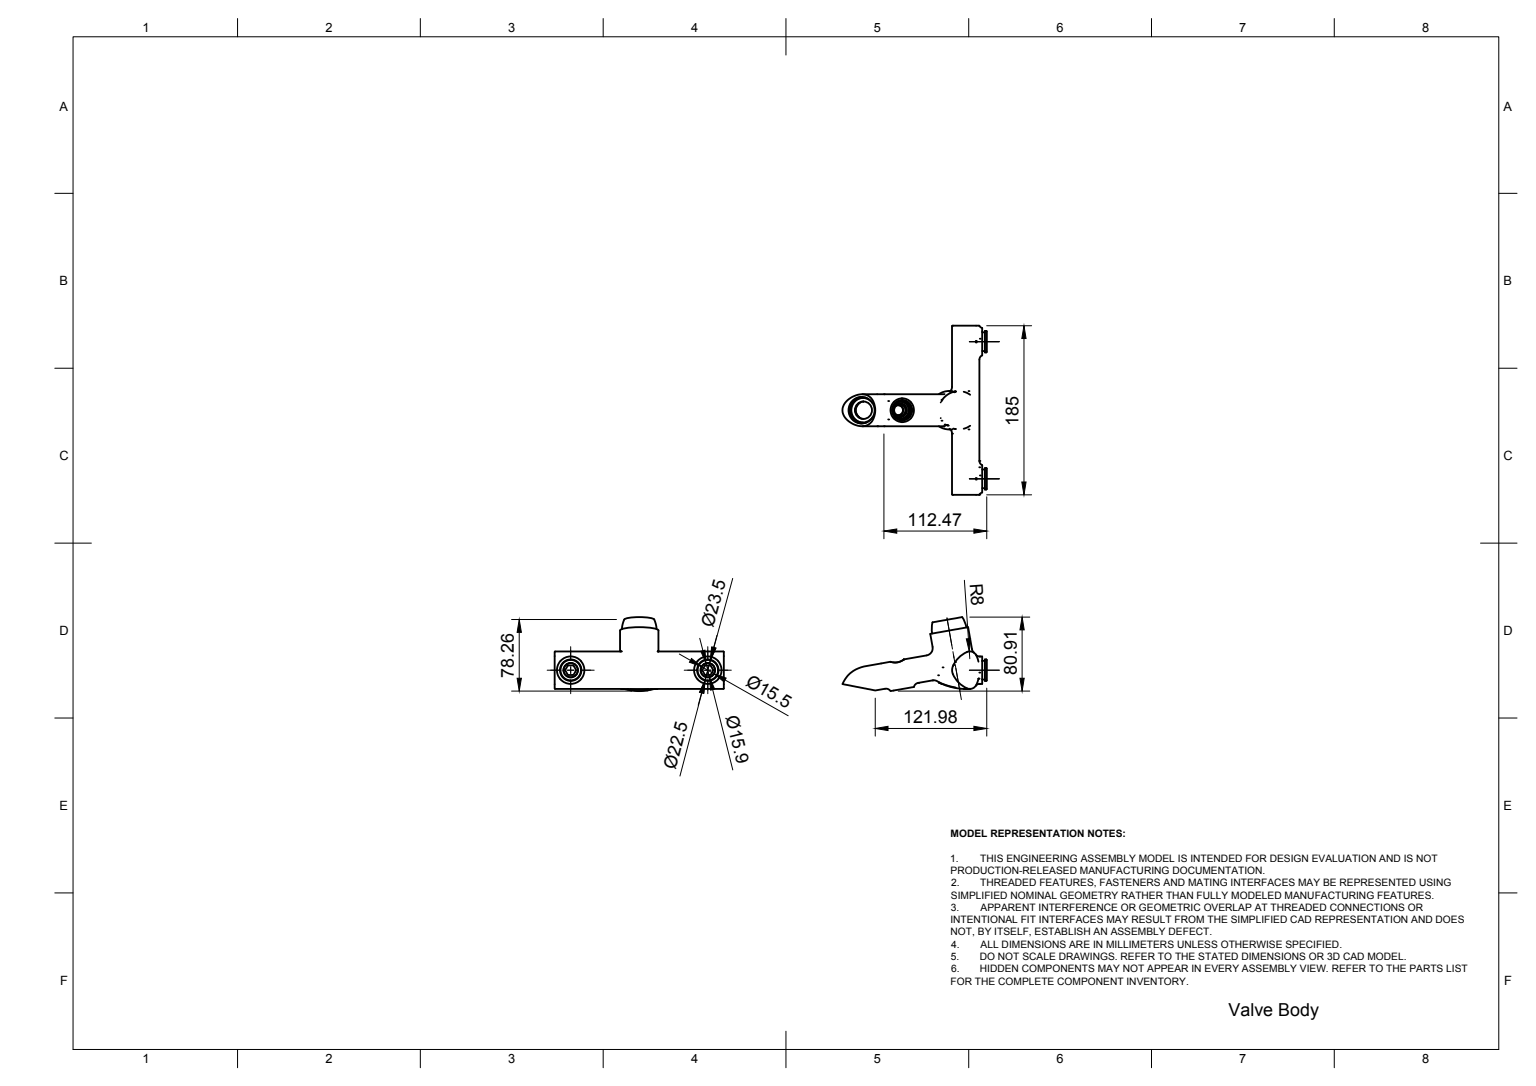
ISO-10303-21;
HEADER;
/* Generated by software containing ST-Developer
 * from STEP Tools, Inc. (www.steptools.com) 
 */

FILE_DESCRIPTION(
/* description */ ('STEP AP214'),
/* implementation_level */ '2;1');

FILE_NAME(
/* name */ 'Valve Body.step',
/* time_stamp */ '2026-10-05T23:18:41-07:00',
/* author */ (''),
/* organization */ (''),
/* preprocessor_version */ 'ST-DEVELOPER v20.2',
/* originating_system */ 'Autodesk Translation Framework v15.15.0.0',
/* authorisation */ '');

FILE_SCHEMA (('AUTOMOTIVE_DESIGN { 1 0 10303 214 3 1 1 }'));
ENDSEC;

DATA;
#10=MECHANICAL_DESIGN_GEOMETRIC_PRESENTATION_REPRESENTATION('',(#100),#221662);
#74=SHAPE_REPRESENTATION_RELATIONSHIP('SRR','None',#221709,#87);
#87=ADVANCED_BREP_SHAPE_REPRESENTATION('',(#79336),#221649);
#100=STYLED_ITEM('',(#221783),#79336);
#113=B_SPLINE_SURFACE_WITH_KNOTS('',3,3,((#122040,#122041,#122042,#122043,
#122044,#122045,#122046,#122047,#122048,#122049,#122050),(#122051,#122052,
#122053,#122054,#122055,#122056,#122057,#122058,#122059,#122060,#122061),
(#122062,#122063,#122064,#122065,#122066,#122067,#122068,#122069,#122070,
#122071,#122072),(#122073,#122074,#122075,#122076,#122077,#122078,#122079,
#122080,#122081,#122082,#122083)),.UNSPECIFIED.,.F.,.F.,.F.,(4,4),(4,1,
1,1,1,1,1,1,4),(0.,1.),(0.,0.125,0.249999999999986,0.374999999999913,0.499999999999809,
0.625000000000008,0.749999999999904,0.8749999999998,1.),.UNSPECIFIED.);
#114=B_SPLINE_SURFACE_WITH_KNOTS('',3,3,((#122246,#122247,#122248,#122249,
#122250,#122251,#122252,#122253,#122254,#122255,#122256),(#122257,#122258,
#122259,#122260,#122261,#122262,#122263,#122264,#122265,#122266,#122267),
(#122268,#122269,#122270,#122271,#122272,#122273,#122274,#122275,#122276,
#122277,#122278),(#122279,#122280,#122281,#122282,#122283,#122284,#122285,
#122286,#122287,#122288,#122289),(#122290,#122291,#122292,#122293,#122294,
#122295,#122296,#122297,#122298,#122299,#122300),(#122301,#122302,#122303,
#122304,#122305,#122306,#122307,#122308,#122309,#122310,#122311),(#122312,
#122313,#122314,#122315,#122316,#122317,#122318,#122319,#122320,#122321,
#122322),(#122323,#122324,#122325,#122326,#122327,#122328,#122329,#122330,
#122331,#122332,#122333),(#122334,#122335,#122336,#122337,#122338,#122339,
#122340,#122341,#122342,#122343,#122344),(#122345,#122346,#122347,#122348,
#122349,#122350,#122351,#122352,#122353,#122354,#122355)),.UNSPECIFIED.,
 .F.,.F.,.F.,(4,3,3,4),(4,1,1,1,1,1,1,1,4),(-0.01,0.,0.978175299313866,
1.),(0.,0.125000000000015,0.25000000000002,0.374999999999975,0.500000000000081,
0.625000000000188,0.750000000000041,0.875000000000148,1.),.UNSPECIFIED.);
#115=B_SPLINE_SURFACE_WITH_KNOTS('',3,3,((#122432,#122433,#122434,#122435,
#122436,#122437,#122438,#122439,#122440,#122441,#122442,#122443,#122444,
#122445,#122446,#122447,#122448,#122449,#122450),(#122451,#122452,#122453,
#122454,#122455,#122456,#122457,#122458,#122459,#122460,#122461,#122462,
#122463,#122464,#122465,#122466,#122467,#122468,#122469),(#122470,#122471,
#122472,#122473,#122474,#122475,#122476,#122477,#122478,#122479,#122480,
#122481,#122482,#122483,#122484,#122485,#122486,#122487,#122488),(#122489,
#122490,#122491,#122492,#122493,#122494,#122495,#122496,#122497,#122498,
#122499,#122500,#122501,#122502,#122503,#122504,#122505,#122506,#122507)),
 .UNSPECIFIED.,.F.,.F.,.F.,(4,4),(4,1,1,1,1,1,1,1,1,1,1,1,1,1,1,1,4),(0.,
1.),(0.,0.0625000000000019,0.12499999999999,0.187499999999977,0.249999999999904,
0.312500000000014,0.37499999999992,0.43750000000003,0.499999999999936,0.562500000000046,
0.624999999999952,0.687499999999859,0.749999999999968,0.812499999999875,
0.874999999999984,0.937499999999891,1.),.UNSPECIFIED.);
#116=B_SPLINE_SURFACE_WITH_KNOTS('',3,3,((#122509,#122510,#122511,#122512,
#122513,#122514,#122515,#122516,#122517,#122518,#122519,#122520,#122521,
#122522,#122523,#122524,#122525,#122526,#122527,#122528,#122529,#122530,
#122531,#122532,#122533,#122534,#122535,#122536,#122537,#122538,#122539,
#122540,#122541,#122542,#122543),(#122544,#122545,#122546,#122547,#122548,
#122549,#122550,#122551,#122552,#122553,#122554,#122555,#122556,#122557,
#122558,#122559,#122560,#122561,#122562,#122563,#122564,#122565,#122566,
#122567,#122568,#122569,#122570,#122571,#122572,#122573,#122574,#122575,
#122576,#122577,#122578),(#122579,#122580,#122581,#122582,#122583,#122584,
#122585,#122586,#122587,#122588,#122589,#122590,#122591,#122592,#122593,
#122594,#122595,#122596,#122597,#122598,#122599,#122600,#122601,#122602,
#122603,#122604,#122605,#122606,#122607,#122608,#122609,#122610,#122611,
#122612,#122613),(#122614,#122615,#122616,#122617,#122618,#122619,#122620,
#122621,#122622,#122623,#122624,#122625,#122626,#122627,#122628,#122629,
#122630,#122631,#122632,#122633,#122634,#122635,#122636,#122637,#122638,
#122639,#122640,#122641,#122642,#122643,#122644,#122645,#122646,#122647,
#122648)),.UNSPECIFIED.,.F.,.F.,.F.,(4,4),(4,1,1,1,1,1,1,1,1,1,1,1,1,1,
1,1,1,1,1,1,1,1,1,1,1,1,1,1,1,1,1,1,4),(0.,1.),(0.,0.031249999999986,0.0625000000000033,
0.0937499999999268,0.124999999999954,0.156249999999982,0.187499999999906,
0.218749999999933,0.249999999999961,0.281249999999885,0.312499999999912,
0.343749999999836,0.374999999999863,0.406249999999891,0.437499999999815,
0.468749999999842,0.49999999999987,0.531249999999794,0.562499999999821,
0.593749999999849,0.624999999999772,0.6562499999998,0.687499999999724,0.718749999999751,
0.749999999999779,0.781249999999703,0.81249999999973,0.843749999999758,
0.874999999999681,0.906249999999709,0.937499999999633,0.96874999999966,
1.),.UNSPECIFIED.);
#117=B_SPLINE_SURFACE_WITH_KNOTS('',3,3,((#122930,#122931,#122932,#122933,
#122934,#122935,#122936,#122937,#122938,#122939,#122940,#122941,#122942,
#122943,#122944,#122945,#122946,#122947,#122948,#122949,#122950,#122951,
#122952,#122953,#122954,#122955,#122956,#122957,#122958,#122959,#122960,
#122961,#122962,#122963,#122964),(#122965,#122966,#122967,#122968,#122969,
#122970,#122971,#122972,#122973,#122974,#122975,#122976,#122977,#122978,
#122979,#122980,#122981,#122982,#122983,#122984,#122985,#122986,#122987,
#122988,#122989,#122990,#122991,#122992,#122993,#122994,#122995,#122996,
#122997,#122998,#122999),(#123000,#123001,#123002,#123003,#123004,#123005,
#123006,#123007,#123008,#123009,#123010,#123011,#123012,#123013,#123014,
#123015,#123016,#123017,#123018,#123019,#123020,#123021,#123022,#123023,
#123024,#123025,#123026,#123027,#123028,#123029,#123030,#123031,#123032,
#123033,#123034),(#123035,#123036,#123037,#123038,#123039,#123040,#123041,
#123042,#123043,#123044,#123045,#123046,#123047,#123048,#123049,#123050,
#123051,#123052,#123053,#123054,#123055,#123056,#123057,#123058,#123059,
#123060,#123061,#123062,#123063,#123064,#123065,#123066,#123067,#123068,
#123069)),.UNSPECIFIED.,.F.,.F.,.F.,(4,4),(4,1,1,1,1,1,1,1,1,1,1,1,1,1,
1,1,1,1,1,1,1,1,1,1,1,1,1,1,1,1,1,1,4),(0.,1.),(0.,0.0312499999999875,0.0624999999999539,
0.0937500000000046,0.12499999999995,0.15625,0.187499999999946,0.218749999999891,
0.249999999999942,0.281249999999887,0.312499999999938,0.343749999999883,
0.374999999999934,0.40624999999988,0.43749999999993,0.468749999999876,0.499999999999821,
0.531249999999872,0.562499999999817,0.593749999999868,0.624999999999813,
0.656249999999864,0.687499999999809,0.71874999999986,0.749999999999805,
0.781249999999751,0.812499999999801,0.843749999999747,0.874999999999797,
0.906249999999743,0.937499999999793,0.968749999999739,1.),.UNSPECIFIED.);
#118=B_SPLINE_SURFACE_WITH_KNOTS('',3,3,((#123453,#123454,#123455,#123456,
#123457,#123458,#123459,#123460,#123461,#123462,#123463,#123464,#123465,
#123466,#123467,#123468,#123469,#123470,#123471,#123472,#123473,#123474,
#123475,#123476,#123477,#123478,#123479,#123480,#123481,#123482,#123483,
#123484,#123485),(#123486,#123487,#123488,#123489,#123490,#123491,#123492,
#123493,#123494,#123495,#123496,#123497,#123498,#123499,#123500,#123501,
#123502,#123503,#123504,#123505,#123506,#123507,#123508,#123509,#123510,
#123511,#123512,#123513,#123514,#123515,#123516,#123517,#123518),(#123519,
#123520,#123521,#123522,#123523,#123524,#123525,#123526,#123527,#123528,
#123529,#123530,#123531,#123532,#123533,#123534,#123535,#123536,#123537,
#123538,#123539,#123540,#123541,#123542,#123543,#123544,#123545,#123546,
#123547,#123548,#123549,#123550,#123551),(#123552,#123553,#123554,#123555,
#123556,#123557,#123558,#123559,#123560,#123561,#123562,#123563,#123564,
#123565,#123566,#123567,#123568,#123569,#123570,#123571,#123572,#123573,
#123574,#123575,#123576,#123577,#123578,#123579,#123580,#123581,#123582,
#123583,#123584)),.UNSPECIFIED.,.F.,.F.,.F.,(4,4),(4,1,1,1,1,1,1,1,1,1,
1,1,1,1,1,1,1,1,1,1,1,1,1,1,1,1,1,1,1,1,4),(0.,1.),(0.,0.0624999999999647,
0.0937499999999471,0.125000000000042,0.156250000000025,0.187500000000007,
0.218749999999989,0.249999999999972,0.281249999999954,0.312499999999937,
0.343750000000032,0.375000000000014,0.40625,0.437499999999979,0.468749999999961,
0.499999999999944,0.531250000000039,0.562500000000021,0.59375,0.624999999999986,
0.656249999999968,0.687499999999951,0.718749999999933,0.750000000000028,
0.781250000000011,0.8125,0.843749999999975,0.874999999999958,0.90624999999994,
0.937499999999923,1.),.UNSPECIFIED.);
#119=B_SPLINE_SURFACE_WITH_KNOTS('',3,3,((#128648,#128649,#128650,#128651,
#128652,#128653,#128654,#128655,#128656,#128657,#128658),(#128659,#128660,
#128661,#128662,#128663,#128664,#128665,#128666,#128667,#128668,#128669),
(#128670,#128671,#128672,#128673,#128674,#128675,#128676,#128677,#128678,
#128679,#128680),(#128681,#128682,#128683,#128684,#128685,#128686,#128687,
#128688,#128689,#128690,#128691)),.UNSPECIFIED.,.F.,.F.,.F.,(4,4),(4,1,
1,1,1,1,1,1,4),(0.,1.),(0.,0.125,0.249999999999986,0.374999999999913,0.499999999999809,
0.625000000000008,0.749999999999904,0.8749999999998,1.),.UNSPECIFIED.);
#120=B_SPLINE_SURFACE_WITH_KNOTS('',3,3,((#128722,#128723,#128724,#128725,
#128726,#128727,#128728,#128729,#128730,#128731,#128732,#128733,#128734,
#128735,#128736,#128737,#128738,#128739,#128740),(#128741,#128742,#128743,
#128744,#128745,#128746,#128747,#128748,#128749,#128750,#128751,#128752,
#128753,#128754,#128755,#128756,#128757,#128758,#128759),(#128760,#128761,
#128762,#128763,#128764,#128765,#128766,#128767,#128768,#128769,#128770,
#128771,#128772,#128773,#128774,#128775,#128776,#128777,#128778),(#128779,
#128780,#128781,#128782,#128783,#128784,#128785,#128786,#128787,#128788,
#128789,#128790,#128791,#128792,#128793,#128794,#128795,#128796,#128797)),
 .UNSPECIFIED.,.F.,.F.,.F.,(4,4),(4,1,1,1,1,1,1,1,1,1,1,1,1,1,1,1,4),(0.,
1.),(0.,0.0625000000000019,0.12499999999999,0.187499999999977,0.249999999999904,
0.312500000000014,0.37499999999992,0.43750000000003,0.499999999999936,0.562500000000046,
0.624999999999952,0.687499999999859,0.749999999999968,0.812499999999875,
0.874999999999984,0.937499999999891,1.),.UNSPECIFIED.);
#121=B_SPLINE_SURFACE_WITH_KNOTS('',3,3,((#128874,#128875,#128876,#128877,
#128878,#128879,#128880,#128881,#128882,#128883,#128884),(#128885,#128886,
#128887,#128888,#128889,#128890,#128891,#128892,#128893,#128894,#128895),
(#128896,#128897,#128898,#128899,#128900,#128901,#128902,#128903,#128904,
#128905,#128906),(#128907,#128908,#128909,#128910,#128911,#128912,#128913,
#128914,#128915,#128916,#128917),(#128918,#128919,#128920,#128921,#128922,
#128923,#128924,#128925,#128926,#128927,#128928),(#128929,#128930,#128931,
#128932,#128933,#128934,#128935,#128936,#128937,#128938,#128939),(#128940,
#128941,#128942,#128943,#128944,#128945,#128946,#128947,#128948,#128949,
#128950)),.UNSPECIFIED.,.F.,.F.,.F.,(4,3,4),(4,1,1,1,1,1,1,1,4),(0.,0.978284469703565,
1.),(0.,0.125000000000015,0.25000000000002,0.374999999999975,0.500000000000081,
0.625000000000188,0.750000000000041,0.875000000000148,1.),.UNSPECIFIED.);
#122=B_SPLINE_SURFACE_WITH_KNOTS('',3,3,((#128952,#128953,#128954,#128955,
#128956,#128957,#128958,#128959,#128960,#128961,#128962,#128963,#128964,
#128965,#128966,#128967,#128968,#128969,#128970,#128971,#128972,#128973,
#128974,#128975,#128976,#128977,#128978,#128979,#128980,#128981,#128982,
#128983,#128984,#128985,#128986),(#128987,#128988,#128989,#128990,#128991,
#128992,#128993,#128994,#128995,#128996,#128997,#128998,#128999,#129000,
#129001,#129002,#129003,#129004,#129005,#129006,#129007,#129008,#129009,
#129010,#129011,#129012,#129013,#129014,#129015,#129016,#129017,#129018,
#129019,#129020,#129021),(#129022,#129023,#129024,#129025,#129026,#129027,
#129028,#129029,#129030,#129031,#129032,#129033,#129034,#129035,#129036,
#129037,#129038,#129039,#129040,#129041,#129042,#129043,#129044,#129045,
#129046,#129047,#129048,#129049,#129050,#129051,#129052,#129053,#129054,
#129055,#129056),(#129057,#129058,#129059,#129060,#129061,#129062,#129063,
#129064,#129065,#129066,#129067,#129068,#129069,#129070,#129071,#129072,
#129073,#129074,#129075,#129076,#129077,#129078,#129079,#129080,#129081,
#129082,#129083,#129084,#129085,#129086,#129087,#129088,#129089,#129090,
#129091)),.UNSPECIFIED.,.F.,.F.,.F.,(4,4),(4,1,1,1,1,1,1,1,1,1,1,1,1,1,
1,1,1,1,1,1,1,1,1,1,1,1,1,1,1,1,1,1,4),(0.,1.),(0.,0.031249999999986,0.0625000000000033,
0.0937499999999268,0.124999999999954,0.156249999999982,0.187499999999906,
0.218749999999933,0.249999999999961,0.281249999999885,0.312499999999912,
0.343749999999836,0.374999999999863,0.406249999999891,0.437499999999815,
0.468749999999842,0.49999999999987,0.531249999999794,0.562499999999821,
0.593749999999849,0.624999999999772,0.6562499999998,0.687499999999724,0.718749999999751,
0.749999999999779,0.781249999999703,0.81249999999973,0.843749999999758,
0.874999999999681,0.906249999999709,0.937499999999633,0.96874999999966,
1.),.UNSPECIFIED.);
#123=B_SPLINE_SURFACE_WITH_KNOTS('',3,3,((#129371,#129372,#129373,#129374,
#129375,#129376,#129377,#129378,#129379,#129380,#129381,#129382,#129383,
#129384,#129385,#129386,#129387,#129388,#129389,#129390,#129391,#129392,
#129393,#129394,#129395,#129396,#129397,#129398,#129399,#129400,#129401,
#129402,#129403),(#129404,#129405,#129406,#129407,#129408,#129409,#129410,
#129411,#129412,#129413,#129414,#129415,#129416,#129417,#129418,#129419,
#129420,#129421,#129422,#129423,#129424,#129425,#129426,#129427,#129428,
#129429,#129430,#129431,#129432,#129433,#129434,#129435,#129436),(#129437,
#129438,#129439,#129440,#129441,#129442,#129443,#129444,#129445,#129446,
#129447,#129448,#129449,#129450,#129451,#129452,#129453,#129454,#129455,
#129456,#129457,#129458,#129459,#129460,#129461,#129462,#129463,#129464,
#129465,#129466,#129467,#129468,#129469),(#129470,#129471,#129472,#129473,
#129474,#129475,#129476,#129477,#129478,#129479,#129480,#129481,#129482,
#129483,#129484,#129485,#129486,#129487,#129488,#129489,#129490,#129491,
#129492,#129493,#129494,#129495,#129496,#129497,#129498,#129499,#129500,
#129501,#129502)),.UNSPECIFIED.,.F.,.F.,.F.,(4,4),(4,1,1,1,1,1,1,1,1,1,
1,1,1,1,1,1,1,1,1,1,1,1,1,1,1,1,1,1,1,1,4),(0.,1.),(0.,0.0624999999999647,
0.0937499999999471,0.125000000000042,0.156250000000025,0.187500000000007,
0.218749999999989,0.249999999999972,0.281249999999954,0.312499999999937,
0.343750000000032,0.375000000000014,0.40625,0.437499999999979,0.468749999999961,
0.499999999999944,0.531250000000039,0.562500000000021,0.59375,0.624999999999986,
0.656249999999968,0.687499999999951,0.718749999999933,0.750000000000028,
0.781250000000011,0.8125,0.843749999999975,0.874999999999958,0.90624999999994,
0.937499999999923,1.),.UNSPECIFIED.);
#124=B_SPLINE_SURFACE_WITH_KNOTS('',3,3,((#129824,#129825,#129826,#129827,
#129828,#129829,#129830,#129831,#129832,#129833,#129834,#129835,#129836,
#129837,#129838,#129839,#129840,#129841,#129842,#129843,#129844,#129845,
#129846,#129847,#129848,#129849,#129850,#129851,#129852,#129853,#129854,
#129855,#129856,#129857,#129858),(#129859,#129860,#129861,#129862,#129863,
#129864,#129865,#129866,#129867,#129868,#129869,#129870,#129871,#129872,
#129873,#129874,#129875,#129876,#129877,#129878,#129879,#129880,#129881,
#129882,#129883,#129884,#129885,#129886,#129887,#129888,#129889,#129890,
#129891,#129892,#129893),(#129894,#129895,#129896,#129897,#129898,#129899,
#129900,#129901,#129902,#129903,#129904,#129905,#129906,#129907,#129908,
#129909,#129910,#129911,#129912,#129913,#129914,#129915,#129916,#129917,
#129918,#129919,#129920,#129921,#129922,#129923,#129924,#129925,#129926,
#129927,#129928),(#129929,#129930,#129931,#129932,#129933,#129934,#129935,
#129936,#129937,#129938,#129939,#129940,#129941,#129942,#129943,#129944,
#129945,#129946,#129947,#129948,#129949,#129950,#129951,#129952,#129953,
#129954,#129955,#129956,#129957,#129958,#129959,#129960,#129961,#129962,
#129963)),.UNSPECIFIED.,.F.,.F.,.F.,(4,4),(4,1,1,1,1,1,1,1,1,1,1,1,1,1,
1,1,1,1,1,1,1,1,1,1,1,1,1,1,1,1,1,1,4),(0.,1.),(0.,0.0312499999999977,0.0624999999999638,
0.0937500000000142,0.124999999999959,0.15625000000001,0.187499999999955,
0.2187499999999,0.24999999999995,0.281249999999895,0.312499999999945,0.34374999999989,
0.374999999999941,0.406249999999886,0.437499999999936,0.468749999999881,
0.499999999999826,0.531249999999877,0.562499999999822,0.593749999999872,
0.624999999999817,0.656249999999867,0.687499999999812,0.718749999999863,
0.749999999999808,0.781249999999753,0.812499999999803,0.843749999999749,
0.874999999999799,0.906249999999744,0.937499999999794,0.968749999999739,
1.),.UNSPECIFIED.);
#125=B_SPLINE_SURFACE_WITH_KNOTS('',1,3,((#129975,#129976,#129977,#129978,
#129979,#129980,#129981,#129982,#129983,#129984,#129985,#129986,#129987,
#129988,#129989,#129990,#129991,#129992,#129993,#129994,#129995,#129996,
#129997,#129998,#129999,#130000,#130001,#130002,#130003,#130004,#130005,
#130006,#130007,#130008,#130009,#130010,#130011,#130012,#130013,#130014,
#130015,#130016,#130017,#130018,#130019,#130020,#130021,#130022,#130023,
#130024,#130025,#130026,#130027,#130028,#130029,#130030,#130031,#130032,
#130033,#130034,#130035,#130036,#130037,#130038,#130039,#130040,#130041,
#130042,#130043,#130044,#130045,#130046,#130047,#130048,#130049,#130050,
#130051,#130052,#130053,#130054,#130055,#130056,#130057,#130058,#130059),
(#130060,#130061,#130062,#130063,#130064,#130065,#130066,#130067,#130068,
#130069,#130070,#130071,#130072,#130073,#130074,#130075,#130076,#130077,
#130078,#130079,#130080,#130081,#130082,#130083,#130084,#130085,#130086,
#130087,#130088,#130089,#130090,#130091,#130092,#130093,#130094,#130095,
#130096,#130097,#130098,#130099,#130100,#130101,#130102,#130103,#130104,
#130105,#130106,#130107,#130108,#130109,#130110,#130111,#130112,#130113,
#130114,#130115,#130116,#130117,#130118,#130119,#130120,#130121,#130122,
#130123,#130124,#130125,#130126,#130127,#130128,#130129,#130130,#130131,
#130132,#130133,#130134,#130135,#130136,#130137,#130138,#130139,#130140,
#130141,#130142,#130143,#130144)),.UNSPECIFIED.,.F.,.F.,.F.,(2,2),(4,1,
1,1,1,1,1,1,1,1,1,1,1,1,1,1,1,1,1,1,1,1,1,1,1,1,1,1,1,1,1,1,1,1,1,1,1,1,
1,1,1,1,1,1,1,1,1,1,1,1,1,1,1,1,1,1,1,1,1,1,1,1,1,1,1,1,1,1,1,1,1,1,1,1,
1,1,1,1,1,1,1,1,4),(0.,1.),(0.,0.0122851866641497,0.0245703733282994,0.0368555599924492,
0.0491407466565989,0.0614259333207486,0.0737111199848983,0.085996306649048,
0.0982814933131977,0.110566679977347,0.122851866641497,0.135137053305647,
0.147422239969797,0.159707426633946,0.171992613298096,0.184277799962246,
0.196562986626395,0.208848173290545,0.221133359954695,0.233418546618845,
0.245703733282994,0.257988919947144,0.270274106611294,0.282559293275443,
0.294844479939593,0.307129666603743,0.319414853267893,0.331700039932042,
0.343985226596192,0.356270413260342,0.368555599924492,0.380840786588641,
0.393125973252791,0.405411159916941,0.41769634658109,0.42998153324524,0.44226671990939,
0.45455190657354,0.466837093237689,0.479122279901839,0.491407466565989,
0.503692653230138,0.515977839894288,0.528263026558438,0.540548213222588,
0.552833399886737,0.565118586550887,0.577403773215037,0.589688959879186,
0.601974146543336,0.614259333207486,0.626544519871636,0.638829706535785,
0.651114893199935,0.663400079864085,0.675685266528234,0.687970453192384,
0.700255639856534,0.712540826520684,0.724826013184833,0.737111199848983,
0.749396386513133,0.761681573177282,0.773966759841432,0.786251946505582,
0.798537133169732,0.810822319833881,0.823107506498031,0.835392693162181,
0.847677879826331,0.85996306649048,0.87224825315463,0.88453343981878,0.896818626482929,
0.909103813147079,0.921388999811229,0.933674186475379,0.945959373139528,
0.958244559803678,0.970529746467828,0.982814933131977,0.995100119796127,
1.),.UNSPECIFIED.);
#126=B_SPLINE_SURFACE_WITH_KNOTS('',1,3,((#130146,#130147,#130148,#130149,
#130150,#130151,#130152,#130153,#130154,#130155,#130156,#130157,#130158,
#130159,#130160,#130161,#130162,#130163,#130164,#130165,#130166,#130167,
#130168,#130169,#130170,#130171,#130172,#130173,#130174,#130175,#130176,
#130177,#130178,#130179,#130180,#130181,#130182,#130183,#130184,#130185,
#130186,#130187,#130188,#130189,#130190,#130191,#130192,#130193,#130194,
#130195,#130196,#130197,#130198,#130199,#130200,#130201,#130202,#130203,
#130204,#130205,#130206,#130207,#130208,#130209,#130210,#130211,#130212,
#130213,#130214,#130215,#130216,#130217,#130218,#130219,#130220,#130221,
#130222,#130223,#130224,#130225,#130226,#130227,#130228,#130229,#130230),
(#130231,#130232,#130233,#130234,#130235,#130236,#130237,#130238,#130239,
#130240,#130241,#130242,#130243,#130244,#130245,#130246,#130247,#130248,
#130249,#130250,#130251,#130252,#130253,#130254,#130255,#130256,#130257,
#130258,#130259,#130260,#130261,#130262,#130263,#130264,#130265,#130266,
#130267,#130268,#130269,#130270,#130271,#130272,#130273,#130274,#130275,
#130276,#130277,#130278,#130279,#130280,#130281,#130282,#130283,#130284,
#130285,#130286,#130287,#130288,#130289,#130290,#130291,#130292,#130293,
#130294,#130295,#130296,#130297,#130298,#130299,#130300,#130301,#130302,
#130303,#130304,#130305,#130306,#130307,#130308,#130309,#130310,#130311,
#130312,#130313,#130314,#130315)),.UNSPECIFIED.,.F.,.F.,.F.,(2,2),(4,1,
1,1,1,1,1,1,1,1,1,1,1,1,1,1,1,1,1,1,1,1,1,1,1,1,1,1,1,1,1,1,1,1,1,1,1,1,
1,1,1,1,1,1,1,1,1,1,1,1,1,1,1,1,1,1,1,1,1,1,1,1,1,1,1,1,1,1,1,1,1,1,1,1,
1,1,1,1,1,1,1,1,4),(0.,1.),(0.,0.0122851866641497,0.0245703733282994,0.0368555599924492,
0.0491407466565989,0.0614259333207486,0.0737111199848983,0.085996306649048,
0.0982814933131977,0.110566679977347,0.122851866641497,0.135137053305647,
0.147422239969797,0.159707426633946,0.171992613298096,0.184277799962246,
0.196562986626395,0.208848173290545,0.221133359954695,0.233418546618845,
0.245703733282994,0.257988919947144,0.270274106611294,0.282559293275443,
0.294844479939593,0.307129666603743,0.319414853267893,0.331700039932042,
0.343985226596192,0.356270413260342,0.368555599924492,0.380840786588641,
0.393125973252791,0.405411159916941,0.41769634658109,0.42998153324524,0.44226671990939,
0.45455190657354,0.466837093237689,0.479122279901839,0.491407466565989,
0.503692653230138,0.515977839894288,0.528263026558438,0.540548213222588,
0.552833399886737,0.565118586550887,0.577403773215037,0.589688959879186,
0.601974146543336,0.614259333207486,0.626544519871636,0.638829706535785,
0.651114893199935,0.663400079864085,0.675685266528234,0.687970453192384,
0.700255639856534,0.712540826520684,0.724826013184833,0.737111199848983,
0.749396386513133,0.761681573177282,0.773966759841432,0.786251946505582,
0.798537133169732,0.810822319833881,0.823107506498031,0.835392693162181,
0.847677879826331,0.85996306649048,0.87224825315463,0.88453343981878,0.896818626482929,
0.909103813147079,0.921388999811229,0.933674186475379,0.945959373139528,
0.958244559803678,0.970529746467828,0.982814933131977,0.995100119796127,
1.),.UNSPECIFIED.);
#127=B_SPLINE_SURFACE_WITH_KNOTS('',3,3,((#132433,#132434,#132435,#132436,
#132437,#132438,#132439,#132440,#132441),(#132442,#132443,#132444,#132445,
#132446,#132447,#132448,#132449,#132450),(#132451,#132452,#132453,#132454,
#132455,#132456,#132457,#132458,#132459),(#132460,#132461,#132462,#132463,
#132464,#132465,#132466,#132467,#132468),(#132469,#132470,#132471,#132472,
#132473,#132474,#132475,#132476,#132477),(#132478,#132479,#132480,#132481,
#132482,#132483,#132484,#132485,#132486)),.UNSPECIFIED.,.F.,.F.,.F.,(4,
2,4),(4,2,3,4),(0.,0.5,1.),(-0.00320679271163163,1.21084430265805,2.42168860531611,
6.01951071788134),.UNSPECIFIED.);
#128=B_SPLINE_SURFACE_WITH_KNOTS('',3,3,((#136533,#136534,#136535,#136536,
#136537,#136538,#136539,#136540,#136541,#136542,#136543,#136544,#136545,
#136546,#136547,#136548,#136549,#136550,#136551,#136552,#136553,#136554),
(#136555,#136556,#136557,#136558,#136559,#136560,#136561,#136562,#136563,
#136564,#136565,#136566,#136567,#136568,#136569,#136570,#136571,#136572,
#136573,#136574,#136575,#136576),(#136577,#136578,#136579,#136580,#136581,
#136582,#136583,#136584,#136585,#136586,#136587,#136588,#136589,#136590,
#136591,#136592,#136593,#136594,#136595,#136596,#136597,#136598),(#136599,
#136600,#136601,#136602,#136603,#136604,#136605,#136606,#136607,#136608,
#136609,#136610,#136611,#136612,#136613,#136614,#136615,#136616,#136617,
#136618,#136619,#136620),(#136621,#136622,#136623,#136624,#136625,#136626,
#136627,#136628,#136629,#136630,#136631,#136632,#136633,#136634,#136635,
#136636,#136637,#136638,#136639,#136640,#136641,#136642),(#136643,#136644,
#136645,#136646,#136647,#136648,#136649,#136650,#136651,#136652,#136653,
#136654,#136655,#136656,#136657,#136658,#136659,#136660,#136661,#136662,
#136663,#136664),(#136665,#136666,#136667,#136668,#136669,#136670,#136671,
#136672,#136673,#136674,#136675,#136676,#136677,#136678,#136679,#136680,
#136681,#136682,#136683,#136684,#136685,#136686),(#136687,#136688,#136689,
#136690,#136691,#136692,#136693,#136694,#136695,#136696,#136697,#136698,
#136699,#136700,#136701,#136702,#136703,#136704,#136705,#136706,#136707,
#136708),(#136709,#136710,#136711,#136712,#136713,#136714,#136715,#136716,
#136717,#136718,#136719,#136720,#136721,#136722,#136723,#136724,#136725,
#136726,#136727,#136728,#136729,#136730),(#136731,#136732,#136733,#136734,
#136735,#136736,#136737,#136738,#136739,#136740,#136741,#136742,#136743,
#136744,#136745,#136746,#136747,#136748,#136749,#136750,#136751,#136752),
(#136753,#136754,#136755,#136756,#136757,#136758,#136759,#136760,#136761,
#136762,#136763,#136764,#136765,#136766,#136767,#136768,#136769,#136770,
#136771,#136772,#136773,#136774),(#136775,#136776,#136777,#136778,#136779,
#136780,#136781,#136782,#136783,#136784,#136785,#136786,#136787,#136788,
#136789,#136790,#136791,#136792,#136793,#136794,#136795,#136796),(#136797,
#136798,#136799,#136800,#136801,#136802,#136803,#136804,#136805,#136806,
#136807,#136808,#136809,#136810,#136811,#136812,#136813,#136814,#136815,
#136816,#136817,#136818)),.UNSPECIFIED.,.F.,.F.,.F.,(4,1,1,1,1,1,1,1,1,
1,4),(4,1,1,1,1,1,1,1,1,1,1,1,1,1,1,1,1,1,1,4),(0.,0.0709766854731603,0.132271619181511,
0.254861486598212,0.377451354014914,0.500041221431615,0.622631088848316,
0.745220956265018,0.867810823681719,0.92910575739007,1.),(0.,0.13235257180777,
0.254901630119635,0.316176159275667,0.346813423853634,0.354472739998076,
0.358302398070297,0.362132056142617,0.369791372287059,0.3774506884316,0.438725217587533,
0.499999746743466,0.622548805055332,0.683823334211265,0.745097863367198,
0.80637239252323,0.867646921679163,0.928921450835096,0.990195979991028,
1.),.UNSPECIFIED.);
#129=B_SPLINE_SURFACE_WITH_KNOTS('',3,3,((#136902,#136903,#136904,#136905,
#136906,#136907,#136908,#136909,#136910,#136911,#136912,#136913,#136914,
#136915,#136916,#136917,#136918,#136919,#136920,#136921,#136922,#136923),
(#136924,#136925,#136926,#136927,#136928,#136929,#136930,#136931,#136932,
#136933,#136934,#136935,#136936,#136937,#136938,#136939,#136940,#136941,
#136942,#136943,#136944,#136945),(#136946,#136947,#136948,#136949,#136950,
#136951,#136952,#136953,#136954,#136955,#136956,#136957,#136958,#136959,
#136960,#136961,#136962,#136963,#136964,#136965,#136966,#136967),(#136968,
#136969,#136970,#136971,#136972,#136973,#136974,#136975,#136976,#136977,
#136978,#136979,#136980,#136981,#136982,#136983,#136984,#136985,#136986,
#136987,#136988,#136989),(#136990,#136991,#136992,#136993,#136994,#136995,
#136996,#136997,#136998,#136999,#137000,#137001,#137002,#137003,#137004,
#137005,#137006,#137007,#137008,#137009,#137010,#137011),(#137012,#137013,
#137014,#137015,#137016,#137017,#137018,#137019,#137020,#137021,#137022,
#137023,#137024,#137025,#137026,#137027,#137028,#137029,#137030,#137031,
#137032,#137033),(#137034,#137035,#137036,#137037,#137038,#137039,#137040,
#137041,#137042,#137043,#137044,#137045,#137046,#137047,#137048,#137049,
#137050,#137051,#137052,#137053,#137054,#137055),(#137056,#137057,#137058,
#137059,#137060,#137061,#137062,#137063,#137064,#137065,#137066,#137067,
#137068,#137069,#137070,#137071,#137072,#137073,#137074,#137075,#137076,
#137077),(#137078,#137079,#137080,#137081,#137082,#137083,#137084,#137085,
#137086,#137087,#137088,#137089,#137090,#137091,#137092,#137093,#137094,
#137095,#137096,#137097,#137098,#137099),(#137100,#137101,#137102,#137103,
#137104,#137105,#137106,#137107,#137108,#137109,#137110,#137111,#137112,
#137113,#137114,#137115,#137116,#137117,#137118,#137119,#137120,#137121),
(#137122,#137123,#137124,#137125,#137126,#137127,#137128,#137129,#137130,
#137131,#137132,#137133,#137134,#137135,#137136,#137137,#137138,#137139,
#137140,#137141,#137142,#137143),(#137144,#137145,#137146,#137147,#137148,
#137149,#137150,#137151,#137152,#137153,#137154,#137155,#137156,#137157,
#137158,#137159,#137160,#137161,#137162,#137163,#137164,#137165),(#137166,
#137167,#137168,#137169,#137170,#137171,#137172,#137173,#137174,#137175,
#137176,#137177,#137178,#137179,#137180,#137181,#137182,#137183,#137184,
#137185,#137186,#137187)),.UNSPECIFIED.,.F.,.F.,.F.,(4,1,1,1,1,1,1,1,1,
1,4),(4,1,1,1,1,1,1,1,1,1,1,1,1,1,1,1,1,1,1,4),(0.,0.0709778601999125,0.132273968651597,
0.254866185554966,0.377458402458335,0.500050619361704,0.622642836265073,
0.745235053168442,0.86782727007181,0.929123378523495,1.),(0.,0.132351844415717,
0.254900175335541,0.316174340795552,0.346811423525508,0.354470694207947,
0.358300329549167,0.362129964890486,0.369789235572925,0.377448506255464,
0.438722671715376,0.499996837175288,0.622545168095112,0.683819333555024,
0.745093499014936,0.806367664474947,0.867641829934859,0.928915995394771,
0.990190160854683,1.),.UNSPECIFIED.);
#130=B_SPLINE_SURFACE_WITH_KNOTS('',3,3,((#137610,#137611,#137612,#137613,
#137614,#137615,#137616,#137617,#137618,#137619,#137620,#137621,#137622,
#137623,#137624,#137625),(#137626,#137627,#137628,#137629,#137630,#137631,
#137632,#137633,#137634,#137635,#137636,#137637,#137638,#137639,#137640,
#137641),(#137642,#137643,#137644,#137645,#137646,#137647,#137648,#137649,
#137650,#137651,#137652,#137653,#137654,#137655,#137656,#137657),(#137658,
#137659,#137660,#137661,#137662,#137663,#137664,#137665,#137666,#137667,
#137668,#137669,#137670,#137671,#137672,#137673),(#137674,#137675,#137676,
#137677,#137678,#137679,#137680,#137681,#137682,#137683,#137684,#137685,
#137686,#137687,#137688,#137689),(#137690,#137691,#137692,#137693,#137694,
#137695,#137696,#137697,#137698,#137699,#137700,#137701,#137702,#137703,
#137704,#137705),(#137706,#137707,#137708,#137709,#137710,#137711,#137712,
#137713,#137714,#137715,#137716,#137717,#137718,#137719,#137720,#137721),
(#137722,#137723,#137724,#137725,#137726,#137727,#137728,#137729,#137730,
#137731,#137732,#137733,#137734,#137735,#137736,#137737),(#137738,#137739,
#137740,#137741,#137742,#137743,#137744,#137745,#137746,#137747,#137748,
#137749,#137750,#137751,#137752,#137753),(#137754,#137755,#137756,#137757,
#137758,#137759,#137760,#137761,#137762,#137763,#137764,#137765,#137766,
#137767,#137768,#137769),(#137770,#137771,#137772,#137773,#137774,#137775,
#137776,#137777,#137778,#137779,#137780,#137781,#137782,#137783,#137784,
#137785),(#137786,#137787,#137788,#137789,#137790,#137791,#137792,#137793,
#137794,#137795,#137796,#137797,#137798,#137799,#137800,#137801),(#137802,
#137803,#137804,#137805,#137806,#137807,#137808,#137809,#137810,#137811,
#137812,#137813,#137814,#137815,#137816,#137817),(#137818,#137819,#137820,
#137821,#137822,#137823,#137824,#137825,#137826,#137827,#137828,#137829,
#137830,#137831,#137832,#137833)),.UNSPECIFIED.,.F.,.F.,.F.,(4,1,1,1,1,
1,1,1,1,1,1,4),(4,1,1,1,1,1,1,1,1,1,1,1,1,4),(0.,0.134085205134682,0.255951223187441,
0.3778172412402,0.499683259292959,0.621549277345718,0.682482286372097,0.743415295398476,
0.804348304424856,0.865281313451235,0.926214322477615,1.),(0.,0.132446393239555,
0.193720576817934,0.254994760396314,0.316268943974693,0.377543127553072,
0.408180219342262,0.438817311131451,0.469454402920641,0.500091494709831,
0.56136567828821,0.622639861866589,0.745188229023347,1.),.UNSPECIFIED.);
#131=B_SPLINE_SURFACE_WITH_KNOTS('',3,3,((#138125,#138126,#138127,#138128,
#138129,#138130,#138131,#138132,#138133),(#138134,#138135,#138136,#138137,
#138138,#138139,#138140,#138141,#138142),(#138143,#138144,#138145,#138146,
#138147,#138148,#138149,#138150,#138151),(#138152,#138153,#138154,#138155,
#138156,#138157,#138158,#138159,#138160),(#138161,#138162,#138163,#138164,
#138165,#138166,#138167,#138168,#138169),(#138170,#138171,#138172,#138173,
#138174,#138175,#138176,#138177,#138178),(#138179,#138180,#138181,#138182,
#138183,#138184,#138185,#138186,#138187),(#138188,#138189,#138190,#138191,
#138192,#138193,#138194,#138195,#138196),(#138197,#138198,#138199,#138200,
#138201,#138202,#138203,#138204,#138205),(#138206,#138207,#138208,#138209,
#138210,#138211,#138212,#138213,#138214),(#138215,#138216,#138217,#138218,
#138219,#138220,#138221,#138222,#138223),(#138224,#138225,#138226,#138227,
#138228,#138229,#138230,#138231,#138232)),.UNSPECIFIED.,.F.,.F.,.F.,(4,
1,1,1,1,1,1,1,1,4),(4,1,1,1,1,1,4),(0.,0.133433046999215,0.194394733712586,
0.255356420425957,0.316318107139328,0.377279793852699,0.499203167279441,
0.621126540706183,0.743049914132925,1.),(0.,0.267979296737124,0.384002950769135,
0.500026604801238,0.616050258833249,0.73207391286526,1.),.UNSPECIFIED.);
#132=B_SPLINE_SURFACE_WITH_KNOTS('',3,3,((#138251,#138252,#138253,#138254,
#138255,#138256,#138257,#138258,#138259),(#138260,#138261,#138262,#138263,
#138264,#138265,#138266,#138267,#138268),(#138269,#138270,#138271,#138272,
#138273,#138274,#138275,#138276,#138277),(#138278,#138279,#138280,#138281,
#138282,#138283,#138284,#138285,#138286),(#138287,#138288,#138289,#138290,
#138291,#138292,#138293,#138294,#138295),(#138296,#138297,#138298,#138299,
#138300,#138301,#138302,#138303,#138304),(#138305,#138306,#138307,#138308,
#138309,#138310,#138311,#138312,#138313),(#138314,#138315,#138316,#138317,
#138318,#138319,#138320,#138321,#138322),(#138323,#138324,#138325,#138326,
#138327,#138328,#138329,#138330,#138331),(#138332,#138333,#138334,#138335,
#138336,#138337,#138338,#138339,#138340),(#138341,#138342,#138343,#138344,
#138345,#138346,#138347,#138348,#138349),(#138350,#138351,#138352,#138353,
#138354,#138355,#138356,#138357,#138358),(#138359,#138360,#138361,#138362,
#138363,#138364,#138365,#138366,#138367)),.UNSPECIFIED.,.F.,.F.,.F.,(4,
1,1,1,1,1,1,1,1,1,4),(4,1,1,1,1,1,4),(0.,0.133046842649236,0.255715309974117,
0.378383777298997,0.501052244623878,0.623720711948759,0.746389179273639,
0.807723412936079,0.86905764659852,0.93039188026096,1.),(0.,0.268199906405258,
0.384249094355361,0.500298282305557,0.61634747025566,0.732396658205762,
1.),.UNSPECIFIED.);
#133=B_SPLINE_SURFACE_WITH_KNOTS('',3,3,((#138412,#138413,#138414,#138415,
#138416,#138417,#138418,#138419,#138420),(#138421,#138422,#138423,#138424,
#138425,#138426,#138427,#138428,#138429),(#138430,#138431,#138432,#138433,
#138434,#138435,#138436,#138437,#138438),(#138439,#138440,#138441,#138442,
#138443,#138444,#138445,#138446,#138447),(#138448,#138449,#138450,#138451,
#138452,#138453,#138454,#138455,#138456),(#138457,#138458,#138459,#138460,
#138461,#138462,#138463,#138464,#138465),(#138466,#138467,#138468,#138469,
#138470,#138471,#138472,#138473,#138474),(#138475,#138476,#138477,#138478,
#138479,#138480,#138481,#138482,#138483),(#138484,#138485,#138486,#138487,
#138488,#138489,#138490,#138491,#138492),(#138493,#138494,#138495,#138496,
#138497,#138498,#138499,#138500,#138501),(#138502,#138503,#138504,#138505,
#138506,#138507,#138508,#138509,#138510),(#138511,#138512,#138513,#138514,
#138515,#138516,#138517,#138518,#138519),(#138520,#138521,#138522,#138523,
#138524,#138525,#138526,#138527,#138528),(#138529,#138530,#138531,#138532,
#138533,#138534,#138535,#138536,#138537),(#138538,#138539,#138540,#138541,
#138542,#138543,#138544,#138545,#138546),(#138547,#138548,#138549,#138550,
#138551,#138552,#138553,#138554,#138555)),.UNSPECIFIED.,.F.,.F.,.F.,(4,
1,1,1,1,1,1,1,1,1,1,1,1,4),(4,1,1,1,1,1,4),(0.,0.130820538487595,0.192157288159239,
0.253494037830883,0.314830787502527,0.376167537174171,0.437504286845815,
0.498841036517459,0.560177786189103,0.621514535860747,0.682851285532391,
0.744188035204036,0.866861534547324,1.),(0.,0.268122375620859,0.384109336577756,
0.500096297534654,0.616083258491645,0.732070219448542,1.),.UNSPECIFIED.);
#134=B_SPLINE_SURFACE_WITH_KNOTS('',3,3,((#138565,#138566,#138567,#138568,
#138569,#138570,#138571),(#138572,#138573,#138574,#138575,#138576,#138577,
#138578),(#138579,#138580,#138581,#138582,#138583,#138584,#138585),(#138586,
#138587,#138588,#138589,#138590,#138591,#138592),(#138593,#138594,#138595,
#138596,#138597,#138598,#138599),(#138600,#138601,#138602,#138603,#138604,
#138605,#138606),(#138607,#138608,#138609,#138610,#138611,#138612,#138613),
(#138614,#138615,#138616,#138617,#138618,#138619,#138620),(#138621,#138622,
#138623,#138624,#138625,#138626,#138627),(#138628,#138629,#138630,#138631,
#138632,#138633,#138634),(#138635,#138636,#138637,#138638,#138639,#138640,
#138641),(#138642,#138643,#138644,#138645,#138646,#138647,#138648)),
 .UNSPECIFIED.,.F.,.F.,.F.,(4,1,1,1,1,1,1,1,1,4),(4,1,1,1,4),(0.,0.25699883636701,
0.378859719476966,0.500720602586923,0.561651044141901,0.622581485696879,
0.683511927251857,0.744442368806835,0.866303251916792,1.),(0.,0.268023493710597,
0.500050957704942,0.732078421699288,1.),.UNSPECIFIED.);
#135=B_SPLINE_SURFACE_WITH_KNOTS('',3,3,((#138716,#138717,#138718,#138719,
#138720,#138721,#138722,#138723,#138724,#138725,#138726,#138727,#138728,
#138729,#138730,#138731),(#138732,#138733,#138734,#138735,#138736,#138737,
#138738,#138739,#138740,#138741,#138742,#138743,#138744,#138745,#138746,
#138747),(#138748,#138749,#138750,#138751,#138752,#138753,#138754,#138755,
#138756,#138757,#138758,#138759,#138760,#138761,#138762,#138763),(#138764,
#138765,#138766,#138767,#138768,#138769,#138770,#138771,#138772,#138773,
#138774,#138775,#138776,#138777,#138778,#138779),(#138780,#138781,#138782,
#138783,#138784,#138785,#138786,#138787,#138788,#138789,#138790,#138791,
#138792,#138793,#138794,#138795),(#138796,#138797,#138798,#138799,#138800,
#138801,#138802,#138803,#138804,#138805,#138806,#138807,#138808,#138809,
#138810,#138811),(#138812,#138813,#138814,#138815,#138816,#138817,#138818,
#138819,#138820,#138821,#138822,#138823,#138824,#138825,#138826,#138827),
(#138828,#138829,#138830,#138831,#138832,#138833,#138834,#138835,#138836,
#138837,#138838,#138839,#138840,#138841,#138842,#138843),(#138844,#138845,
#138846,#138847,#138848,#138849,#138850,#138851,#138852,#138853,#138854,
#138855,#138856,#138857,#138858,#138859),(#138860,#138861,#138862,#138863,
#138864,#138865,#138866,#138867,#138868,#138869,#138870,#138871,#138872,
#138873,#138874,#138875),(#138876,#138877,#138878,#138879,#138880,#138881,
#138882,#138883,#138884,#138885,#138886,#138887,#138888,#138889,#138890,
#138891),(#138892,#138893,#138894,#138895,#138896,#138897,#138898,#138899,
#138900,#138901,#138902,#138903,#138904,#138905,#138906,#138907),(#138908,
#138909,#138910,#138911,#138912,#138913,#138914,#138915,#138916,#138917,
#138918,#138919,#138920,#138921,#138922,#138923),(#138924,#138925,#138926,
#138927,#138928,#138929,#138930,#138931,#138932,#138933,#138934,#138935,
#138936,#138937,#138938,#138939)),.UNSPECIFIED.,.F.,.F.,.F.,(4,1,1,1,1,
1,1,1,1,1,1,4),(4,1,1,1,1,1,1,1,1,1,1,1,1,4),(0.,0.134085205130259,0.25595122318364,
0.377817241237021,0.499683259290403,0.621549277343784,0.682482286370475,
0.743415295397166,0.804348304423856,0.865281313450547,0.926214322477238,
1.),(0.,0.132425037814215,0.193700746780136,0.254976455746057,0.316252164711979,
0.3775278736779,0.40816572816086,0.438803582643821,0.469441437126781,0.500079291609742,
0.561355000575663,0.622630709541584,0.745182127473427,1.),.UNSPECIFIED.);
#136=B_SPLINE_SURFACE_WITH_KNOTS('',3,3,((#140502,#140503,#140504,#140505,
#140506,#140507),(#140508,#140509,#140510,#140511,#140512,#140513),(#140514,
#140515,#140516,#140517,#140518,#140519),(#140520,#140521,#140522,#140523,
#140524,#140525),(#140526,#140527,#140528,#140529,#140530,#140531)),
 .UNSPECIFIED.,.F.,.F.,.F.,(4,1,4),(4,1,1,4),(0.,0.369957079162583,1.),
(0.,0.342988625591935,0.659504826702446,1.),.UNSPECIFIED.);
#137=B_SPLINE_SURFACE_WITH_KNOTS('',3,3,((#141306,#141307,#141308,#141309,
#141310,#141311,#141312,#141313),(#141314,#141315,#141316,#141317,#141318,
#141319,#141320,#141321),(#141322,#141323,#141324,#141325,#141326,#141327,
#141328,#141329),(#141330,#141331,#141332,#141333,#141334,#141335,#141336,
#141337),(#141338,#141339,#141340,#141341,#141342,#141343,#141344,#141345),
(#141346,#141347,#141348,#141349,#141350,#141351,#141352,#141353),(#141354,
#141355,#141356,#141357,#141358,#141359,#141360,#141361),(#141362,#141363,
#141364,#141365,#141366,#141367,#141368,#141369),(#141370,#141371,#141372,
#141373,#141374,#141375,#141376,#141377),(#141378,#141379,#141380,#141381,
#141382,#141383,#141384,#141385),(#141386,#141387,#141388,#141389,#141390,
#141391,#141392,#141393),(#141394,#141395,#141396,#141397,#141398,#141399,
#141400,#141401)),.UNSPECIFIED.,.F.,.F.,.F.,(4,1,1,1,1,1,1,1,1,4),(4,1,
1,1,1,4),(0.,0.132237188173058,0.254692642818978,0.499603552110817,0.622059006756737,
0.744514461402656,0.805742188725616,0.866969916048576,0.928197643371536,
1.),(0.,0.368244530951745,0.72001943774428,0.807963164442414,0.895906891140547,
1.),.UNSPECIFIED.);
#138=B_SPLINE_SURFACE_WITH_KNOTS('',3,3,((#142290,#142291,#142292,#142293,
#142294,#142295,#142296,#142297,#142298,#142299,#142300,#142301,#142302,
#142303,#142304,#142305,#142306),(#142307,#142308,#142309,#142310,#142311,
#142312,#142313,#142314,#142315,#142316,#142317,#142318,#142319,#142320,
#142321,#142322,#142323),(#142324,#142325,#142326,#142327,#142328,#142329,
#142330,#142331,#142332,#142333,#142334,#142335,#142336,#142337,#142338,
#142339,#142340),(#142341,#142342,#142343,#142344,#142345,#142346,#142347,
#142348,#142349,#142350,#142351,#142352,#142353,#142354,#142355,#142356,
#142357),(#142358,#142359,#142360,#142361,#142362,#142363,#142364,#142365,
#142366,#142367,#142368,#142369,#142370,#142371,#142372,#142373,#142374),
(#142375,#142376,#142377,#142378,#142379,#142380,#142381,#142382,#142383,
#142384,#142385,#142386,#142387,#142388,#142389,#142390,#142391),(#142392,
#142393,#142394,#142395,#142396,#142397,#142398,#142399,#142400,#142401,
#142402,#142403,#142404,#142405,#142406,#142407,#142408),(#142409,#142410,
#142411,#142412,#142413,#142414,#142415,#142416,#142417,#142418,#142419,
#142420,#142421,#142422,#142423,#142424,#142425),(#142426,#142427,#142428,
#142429,#142430,#142431,#142432,#142433,#142434,#142435,#142436,#142437,
#142438,#142439,#142440,#142441,#142442),(#142443,#142444,#142445,#142446,
#142447,#142448,#142449,#142450,#142451,#142452,#142453,#142454,#142455,
#142456,#142457,#142458,#142459),(#142460,#142461,#142462,#142463,#142464,
#142465,#142466,#142467,#142468,#142469,#142470,#142471,#142472,#142473,
#142474,#142475,#142476)),.UNSPECIFIED.,.F.,.F.,.F.,(4,1,1,1,1,1,1,1,4),
(4,1,1,1,1,1,1,1,1,1,1,1,1,1,4),(0.,0.0889679837912601,0.269044155127216,
0.449120326463171,0.629196497799126,0.719234583467104,0.809272669135082,
0.899313189025203,1.),(0.,0.0299186510352439,0.0465421302688725,0.0548538698856868,
0.0631656095025011,0.0714773491193154,0.0797890887361297,0.0964125679697582,
0.113036047203387,0.146283005670644,0.212776922605158,0.279270839539673,
0.412258673408701,0.678234341146759,1.),.UNSPECIFIED.);
#139=B_SPLINE_SURFACE_WITH_KNOTS('',3,3,((#142494,#142495,#142496,#142497,
#142498,#142499,#142500,#142501,#142502,#142503,#142504,#142505,#142506,
#142507,#142508,#142509,#142510),(#142511,#142512,#142513,#142514,#142515,
#142516,#142517,#142518,#142519,#142520,#142521,#142522,#142523,#142524,
#142525,#142526,#142527),(#142528,#142529,#142530,#142531,#142532,#142533,
#142534,#142535,#142536,#142537,#142538,#142539,#142540,#142541,#142542,
#142543,#142544),(#142545,#142546,#142547,#142548,#142549,#142550,#142551,
#142552,#142553,#142554,#142555,#142556,#142557,#142558,#142559,#142560,
#142561),(#142562,#142563,#142564,#142565,#142566,#142567,#142568,#142569,
#142570,#142571,#142572,#142573,#142574,#142575,#142576,#142577,#142578),
(#142579,#142580,#142581,#142582,#142583,#142584,#142585,#142586,#142587,
#142588,#142589,#142590,#142591,#142592,#142593,#142594,#142595),(#142596,
#142597,#142598,#142599,#142600,#142601,#142602,#142603,#142604,#142605,
#142606,#142607,#142608,#142609,#142610,#142611,#142612),(#142613,#142614,
#142615,#142616,#142617,#142618,#142619,#142620,#142621,#142622,#142623,
#142624,#142625,#142626,#142627,#142628,#142629),(#142630,#142631,#142632,
#142633,#142634,#142635,#142636,#142637,#142638,#142639,#142640,#142641,
#142642,#142643,#142644,#142645,#142646),(#142647,#142648,#142649,#142650,
#142651,#142652,#142653,#142654,#142655,#142656,#142657,#142658,#142659,
#142660,#142661,#142662,#142663),(#142664,#142665,#142666,#142667,#142668,
#142669,#142670,#142671,#142672,#142673,#142674,#142675,#142676,#142677,
#142678,#142679,#142680)),.UNSPECIFIED.,.F.,.F.,.F.,(4,1,1,1,1,1,1,1,4),
(4,1,1,1,1,1,1,1,1,1,1,1,1,1,4),(0.,0.100847834071465,0.1908968616028,0.280915298912381,
0.370933736221962,0.550970610841123,0.731007485460285,0.911044360079447,
1.),(0.,0.0299179598037716,0.0465410175397665,0.054852546407764,0.0631640752757615,
0.0714756041437589,0.0797871330117564,0.0964101907477513,0.113033248483746,
0.146279363955736,0.212771594899716,0.279263825843695,0.412248287731655,
0.678217211507574,1.),.UNSPECIFIED.);
#140=B_SPLINE_SURFACE_WITH_KNOTS('',3,3,((#142692,#142693,#142694,#142695,
#142696,#142697,#142698,#142699),(#142700,#142701,#142702,#142703,#142704,
#142705,#142706,#142707),(#142708,#142709,#142710,#142711,#142712,#142713,
#142714,#142715),(#142716,#142717,#142718,#142719,#142720,#142721,#142722,
#142723),(#142724,#142725,#142726,#142727,#142728,#142729,#142730,#142731),
(#142732,#142733,#142734,#142735,#142736,#142737,#142738,#142739),(#142740,
#142741,#142742,#142743,#142744,#142745,#142746,#142747),(#142748,#142749,
#142750,#142751,#142752,#142753,#142754,#142755),(#142756,#142757,#142758,
#142759,#142760,#142761,#142762,#142763),(#142764,#142765,#142766,#142767,
#142768,#142769,#142770,#142771),(#142772,#142773,#142774,#142775,#142776,
#142777,#142778,#142779),(#142780,#142781,#142782,#142783,#142784,#142785,
#142786,#142787)),.UNSPECIFIED.,.F.,.F.,.F.,(4,1,1,1,1,1,1,1,1,4),(4,1,
1,1,1,4),(0.,0.0720826203636762,0.133291887827124,0.194500937409253,0.255709986991381,
0.378128086155638,0.500546185319895,0.745382383648409,0.867800482812665,
1.),(0.,0.368244531554185,0.720019439162548,0.807963166064639,0.895906892966729,
1.),.UNSPECIFIED.);
#141=B_SPLINE_SURFACE_WITH_KNOTS('',3,3,((#144028,#144029,#144030,#144031),
(#144032,#144033,#144034,#144035),(#144036,#144037,#144038,#144039),(#144040,
#144041,#144042,#144043),(#144044,#144045,#144046,#144047),(#144048,#144049,
#144050,#144051),(#144052,#144053,#144054,#144055)),.UNSPECIFIED.,.F.,.F.,
 .F.,(4,1,1,1,4),(4,4),(0.,0.244135329830522,0.48749215556374,0.730848981296959,
1.),(0.,1.),.UNSPECIFIED.);
#142=B_SPLINE_SURFACE_WITH_KNOTS('',3,3,((#144080,#144081,#144082,#144083),
(#144084,#144085,#144086,#144087),(#144088,#144089,#144090,#144091),(#144092,
#144093,#144094,#144095)),.UNSPECIFIED.,.F.,.F.,.F.,(4,4),(4,4),(0.,1.),
(0.,1.),.UNSPECIFIED.);
#143=B_SPLINE_SURFACE_WITH_KNOTS('',3,3,((#144143,#144144,#144145,#144146),
(#144147,#144148,#144149,#144150),(#144151,#144152,#144153,#144154),(#144155,
#144156,#144157,#144158)),.UNSPECIFIED.,.F.,.F.,.F.,(4,4),(4,4),(0.,1.),
(0.,1.),.UNSPECIFIED.);
#144=B_SPLINE_SURFACE_WITH_KNOTS('',3,3,((#144194,#144195,#144196,#144197),
(#144198,#144199,#144200,#144201),(#144202,#144203,#144204,#144205),(#144206,
#144207,#144208,#144209)),.UNSPECIFIED.,.F.,.F.,.F.,(4,4),(4,4),(0.,1.),
(0.,1.),.UNSPECIFIED.);
#145=B_SPLINE_SURFACE_WITH_KNOTS('',3,3,((#144342,#144343,#144344,#144345,
#144346,#144347),(#144348,#144349,#144350,#144351,#144352,#144353),(#144354,
#144355,#144356,#144357,#144358,#144359),(#144360,#144361,#144362,#144363,
#144364,#144365),(#144366,#144367,#144368,#144369,#144370,#144371)),
 .UNSPECIFIED.,.F.,.F.,.F.,(4,1,4),(4,1,1,4),(0.,0.697012231186303,1.),
(0.,0.257158083013883,0.500013148495854,1.),.UNSPECIFIED.);
#146=B_SPLINE_SURFACE_WITH_KNOTS('',3,3,((#144608,#144609,#144610,#144611,
#144612,#144613,#144614,#144615,#144616),(#144617,#144618,#144619,#144620,
#144621,#144622,#144623,#144624,#144625),(#144626,#144627,#144628,#144629,
#144630,#144631,#144632,#144633,#144634),(#144635,#144636,#144637,#144638,
#144639,#144640,#144641,#144642,#144643),(#144644,#144645,#144646,#144647,
#144648,#144649,#144650,#144651,#144652),(#144653,#144654,#144655,#144656,
#144657,#144658,#144659,#144660,#144661)),.UNSPECIFIED.,.F.,.F.,.F.,(4,
1,1,4),(4,1,1,1,1,1,4),(0.,0.131537245772329,0.300810603491857,1.),(0.,
0.135760677797667,0.257212789613593,0.378664901429518,0.500117013245444,
0.743021236877295,1.),.UNSPECIFIED.);
#147=B_SPLINE_SURFACE_WITH_KNOTS('',3,3,((#144666,#144667,#144668,#144669),
(#144670,#144671,#144672,#144673),(#144674,#144675,#144676,#144677),(#144678,
#144679,#144680,#144681)),.UNSPECIFIED.,.F.,.F.,.F.,(4,4),(4,4),(0.,1.),
(0.,1.),.UNSPECIFIED.);
#148=B_SPLINE_SURFACE_WITH_KNOTS('',3,3,((#144814,#144815,#144816,#144817,
#144818,#144819,#144820),(#144821,#144822,#144823,#144824,#144825,#144826,
#144827),(#144828,#144829,#144830,#144831,#144832,#144833,#144834),(#144835,
#144836,#144837,#144838,#144839,#144840,#144841),(#144842,#144843,#144844,
#144845,#144846,#144847,#144848)),.UNSPECIFIED.,.F.,.F.,.F.,(4,1,4),(4,
1,1,1,4),(0.,0.434785331173339,1.),(0.,0.317132125632511,0.510431545616903,
0.703730965601296,1.),.UNSPECIFIED.);
#149=B_SPLINE_SURFACE_WITH_KNOTS('',3,3,((#145067,#145068,#145069,#145070,
#145071,#145072,#145073),(#145074,#145075,#145076,#145077,#145078,#145079,
#145080),(#145081,#145082,#145083,#145084,#145085,#145086,#145087),(#145088,
#145089,#145090,#145091,#145092,#145093,#145094)),.UNSPECIFIED.,.F.,.F.,
 .F.,(4,4),(4,1,1,1,4),(0.,1.),(0.,0.317106921791329,0.510285028193446,
0.703322658299063,1.),.UNSPECIFIED.);
#150=B_SPLINE_SURFACE_WITH_KNOTS('',3,3,((#145106,#145107,#145108,#145109,
#145110,#145111),(#145112,#145113,#145114,#145115,#145116,#145117),(#145118,
#145119,#145120,#145121,#145122,#145123),(#145124,#145125,#145126,#145127,
#145128,#145129)),.UNSPECIFIED.,.F.,.F.,.F.,(4,4),(4,1,1,4),(0.,1.),(0.,
0.342987585047177,0.659504136375237,1.),.UNSPECIFIED.);
#151=B_SPLINE_SURFACE_WITH_KNOTS('',3,3,((#145239,#145240,#145241,#145242),
(#145243,#145244,#145245,#145246),(#145247,#145248,#145249,#145250),(#145251,
#145252,#145253,#145254)),.UNSPECIFIED.,.F.,.F.,.F.,(4,4),(4,4),(0.,1.),
(0.,1.),.UNSPECIFIED.);
#152=B_SPLINE_SURFACE_WITH_KNOTS('',3,3,((#147022,#147023,#147024,#147025,
#147026),(#147027,#147028,#147029,#147030,#147031),(#147032,#147033,#147034,
#147035,#147036),(#147037,#147038,#147039,#147040,#147041),(#147042,#147043,
#147044,#147045,#147046),(#147047,#147048,#147049,#147050,#147051),(#147052,
#147053,#147054,#147055,#147056),(#147057,#147058,#147059,#147060,#147061),
(#147062,#147063,#147064,#147065,#147066),(#147067,#147068,#147069,#147070,
#147071),(#147072,#147073,#147074,#147075,#147076),(#147077,#147078,#147079,
#147080,#147081),(#147082,#147083,#147084,#147085,#147086),(#147087,#147088,
#147089,#147090,#147091),(#147092,#147093,#147094,#147095,#147096)),
 .UNSPECIFIED.,.F.,.F.,.F.,(4,1,1,1,1,1,1,1,1,1,1,1,4),(4,1,4),(0.,0.132758396201778,
0.255171695067938,0.316378344501018,0.377584993934098,0.438791643367178,
0.499998292800258,0.561204942233338,0.622411591666418,0.683618241099498,
0.744824890532579,0.867238189398739,1.),(0.,0.579456290792951,1.),
 .UNSPECIFIED.);
#153=B_SPLINE_SURFACE_WITH_KNOTS('',3,3,((#148668,#148669,#148670,#148671,
#148672,#148673,#148674),(#148675,#148676,#148677,#148678,#148679,#148680,
#148681),(#148682,#148683,#148684,#148685,#148686,#148687,#148688),(#148689,
#148690,#148691,#148692,#148693,#148694,#148695),(#148696,#148697,#148698,
#148699,#148700,#148701,#148702),(#148703,#148704,#148705,#148706,#148707,
#148708,#148709),(#148710,#148711,#148712,#148713,#148714,#148715,#148716),
(#148717,#148718,#148719,#148720,#148721,#148722,#148723),(#148724,#148725,
#148726,#148727,#148728,#148729,#148730)),.UNSPECIFIED.,.F.,.F.,.F.,(4,
1,1,1,1,1,4),(4,1,1,1,4),(0.,0.132239664806569,0.254822586974579,0.4999884313106,
0.62257135347861,0.74515427564662,1.),(0.,0.263399375189117,0.5001298925661,
0.736860409943177,1.),.UNSPECIFIED.);
#154=B_SPLINE_SURFACE_WITH_KNOTS('',3,3,((#149012,#149013,#149014,#149015,
#149016,#149017,#149018),(#149019,#149020,#149021,#149022,#149023,#149024,
#149025),(#149026,#149027,#149028,#149029,#149030,#149031,#149032),(#149033,
#149034,#149035,#149036,#149037,#149038,#149039),(#149040,#149041,#149042,
#149043,#149044,#149045,#149046),(#149047,#149048,#149049,#149050,#149051,
#149052,#149053),(#149054,#149055,#149056,#149057,#149058,#149059,#149060),
(#149061,#149062,#149063,#149064,#149065,#149066,#149067),(#149068,#149069,
#149070,#149071,#149072,#149073,#149074),(#149075,#149076,#149077,#149078,
#149079,#149080,#149081),(#149082,#149083,#149084,#149085,#149086,#149087,
#149088),(#149089,#149090,#149091,#149092,#149093,#149094,#149095),(#149096,
#149097,#149098,#149099,#149100,#149101,#149102),(#149103,#149104,#149105,
#149106,#149107,#149108,#149109),(#149110,#149111,#149112,#149113,#149114,
#149115,#149116)),.UNSPECIFIED.,.F.,.F.,.F.,(4,1,1,1,1,1,1,1,1,1,1,1,4),
(4,1,1,1,4),(0.,0.132202892489769,0.193512430520198,0.254821968550627,0.316131506581056,
0.377441044611485,0.438750582641914,0.500060120672344,0.561369658702773,
0.622679196733201,0.74529827279406,0.867917348854918,1.),(0.,0.262289949012551,
0.500131074192934,0.737972199373412,1.),.UNSPECIFIED.);
#155=B_SPLINE_SURFACE_WITH_KNOTS('',3,3,((#149465,#149466,#149467,#149468,
#149469,#149470,#149471),(#149472,#149473,#149474,#149475,#149476,#149477,
#149478),(#149479,#149480,#149481,#149482,#149483,#149484,#149485),(#149486,
#149487,#149488,#149489,#149490,#149491,#149492),(#149493,#149494,#149495,
#149496,#149497,#149498,#149499),(#149500,#149501,#149502,#149503,#149504,
#149505,#149506),(#149507,#149508,#149509,#149510,#149511,#149512,#149513),
(#149514,#149515,#149516,#149517,#149518,#149519,#149520),(#149521,#149522,
#149523,#149524,#149525,#149526,#149527)),.UNSPECIFIED.,.F.,.F.,.F.,(4,
1,1,1,1,1,4),(4,1,1,1,4),(0.,0.132239677404676,0.254822595509748,0.499988431719892,
0.622571349824964,0.745154267930036,1.),(0.,0.263425190538822,0.500155220443197,
0.736885250347666,1.),.UNSPECIFIED.);
#156=B_SPLINE_SURFACE_WITH_KNOTS('',3,3,((#149635,#149636,#149637,#149638,
#149639,#149640,#149641),(#149642,#149643,#149644,#149645,#149646,#149647,
#149648),(#149649,#149650,#149651,#149652,#149653,#149654,#149655),(#149656,
#149657,#149658,#149659,#149660,#149661,#149662),(#149663,#149664,#149665,
#149666,#149667,#149668,#149669),(#149670,#149671,#149672,#149673,#149674,
#149675,#149676),(#149677,#149678,#149679,#149680,#149681,#149682,#149683),
(#149684,#149685,#149686,#149687,#149688,#149689,#149690),(#149691,#149692,
#149693,#149694,#149695,#149696,#149697),(#149698,#149699,#149700,#149701,
#149702,#149703,#149704),(#149705,#149706,#149707,#149708,#149709,#149710,
#149711),(#149712,#149713,#149714,#149715,#149716,#149717,#149718),(#149719,
#149720,#149721,#149722,#149723,#149724,#149725)),.UNSPECIFIED.,.F.,.F.,
 .F.,(4,1,1,1,1,1,1,1,1,1,4),(4,1,1,1,4),(0.,0.132545826215179,0.255032336533119,
0.377518846851059,0.438762102010029,0.500005357168999,0.561248612327969,
0.622491867486939,0.744978377804879,0.867464888122819,1.),(0.,0.262900516152029,
0.500175417475005,0.737450318797982,1.),.UNSPECIFIED.);
#157=B_SPLINE_SURFACE_WITH_KNOTS('',3,3,((#150344,#150345,#150346,#150347,
#150348,#150349,#150350),(#150351,#150352,#150353,#150354,#150355,#150356,
#150357),(#150358,#150359,#150360,#150361,#150362,#150363,#150364),(#150365,
#150366,#150367,#150368,#150369,#150370,#150371),(#150372,#150373,#150374,
#150375,#150376,#150377,#150378),(#150379,#150380,#150381,#150382,#150383,
#150384,#150385),(#150386,#150387,#150388,#150389,#150390,#150391,#150392),
(#150393,#150394,#150395,#150396,#150397,#150398,#150399),(#150400,#150401,
#150402,#150403,#150404,#150405,#150406)),.UNSPECIFIED.,.F.,.F.,.F.,(4,
1,1,1,1,1,4),(4,1,1,1,4),(0.,0.132239677404625,0.254822595509704,0.499988431719863,
0.622571349824942,0.745154267930021,1.),(0.,0.26342519053886,0.500155220443287,
0.736885250347713,1.),.UNSPECIFIED.);
#158=B_SPLINE_SURFACE_WITH_KNOTS('',3,3,((#150712,#150713,#150714,#150715,
#150716,#150717,#150718),(#150719,#150720,#150721,#150722,#150723,#150724,
#150725),(#150726,#150727,#150728,#150729,#150730,#150731,#150732),(#150733,
#150734,#150735,#150736,#150737,#150738,#150739),(#150740,#150741,#150742,
#150743,#150744,#150745,#150746),(#150747,#150748,#150749,#150750,#150751,
#150752,#150753),(#150754,#150755,#150756,#150757,#150758,#150759,#150760),
(#150761,#150762,#150763,#150764,#150765,#150766,#150767),(#150768,#150769,
#150770,#150771,#150772,#150773,#150774),(#150775,#150776,#150777,#150778,
#150779,#150780,#150781),(#150782,#150783,#150784,#150785,#150786,#150787,
#150788),(#150789,#150790,#150791,#150792,#150793,#150794,#150795),(#150796,
#150797,#150798,#150799,#150800,#150801,#150802)),.UNSPECIFIED.,.F.,.F.,
 .F.,(4,1,1,1,1,1,1,1,1,1,4),(4,1,1,1,4),(0.,0.132545826214933,0.255032336532908,
0.377518846850882,0.43876210200987,0.500005357168857,0.561248612327844,
0.622491867486832,0.744978377804806,0.867464888122781,1.),(0.,0.262905612958216,
0.500178847936523,0.737452082914831,1.),.UNSPECIFIED.);
#159=B_SPLINE_SURFACE_WITH_KNOTS('',3,3,((#150892,#150893,#150894,#150895,
#150896,#150897,#150898),(#150899,#150900,#150901,#150902,#150903,#150904,
#150905),(#150906,#150907,#150908,#150909,#150910,#150911,#150912),(#150913,
#150914,#150915,#150916,#150917,#150918,#150919),(#150920,#150921,#150922,
#150923,#150924,#150925,#150926),(#150927,#150928,#150929,#150930,#150931,
#150932,#150933),(#150934,#150935,#150936,#150937,#150938,#150939,#150940),
(#150941,#150942,#150943,#150944,#150945,#150946,#150947),(#150948,#150949,
#150950,#150951,#150952,#150953,#150954)),.UNSPECIFIED.,.F.,.F.,.F.,(4,
1,1,1,1,1,4),(4,1,1,1,4),(0.,0.132239664806391,0.254822586974288,0.499988431310081,
0.622571353477978,0.745154275645875,1.),(0.,0.263399375189117,0.5001298925661,
0.736860409943082,1.),.UNSPECIFIED.);
#160=B_SPLINE_SURFACE_WITH_KNOTS('',3,3,((#151226,#151227,#151228,#151229,
#151230,#151231,#151232),(#151233,#151234,#151235,#151236,#151237,#151238,
#151239),(#151240,#151241,#151242,#151243,#151244,#151245,#151246),(#151247,
#151248,#151249,#151250,#151251,#151252,#151253),(#151254,#151255,#151256,
#151257,#151258,#151259,#151260),(#151261,#151262,#151263,#151264,#151265,
#151266,#151267),(#151268,#151269,#151270,#151271,#151272,#151273,#151274),
(#151275,#151276,#151277,#151278,#151279,#151280,#151281),(#151282,#151283,
#151284,#151285,#151286,#151287,#151288),(#151289,#151290,#151291,#151292,
#151293,#151294,#151295),(#151296,#151297,#151298,#151299,#151300,#151301,
#151302),(#151303,#151304,#151305,#151306,#151307,#151308,#151309),(#151310,
#151311,#151312,#151313,#151314,#151315,#151316),(#151317,#151318,#151319,
#151320,#151321,#151322,#151323),(#151324,#151325,#151326,#151327,#151328,
#151329,#151330)),.UNSPECIFIED.,.F.,.F.,.F.,(4,1,1,1,1,1,1,1,1,1,1,1,4),
(4,1,1,1,4),(0.,0.132202892489662,0.193512430520099,0.254821968550535,0.316131506580972,
0.377441044611408,0.438750582641845,0.500060120672282,0.561369658702718,
0.622679196733155,0.745298272794028,0.867917348854901,1.),(0.,0.262289949012583,
0.500131074192996,0.737972199373408,1.),.UNSPECIFIED.);
#161=B_SPLINE_SURFACE_WITH_KNOTS('',3,3,((#151468,#151469,#151470,#151471,
#151472,#151473,#151474,#151475,#151476,#151477,#151478),(#151479,#151480,
#151481,#151482,#151483,#151484,#151485,#151486,#151487,#151488,#151489),
(#151490,#151491,#151492,#151493,#151494,#151495,#151496,#151497,#151498,
#151499,#151500),(#151501,#151502,#151503,#151504,#151505,#151506,#151507,
#151508,#151509,#151510,#151511),(#151512,#151513,#151514,#151515,#151516,
#151517,#151518,#151519,#151520,#151521,#151522),(#151523,#151524,#151525,
#151526,#151527,#151528,#151529,#151530,#151531,#151532,#151533),(#151534,
#151535,#151536,#151537,#151538,#151539,#151540,#151541,#151542,#151543,
#151544),(#151545,#151546,#151547,#151548,#151549,#151550,#151551,#151552,
#151553,#151554,#151555),(#151556,#151557,#151558,#151559,#151560,#151561,
#151562,#151563,#151564,#151565,#151566)),.UNSPECIFIED.,.F.,.F.,.F.,(4,
1,1,1,1,1,4),(4,1,1,1,1,1,1,1,4),(0.,0.254208751460181,0.499694013842769,
0.622436645034063,0.745179276225357,0.86792190741665,1.),(0.,0.138828491142032,
0.259244177039013,0.379659862935897,0.500075548832782,0.620491234729763,
0.740906920626647,0.861322606523628,1.),.UNSPECIFIED.);
#162=B_SPLINE_SURFACE_WITH_KNOTS('',3,3,((#151636,#151637,#151638,#151639,
#151640,#151641,#151642),(#151643,#151644,#151645,#151646,#151647,#151648,
#151649),(#151650,#151651,#151652,#151653,#151654,#151655,#151656),(#151657,
#151658,#151659,#151660,#151661,#151662,#151663),(#151664,#151665,#151666,
#151667,#151668,#151669,#151670),(#151671,#151672,#151673,#151674,#151675,
#151676,#151677),(#151678,#151679,#151680,#151681,#151682,#151683,#151684)),
 .UNSPECIFIED.,.F.,.F.,.F.,(4,1,1,1,4),(4,1,1,1,4),(0.,0.257623699974245,
0.499835655335243,0.742047610696241,1.),(0.,0.259937323174334,0.500055099785869,
0.740172876397403,1.),.UNSPECIFIED.);
#163=B_SPLINE_SURFACE_WITH_KNOTS('',3,3,((#151804,#151805,#151806,#151807,
#151808,#151809,#151810,#151811,#151812,#151813,#151814),(#151815,#151816,
#151817,#151818,#151819,#151820,#151821,#151822,#151823,#151824,#151825),
(#151826,#151827,#151828,#151829,#151830,#151831,#151832,#151833,#151834,
#151835,#151836),(#151837,#151838,#151839,#151840,#151841,#151842,#151843,
#151844,#151845,#151846,#151847),(#151848,#151849,#151850,#151851,#151852,
#151853,#151854,#151855,#151856,#151857,#151858),(#151859,#151860,#151861,
#151862,#151863,#151864,#151865,#151866,#151867,#151868,#151869),(#151870,
#151871,#151872,#151873,#151874,#151875,#151876,#151877,#151878,#151879,
#151880)),.UNSPECIFIED.,.F.,.F.,.F.,(4,1,1,1,4),(4,1,1,1,1,1,1,1,4),(0.,
0.258806803182955,0.500771503994781,0.742736204806219,1.),(0.,0.146126082968561,
0.264104099863688,0.382082116758815,0.500060133653942,0.618038150549069,
0.736016167444196,0.853994184339323,1.),.UNSPECIFIED.);
#164=B_SPLINE_SURFACE_WITH_KNOTS('',3,3,((#151953,#151954,#151955,#151956,
#151957,#151958,#151959),(#151960,#151961,#151962,#151963,#151964,#151965,
#151966),(#151967,#151968,#151969,#151970,#151971,#151972,#151973),(#151974,
#151975,#151976,#151977,#151978,#151979,#151980),(#151981,#151982,#151983,
#151984,#151985,#151986,#151987),(#151988,#151989,#151990,#151991,#151992,
#151993,#151994),(#151995,#151996,#151997,#151998,#151999,#152000,#152001),
(#152002,#152003,#152004,#152005,#152006,#152007,#152008),(#152009,#152010,
#152011,#152012,#152013,#152014,#152015),(#152016,#152017,#152018,#152019,
#152020,#152021,#152022),(#152023,#152024,#152025,#152026,#152027,#152028,
#152029),(#152030,#152031,#152032,#152033,#152034,#152035,#152036),(#152037,
#152038,#152039,#152040,#152041,#152042,#152043),(#152044,#152045,#152046,
#152047,#152048,#152049,#152050),(#152051,#152052,#152053,#152054,#152055,
#152056,#152057),(#152058,#152059,#152060,#152061,#152062,#152063,#152064),
(#152065,#152066,#152067,#152068,#152069,#152070,#152071),(#152072,#152073,
#152074,#152075,#152076,#152077,#152078),(#152079,#152080,#152081,#152082,
#152083,#152084,#152085),(#152086,#152087,#152088,#152089,#152090,#152091,
#152092),(#152093,#152094,#152095,#152096,#152097,#152098,#152099),(#152100,
#152101,#152102,#152103,#152104,#152105,#152106),(#152107,#152108,#152109,
#152110,#152111,#152112,#152113),(#152114,#152115,#152116,#152117,#152118,
#152119,#152120),(#152121,#152122,#152123,#152124,#152125,#152126,#152127),
(#152128,#152129,#152130,#152131,#152132,#152133,#152134),(#152135,#152136,
#152137,#152138,#152139,#152140,#152141),(#152142,#152143,#152144,#152145,
#152146,#152147,#152148),(#152149,#152150,#152151,#152152,#152153,#152154,
#152155),(#152156,#152157,#152158,#152159,#152160,#152161,#152162),(#152163,
#152164,#152165,#152166,#152167,#152168,#152169),(#152170,#152171,#152172,
#152173,#152174,#152175,#152176),(#152177,#152178,#152179,#152180,#152181,
#152182,#152183)),.UNSPECIFIED.,.F.,.F.,.F.,(4,1,1,1,1,1,1,1,1,1,1,1,1,
1,1,1,1,1,1,1,1,1,1,1,1,1,1,1,1,1,4),(4,1,1,1,4),(0.,0.0658304936520168,
0.0968410489872127,0.127851604322409,0.158862159657605,0.1898727149928,
0.220883270327996,0.251893825663192,0.313914936333584,0.34492549166878,
0.375936047003976,0.391441324671574,0.406946602339172,0.437957157674368,
0.468967713009564,0.49997826834476,0.530988823679956,0.561999379015152,
0.593009934350347,0.608515212017945,0.624020489685543,0.655031045020739,
0.686041600355935,0.748062711026327,0.779073266361523,0.810083821696719,
0.841094377031915,0.872104932367111,0.903115487702307,0.934126043037503,
1.),(0.,0.336621216511749,0.510184141880342,0.683747067249001,1.),
 .UNSPECIFIED.);
#165=B_SPLINE_SURFACE_WITH_KNOTS('',3,3,((#152443,#152444,#152445,#152446,
#152447,#152448,#152449,#152450,#152451,#152452,#152453),(#152454,#152455,
#152456,#152457,#152458,#152459,#152460,#152461,#152462,#152463,#152464),
(#152465,#152466,#152467,#152468,#152469,#152470,#152471,#152472,#152473,
#152474,#152475),(#152476,#152477,#152478,#152479,#152480,#152481,#152482,
#152483,#152484,#152485,#152486),(#152487,#152488,#152489,#152490,#152491,
#152492,#152493,#152494,#152495,#152496,#152497),(#152498,#152499,#152500,
#152501,#152502,#152503,#152504,#152505,#152506,#152507,#152508),(#152509,
#152510,#152511,#152512,#152513,#152514,#152515,#152516,#152517,#152518,
#152519),(#152520,#152521,#152522,#152523,#152524,#152525,#152526,#152527,
#152528,#152529,#152530),(#152531,#152532,#152533,#152534,#152535,#152536,
#152537,#152538,#152539,#152540,#152541),(#152542,#152543,#152544,#152545,
#152546,#152547,#152548,#152549,#152550,#152551,#152552),(#152553,#152554,
#152555,#152556,#152557,#152558,#152559,#152560,#152561,#152562,#152563),
(#152564,#152565,#152566,#152567,#152568,#152569,#152570,#152571,#152572,
#152573,#152574),(#152575,#152576,#152577,#152578,#152579,#152580,#152581,
#152582,#152583,#152584,#152585),(#152586,#152587,#152588,#152589,#152590,
#152591,#152592,#152593,#152594,#152595,#152596),(#152597,#152598,#152599,
#152600,#152601,#152602,#152603,#152604,#152605,#152606,#152607),(#152608,
#152609,#152610,#152611,#152612,#152613,#152614,#152615,#152616,#152617,
#152618),(#152619,#152620,#152621,#152622,#152623,#152624,#152625,#152626,
#152627,#152628,#152629),(#152630,#152631,#152632,#152633,#152634,#152635,
#152636,#152637,#152638,#152639,#152640),(#152641,#152642,#152643,#152644,
#152645,#152646,#152647,#152648,#152649,#152650,#152651),(#152652,#152653,
#152654,#152655,#152656,#152657,#152658,#152659,#152660,#152661,#152662)),
 .UNSPECIFIED.,.F.,.F.,.F.,(4,1,1,1,1,1,1,1,1,1,1,1,1,1,1,1,1,4),(4,1,1,
1,1,1,1,1,4),(0.,0.0708680261420804,0.132162830392948,0.254752438894683,
0.316047243145551,0.377342047396419,0.438636851647286,0.46928425377272,
0.499931655898154,0.530579058023588,0.561226460149022,0.622521264399889,
0.683816068650757,0.745110872901625,0.806405677152492,0.86770048140336,
0.928995285654228,1.),(0.,0.136846366314673,0.257938577852228,0.379030789389783,
0.500123000927338,0.621215212464893,0.742307424002448,0.863399635540003,
1.),.UNSPECIFIED.);
#166=B_SPLINE_SURFACE_WITH_KNOTS('',3,3,((#152674,#152675,#152676,#152677,
#152678,#152679,#152680,#152681,#152682,#152683,#152684),(#152685,#152686,
#152687,#152688,#152689,#152690,#152691,#152692,#152693,#152694,#152695),
(#152696,#152697,#152698,#152699,#152700,#152701,#152702,#152703,#152704,
#152705,#152706),(#152707,#152708,#152709,#152710,#152711,#152712,#152713,
#152714,#152715,#152716,#152717),(#152718,#152719,#152720,#152721,#152722,
#152723,#152724,#152725,#152726,#152727,#152728),(#152729,#152730,#152731,
#152732,#152733,#152734,#152735,#152736,#152737,#152738,#152739),(#152740,
#152741,#152742,#152743,#152744,#152745,#152746,#152747,#152748,#152749,
#152750),(#152751,#152752,#152753,#152754,#152755,#152756,#152757,#152758,
#152759,#152760,#152761),(#152762,#152763,#152764,#152765,#152766,#152767,
#152768,#152769,#152770,#152771,#152772),(#152773,#152774,#152775,#152776,
#152777,#152778,#152779,#152780,#152781,#152782,#152783)),.UNSPECIFIED.,
 .F.,.F.,.F.,(4,1,1,1,1,1,1,4),(4,1,1,1,1,1,1,1,4),(0.,0.132043267539266,
0.254787356474467,0.377531445409669,0.500275534344871,0.623019623280073,
0.745763712215274,1.),(0.,0.138828554116791,0.259244178532127,0.379659802947559,
0.500075427362895,0.620491051778231,0.740906676193567,0.861322300609,1.),
 .UNSPECIFIED.);
#167=B_SPLINE_SURFACE_WITH_KNOTS('',3,3,((#153064,#153065,#153066,#153067,
#153068,#153069,#153070,#153071,#153072),(#153073,#153074,#153075,#153076,
#153077,#153078,#153079,#153080,#153081),(#153082,#153083,#153084,#153085,
#153086,#153087,#153088,#153089,#153090),(#153091,#153092,#153093,#153094,
#153095,#153096,#153097,#153098,#153099),(#153100,#153101,#153102,#153103,
#153104,#153105,#153106,#153107,#153108),(#153109,#153110,#153111,#153112,
#153113,#153114,#153115,#153116,#153117),(#153118,#153119,#153120,#153121,
#153122,#153123,#153124,#153125,#153126)),.UNSPECIFIED.,.F.,.F.,.F.,(4,
1,1,1,4),(4,1,1,1,1,1,4),(0.,0.257122326414864,0.49891834990865,0.740714373402823,
1.),(0.,0.264098460225707,0.382080501845444,0.500062543465087,0.618044585084824,
0.736026626704467,1.),.UNSPECIFIED.);
#168=B_SPLINE_SURFACE_WITH_KNOTS('',3,3,((#153186,#153187,#153188,#153189,
#153190,#153191,#153192),(#153193,#153194,#153195,#153196,#153197,#153198,
#153199),(#153200,#153201,#153202,#153203,#153204,#153205,#153206),(#153207,
#153208,#153209,#153210,#153211,#153212,#153213),(#153214,#153215,#153216,
#153217,#153218,#153219,#153220),(#153221,#153222,#153223,#153224,#153225,
#153226,#153227),(#153228,#153229,#153230,#153231,#153232,#153233,#153234)),
 .UNSPECIFIED.,.F.,.F.,.F.,(4,1,1,1,4),(4,1,1,1,4),(0.,0.257735074161703,
0.499844908300334,0.741954742438964,1.),(0.,0.259940639367695,0.500057872218097,
0.740175105068594,1.),.UNSPECIFIED.);
#169=B_SPLINE_SURFACE_WITH_KNOTS('',3,3,((#153359,#153360,#153361,#153362,
#153363,#153364,#153365),(#153366,#153367,#153368,#153369,#153370,#153371,
#153372),(#153373,#153374,#153375,#153376,#153377,#153378,#153379),(#153380,
#153381,#153382,#153383,#153384,#153385,#153386),(#153387,#153388,#153389,
#153390,#153391,#153392,#153393),(#153394,#153395,#153396,#153397,#153398,
#153399,#153400),(#153401,#153402,#153403,#153404,#153405,#153406,#153407),
(#153408,#153409,#153410,#153411,#153412,#153413,#153414),(#153415,#153416,
#153417,#153418,#153419,#153420,#153421),(#153422,#153423,#153424,#153425,
#153426,#153427,#153428),(#153429,#153430,#153431,#153432,#153433,#153434,
#153435),(#153436,#153437,#153438,#153439,#153440,#153441,#153442)),
 .UNSPECIFIED.,.F.,.F.,.F.,(4,1,1,1,1,1,1,1,1,4),(4,1,1,1,4),(0.,0.131942207186592,
0.254618794764067,0.377295382341543,0.499971969919018,0.561310263707756,
0.622648557496493,0.745325145073969,0.868001732651444,1.),(0.,0.257681345106317,
0.499753140798927,0.741824936491634,1.),.UNSPECIFIED.);
#170=B_SPLINE_SURFACE_WITH_KNOTS('',3,3,((#153886,#153887,#153888,#153889,
#153890,#153891,#153892),(#153893,#153894,#153895,#153896,#153897,#153898,
#153899),(#153900,#153901,#153902,#153903,#153904,#153905,#153906),(#153907,
#153908,#153909,#153910,#153911,#153912,#153913),(#153914,#153915,#153916,
#153917,#153918,#153919,#153920),(#153921,#153922,#153923,#153924,#153925,
#153926,#153927),(#153928,#153929,#153930,#153931,#153932,#153933,#153934),
(#153935,#153936,#153937,#153938,#153939,#153940,#153941),(#153942,#153943,
#153944,#153945,#153946,#153947,#153948),(#153949,#153950,#153951,#153952,
#153953,#153954,#153955),(#153956,#153957,#153958,#153959,#153960,#153961,
#153962),(#153963,#153964,#153965,#153966,#153967,#153968,#153969),(#153970,
#153971,#153972,#153973,#153974,#153975,#153976),(#153977,#153978,#153979,
#153980,#153981,#153982,#153983)),.UNSPECIFIED.,.F.,.F.,.F.,(4,1,1,1,1,
1,1,1,1,1,1,4),(4,1,1,1,4),(0.,0.132195054850011,0.254794129835051,0.316093667327571,
0.377393204820091,0.438692742312611,0.499992279805131,0.561291817297652,
0.622591354790172,0.745190429775212,0.867789504760252,1.),(0.,0.261340468241408,
0.500099147644516,0.738857827047623,1.),.UNSPECIFIED.);
#171=B_SPLINE_SURFACE_WITH_KNOTS('',3,3,((#154202,#154203,#154204,#154205,
#154206),(#154207,#154208,#154209,#154210,#154211),(#154212,#154213,#154214,
#154215,#154216),(#154217,#154218,#154219,#154220,#154221)),
 .UNSPECIFIED.,.F.,.F.,.F.,(4,4),(4,1,4),(0.,1.),(0.,0.50287827766393,1.),
 .UNSPECIFIED.);
#172=B_SPLINE_SURFACE_WITH_KNOTS('',3,3,((#154416,#154417,#154418,#154419,
#154420,#154421,#154422),(#154423,#154424,#154425,#154426,#154427,#154428,
#154429),(#154430,#154431,#154432,#154433,#154434,#154435,#154436),(#154437,
#154438,#154439,#154440,#154441,#154442,#154443),(#154444,#154445,#154446,
#154447,#154448,#154449,#154450),(#154451,#154452,#154453,#154454,#154455,
#154456,#154457),(#154458,#154459,#154460,#154461,#154462,#154463,#154464),
(#154465,#154466,#154467,#154468,#154469,#154470,#154471),(#154472,#154473,
#154474,#154475,#154476,#154477,#154478),(#154479,#154480,#154481,#154482,
#154483,#154484,#154485),(#154486,#154487,#154488,#154489,#154490,#154491,
#154492),(#154493,#154494,#154495,#154496,#154497,#154498,#154499),(#154500,
#154501,#154502,#154503,#154504,#154505,#154506),(#154507,#154508,#154509,
#154510,#154511,#154512,#154513)),.UNSPECIFIED.,.F.,.F.,.F.,(4,1,1,1,1,
1,1,1,1,1,1,4),(4,1,1,1,4),(0.,0.132195054849916,0.25479412983497,0.316093667327497,
0.377393204820023,0.43869274231255,0.499992279805077,0.561291817297604,
0.622591354790131,0.745190429775184,0.867789504760238,1.),(0.,0.261340468241415,
0.50009914764452,0.738857827047626,1.),.UNSPECIFIED.);
#173=B_SPLINE_SURFACE_WITH_KNOTS('',3,3,((#154716,#154717,#154718,#154719,
#154720,#154721,#154722),(#154723,#154724,#154725,#154726,#154727,#154728,
#154729),(#154730,#154731,#154732,#154733,#154734,#154735,#154736),(#154737,
#154738,#154739,#154740,#154741,#154742,#154743),(#154744,#154745,#154746,
#154747,#154748,#154749,#154750),(#154751,#154752,#154753,#154754,#154755,
#154756,#154757),(#154758,#154759,#154760,#154761,#154762,#154763,#154764),
(#154765,#154766,#154767,#154768,#154769,#154770,#154771),(#154772,#154773,
#154774,#154775,#154776,#154777,#154778),(#154779,#154780,#154781,#154782,
#154783,#154784,#154785),(#154786,#154787,#154788,#154789,#154790,#154791,
#154792),(#154793,#154794,#154795,#154796,#154797,#154798,#154799),(#154800,
#154801,#154802,#154803,#154804,#154805,#154806)),.UNSPECIFIED.,.F.,.F.,
 .F.,(4,1,1,1,1,1,1,1,1,1,4),(4,1,1,1,4),(0.,0.132030874480919,0.19336634824744,
0.254701822013961,0.316037295780482,0.377372769547002,0.500043717080044,
0.622714664613086,0.745385612146127,0.868056559679169,1.),(0.,0.260567545092337,
0.500088901308193,0.73961025752405,1.),.UNSPECIFIED.);
#174=B_SPLINE_SURFACE_WITH_KNOTS('',3,3,((#155084,#155085,#155086,#155087),
(#155088,#155089,#155090,#155091),(#155092,#155093,#155094,#155095),(#155096,
#155097,#155098,#155099),(#155100,#155101,#155102,#155103),(#155104,#155105,
#155106,#155107),(#155108,#155109,#155110,#155111),(#155112,#155113,#155114,
#155115),(#155116,#155117,#155118,#155119),(#155120,#155121,#155122,#155123),
(#155124,#155125,#155126,#155127),(#155128,#155129,#155130,#155131),(#155132,
#155133,#155134,#155135),(#155136,#155137,#155138,#155139),(#155140,#155141,
#155142,#155143),(#155144,#155145,#155146,#155147)),.UNSPECIFIED.,.F.,.F.,
 .F.,(4,1,1,1,1,1,1,1,1,1,1,1,1,4),(4,4),(0.,0.131636988977778,0.193017807710131,
0.254398626442485,0.315779445174839,0.377160263907192,0.499921901371899,
0.561302720104253,0.622683538836606,0.68406435756896,0.745445176301313,
0.806825995033667,0.86820681376602,1.),(0.,1.),.UNSPECIFIED.);
#175=B_SPLINE_SURFACE_WITH_KNOTS('',3,3,((#155542,#155543,#155544,#155545,
#155546),(#155547,#155548,#155549,#155550,#155551),(#155552,#155553,#155554,
#155555,#155556),(#155557,#155558,#155559,#155560,#155561),(#155562,#155563,
#155564,#155565,#155566),(#155567,#155568,#155569,#155570,#155571),(#155572,
#155573,#155574,#155575,#155576),(#155577,#155578,#155579,#155580,#155581),
(#155582,#155583,#155584,#155585,#155586),(#155587,#155588,#155589,#155590,
#155591),(#155592,#155593,#155594,#155595,#155596),(#155597,#155598,#155599,
#155600,#155601),(#155602,#155603,#155604,#155605,#155606),(#155607,#155608,
#155609,#155610,#155611),(#155612,#155613,#155614,#155615,#155616)),
 .UNSPECIFIED.,.F.,.F.,.F.,(4,1,1,1,1,1,1,1,1,1,1,1,4),(4,1,4),(0.,0.132758396228893,
0.255171695213975,0.316378344706517,0.377584994199058,0.438791643691599,
0.49999829318414,0.561204942676681,0.622411592169222,0.683618241661764,
0.744824891154305,0.867238190139387,1.),(0.,0.579500129312416,1.),
 .UNSPECIFIED.);
#245=FACE_BOUND('',#23999,.T.);
#246=FACE_BOUND('',#24007,.T.);
#247=FACE_BOUND('',#24009,.T.);
#248=FACE_BOUND('',#24078,.T.);
#249=FACE_BOUND('',#24086,.T.);
#250=FACE_BOUND('',#24088,.T.);
#251=FACE_BOUND('',#24096,.T.);
#252=FACE_BOUND('',#24098,.T.);
#253=FACE_BOUND('',#24167,.T.);
#254=FACE_BOUND('',#24175,.T.);
#255=FACE_BOUND('',#24180,.T.);
#256=FACE_BOUND('',#24242,.T.);
#257=FACE_BOUND('',#24244,.T.);
#258=FACE_BOUND('',#24267,.T.);
#259=FACE_BOUND('',#24269,.T.);
#260=FACE_BOUND('',#24271,.T.);
#261=FACE_BOUND('',#24339,.T.);
#262=FACE_BOUND('',#24341,.T.);
#263=FACE_BOUND('',#24394,.T.);
#264=FACE_BOUND('',#24425,.T.);
#265=FACE_BOUND('',#24455,.T.);
#266=FACE_BOUND('',#24474,.T.);
#267=FACE_BOUND('',#24478,.T.);
#268=FACE_BOUND('',#24480,.T.);
#1729=(
BOUNDED_CURVE()
B_SPLINE_CURVE(3,(#113475,#113476,#113477,#113478,#113479,#113480,#113481,
#113482,#113483,#113484,#113485,#113486,#113487,#113488,#113489,#113490),
 .UNSPECIFIED.,.F.,.F.)
B_SPLINE_CURVE_WITH_KNOTS((4,1,1,1,1,1,1,1,1,1,1,1,1,4),(0.,0.060042788247584,
0.141371222377395,0.225595544932924,0.308864429207092,0.38816486004432,
0.463257434984739,0.536512885135913,0.611617817006763,0.691030118817633,
0.774478150226589,0.858703197204449,0.940023204544441,1.),.UNSPECIFIED.)
CURVE()
GEOMETRIC_REPRESENTATION_ITEM()
RATIONAL_B_SPLINE_CURVE((1.00001389582334,1.00001389582334,1.00001389582334,
1.00001389582334,1.00001389582334,1.00001389582334,1.00001389582334,1.00001389582334,
1.00001389582334,1.00001389582334,1.00001389582334,1.00001389582334,1.00001389582334,
1.00001389582334,1.00001389582334,1.00001389582334))
REPRESENTATION_ITEM('')
);
#1730=(
BOUNDED_CURVE()
B_SPLINE_CURVE(3,(#113496,#113497,#113498,#113499,#113500,#113501,#113502,
#113503,#113504,#113505,#113506,#113507,#113508,#113509,#113510,#113511),
 .UNSPECIFIED.,.F.,.F.)
B_SPLINE_CURVE_WITH_KNOTS((4,1,1,1,1,1,1,1,1,1,1,1,1,4),(0.,0.0613883734612031,
0.142549216299429,0.226569566267063,0.309514053988871,0.388483661117508,
0.463334217441732,0.536400941313595,0.611266764348142,0.690361351445686,
0.773496593681541,0.857520919530913,0.93867542130663,1.),.UNSPECIFIED.)
CURVE()
GEOMETRIC_REPRESENTATION_ITEM()
RATIONAL_B_SPLINE_CURVE((1.00001399653248,1.00001399653248,1.00001399653248,
1.00001399653248,1.00001399653248,1.00001399653248,1.00001399653248,1.00001399653248,
1.00001399653248,1.00001399653248,1.00001399653248,1.00001399653248,1.00001399653248,
1.00001399653248,1.00001399653248,1.00001399653248))
REPRESENTATION_ITEM('')
);
#1731=(
BOUNDED_CURVE()
B_SPLINE_CURVE(2,(#115636,#115637,#115638),.UNSPECIFIED.,.F.,.F.)
B_SPLINE_CURVE_WITH_KNOTS((3,3),(-1.23975190889131,-0.413328514141033),
 .UNSPECIFIED.)
CURVE()
GEOMETRIC_REPRESENTATION_ITEM()
RATIONAL_B_SPLINE_CURVE((1.30231782319316,1.50378709162254,1.30231782319316))
REPRESENTATION_ITEM('')
);
#1732=(
BOUNDED_CURVE()
B_SPLINE_CURVE(2,(#115640,#115641,#115642),.UNSPECIFIED.,.F.,.F.)
B_SPLINE_CURVE_WITH_KNOTS((3,3),(-1.23975190893748,-0.413328514094878),
 .UNSPECIFIED.)
CURVE()
GEOMETRIC_REPRESENTATION_ITEM()
RATIONAL_B_SPLINE_CURVE((1.30231782317067,1.50378709164506,1.30231782317066))
REPRESENTATION_ITEM('')
);
#1733=(
BOUNDED_CURVE()
B_SPLINE_CURVE(2,(#115644,#115645,#115646),.UNSPECIFIED.,.F.,.F.)
B_SPLINE_CURVE_WITH_KNOTS((3,3),(-1.23975190893749,-0.413328514094885),
 .UNSPECIFIED.)
CURVE()
GEOMETRIC_REPRESENTATION_ITEM()
RATIONAL_B_SPLINE_CURVE((1.30231782317067,1.50378709164507,1.30231782317067))
REPRESENTATION_ITEM('')
);
#1734=(
BOUNDED_CURVE()
B_SPLINE_CURVE(2,(#115648,#115649,#115650),.UNSPECIFIED.,.F.,.F.)
B_SPLINE_CURVE_WITH_KNOTS((3,3),(0.413328514141046,0.826540211516179),
 .UNSPECIFIED.)
CURVE()
GEOMETRIC_REPRESENTATION_ITEM()
RATIONAL_B_SPLINE_CURVE((1.30231782319316,1.40305245740785,1.40305245740785))
REPRESENTATION_ITEM('')
);
#1735=(
BOUNDED_CURVE()
B_SPLINE_CURVE(2,(#115653,#115654,#115655),.UNSPECIFIED.,.F.,.F.)
B_SPLINE_CURVE_WITH_KNOTS((3,3),(0.826540211516179,1.23975190889131),
 .UNSPECIFIED.)
CURVE()
GEOMETRIC_REPRESENTATION_ITEM()
RATIONAL_B_SPLINE_CURVE((1.40305245740785,1.40305245740785,1.30231782319316))
REPRESENTATION_ITEM('')
);
#1736=(
BOUNDED_CURVE()
B_SPLINE_CURVE(2,(#115657,#115658,#115659),.UNSPECIFIED.,.F.,.F.)
B_SPLINE_CURVE_WITH_KNOTS((3,3),(0.413328514094879,1.23975190893749),
 .UNSPECIFIED.)
CURVE()
GEOMETRIC_REPRESENTATION_ITEM()
RATIONAL_B_SPLINE_CURVE((1.30231782317066,1.50378709164507,1.30231782317066))
REPRESENTATION_ITEM('')
);
#1737=(
BOUNDED_CURVE()
B_SPLINE_CURVE(2,(#115660,#115661,#115662),.UNSPECIFIED.,.F.,.F.)
B_SPLINE_CURVE_WITH_KNOTS((3,3),(0.413328514094884,1.23975190893748),
 .UNSPECIFIED.)
CURVE()
GEOMETRIC_REPRESENTATION_ITEM()
RATIONAL_B_SPLINE_CURVE((1.30231782317066,1.50378709164505,1.30231782317065))
REPRESENTATION_ITEM('')
);
#1738=(
BOUNDED_CURVE()
B_SPLINE_CURVE(3,(#116718,#116719,#116720,#116721,#116722,#116723,#116724,
#116725,#116726),.UNSPECIFIED.,.F.,.F.)
B_SPLINE_CURVE_WITH_KNOTS((4,1,1,1,1,1,4),(0.498245638802688,0.561105453430608,
0.658744313843059,0.756748145426417,0.857662812773838,0.964062246408474,
1.),.UNSPECIFIED.)
CURVE()
GEOMETRIC_REPRESENTATION_ITEM()
RATIONAL_B_SPLINE_CURVE((1.1080784066728,1.1080784066728,1.1080784066728,
1.1080784066728,1.1080784066728,1.1080784066728,1.1080784066728,1.1080784066728,
1.1080784066728))
REPRESENTATION_ITEM('')
);
#1739=(
BOUNDED_CURVE()
B_SPLINE_CURVE(2,(#116783,#116784,#116785),.UNSPECIFIED.,.F.,.F.)
B_SPLINE_CURVE_WITH_KNOTS((3,3),(-1.23975190889132,-0.413328514141037),
 .UNSPECIFIED.)
CURVE()
GEOMETRIC_REPRESENTATION_ITEM()
RATIONAL_B_SPLINE_CURVE((1.30231782319316,1.50378709162254,1.30231782319316))
REPRESENTATION_ITEM('')
);
#1740=(
BOUNDED_CURVE()
B_SPLINE_CURVE(2,(#116787,#116788,#116789),.UNSPECIFIED.,.F.,.F.)
B_SPLINE_CURVE_WITH_KNOTS((3,3),(-1.23975190893749,-0.413328514094873),
 .UNSPECIFIED.)
CURVE()
GEOMETRIC_REPRESENTATION_ITEM()
RATIONAL_B_SPLINE_CURVE((1.30231782317066,1.50378709164507,1.30231782317066))
REPRESENTATION_ITEM('')
);
#1741=(
BOUNDED_CURVE()
B_SPLINE_CURVE(2,(#116791,#116792,#116793),.UNSPECIFIED.,.F.,.F.)
B_SPLINE_CURVE_WITH_KNOTS((3,3),(-1.23975190893748,-0.413328514094879),
 .UNSPECIFIED.)
CURVE()
GEOMETRIC_REPRESENTATION_ITEM()
RATIONAL_B_SPLINE_CURVE((1.30231782317065,1.50378709164505,1.30231782317066))
REPRESENTATION_ITEM('')
);
#1742=(
BOUNDED_CURVE()
B_SPLINE_CURVE(2,(#116795,#116796,#116797),.UNSPECIFIED.,.F.,.F.)
B_SPLINE_CURVE_WITH_KNOTS((3,3),(0.413328514141045,0.826540211516179),
 .UNSPECIFIED.)
CURVE()
GEOMETRIC_REPRESENTATION_ITEM()
RATIONAL_B_SPLINE_CURVE((1.30231782319316,1.40305245740785,1.40305245740785))
REPRESENTATION_ITEM('')
);
#1743=(
BOUNDED_CURVE()
B_SPLINE_CURVE(2,(#116800,#116801,#116802),.UNSPECIFIED.,.F.,.F.)
B_SPLINE_CURVE_WITH_KNOTS((3,3),(0.826540211516179,1.23975190889132),
 .UNSPECIFIED.)
CURVE()
GEOMETRIC_REPRESENTATION_ITEM()
RATIONAL_B_SPLINE_CURVE((1.40305245740785,1.40305245740785,1.30231782319316))
REPRESENTATION_ITEM('')
);
#1744=(
BOUNDED_CURVE()
B_SPLINE_CURVE(2,(#116804,#116805,#116806),.UNSPECIFIED.,.F.,.F.)
B_SPLINE_CURVE_WITH_KNOTS((3,3),(0.41332851409488,1.23975190893749),
 .UNSPECIFIED.)
CURVE()
GEOMETRIC_REPRESENTATION_ITEM()
RATIONAL_B_SPLINE_CURVE((1.30231782317066,1.50378709164506,1.30231782317066))
REPRESENTATION_ITEM('')
);
#1745=(
BOUNDED_CURVE()
B_SPLINE_CURVE(2,(#116807,#116808,#116809),.UNSPECIFIED.,.F.,.F.)
B_SPLINE_CURVE_WITH_KNOTS((3,3),(0.413328514094886,1.23975190893748),
 .UNSPECIFIED.)
CURVE()
GEOMETRIC_REPRESENTATION_ITEM()
RATIONAL_B_SPLINE_CURVE((1.30231782317066,1.50378709164505,1.30231782317066))
REPRESENTATION_ITEM('')
);
#1746=(
BOUNDED_CURVE()
B_SPLINE_CURVE(3,(#117409,#117410,#117411,#117412,#117413,#117414,#117415,
#117416,#117417),.UNSPECIFIED.,.F.,.F.)
B_SPLINE_CURVE_WITH_KNOTS((4,1,1,1,1,1,4),(0.,0.135223490006101,0.368372760690441,
0.577807692760591,0.764911637581468,0.932796326685917,1.),.UNSPECIFIED.)
CURVE()
GEOMETRIC_REPRESENTATION_ITEM()
RATIONAL_B_SPLINE_CURVE((1.17156684956244,1.17156684956244,1.17156684956244,
1.17156684956244,1.17156684956244,1.17156684956244,1.17156684956244,1.17156684956244,
1.17156684956244))
REPRESENTATION_ITEM('')
);
#1747=(
BOUNDED_CURVE()
B_SPLINE_CURVE(3,(#117607,#117608,#117609,#117610,#117611,#117612,#117613),
 .UNSPECIFIED.,.F.,.F.)
B_SPLINE_CURVE_WITH_KNOTS((4,1,1,1,4),(0.,0.291641690547774,0.569344832932309,
0.824487948659488,0.999999966448407),.UNSPECIFIED.)
CURVE()
GEOMETRIC_REPRESENTATION_ITEM()
RATIONAL_B_SPLINE_CURVE((1.14438518125604,1.14438518125604,1.14438518125604,
1.14438518125604,1.14438518125604,1.14438518125604,1.14438518125604))
REPRESENTATION_ITEM('')
);
#1748=(
BOUNDED_CURVE()
B_SPLINE_CURVE(3,(#118540,#118541,#118542,#118543),.UNSPECIFIED.,.F.,.F.)
B_SPLINE_CURVE_WITH_KNOTS((4,4),(0.,1.),.UNSPECIFIED.)
CURVE()
GEOMETRIC_REPRESENTATION_ITEM()
RATIONAL_B_SPLINE_CURVE((1.02979156448796,0.990068747199373,0.990069478517477,
1.02979375844227))
REPRESENTATION_ITEM('')
);
#1749=(
BOUNDED_CURVE()
B_SPLINE_CURVE(3,(#120387,#120388,#120389,#120390),.UNSPECIFIED.,.F.,.F.)
B_SPLINE_CURVE_WITH_KNOTS((4,4),(0.,1.),.UNSPECIFIED.)
CURVE()
GEOMETRIC_REPRESENTATION_ITEM()
RATIONAL_B_SPLINE_CURVE((1.0350339969107,0.988321903155915,0.988322001030004,
1.03503429053297))
REPRESENTATION_ITEM('')
);
#1750=(
BOUNDED_CURVE()
B_SPLINE_CURVE(3,(#125894,#125895,#125896,#125897),.UNSPECIFIED.,.F.,.F.)
B_SPLINE_CURVE_WITH_KNOTS((4,4),(0.,1.),.UNSPECIFIED.)
CURVE()
GEOMETRIC_REPRESENTATION_ITEM()
RATIONAL_B_SPLINE_CURVE((1.1194923501161,1.03775180012471,0.997948145087754,
1.00008138500524))
REPRESENTATION_ITEM('')
);
#1751=(
BOUNDED_CURVE()
B_SPLINE_CURVE(3,(#125956,#125957,#125958,#125959,#125960,#125961),
 .UNSPECIFIED.,.F.,.F.)
B_SPLINE_CURVE_WITH_KNOTS((4,1,1,4),(0.,0.0439726678853666,0.554904538801605,
1.),.UNSPECIFIED.)
CURVE()
GEOMETRIC_REPRESENTATION_ITEM()
RATIONAL_B_SPLINE_CURVE((1.11949037511337,1.11949037511337,1.11949037511337,
1.11949037511337,1.11949037511337,1.11949037511337))
REPRESENTATION_ITEM('')
);
#1752=(
BOUNDED_CURVE()
B_SPLINE_CURVE(3,(#126614,#126615,#126616,#126617),.UNSPECIFIED.,.F.,.F.)
B_SPLINE_CURVE_WITH_KNOTS((4,4),(0.,0.999999993839391),.UNSPECIFIED.)
CURVE()
GEOMETRIC_REPRESENTATION_ITEM()
RATIONAL_B_SPLINE_CURVE((1.03503360228858,0.988322081496627,0.988322132570662,
1.03503375551068))
REPRESENTATION_ITEM('')
);
#1753=(
BOUNDED_CURVE()
B_SPLINE_CURVE(3,(#126731,#126732,#126733,#126734),.UNSPECIFIED.,.F.,.F.)
B_SPLINE_CURVE_WITH_KNOTS((4,4),(0.,1.),.UNSPECIFIED.)
CURVE()
GEOMETRIC_REPRESENTATION_ITEM()
RATIONAL_B_SPLINE_CURVE((1.03503398156237,0.988321878442041,0.988322006146192,
1.03503436467482))
REPRESENTATION_ITEM('')
);
#1754=(
BOUNDED_CURVE()
B_SPLINE_CURVE(3,(#131531,#131532,#131533,#131534),.UNSPECIFIED.,.F.,.F.)
B_SPLINE_CURVE_WITH_KNOTS((4,4),(2.53618980579517E-5,1.),.UNSPECIFIED.)
CURVE()
GEOMETRIC_REPRESENTATION_ITEM()
RATIONAL_B_SPLINE_CURVE((1.00144258776943,0.992211728886904,1.02728082050576,
1.10664986262599))
REPRESENTATION_ITEM('')
);
#1755=(
BOUNDED_CURVE()
B_SPLINE_CURVE(3,(#131667,#131668,#131669,#131670),.UNSPECIFIED.,.F.,.F.)
B_SPLINE_CURVE_WITH_KNOTS((4,4),(0.,0.99998151481627),.UNSPECIFIED.)
CURVE()
GEOMETRIC_REPRESENTATION_ITEM()
RATIONAL_B_SPLINE_CURVE((1.10666105100836,1.05697038096492,1.02464192514604,
1.00967568355171))
REPRESENTATION_ITEM('')
);
#1756=(
BOUNDED_CURVE()
B_SPLINE_CURVE(3,(#135216,#135217,#135218,#135219),.UNSPECIFIED.,.F.,.F.)
B_SPLINE_CURVE_WITH_KNOTS((4,4),(0.,1.),.UNSPECIFIED.)
CURVE()
GEOMETRIC_REPRESENTATION_ITEM()
RATIONAL_B_SPLINE_CURVE((1.1715918217896,0.942817810547867,0.942802727064813,
1.17154657134044))
REPRESENTATION_ITEM('')
);
#1757=(
BOUNDED_CURVE()
B_SPLINE_CURVE(3,(#139977,#139978,#139979,#139980),.UNSPECIFIED.,.F.,.F.)
B_SPLINE_CURVE_WITH_KNOTS((4,4),(0.,1.),.UNSPECIFIED.)
CURVE()
GEOMETRIC_REPRESENTATION_ITEM()
RATIONAL_B_SPLINE_CURVE((1.1728399592297,0.86224977517439,0.970253168357341,
1.49685013877855))
REPRESENTATION_ITEM('')
);
#1758=(
BOUNDED_CURVE()
B_SPLINE_CURVE(3,(#145857,#145858,#145859,#145860,#145861,#145862,#145863,
#145864,#145865,#145866,#145867,#145868,#145869),.UNSPECIFIED.,.F.,.F.)
B_SPLINE_CURVE_WITH_KNOTS((4,1,1,1,1,1,1,1,1,1,4),(0.,0.0361770017020252,
0.110322638446908,0.191341394631034,0.279299595253617,0.374729923390192,
0.478819817310066,0.592531700959653,0.717431194571663,0.855542845896087,
1.),.UNSPECIFIED.)
CURVE()
GEOMETRIC_REPRESENTATION_ITEM()
RATIONAL_B_SPLINE_CURVE((1.17157173846247,1.17157173846247,1.17157173846247,
1.17157173846247,1.17157173846247,1.17157173846247,1.17157173846247,1.17157173846247,
1.17157173846247,1.17157173846247,1.17157173846247,1.17157173846247,1.17157173846247))
REPRESENTATION_ITEM('')
);
#1759=(
BOUNDED_CURVE()
B_SPLINE_CURVE(3,(#146006,#146007,#146008,#146009),.UNSPECIFIED.,.F.,.F.)
B_SPLINE_CURVE_WITH_KNOTS((4,4),(0.,0.999997706678458),.UNSPECIFIED.)
CURVE()
GEOMETRIC_REPRESENTATION_ITEM()
RATIONAL_B_SPLINE_CURVE((1.17153882871445,0.942808335086217,0.942820391063934,
1.1715749966476))
REPRESENTATION_ITEM('')
);
#1760=(
BOUNDED_CURVE()
B_SPLINE_CURVE(3,(#146190,#146191,#146192,#146193),.UNSPECIFIED.,.F.,.F.)
B_SPLINE_CURVE_WITH_KNOTS((4,4),(0.,1.),.UNSPECIFIED.)
CURVE()
GEOMETRIC_REPRESENTATION_ITEM()
RATIONAL_B_SPLINE_CURVE((1.07476116149506,0.975082344906196,0.975079612909692,
1.07475296550555))
REPRESENTATION_ITEM('')
);
#1761=(
BOUNDED_CURVE()
B_SPLINE_CURVE(3,(#148249,#148250,#148251,#148252),.UNSPECIFIED.,.F.,.F.)
B_SPLINE_CURVE_WITH_KNOTS((4,4),(0.,1.),.UNSPECIFIED.)
CURVE()
GEOMETRIC_REPRESENTATION_ITEM()
RATIONAL_B_SPLINE_CURVE((1.06562254279167,0.920748224239219,1.01575223807641,
1.35063458430324))
REPRESENTATION_ITEM('')
);
#1762=(
BOUNDED_CURVE()
B_SPLINE_CURVE(3,(#155076,#155077,#155078,#155079),.UNSPECIFIED.,.F.,.F.)
B_SPLINE_CURVE_WITH_KNOTS((4,4),(0.,1.),.UNSPECIFIED.)
CURVE()
GEOMETRIC_REPRESENTATION_ITEM()
RATIONAL_B_SPLINE_CURVE((1.00307588690503,1.01543948096341,1.06507487566662,
1.15198207101464))
REPRESENTATION_ITEM('')
);
#1763=(
BOUNDED_CURVE()
B_SPLINE_CURVE(3,(#155449,#155450,#155451,#155452),.UNSPECIFIED.,.F.,.F.)
B_SPLINE_CURVE_WITH_KNOTS((4,4),(0.,1.),.UNSPECIFIED.)
CURVE()
GEOMETRIC_REPRESENTATION_ITEM()
RATIONAL_B_SPLINE_CURVE((1.02461141564327,0.991255872256879,0.991805091524064,
1.02625907344483))
REPRESENTATION_ITEM('')
);
#1764=(
BOUNDED_CURVE()
B_SPLINE_CURVE(3,(#156152,#156153,#156154,#156155),.UNSPECIFIED.,.F.,.F.)
B_SPLINE_CURVE_WITH_KNOTS((4,4),(1.38694351006516E-5,1.),.UNSPECIFIED.)
CURVE()
GEOMETRIC_REPRESENTATION_ITEM()
RATIONAL_B_SPLINE_CURVE((1.12701103586907,0.957656401969315,0.957662988299714,
1.12703079486027))
REPRESENTATION_ITEM('')
);
#1765=(
BOUNDED_CURVE()
B_SPLINE_CURVE(3,(#156811,#156812,#156813,#156814,#156815,#156816,#156817,
#156818,#156819,#156820),.UNSPECIFIED.,.F.,.F.)
B_SPLINE_CURVE_WITH_KNOTS((4,1,1,1,1,1,1,4),(0.,0.137093559948487,0.289586259168106,
0.458249167268145,0.635927168939495,0.81211997438687,0.983002488738192,
0.999999802202788),.UNSPECIFIED.)
CURVE()
GEOMETRIC_REPRESENTATION_ITEM()
RATIONAL_B_SPLINE_CURVE((1.17111220952591,1.17111220952591,1.17111220952591,
1.17111220952591,1.17111220952591,1.17111220952591,1.17111220952591,1.17111220952591,
1.17111220952591,1.17111220952591))
REPRESENTATION_ITEM('')
);
#1806=TOROIDAL_SURFACE('',#79562,11.,0.5);
#1807=TOROIDAL_SURFACE('',#79569,11.75,0.5);
#1808=TOROIDAL_SURFACE('',#79572,10.5,0.5);
#1809=TOROIDAL_SURFACE('',#79582,10.5,0.5);
#1810=TOROIDAL_SURFACE('',#79596,8.25,0.5);
#1811=TOROIDAL_SURFACE('',#79627,7.,0.5);
#1812=TOROIDAL_SURFACE('',#79657,10.,0.5);
#1813=TOROIDAL_SURFACE('',#79691,10.,0.5);
#1814=TOROIDAL_SURFACE('',#79762,26.,1.5);
#1815=TOROIDAL_SURFACE('',#79767,7.,1.5);
#1816=TOROIDAL_SURFACE('',#79770,26.,1.5);
#1817=TOROIDAL_SURFACE('',#79776,66.,1.5);
#1818=TOROIDAL_SURFACE('',#79792,4.,1.5);
#1819=TOROIDAL_SURFACE('',#79796,4.,1.5);
#1820=TOROIDAL_SURFACE('',#79803,4.,1.5);
#1821=TOROIDAL_SURFACE('',#79808,4.,1.5);
#1822=TOROIDAL_SURFACE('',#79811,36.,1.5);
#1823=TOROIDAL_SURFACE('',#79813,36.,1.5);
#1824=TOROIDAL_SURFACE('',#79817,36.,1.5);
#1825=TOROIDAL_SURFACE('',#79885,66.,1.5);
#1826=TOROIDAL_SURFACE('',#79890,26.,1.5);
#1827=TOROIDAL_SURFACE('',#79895,7.,1.5);
#1828=TOROIDAL_SURFACE('',#79898,26.,1.5);
#1829=TOROIDAL_SURFACE('',#79903,4.,1.5);
#1830=TOROIDAL_SURFACE('',#79906,36.,1.5);
#1831=TOROIDAL_SURFACE('',#79908,36.,1.5);
#1832=TOROIDAL_SURFACE('',#79910,4.,1.5);
#1833=TOROIDAL_SURFACE('',#79914,4.,1.5);
#1834=TOROIDAL_SURFACE('',#79921,4.,1.5);
#1835=TOROIDAL_SURFACE('',#79928,36.,1.5);
#1836=TOROIDAL_SURFACE('',#80002,36.5,1.);
#1837=TOROIDAL_SURFACE('',#80005,66.5,1.);
#1838=TOROIDAL_SURFACE('',#80008,4.5,1.);
#1839=TOROIDAL_SURFACE('',#80012,4.5,1.);
#1840=TOROIDAL_SURFACE('',#80022,14.,1.5);
#1841=TOROIDAL_SURFACE('',#80027,14.,1.5);
#1842=TOROIDAL_SURFACE('',#80031,8.016437378118,1.5);
#1843=TOROIDAL_SURFACE('',#80089,4.498378496899,1.);
#1844=TOROIDAL_SURFACE('',#80091,14.5,1.);
#1845=TOROIDAL_SURFACE('',#80097,14.5,1.);
#1846=TOROIDAL_SURFACE('',#80104,14.5,1.);
#1847=TOROIDAL_SURFACE('',#80111,14.5,1.);
#1848=TOROIDAL_SURFACE('',#80114,4.498378496898,1.);
#1849=TOROIDAL_SURFACE('',#80131,26.64683059909,1.);
#1850=TOROIDAL_SURFACE('',#80154,10.5,1.);
#1851=TOROIDAL_SURFACE('',#80169,10.5,1.);
#1852=TOROIDAL_SURFACE('',#80170,10.55051025722,1.);
#1853=TOROIDAL_SURFACE('',#80173,2.449489742783,1.);
#1854=TOROIDAL_SURFACE('',#80182,2.449489742783,1.);
#1855=TOROIDAL_SURFACE('',#80184,10.55051025722,1.);
#1856=TOROIDAL_SURFACE('',#80186,13.,1.5);
#1857=TOROIDAL_SURFACE('',#80197,3.998378496899,1.5);
#1858=TOROIDAL_SURFACE('',#80227,39.5,0.5);
#1859=TOROIDAL_SURFACE('',#80239,39.5,0.5);
#1860=TOROIDAL_SURFACE('',#80264,7.5,0.5);
#1861=TOROIDAL_SURFACE('',#80267,29.5,0.5);
#1862=TOROIDAL_SURFACE('',#80270,29.5,0.5);
#1863=TOROIDAL_SURFACE('',#80276,7.5,0.5);
#1864=TOROIDAL_SURFACE('',#80284,29.5,0.5);
#1865=TOROIDAL_SURFACE('',#80287,29.5,0.5);
#1866=TOROIDAL_SURFACE('',#80290,7.5,0.5);
#1867=TOROIDAL_SURFACE('',#80294,7.5,0.5);
#1868=TOROIDAL_SURFACE('',#80326,3.998378496898,1.5);
#1869=TOROIDAL_SURFACE('',#80333,13.,1.5);
#1870=TOROIDAL_SURFACE('',#80345,3.,1.5);
#1871=TOROIDAL_SURFACE('',#80355,3.,1.5);
#1872=TOROIDAL_SURFACE('',#80359,36.5,1.);
#1873=TOROIDAL_SURFACE('',#80360,66.5,1.);
#1874=TOROIDAL_SURFACE('',#80367,14.,1.5);
#1875=TOROIDAL_SURFACE('',#80370,14.,1.5);
#1876=TOROIDAL_SURFACE('',#80371,26.6468278765,1.);
#1877=TOROIDAL_SURFACE('',#80375,8.,1.5);
#1910=CONICAL_SURFACE('',#79555,9.799780026165,0.785375619840672);
#1911=CONICAL_SURFACE('',#79616,13.79977495601,0.785381825805275);
#1912=CONICAL_SURFACE('',#79634,5.799851372624,0.785372339464152);
#1913=CONICAL_SURFACE('',#79652,16.375,0.21711131448682);
#1914=CONICAL_SURFACE('',#79653,17.175,0.7853981625);
#1915=CONICAL_SURFACE('',#79664,8.699805279292,0.785376526397671);
#1916=CONICAL_SURFACE('',#79681,11.25,0.7853981625);
#1917=CONICAL_SURFACE('',#79688,7.75000000000001,1.04719755);
#1918=CONICAL_SURFACE('',#79689,7.95,0.7853981625);
#1919=CONICAL_SURFACE('',#79698,8.699805279292,0.785376526397671);
#1920=CONICAL_SURFACE('',#79716,11.25,0.7853981625);
#1921=CONICAL_SURFACE('',#79723,7.75000000000001,1.04719755);
#1922=CONICAL_SURFACE('',#79724,7.95,0.7853981625);
#1923=CONICAL_SURFACE('',#80315,9.79989529474,0.785387399312301);
#1975=ORIENTED_CLOSED_SHELL('',*,#79318,.F.);
#1976=ORIENTED_CLOSED_SHELL('',*,#79319,.F.);
#1977=ORIENTED_CLOSED_SHELL('',*,#79320,.F.);
#1978=ORIENTED_CLOSED_SHELL('',*,#79321,.F.);
#1980=CYLINDRICAL_SURFACE('',#79490,1.5);
#1981=CYLINDRICAL_SURFACE('',#79491,20.5);
#1982=CYLINDRICAL_SURFACE('',#79498,1.5);
#1983=CYLINDRICAL_SURFACE('',#79499,20.5);
#1984=CYLINDRICAL_SURFACE('',#79500,20.5);
#1985=CYLINDRICAL_SURFACE('',#79503,1.5);
#1986=CYLINDRICAL_SURFACE('',#79507,20.5);
#1987=CYLINDRICAL_SURFACE('',#79512,1.5);
#1988=CYLINDRICAL_SURFACE('',#79515,8.4);
#1989=CYLINDRICAL_SURFACE('',#79517,8.4);
#1990=CYLINDRICAL_SURFACE('',#79518,8.4);
#1991=CYLINDRICAL_SURFACE('',#79519,8.4);
#1992=CYLINDRICAL_SURFACE('',#79521,8.4);
#1993=CYLINDRICAL_SURFACE('',#79522,8.4);
#1994=CYLINDRICAL_SURFACE('',#79524,17.);
#1995=CYLINDRICAL_SURFACE('',#79525,17.);
#1996=CYLINDRICAL_SURFACE('',#79526,17.);
#1997=CYLINDRICAL_SURFACE('',#79527,17.);
#1998=CYLINDRICAL_SURFACE('',#79528,17.);
#1999=CYLINDRICAL_SURFACE('',#79530,16.375);
#2000=CYLINDRICAL_SURFACE('',#79533,16.375);
#2001=CYLINDRICAL_SURFACE('',#79534,16.375);
#2002=CYLINDRICAL_SURFACE('',#79539,20.5);
#2003=CYLINDRICAL_SURFACE('',#79549,11.);
#2004=CYLINDRICAL_SURFACE('',#79558,10.5);
#2005=CYLINDRICAL_SURFACE('',#79565,11.25);
#2006=CYLINDRICAL_SURFACE('',#79577,11.);
#2007=CYLINDRICAL_SURFACE('',#79578,21.);
#2008=CYLINDRICAL_SURFACE('',#79586,40.);
#2009=CYLINDRICAL_SURFACE('',#79593,9.500000000001);
#2010=CYLINDRICAL_SURFACE('',#79601,7.75);
#2011=CYLINDRICAL_SURFACE('',#79603,6.5);
#2012=CYLINDRICAL_SURFACE('',#79607,9.5);
#2013=CYLINDRICAL_SURFACE('',#79612,13.5);
#2014=CYLINDRICAL_SURFACE('',#79618,14.5);
#2015=CYLINDRICAL_SURFACE('',#79621,7.25);
#2016=CYLINDRICAL_SURFACE('',#79632,6.5);
#2017=CYLINDRICAL_SURFACE('',#79638,5.5);
#2018=CYLINDRICAL_SURFACE('',#79641,9.50000000000001);
#2019=CYLINDRICAL_SURFACE('',#79644,37.5);
#2020=CYLINDRICAL_SURFACE('',#79647,16.375);
#2021=CYLINDRICAL_SURFACE('',#79648,16.);
#2022=CYLINDRICAL_SURFACE('',#79656,17.);
#2023=CYLINDRICAL_SURFACE('',#79662,9.49999999999999);
#2024=CYLINDRICAL_SURFACE('',#79666,8.4);
#2025=CYLINDRICAL_SURFACE('',#79667,12.);
#2026=CYLINDRICAL_SURFACE('',#79669,37.5);
#2027=CYLINDRICAL_SURFACE('',#79672,8.5);
#2028=CYLINDRICAL_SURFACE('',#79674,10.25);
#2029=CYLINDRICAL_SURFACE('',#79677,11.75);
#2030=CYLINDRICAL_SURFACE('',#79683,7.75000000000001);
#2031=CYLINDRICAL_SURFACE('',#79696,9.49999999999999);
#2032=CYLINDRICAL_SURFACE('',#79700,8.4);
#2033=CYLINDRICAL_SURFACE('',#79702,12.);
#2034=CYLINDRICAL_SURFACE('',#79704,37.5);
#2035=CYLINDRICAL_SURFACE('',#79707,8.5);
#2036=CYLINDRICAL_SURFACE('',#79709,10.25);
#2037=CYLINDRICAL_SURFACE('',#79712,11.75);
#2038=CYLINDRICAL_SURFACE('',#79718,7.75000000000001);
#2039=CYLINDRICAL_SURFACE('',#79735,1.5);
#2040=CYLINDRICAL_SURFACE('',#79740,18.5);
#2041=CYLINDRICAL_SURFACE('',#79748,0.999999999999999);
#2042=CYLINDRICAL_SURFACE('',#79753,1.5);
#2043=CYLINDRICAL_SURFACE('',#79755,20.5);
#2044=CYLINDRICAL_SURFACE('',#79757,0.999999999999999);
#2045=CYLINDRICAL_SURFACE('',#79775,1.5);
#2046=CYLINDRICAL_SURFACE('',#79795,27.5);
#2047=CYLINDRICAL_SURFACE('',#79806,27.5);
#2048=CYLINDRICAL_SURFACE('',#79807,67.5);
#2049=CYLINDRICAL_SURFACE('',#79812,1.5);
#2050=CYLINDRICAL_SURFACE('',#79814,5.5);
#2051=CYLINDRICAL_SURFACE('',#79815,37.5);
#2052=CYLINDRICAL_SURFACE('',#79819,37.5);
#2053=CYLINDRICAL_SURFACE('',#79820,5.5);
#2054=CYLINDRICAL_SURFACE('',#79844,1.5);
#2055=CYLINDRICAL_SURFACE('',#79848,1.);
#2056=CYLINDRICAL_SURFACE('',#79851,0.999999999999999);
#2057=CYLINDRICAL_SURFACE('',#79853,1.5);
#2058=CYLINDRICAL_SURFACE('',#79861,18.5);
#2059=CYLINDRICAL_SURFACE('',#79865,20.5);
#2060=CYLINDRICAL_SURFACE('',#79888,1.5);
#2061=CYLINDRICAL_SURFACE('',#79902,27.5);
#2062=CYLINDRICAL_SURFACE('',#79907,1.5);
#2063=CYLINDRICAL_SURFACE('',#79912,67.5);
#2064=CYLINDRICAL_SURFACE('',#79913,27.5);
#2065=CYLINDRICAL_SURFACE('',#79924,5.5);
#2066=CYLINDRICAL_SURFACE('',#79925,5.5);
#2067=CYLINDRICAL_SURFACE('',#79926,37.5);
#2068=CYLINDRICAL_SURFACE('',#79930,37.5);
#2069=CYLINDRICAL_SURFACE('',#79963,1.5);
#2070=CYLINDRICAL_SURFACE('',#79968,15.5);
#2071=CYLINDRICAL_SURFACE('',#79971,15.5);
#2072=CYLINDRICAL_SURFACE('',#79974,5.498378496899);
#2073=CYLINDRICAL_SURFACE('',#79976,5.498378496898);
#2074=CYLINDRICAL_SURFACE('',#79979,1.);
#2075=CYLINDRICAL_SURFACE('',#79981,1.);
#2076=CYLINDRICAL_SURFACE('',#79985,1.5);
#2077=CYLINDRICAL_SURFACE('',#79986,1.5);
#2078=CYLINDRICAL_SURFACE('',#80010,5.5);
#2079=CYLINDRICAL_SURFACE('',#80018,1.5);
#2080=CYLINDRICAL_SURFACE('',#80024,15.5);
#2081=CYLINDRICAL_SURFACE('',#80035,9.51643737811801);
#2082=CYLINDRICAL_SURFACE('',#80039,9.51643737811801);
#2083=CYLINDRICAL_SURFACE('',#80049,12.);
#2084=CYLINDRICAL_SURFACE('',#80053,12.);
#2085=CYLINDRICAL_SURFACE('',#80057,18.);
#2086=CYLINDRICAL_SURFACE('',#80062,18.);
#2087=CYLINDRICAL_SURFACE('',#80064,8.);
#2088=CYLINDRICAL_SURFACE('',#80066,8.);
#2089=CYLINDRICAL_SURFACE('',#80079,1.5);
#2090=CYLINDRICAL_SURFACE('',#80082,15.5);
#2091=CYLINDRICAL_SURFACE('',#80087,5.498378496899);
#2092=CYLINDRICAL_SURFACE('',#80094,0.999999999999999);
#2093=CYLINDRICAL_SURFACE('',#80100,0.999999999999999);
#2094=CYLINDRICAL_SURFACE('',#80101,1.5);
#2095=CYLINDRICAL_SURFACE('',#80108,0.999999999999999);
#2096=CYLINDRICAL_SURFACE('',#80116,5.498378496898);
#2097=CYLINDRICAL_SURFACE('',#80117,27.6468278765);
#2098=CYLINDRICAL_SURFACE('',#80122,27.64683059909);
#2099=CYLINDRICAL_SURFACE('',#80135,1.5);
#2100=CYLINDRICAL_SURFACE('',#80137,1.5);
#2101=CYLINDRICAL_SURFACE('',#80142,1.5);
#2102=CYLINDRICAL_SURFACE('',#80143,9.500000000001);
#2103=CYLINDRICAL_SURFACE('',#80159,11.5);
#2104=CYLINDRICAL_SURFACE('',#80160,11.5);
#2105=CYLINDRICAL_SURFACE('',#80162,1.);
#2106=CYLINDRICAL_SURFACE('',#80165,1.);
#2107=CYLINDRICAL_SURFACE('',#80174,1.5);
#2108=CYLINDRICAL_SURFACE('',#80176,1.);
#2109=CYLINDRICAL_SURFACE('',#80188,1.5);
#2110=CYLINDRICAL_SURFACE('',#80192,1.5);
#2111=CYLINDRICAL_SURFACE('',#80202,27.49622463646);
#2112=CYLINDRICAL_SURFACE('',#80205,1.5);
#2113=CYLINDRICAL_SURFACE('',#80206,18.5);
#2114=CYLINDRICAL_SURFACE('',#80207,18.5);
#2115=CYLINDRICAL_SURFACE('',#80219,15.);
#2116=CYLINDRICAL_SURFACE('',#80223,15.);
#2117=CYLINDRICAL_SURFACE('',#80233,40.);
#2118=CYLINDRICAL_SURFACE('',#80234,8.);
#2119=CYLINDRICAL_SURFACE('',#80237,40.);
#2120=CYLINDRICAL_SURFACE('',#80244,40.);
#2121=CYLINDRICAL_SURFACE('',#80245,8.);
#2122=CYLINDRICAL_SURFACE('',#80261,15.);
#2123=CYLINDRICAL_SURFACE('',#80262,15.);
#2124=CYLINDRICAL_SURFACE('',#80263,40.);
#2125=CYLINDRICAL_SURFACE('',#80277,30.);
#2126=CYLINDRICAL_SURFACE('',#80279,30.);
#2127=CYLINDRICAL_SURFACE('',#80281,30.);
#2128=CYLINDRICAL_SURFACE('',#80297,30.);
#2129=CYLINDRICAL_SURFACE('',#80301,30.);
#2130=CYLINDRICAL_SURFACE('',#80304,30.);
#2131=CYLINDRICAL_SURFACE('',#80310,13.);
#2132=CYLINDRICAL_SURFACE('',#80311,13.);
#2133=CYLINDRICAL_SURFACE('',#80316,1.5);
#2134=CYLINDRICAL_SURFACE('',#80331,1.5);
#2135=CYLINDRICAL_SURFACE('',#80332,1.5);
#2136=CYLINDRICAL_SURFACE('',#80334,1.5);
#2137=CYLINDRICAL_SURFACE('',#80340,1.5);
#2138=CYLINDRICAL_SURFACE('',#80341,70.);
#2139=CYLINDRICAL_SURFACE('',#80342,30.);
#2140=CYLINDRICAL_SURFACE('',#80343,1.5);
#2141=CYLINDRICAL_SURFACE('',#80347,67.5);
#2142=CYLINDRICAL_SURFACE('',#80349,1.5);
#2143=CYLINDRICAL_SURFACE('',#80352,1.5);
#2144=CYLINDRICAL_SURFACE('',#80357,1.5);
#2145=CYLINDRICAL_SURFACE('',#80361,1.5);
#2146=CYLINDRICAL_SURFACE('',#80368,1.5);
#2147=CYLINDRICAL_SURFACE('',#80369,1.5);
#2148=CYLINDRICAL_SURFACE('',#80373,0.999999999999999);
#2149=CYLINDRICAL_SURFACE('',#80378,20.5);
#2389=(
BOUNDED_SURFACE()
B_SPLINE_SURFACE(3,3,((#106617,#106618,#106619,#106620,#106621,#106622,
#106623,#106624,#106625),(#106626,#106627,#106628,#106629,#106630,#106631,
#106632,#106633,#106634),(#106635,#106636,#106637,#106638,#106639,#106640,
#106641,#106642,#106643),(#106644,#106645,#106646,#106647,#106648,#106649,
#106650,#106651,#106652)),.UNSPECIFIED.,.F.,.F.,.F.)
B_SPLINE_SURFACE_WITH_KNOTS((4,4),(4,1,1,1,1,1,4),(0.,1.),(0.,0.170731713964461,
0.369331369271742,0.571283666971615,0.772321449964879,0.980780822111612,
1.),.UNSPECIFIED.)
GEOMETRIC_REPRESENTATION_ITEM()
RATIONAL_B_SPLINE_SURFACE(((1.469253866242,1.469253866242,1.469253866242,
1.469253866242,1.469253866242,1.469253866242,1.469253866242,1.469253866242,
1.469253866242),(0.843582044586,0.843582044586,0.843582044586,0.843582044586,
0.843582044586,0.843582044586,0.843582044586,0.843582044586,0.843582044586),
(0.843582044586,0.843582044586,0.843582044586,0.843582044586,0.843582044586,
0.843582044586,0.843582044586,0.843582044586,0.843582044586),(1.469253866242,
1.469253866242,1.469253866242,1.469253866242,1.469253866242,1.469253866242,
1.469253866242,1.469253866242,1.469253866242)))
REPRESENTATION_ITEM('')
SURFACE()
);
#2390=(
BOUNDED_SURFACE()
B_SPLINE_SURFACE(3,3,((#106672,#106673,#106674,#106675,#106676,#106677,
#106678,#106679,#106680,#106681,#106682,#106683,#106684,#106685,#106686,
#106687,#106688,#106689,#106690,#106691),(#106692,#106693,#106694,#106695,
#106696,#106697,#106698,#106699,#106700,#106701,#106702,#106703,#106704,
#106705,#106706,#106707,#106708,#106709,#106710,#106711),(#106712,#106713,
#106714,#106715,#106716,#106717,#106718,#106719,#106720,#106721,#106722,
#106723,#106724,#106725,#106726,#106727,#106728,#106729,#106730,#106731),
(#106732,#106733,#106734,#106735,#106736,#106737,#106738,#106739,#106740,
#106741,#106742,#106743,#106744,#106745,#106746,#106747,#106748,#106749,
#106750,#106751)),.UNSPECIFIED.,.F.,.F.,.F.)
B_SPLINE_SURFACE_WITH_KNOTS((4,4),(4,1,1,1,1,1,1,1,1,1,1,1,1,1,1,1,1,4),
(0.,1.),(0.,0.0396611801962909,0.0991280080993822,0.158967060305227,0.213500355613908,
0.265743805592041,0.31877970559442,0.372320929804579,0.42550049560743,0.477326879186013,
0.531755535132276,0.594383860510548,0.661759309442457,0.728996536779342,
0.791903310438717,0.857857310969531,0.931521029517504,1.),.UNSPECIFIED.)
GEOMETRIC_REPRESENTATION_ITEM()
RATIONAL_B_SPLINE_SURFACE(((1.186027134151,1.186027134151,1.186027134151,
1.186027134151,1.186027134151,1.186027134151,1.186027134151,1.186027134151,
1.186027134151,1.186027134151,1.186027134151,1.186027134151,1.186027134151,
1.186027134151,1.186027134151,1.186027134151,1.186027134151,1.186027134151,
1.186027134151,1.186027134151),(0.9379909552829,0.9379909552829,0.9379909552829,
0.9379909552829,0.9379909552829,0.9379909552829,0.9379909552829,0.9379909552829,
0.9379909552829,0.9379909552829,0.9379909552829,0.9379909552829,0.9379909552829,
0.9379909552829,0.9379909552829,0.9379909552829,0.9379909552829,0.9379909552829,
0.9379909552829,0.9379909552829),(0.9379909552829,0.9379909552829,0.9379909552829,
0.9379909552829,0.9379909552829,0.9379909552829,0.9379909552829,0.9379909552829,
0.9379909552829,0.9379909552829,0.9379909552829,0.9379909552829,0.9379909552829,
0.9379909552829,0.9379909552829,0.9379909552829,0.9379909552829,0.9379909552829,
0.9379909552829,0.9379909552829),(1.186027134151,1.186027134151,1.186027134151,
1.186027134151,1.186027134151,1.186027134151,1.186027134151,1.186027134151,
1.186027134151,1.186027134151,1.186027134151,1.186027134151,1.186027134151,
1.186027134151,1.186027134151,1.186027134151,1.186027134151,1.186027134151,
1.186027134151,1.186027134151)))
REPRESENTATION_ITEM('')
SURFACE()
);
#2391=(
BOUNDED_SURFACE()
B_SPLINE_SURFACE(3,3,((#106769,#106770,#106771,#106772,#106773,#106774,
#106775,#106776,#106777,#106778,#106779,#106780,#106781,#106782,#106783,
#106784,#106785,#106786,#106787,#106788),(#106789,#106790,#106791,#106792,
#106793,#106794,#106795,#106796,#106797,#106798,#106799,#106800,#106801,
#106802,#106803,#106804,#106805,#106806,#106807,#106808),(#106809,#106810,
#106811,#106812,#106813,#106814,#106815,#106816,#106817,#106818,#106819,
#106820,#106821,#106822,#106823,#106824,#106825,#106826,#106827,#106828),
(#106829,#106830,#106831,#106832,#106833,#106834,#106835,#106836,#106837,
#106838,#106839,#106840,#106841,#106842,#106843,#106844,#106845,#106846,
#106847,#106848)),.UNSPECIFIED.,.F.,.F.,.F.)
B_SPLINE_SURFACE_WITH_KNOTS((4,4),(4,1,1,1,1,1,1,1,1,1,1,1,1,1,1,1,1,4),
(0.,1.),(0.,0.0294841287779505,0.0658109628884052,0.105749498424659,0.149530724255755,
0.197388379273207,0.249559161241624,0.306281102763413,0.367810676903299,
0.434427999245631,0.506607662324375,0.585506710794748,0.670705086525465,
0.75370766324414,0.832219267034226,0.905244950763814,0.970572923362877,
1.),.UNSPECIFIED.)
GEOMETRIC_REPRESENTATION_ITEM()
RATIONAL_B_SPLINE_SURFACE(((1.204673293213,1.204673293213,1.204673293213,
1.204673293213,1.204673293213,1.204673293213,1.204673293213,1.204673293213,
1.204673293213,1.204673293213,1.204673293213,1.204673293213,1.204673293213,
1.204673293213,1.204673293213,1.204673293213,1.204673293213,1.204673293213,
1.204673293213,1.204673293213),(0.931775568929,0.931775568929,0.931775568929,
0.931775568929,0.931775568929,0.931775568929,0.931775568929,0.931775568929,
0.931775568929,0.931775568929,0.931775568929,0.931775568929,0.931775568929,
0.931775568929,0.931775568929,0.931775568929,0.931775568929,0.931775568929,
0.931775568929,0.931775568929),(0.931775568929,0.931775568929,0.931775568929,
0.931775568929,0.931775568929,0.931775568929,0.931775568929,0.931775568929,
0.931775568929,0.931775568929,0.931775568929,0.931775568929,0.931775568929,
0.931775568929,0.931775568929,0.931775568929,0.931775568929,0.931775568929,
0.931775568929,0.931775568929),(1.204673293213,1.204673293213,1.204673293213,
1.204673293213,1.204673293213,1.204673293213,1.204673293213,1.204673293213,
1.204673293213,1.204673293213,1.204673293213,1.204673293213,1.204673293213,
1.204673293213,1.204673293213,1.204673293213,1.204673293213,1.204673293213,
1.204673293213,1.204673293213)))
REPRESENTATION_ITEM('')
SURFACE()
);
#2392=(
BOUNDED_SURFACE()
B_SPLINE_SURFACE(3,3,((#106891,#106892,#106893,#106894,#106895,#106896,
#106897,#106898,#106899),(#106900,#106901,#106902,#106903,#106904,#106905,
#106906,#106907,#106908),(#106909,#106910,#106911,#106912,#106913,#106914,
#106915,#106916,#106917),(#106918,#106919,#106920,#106921,#106922,#106923,
#106924,#106925,#106926)),.UNSPECIFIED.,.F.,.F.,.F.)
B_SPLINE_SURFACE_WITH_KNOTS((4,4),(4,1,1,1,1,1,4),(0.,1.),(0.,0.0142463491922952,
0.215979712627769,0.410391612199461,0.611571691500493,0.81768157648455,
1.),.UNSPECIFIED.)
GEOMETRIC_REPRESENTATION_ITEM()
RATIONAL_B_SPLINE_SURFACE(((1.469254032395,1.469254032395,1.469254032395,
1.469254032395,1.469254032395,1.469254032395,1.469254032395,1.469254032395,
1.469254032395),(0.8435819892018,0.8435819892018,0.8435819892018,0.8435819892018,
0.8435819892018,0.8435819892018,0.8435819892018,0.8435819892018,0.8435819892018),
(0.8435819892018,0.8435819892018,0.8435819892018,0.8435819892018,0.8435819892018,
0.8435819892018,0.8435819892018,0.8435819892018,0.8435819892018),(1.469254032395,
1.469254032395,1.469254032395,1.469254032395,1.469254032395,1.469254032395,
1.469254032395,1.469254032395,1.469254032395)))
REPRESENTATION_ITEM('')
SURFACE()
);
#2393=(
BOUNDED_SURFACE()
B_SPLINE_SURFACE(3,3,((#106952,#106953,#106954,#106955,#106956,#106957,
#106958,#106959,#106960,#106961,#106962,#106963,#106964,#106965,#106966,
#106967,#106968,#106969,#106970),(#106971,#106972,#106973,#106974,#106975,
#106976,#106977,#106978,#106979,#106980,#106981,#106982,#106983,#106984,
#106985,#106986,#106987,#106988,#106989),(#106990,#106991,#106992,#106993,
#106994,#106995,#106996,#106997,#106998,#106999,#107000,#107001,#107002,
#107003,#107004,#107005,#107006,#107007,#107008),(#107009,#107010,#107011,
#107012,#107013,#107014,#107015,#107016,#107017,#107018,#107019,#107020,
#107021,#107022,#107023,#107024,#107025,#107026,#107027)),.UNSPECIFIED.,
 .F.,.F.,.F.)
B_SPLINE_SURFACE_WITH_KNOTS((4,4),(4,1,1,1,1,1,1,1,1,1,1,1,1,1,1,1,4),(0.,
1.),(0.,0.036181255324217,0.099722007940329,0.168833416481539,0.243160050304141,
0.324333552794184,0.412835986179286,0.500211138210296,0.582010035481769,
0.656172226852367,0.722805119287517,0.782471486007149,0.835893769847624,
0.883837058018828,0.927058268252567,0.966313597455318,1.),.UNSPECIFIED.)
GEOMETRIC_REPRESENTATION_ITEM()
RATIONAL_B_SPLINE_SURFACE(((1.204709660399,1.204709660399,1.204709660399,
1.204709660399,1.204709660399,1.204709660399,1.204709660399,1.204709660399,
1.204709660399,1.204709660399,1.204709660399,1.204709660399,1.204709660399,
1.204709660399,1.204709660399,1.204709660399,1.204709660399,1.204709660399,
1.204709660399),(0.9317634465338,0.9317634465338,0.9317634465338,0.9317634465338,
0.9317634465338,0.9317634465338,0.9317634465338,0.9317634465338,0.9317634465338,
0.9317634465338,0.9317634465338,0.9317634465338,0.9317634465338,0.9317634465338,
0.9317634465338,0.9317634465338,0.9317634465338,0.9317634465338,0.9317634465338),
(0.9317634465338,0.9317634465338,0.9317634465338,0.9317634465338,0.9317634465338,
0.9317634465338,0.9317634465338,0.9317634465338,0.9317634465338,0.9317634465338,
0.9317634465338,0.9317634465338,0.9317634465338,0.9317634465338,0.9317634465338,
0.9317634465338,0.9317634465338,0.9317634465338,0.9317634465338),(1.204709660399,
1.204709660399,1.204709660399,1.204709660399,1.204709660399,1.204709660399,
1.204709660399,1.204709660399,1.204709660399,1.204709660399,1.204709660399,
1.204709660399,1.204709660399,1.204709660399,1.204709660399,1.204709660399,
1.204709660399,1.204709660399,1.204709660399)))
REPRESENTATION_ITEM('')
SURFACE()
);
#2394=(
BOUNDED_SURFACE()
B_SPLINE_SURFACE(3,3,((#107055,#107056,#107057,#107058,#107059,#107060,
#107061,#107062,#107063,#107064,#107065,#107066,#107067,#107068,#107069,
#107070,#107071,#107072,#107073,#107074),(#107075,#107076,#107077,#107078,
#107079,#107080,#107081,#107082,#107083,#107084,#107085,#107086,#107087,
#107088,#107089,#107090,#107091,#107092,#107093,#107094),(#107095,#107096,
#107097,#107098,#107099,#107100,#107101,#107102,#107103,#107104,#107105,
#107106,#107107,#107108,#107109,#107110,#107111,#107112,#107113,#107114),
(#107115,#107116,#107117,#107118,#107119,#107120,#107121,#107122,#107123,
#107124,#107125,#107126,#107127,#107128,#107129,#107130,#107131,#107132,
#107133,#107134)),.UNSPECIFIED.,.F.,.F.,.F.)
B_SPLINE_SURFACE_WITH_KNOTS((4,4),(4,1,1,1,1,1,1,1,1,1,1,1,1,1,1,1,1,4),
(0.,1.),(0.,0.0634473073458767,0.137474475480583,0.203439315591922,0.266070813426101,
0.333494447777073,0.401437472430427,0.464401084256882,0.51858368764375,
0.569769560865856,0.622221496328389,0.67514181525029,0.727526446084146,
0.778774499915783,0.832231436034466,0.891640084181608,0.951727885385323,
1.),.UNSPECIFIED.)
GEOMETRIC_REPRESENTATION_ITEM()
RATIONAL_B_SPLINE_SURFACE(((1.186029185783,1.186029185783,1.186029185783,
1.186029185783,1.186029185783,1.186029185783,1.186029185783,1.186029185783,
1.186029185783,1.186029185783,1.186029185783,1.186029185783,1.186029185783,
1.186029185783,1.186029185783,1.186029185783,1.186029185783,1.186029185783,
1.186029185783,1.186029185783),(0.9379902714058,0.9379902714058,0.9379902714058,
0.9379902714058,0.9379902714058,0.9379902714058,0.9379902714058,0.9379902714058,
0.9379902714058,0.9379902714058,0.9379902714058,0.9379902714058,0.9379902714058,
0.9379902714058,0.9379902714058,0.9379902714058,0.9379902714058,0.9379902714058,
0.9379902714058,0.9379902714058),(0.9379902714058,0.9379902714058,0.9379902714058,
0.9379902714058,0.9379902714058,0.9379902714058,0.9379902714058,0.9379902714058,
0.9379902714058,0.9379902714058,0.9379902714058,0.9379902714058,0.9379902714058,
0.9379902714058,0.9379902714058,0.9379902714058,0.9379902714058,0.9379902714058,
0.9379902714058,0.9379902714058),(1.186029185783,1.186029185783,1.186029185783,
1.186029185783,1.186029185783,1.186029185783,1.186029185783,1.186029185783,
1.186029185783,1.186029185783,1.186029185783,1.186029185783,1.186029185783,
1.186029185783,1.186029185783,1.186029185783,1.186029185783,1.186029185783,
1.186029185783,1.186029185783)))
REPRESENTATION_ITEM('')
SURFACE()
);
#2395=(
BOUNDED_SURFACE()
B_SPLINE_SURFACE(3,3,((#107227,#107228,#107229,#107230,#107231,#107232,
#107233,#107234,#107235,#107236,#107237,#107238,#107239,#107240,#107241,
#107242,#107243,#107244),(#107245,#107246,#107247,#107248,#107249,#107250,
#107251,#107252,#107253,#107254,#107255,#107256,#107257,#107258,#107259,
#107260,#107261,#107262),(#107263,#107264,#107265,#107266,#107267,#107268,
#107269,#107270,#107271,#107272,#107273,#107274,#107275,#107276,#107277,
#107278,#107279,#107280),(#107281,#107282,#107283,#107284,#107285,#107286,
#107287,#107288,#107289,#107290,#107291,#107292,#107293,#107294,#107295,
#107296,#107297,#107298)),.UNSPECIFIED.,.F.,.F.,.F.)
B_SPLINE_SURFACE_WITH_KNOTS((4,4),(4,1,1,1,1,1,1,1,1,1,1,1,1,1,1,4),(0.,
1.),(0.,0.10132397085951,0.219927044777174,0.32793320705097,0.424979133082566,
0.511366209904966,0.588468326001569,0.657700207042955,0.720289724582783,
0.776922704267249,0.828179553385519,0.874662083720489,0.91698653274977,
0.955782383375446,0.991693741530312,1.),.UNSPECIFIED.)
GEOMETRIC_REPRESENTATION_ITEM()
RATIONAL_B_SPLINE_SURFACE(((1.284279766139,1.284279766139,1.284279766139,
1.284279766139,1.284279766139,1.284279766139,1.284279766139,1.284279766139,
1.284279766139,1.284279766139,1.284279766139,1.284279766139,1.284279766139,
1.284279766139,1.284279766139,1.284279766139,1.284279766139,1.284279766139),
(0.9052400779535,0.9052400779535,0.9052400779535,0.9052400779535,0.9052400779535,
0.9052400779535,0.9052400779535,0.9052400779535,0.9052400779535,0.9052400779535,
0.9052400779535,0.9052400779535,0.9052400779535,0.9052400779535,0.9052400779535,
0.9052400779535,0.9052400779535,0.9052400779535),(0.9052400779535,0.9052400779535,
0.9052400779535,0.9052400779535,0.9052400779535,0.9052400779535,0.9052400779535,
0.9052400779535,0.9052400779535,0.9052400779535,0.9052400779535,0.9052400779535,
0.9052400779535,0.9052400779535,0.9052400779535,0.9052400779535,0.9052400779535,
0.9052400779535),(1.284279766139,1.284279766139,1.284279766139,1.284279766139,
1.284279766139,1.284279766139,1.284279766139,1.284279766139,1.284279766139,
1.284279766139,1.284279766139,1.284279766139,1.284279766139,1.284279766139,
1.284279766139,1.284279766139,1.284279766139,1.284279766139)))
REPRESENTATION_ITEM('')
SURFACE()
);
#2396=(
BOUNDED_SURFACE()
B_SPLINE_SURFACE(3,3,((#107767,#107768,#107769,#107770,#107771,#107772,
#107773,#107774,#107775,#107776,#107777,#107778,#107779,#107780,#107781,
#107782,#107783,#107784,#107785,#107786,#107787,#107788,#107789,#107790,
#107791,#107792,#107793,#107794,#107795,#107796,#107797,#107798,#107799),
(#107800,#107801,#107802,#107803,#107804,#107805,#107806,#107807,#107808,
#107809,#107810,#107811,#107812,#107813,#107814,#107815,#107816,#107817,
#107818,#107819,#107820,#107821,#107822,#107823,#107824,#107825,#107826,
#107827,#107828,#107829,#107830,#107831,#107832),(#107833,#107834,#107835,
#107836,#107837,#107838,#107839,#107840,#107841,#107842,#107843,#107844,
#107845,#107846,#107847,#107848,#107849,#107850,#107851,#107852,#107853,
#107854,#107855,#107856,#107857,#107858,#107859,#107860,#107861,#107862,
#107863,#107864,#107865),(#107866,#107867,#107868,#107869,#107870,#107871,
#107872,#107873,#107874,#107875,#107876,#107877,#107878,#107879,#107880,
#107881,#107882,#107883,#107884,#107885,#107886,#107887,#107888,#107889,
#107890,#107891,#107892,#107893,#107894,#107895,#107896,#107897,#107898)),
 .UNSPECIFIED.,.F.,.F.,.F.)
B_SPLINE_SURFACE_WITH_KNOTS((4,4),(4,1,1,1,1,1,1,1,1,1,1,1,1,1,1,1,1,1,
1,1,1,1,1,1,1,1,1,1,1,1,4),(0.,1.),(0.,0.0644716348476169,0.137167075810373,
0.211054732176919,0.283781237138607,0.353003626042113,0.416381685205945,
0.471964431181103,0.521223312478128,0.565576440751156,0.605617803352698,
0.641934173237287,0.675008141068028,0.705215849646144,0.732928243655327,
0.758516244890887,0.78233549305937,0.804479039034365,0.824836899490745,
0.843461996593347,0.860503635413291,0.876112967850447,0.890506098780472,
0.904021603335236,0.917013597842901,0.930049136530003,0.944066490933434,
0.959054067042945,0.973766036233171,0.986879426257445,1.),.UNSPECIFIED.)
GEOMETRIC_REPRESENTATION_ITEM()
RATIONAL_B_SPLINE_SURFACE(((1.095545407101,1.095545407101,1.095545407101,
1.095545407101,1.095545407101,1.095545407101,1.095545407101,1.095545407101,
1.095545407101,1.095545407101,1.095545407101,1.095545407101,1.095545407101,
1.095545407101,1.095545407101,1.095545407101,1.095545407101,1.095545407101,
1.095545407101,1.095545407101,1.095545407101,1.095545407101,1.095545407101,
1.095545407101,1.095545407101,1.095545407101,1.095545407101,1.095545407101,
1.095545407101,1.095545407101,1.095545407101,1.095545407101,1.095545407101),
(0.9681515309662,0.9681515309662,0.9681515309662,0.9681515309662,0.9681515309662,
0.9681515309662,0.9681515309662,0.9681515309662,0.9681515309662,0.9681515309662,
0.9681515309662,0.9681515309662,0.9681515309662,0.9681515309662,0.9681515309662,
0.9681515309662,0.9681515309662,0.9681515309662,0.9681515309662,0.9681515309662,
0.9681515309662,0.9681515309662,0.9681515309662,0.9681515309662,0.9681515309662,
0.9681515309662,0.9681515309662,0.9681515309662,0.9681515309662,0.9681515309662,
0.9681515309662,0.9681515309662,0.9681515309662),(0.9681515309662,0.9681515309662,
0.9681515309662,0.9681515309662,0.9681515309662,0.9681515309662,0.9681515309662,
0.9681515309662,0.9681515309662,0.9681515309662,0.9681515309662,0.9681515309662,
0.9681515309662,0.9681515309662,0.9681515309662,0.9681515309662,0.9681515309662,
0.9681515309662,0.9681515309662,0.9681515309662,0.9681515309662,0.9681515309662,
0.9681515309662,0.9681515309662,0.9681515309662,0.9681515309662,0.9681515309662,
0.9681515309662,0.9681515309662,0.9681515309662,0.9681515309662,0.9681515309662,
0.9681515309662),(1.095545407101,1.095545407101,1.095545407101,1.095545407101,
1.095545407101,1.095545407101,1.095545407101,1.095545407101,1.095545407101,
1.095545407101,1.095545407101,1.095545407101,1.095545407101,1.095545407101,
1.095545407101,1.095545407101,1.095545407101,1.095545407101,1.095545407101,
1.095545407101,1.095545407101,1.095545407101,1.095545407101,1.095545407101,
1.095545407101,1.095545407101,1.095545407101,1.095545407101,1.095545407101,
1.095545407101,1.095545407101,1.095545407101,1.095545407101)))
REPRESENTATION_ITEM('')
SURFACE()
);
#2397=(
BOUNDED_SURFACE()
B_SPLINE_SURFACE(3,3,((#107915,#107916,#107917,#107918,#107919,#107920,
#107921,#107922,#107923,#107924,#107925,#107926,#107927,#107928,#107929,
#107930,#107931),(#107932,#107933,#107934,#107935,#107936,#107937,#107938,
#107939,#107940,#107941,#107942,#107943,#107944,#107945,#107946,#107947,
#107948),(#107949,#107950,#107951,#107952,#107953,#107954,#107955,#107956,
#107957,#107958,#107959,#107960,#107961,#107962,#107963,#107964,#107965),
(#107966,#107967,#107968,#107969,#107970,#107971,#107972,#107973,#107974,
#107975,#107976,#107977,#107978,#107979,#107980,#107981,#107982)),
 .UNSPECIFIED.,.F.,.F.,.F.)
B_SPLINE_SURFACE_WITH_KNOTS((4,4),(4,1,1,1,1,1,1,1,1,1,1,1,1,1,4),(0.,1.),
(0.,0.0956146431540125,0.200570336486981,0.29617085639003,0.382446369780954,
0.459533334763256,0.527981368507571,0.590340486919798,0.649866246025106,
0.709565784246277,0.769912468560832,0.830222740675431,0.890369247895391,
0.9504555950694,1.),.UNSPECIFIED.)
GEOMETRIC_REPRESENTATION_ITEM()
RATIONAL_B_SPLINE_SURFACE(((1.220899632035,1.220899632035,1.220899632035,
1.220899632035,1.220899632035,1.220899632035,1.220899632035,1.220899632035,
1.220899632035,1.220899632035,1.220899632035,1.220899632035,1.220899632035,
1.220899632035,1.220899632035,1.220899632035,1.220899632035),(0.9263667893217,
0.9263667893217,0.9263667893217,0.9263667893217,0.9263667893217,0.9263667893217,
0.9263667893217,0.9263667893217,0.9263667893217,0.9263667893217,0.9263667893217,
0.9263667893217,0.9263667893217,0.9263667893217,0.9263667893217,0.9263667893217,
0.9263667893217),(0.9263667893217,0.9263667893217,0.9263667893217,0.9263667893217,
0.9263667893217,0.9263667893217,0.9263667893217,0.9263667893217,0.9263667893217,
0.9263667893217,0.9263667893217,0.9263667893217,0.9263667893217,0.9263667893217,
0.9263667893217,0.9263667893217,0.9263667893217),(1.220899632035,1.220899632035,
1.220899632035,1.220899632035,1.220899632035,1.220899632035,1.220899632035,
1.220899632035,1.220899632035,1.220899632035,1.220899632035,1.220899632035,
1.220899632035,1.220899632035,1.220899632035,1.220899632035,1.220899632035)))
REPRESENTATION_ITEM('')
SURFACE()
);
#2398=(
BOUNDED_SURFACE()
B_SPLINE_SURFACE(3,3,((#107984,#107985,#107986,#107987,#107988,#107989,
#107990,#107991,#107992,#107993,#107994,#107995,#107996,#107997),(#107998,
#107999,#108000,#108001,#108002,#108003,#108004,#108005,#108006,#108007,
#108008,#108009,#108010,#108011),(#108012,#108013,#108014,#108015,#108016,
#108017,#108018,#108019,#108020,#108021,#108022,#108023,#108024,#108025),
(#108026,#108027,#108028,#108029,#108030,#108031,#108032,#108033,#108034,
#108035,#108036,#108037,#108038,#108039),(#108040,#108041,#108042,#108043,
#108044,#108045,#108046,#108047,#108048,#108049,#108050,#108051,#108052,
#108053),(#108054,#108055,#108056,#108057,#108058,#108059,#108060,#108061,
#108062,#108063,#108064,#108065,#108066,#108067),(#108068,#108069,#108070,
#108071,#108072,#108073,#108074,#108075,#108076,#108077,#108078,#108079,
#108080,#108081)),.UNSPECIFIED.,.F.,.F.,.F.)
B_SPLINE_SURFACE_WITH_KNOTS((4,3,4),(4,1,1,1,1,1,1,1,1,1,1,4),(0.,0.5,1.),
(0.,0.0583353807888762,0.12799724109847,0.204577536604604,0.288006073180643,
0.378737316341168,0.478075810040363,0.587386075028147,0.707620337333203,
0.838547292329974,0.975947862327006,1.),.UNSPECIFIED.)
GEOMETRIC_REPRESENTATION_ITEM()
RATIONAL_B_SPLINE_SURFACE(((1.174660538235,1.174660538235,1.174660538235,
1.174660538235,1.174660538235,1.174660538235,1.174660538235,1.174660538235,
1.174660538235,1.174660538235,1.174660538235,1.174660538235,1.174660538235,
1.174660538235),(0.9417798205884,0.9417798205884,0.9417798205884,0.9417798205884,
0.9417798205884,0.9417798205884,0.9417798205884,0.9417798205884,0.9417798205884,
0.9417798205884,0.9417798205884,0.9417798205884,0.9417798205884,0.9417798205884),
(0.9417798205884,0.9417798205884,0.9417798205884,0.9417798205884,0.9417798205884,
0.9417798205884,0.9417798205884,0.9417798205884,0.9417798205884,0.9417798205884,
0.9417798205884,0.9417798205884,0.9417798205884,0.9417798205884),(1.174660538235,
1.174660538235,1.174660538235,1.174660538235,1.174660538235,1.174660538235,
1.174660538235,1.174660538235,1.174660538235,1.174660538235,1.174660538235,
1.174660538235,1.174660538235,1.174660538235),(0.9417798205884,0.9417798205884,
0.9417798205884,0.9417798205884,0.9417798205884,0.9417798205884,0.9417798205884,
0.9417798205884,0.9417798205884,0.9417798205884,0.9417798205884,0.9417798205884,
0.9417798205884,0.9417798205884),(0.9417798205884,0.9417798205884,0.9417798205884,
0.9417798205884,0.9417798205884,0.9417798205884,0.9417798205884,0.9417798205884,
0.9417798205884,0.9417798205884,0.9417798205884,0.9417798205884,0.9417798205884,
0.9417798205884),(1.174660538235,1.174660538235,1.174660538235,1.174660538235,
1.174660538235,1.174660538235,1.174660538235,1.174660538235,1.174660538235,
1.174660538235,1.174660538235,1.174660538235,1.174660538235,1.174660538235)))
REPRESENTATION_ITEM('')
SURFACE()
);
#2399=(
BOUNDED_SURFACE()
B_SPLINE_SURFACE(3,3,((#108137,#108138,#108139,#108140,#108141,#108142,
#108143,#108144,#108145,#108146,#108147,#108148,#108149,#108150,#108151,
#108152,#108153),(#108154,#108155,#108156,#108157,#108158,#108159,#108160,
#108161,#108162,#108163,#108164,#108165,#108166,#108167,#108168,#108169,
#108170),(#108171,#108172,#108173,#108174,#108175,#108176,#108177,#108178,
#108179,#108180,#108181,#108182,#108183,#108184,#108185,#108186,#108187),
(#108188,#108189,#108190,#108191,#108192,#108193,#108194,#108195,#108196,
#108197,#108198,#108199,#108200,#108201,#108202,#108203,#108204)),
 .UNSPECIFIED.,.F.,.F.,.F.)
B_SPLINE_SURFACE_WITH_KNOTS((4,4),(4,1,1,1,1,1,1,1,1,1,1,1,1,1,4),(0.,1.),
(0.,0.0421741349720486,0.122382017207444,0.194203536901675,0.257534399271218,
0.321534135544779,0.38726227689901,0.452657895941669,0.516567929355648,
0.579748305445392,0.647421910672303,0.723873761459194,0.810175603109662,
0.905570261612151,1.),.UNSPECIFIED.)
GEOMETRIC_REPRESENTATION_ITEM()
RATIONAL_B_SPLINE_SURFACE(((1.219577374139,1.219577374139,1.219577374139,
1.219577374139,1.219577374139,1.219577374139,1.219577374139,1.219577374139,
1.219577374139,1.219577374139,1.219577374139,1.219577374139,1.219577374139,
1.219577374139,1.219577374139,1.219577374139,1.219577374139),(0.9268075419537,
0.9268075419537,0.9268075419537,0.9268075419537,0.9268075419537,0.9268075419537,
0.9268075419537,0.9268075419537,0.9268075419537,0.9268075419537,0.9268075419537,
0.9268075419537,0.9268075419537,0.9268075419537,0.9268075419537,0.9268075419537,
0.9268075419537),(0.9268075419537,0.9268075419537,0.9268075419537,0.9268075419537,
0.9268075419537,0.9268075419537,0.9268075419537,0.9268075419537,0.9268075419537,
0.9268075419537,0.9268075419537,0.9268075419537,0.9268075419537,0.9268075419537,
0.9268075419537,0.9268075419537,0.9268075419537),(1.219577374139,1.219577374139,
1.219577374139,1.219577374139,1.219577374139,1.219577374139,1.219577374139,
1.219577374139,1.219577374139,1.219577374139,1.219577374139,1.219577374139,
1.219577374139,1.219577374139,1.219577374139,1.219577374139,1.219577374139)))
REPRESENTATION_ITEM('')
SURFACE()
);
#2400=(
BOUNDED_SURFACE()
B_SPLINE_SURFACE(3,3,((#108545,#108546,#108547,#108548,#108549,#108550,
#108551,#108552,#108553,#108554,#108555,#108556,#108557,#108558,#108559,
#108560,#108561,#108562),(#108563,#108564,#108565,#108566,#108567,#108568,
#108569,#108570,#108571,#108572,#108573,#108574,#108575,#108576,#108577,
#108578,#108579,#108580),(#108581,#108582,#108583,#108584,#108585,#108586,
#108587,#108588,#108589,#108590,#108591,#108592,#108593,#108594,#108595,
#108596,#108597,#108598),(#108599,#108600,#108601,#108602,#108603,#108604,
#108605,#108606,#108607,#108608,#108609,#108610,#108611,#108612,#108613,
#108614,#108615,#108616)),.UNSPECIFIED.,.F.,.F.,.F.)
B_SPLINE_SURFACE_WITH_KNOTS((4,4),(4,1,1,1,1,1,1,1,1,1,1,1,1,1,1,4),(0.,
1.),(0.,0.00785484539651376,0.0438075231225187,0.0829336925491939,0.125798873740089,
0.172955219979332,0.224941148148525,0.282279526175794,0.345470718132813,
0.415012619574855,0.491463209282815,0.575434444650706,0.667777195884821,
0.770833971303908,0.887651863786679,1.),.UNSPECIFIED.)
GEOMETRIC_REPRESENTATION_ITEM()
RATIONAL_B_SPLINE_SURFACE(((1.284338682996,1.284338682996,1.284338682996,
1.284338682996,1.284338682996,1.284338682996,1.284338682996,1.284338682996,
1.284338682996,1.284338682996,1.284338682996,1.284338682996,1.284338682996,
1.284338682996,1.284338682996,1.284338682996,1.284338682996,1.284338682996),
(0.9052204390014,0.9052204390014,0.9052204390014,0.9052204390014,0.9052204390014,
0.9052204390014,0.9052204390014,0.9052204390014,0.9052204390014,0.9052204390014,
0.9052204390014,0.9052204390014,0.9052204390014,0.9052204390014,0.9052204390014,
0.9052204390014,0.9052204390014,0.9052204390014),(0.9052204390014,0.9052204390014,
0.9052204390014,0.9052204390014,0.9052204390014,0.9052204390014,0.9052204390014,
0.9052204390014,0.9052204390014,0.9052204390014,0.9052204390014,0.9052204390014,
0.9052204390014,0.9052204390014,0.9052204390014,0.9052204390014,0.9052204390014,
0.9052204390014),(1.284338682996,1.284338682996,1.284338682996,1.284338682996,
1.284338682996,1.284338682996,1.284338682996,1.284338682996,1.284338682996,
1.284338682996,1.284338682996,1.284338682996,1.284338682996,1.284338682996,
1.284338682996,1.284338682996,1.284338682996,1.284338682996)))
REPRESENTATION_ITEM('')
SURFACE()
);
#2401=(
BOUNDED_SURFACE()
B_SPLINE_SURFACE(3,3,((#108761,#108762,#108763,#108764,#108765,#108766,
#108767),(#108768,#108769,#108770,#108771,#108772,#108773,#108774),(#108775,
#108776,#108777,#108778,#108779,#108780,#108781),(#108782,#108783,#108784,
#108785,#108786,#108787,#108788)),.UNSPECIFIED.,.F.,.F.,.F.)
B_SPLINE_SURFACE_WITH_KNOTS((4,4),(4,1,1,1,4),(0.173609205866266,0.826397151609457),
(0.734662338499708,0.745916192959342,0.809036419626865,0.87313299624406,
0.92104874395541),.UNSPECIFIED.)
GEOMETRIC_REPRESENTATION_ITEM()
RATIONAL_B_SPLINE_SURFACE(((1.0407131654991,1.0407131654991,1.0407131654991,
1.0407131654991,1.0407131654991,1.0407131654991,1.0407131654991),(0.98642841615643,
0.98642841615643,0.98642841615643,0.98642841615643,0.98642841615643,0.98642841615643,
0.98642841615643),(0.986428944838583,0.986428944838583,0.986428944838583,
0.986428944838583,0.986428944838583,0.986428944838583,0.986428944838583),
(1.04071475154556,1.04071475154556,1.04071475154556,1.04071475154556,1.04071475154556,
1.04071475154556,1.04071475154556)))
REPRESENTATION_ITEM('')
SURFACE()
);
#2402=(
BOUNDED_SURFACE()
B_SPLINE_SURFACE(3,3,((#108828,#108829,#108830,#108831,#108832,#108833,
#108834,#108835,#108836,#108837,#108838,#108839,#108840,#108841,#108842,
#108843,#108844),(#108845,#108846,#108847,#108848,#108849,#108850,#108851,
#108852,#108853,#108854,#108855,#108856,#108857,#108858,#108859,#108860,
#108861),(#108862,#108863,#108864,#108865,#108866,#108867,#108868,#108869,
#108870,#108871,#108872,#108873,#108874,#108875,#108876,#108877,#108878),
(#108879,#108880,#108881,#108882,#108883,#108884,#108885,#108886,#108887,
#108888,#108889,#108890,#108891,#108892,#108893,#108894,#108895)),
 .UNSPECIFIED.,.F.,.F.,.F.)
B_SPLINE_SURFACE_WITH_KNOTS((4,4),(4,1,1,1,1,1,1,1,1,1,1,1,1,1,4),(0.,1.),
(0.,0.0494607190127907,0.109552090730043,0.169758737534662,0.230148354533949,
0.290560261854406,0.350306525877549,0.40987255925942,0.472274987329372,
0.540774950770296,0.617873523590501,0.704101656323432,0.799618934750072,
0.904474902078167,1.),.UNSPECIFIED.)
GEOMETRIC_REPRESENTATION_ITEM()
RATIONAL_B_SPLINE_SURFACE(((1.220899718882,1.220899718882,1.220899718882,
1.220899718882,1.220899718882,1.220899718882,1.220899718882,1.220899718882,
1.220899718882,1.220899718882,1.220899718882,1.220899718882,1.220899718882,
1.220899718882,1.220899718882,1.220899718882,1.220899718882),(0.9263667603727,
0.9263667603727,0.9263667603727,0.9263667603727,0.9263667603727,0.9263667603727,
0.9263667603727,0.9263667603727,0.9263667603727,0.9263667603727,0.9263667603727,
0.9263667603727,0.9263667603727,0.9263667603727,0.9263667603727,0.9263667603727,
0.9263667603727),(0.9263667603727,0.9263667603727,0.9263667603727,0.9263667603727,
0.9263667603727,0.9263667603727,0.9263667603727,0.9263667603727,0.9263667603727,
0.9263667603727,0.9263667603727,0.9263667603727,0.9263667603727,0.9263667603727,
0.9263667603727,0.9263667603727,0.9263667603727),(1.220899718882,1.220899718882,
1.220899718882,1.220899718882,1.220899718882,1.220899718882,1.220899718882,
1.220899718882,1.220899718882,1.220899718882,1.220899718882,1.220899718882,
1.220899718882,1.220899718882,1.220899718882,1.220899718882,1.220899718882)))
REPRESENTATION_ITEM('')
SURFACE()
);
#2403=(
BOUNDED_SURFACE()
B_SPLINE_SURFACE(3,3,((#108897,#108898,#108899,#108900,#108901,#108902,
#108903,#108904,#108905,#108906,#108907,#108908,#108909,#108910,#108911,
#108912,#108913),(#108914,#108915,#108916,#108917,#108918,#108919,#108920,
#108921,#108922,#108923,#108924,#108925,#108926,#108927,#108928,#108929,
#108930),(#108931,#108932,#108933,#108934,#108935,#108936,#108937,#108938,
#108939,#108940,#108941,#108942,#108943,#108944,#108945,#108946,#108947),
(#108948,#108949,#108950,#108951,#108952,#108953,#108954,#108955,#108956,
#108957,#108958,#108959,#108960,#108961,#108962,#108963,#108964)),
 .UNSPECIFIED.,.F.,.F.,.F.)
B_SPLINE_SURFACE_WITH_KNOTS((4,4),(4,1,1,1,1,1,1,1,1,1,1,1,1,1,4),(0.,1.),
(0.,0.0934555018707438,0.190098316562109,0.277412276927369,0.35430591142789,
0.422006518582467,0.485074288423762,0.548771616802643,0.613848873864871,
0.679223443651306,0.742843206526981,0.805944165791561,0.877524725574254,
0.957638281560363,1.),.UNSPECIFIED.)
GEOMETRIC_REPRESENTATION_ITEM()
RATIONAL_B_SPLINE_SURFACE(((1.219577491546,1.219577491546,1.219577491546,
1.219577491546,1.219577491546,1.219577491546,1.219577491546,1.219577491546,
1.219577491546,1.219577491546,1.219577491546,1.219577491546,1.219577491546,
1.219577491546,1.219577491546,1.219577491546,1.219577491546),(0.9268075028179,
0.9268075028179,0.9268075028179,0.9268075028179,0.9268075028179,0.9268075028179,
0.9268075028179,0.9268075028179,0.9268075028179,0.9268075028179,0.9268075028179,
0.9268075028179,0.9268075028179,0.9268075028179,0.9268075028179,0.9268075028179,
0.9268075028179),(0.9268075028179,0.9268075028179,0.9268075028179,0.9268075028179,
0.9268075028179,0.9268075028179,0.9268075028179,0.9268075028179,0.9268075028179,
0.9268075028179,0.9268075028179,0.9268075028179,0.9268075028179,0.9268075028179,
0.9268075028179,0.9268075028179,0.9268075028179),(1.219577491546,1.219577491546,
1.219577491546,1.219577491546,1.219577491546,1.219577491546,1.219577491546,
1.219577491546,1.219577491546,1.219577491546,1.219577491546,1.219577491546,
1.219577491546,1.219577491546,1.219577491546,1.219577491546,1.219577491546)))
REPRESENTATION_ITEM('')
SURFACE()
);
#2404=(
BOUNDED_SURFACE()
B_SPLINE_SURFACE(3,3,((#108983,#108984,#108985,#108986,#108987,#108988,
#108989,#108990,#108991,#108992,#108993,#108994,#108995,#108996),(#108997,
#108998,#108999,#109000,#109001,#109002,#109003,#109004,#109005,#109006,
#109007,#109008,#109009,#109010),(#109011,#109012,#109013,#109014,#109015,
#109016,#109017,#109018,#109019,#109020,#109021,#109022,#109023,#109024),
(#109025,#109026,#109027,#109028,#109029,#109030,#109031,#109032,#109033,
#109034,#109035,#109036,#109037,#109038),(#109039,#109040,#109041,#109042,
#109043,#109044,#109045,#109046,#109047,#109048,#109049,#109050,#109051,
#109052),(#109053,#109054,#109055,#109056,#109057,#109058,#109059,#109060,
#109061,#109062,#109063,#109064,#109065,#109066),(#109067,#109068,#109069,
#109070,#109071,#109072,#109073,#109074,#109075,#109076,#109077,#109078,
#109079,#109080)),.UNSPECIFIED.,.F.,.F.,.F.)
B_SPLINE_SURFACE_WITH_KNOTS((4,3,4),(4,1,1,1,1,1,1,1,1,1,1,4),(0.,0.5,1.),
(0.,0.0457158190500442,0.186722884538372,0.317871899774413,0.436483936855332,
0.542898565175996,0.638400280945175,0.724959173697019,0.804412779028879,
0.877341467334142,0.943792148331645,1.),.UNSPECIFIED.)
GEOMETRIC_REPRESENTATION_ITEM()
RATIONAL_B_SPLINE_SURFACE(((1.174644569129,1.174644569129,1.174644569129,
1.174644569129,1.174644569129,1.174644569129,1.174644569129,1.174644569129,
1.174644569129,1.174644569129,1.174644569129,1.174644569129,1.174644569129,
1.174644569129),(0.9417851436237,0.9417851436237,0.9417851436237,0.9417851436237,
0.9417851436237,0.9417851436237,0.9417851436237,0.9417851436237,0.9417851436237,
0.9417851436237,0.9417851436237,0.9417851436237,0.9417851436237,0.9417851436237),
(0.9417851436237,0.9417851436237,0.9417851436237,0.9417851436237,0.9417851436237,
0.9417851436237,0.9417851436237,0.9417851436237,0.9417851436237,0.9417851436237,
0.9417851436237,0.9417851436237,0.9417851436237,0.9417851436237),(1.174644569129,
1.174644569129,1.174644569129,1.174644569129,1.174644569129,1.174644569129,
1.174644569129,1.174644569129,1.174644569129,1.174644569129,1.174644569129,
1.174644569129,1.174644569129,1.174644569129),(0.9417851436237,0.9417851436237,
0.9417851436237,0.9417851436237,0.9417851436237,0.9417851436237,0.9417851436237,
0.9417851436237,0.9417851436237,0.9417851436237,0.9417851436237,0.9417851436237,
0.9417851436237,0.9417851436237),(0.9417851436237,0.9417851436237,0.9417851436237,
0.9417851436237,0.9417851436237,0.9417851436237,0.9417851436237,0.9417851436237,
0.9417851436237,0.9417851436237,0.9417851436237,0.9417851436237,0.9417851436237,
0.9417851436237),(1.174644569129,1.174644569129,1.174644569129,1.174644569129,
1.174644569129,1.174644569129,1.174644569129,1.174644569129,1.174644569129,
1.174644569129,1.174644569129,1.174644569129,1.174644569129,1.174644569129)))
REPRESENTATION_ITEM('')
SURFACE()
);
#2405=(
BOUNDED_SURFACE()
B_SPLINE_SURFACE(2,2,((#111271,#111272,#111273,#111274,#111275,#111276,
#111277,#111278,#111279),(#111280,#111281,#111282,#111283,#111284,#111285,
#111286,#111287,#111288),(#111289,#111290,#111291,#111292,#111293,#111294,
#111295,#111296,#111297)),.UNSPECIFIED.,.F.,.T.,.F.)
B_SPLINE_SURFACE_WITH_KNOTS((3,3),(3,2,2,2,3),(-0.000347234788822782,0.411138013168365),
(-3.14159265358979,-1.5707963267949,0.,1.5707963267949,3.14159265358979),
 .UNSPECIFIED.)
GEOMETRIC_REPRESENTATION_ITEM()
RATIONAL_B_SPLINE_SURFACE(((1.,0.707106781186548,1.,0.707106781186548,1.,
0.707106781186548,1.,0.707106781186548,1.),(0.978909540707877,0.692193574402748,
0.978909540707877,0.692193574402748,0.978909540707877,0.692193574402748,
0.978909540707877,0.692193574402748,0.978909540707877),(1.,0.707106781186548,
1.,0.707106781186548,1.,0.707106781186548,1.,0.707106781186548,1.)))
REPRESENTATION_ITEM('')
SURFACE()
);
#2406=(
BOUNDED_SURFACE()
B_SPLINE_SURFACE(3,3,((#116850,#116851,#116852,#116853,#116854,#116855,
#116856,#116857),(#116858,#116859,#116860,#116861,#116862,#116863,#116864,
#116865),(#116866,#116867,#116868,#116869,#116870,#116871,#116872,#116873),
(#116874,#116875,#116876,#116877,#116878,#116879,#116880,#116881)),
 .UNSPECIFIED.,.F.,.F.,.F.)
B_SPLINE_SURFACE_WITH_KNOTS((4,4),(4,1,1,1,1,4),(0.,1.),(0.,0.029644668996018,
0.295068368107701,0.594721077667762,0.933272474288206,1.),.UNSPECIFIED.)
GEOMETRIC_REPRESENTATION_ITEM()
RATIONAL_B_SPLINE_SURFACE(((1.155703625555,1.155703625555,1.155703625555,
1.155703625555,1.155703625555,1.155703625555,1.155703625555,1.155703625555),
(0.9480987914817,0.9480987914817,0.9480987914817,0.9480987914817,0.9480987914817,
0.9480987914817,0.9480987914817,0.9480987914817),(0.9480987914817,0.9480987914817,
0.9480987914817,0.9480987914817,0.9480987914817,0.9480987914817,0.9480987914817,
0.9480987914817),(1.155703625555,1.155703625555,1.155703625555,1.155703625555,
1.155703625555,1.155703625555,1.155703625555,1.155703625555)))
REPRESENTATION_ITEM('')
SURFACE()
);
#2407=(
BOUNDED_SURFACE()
B_SPLINE_SURFACE(3,3,((#116993,#116994,#116995,#116996,#116997,#116998,
#116999,#117000,#117001,#117002,#117003,#117004,#117005,#117006),(#117007,
#117008,#117009,#117010,#117011,#117012,#117013,#117014,#117015,#117016,
#117017,#117018,#117019,#117020),(#117021,#117022,#117023,#117024,#117025,
#117026,#117027,#117028,#117029,#117030,#117031,#117032,#117033,#117034),
(#117035,#117036,#117037,#117038,#117039,#117040,#117041,#117042,#117043,
#117044,#117045,#117046,#117047,#117048)),.UNSPECIFIED.,.F.,.F.,.F.)
B_SPLINE_SURFACE_WITH_KNOTS((4,4),(4,1,1,1,1,1,1,1,1,1,1,4),(0.,1.),(0.,
0.0973878961741514,0.197407551664285,0.282741541036489,0.368602466936746,
0.462528035468287,0.558082759241583,0.651875585473768,0.746019006514905,
0.842958604322709,0.945166921256564,1.),.UNSPECIFIED.)
GEOMETRIC_REPRESENTATION_ITEM()
RATIONAL_B_SPLINE_SURFACE(((1.120036296291,1.120036296291,1.120036296291,
1.120036296291,1.120036296291,1.120036296291,1.120036296291,1.120036296291,
1.120036296291,1.120036296291,1.120036296291,1.120036296291,1.120036296291,
1.120036296291),(0.9599879012363,0.9599879012363,0.9599879012363,0.9599879012363,
0.9599879012363,0.9599879012363,0.9599879012363,0.9599879012363,0.9599879012363,
0.9599879012363,0.9599879012363,0.9599879012363,0.9599879012363,0.9599879012363),
(0.9599879012363,0.9599879012363,0.9599879012363,0.9599879012363,0.9599879012363,
0.9599879012363,0.9599879012363,0.9599879012363,0.9599879012363,0.9599879012363,
0.9599879012363,0.9599879012363,0.9599879012363,0.9599879012363),(1.120036296291,
1.120036296291,1.120036296291,1.120036296291,1.120036296291,1.120036296291,
1.120036296291,1.120036296291,1.120036296291,1.120036296291,1.120036296291,
1.120036296291,1.120036296291,1.120036296291)))
REPRESENTATION_ITEM('')
SURFACE()
);
#2408=(
BOUNDED_SURFACE()
B_SPLINE_SURFACE(3,3,((#117119,#117120,#117121,#117122,#117123,#117124,
#117125,#117126,#117127,#117128,#117129,#117130,#117131),(#117132,#117133,
#117134,#117135,#117136,#117137,#117138,#117139,#117140,#117141,#117142,
#117143,#117144),(#117145,#117146,#117147,#117148,#117149,#117150,#117151,
#117152,#117153,#117154,#117155,#117156,#117157),(#117158,#117159,#117160,
#117161,#117162,#117163,#117164,#117165,#117166,#117167,#117168,#117169,
#117170)),.UNSPECIFIED.,.F.,.F.,.F.)
B_SPLINE_SURFACE_WITH_KNOTS((4,4),(4,1,1,1,1,1,1,1,1,1,4),(0.,1.),(0.,0.0998120955522525,
0.242016858642978,0.370462774661701,0.48666884032665,0.592130131858907,
0.688274163622353,0.775605045484402,0.855250354769886,0.929728823459487,
1.),.UNSPECIFIED.)
GEOMETRIC_REPRESENTATION_ITEM()
RATIONAL_B_SPLINE_SURFACE(((1.293938747545,1.293938747545,1.293938747545,
1.293938747545,1.293938747545,1.293938747545,1.293938747545,1.293938747545,
1.293938747545,1.293938747545,1.293938747545,1.293938747545,1.293938747545),
(0.9020204174849,0.9020204174849,0.9020204174849,0.9020204174849,0.9020204174849,
0.9020204174849,0.9020204174849,0.9020204174849,0.9020204174849,0.9020204174849,
0.9020204174849,0.9020204174849,0.9020204174849),(0.9020204174849,0.9020204174849,
0.9020204174849,0.9020204174849,0.9020204174849,0.9020204174849,0.9020204174849,
0.9020204174849,0.9020204174849,0.9020204174849,0.9020204174849,0.9020204174849,
0.9020204174849),(1.293938747545,1.293938747545,1.293938747545,1.293938747545,
1.293938747545,1.293938747545,1.293938747545,1.293938747545,1.293938747545,
1.293938747545,1.293938747545,1.293938747545,1.293938747545)))
REPRESENTATION_ITEM('')
SURFACE()
);
#2409=(
BOUNDED_SURFACE()
B_SPLINE_SURFACE(3,3,((#117275,#117276,#117277,#117278,#117279,#117280),
(#117281,#117282,#117283,#117284,#117285,#117286),(#117287,#117288,#117289,
#117290,#117291,#117292),(#117293,#117294,#117295,#117296,#117297,#117298)),
 .UNSPECIFIED.,.F.,.F.,.F.)
B_SPLINE_SURFACE_WITH_KNOTS((4,4),(4,1,1,4),(0.,1.),(0.,0.285815104154731,
0.750510867666097,1.),.UNSPECIFIED.)
GEOMETRIC_REPRESENTATION_ITEM()
RATIONAL_B_SPLINE_SURFACE(((1.365416124288,1.365416124288,1.365416124288,
1.365416124288,1.365416124288,1.365416124288),(0.8781946252374,0.8781946252374,
0.8781946252374,0.8781946252374,0.8781946252374,0.8781946252374),(0.8781946252374,
0.8781946252374,0.8781946252374,0.8781946252374,0.8781946252374,0.8781946252374),
(1.365416124288,1.365416124288,1.365416124288,1.365416124288,1.365416124288,
1.365416124288)))
REPRESENTATION_ITEM('')
SURFACE()
);
#2410=(
BOUNDED_SURFACE()
B_SPLINE_SURFACE(3,3,((#117370,#117371,#117372,#117373,#117374,#117375,
#117376,#117377,#117378),(#117379,#117380,#117381,#117382,#117383,#117384,
#117385,#117386,#117387),(#117388,#117389,#117390,#117391,#117392,#117393,
#117394,#117395,#117396),(#117397,#117398,#117399,#117400,#117401,#117402,
#117403,#117404,#117405)),.UNSPECIFIED.,.F.,.F.,.F.)
B_SPLINE_SURFACE_WITH_KNOTS((4,4),(4,1,1,1,1,1,4),(0.,1.),(0.,0.16964553092277,
0.380015263105082,0.568987634495723,0.737810837959708,0.889292577451102,
1.),.UNSPECIFIED.)
GEOMETRIC_REPRESENTATION_ITEM()
RATIONAL_B_SPLINE_SURFACE(((1.365402191724,1.365402191724,1.365402191724,
1.365402191724,1.365402191724,1.365402191724,1.365402191724,1.365402191724,
1.365402191724),(0.8781992694255,0.8781992694255,0.8781992694255,0.8781992694255,
0.8781992694255,0.8781992694255,0.8781992694255,0.8781992694255,0.8781992694255),
(0.8781992694255,0.8781992694255,0.8781992694255,0.8781992694255,0.8781992694255,
0.8781992694255,0.8781992694255,0.8781992694255,0.8781992694255),(1.365402191724,
1.365402191724,1.365402191724,1.365402191724,1.365402191724,1.365402191724,
1.365402191724,1.365402191724,1.365402191724)))
REPRESENTATION_ITEM('')
SURFACE()
);
#2411=(
BOUNDED_SURFACE()
B_SPLINE_SURFACE(3,3,((#117540,#117541,#117542,#117543,#117544,#117545,
#117546,#117547,#117548,#117549,#117550,#117551,#117552,#117553,#117554),
(#117555,#117556,#117557,#117558,#117559,#117560,#117561,#117562,#117563,
#117564,#117565,#117566,#117567,#117568,#117569),(#117570,#117571,#117572,
#117573,#117574,#117575,#117576,#117577,#117578,#117579,#117580,#117581,
#117582,#117583,#117584),(#117585,#117586,#117587,#117588,#117589,#117590,
#117591,#117592,#117593,#117594,#117595,#117596,#117597,#117598,#117599)),
 .UNSPECIFIED.,.F.,.F.,.F.)
B_SPLINE_SURFACE_WITH_KNOTS((4,4),(4,1,1,1,1,1,1,1,1,1,1,1,4),(0.,1.),(0.,
0.0133121513771896,0.155629666020943,0.286186478435823,0.406137126501649,
0.515333723729991,0.614145412195474,0.703320557553204,0.783598098684785,
0.855708888389128,0.920381450070005,0.978344668750669,1.),.UNSPECIFIED.)
GEOMETRIC_REPRESENTATION_ITEM()
RATIONAL_B_SPLINE_SURFACE(((1.250202018407,1.250202018407,1.250202018407,
1.250202018407,1.250202018407,1.250202018407,1.250202018407,1.250202018407,
1.250202018407,1.250202018407,1.250202018407,1.250202018407,1.250202018407,
1.250202018407,1.250202018407),(0.9165993271976,0.9165993271976,0.9165993271976,
0.9165993271976,0.9165993271976,0.9165993271976,0.9165993271976,0.9165993271976,
0.9165993271976,0.9165993271976,0.9165993271976,0.9165993271976,0.9165993271976,
0.9165993271976,0.9165993271976),(0.9165993271976,0.9165993271976,0.9165993271976,
0.9165993271976,0.9165993271976,0.9165993271976,0.9165993271976,0.9165993271976,
0.9165993271976,0.9165993271976,0.9165993271976,0.9165993271976,0.9165993271976,
0.9165993271976,0.9165993271976),(1.250202018407,1.250202018407,1.250202018407,
1.250202018407,1.250202018407,1.250202018407,1.250202018407,1.250202018407,
1.250202018407,1.250202018407,1.250202018407,1.250202018407,1.250202018407,
1.250202018407,1.250202018407)))
REPRESENTATION_ITEM('')
SURFACE()
);
#2412=(
BOUNDED_SURFACE()
B_SPLINE_SURFACE(3,3,((#117620,#117621,#117622,#117623,#117624,#117625,
#117626,#117627,#117628,#117629,#117630,#117631,#117632,#117633,#117634),
(#117635,#117636,#117637,#117638,#117639,#117640,#117641,#117642,#117643,
#117644,#117645,#117646,#117647,#117648,#117649),(#117650,#117651,#117652,
#117653,#117654,#117655,#117656,#117657,#117658,#117659,#117660,#117661,
#117662,#117663,#117664),(#117665,#117666,#117667,#117668,#117669,#117670,
#117671,#117672,#117673,#117674,#117675,#117676,#117677,#117678,#117679)),
 .UNSPECIFIED.,.F.,.F.,.F.)
B_SPLINE_SURFACE_WITH_KNOTS((4,4),(4,1,1,1,1,1,1,1,1,1,1,1,4),(0.,1.),(0.,
0.0993304258737296,0.195288926245669,0.279764193611795,0.357478306071918,
0.437884275258005,0.519144483225908,0.599505042528899,0.680729928008849,
0.764271760028651,0.850469396333162,0.939451116239952,1.),.UNSPECIFIED.)
GEOMETRIC_REPRESENTATION_ITEM()
RATIONAL_B_SPLINE_SURFACE(((1.519035604992,1.519035604992,1.519035604992,
1.519035604992,1.519035604992,1.519035604992,1.519035604992,1.519035604992,
1.519035604992,1.519035604992,1.519035604992,1.519035604992,1.519035604992,
1.519035604992,1.519035604992),(0.8269881316694,0.8269881316694,0.8269881316694,
0.8269881316694,0.8269881316694,0.8269881316694,0.8269881316694,0.8269881316694,
0.8269881316694,0.8269881316694,0.8269881316694,0.8269881316694,0.8269881316694,
0.8269881316694,0.8269881316694),(0.8269881316694,0.8269881316694,0.8269881316694,
0.8269881316694,0.8269881316694,0.8269881316694,0.8269881316694,0.8269881316694,
0.8269881316694,0.8269881316694,0.8269881316694,0.8269881316694,0.8269881316694,
0.8269881316694,0.8269881316694),(1.519035604992,1.519035604992,1.519035604992,
1.519035604992,1.519035604992,1.519035604992,1.519035604992,1.519035604992,
1.519035604992,1.519035604992,1.519035604992,1.519035604992,1.519035604992,
1.519035604992,1.519035604992)))
REPRESENTATION_ITEM('')
SURFACE()
);
#2413=(
BOUNDED_SURFACE()
B_SPLINE_SURFACE(3,3,((#117877,#117878,#117879,#117880,#117881,#117882,
#117883,#117884,#117885),(#117886,#117887,#117888,#117889,#117890,#117891,
#117892,#117893,#117894),(#117895,#117896,#117897,#117898,#117899,#117900,
#117901,#117902,#117903),(#117904,#117905,#117906,#117907,#117908,#117909,
#117910,#117911,#117912)),.UNSPECIFIED.,.F.,.F.,.F.)
B_SPLINE_SURFACE_WITH_KNOTS((4,4),(4,1,1,1,1,1,4),(0.,1.),(0.,0.192791195394506,
0.411717423884289,0.621651126749646,0.812473561049781,0.973652979997317,
1.),.UNSPECIFIED.)
GEOMETRIC_REPRESENTATION_ITEM()
RATIONAL_B_SPLINE_SURFACE(((1.365114458785,1.365114458785,1.365114458785,
1.365114458785,1.365114458785,1.365114458785,1.365114458785,1.365114458785,
1.365114458785),(0.878295180405,0.878295180405,0.878295180405,0.878295180405,
0.878295180405,0.878295180405,0.878295180405,0.878295180405,0.878295180405),
(0.878295180405,0.878295180405,0.878295180405,0.878295180405,0.878295180405,
0.878295180405,0.878295180405,0.878295180405,0.878295180405),(1.365114458785,
1.365114458785,1.365114458785,1.365114458785,1.365114458785,1.365114458785,
1.365114458785,1.365114458785,1.365114458785)))
REPRESENTATION_ITEM('')
SURFACE()
);
#2414=(
BOUNDED_SURFACE()
B_SPLINE_SURFACE(3,3,((#117949,#117950,#117951,#117952,#117953,#117954,
#117955,#117956,#117957,#117958,#117959,#117960,#117961,#117962,#117963,
#117964,#117965),(#117966,#117967,#117968,#117969,#117970,#117971,#117972,
#117973,#117974,#117975,#117976,#117977,#117978,#117979,#117980,#117981,
#117982),(#117983,#117984,#117985,#117986,#117987,#117988,#117989,#117990,
#117991,#117992,#117993,#117994,#117995,#117996,#117997,#117998,#117999),
(#118000,#118001,#118002,#118003,#118004,#118005,#118006,#118007,#118008,
#118009,#118010,#118011,#118012,#118013,#118014,#118015,#118016)),
 .UNSPECIFIED.,.F.,.F.,.F.)
B_SPLINE_SURFACE_WITH_KNOTS((4,4),(4,1,1,1,1,1,1,1,1,1,1,1,1,1,4),(0.,1.),
(0.,0.0494607190127907,0.109552090730043,0.169758737534662,0.230148354533949,
0.290560261854406,0.350306525877549,0.40987255925942,0.472274987329372,
0.540774950770296,0.617873523590501,0.704101656323432,0.799618934750072,
0.904474902078167,1.),.UNSPECIFIED.)
GEOMETRIC_REPRESENTATION_ITEM()
RATIONAL_B_SPLINE_SURFACE(((1.220899718882,1.220899718882,1.220899718882,
1.220899718882,1.220899718882,1.220899718882,1.220899718882,1.220899718882,
1.220899718882,1.220899718882,1.220899718882,1.220899718882,1.220899718882,
1.220899718882,1.220899718882,1.220899718882,1.220899718882),(0.9263667603727,
0.9263667603727,0.9263667603727,0.9263667603727,0.9263667603727,0.9263667603727,
0.9263667603727,0.9263667603727,0.9263667603727,0.9263667603727,0.9263667603727,
0.9263667603727,0.9263667603727,0.9263667603727,0.9263667603727,0.9263667603727,
0.9263667603727),(0.9263667603727,0.9263667603727,0.9263667603727,0.9263667603727,
0.9263667603727,0.9263667603727,0.9263667603727,0.9263667603727,0.9263667603727,
0.9263667603727,0.9263667603727,0.9263667603727,0.9263667603727,0.9263667603727,
0.9263667603727,0.9263667603727,0.9263667603727),(1.220899718882,1.220899718882,
1.220899718882,1.220899718882,1.220899718882,1.220899718882,1.220899718882,
1.220899718882,1.220899718882,1.220899718882,1.220899718882,1.220899718882,
1.220899718882,1.220899718882,1.220899718882,1.220899718882,1.220899718882)))
REPRESENTATION_ITEM('')
SURFACE()
);
#2415=(
BOUNDED_SURFACE()
B_SPLINE_SURFACE(3,3,((#118215,#118216,#118217,#118218,#118219,#118220),
(#118221,#118222,#118223,#118224,#118225,#118226),(#118227,#118228,#118229,
#118230,#118231,#118232),(#118233,#118234,#118235,#118236,#118237,#118238)),
 .UNSPECIFIED.,.F.,.F.,.F.)
B_SPLINE_SURFACE_WITH_KNOTS((4,4),(4,1,1,4),(0.,1.),(0.,0.447612208701937,
0.9386901437205,1.),.UNSPECIFIED.)
GEOMETRIC_REPRESENTATION_ITEM()
RATIONAL_B_SPLINE_SURFACE(((1.132184188967,1.132184188967,1.132184188967,
1.132184188967,1.132184188967,1.132184188967),(0.9559386036777,0.9559386036777,
0.9559386036777,0.9559386036777,0.9559386036777,0.9559386036777),(0.9559386036777,
0.9559386036777,0.9559386036777,0.9559386036777,0.9559386036777,0.9559386036777),
(1.132184188967,1.132184188967,1.132184188967,1.132184188967,1.132184188967,
1.132184188967)))
REPRESENTATION_ITEM('')
SURFACE()
);
#2416=(
BOUNDED_SURFACE()
B_SPLINE_SURFACE(3,3,((#118311,#118312,#118313,#118314,#118315,#118316,
#118317,#118318,#118319,#118320,#118321,#118322,#118323),(#118324,#118325,
#118326,#118327,#118328,#118329,#118330,#118331,#118332,#118333,#118334,
#118335,#118336),(#118337,#118338,#118339,#118340,#118341,#118342,#118343,
#118344,#118345,#118346,#118347,#118348,#118349),(#118350,#118351,#118352,
#118353,#118354,#118355,#118356,#118357,#118358,#118359,#118360,#118361,
#118362)),.UNSPECIFIED.,.F.,.F.,.F.)
B_SPLINE_SURFACE_WITH_KNOTS((4,4),(4,1,1,1,1,1,1,1,1,1,4),(0.,1.),(0.,0.0726579731238688,
0.165540666880435,0.265778081450179,0.365083883521996,0.460784315560169,
0.55478726880033,0.657326573221902,0.774847166279867,0.904679558230862,
1.),.UNSPECIFIED.)
GEOMETRIC_REPRESENTATION_ITEM()
RATIONAL_B_SPLINE_SURFACE(((1.132183962178,1.132183962178,1.132183962178,
1.132183962178,1.132183962178,1.132183962178,1.132183962178,1.132183962178,
1.132183962178,1.132183962178,1.132183962178,1.132183962178,1.132183962178),
(0.955938679274,0.955938679274,0.955938679274,0.955938679274,0.955938679274,
0.955938679274,0.955938679274,0.955938679274,0.955938679274,0.955938679274,
0.955938679274,0.955938679274,0.955938679274),(0.955938679274,0.955938679274,
0.955938679274,0.955938679274,0.955938679274,0.955938679274,0.955938679274,
0.955938679274,0.955938679274,0.955938679274,0.955938679274,0.955938679274,
0.955938679274),(1.132183962178,1.132183962178,1.132183962178,1.132183962178,
1.132183962178,1.132183962178,1.132183962178,1.132183962178,1.132183962178,
1.132183962178,1.132183962178,1.132183962178,1.132183962178)))
REPRESENTATION_ITEM('')
SURFACE()
);
#2417=(
BOUNDED_SURFACE()
B_SPLINE_SURFACE(3,3,((#118632,#118633,#118634,#118635,#118636,#118637,
#118638,#118639,#118640,#118641,#118642,#118643,#118644,#118645,#118646,
#118647,#118648,#118649,#118650,#118651,#118652,#118653),(#118654,#118655,
#118656,#118657,#118658,#118659,#118660,#118661,#118662,#118663,#118664,
#118665,#118666,#118667,#118668,#118669,#118670,#118671,#118672,#118673,
#118674,#118675),(#118676,#118677,#118678,#118679,#118680,#118681,#118682,
#118683,#118684,#118685,#118686,#118687,#118688,#118689,#118690,#118691,
#118692,#118693,#118694,#118695,#118696,#118697),(#118698,#118699,#118700,
#118701,#118702,#118703,#118704,#118705,#118706,#118707,#118708,#118709,
#118710,#118711,#118712,#118713,#118714,#118715,#118716,#118717,#118718,
#118719)),.UNSPECIFIED.,.F.,.F.,.F.)
B_SPLINE_SURFACE_WITH_KNOTS((4,4),(4,1,1,1,1,1,1,1,1,1,1,1,1,1,1,1,1,1,
1,4),(0.,1.),(0.,0.00179852648676455,0.0684134361341035,0.138569448512766,
0.212049560253872,0.281023409010827,0.341871044231178,0.39611355557608,
0.444140369343199,0.487339341535663,0.530585789342856,0.575339323721559,
0.620494040055896,0.664485227938823,0.706756351680787,0.752682439877936,
0.80459823145977,0.863065026247903,0.928980423200659,1.),.UNSPECIFIED.)
GEOMETRIC_REPRESENTATION_ITEM()
RATIONAL_B_SPLINE_SURFACE(((1.255321138723,1.255321138723,1.255321138723,
1.255321138723,1.255321138723,1.255321138723,1.255321138723,1.255321138723,
1.255321138723,1.255321138723,1.255321138723,1.255321138723,1.255321138723,
1.255321138723,1.255321138723,1.255321138723,1.255321138723,1.255321138723,
1.255321138723,1.255321138723,1.255321138723,1.255321138723),(0.914892953759,
0.914892953759,0.914892953759,0.914892953759,0.914892953759,0.914892953759,
0.914892953759,0.914892953759,0.914892953759,0.914892953759,0.914892953759,
0.914892953759,0.914892953759,0.914892953759,0.914892953759,0.914892953759,
0.914892953759,0.914892953759,0.914892953759,0.914892953759,0.914892953759,
0.914892953759),(0.914892953759,0.914892953759,0.914892953759,0.914892953759,
0.914892953759,0.914892953759,0.914892953759,0.914892953759,0.914892953759,
0.914892953759,0.914892953759,0.914892953759,0.914892953759,0.914892953759,
0.914892953759,0.914892953759,0.914892953759,0.914892953759,0.914892953759,
0.914892953759,0.914892953759,0.914892953759),(1.255321138723,1.255321138723,
1.255321138723,1.255321138723,1.255321138723,1.255321138723,1.255321138723,
1.255321138723,1.255321138723,1.255321138723,1.255321138723,1.255321138723,
1.255321138723,1.255321138723,1.255321138723,1.255321138723,1.255321138723,
1.255321138723,1.255321138723,1.255321138723,1.255321138723,1.255321138723)))
REPRESENTATION_ITEM('')
SURFACE()
);
#2418=(
BOUNDED_SURFACE()
B_SPLINE_SURFACE(3,3,((#118976,#118977,#118978,#118979,#118980),(#118981,
#118982,#118983,#118984,#118985),(#118986,#118987,#118988,#118989,#118990),
(#118991,#118992,#118993,#118994,#118995)),.UNSPECIFIED.,.F.,.F.,.F.)
B_SPLINE_SURFACE_WITH_KNOTS((4,4),(4,1,4),(0.,1.),(0.,0.469552763526497,
1.),.UNSPECIFIED.)
GEOMETRIC_REPRESENTATION_ITEM()
RATIONAL_B_SPLINE_SURFACE(((1.365422134914,1.365422134914,1.365422134914,
1.365422134914,1.365422134914),(0.8781926216954,0.8781926216954,0.8781926216954,
0.8781926216954,0.8781926216954),(0.8781926216954,0.8781926216954,0.8781926216954,
0.8781926216954,0.8781926216954),(1.365422134914,1.365422134914,1.365422134914,
1.365422134914,1.365422134914)))
REPRESENTATION_ITEM('')
SURFACE()
);
#2419=(
BOUNDED_SURFACE()
B_SPLINE_SURFACE(3,3,((#119003,#119004,#119005,#119006,#119007,#119008,
#119009,#119010,#119011,#119012,#119013,#119014,#119015,#119016,#119017),
(#119018,#119019,#119020,#119021,#119022,#119023,#119024,#119025,#119026,
#119027,#119028,#119029,#119030,#119031,#119032),(#119033,#119034,#119035,
#119036,#119037,#119038,#119039,#119040,#119041,#119042,#119043,#119044,
#119045,#119046,#119047),(#119048,#119049,#119050,#119051,#119052,#119053,
#119054,#119055,#119056,#119057,#119058,#119059,#119060,#119061,#119062)),
 .UNSPECIFIED.,.F.,.F.,.F.)
B_SPLINE_SURFACE_WITH_KNOTS((4,4),(4,1,1,1,1,1,1,1,1,1,1,1,4),(0.,1.),(0.,
0.0436634499300064,0.166198886318839,0.276683120299012,0.375301849455497,
0.46256216640866,0.540611125333518,0.612179050794216,0.680223368266989,
0.748962133643248,0.825081182648611,0.91081093482415,1.),.UNSPECIFIED.)
GEOMETRIC_REPRESENTATION_ITEM()
RATIONAL_B_SPLINE_SURFACE(((1.351003587175,1.351003587175,1.351003587175,
1.351003587175,1.351003587175,1.351003587175,1.351003587175,1.351003587175,
1.351003587175,1.351003587175,1.351003587175,1.351003587175,1.351003587175,
1.351003587175,1.351003587175),(0.882998804275,0.882998804275,0.882998804275,
0.882998804275,0.882998804275,0.882998804275,0.882998804275,0.882998804275,
0.882998804275,0.882998804275,0.882998804275,0.882998804275,0.882998804275,
0.882998804275,0.882998804275),(0.882998804275,0.882998804275,0.882998804275,
0.882998804275,0.882998804275,0.882998804275,0.882998804275,0.882998804275,
0.882998804275,0.882998804275,0.882998804275,0.882998804275,0.882998804275,
0.882998804275,0.882998804275),(1.351003587175,1.351003587175,1.351003587175,
1.351003587175,1.351003587175,1.351003587175,1.351003587175,1.351003587175,
1.351003587175,1.351003587175,1.351003587175,1.351003587175,1.351003587175,
1.351003587175,1.351003587175)))
REPRESENTATION_ITEM('')
SURFACE()
);
#2420=(
BOUNDED_SURFACE()
B_SPLINE_SURFACE(3,3,((#119272,#119273,#119274,#119275,#119276,#119277,
#119278,#119279,#119280,#119281,#119282,#119283,#119284,#119285,#119286,
#119287,#119288),(#119289,#119290,#119291,#119292,#119293,#119294,#119295,
#119296,#119297,#119298,#119299,#119300,#119301,#119302,#119303,#119304,
#119305),(#119306,#119307,#119308,#119309,#119310,#119311,#119312,#119313,
#119314,#119315,#119316,#119317,#119318,#119319,#119320,#119321,#119322),
(#119323,#119324,#119325,#119326,#119327,#119328,#119329,#119330,#119331,
#119332,#119333,#119334,#119335,#119336,#119337,#119338,#119339)),
 .UNSPECIFIED.,.F.,.F.,.F.)
B_SPLINE_SURFACE_WITH_KNOTS((4,4),(4,1,1,1,1,1,1,1,1,1,1,1,1,1,4),(0.,1.),
(0.,0.0934555018707438,0.190098316562109,0.277412276927369,0.35430591142789,
0.422006518582467,0.485074288423762,0.548771616802643,0.613848873864871,
0.679223443651306,0.742843206526981,0.805944165791561,0.877524725574254,
0.957638281560363,1.),.UNSPECIFIED.)
GEOMETRIC_REPRESENTATION_ITEM()
RATIONAL_B_SPLINE_SURFACE(((1.219577491546,1.219577491546,1.219577491546,
1.219577491546,1.219577491546,1.219577491546,1.219577491546,1.219577491546,
1.219577491546,1.219577491546,1.219577491546,1.219577491546,1.219577491546,
1.219577491546,1.219577491546,1.219577491546,1.219577491546),(0.9268075028179,
0.9268075028179,0.9268075028179,0.9268075028179,0.9268075028179,0.9268075028179,
0.9268075028179,0.9268075028179,0.9268075028179,0.9268075028179,0.9268075028179,
0.9268075028179,0.9268075028179,0.9268075028179,0.9268075028179,0.9268075028179,
0.9268075028179),(0.9268075028179,0.9268075028179,0.9268075028179,0.9268075028179,
0.9268075028179,0.9268075028179,0.9268075028179,0.9268075028179,0.9268075028179,
0.9268075028179,0.9268075028179,0.9268075028179,0.9268075028179,0.9268075028179,
0.9268075028179,0.9268075028179,0.9268075028179),(1.219577491546,1.219577491546,
1.219577491546,1.219577491546,1.219577491546,1.219577491546,1.219577491546,
1.219577491546,1.219577491546,1.219577491546,1.219577491546,1.219577491546,
1.219577491546,1.219577491546,1.219577491546,1.219577491546,1.219577491546)))
REPRESENTATION_ITEM('')
SURFACE()
);
#2421=(
BOUNDED_SURFACE()
B_SPLINE_SURFACE(3,3,((#119374,#119375,#119376,#119377,#119378,#119379,
#119380,#119381,#119382,#119383,#119384,#119385),(#119386,#119387,#119388,
#119389,#119390,#119391,#119392,#119393,#119394,#119395,#119396,#119397),
(#119398,#119399,#119400,#119401,#119402,#119403,#119404,#119405,#119406,
#119407,#119408,#119409),(#119410,#119411,#119412,#119413,#119414,#119415,
#119416,#119417,#119418,#119419,#119420,#119421)),.UNSPECIFIED.,.F.,.F.,
 .F.)
B_SPLINE_SURFACE_WITH_KNOTS((4,4),(4,1,1,1,1,1,1,1,1,4),(0.,1.),(0.,0.0491574788676924,
0.219592918841423,0.374383193798209,0.513141463206398,0.639408605121616,
0.757222110220193,0.870630976300795,0.983497613603143,1.),.UNSPECIFIED.)
GEOMETRIC_REPRESENTATION_ITEM()
RATIONAL_B_SPLINE_SURFACE(((1.035729017359,1.035729017359,1.035729017359,
1.035729017359,1.035729017359,1.035729017359,1.035729017359,1.035729017359,
1.035729017359,1.035729017359,1.035729017359,1.035729017359),(0.988090327547,
0.988090327547,0.988090327547,0.988090327547,0.988090327547,0.988090327547,
0.988090327547,0.988090327547,0.988090327547,0.988090327547,0.988090327547,
0.988090327547),(0.988090327547,0.988090327547,0.988090327547,0.988090327547,
0.988090327547,0.988090327547,0.988090327547,0.988090327547,0.988090327547,
0.988090327547,0.988090327547,0.988090327547),(1.035729017359,1.035729017359,
1.035729017359,1.035729017359,1.035729017359,1.035729017359,1.035729017359,
1.035729017359,1.035729017359,1.035729017359,1.035729017359,1.035729017359)))
REPRESENTATION_ITEM('')
SURFACE()
);
#2422=(
BOUNDED_SURFACE()
B_SPLINE_SURFACE(3,3,((#119834,#119835,#119836,#119837,#119838,#119839,
#119840,#119841,#119842),(#119843,#119844,#119845,#119846,#119847,#119848,
#119849,#119850,#119851),(#119852,#119853,#119854,#119855,#119856,#119857,
#119858,#119859,#119860),(#119861,#119862,#119863,#119864,#119865,#119866,
#119867,#119868,#119869)),.UNSPECIFIED.,.F.,.F.,.F.)
B_SPLINE_SURFACE_WITH_KNOTS((4,4),(4,1,1,1,1,1,4),(0.,1.),(0.,0.124217072598013,
0.310755649966071,0.499972699325182,0.689255533447521,0.875770604197989,
1.),.UNSPECIFIED.)
GEOMETRIC_REPRESENTATION_ITEM()
RATIONAL_B_SPLINE_SURFACE(((1.043303594112,1.043303594112,1.043303594112,
1.043303594112,1.043303594112,1.043303594112,1.043303594112,1.043303594112,
1.043303594112),(0.9855654686295,0.9855654686295,0.9855654686295,0.9855654686295,
0.9855654686295,0.9855654686295,0.9855654686295,0.9855654686295,0.9855654686295),
(0.9855654686295,0.9855654686295,0.9855654686295,0.9855654686295,0.9855654686295,
0.9855654686295,0.9855654686295,0.9855654686295,0.9855654686295),(1.043303594112,
1.043303594112,1.043303594112,1.043303594112,1.043303594112,1.043303594112,
1.043303594112,1.043303594112,1.043303594112)))
REPRESENTATION_ITEM('')
SURFACE()
);
#2423=(
BOUNDED_SURFACE()
B_SPLINE_SURFACE(3,3,((#119949,#119950,#119951,#119952,#119953,#119954),
(#119955,#119956,#119957,#119958,#119959,#119960),(#119961,#119962,#119963,
#119964,#119965,#119966),(#119967,#119968,#119969,#119970,#119971,#119972)),
 .UNSPECIFIED.,.F.,.F.,.F.)
B_SPLINE_SURFACE_WITH_KNOTS((4,4),(4,1,1,4),(0.,1.),(0.,0.290351630545127,
0.6856968431484,1.),.UNSPECIFIED.)
GEOMETRIC_REPRESENTATION_ITEM()
RATIONAL_B_SPLINE_SURFACE(((1.04998815347,1.04998815347,1.04998815347,1.04998815347,
1.04998815347,1.04998815347),(0.9833372821767,0.9833372821767,0.9833372821767,
0.9833372821767,0.9833372821767,0.9833372821767),(0.9833372821767,0.9833372821767,
0.9833372821767,0.9833372821767,0.9833372821767,0.9833372821767),(1.04998815347,
1.04998815347,1.04998815347,1.04998815347,1.04998815347,1.04998815347)))
REPRESENTATION_ITEM('')
SURFACE()
);
#2424=(
BOUNDED_SURFACE()
B_SPLINE_SURFACE(3,3,((#119986,#119987,#119988,#119989,#119990,#119991,
#119992,#119993,#119994,#119995,#119996,#119997,#119998,#119999,#120000,
#120001,#120002,#120003,#120004,#120005,#120006,#120007,#120008,#120009,
#120010,#120011),(#120012,#120013,#120014,#120015,#120016,#120017,#120018,
#120019,#120020,#120021,#120022,#120023,#120024,#120025,#120026,#120027,
#120028,#120029,#120030,#120031,#120032,#120033,#120034,#120035,#120036,
#120037),(#120038,#120039,#120040,#120041,#120042,#120043,#120044,#120045,
#120046,#120047,#120048,#120049,#120050,#120051,#120052,#120053,#120054,
#120055,#120056,#120057,#120058,#120059,#120060,#120061,#120062,#120063),
(#120064,#120065,#120066,#120067,#120068,#120069,#120070,#120071,#120072,
#120073,#120074,#120075,#120076,#120077,#120078,#120079,#120080,#120081,
#120082,#120083,#120084,#120085,#120086,#120087,#120088,#120089)),
 .UNSPECIFIED.,.F.,.F.,.F.)
B_SPLINE_SURFACE_WITH_KNOTS((4,4),(4,1,1,1,1,1,1,1,1,1,1,1,1,1,1,1,1,1,
1,1,1,1,1,4),(0.,1.),(0.,0.0604690860171424,0.125750773183185,0.184471262697933,
0.23763259918399,0.285727129729686,0.328587237304838,0.367339669645258,
0.404193671801395,0.441150852354512,0.478525964786371,0.515930821440246,
0.552912972270284,0.589583703038061,0.62782560752874,0.669834379167559,
0.716144402441833,0.760844285447638,0.806281350038666,0.853281683657045,
0.900484124800725,0.947112731733202,0.993172991216528,1.),.UNSPECIFIED.)
GEOMETRIC_REPRESENTATION_ITEM()
RATIONAL_B_SPLINE_SURFACE(((1.050211534691,1.050211534691,1.050211534691,
1.050211534691,1.050211534691,1.050211534691,1.050211534691,1.050211534691,
1.050211534691,1.050211534691,1.050211534691,1.050211534691,1.050211534691,
1.050211534691,1.050211534691,1.050211534691,1.050211534691,1.050211534691,
1.050211534691,1.050211534691,1.050211534691,1.050211534691,1.050211534691,
1.050211534691,1.050211534691,1.050211534691),(0.9832628217698,0.9832628217698,
0.9832628217698,0.9832628217698,0.9832628217698,0.9832628217698,0.9832628217698,
0.9832628217698,0.9832628217698,0.9832628217698,0.9832628217698,0.9832628217698,
0.9832628217698,0.9832628217698,0.9832628217698,0.9832628217698,0.9832628217698,
0.9832628217698,0.9832628217698,0.9832628217698,0.9832628217698,0.9832628217698,
0.9832628217698,0.9832628217698,0.9832628217698,0.9832628217698),(0.9832628217698,
0.9832628217698,0.9832628217698,0.9832628217698,0.9832628217698,0.9832628217698,
0.9832628217698,0.9832628217698,0.9832628217698,0.9832628217698,0.9832628217698,
0.9832628217698,0.9832628217698,0.9832628217698,0.9832628217698,0.9832628217698,
0.9832628217698,0.9832628217698,0.9832628217698,0.9832628217698,0.9832628217698,
0.9832628217698,0.9832628217698,0.9832628217698,0.9832628217698,0.9832628217698),
(1.050211534691,1.050211534691,1.050211534691,1.050211534691,1.050211534691,
1.050211534691,1.050211534691,1.050211534691,1.050211534691,1.050211534691,
1.050211534691,1.050211534691,1.050211534691,1.050211534691,1.050211534691,
1.050211534691,1.050211534691,1.050211534691,1.050211534691,1.050211534691,
1.050211534691,1.050211534691,1.050211534691,1.050211534691,1.050211534691,
1.050211534691)))
REPRESENTATION_ITEM('')
SURFACE()
);
#2425=(
BOUNDED_SURFACE()
B_SPLINE_SURFACE(3,3,((#120354,#120355,#120356,#120357,#120358,#120359,
#120360,#120361),(#120362,#120363,#120364,#120365,#120366,#120367,#120368,
#120369),(#120370,#120371,#120372,#120373,#120374,#120375,#120376,#120377),
(#120378,#120379,#120380,#120381,#120382,#120383,#120384,#120385)),
 .UNSPECIFIED.,.F.,.F.,.F.)
B_SPLINE_SURFACE_WITH_KNOTS((4,4),(4,1,1,1,1,4),(0.,1.),(0.,0.115906347737713,
0.324457197714345,0.557614394200552,0.816082473111432,1.),.UNSPECIFIED.)
GEOMETRIC_REPRESENTATION_ITEM()
RATIONAL_B_SPLINE_SURFACE(((1.04998793531,1.04998793531,1.04998793531,1.04998793531,
1.04998793531,1.04998793531,1.04998793531,1.04998793531),(0.9833373548966,
0.9833373548966,0.9833373548966,0.9833373548966,0.9833373548966,0.9833373548966,
0.9833373548966,0.9833373548966),(0.9833373548966,0.9833373548966,0.9833373548966,
0.9833373548966,0.9833373548966,0.9833373548966,0.9833373548966,0.9833373548966),
(1.04998793531,1.04998793531,1.04998793531,1.04998793531,1.04998793531,
1.04998793531,1.04998793531,1.04998793531)))
REPRESENTATION_ITEM('')
SURFACE()
);
#2426=(
BOUNDED_SURFACE()
B_SPLINE_SURFACE(3,3,((#120428,#120429,#120430,#120431,#120432,#120433),
(#120434,#120435,#120436,#120437,#120438,#120439),(#120440,#120441,#120442,
#120443,#120444,#120445),(#120446,#120447,#120448,#120449,#120450,#120451)),
 .UNSPECIFIED.,.F.,.F.,.F.)
B_SPLINE_SURFACE_WITH_KNOTS((4,4),(4,1,1,4),(0.,1.),(0.,0.261439365657105,
0.646008272416107,1.),.UNSPECIFIED.)
GEOMETRIC_REPRESENTATION_ITEM()
RATIONAL_B_SPLINE_SURFACE(((1.043303932823,1.043303932823,1.043303932823,
1.043303932823,1.043303932823,1.043303932823),(0.9855653557257,0.9855653557257,
0.9855653557257,0.9855653557257,0.9855653557257,0.9855653557257),(0.9855653557257,
0.9855653557257,0.9855653557257,0.9855653557257,0.9855653557257,0.9855653557257),
(1.043303932823,1.043303932823,1.043303932823,1.043303932823,1.043303932823,
1.043303932823)))
REPRESENTATION_ITEM('')
SURFACE()
);
#2427=(
BOUNDED_SURFACE()
B_SPLINE_SURFACE(3,3,((#120512,#120513,#120514,#120515,#120516,#120517),
(#120518,#120519,#120520,#120521,#120522,#120523),(#120524,#120525,#120526,
#120527,#120528,#120529),(#120530,#120531,#120532,#120533,#120534,#120535)),
 .UNSPECIFIED.,.F.,.F.,.F.)
B_SPLINE_SURFACE_WITH_KNOTS((4,4),(4,1,1,4),(0.,1.),(0.,0.338411219840004,
0.730847710170391,1.),.UNSPECIFIED.)
GEOMETRIC_REPRESENTATION_ITEM()
RATIONAL_B_SPLINE_SURFACE(((1.043304304122,1.043304304122,1.043304304122,
1.043304304122,1.043304304122,1.043304304122),(0.9855652319594,0.9855652319594,
0.9855652319594,0.9855652319594,0.9855652319594,0.9855652319594),(0.9855652319594,
0.9855652319594,0.9855652319594,0.9855652319594,0.9855652319594,0.9855652319594),
(1.043304304122,1.043304304122,1.043304304122,1.043304304122,1.043304304122,
1.043304304122)))
REPRESENTATION_ITEM('')
SURFACE()
);
#2428=(
BOUNDED_SURFACE()
B_SPLINE_SURFACE(3,3,((#120599,#120600,#120601,#120602,#120603,#120604,
#120605,#120606,#120607),(#120608,#120609,#120610,#120611,#120612,#120613,
#120614,#120615,#120616),(#120617,#120618,#120619,#120620,#120621,#120622,
#120623,#120624,#120625),(#120626,#120627,#120628,#120629,#120630,#120631,
#120632,#120633,#120634)),.UNSPECIFIED.,.F.,.F.,.F.)
B_SPLINE_SURFACE_WITH_KNOTS((4,4),(4,1,1,1,1,1,4),(0.,1.),(0.,0.145600865509264,
0.314399883400269,0.481396351840591,0.652048510615264,0.82890573043304,
1.),.UNSPECIFIED.)
GEOMETRIC_REPRESENTATION_ITEM()
RATIONAL_B_SPLINE_SURFACE(((1.057416537047,1.057416537047,1.057416537047,
1.057416537047,1.057416537047,1.057416537047,1.057416537047,1.057416537047,
1.057416537047),(0.9808611543175,0.9808611543175,0.9808611543175,0.9808611543175,
0.9808611543175,0.9808611543175,0.9808611543175,0.9808611543175,0.9808611543175),
(0.9808611543175,0.9808611543175,0.9808611543175,0.9808611543175,0.9808611543175,
0.9808611543175,0.9808611543175,0.9808611543175,0.9808611543175),(1.057416537047,
1.057416537047,1.057416537047,1.057416537047,1.057416537047,1.057416537047,
1.057416537047,1.057416537047,1.057416537047)))
REPRESENTATION_ITEM('')
SURFACE()
);
#2429=(
BOUNDED_SURFACE()
B_SPLINE_SURFACE(3,3,((#120749,#120750,#120751,#120752,#120753,#120754,
#120755,#120756,#120757),(#120758,#120759,#120760,#120761,#120762,#120763,
#120764,#120765,#120766),(#120767,#120768,#120769,#120770,#120771,#120772,
#120773,#120774,#120775),(#120776,#120777,#120778,#120779,#120780,#120781,
#120782,#120783,#120784)),.UNSPECIFIED.,.F.,.F.,.F.)
B_SPLINE_SURFACE_WITH_KNOTS((4,4),(4,1,1,1,1,1,4),(0.,1.),(0.,0.145967497811959,
0.326469868263455,0.503631939312401,0.67673102833901,0.85125569646002,1.),
 .UNSPECIFIED.)
GEOMETRIC_REPRESENTATION_ITEM()
RATIONAL_B_SPLINE_SURFACE(((1.057410488177,1.057410488177,1.057410488177,
1.057410488177,1.057410488177,1.057410488177,1.057410488177,1.057410488177,
1.057410488177),(0.9808631706077,0.9808631706077,0.9808631706077,0.9808631706077,
0.9808631706077,0.9808631706077,0.9808631706077,0.9808631706077,0.9808631706077),
(0.9808631706077,0.9808631706077,0.9808631706077,0.9808631706077,0.9808631706077,
0.9808631706077,0.9808631706077,0.9808631706077,0.9808631706077),(1.057410488177,
1.057410488177,1.057410488177,1.057410488177,1.057410488177,1.057410488177,
1.057410488177,1.057410488177,1.057410488177)))
REPRESENTATION_ITEM('')
SURFACE()
);
#2430=(
BOUNDED_SURFACE()
B_SPLINE_SURFACE(3,3,((#120879,#120880,#120881,#120882,#120883,#120884,
#120885,#120886,#120887,#120888),(#120889,#120890,#120891,#120892,#120893,
#120894,#120895,#120896,#120897,#120898),(#120899,#120900,#120901,#120902,
#120903,#120904,#120905,#120906,#120907,#120908),(#120909,#120910,#120911,
#120912,#120913,#120914,#120915,#120916,#120917,#120918),(#120919,#120920,
#120921,#120922,#120923,#120924,#120925,#120926,#120927,#120928),(#120929,
#120930,#120931,#120932,#120933,#120934,#120935,#120936,#120937,#120938),
(#120939,#120940,#120941,#120942,#120943,#120944,#120945,#120946,#120947,
#120948)),.UNSPECIFIED.,.F.,.F.,.F.)
B_SPLINE_SURFACE_WITH_KNOTS((4,3,4),(4,1,1,1,1,1,1,4),(0.,0.5,1.),(0.,0.161025004538591,
0.369602103221435,0.554126466977726,0.718053106645468,0.864942898489644,
0.996691241096418,1.),.UNSPECIFIED.)
GEOMETRIC_REPRESENTATION_ITEM()
RATIONAL_B_SPLINE_SURFACE(((1.201213809876,1.201213809876,1.201213809876,
1.201213809876,1.201213809876,1.201213809876,1.201213809876,1.201213809876,
1.201213809876,1.201213809876),(0.9329287300413,0.9329287300413,0.9329287300413,
0.9329287300413,0.9329287300413,0.9329287300413,0.9329287300413,0.9329287300413,
0.9329287300413,0.9329287300413),(0.9329287300413,0.9329287300413,0.9329287300413,
0.9329287300413,0.9329287300413,0.9329287300413,0.9329287300413,0.9329287300413,
0.9329287300413,0.9329287300413),(1.201213809876,1.201213809876,1.201213809876,
1.201213809876,1.201213809876,1.201213809876,1.201213809876,1.201213809876,
1.201213809876,1.201213809876),(0.9329287300413,0.9329287300413,0.9329287300413,
0.9329287300413,0.9329287300413,0.9329287300413,0.9329287300413,0.9329287300413,
0.9329287300413,0.9329287300413),(0.9329287300413,0.9329287300413,0.9329287300413,
0.9329287300413,0.9329287300413,0.9329287300413,0.9329287300413,0.9329287300413,
0.9329287300413,0.9329287300413),(1.201213809876,1.201213809876,1.201213809876,
1.201213809876,1.201213809876,1.201213809876,1.201213809876,1.201213809876,
1.201213809876,1.201213809876)))
REPRESENTATION_ITEM('')
SURFACE()
);
#2431=(
BOUNDED_SURFACE()
B_SPLINE_SURFACE(3,3,((#121035,#121036,#121037,#121038,#121039,#121040,
#121041,#121042,#121043,#121044),(#121045,#121046,#121047,#121048,#121049,
#121050,#121051,#121052,#121053,#121054),(#121055,#121056,#121057,#121058,
#121059,#121060,#121061,#121062,#121063,#121064),(#121065,#121066,#121067,
#121068,#121069,#121070,#121071,#121072,#121073,#121074),(#121075,#121076,
#121077,#121078,#121079,#121080,#121081,#121082,#121083,#121084),(#121085,
#121086,#121087,#121088,#121089,#121090,#121091,#121092,#121093,#121094),
(#121095,#121096,#121097,#121098,#121099,#121100,#121101,#121102,#121103,
#121104)),.UNSPECIFIED.,.F.,.F.,.F.)
B_SPLINE_SURFACE_WITH_KNOTS((4,3,4),(4,1,1,1,1,1,1,4),(0.,0.5,1.),(0.,0.00259132042105358,
0.133683284416713,0.278707201971115,0.438527579442401,0.616079075546092,
0.815708952652196,1.),.UNSPECIFIED.)
GEOMETRIC_REPRESENTATION_ITEM()
RATIONAL_B_SPLINE_SURFACE(((1.201171733823,1.201171733823,1.201171733823,
1.201171733823,1.201171733823,1.201171733823,1.201171733823,1.201171733823,
1.201171733823,1.201171733823),(0.9329427553922,0.9329427553922,0.9329427553922,
0.9329427553922,0.9329427553922,0.9329427553922,0.9329427553922,0.9329427553922,
0.9329427553922,0.9329427553922),(0.9329427553922,0.9329427553922,0.9329427553922,
0.9329427553922,0.9329427553922,0.9329427553922,0.9329427553922,0.9329427553922,
0.9329427553922,0.9329427553922),(1.201171733823,1.201171733823,1.201171733823,
1.201171733823,1.201171733823,1.201171733823,1.201171733823,1.201171733823,
1.201171733823,1.201171733823),(0.9329427553922,0.9329427553922,0.9329427553922,
0.9329427553922,0.9329427553922,0.9329427553922,0.9329427553922,0.9329427553922,
0.9329427553922,0.9329427553922),(0.9329427553922,0.9329427553922,0.9329427553922,
0.9329427553922,0.9329427553922,0.9329427553922,0.9329427553922,0.9329427553922,
0.9329427553922,0.9329427553922),(1.201171733823,1.201171733823,1.201171733823,
1.201171733823,1.201171733823,1.201171733823,1.201171733823,1.201171733823,
1.201171733823,1.201171733823)))
REPRESENTATION_ITEM('')
SURFACE()
);
#2432=(
BOUNDED_SURFACE()
B_SPLINE_SURFACE(3,3,((#121106,#121107,#121108,#121109,#121110,#121111,
#121112,#121113,#121114,#121115,#121116,#121117),(#121118,#121119,#121120,
#121121,#121122,#121123,#121124,#121125,#121126,#121127,#121128,#121129),
(#121130,#121131,#121132,#121133,#121134,#121135,#121136,#121137,#121138,
#121139,#121140,#121141),(#121142,#121143,#121144,#121145,#121146,#121147,
#121148,#121149,#121150,#121151,#121152,#121153),(#121154,#121155,#121156,
#121157,#121158,#121159,#121160,#121161,#121162,#121163,#121164,#121165),
(#121166,#121167,#121168,#121169,#121170,#121171,#121172,#121173,#121174,
#121175,#121176,#121177),(#121178,#121179,#121180,#121181,#121182,#121183,
#121184,#121185,#121186,#121187,#121188,#121189)),.UNSPECIFIED.,.F.,.F.,
 .F.)
B_SPLINE_SURFACE_WITH_KNOTS((4,3,4),(4,1,1,1,1,1,1,1,1,4),(0.,0.5,1.),(0.,
0.000255491591619197,0.127239783683594,0.253487500080297,0.379079641346161,
0.504106145120676,0.628664885620248,0.752853160032759,0.87675838090237,
1.),.UNSPECIFIED.)
GEOMETRIC_REPRESENTATION_ITEM()
RATIONAL_B_SPLINE_SURFACE(((1.193844362293,1.193844362293,1.193844362293,
1.193844362293,1.193844362293,1.193844362293,1.193844362293,1.193844362293,
1.193844362293,1.193844362293,1.193844362293,1.193844362293),(0.9353852125691,
0.9353852125691,0.9353852125691,0.9353852125691,0.9353852125691,0.9353852125691,
0.9353852125691,0.9353852125691,0.9353852125691,0.9353852125691,0.9353852125691,
0.9353852125691),(0.9353852125691,0.9353852125691,0.9353852125691,0.9353852125691,
0.9353852125691,0.9353852125691,0.9353852125691,0.9353852125691,0.9353852125691,
0.9353852125691,0.9353852125691,0.9353852125691),(1.193844362293,1.193844362293,
1.193844362293,1.193844362293,1.193844362293,1.193844362293,1.193844362293,
1.193844362293,1.193844362293,1.193844362293,1.193844362293,1.193844362293),
(0.9353852125691,0.9353852125691,0.9353852125691,0.9353852125691,0.9353852125691,
0.9353852125691,0.9353852125691,0.9353852125691,0.9353852125691,0.9353852125691,
0.9353852125691,0.9353852125691),(0.9353852125691,0.9353852125691,0.9353852125691,
0.9353852125691,0.9353852125691,0.9353852125691,0.9353852125691,0.9353852125691,
0.9353852125691,0.9353852125691,0.9353852125691,0.9353852125691),(1.193844362293,
1.193844362293,1.193844362293,1.193844362293,1.193844362293,1.193844362293,
1.193844362293,1.193844362293,1.193844362293,1.193844362293,1.193844362293,
1.193844362293)))
REPRESENTATION_ITEM('')
SURFACE()
);
#2433=(
BOUNDED_SURFACE()
B_SPLINE_SURFACE(3,3,((#121191,#121192,#121193,#121194,#121195,#121196,
#121197,#121198,#121199,#121200,#121201,#121202,#121203,#121204,#121205,
#121206,#121207,#121208,#121209,#121210,#121211,#121212,#121213,#121214,
#121215,#121216,#121217,#121218,#121219,#121220,#121221,#121222,#121223,
#121224),(#121225,#121226,#121227,#121228,#121229,#121230,#121231,#121232,
#121233,#121234,#121235,#121236,#121237,#121238,#121239,#121240,#121241,
#121242,#121243,#121244,#121245,#121246,#121247,#121248,#121249,#121250,
#121251,#121252,#121253,#121254,#121255,#121256,#121257,#121258),(#121259,
#121260,#121261,#121262,#121263,#121264,#121265,#121266,#121267,#121268,
#121269,#121270,#121271,#121272,#121273,#121274,#121275,#121276,#121277,
#121278,#121279,#121280,#121281,#121282,#121283,#121284,#121285,#121286,
#121287,#121288,#121289,#121290,#121291,#121292),(#121293,#121294,#121295,
#121296,#121297,#121298,#121299,#121300,#121301,#121302,#121303,#121304,
#121305,#121306,#121307,#121308,#121309,#121310,#121311,#121312,#121313,
#121314,#121315,#121316,#121317,#121318,#121319,#121320,#121321,#121322,
#121323,#121324,#121325,#121326),(#121327,#121328,#121329,#121330,#121331,
#121332,#121333,#121334,#121335,#121336,#121337,#121338,#121339,#121340,
#121341,#121342,#121343,#121344,#121345,#121346,#121347,#121348,#121349,
#121350,#121351,#121352,#121353,#121354,#121355,#121356,#121357,#121358,
#121359,#121360),(#121361,#121362,#121363,#121364,#121365,#121366,#121367,
#121368,#121369,#121370,#121371,#121372,#121373,#121374,#121375,#121376,
#121377,#121378,#121379,#121380,#121381,#121382,#121383,#121384,#121385,
#121386,#121387,#121388,#121389,#121390,#121391,#121392,#121393,#121394),
(#121395,#121396,#121397,#121398,#121399,#121400,#121401,#121402,#121403,
#121404,#121405,#121406,#121407,#121408,#121409,#121410,#121411,#121412,
#121413,#121414,#121415,#121416,#121417,#121418,#121419,#121420,#121421,
#121422,#121423,#121424,#121425,#121426,#121427,#121428)),.UNSPECIFIED.,
 .F.,.F.,.F.)
B_SPLINE_SURFACE_WITH_KNOTS((4,3,4),(4,1,1,1,1,1,1,1,1,1,1,1,1,1,1,1,1,
1,1,1,1,1,1,1,1,1,1,1,1,1,1,4),(0.,0.5,1.),(0.,0.00390411019570353,0.0280798877427953,
0.0549594760925253,0.084482057830751,0.116603170427511,0.15129817037668,
0.188488834966683,0.227507129809145,0.267411106706363,0.307272885523456,
0.346360547263377,0.385850664440005,0.42467066457681,0.461154766662463,
0.495850904898193,0.529827873260416,0.564306064772395,0.600347337077154,
0.637306063447508,0.674154674464573,0.71211198969174,0.750908172946504,
0.789490910831634,0.826793915174607,0.861784930834985,0.894042278866944,
0.923582402081779,0.950408852900018,0.974512143542049,0.995871943984923,
1.),.UNSPECIFIED.)
GEOMETRIC_REPRESENTATION_ITEM()
RATIONAL_B_SPLINE_SURFACE(((1.182964165402,1.182964165402,1.182964165402,
1.182964165402,1.182964165402,1.182964165402,1.182964165402,1.182964165402,
1.182964165402,1.182964165402,1.182964165402,1.182964165402,1.182964165402,
1.182964165402,1.182964165402,1.182964165402,1.182964165402,1.182964165402,
1.182964165402,1.182964165402,1.182964165402,1.182964165402,1.182964165402,
1.182964165402,1.182964165402,1.182964165402,1.182964165402,1.182964165402,
1.182964165402,1.182964165402,1.182964165402,1.182964165402,1.182964165402,
1.182964165402),(0.9390119448661,0.9390119448661,0.9390119448661,0.9390119448661,
0.9390119448661,0.9390119448661,0.9390119448661,0.9390119448661,0.9390119448661,
0.9390119448661,0.9390119448661,0.9390119448661,0.9390119448661,0.9390119448661,
0.9390119448661,0.9390119448661,0.9390119448661,0.9390119448661,0.9390119448661,
0.9390119448661,0.9390119448661,0.9390119448661,0.9390119448661,0.9390119448661,
0.9390119448661,0.9390119448661,0.9390119448661,0.9390119448661,0.9390119448661,
0.9390119448661,0.9390119448661,0.9390119448661,0.9390119448661,0.9390119448661),
(0.9390119448661,0.9390119448661,0.9390119448661,0.9390119448661,0.9390119448661,
0.9390119448661,0.9390119448661,0.9390119448661,0.9390119448661,0.9390119448661,
0.9390119448661,0.9390119448661,0.9390119448661,0.9390119448661,0.9390119448661,
0.9390119448661,0.9390119448661,0.9390119448661,0.9390119448661,0.9390119448661,
0.9390119448661,0.9390119448661,0.9390119448661,0.9390119448661,0.9390119448661,
0.9390119448661,0.9390119448661,0.9390119448661,0.9390119448661,0.9390119448661,
0.9390119448661,0.9390119448661,0.9390119448661,0.9390119448661),(1.182964165402,
1.182964165402,1.182964165402,1.182964165402,1.182964165402,1.182964165402,
1.182964165402,1.182964165402,1.182964165402,1.182964165402,1.182964165402,
1.182964165402,1.182964165402,1.182964165402,1.182964165402,1.182964165402,
1.182964165402,1.182964165402,1.182964165402,1.182964165402,1.182964165402,
1.182964165402,1.182964165402,1.182964165402,1.182964165402,1.182964165402,
1.182964165402,1.182964165402,1.182964165402,1.182964165402,1.182964165402,
1.182964165402,1.182964165402,1.182964165402),(0.9390119448661,0.9390119448661,
0.9390119448661,0.9390119448661,0.9390119448661,0.9390119448661,0.9390119448661,
0.9390119448661,0.9390119448661,0.9390119448661,0.9390119448661,0.9390119448661,
0.9390119448661,0.9390119448661,0.9390119448661,0.9390119448661,0.9390119448661,
0.9390119448661,0.9390119448661,0.9390119448661,0.9390119448661,0.9390119448661,
0.9390119448661,0.9390119448661,0.9390119448661,0.9390119448661,0.9390119448661,
0.9390119448661,0.9390119448661,0.9390119448661,0.9390119448661,0.9390119448661,
0.9390119448661,0.9390119448661),(0.9390119448661,0.9390119448661,0.9390119448661,
0.9390119448661,0.9390119448661,0.9390119448661,0.9390119448661,0.9390119448661,
0.9390119448661,0.9390119448661,0.9390119448661,0.9390119448661,0.9390119448661,
0.9390119448661,0.9390119448661,0.9390119448661,0.9390119448661,0.9390119448661,
0.9390119448661,0.9390119448661,0.9390119448661,0.9390119448661,0.9390119448661,
0.9390119448661,0.9390119448661,0.9390119448661,0.9390119448661,0.9390119448661,
0.9390119448661,0.9390119448661,0.9390119448661,0.9390119448661,0.9390119448661,
0.9390119448661),(1.182964165402,1.182964165402,1.182964165402,1.182964165402,
1.182964165402,1.182964165402,1.182964165402,1.182964165402,1.182964165402,
1.182964165402,1.182964165402,1.182964165402,1.182964165402,1.182964165402,
1.182964165402,1.182964165402,1.182964165402,1.182964165402,1.182964165402,
1.182964165402,1.182964165402,1.182964165402,1.182964165402,1.182964165402,
1.182964165402,1.182964165402,1.182964165402,1.182964165402,1.182964165402,
1.182964165402,1.182964165402,1.182964165402,1.182964165402,1.182964165402)))
REPRESENTATION_ITEM('')
SURFACE()
);
#2434=(
BOUNDED_SURFACE()
B_SPLINE_SURFACE(3,3,((#121430,#121431,#121432,#121433,#121434,#121435,
#121436,#121437,#121438,#121439,#121440,#121441),(#121442,#121443,#121444,
#121445,#121446,#121447,#121448,#121449,#121450,#121451,#121452,#121453),
(#121454,#121455,#121456,#121457,#121458,#121459,#121460,#121461,#121462,
#121463,#121464,#121465),(#121466,#121467,#121468,#121469,#121470,#121471,
#121472,#121473,#121474,#121475,#121476,#121477),(#121478,#121479,#121480,
#121481,#121482,#121483,#121484,#121485,#121486,#121487,#121488,#121489),
(#121490,#121491,#121492,#121493,#121494,#121495,#121496,#121497,#121498,
#121499,#121500,#121501),(#121502,#121503,#121504,#121505,#121506,#121507,
#121508,#121509,#121510,#121511,#121512,#121513)),.UNSPECIFIED.,.F.,.F.,
 .F.)
B_SPLINE_SURFACE_WITH_KNOTS((4,3,4),(4,1,1,1,1,1,1,1,1,4),(0.,0.5,1.),(0.,
0.121577744739987,0.2454785297075,0.369661120308666,0.494217098932518,0.61923924716235,
0.744819531284461,0.871051615748787,0.998028327089304,1.),.UNSPECIFIED.)
GEOMETRIC_REPRESENTATION_ITEM()
RATIONAL_B_SPLINE_SURFACE(((1.193843399739,1.193843399739,1.193843399739,
1.193843399739,1.193843399739,1.193843399739,1.193843399739,1.193843399739,
1.193843399739,1.193843399739,1.193843399739,1.193843399739),(0.9353855334202,
0.9353855334202,0.9353855334202,0.9353855334202,0.9353855334202,0.9353855334202,
0.9353855334202,0.9353855334202,0.9353855334202,0.9353855334202,0.9353855334202,
0.9353855334202),(0.9353855334202,0.9353855334202,0.9353855334202,0.9353855334202,
0.9353855334202,0.9353855334202,0.9353855334202,0.9353855334202,0.9353855334202,
0.9353855334202,0.9353855334202,0.9353855334202),(1.193843399739,1.193843399739,
1.193843399739,1.193843399739,1.193843399739,1.193843399739,1.193843399739,
1.193843399739,1.193843399739,1.193843399739,1.193843399739,1.193843399739),
(0.9353855334202,0.9353855334202,0.9353855334202,0.9353855334202,0.9353855334202,
0.9353855334202,0.9353855334202,0.9353855334202,0.9353855334202,0.9353855334202,
0.9353855334202,0.9353855334202),(0.9353855334202,0.9353855334202,0.9353855334202,
0.9353855334202,0.9353855334202,0.9353855334202,0.9353855334202,0.9353855334202,
0.9353855334202,0.9353855334202,0.9353855334202,0.9353855334202),(1.193843399739,
1.193843399739,1.193843399739,1.193843399739,1.193843399739,1.193843399739,
1.193843399739,1.193843399739,1.193843399739,1.193843399739,1.193843399739,
1.193843399739)))
REPRESENTATION_ITEM('')
SURFACE()
);
#2435=(
BOUNDED_SURFACE()
B_SPLINE_SURFACE(3,3,((#121515,#121516,#121517,#121518,#121519,#121520,
#121521,#121522,#121523,#121524),(#121525,#121526,#121527,#121528,#121529,
#121530,#121531,#121532,#121533,#121534),(#121535,#121536,#121537,#121538,
#121539,#121540,#121541,#121542,#121543,#121544),(#121545,#121546,#121547,
#121548,#121549,#121550,#121551,#121552,#121553,#121554),(#121555,#121556,
#121557,#121558,#121559,#121560,#121561,#121562,#121563,#121564),(#121565,
#121566,#121567,#121568,#121569,#121570,#121571,#121572,#121573,#121574),
(#121575,#121576,#121577,#121578,#121579,#121580,#121581,#121582,#121583,
#121584)),.UNSPECIFIED.,.F.,.F.,.F.)
B_SPLINE_SURFACE_WITH_KNOTS((4,3,4),(4,1,1,1,1,1,1,4),(0.,0.5,1.),(0.,0.213585163989469,
0.405450323624376,0.577282704132798,0.731642183256355,0.871392511498999,
0.997433055266827,1.),.UNSPECIFIED.)
GEOMETRIC_REPRESENTATION_ITEM()
RATIONAL_B_SPLINE_SURFACE(((1.201113977633,1.201113977633,1.201113977633,
1.201113977633,1.201113977633,1.201113977633,1.201113977633,1.201113977633,
1.201113977633,1.201113977633),(0.9329620074556,0.9329620074556,0.9329620074556,
0.9329620074556,0.9329620074556,0.9329620074556,0.9329620074556,0.9329620074556,
0.9329620074556,0.9329620074556),(0.9329620074556,0.9329620074556,0.9329620074556,
0.9329620074556,0.9329620074556,0.9329620074556,0.9329620074556,0.9329620074556,
0.9329620074556,0.9329620074556),(1.201113977633,1.201113977633,1.201113977633,
1.201113977633,1.201113977633,1.201113977633,1.201113977633,1.201113977633,
1.201113977633,1.201113977633),(0.9329620074556,0.9329620074556,0.9329620074556,
0.9329620074556,0.9329620074556,0.9329620074556,0.9329620074556,0.9329620074556,
0.9329620074556,0.9329620074556),(0.9329620074556,0.9329620074556,0.9329620074556,
0.9329620074556,0.9329620074556,0.9329620074556,0.9329620074556,0.9329620074556,
0.9329620074556,0.9329620074556),(1.201113977633,1.201113977633,1.201113977633,
1.201113977633,1.201113977633,1.201113977633,1.201113977633,1.201113977633,
1.201113977633,1.201113977633)))
REPRESENTATION_ITEM('')
SURFACE()
);
#2436=(
BOUNDED_SURFACE()
B_SPLINE_SURFACE(3,3,((#121603,#121604,#121605,#121606,#121607,#121608,
#121609,#121610,#121611,#121612,#121613),(#121614,#121615,#121616,#121617,
#121618,#121619,#121620,#121621,#121622,#121623,#121624),(#121625,#121626,
#121627,#121628,#121629,#121630,#121631,#121632,#121633,#121634,#121635),
(#121636,#121637,#121638,#121639,#121640,#121641,#121642,#121643,#121644,
#121645,#121646),(#121647,#121648,#121649,#121650,#121651,#121652,#121653,
#121654,#121655,#121656,#121657),(#121658,#121659,#121660,#121661,#121662,
#121663,#121664,#121665,#121666,#121667,#121668),(#121669,#121670,#121671,
#121672,#121673,#121674,#121675,#121676,#121677,#121678,#121679)),
 .UNSPECIFIED.,.F.,.F.,.F.)
B_SPLINE_SURFACE_WITH_KNOTS((4,3,4),(4,1,1,1,1,1,1,1,4),(0.,0.5,1.),(0.,
0.00181797331928698,0.105490767602339,0.219958045817536,0.345909152683817,
0.484805134723122,0.638614040911334,0.809850477822227,1.),.UNSPECIFIED.)
GEOMETRIC_REPRESENTATION_ITEM()
RATIONAL_B_SPLINE_SURFACE(((1.201132896331,1.201132896331,1.201132896331,
1.201132896331,1.201132896331,1.201132896331,1.201132896331,1.201132896331,
1.201132896331,1.201132896331,1.201132896331),(0.932955701223,0.932955701223,
0.932955701223,0.932955701223,0.932955701223,0.932955701223,0.932955701223,
0.932955701223,0.932955701223,0.932955701223,0.932955701223),(0.932955701223,
0.932955701223,0.932955701223,0.932955701223,0.932955701223,0.932955701223,
0.932955701223,0.932955701223,0.932955701223,0.932955701223,0.932955701223),
(1.201132896331,1.201132896331,1.201132896331,1.201132896331,1.201132896331,
1.201132896331,1.201132896331,1.201132896331,1.201132896331,1.201132896331,
1.201132896331),(0.932955701223,0.932955701223,0.932955701223,0.932955701223,
0.932955701223,0.932955701223,0.932955701223,0.932955701223,0.932955701223,
0.932955701223,0.932955701223),(0.932955701223,0.932955701223,0.932955701223,
0.932955701223,0.932955701223,0.932955701223,0.932955701223,0.932955701223,
0.932955701223,0.932955701223,0.932955701223),(1.201132896331,1.201132896331,
1.201132896331,1.201132896331,1.201132896331,1.201132896331,1.201132896331,
1.201132896331,1.201132896331,1.201132896331,1.201132896331)))
REPRESENTATION_ITEM('')
SURFACE()
);
#2437=(
BOUNDED_SURFACE()
B_SPLINE_SURFACE(3,3,((#121681,#121682,#121683,#121684,#121685,#121686,
#121687,#121688,#121689),(#121690,#121691,#121692,#121693,#121694,#121695,
#121696,#121697,#121698),(#121699,#121700,#121701,#121702,#121703,#121704,
#121705,#121706,#121707),(#121708,#121709,#121710,#121711,#121712,#121713,
#121714,#121715,#121716),(#121717,#121718,#121719,#121720,#121721,#121722,
#121723,#121724,#121725),(#121726,#121727,#121728,#121729,#121730,#121731,
#121732,#121733,#121734),(#121735,#121736,#121737,#121738,#121739,#121740,
#121741,#121742,#121743)),.UNSPECIFIED.,.F.,.F.,.F.)
B_SPLINE_SURFACE_WITH_KNOTS((4,3,4),(4,1,1,1,1,1,4),(0.,0.5,1.),(0.,0.146812258466779,
0.312562551467087,0.499888765632735,0.688675725217384,0.852980904228354,
1.),.UNSPECIFIED.)
GEOMETRIC_REPRESENTATION_ITEM()
RATIONAL_B_SPLINE_SURFACE(((1.193840868885,1.193840868885,1.193840868885,
1.193840868885,1.193840868885,1.193840868885,1.193840868885,1.193840868885,
1.193840868885),(0.9353863770384,0.9353863770384,0.9353863770384,0.9353863770384,
0.9353863770384,0.9353863770384,0.9353863770384,0.9353863770384,0.9353863770384),
(0.9353863770384,0.9353863770384,0.9353863770384,0.9353863770384,0.9353863770384,
0.9353863770384,0.9353863770384,0.9353863770384,0.9353863770384),(1.193840868885,
1.193840868885,1.193840868885,1.193840868885,1.193840868885,1.193840868885,
1.193840868885,1.193840868885,1.193840868885),(0.9353863770384,0.9353863770384,
0.9353863770384,0.9353863770384,0.9353863770384,0.9353863770384,0.9353863770384,
0.9353863770384,0.9353863770384),(0.9353863770384,0.9353863770384,0.9353863770384,
0.9353863770384,0.9353863770384,0.9353863770384,0.9353863770384,0.9353863770384,
0.9353863770384),(1.193840868885,1.193840868885,1.193840868885,1.193840868885,
1.193840868885,1.193840868885,1.193840868885,1.193840868885,1.193840868885)))
REPRESENTATION_ITEM('')
SURFACE()
);
#2438=(
BOUNDED_SURFACE()
B_SPLINE_SURFACE(3,3,((#121820,#121821,#121822,#121823,#121824,#121825,
#121826,#121827,#121828,#121829,#121830,#121831),(#121832,#121833,#121834,
#121835,#121836,#121837,#121838,#121839,#121840,#121841,#121842,#121843),
(#121844,#121845,#121846,#121847,#121848,#121849,#121850,#121851,#121852,
#121853,#121854,#121855),(#121856,#121857,#121858,#121859,#121860,#121861,
#121862,#121863,#121864,#121865,#121866,#121867),(#121868,#121869,#121870,
#121871,#121872,#121873,#121874,#121875,#121876,#121877,#121878,#121879),
(#121880,#121881,#121882,#121883,#121884,#121885,#121886,#121887,#121888,
#121889,#121890,#121891),(#121892,#121893,#121894,#121895,#121896,#121897,
#121898,#121899,#121900,#121901,#121902,#121903)),.UNSPECIFIED.,.F.,.F.,
 .F.)
B_SPLINE_SURFACE_WITH_KNOTS((4,3,4),(4,1,1,1,1,1,1,1,1,4),(0.,0.5,1.),(0.,
0.1150816828504,0.247731000070067,0.394496984674143,0.542441014806786,0.677432974789258,
0.797298327727755,0.903511214341264,0.999875262137635,1.),.UNSPECIFIED.)
GEOMETRIC_REPRESENTATION_ITEM()
RATIONAL_B_SPLINE_SURFACE(((1.193841606841,1.193841606841,1.193841606841,
1.193841606841,1.193841606841,1.193841606841,1.193841606841,1.193841606841,
1.193841606841,1.193841606841,1.193841606841,1.193841606841),(0.9353861310531,
0.9353861310531,0.9353861310531,0.9353861310531,0.9353861310531,0.9353861310531,
0.9353861310531,0.9353861310531,0.9353861310531,0.9353861310531,0.9353861310531,
0.9353861310531),(0.9353861310531,0.9353861310531,0.9353861310531,0.9353861310531,
0.9353861310531,0.9353861310531,0.9353861310531,0.9353861310531,0.9353861310531,
0.9353861310531,0.9353861310531,0.9353861310531),(1.193841606841,1.193841606841,
1.193841606841,1.193841606841,1.193841606841,1.193841606841,1.193841606841,
1.193841606841,1.193841606841,1.193841606841,1.193841606841,1.193841606841),
(0.9353861310531,0.9353861310531,0.9353861310531,0.9353861310531,0.9353861310531,
0.9353861310531,0.9353861310531,0.9353861310531,0.9353861310531,0.9353861310531,
0.9353861310531,0.9353861310531),(0.9353861310531,0.9353861310531,0.9353861310531,
0.9353861310531,0.9353861310531,0.9353861310531,0.9353861310531,0.9353861310531,
0.9353861310531,0.9353861310531,0.9353861310531,0.9353861310531),(1.193841606841,
1.193841606841,1.193841606841,1.193841606841,1.193841606841,1.193841606841,
1.193841606841,1.193841606841,1.193841606841,1.193841606841,1.193841606841,
1.193841606841)))
REPRESENTATION_ITEM('')
SURFACE()
);
#2439=(
BOUNDED_SURFACE()
B_SPLINE_SURFACE(3,3,((#123619,#123620,#123621,#123622,#123623,#123624,
#123625,#123626),(#123627,#123628,#123629,#123630,#123631,#123632,#123633,
#123634),(#123635,#123636,#123637,#123638,#123639,#123640,#123641,#123642),
(#123643,#123644,#123645,#123646,#123647,#123648,#123649,#123650)),
 .UNSPECIFIED.,.F.,.F.,.F.)
B_SPLINE_SURFACE_WITH_KNOTS((4,4),(4,1,1,1,1,4),(0.,1.),(0.,0.0246171264152833,
0.291238908164661,0.592562353394222,0.933298045148062,1.),.UNSPECIFIED.)
GEOMETRIC_REPRESENTATION_ITEM()
RATIONAL_B_SPLINE_SURFACE(((1.155702096291,1.155702096291,1.155702096291,
1.155702096291,1.155702096291,1.155702096291,1.155702096291,1.155702096291),
(0.9480993012362,0.9480993012362,0.9480993012362,0.9480993012362,0.9480993012362,
0.9480993012362,0.9480993012362,0.9480993012362),(0.9480993012362,0.9480993012362,
0.9480993012362,0.9480993012362,0.9480993012362,0.9480993012362,0.9480993012362,
0.9480993012362),(1.155702096291,1.155702096291,1.155702096291,1.155702096291,
1.155702096291,1.155702096291,1.155702096291,1.155702096291)))
REPRESENTATION_ITEM('')
SURFACE()
);
#2440=(
BOUNDED_SURFACE()
B_SPLINE_SURFACE(3,3,((#123749,#123750,#123751,#123752,#123753,#123754,
#123755,#123756,#123757,#123758,#123759,#123760,#123761,#123762,#123763),
(#123764,#123765,#123766,#123767,#123768,#123769,#123770,#123771,#123772,
#123773,#123774,#123775,#123776,#123777,#123778),(#123779,#123780,#123781,
#123782,#123783,#123784,#123785,#123786,#123787,#123788,#123789,#123790,
#123791,#123792,#123793),(#123794,#123795,#123796,#123797,#123798,#123799,
#123800,#123801,#123802,#123803,#123804,#123805,#123806,#123807,#123808)),
 .UNSPECIFIED.,.F.,.F.,.F.)
B_SPLINE_SURFACE_WITH_KNOTS((4,4),(4,1,1,1,1,1,1,1,1,1,1,1,4),(0.,1.),(0.,
0.0727177819492164,0.16359452595188,0.250961907386609,0.334788546033315,
0.415442620198573,0.49511203377138,0.575859115958059,0.655273963838798,
0.731996243944222,0.814480068027282,0.906324996644106,1.),.UNSPECIFIED.)
GEOMETRIC_REPRESENTATION_ITEM()
RATIONAL_B_SPLINE_SURFACE(((1.519033843966,1.519033843966,1.519033843966,
1.519033843966,1.519033843966,1.519033843966,1.519033843966,1.519033843966,
1.519033843966,1.519033843966,1.519033843966,1.519033843966,1.519033843966,
1.519033843966,1.519033843966),(0.8269887186781,0.8269887186781,0.8269887186781,
0.8269887186781,0.8269887186781,0.8269887186781,0.8269887186781,0.8269887186781,
0.8269887186781,0.8269887186781,0.8269887186781,0.8269887186781,0.8269887186781,
0.8269887186781,0.8269887186781),(0.8269887186781,0.8269887186781,0.8269887186781,
0.8269887186781,0.8269887186781,0.8269887186781,0.8269887186781,0.8269887186781,
0.8269887186781,0.8269887186781,0.8269887186781,0.8269887186781,0.8269887186781,
0.8269887186781,0.8269887186781),(1.519033843966,1.519033843966,1.519033843966,
1.519033843966,1.519033843966,1.519033843966,1.519033843966,1.519033843966,
1.519033843966,1.519033843966,1.519033843966,1.519033843966,1.519033843966,
1.519033843966,1.519033843966)))
REPRESENTATION_ITEM('')
SURFACE()
);
#2441=(
BOUNDED_SURFACE()
B_SPLINE_SURFACE(3,3,((#124103,#124104,#124105,#124106,#124107,#124108,
#124109,#124110,#124111,#124112),(#124113,#124114,#124115,#124116,#124117,
#124118,#124119,#124120,#124121,#124122),(#124123,#124124,#124125,#124126,
#124127,#124128,#124129,#124130,#124131,#124132),(#124133,#124134,#124135,
#124136,#124137,#124138,#124139,#124140,#124141,#124142)),.UNSPECIFIED.,
 .F.,.F.,.F.)
B_SPLINE_SURFACE_WITH_KNOTS((4,4),(4,1,1,1,1,1,1,4),(0.,1.),(0.,0.0442218692304281,
0.265842058411036,0.466113430548006,0.645383516910958,0.805695668205441,
0.948933238513881,1.),.UNSPECIFIED.)
GEOMETRIC_REPRESENTATION_ITEM()
RATIONAL_B_SPLINE_SURFACE(((1.365422972509,1.365422972509,1.365422972509,
1.365422972509,1.365422972509,1.365422972509,1.365422972509,1.365422972509,
1.365422972509,1.365422972509),(0.878192342497,0.878192342497,0.878192342497,
0.878192342497,0.878192342497,0.878192342497,0.878192342497,0.878192342497,
0.878192342497,0.878192342497),(0.878192342497,0.878192342497,0.878192342497,
0.878192342497,0.878192342497,0.878192342497,0.878192342497,0.878192342497,
0.878192342497,0.878192342497),(1.365422972509,1.365422972509,1.365422972509,
1.365422972509,1.365422972509,1.365422972509,1.365422972509,1.365422972509,
1.365422972509,1.365422972509)))
REPRESENTATION_ITEM('')
SURFACE()
);
#2442=(
BOUNDED_SURFACE()
B_SPLINE_SURFACE(3,3,((#124201,#124202,#124203,#124204,#124205,#124206,
#124207,#124208,#124209,#124210,#124211,#124212,#124213,#124214,#124215),
(#124216,#124217,#124218,#124219,#124220,#124221,#124222,#124223,#124224,
#124225,#124226,#124227,#124228,#124229,#124230),(#124231,#124232,#124233,
#124234,#124235,#124236,#124237,#124238,#124239,#124240,#124241,#124242,
#124243,#124244,#124245),(#124246,#124247,#124248,#124249,#124250,#124251,
#124252,#124253,#124254,#124255,#124256,#124257,#124258,#124259,#124260)),
 .UNSPECIFIED.,.F.,.F.,.F.)
B_SPLINE_SURFACE_WITH_KNOTS((4,4),(4,1,1,1,1,1,1,1,1,1,1,1,4),(0.,1.),(0.,
0.0084168370653201,0.153296921706747,0.285251477789455,0.405485980176222,
0.5143437021125,0.612495974405379,0.700795271015088,0.780077840916837,0.851172072538887,
0.914904276103888,0.972101275929351,1.),.UNSPECIFIED.)
GEOMETRIC_REPRESENTATION_ITEM()
RATIONAL_B_SPLINE_SURFACE(((1.250208738268,1.250208738268,1.250208738268,
1.250208738268,1.250208738268,1.250208738268,1.250208738268,1.250208738268,
1.250208738268,1.250208738268,1.250208738268,1.250208738268,1.250208738268,
1.250208738268,1.250208738268),(0.916597087244,0.916597087244,0.916597087244,
0.916597087244,0.916597087244,0.916597087244,0.916597087244,0.916597087244,
0.916597087244,0.916597087244,0.916597087244,0.916597087244,0.916597087244,
0.916597087244,0.916597087244),(0.916597087244,0.916597087244,0.916597087244,
0.916597087244,0.916597087244,0.916597087244,0.916597087244,0.916597087244,
0.916597087244,0.916597087244,0.916597087244,0.916597087244,0.916597087244,
0.916597087244,0.916597087244),(1.250208738268,1.250208738268,1.250208738268,
1.250208738268,1.250208738268,1.250208738268,1.250208738268,1.250208738268,
1.250208738268,1.250208738268,1.250208738268,1.250208738268,1.250208738268,
1.250208738268,1.250208738268)))
REPRESENTATION_ITEM('')
SURFACE()
);
#2443=(
BOUNDED_SURFACE()
B_SPLINE_SURFACE(3,3,((#124437,#124438,#124439,#124440,#124441,#124442),
(#124443,#124444,#124445,#124446,#124447,#124448),(#124449,#124450,#124451,
#124452,#124453,#124454),(#124455,#124456,#124457,#124458,#124459,#124460)),
 .UNSPECIFIED.,.F.,.F.,.F.)
B_SPLINE_SURFACE_WITH_KNOTS((4,4),(4,1,1,4),(0.,1.),(0.,0.0668296872169646,
0.628269522946755,1.),.UNSPECIFIED.)
GEOMETRIC_REPRESENTATION_ITEM()
RATIONAL_B_SPLINE_SURFACE(((1.365416977784,1.365416977784,1.365416977784,
1.365416977784,1.365416977784,1.365416977784),(0.8781943407385,0.8781943407385,
0.8781943407385,0.8781943407385,0.8781943407385,0.8781943407385),(0.8781943407385,
0.8781943407385,0.8781943407385,0.8781943407385,0.8781943407385,0.8781943407385),
(1.365416977784,1.365416977784,1.365416977784,1.365416977784,1.365416977784,
1.365416977784)))
REPRESENTATION_ITEM('')
SURFACE()
);
#2444=(
BOUNDED_SURFACE()
B_SPLINE_SURFACE(3,3,((#124474,#124475,#124476,#124477,#124478,#124479,
#124480,#124481,#124482,#124483,#124484,#124485,#124486,#124487,#124488),
(#124489,#124490,#124491,#124492,#124493,#124494,#124495,#124496,#124497,
#124498,#124499,#124500,#124501,#124502,#124503),(#124504,#124505,#124506,
#124507,#124508,#124509,#124510,#124511,#124512,#124513,#124514,#124515,
#124516,#124517,#124518),(#124519,#124520,#124521,#124522,#124523,#124524,
#124525,#124526,#124527,#124528,#124529,#124530,#124531,#124532,#124533)),
 .UNSPECIFIED.,.F.,.F.,.F.)
B_SPLINE_SURFACE_WITH_KNOTS((4,4),(4,1,1,1,1,1,1,1,1,1,1,1,4),(0.,1.),(0.,
0.100036646536872,0.223693703070815,0.335641994831635,0.437371524654234,
0.529770444704687,0.614003043110945,0.692082215426747,0.767474713817308,
0.84177692890213,0.916098301259391,0.991595887369207,1.),.UNSPECIFIED.)
GEOMETRIC_REPRESENTATION_ITEM()
RATIONAL_B_SPLINE_SURFACE(((1.293938210524,1.293938210524,1.293938210524,
1.293938210524,1.293938210524,1.293938210524,1.293938210524,1.293938210524,
1.293938210524,1.293938210524,1.293938210524,1.293938210524,1.293938210524,
1.293938210524,1.293938210524),(0.9020205964919,0.9020205964919,0.9020205964919,
0.9020205964919,0.9020205964919,0.9020205964919,0.9020205964919,0.9020205964919,
0.9020205964919,0.9020205964919,0.9020205964919,0.9020205964919,0.9020205964919,
0.9020205964919,0.9020205964919),(0.9020205964919,0.9020205964919,0.9020205964919,
0.9020205964919,0.9020205964919,0.9020205964919,0.9020205964919,0.9020205964919,
0.9020205964919,0.9020205964919,0.9020205964919,0.9020205964919,0.9020205964919,
0.9020205964919,0.9020205964919),(1.293938210524,1.293938210524,1.293938210524,
1.293938210524,1.293938210524,1.293938210524,1.293938210524,1.293938210524,
1.293938210524,1.293938210524,1.293938210524,1.293938210524,1.293938210524,
1.293938210524,1.293938210524)))
REPRESENTATION_ITEM('')
SURFACE()
);
#2445=(
BOUNDED_SURFACE()
B_SPLINE_SURFACE(3,3,((#124740,#124741,#124742,#124743,#124744,#124745,
#124746,#124747),(#124748,#124749,#124750,#124751,#124752,#124753,#124754,
#124755),(#124756,#124757,#124758,#124759,#124760,#124761,#124762,#124763),
(#124764,#124765,#124766,#124767,#124768,#124769,#124770,#124771)),
 .UNSPECIFIED.,.F.,.F.,.F.)
B_SPLINE_SURFACE_WITH_KNOTS((4,4),(4,1,1,1,1,4),(0.,1.),(0.,0.156651639089242,
0.358591440264207,0.564674709448518,0.789411493920748,1.),.UNSPECIFIED.)
GEOMETRIC_REPRESENTATION_ITEM()
RATIONAL_B_SPLINE_SURFACE(((1.12003765321,1.12003765321,1.12003765321,1.12003765321,
1.12003765321,1.12003765321,1.12003765321,1.12003765321),(0.9599874489302,
0.9599874489302,0.9599874489302,0.9599874489302,0.9599874489302,0.9599874489302,
0.9599874489302,0.9599874489302),(0.9599874489302,0.9599874489302,0.9599874489302,
0.9599874489302,0.9599874489302,0.9599874489302,0.9599874489302,0.9599874489302),
(1.12003765321,1.12003765321,1.12003765321,1.12003765321,1.12003765321,
1.12003765321,1.12003765321,1.12003765321)))
REPRESENTATION_ITEM('')
SURFACE()
);
#2446=(
BOUNDED_SURFACE()
B_SPLINE_SURFACE(3,3,((#124774,#124775,#124776,#124777,#124778,#124779,
#124780,#124781,#124782,#124783,#124784,#124785,#124786,#124787,#124788,
#124789,#124790),(#124791,#124792,#124793,#124794,#124795,#124796,#124797,
#124798,#124799,#124800,#124801,#124802,#124803,#124804,#124805,#124806,
#124807),(#124808,#124809,#124810,#124811,#124812,#124813,#124814,#124815,
#124816,#124817,#124818,#124819,#124820,#124821,#124822,#124823,#124824),
(#124825,#124826,#124827,#124828,#124829,#124830,#124831,#124832,#124833,
#124834,#124835,#124836,#124837,#124838,#124839,#124840,#124841)),
 .UNSPECIFIED.,.F.,.F.,.F.)
B_SPLINE_SURFACE_WITH_KNOTS((4,4),(4,1,1,1,1,1,1,1,1,1,1,1,1,1,4),(0.,1.),
(0.,0.0956146431540125,0.200570336486981,0.29617085639003,0.382446369780954,
0.459533334763256,0.527981368507571,0.590340486919798,0.649866246025106,
0.709565784246277,0.769912468560832,0.830222740675431,0.890369247895391,
0.9504555950694,1.),.UNSPECIFIED.)
GEOMETRIC_REPRESENTATION_ITEM()
RATIONAL_B_SPLINE_SURFACE(((1.220899632035,1.220899632035,1.220899632035,
1.220899632035,1.220899632035,1.220899632035,1.220899632035,1.220899632035,
1.220899632035,1.220899632035,1.220899632035,1.220899632035,1.220899632035,
1.220899632035,1.220899632035,1.220899632035,1.220899632035),(0.9263667893217,
0.9263667893217,0.9263667893217,0.9263667893217,0.9263667893217,0.9263667893217,
0.9263667893217,0.9263667893217,0.9263667893217,0.9263667893217,0.9263667893217,
0.9263667893217,0.9263667893217,0.9263667893217,0.9263667893217,0.9263667893217,
0.9263667893217),(0.9263667893217,0.9263667893217,0.9263667893217,0.9263667893217,
0.9263667893217,0.9263667893217,0.9263667893217,0.9263667893217,0.9263667893217,
0.9263667893217,0.9263667893217,0.9263667893217,0.9263667893217,0.9263667893217,
0.9263667893217,0.9263667893217,0.9263667893217),(1.220899632035,1.220899632035,
1.220899632035,1.220899632035,1.220899632035,1.220899632035,1.220899632035,
1.220899632035,1.220899632035,1.220899632035,1.220899632035,1.220899632035,
1.220899632035,1.220899632035,1.220899632035,1.220899632035,1.220899632035)))
REPRESENTATION_ITEM('')
SURFACE()
);
#2447=(
BOUNDED_SURFACE()
B_SPLINE_SURFACE(3,3,((#125007,#125008,#125009,#125010,#125011,#125012,
#125013,#125014,#125015,#125016),(#125017,#125018,#125019,#125020,#125021,
#125022,#125023,#125024,#125025,#125026),(#125027,#125028,#125029,#125030,
#125031,#125032,#125033,#125034,#125035,#125036),(#125037,#125038,#125039,
#125040,#125041,#125042,#125043,#125044,#125045,#125046)),.UNSPECIFIED.,
 .F.,.F.,.F.)
B_SPLINE_SURFACE_WITH_KNOTS((4,4),(4,1,1,1,1,1,1,4),(0.,1.),(0.,0.0291077785832009,
0.175697498314966,0.342920964150671,0.52427955765036,0.713524484672767,
0.905557751001572,1.),.UNSPECIFIED.)
GEOMETRIC_REPRESENTATION_ITEM()
RATIONAL_B_SPLINE_SURFACE(((1.365112687886,1.365112687886,1.365112687886,
1.365112687886,1.365112687886,1.365112687886,1.365112687886,1.365112687886,
1.365112687886,1.365112687886),(0.8782957707048,0.8782957707048,0.8782957707048,
0.8782957707048,0.8782957707048,0.8782957707048,0.8782957707048,0.8782957707048,
0.8782957707048,0.8782957707048),(0.8782957707048,0.8782957707048,0.8782957707048,
0.8782957707048,0.8782957707048,0.8782957707048,0.8782957707048,0.8782957707048,
0.8782957707048,0.8782957707048),(1.365112687886,1.365112687886,1.365112687886,
1.365112687886,1.365112687886,1.365112687886,1.365112687886,1.365112687886,
1.365112687886,1.365112687886)))
REPRESENTATION_ITEM('')
SURFACE()
);
#2448=(
BOUNDED_SURFACE()
B_SPLINE_SURFACE(3,3,((#125089,#125090,#125091,#125092,#125093),(#125094,
#125095,#125096,#125097,#125098),(#125099,#125100,#125101,#125102,#125103),
(#125104,#125105,#125106,#125107,#125108)),.UNSPECIFIED.,.F.,.F.,.F.)
B_SPLINE_SURFACE_WITH_KNOTS((4,4),(4,1,4),(0.,1.),(0.,0.328690768122142,
1.),.UNSPECIFIED.)
GEOMETRIC_REPRESENTATION_ITEM()
RATIONAL_B_SPLINE_SURFACE(((1.365414096237,1.365414096237,1.365414096237,
1.365414096237,1.365414096237),(0.8781953012543,0.8781953012543,0.8781953012543,
0.8781953012543,0.8781953012543),(0.8781953012543,0.8781953012543,0.8781953012543,
0.8781953012543,0.8781953012543),(1.365414096237,1.365414096237,1.365414096237,
1.365414096237,1.365414096237)))
REPRESENTATION_ITEM('')
SURFACE()
);
#2449=(
BOUNDED_SURFACE()
B_SPLINE_SURFACE(3,3,((#125118,#125119,#125120,#125121,#125122,#125123,
#125124,#125125,#125126,#125127,#125128,#125129,#125130,#125131,#125132,
#125133,#125134,#125135,#125136,#125137),(#125138,#125139,#125140,#125141,
#125142,#125143,#125144,#125145,#125146,#125147,#125148,#125149,#125150,
#125151,#125152,#125153,#125154,#125155,#125156,#125157),(#125158,#125159,
#125160,#125161,#125162,#125163,#125164,#125165,#125166,#125167,#125168,
#125169,#125170,#125171,#125172,#125173,#125174,#125175,#125176,#125177),
(#125178,#125179,#125180,#125181,#125182,#125183,#125184,#125185,#125186,
#125187,#125188,#125189,#125190,#125191,#125192,#125193,#125194,#125195,
#125196,#125197)),.UNSPECIFIED.,.F.,.F.,.F.)
B_SPLINE_SURFACE_WITH_KNOTS((4,4),(4,1,1,1,1,1,1,1,1,1,1,1,1,1,1,1,1,4),
(0.,1.),(0.,0.0437810757388625,0.14954997921505,0.246647238721872,0.335632768061324,
0.417102216875795,0.491694466527586,0.560145818346898,0.623130978563885,
0.681070799832575,0.734496942850944,0.783914635620664,0.829348379595357,
0.870873757986737,0.909008250330309,0.944496730233535,0.978199195579797,
1.),.UNSPECIFIED.)
GEOMETRIC_REPRESENTATION_ITEM()
RATIONAL_B_SPLINE_SURFACE(((1.350953897201,1.350953897201,1.350953897201,
1.350953897201,1.350953897201,1.350953897201,1.350953897201,1.350953897201,
1.350953897201,1.350953897201,1.350953897201,1.350953897201,1.350953897201,
1.350953897201,1.350953897201,1.350953897201,1.350953897201,1.350953897201,
1.350953897201,1.350953897201),(0.8830153675996,0.8830153675996,0.8830153675996,
0.8830153675996,0.8830153675996,0.8830153675996,0.8830153675996,0.8830153675996,
0.8830153675996,0.8830153675996,0.8830153675996,0.8830153675996,0.8830153675996,
0.8830153675996,0.8830153675996,0.8830153675996,0.8830153675996,0.8830153675996,
0.8830153675996,0.8830153675996),(0.8830153675996,0.8830153675996,0.8830153675996,
0.8830153675996,0.8830153675996,0.8830153675996,0.8830153675996,0.8830153675996,
0.8830153675996,0.8830153675996,0.8830153675996,0.8830153675996,0.8830153675996,
0.8830153675996,0.8830153675996,0.8830153675996,0.8830153675996,0.8830153675996,
0.8830153675996,0.8830153675996),(1.350953897201,1.350953897201,1.350953897201,
1.350953897201,1.350953897201,1.350953897201,1.350953897201,1.350953897201,
1.350953897201,1.350953897201,1.350953897201,1.350953897201,1.350953897201,
1.350953897201,1.350953897201,1.350953897201,1.350953897201,1.350953897201,
1.350953897201,1.350953897201)))
REPRESENTATION_ITEM('')
SURFACE()
);
#2450=(
BOUNDED_SURFACE()
B_SPLINE_SURFACE(3,3,((#125421,#125422,#125423,#125424,#125425,#125426,
#125427,#125428,#125429,#125430,#125431,#125432,#125433,#125434,#125435,
#125436,#125437,#125438,#125439,#125440,#125441,#125442),(#125443,#125444,
#125445,#125446,#125447,#125448,#125449,#125450,#125451,#125452,#125453,
#125454,#125455,#125456,#125457,#125458,#125459,#125460,#125461,#125462,
#125463,#125464),(#125465,#125466,#125467,#125468,#125469,#125470,#125471,
#125472,#125473,#125474,#125475,#125476,#125477,#125478,#125479,#125480,
#125481,#125482,#125483,#125484,#125485,#125486),(#125487,#125488,#125489,
#125490,#125491,#125492,#125493,#125494,#125495,#125496,#125497,#125498,
#125499,#125500,#125501,#125502,#125503,#125504,#125505,#125506,#125507,
#125508)),.UNSPECIFIED.,.F.,.F.,.F.)
B_SPLINE_SURFACE_WITH_KNOTS((4,4),(4,1,1,1,1,1,1,1,1,1,1,1,1,1,1,1,1,1,
1,4),(0.,1.),(0.,0.0711383255328258,0.137163359302248,0.195720435393546,
0.247715273019436,0.293698370802659,0.336008737306656,0.380005256943101,
0.425168878602564,0.469947554154179,0.513213820955286,0.55641075188751,
0.604436817371917,0.658671873052936,0.719515049298376,0.788488856663347,
0.862062739446009,0.932266724631227,0.998927768427254,1.),.UNSPECIFIED.)
GEOMETRIC_REPRESENTATION_ITEM()
RATIONAL_B_SPLINE_SURFACE(((1.255321345493,1.255321345493,1.255321345493,
1.255321345493,1.255321345493,1.255321345493,1.255321345493,1.255321345493,
1.255321345493,1.255321345493,1.255321345493,1.255321345493,1.255321345493,
1.255321345493,1.255321345493,1.255321345493,1.255321345493,1.255321345493,
1.255321345493,1.255321345493,1.255321345493,1.255321345493),(0.9148928848357,
0.9148928848357,0.9148928848357,0.9148928848357,0.9148928848357,0.9148928848357,
0.9148928848357,0.9148928848357,0.9148928848357,0.9148928848357,0.9148928848357,
0.9148928848357,0.9148928848357,0.9148928848357,0.9148928848357,0.9148928848357,
0.9148928848357,0.9148928848357,0.9148928848357,0.9148928848357,0.9148928848357,
0.9148928848357),(0.9148928848357,0.9148928848357,0.9148928848357,0.9148928848357,
0.9148928848357,0.9148928848357,0.9148928848357,0.9148928848357,0.9148928848357,
0.9148928848357,0.9148928848357,0.9148928848357,0.9148928848357,0.9148928848357,
0.9148928848357,0.9148928848357,0.9148928848357,0.9148928848357,0.9148928848357,
0.9148928848357,0.9148928848357,0.9148928848357),(1.255321345493,1.255321345493,
1.255321345493,1.255321345493,1.255321345493,1.255321345493,1.255321345493,
1.255321345493,1.255321345493,1.255321345493,1.255321345493,1.255321345493,
1.255321345493,1.255321345493,1.255321345493,1.255321345493,1.255321345493,
1.255321345493,1.255321345493,1.255321345493,1.255321345493,1.255321345493)))
REPRESENTATION_ITEM('')
SURFACE()
);
#2451=(
BOUNDED_SURFACE()
B_SPLINE_SURFACE(3,3,((#125841,#125842,#125843,#125844,#125845,#125846,
#125847,#125848,#125849,#125850,#125851,#125852,#125853),(#125854,#125855,
#125856,#125857,#125858,#125859,#125860,#125861,#125862,#125863,#125864,
#125865,#125866),(#125867,#125868,#125869,#125870,#125871,#125872,#125873,
#125874,#125875,#125876,#125877,#125878,#125879),(#125880,#125881,#125882,
#125883,#125884,#125885,#125886,#125887,#125888,#125889,#125890,#125891,
#125892)),.UNSPECIFIED.,.F.,.F.,.F.)
B_SPLINE_SURFACE_WITH_KNOTS((4,4),(4,1,1,1,1,1,1,1,1,1,4),(0.,1.),(0.,0.0952638051529656,
0.22509444570554,0.342634254506935,0.445180680757504,0.539182519786869,
0.634901504810863,0.734230912844932,0.834482617338388,0.927390396537817,
1.),.UNSPECIFIED.)
GEOMETRIC_REPRESENTATION_ITEM()
RATIONAL_B_SPLINE_SURFACE(((1.132183978984,1.132183978984,1.132183978984,
1.132183978984,1.132183978984,1.132183978984,1.132183978984,1.132183978984,
1.132183978984,1.132183978984,1.132183978984,1.132183978984,1.132183978984),
(0.9559386736722,0.9559386736722,0.9559386736722,0.9559386736722,0.9559386736722,
0.9559386736722,0.9559386736722,0.9559386736722,0.9559386736722,0.9559386736722,
0.9559386736722,0.9559386736722,0.9559386736722),(0.9559386736722,0.9559386736722,
0.9559386736722,0.9559386736722,0.9559386736722,0.9559386736722,0.9559386736722,
0.9559386736722,0.9559386736722,0.9559386736722,0.9559386736722,0.9559386736722,
0.9559386736722),(1.132183978984,1.132183978984,1.132183978984,1.132183978984,
1.132183978984,1.132183978984,1.132183978984,1.132183978984,1.132183978984,
1.132183978984,1.132183978984,1.132183978984,1.132183978984)))
REPRESENTATION_ITEM('')
SURFACE()
);
#2452=(
BOUNDED_SURFACE()
B_SPLINE_SURFACE(3,3,((#125932,#125933,#125934,#125935,#125936,#125937),
(#125938,#125939,#125940,#125941,#125942,#125943),(#125944,#125945,#125946,
#125947,#125948,#125949),(#125950,#125951,#125952,#125953,#125954,#125955)),
 .UNSPECIFIED.,.F.,.F.,.F.)
B_SPLINE_SURFACE_WITH_KNOTS((4,4),(4,1,1,4),(0.,1.),(0.,0.0615355941999108,
0.552403092261162,1.),.UNSPECIFIED.)
GEOMETRIC_REPRESENTATION_ITEM()
RATIONAL_B_SPLINE_SURFACE(((1.132184177625,1.132184177625,1.132184177625,
1.132184177625,1.132184177625,1.132184177625),(0.9559386074585,0.9559386074585,
0.9559386074585,0.9559386074585,0.9559386074585,0.9559386074585),(0.9559386074585,
0.9559386074585,0.9559386074585,0.9559386074585,0.9559386074585,0.9559386074585),
(1.132184177625,1.132184177625,1.132184177625,1.132184177625,1.132184177625,
1.132184177625)))
REPRESENTATION_ITEM('')
SURFACE()
);
#2453=(
BOUNDED_SURFACE()
B_SPLINE_SURFACE(3,3,((#125982,#125983,#125984,#125985,#125986,#125987,
#125988,#125989,#125990,#125991,#125992,#125993,#125994,#125995,#125996,
#125997,#125998),(#125999,#126000,#126001,#126002,#126003,#126004,#126005,
#126006,#126007,#126008,#126009,#126010,#126011,#126012,#126013,#126014,
#126015),(#126016,#126017,#126018,#126019,#126020,#126021,#126022,#126023,
#126024,#126025,#126026,#126027,#126028,#126029,#126030,#126031,#126032),
(#126033,#126034,#126035,#126036,#126037,#126038,#126039,#126040,#126041,
#126042,#126043,#126044,#126045,#126046,#126047,#126048,#126049)),
 .UNSPECIFIED.,.F.,.F.,.F.)
B_SPLINE_SURFACE_WITH_KNOTS((4,4),(4,1,1,1,1,1,1,1,1,1,1,1,1,1,4),(0.,1.),
(0.,0.0421741349720486,0.122382017207444,0.194203536901675,0.257534399271218,
0.321534135544779,0.38726227689901,0.452657895941669,0.516567929355648,
0.579748305445392,0.647421910672303,0.723873761459194,0.810175603109662,
0.905570261612151,1.),.UNSPECIFIED.)
GEOMETRIC_REPRESENTATION_ITEM()
RATIONAL_B_SPLINE_SURFACE(((1.219577374139,1.219577374139,1.219577374139,
1.219577374139,1.219577374139,1.219577374139,1.219577374139,1.219577374139,
1.219577374139,1.219577374139,1.219577374139,1.219577374139,1.219577374139,
1.219577374139,1.219577374139,1.219577374139,1.219577374139),(0.9268075419537,
0.9268075419537,0.9268075419537,0.9268075419537,0.9268075419537,0.9268075419537,
0.9268075419537,0.9268075419537,0.9268075419537,0.9268075419537,0.9268075419537,
0.9268075419537,0.9268075419537,0.9268075419537,0.9268075419537,0.9268075419537,
0.9268075419537),(0.9268075419537,0.9268075419537,0.9268075419537,0.9268075419537,
0.9268075419537,0.9268075419537,0.9268075419537,0.9268075419537,0.9268075419537,
0.9268075419537,0.9268075419537,0.9268075419537,0.9268075419537,0.9268075419537,
0.9268075419537,0.9268075419537,0.9268075419537),(1.219577374139,1.219577374139,
1.219577374139,1.219577374139,1.219577374139,1.219577374139,1.219577374139,
1.219577374139,1.219577374139,1.219577374139,1.219577374139,1.219577374139,
1.219577374139,1.219577374139,1.219577374139,1.219577374139,1.219577374139)))
REPRESENTATION_ITEM('')
SURFACE()
);
#2454=(
BOUNDED_SURFACE()
B_SPLINE_SURFACE(3,3,((#126077,#126078,#126079,#126080,#126081,#126082,
#126083,#126084,#126085,#126086,#126087,#126088),(#126089,#126090,#126091,
#126092,#126093,#126094,#126095,#126096,#126097,#126098,#126099,#126100),
(#126101,#126102,#126103,#126104,#126105,#126106,#126107,#126108,#126109,
#126110,#126111,#126112),(#126113,#126114,#126115,#126116,#126117,#126118,
#126119,#126120,#126121,#126122,#126123,#126124)),.UNSPECIFIED.,.F.,.F.,
 .F.)
B_SPLINE_SURFACE_WITH_KNOTS((4,4),(4,1,1,1,1,1,1,1,1,4),(0.,1.),(0.,0.0164345215705728,
0.129301162013314,0.242710853927909,0.360524593523248,0.486789420086521,
0.625540658542323,0.780319654457662,0.950754978076216,1.),.UNSPECIFIED.)
GEOMETRIC_REPRESENTATION_ITEM()
RATIONAL_B_SPLINE_SURFACE(((1.03572903915,1.03572903915,1.03572903915,1.03572903915,
1.03572903915,1.03572903915,1.03572903915,1.03572903915,1.03572903915,1.03572903915,
1.03572903915,1.03572903915),(0.9880903202835,0.9880903202835,0.9880903202835,
0.9880903202835,0.9880903202835,0.9880903202835,0.9880903202835,0.9880903202835,
0.9880903202835,0.9880903202835,0.9880903202835,0.9880903202835),(0.9880903202835,
0.9880903202835,0.9880903202835,0.9880903202835,0.9880903202835,0.9880903202835,
0.9880903202835,0.9880903202835,0.9880903202835,0.9880903202835,0.9880903202835,
0.9880903202835),(1.03572903915,1.03572903915,1.03572903915,1.03572903915,
1.03572903915,1.03572903915,1.03572903915,1.03572903915,1.03572903915,1.03572903915,
1.03572903915,1.03572903915)))
REPRESENTATION_ITEM('')
SURFACE()
);
#2455=(
BOUNDED_SURFACE()
B_SPLINE_SURFACE(3,3,((#126575,#126576,#126577,#126578,#126579,#126580,
#126581,#126582,#126583),(#126584,#126585,#126586,#126587,#126588,#126589,
#126590,#126591,#126592),(#126593,#126594,#126595,#126596,#126597,#126598,
#126599,#126600,#126601),(#126602,#126603,#126604,#126605,#126606,#126607,
#126608,#126609,#126610)),.UNSPECIFIED.,.F.,.F.,.F.)
B_SPLINE_SURFACE_WITH_KNOTS((4,4),(4,1,1,1,1,1,4),(0.,1.),(0.,0.124217072386526,
0.310755650559109,0.499972700734522,0.689255535673335,0.875770607228338,
1.),.UNSPECIFIED.)
GEOMETRIC_REPRESENTATION_ITEM()
RATIONAL_B_SPLINE_SURFACE(((1.04330354939,1.04330354939,1.04330354939,1.04330354939,
1.04330354939,1.04330354939,1.04330354939,1.04330354939,1.04330354939),
(0.9855654835368,0.9855654835368,0.9855654835368,0.9855654835368,0.9855654835368,
0.9855654835368,0.9855654835368,0.9855654835368,0.9855654835368),(0.9855654835368,
0.9855654835368,0.9855654835368,0.9855654835368,0.9855654835368,0.9855654835368,
0.9855654835368,0.9855654835368,0.9855654835368),(1.04330354939,1.04330354939,
1.04330354939,1.04330354939,1.04330354939,1.04330354939,1.04330354939,1.04330354939,
1.04330354939)))
REPRESENTATION_ITEM('')
SURFACE()
);
#2456=(
BOUNDED_SURFACE()
B_SPLINE_SURFACE(3,3,((#126654,#126655,#126656,#126657,#126658,#126659,
#126660,#126661,#126662,#126663,#126664,#126665,#126666,#126667,#126668,
#126669,#126670,#126671,#126672),(#126673,#126674,#126675,#126676,#126677,
#126678,#126679,#126680,#126681,#126682,#126683,#126684,#126685,#126686,
#126687,#126688,#126689,#126690,#126691),(#126692,#126693,#126694,#126695,
#126696,#126697,#126698,#126699,#126700,#126701,#126702,#126703,#126704,
#126705,#126706,#126707,#126708,#126709,#126710),(#126711,#126712,#126713,
#126714,#126715,#126716,#126717,#126718,#126719,#126720,#126721,#126722,
#126723,#126724,#126725,#126726,#126727,#126728,#126729)),.UNSPECIFIED.,
 .F.,.F.,.F.)
B_SPLINE_SURFACE_WITH_KNOTS((4,4),(4,1,1,1,1,1,1,1,1,1,1,1,1,1,1,1,4),(0.,
1.),(0.,0.0799280122799653,0.16360439135842,0.238188789720562,0.304013208895698,
0.361552441990052,0.412607959769593,0.462371825350478,0.513679071869309,
0.566147489952465,0.617336562641754,0.665597869256093,0.718768591516355,
0.778520204495205,0.846090350205214,0.922943284356756,1.),.UNSPECIFIED.)
GEOMETRIC_REPRESENTATION_ITEM()
RATIONAL_B_SPLINE_SURFACE(((1.057421706335,1.057421706335,1.057421706335,
1.057421706335,1.057421706335,1.057421706335,1.057421706335,1.057421706335,
1.057421706335,1.057421706335,1.057421706335,1.057421706335,1.057421706335,
1.057421706335,1.057421706335,1.057421706335,1.057421706335,1.057421706335,
1.057421706335),(0.9808594312216,0.9808594312216,0.9808594312216,0.9808594312216,
0.9808594312216,0.9808594312216,0.9808594312216,0.9808594312216,0.9808594312216,
0.9808594312216,0.9808594312216,0.9808594312216,0.9808594312216,0.9808594312216,
0.9808594312216,0.9808594312216,0.9808594312216,0.9808594312216,0.9808594312216),
(0.9808594312216,0.9808594312216,0.9808594312216,0.9808594312216,0.9808594312216,
0.9808594312216,0.9808594312216,0.9808594312216,0.9808594312216,0.9808594312216,
0.9808594312216,0.9808594312216,0.9808594312216,0.9808594312216,0.9808594312216,
0.9808594312216,0.9808594312216,0.9808594312216,0.9808594312216),(1.057421706335,
1.057421706335,1.057421706335,1.057421706335,1.057421706335,1.057421706335,
1.057421706335,1.057421706335,1.057421706335,1.057421706335,1.057421706335,
1.057421706335,1.057421706335,1.057421706335,1.057421706335,1.057421706335,
1.057421706335,1.057421706335,1.057421706335)))
REPRESENTATION_ITEM('')
SURFACE()
);
#2457=(
BOUNDED_SURFACE()
B_SPLINE_SURFACE(3,3,((#126949,#126950,#126951,#126952,#126953,#126954),
(#126955,#126956,#126957,#126958,#126959,#126960),(#126961,#126962,#126963,
#126964,#126965,#126966),(#126967,#126968,#126969,#126970,#126971,#126972)),
 .UNSPECIFIED.,.F.,.F.,.F.)
B_SPLINE_SURFACE_WITH_KNOTS((4,4),(4,1,1,4),(0.,1.),(0.,0.261439365399046,
0.646008272605236,1.),.UNSPECIFIED.)
GEOMETRIC_REPRESENTATION_ITEM()
RATIONAL_B_SPLINE_SURFACE(((1.043303915571,1.043303915571,1.043303915571,
1.043303915571,1.043303915571,1.043303915571),(0.9855653614763,0.9855653614763,
0.9855653614763,0.9855653614763,0.9855653614763,0.9855653614763),(0.9855653614763,
0.9855653614763,0.9855653614763,0.9855653614763,0.9855653614763,0.9855653614763),
(1.043303915571,1.043303915571,1.043303915571,1.043303915571,1.043303915571,
1.043303915571)))
REPRESENTATION_ITEM('')
SURFACE()
);
#2458=(
BOUNDED_SURFACE()
B_SPLINE_SURFACE(3,3,((#127033,#127034,#127035,#127036,#127037,#127038),
(#127039,#127040,#127041,#127042,#127043,#127044),(#127045,#127046,#127047,
#127048,#127049,#127050),(#127051,#127052,#127053,#127054,#127055,#127056)),
 .UNSPECIFIED.,.F.,.F.,.F.)
B_SPLINE_SURFACE_WITH_KNOTS((4,4),(4,1,1,4),(0.,1.),(0.,0.338411218706876,
0.730847706276313,1.),.UNSPECIFIED.)
GEOMETRIC_REPRESENTATION_ITEM()
RATIONAL_B_SPLINE_SURFACE(((1.043304339832,1.043304339832,1.043304339832,
1.043304339832,1.043304339832,1.043304339832),(0.9855652200561,0.9855652200561,
0.9855652200561,0.9855652200561,0.9855652200561,0.9855652200561),(0.9855652200561,
0.9855652200561,0.9855652200561,0.9855652200561,0.9855652200561,0.9855652200561),
(1.043304339832,1.043304339832,1.043304339832,1.043304339832,1.043304339832,
1.043304339832)))
REPRESENTATION_ITEM('')
SURFACE()
);
#2459=(
BOUNDED_SURFACE()
B_SPLINE_SURFACE(3,3,((#127120,#127121,#127122,#127123,#127124,#127125),
(#127126,#127127,#127128,#127129,#127130,#127131),(#127132,#127133,#127134,
#127135,#127136,#127137),(#127138,#127139,#127140,#127141,#127142,#127143)),
 .UNSPECIFIED.,.F.,.F.,.F.)
B_SPLINE_SURFACE_WITH_KNOTS((4,4),(4,1,1,4),(0.,1.),(0.,0.29605416480998,
0.688995950644091,1.),.UNSPECIFIED.)
GEOMETRIC_REPRESENTATION_ITEM()
RATIONAL_B_SPLINE_SURFACE(((1.049988055972,1.049988055972,1.049988055972,
1.049988055972,1.049988055972,1.049988055972),(0.983337314676,0.983337314676,
0.983337314676,0.983337314676,0.983337314676,0.983337314676),(0.983337314676,
0.983337314676,0.983337314676,0.983337314676,0.983337314676,0.983337314676),
(1.049988055972,1.049988055972,1.049988055972,1.049988055972,1.049988055972,
1.049988055972)))
REPRESENTATION_ITEM('')
SURFACE()
);
#2460=(
BOUNDED_SURFACE()
B_SPLINE_SURFACE(3,3,((#127157,#127158,#127159,#127160,#127161,#127162,
#127163,#127164,#127165,#127166,#127167,#127168),(#127169,#127170,#127171,
#127172,#127173,#127174,#127175,#127176,#127177,#127178,#127179,#127180),
(#127181,#127182,#127183,#127184,#127185,#127186,#127187,#127188,#127189,
#127190,#127191,#127192),(#127193,#127194,#127195,#127196,#127197,#127198,
#127199,#127200,#127201,#127202,#127203,#127204)),.UNSPECIFIED.,.F.,.F.,
 .F.)
B_SPLINE_SURFACE_WITH_KNOTS((4,4),(4,1,1,1,1,1,1,1,1,4),(0.,1.),(0.,0.0415070947502971,
0.154210972284995,0.269286157242448,0.38315843713789,0.490653949298758,
0.603397292452659,0.728418373951416,0.867462240539534,1.),.UNSPECIFIED.)
GEOMETRIC_REPRESENTATION_ITEM()
RATIONAL_B_SPLINE_SURFACE(((1.050209251113,1.050209251113,1.050209251113,
1.050209251113,1.050209251113,1.050209251113,1.050209251113,1.050209251113,
1.050209251113,1.050209251113,1.050209251113,1.050209251113),(0.9832635829624,
0.9832635829624,0.9832635829624,0.9832635829624,0.9832635829624,0.9832635829624,
0.9832635829624,0.9832635829624,0.9832635829624,0.9832635829624,0.9832635829624,
0.9832635829624),(0.9832635829624,0.9832635829624,0.9832635829624,0.9832635829624,
0.9832635829624,0.9832635829624,0.9832635829624,0.9832635829624,0.9832635829624,
0.9832635829624,0.9832635829624,0.9832635829624),(1.050209251113,1.050209251113,
1.050209251113,1.050209251113,1.050209251113,1.050209251113,1.050209251113,
1.050209251113,1.050209251113,1.050209251113,1.050209251113,1.050209251113)))
REPRESENTATION_ITEM('')
SURFACE()
);
#2461=(
BOUNDED_SURFACE()
B_SPLINE_SURFACE(3,3,((#127358,#127359,#127360,#127361,#127362,#127363,
#127364,#127365),(#127366,#127367,#127368,#127369,#127370,#127371,#127372,
#127373),(#127374,#127375,#127376,#127377,#127378,#127379,#127380,#127381),
(#127382,#127383,#127384,#127385,#127386,#127387,#127388,#127389)),
 .UNSPECIFIED.,.F.,.F.,.F.)
B_SPLINE_SURFACE_WITH_KNOTS((4,4),(4,1,1,1,1,4),(0.,1.),(0.,0.20131167769844,
0.447511967106375,0.696970531427775,0.944927146503993,1.),.UNSPECIFIED.)
GEOMETRIC_REPRESENTATION_ITEM()
RATIONAL_B_SPLINE_SURFACE(((1.050193937179,1.050193937179,1.050193937179,
1.050193937179,1.050193937179,1.050193937179,1.050193937179,1.050193937179),
(0.9832686876072,0.9832686876072,0.9832686876072,0.9832686876072,0.9832686876071,
0.9832686876072,0.9832686876072,0.9832686876072),(0.9832686876072,0.9832686876072,
0.9832686876072,0.9832686876072,0.9832686876071,0.9832686876072,0.9832686876072,
0.9832686876072),(1.050193937179,1.050193937179,1.050193937179,1.050193937179,
1.050193937179,1.050193937179,1.050193937179,1.050193937179)))
REPRESENTATION_ITEM('')
SURFACE()
);
#2462=(
BOUNDED_SURFACE()
B_SPLINE_SURFACE(3,3,((#127425,#127426,#127427,#127428,#127429,#127430),
(#127431,#127432,#127433,#127434,#127435,#127436),(#127437,#127438,#127439,
#127440,#127441,#127442),(#127443,#127444,#127445,#127446,#127447,#127448)),
 .UNSPECIFIED.,.F.,.F.,.F.)
B_SPLINE_SURFACE_WITH_KNOTS((4,4),(4,1,1,4),(0.,1.),(0.,0.314367621060507,
0.711949844500348,1.),.UNSPECIFIED.)
GEOMETRIC_REPRESENTATION_ITEM()
RATIONAL_B_SPLINE_SURFACE(((1.049987137241,1.049987137241,1.049987137241,
1.049987137241,1.049987137241,1.049987137241),(0.9833376209197,0.9833376209197,
0.9833376209197,0.9833376209197,0.9833376209197,0.9833376209197),(0.9833376209197,
0.9833376209197,0.9833376209197,0.9833376209197,0.9833376209197,0.9833376209197),
(1.049987137241,1.049987137241,1.049987137241,1.049987137241,1.049987137241,
1.049987137241)))
REPRESENTATION_ITEM('')
SURFACE()
);
#2463=(
BOUNDED_SURFACE()
B_SPLINE_SURFACE(3,3,((#127489,#127490,#127491,#127492,#127493,#127494,
#127495,#127496,#127497,#127498),(#127499,#127500,#127501,#127502,#127503,
#127504,#127505,#127506,#127507,#127508),(#127509,#127510,#127511,#127512,
#127513,#127514,#127515,#127516,#127517,#127518),(#127519,#127520,#127521,
#127522,#127523,#127524,#127525,#127526,#127527,#127528),(#127529,#127530,
#127531,#127532,#127533,#127534,#127535,#127536,#127537,#127538),(#127539,
#127540,#127541,#127542,#127543,#127544,#127545,#127546,#127547,#127548),
(#127549,#127550,#127551,#127552,#127553,#127554,#127555,#127556,#127557,
#127558)),.UNSPECIFIED.,.F.,.F.,.F.)
B_SPLINE_SURFACE_WITH_KNOTS((4,3,4),(4,1,1,1,1,1,1,4),(0.,0.5,1.),(0.,0.161024836461119,
0.369601718395748,0.554125890569757,0.718052359943506,0.864941999117123,
0.996690204747089,1.),.UNSPECIFIED.)
GEOMETRIC_REPRESENTATION_ITEM()
RATIONAL_B_SPLINE_SURFACE(((1.201213809875,1.201213809875,1.201213809875,
1.201213809875,1.201213809875,1.201213809875,1.201213809875,1.201213809875,
1.201213809875,1.201213809875),(0.9329287300417,0.9329287300417,0.9329287300417,
0.9329287300417,0.9329287300417,0.9329287300417,0.9329287300417,0.9329287300417,
0.9329287300417,0.9329287300417),(0.9329287300417,0.9329287300417,0.9329287300417,
0.9329287300417,0.9329287300417,0.9329287300417,0.9329287300417,0.9329287300417,
0.9329287300417,0.9329287300417),(1.201213809875,1.201213809875,1.201213809875,
1.201213809875,1.201213809875,1.201213809875,1.201213809875,1.201213809875,
1.201213809875,1.201213809875),(0.9329287300417,0.9329287300417,0.9329287300417,
0.9329287300417,0.9329287300417,0.9329287300417,0.9329287300417,0.9329287300417,
0.9329287300417,0.9329287300417),(0.9329287300417,0.9329287300417,0.9329287300417,
0.9329287300417,0.9329287300417,0.9329287300417,0.9329287300417,0.9329287300417,
0.9329287300417,0.9329287300417),(1.201213809875,1.201213809875,1.201213809875,
1.201213809875,1.201213809875,1.201213809875,1.201213809875,1.201213809875,
1.201213809875,1.201213809875)))
REPRESENTATION_ITEM('')
SURFACE()
);
#2464=(
BOUNDED_SURFACE()
B_SPLINE_SURFACE(3,3,((#127645,#127646,#127647,#127648,#127649,#127650,
#127651,#127652,#127653,#127654),(#127655,#127656,#127657,#127658,#127659,
#127660,#127661,#127662,#127663,#127664),(#127665,#127666,#127667,#127668,
#127669,#127670,#127671,#127672,#127673,#127674),(#127675,#127676,#127677,
#127678,#127679,#127680,#127681,#127682,#127683,#127684),(#127685,#127686,
#127687,#127688,#127689,#127690,#127691,#127692,#127693,#127694),(#127695,
#127696,#127697,#127698,#127699,#127700,#127701,#127702,#127703,#127704),
(#127705,#127706,#127707,#127708,#127709,#127710,#127711,#127712,#127713,
#127714)),.UNSPECIFIED.,.F.,.F.,.F.)
B_SPLINE_SURFACE_WITH_KNOTS((4,3,4),(4,1,1,1,1,1,1,4),(0.,0.5,1.),(0.,0.0025907538636228,
0.133682793303005,0.278706793926935,0.438527262608492,0.616078859653579,
0.815708849792895,1.),.UNSPECIFIED.)
GEOMETRIC_REPRESENTATION_ITEM()
RATIONAL_B_SPLINE_SURFACE(((1.201171733822,1.201171733822,1.201171733822,
1.201171733822,1.201171733822,1.201171733822,1.201171733822,1.201171733822,
1.201171733822,1.201171733822),(0.9329427553926,0.9329427553926,0.9329427553926,
0.9329427553926,0.9329427553926,0.9329427553926,0.9329427553926,0.9329427553926,
0.9329427553926,0.9329427553926),(0.9329427553926,0.9329427553926,0.9329427553926,
0.9329427553926,0.9329427553926,0.9329427553926,0.9329427553926,0.9329427553926,
0.9329427553926,0.9329427553926),(1.201171733822,1.201171733822,1.201171733822,
1.201171733822,1.201171733822,1.201171733822,1.201171733822,1.201171733822,
1.201171733822,1.201171733822),(0.9329427553926,0.9329427553926,0.9329427553926,
0.9329427553926,0.9329427553926,0.9329427553926,0.9329427553926,0.9329427553926,
0.9329427553926,0.9329427553926),(0.9329427553926,0.9329427553926,0.9329427553926,
0.9329427553926,0.9329427553926,0.9329427553926,0.9329427553926,0.9329427553926,
0.9329427553926,0.9329427553926),(1.201171733822,1.201171733822,1.201171733822,
1.201171733822,1.201171733822,1.201171733822,1.201171733822,1.201171733822,
1.201171733822,1.201171733822)))
REPRESENTATION_ITEM('')
SURFACE()
);
#2465=(
BOUNDED_SURFACE()
B_SPLINE_SURFACE(3,3,((#127716,#127717,#127718,#127719,#127720,#127721,
#127722,#127723,#127724,#127725,#127726,#127727,#127728,#127729,#127730,
#127731,#127732,#127733,#127734,#127735,#127736,#127737,#127738,#127739,
#127740,#127741),(#127742,#127743,#127744,#127745,#127746,#127747,#127748,
#127749,#127750,#127751,#127752,#127753,#127754,#127755,#127756,#127757,
#127758,#127759,#127760,#127761,#127762,#127763,#127764,#127765,#127766,
#127767),(#127768,#127769,#127770,#127771,#127772,#127773,#127774,#127775,
#127776,#127777,#127778,#127779,#127780,#127781,#127782,#127783,#127784,
#127785,#127786,#127787,#127788,#127789,#127790,#127791,#127792,#127793),
(#127794,#127795,#127796,#127797,#127798,#127799,#127800,#127801,#127802,
#127803,#127804,#127805,#127806,#127807,#127808,#127809,#127810,#127811,
#127812,#127813,#127814,#127815,#127816,#127817,#127818,#127819),(#127820,
#127821,#127822,#127823,#127824,#127825,#127826,#127827,#127828,#127829,
#127830,#127831,#127832,#127833,#127834,#127835,#127836,#127837,#127838,
#127839,#127840,#127841,#127842,#127843,#127844,#127845),(#127846,#127847,
#127848,#127849,#127850,#127851,#127852,#127853,#127854,#127855,#127856,
#127857,#127858,#127859,#127860,#127861,#127862,#127863,#127864,#127865,
#127866,#127867,#127868,#127869,#127870,#127871),(#127872,#127873,#127874,
#127875,#127876,#127877,#127878,#127879,#127880,#127881,#127882,#127883,
#127884,#127885,#127886,#127887,#127888,#127889,#127890,#127891,#127892,
#127893,#127894,#127895,#127896,#127897)),.UNSPECIFIED.,.F.,.F.,.F.)
B_SPLINE_SURFACE_WITH_KNOTS((4,3,4),(4,1,1,1,1,1,1,1,1,1,1,1,1,1,1,1,1,
1,1,1,1,1,1,4),(0.,0.5,1.),(0.,0.00338709104151123,0.0292031644766076,0.0596169482905785,
0.0941190289168756,0.132291998012268,0.173832504660512,0.218910698019246,
0.268547982014753,0.323764747156882,0.385760267159764,0.456177213623959,
0.530980523979295,0.603593295594907,0.667945269850854,0.724945053578612,
0.775984643286146,0.822177899369198,0.864653703764676,0.903649038429262,
0.93888404941214,0.969960836451304,0.99638734008221,1.),.UNSPECIFIED.)
GEOMETRIC_REPRESENTATION_ITEM()
RATIONAL_B_SPLINE_SURFACE(((1.193841844068,1.193841844068,1.193841844068,
1.193841844068,1.193841844068,1.193841844068,1.193841844068,1.193841844068,
1.193841844068,1.193841844068,1.193841844068,1.193841844068,1.193841844068,
1.193841844068,1.193841844068,1.193841844068,1.193841844068,1.193841844068,
1.193841844068,1.193841844068,1.193841844068,1.193841844068,1.193841844068,
1.193841844068,1.193841844068,1.193841844068),(0.9353860519774,0.9353860519774,
0.9353860519774,0.9353860519774,0.9353860519774,0.9353860519774,0.9353860519774,
0.9353860519774,0.9353860519774,0.9353860519774,0.9353860519774,0.9353860519774,
0.9353860519774,0.9353860519774,0.9353860519774,0.9353860519774,0.9353860519774,
0.9353860519774,0.9353860519774,0.9353860519774,0.9353860519774,0.9353860519774,
0.9353860519774,0.9353860519774,0.9353860519774,0.9353860519774),(0.9353860519774,
0.9353860519774,0.9353860519774,0.9353860519774,0.9353860519774,0.9353860519774,
0.9353860519774,0.9353860519774,0.9353860519774,0.9353860519774,0.9353860519774,
0.9353860519774,0.9353860519774,0.9353860519774,0.9353860519774,0.9353860519774,
0.9353860519774,0.9353860519774,0.9353860519774,0.9353860519774,0.9353860519774,
0.9353860519774,0.9353860519774,0.9353860519774,0.9353860519774,0.9353860519774),
(1.193841844068,1.193841844068,1.193841844068,1.193841844068,1.193841844068,
1.193841844068,1.193841844068,1.193841844068,1.193841844068,1.193841844068,
1.193841844068,1.193841844068,1.193841844068,1.193841844068,1.193841844068,
1.193841844068,1.193841844068,1.193841844068,1.193841844068,1.193841844068,
1.193841844068,1.193841844068,1.193841844068,1.193841844068,1.193841844068,
1.193841844068),(0.9353860519774,0.9353860519774,0.9353860519774,0.9353860519774,
0.9353860519774,0.9353860519774,0.9353860519774,0.9353860519774,0.9353860519774,
0.9353860519774,0.9353860519774,0.9353860519774,0.9353860519774,0.9353860519774,
0.9353860519774,0.9353860519774,0.9353860519774,0.9353860519774,0.9353860519774,
0.9353860519774,0.9353860519774,0.9353860519774,0.9353860519774,0.9353860519774,
0.9353860519774,0.9353860519774),(0.9353860519774,0.9353860519774,0.9353860519774,
0.9353860519774,0.9353860519774,0.9353860519774,0.9353860519774,0.9353860519774,
0.9353860519774,0.9353860519774,0.9353860519774,0.9353860519774,0.9353860519774,
0.9353860519774,0.9353860519774,0.9353860519774,0.9353860519774,0.9353860519774,
0.9353860519774,0.9353860519774,0.9353860519774,0.9353860519774,0.9353860519774,
0.9353860519774,0.9353860519774,0.9353860519774),(1.193841844068,1.193841844068,
1.193841844068,1.193841844068,1.193841844068,1.193841844068,1.193841844068,
1.193841844068,1.193841844068,1.193841844068,1.193841844068,1.193841844068,
1.193841844068,1.193841844068,1.193841844068,1.193841844068,1.193841844068,
1.193841844068,1.193841844068,1.193841844068,1.193841844068,1.193841844068,
1.193841844068,1.193841844068,1.193841844068,1.193841844068)))
REPRESENTATION_ITEM('')
SURFACE()
);
#2466=(
BOUNDED_SURFACE()
B_SPLINE_SURFACE(3,3,((#127899,#127900,#127901,#127902,#127903,#127904,
#127905,#127906,#127907,#127908),(#127909,#127910,#127911,#127912,#127913,
#127914,#127915,#127916,#127917,#127918),(#127919,#127920,#127921,#127922,
#127923,#127924,#127925,#127926,#127927,#127928),(#127929,#127930,#127931,
#127932,#127933,#127934,#127935,#127936,#127937,#127938),(#127939,#127940,
#127941,#127942,#127943,#127944,#127945,#127946,#127947,#127948),(#127949,
#127950,#127951,#127952,#127953,#127954,#127955,#127956,#127957,#127958),
(#127959,#127960,#127961,#127962,#127963,#127964,#127965,#127966,#127967,
#127968)),.UNSPECIFIED.,.F.,.F.,.F.)
B_SPLINE_SURFACE_WITH_KNOTS((4,3,4),(4,1,1,1,1,1,1,4),(0.,0.5,1.),(0.,0.213585283551531,
0.4054505508447,0.577283027769576,0.731642593504136,0.871393000159704,0.997433614646813,
1.),.UNSPECIFIED.)
GEOMETRIC_REPRESENTATION_ITEM()
RATIONAL_B_SPLINE_SURFACE(((1.201113977633,1.201113977633,1.201113977633,
1.201113977633,1.201113977633,1.201113977633,1.201113977633,1.201113977633,
1.201113977633,1.201113977633),(0.9329620074556,0.9329620074556,0.9329620074556,
0.9329620074556,0.9329620074556,0.9329620074556,0.9329620074556,0.9329620074556,
0.9329620074556,0.9329620074556),(0.9329620074556,0.9329620074556,0.9329620074556,
0.9329620074556,0.9329620074556,0.9329620074556,0.9329620074556,0.9329620074556,
0.9329620074556,0.9329620074556),(1.201113977633,1.201113977633,1.201113977633,
1.201113977633,1.201113977633,1.201113977633,1.201113977633,1.201113977633,
1.201113977633,1.201113977633),(0.9329620074556,0.9329620074556,0.9329620074556,
0.9329620074556,0.9329620074556,0.9329620074556,0.9329620074556,0.9329620074556,
0.9329620074556,0.9329620074556),(0.9329620074556,0.9329620074556,0.9329620074556,
0.9329620074556,0.9329620074556,0.9329620074556,0.9329620074556,0.9329620074556,
0.9329620074556,0.9329620074556),(1.201113977633,1.201113977633,1.201113977633,
1.201113977633,1.201113977633,1.201113977633,1.201113977633,1.201113977633,
1.201113977633,1.201113977633)))
REPRESENTATION_ITEM('')
SURFACE()
);
#2467=(
BOUNDED_SURFACE()
B_SPLINE_SURFACE(3,3,((#127987,#127988,#127989,#127990,#127991,#127992,
#127993,#127994,#127995,#127996,#127997),(#127998,#127999,#128000,#128001,
#128002,#128003,#128004,#128005,#128006,#128007,#128008),(#128009,#128010,
#128011,#128012,#128013,#128014,#128015,#128016,#128017,#128018,#128019),
(#128020,#128021,#128022,#128023,#128024,#128025,#128026,#128027,#128028,
#128029,#128030),(#128031,#128032,#128033,#128034,#128035,#128036,#128037,
#128038,#128039,#128040,#128041),(#128042,#128043,#128044,#128045,#128046,
#128047,#128048,#128049,#128050,#128051,#128052),(#128053,#128054,#128055,
#128056,#128057,#128058,#128059,#128060,#128061,#128062,#128063)),
 .UNSPECIFIED.,.F.,.F.,.F.)
B_SPLINE_SURFACE_WITH_KNOTS((4,3,4),(4,1,1,1,1,1,1,1,4),(0.,0.5,1.),(0.,
0.00181835876594797,0.105491111993237,0.219958345253759,0.345909403004321,
0.484805331232095,0.638614178236773,0.80985054968314,1.),.UNSPECIFIED.)
GEOMETRIC_REPRESENTATION_ITEM()
RATIONAL_B_SPLINE_SURFACE(((1.201132896331,1.201132896331,1.201132896331,
1.201132896331,1.201132896331,1.201132896331,1.201132896331,1.201132896331,
1.201132896331,1.201132896331,1.201132896331),(0.9329557012229,0.9329557012229,
0.9329557012229,0.9329557012229,0.9329557012229,0.9329557012229,0.9329557012229,
0.9329557012229,0.9329557012229,0.9329557012229,0.9329557012229),(0.9329557012229,
0.9329557012229,0.9329557012229,0.9329557012229,0.9329557012229,0.9329557012229,
0.9329557012229,0.9329557012229,0.9329557012229,0.9329557012229,0.9329557012229),
(1.201132896331,1.201132896331,1.201132896331,1.201132896331,1.201132896331,
1.201132896331,1.201132896331,1.201132896331,1.201132896331,1.201132896331,
1.201132896331),(0.9329557012229,0.9329557012229,0.9329557012229,0.9329557012229,
0.9329557012229,0.9329557012229,0.9329557012229,0.9329557012229,0.9329557012229,
0.9329557012229,0.9329557012229),(0.9329557012229,0.9329557012229,0.9329557012229,
0.9329557012229,0.9329557012229,0.9329557012229,0.9329557012229,0.9329557012229,
0.9329557012229,0.9329557012229,0.9329557012229),(1.201132896331,1.201132896331,
1.201132896331,1.201132896331,1.201132896331,1.201132896331,1.201132896331,
1.201132896331,1.201132896331,1.201132896331,1.201132896331)))
REPRESENTATION_ITEM('')
SURFACE()
);
#2468=(
BOUNDED_SURFACE()
B_SPLINE_SURFACE(3,3,((#128065,#128066,#128067,#128068,#128069,#128070,
#128071,#128072,#128073,#128074,#128075,#128076),(#128077,#128078,#128079,
#128080,#128081,#128082,#128083,#128084,#128085,#128086,#128087,#128088),
(#128089,#128090,#128091,#128092,#128093,#128094,#128095,#128096,#128097,
#128098,#128099,#128100),(#128101,#128102,#128103,#128104,#128105,#128106,
#128107,#128108,#128109,#128110,#128111,#128112),(#128113,#128114,#128115,
#128116,#128117,#128118,#128119,#128120,#128121,#128122,#128123,#128124),
(#128125,#128126,#128127,#128128,#128129,#128130,#128131,#128132,#128133,
#128134,#128135,#128136),(#128137,#128138,#128139,#128140,#128141,#128142,
#128143,#128144,#128145,#128146,#128147,#128148)),.UNSPECIFIED.,.F.,.F.,
 .F.)
B_SPLINE_SURFACE_WITH_KNOTS((4,3,4),(4,1,1,1,1,1,1,1,1,4),(0.,0.5,1.),(0.,
0.000255346721705583,0.127238168179912,0.25348490093621,0.379076505598381,
0.504103162940652,0.628662748636027,0.752852442580265,0.876759085909055,
1.),.UNSPECIFIED.)
GEOMETRIC_REPRESENTATION_ITEM()
RATIONAL_B_SPLINE_SURFACE(((1.193842470635,1.193842470635,1.193842470635,
1.193842470635,1.193842470635,1.193842470635,1.193842470635,1.193842470635,
1.193842470635,1.193842470635,1.193842470635,1.193842470635),(0.9353858431218,
0.9353858431218,0.9353858431218,0.9353858431218,0.9353858431218,0.9353858431218,
0.9353858431218,0.9353858431218,0.9353858431218,0.9353858431218,0.9353858431218,
0.9353858431218),(0.9353858431218,0.9353858431218,0.9353858431218,0.9353858431218,
0.9353858431218,0.9353858431218,0.9353858431218,0.9353858431218,0.9353858431218,
0.9353858431218,0.9353858431218,0.9353858431218),(1.193842470635,1.193842470635,
1.193842470635,1.193842470635,1.193842470635,1.193842470635,1.193842470635,
1.193842470635,1.193842470635,1.193842470635,1.193842470635,1.193842470635),
(0.9353858431218,0.9353858431218,0.9353858431218,0.9353858431218,0.9353858431218,
0.9353858431218,0.9353858431218,0.9353858431218,0.9353858431218,0.9353858431218,
0.9353858431218,0.9353858431218),(0.9353858431218,0.9353858431218,0.9353858431218,
0.9353858431218,0.9353858431218,0.9353858431218,0.9353858431218,0.9353858431218,
0.9353858431218,0.9353858431218,0.9353858431218,0.9353858431218),(1.193842470635,
1.193842470635,1.193842470635,1.193842470635,1.193842470635,1.193842470635,
1.193842470635,1.193842470635,1.193842470635,1.193842470635,1.193842470635,
1.193842470635)))
REPRESENTATION_ITEM('')
SURFACE()
);
#2469=(
BOUNDED_SURFACE()
B_SPLINE_SURFACE(3,3,((#128150,#128151,#128152,#128153,#128154,#128155,
#128156,#128157,#128158,#128159,#128160,#128161,#128162,#128163,#128164,
#128165,#128166,#128167,#128168,#128169),(#128170,#128171,#128172,#128173,
#128174,#128175,#128176,#128177,#128178,#128179,#128180,#128181,#128182,
#128183,#128184,#128185,#128186,#128187,#128188,#128189),(#128190,#128191,
#128192,#128193,#128194,#128195,#128196,#128197,#128198,#128199,#128200,
#128201,#128202,#128203,#128204,#128205,#128206,#128207,#128208,#128209),
(#128210,#128211,#128212,#128213,#128214,#128215,#128216,#128217,#128218,
#128219,#128220,#128221,#128222,#128223,#128224,#128225,#128226,#128227,
#128228,#128229),(#128230,#128231,#128232,#128233,#128234,#128235,#128236,
#128237,#128238,#128239,#128240,#128241,#128242,#128243,#128244,#128245,
#128246,#128247,#128248,#128249),(#128250,#128251,#128252,#128253,#128254,
#128255,#128256,#128257,#128258,#128259,#128260,#128261,#128262,#128263,
#128264,#128265,#128266,#128267,#128268,#128269),(#128270,#128271,#128272,
#128273,#128274,#128275,#128276,#128277,#128278,#128279,#128280,#128281,
#128282,#128283,#128284,#128285,#128286,#128287,#128288,#128289)),
 .UNSPECIFIED.,.F.,.F.,.F.)
B_SPLINE_SURFACE_WITH_KNOTS((4,3,4),(4,1,1,1,1,1,1,1,1,1,1,1,1,1,1,1,1,
4),(0.,0.5,1.),(0.,0.0489590947384862,0.106545697307053,0.169926417435894,
0.240019733012254,0.317744348497442,0.399711066482656,0.479868307731546,
0.557020357792415,0.630152704112907,0.698243580475678,0.760671732039233,
0.81767991258728,0.869583135240796,0.916669699502804,0.959206322109519,
0.997448988846953,1.),.UNSPECIFIED.)
GEOMETRIC_REPRESENTATION_ITEM()
RATIONAL_B_SPLINE_SURFACE(((1.182965384822,1.182965384822,1.182965384822,
1.182965384822,1.182965384822,1.182965384822,1.182965384822,1.182965384822,
1.182965384822,1.182965384822,1.182965384822,1.182965384822,1.182965384822,
1.182965384822,1.182965384822,1.182965384822,1.182965384822,1.182965384822,
1.182965384822,1.182965384822),(0.9390115383926,0.9390115383926,0.9390115383926,
0.9390115383926,0.9390115383926,0.9390115383926,0.9390115383926,0.9390115383926,
0.9390115383926,0.9390115383926,0.9390115383926,0.9390115383926,0.9390115383926,
0.9390115383926,0.9390115383926,0.9390115383926,0.9390115383926,0.9390115383926,
0.9390115383926,0.9390115383926),(0.9390115383926,0.9390115383926,0.9390115383926,
0.9390115383926,0.9390115383926,0.9390115383926,0.9390115383926,0.9390115383926,
0.9390115383926,0.9390115383926,0.9390115383926,0.9390115383926,0.9390115383926,
0.9390115383926,0.9390115383926,0.9390115383926,0.9390115383926,0.9390115383926,
0.9390115383926,0.9390115383926),(1.182965384822,1.182965384822,1.182965384822,
1.182965384822,1.182965384822,1.182965384822,1.182965384822,1.182965384822,
1.182965384822,1.182965384822,1.182965384822,1.182965384822,1.182965384822,
1.182965384822,1.182965384822,1.182965384822,1.182965384822,1.182965384822,
1.182965384822,1.182965384822),(0.9390115383926,0.9390115383926,0.9390115383926,
0.9390115383926,0.9390115383926,0.9390115383926,0.9390115383926,0.9390115383926,
0.9390115383926,0.9390115383926,0.9390115383926,0.9390115383926,0.9390115383926,
0.9390115383926,0.9390115383926,0.9390115383926,0.9390115383926,0.9390115383926,
0.9390115383926,0.9390115383926),(0.9390115383926,0.9390115383926,0.9390115383926,
0.9390115383926,0.9390115383926,0.9390115383926,0.9390115383926,0.9390115383926,
0.9390115383926,0.9390115383926,0.9390115383926,0.9390115383926,0.9390115383926,
0.9390115383926,0.9390115383926,0.9390115383926,0.9390115383926,0.9390115383926,
0.9390115383926,0.9390115383926),(1.182965384822,1.182965384822,1.182965384822,
1.182965384822,1.182965384822,1.182965384822,1.182965384822,1.182965384822,
1.182965384822,1.182965384822,1.182965384822,1.182965384822,1.182965384822,
1.182965384822,1.182965384822,1.182965384822,1.182965384822,1.182965384822,
1.182965384822,1.182965384822)))
REPRESENTATION_ITEM('')
SURFACE()
);
#2470=(
BOUNDED_SURFACE()
B_SPLINE_SURFACE(3,3,((#128308,#128309,#128310,#128311,#128312,#128313,
#128314,#128315,#128316,#128317,#128318,#128319,#128320,#128321,#128322,
#128323,#128324,#128325,#128326),(#128327,#128328,#128329,#128330,#128331,
#128332,#128333,#128334,#128335,#128336,#128337,#128338,#128339,#128340,
#128341,#128342,#128343,#128344,#128345),(#128346,#128347,#128348,#128349,
#128350,#128351,#128352,#128353,#128354,#128355,#128356,#128357,#128358,
#128359,#128360,#128361,#128362,#128363,#128364),(#128365,#128366,#128367,
#128368,#128369,#128370,#128371,#128372,#128373,#128374,#128375,#128376,
#128377,#128378,#128379,#128380,#128381,#128382,#128383),(#128384,#128385,
#128386,#128387,#128388,#128389,#128390,#128391,#128392,#128393,#128394,
#128395,#128396,#128397,#128398,#128399,#128400,#128401,#128402),(#128403,
#128404,#128405,#128406,#128407,#128408,#128409,#128410,#128411,#128412,
#128413,#128414,#128415,#128416,#128417,#128418,#128419,#128420,#128421),
(#128422,#128423,#128424,#128425,#128426,#128427,#128428,#128429,#128430,
#128431,#128432,#128433,#128434,#128435,#128436,#128437,#128438,#128439,
#128440)),.UNSPECIFIED.,.F.,.F.,.F.)
B_SPLINE_SURFACE_WITH_KNOTS((4,3,4),(4,1,1,1,1,1,1,1,1,1,1,1,1,1,1,1,4),
(0.,0.5,1.),(0.,0.00198169918793633,0.0506821482100691,0.105488478666356,
0.16376961522165,0.222938538024466,0.281407831568016,0.339150728322178,
0.397207423178538,0.457726780737408,0.522920886388937,0.594978378611854,
0.675924491902483,0.762809530116442,0.849642958155992,0.931396381678324,
1.),.UNSPECIFIED.)
GEOMETRIC_REPRESENTATION_ITEM()
RATIONAL_B_SPLINE_SURFACE(((1.18298561069,1.18298561069,1.18298561069,1.18298561069,
1.18298561069,1.18298561069,1.18298561069,1.18298561069,1.18298561069,1.18298561069,
1.18298561069,1.18298561069,1.18298561069,1.18298561069,1.18298561069,1.18298561069,
1.18298561069,1.18298561069,1.18298561069),(0.9390047964366,0.9390047964366,
0.9390047964366,0.9390047964366,0.9390047964366,0.9390047964366,0.9390047964366,
0.9390047964366,0.9390047964366,0.9390047964366,0.9390047964366,0.9390047964366,
0.9390047964366,0.9390047964366,0.9390047964366,0.9390047964366,0.9390047964366,
0.9390047964366,0.9390047964366),(0.9390047964366,0.9390047964366,0.9390047964366,
0.9390047964366,0.9390047964366,0.9390047964366,0.9390047964366,0.9390047964366,
0.9390047964366,0.9390047964366,0.9390047964366,0.9390047964366,0.9390047964366,
0.9390047964366,0.9390047964366,0.9390047964366,0.9390047964366,0.9390047964366,
0.9390047964366),(1.18298561069,1.18298561069,1.18298561069,1.18298561069,
1.18298561069,1.18298561069,1.18298561069,1.18298561069,1.18298561069,1.18298561069,
1.18298561069,1.18298561069,1.18298561069,1.18298561069,1.18298561069,1.18298561069,
1.18298561069,1.18298561069,1.18298561069),(0.9390047964366,0.9390047964366,
0.9390047964366,0.9390047964366,0.9390047964366,0.9390047964366,0.9390047964366,
0.9390047964366,0.9390047964366,0.9390047964366,0.9390047964366,0.9390047964366,
0.9390047964366,0.9390047964366,0.9390047964366,0.9390047964366,0.9390047964366,
0.9390047964366,0.9390047964366),(0.9390047964366,0.9390047964366,0.9390047964366,
0.9390047964366,0.9390047964366,0.9390047964366,0.9390047964366,0.9390047964366,
0.9390047964366,0.9390047964366,0.9390047964366,0.9390047964366,0.9390047964366,
0.9390047964366,0.9390047964366,0.9390047964366,0.9390047964366,0.9390047964366,
0.9390047964366),(1.18298561069,1.18298561069,1.18298561069,1.18298561069,
1.18298561069,1.18298561069,1.18298561069,1.18298561069,1.18298561069,1.18298561069,
1.18298561069,1.18298561069,1.18298561069,1.18298561069,1.18298561069,1.18298561069,
1.18298561069,1.18298561069,1.18298561069)))
REPRESENTATION_ITEM('')
SURFACE()
);
#2471=(
BOUNDED_SURFACE()
B_SPLINE_SURFACE(3,3,((#128523,#128524,#128525,#128526,#128527,#128528,
#128529,#128530,#128531,#128532,#128533,#128534),(#128535,#128536,#128537,
#128538,#128539,#128540,#128541,#128542,#128543,#128544,#128545,#128546),
(#128547,#128548,#128549,#128550,#128551,#128552,#128553,#128554,#128555,
#128556,#128557,#128558),(#128559,#128560,#128561,#128562,#128563,#128564,
#128565,#128566,#128567,#128568,#128569,#128570),(#128571,#128572,#128573,
#128574,#128575,#128576,#128577,#128578,#128579,#128580,#128581,#128582),
(#128583,#128584,#128585,#128586,#128587,#128588,#128589,#128590,#128591,
#128592,#128593,#128594),(#128595,#128596,#128597,#128598,#128599,#128600,
#128601,#128602,#128603,#128604,#128605,#128606)),.UNSPECIFIED.,.F.,.F.,
 .F.)
B_SPLINE_SURFACE_WITH_KNOTS((4,3,4),(4,1,1,1,1,1,1,1,1,4),(0.,0.5,1.),(0.,
0.121564102375813,0.245468926981195,0.369653809053026,0.494206194236183,
0.619223276452004,0.744802842314215,0.871034840780298,0.998000117655881,
1.),.UNSPECIFIED.)
GEOMETRIC_REPRESENTATION_ITEM()
RATIONAL_B_SPLINE_SURFACE(((1.193853494575,1.193853494575,1.193853494575,
1.193853494575,1.193853494575,1.193853494575,1.193853494575,1.193853494575,
1.193853494575,1.193853494575,1.193853494575,1.193853494575),(0.9353821684751,
0.9353821684751,0.9353821684751,0.9353821684751,0.9353821684751,0.9353821684751,
0.9353821684751,0.9353821684751,0.9353821684751,0.9353821684751,0.9353821684751,
0.9353821684751),(0.9353821684751,0.9353821684751,0.9353821684751,0.9353821684751,
0.9353821684751,0.9353821684751,0.9353821684751,0.9353821684751,0.9353821684751,
0.9353821684751,0.9353821684751,0.9353821684751),(1.193853494575,1.193853494575,
1.193853494575,1.193853494575,1.193853494575,1.193853494575,1.193853494575,
1.193853494575,1.193853494575,1.193853494575,1.193853494575,1.193853494575),
(0.9353821684751,0.9353821684751,0.9353821684751,0.9353821684751,0.9353821684751,
0.9353821684751,0.9353821684751,0.9353821684751,0.9353821684751,0.9353821684751,
0.9353821684751,0.9353821684751),(0.9353821684751,0.9353821684751,0.9353821684751,
0.9353821684751,0.9353821684751,0.9353821684751,0.9353821684751,0.9353821684751,
0.9353821684751,0.9353821684751,0.9353821684751,0.9353821684751),(1.193853494575,
1.193853494575,1.193853494575,1.193853494575,1.193853494575,1.193853494575,
1.193853494575,1.193853494575,1.193853494575,1.193853494575,1.193853494575,
1.193853494575)))
REPRESENTATION_ITEM('')
SURFACE()
);
#2472=(
BOUNDED_SURFACE()
B_SPLINE_SURFACE(3,3,((#130378,#130379,#130380,#130381,#130382),(#130383,
#130384,#130385,#130386,#130387),(#130388,#130389,#130390,#130391,#130392),
(#130393,#130394,#130395,#130396,#130397)),.UNSPECIFIED.,.F.,.F.,.F.)
B_SPLINE_SURFACE_WITH_KNOTS((4,4),(4,1,4),(0.,1.),(0.,0.0723197122150453,
1.),.UNSPECIFIED.)
GEOMETRIC_REPRESENTATION_ITEM()
RATIONAL_B_SPLINE_SURFACE(((1.229651833258,1.229651833258,1.229651833258,
1.229651833258,1.229651833258),(0.9234493889141,0.9234493889141,0.9234493889141,
0.9234493889141,0.9234493889141),(0.9234493889141,0.9234493889141,0.9234493889141,
0.9234493889141,0.9234493889141),(1.229651833258,1.229651833258,1.229651833258,
1.229651833258,1.229651833258)))
REPRESENTATION_ITEM('')
SURFACE()
);
#2473=(
BOUNDED_SURFACE()
B_SPLINE_SURFACE(3,3,((#130463,#130464,#130465,#130466,#130467,#130468,
#130469,#130470,#130471,#130472,#130473,#130474,#130475,#130476,#130477,
#130478,#130479,#130480,#130481,#130482),(#130483,#130484,#130485,#130486,
#130487,#130488,#130489,#130490,#130491,#130492,#130493,#130494,#130495,
#130496,#130497,#130498,#130499,#130500,#130501,#130502),(#130503,#130504,
#130505,#130506,#130507,#130508,#130509,#130510,#130511,#130512,#130513,
#130514,#130515,#130516,#130517,#130518,#130519,#130520,#130521,#130522),
(#130523,#130524,#130525,#130526,#130527,#130528,#130529,#130530,#130531,
#130532,#130533,#130534,#130535,#130536,#130537,#130538,#130539,#130540,
#130541,#130542)),.UNSPECIFIED.,.F.,.F.,.F.)
B_SPLINE_SURFACE_WITH_KNOTS((4,4),(4,1,1,1,1,1,1,1,1,1,1,1,1,1,1,1,1,4),
(0.,1.),(0.,0.0396611801962909,0.0991280080993822,0.158967060305227,0.213500355613908,
0.265743805592041,0.31877970559442,0.372320929804579,0.42550049560743,0.477326879186013,
0.531755535132276,0.594383860510548,0.661759309442457,0.728996536779342,
0.791903310438717,0.857857310969531,0.931521029517504,1.),.UNSPECIFIED.)
GEOMETRIC_REPRESENTATION_ITEM()
RATIONAL_B_SPLINE_SURFACE(((1.186027134151,1.186027134151,1.186027134151,
1.186027134151,1.186027134151,1.186027134151,1.186027134151,1.186027134151,
1.186027134151,1.186027134151,1.186027134151,1.186027134151,1.186027134151,
1.186027134151,1.186027134151,1.186027134151,1.186027134151,1.186027134151,
1.186027134151,1.186027134151),(0.9379909552829,0.9379909552829,0.9379909552829,
0.9379909552829,0.9379909552829,0.9379909552829,0.9379909552829,0.9379909552829,
0.9379909552829,0.9379909552829,0.9379909552829,0.9379909552829,0.9379909552829,
0.9379909552829,0.9379909552829,0.9379909552829,0.9379909552829,0.9379909552829,
0.9379909552829,0.9379909552829),(0.9379909552829,0.9379909552829,0.9379909552829,
0.9379909552829,0.9379909552829,0.9379909552829,0.9379909552829,0.9379909552829,
0.9379909552829,0.9379909552829,0.9379909552829,0.9379909552829,0.9379909552829,
0.9379909552829,0.9379909552829,0.9379909552829,0.9379909552829,0.9379909552829,
0.9379909552829,0.9379909552829),(1.186027134151,1.186027134151,1.186027134151,
1.186027134151,1.186027134151,1.186027134151,1.186027134151,1.186027134151,
1.186027134151,1.186027134151,1.186027134151,1.186027134151,1.186027134151,
1.186027134151,1.186027134151,1.186027134151,1.186027134151,1.186027134151,
1.186027134151,1.186027134151)))
REPRESENTATION_ITEM('')
SURFACE()
);
#2474=(
BOUNDED_SURFACE()
B_SPLINE_SURFACE(3,3,((#131452,#131453,#131454,#131455,#131456,#131457,
#131458,#131459,#131460,#131461,#131462,#131463,#131464,#131465,#131466,
#131467,#131468,#131469),(#131470,#131471,#131472,#131473,#131474,#131475,
#131476,#131477,#131478,#131479,#131480,#131481,#131482,#131483,#131484,
#131485,#131486,#131487),(#131488,#131489,#131490,#131491,#131492,#131493,
#131494,#131495,#131496,#131497,#131498,#131499,#131500,#131501,#131502,
#131503,#131504,#131505),(#131506,#131507,#131508,#131509,#131510,#131511,
#131512,#131513,#131514,#131515,#131516,#131517,#131518,#131519,#131520,
#131521,#131522,#131523)),.UNSPECIFIED.,.F.,.F.,.F.)
B_SPLINE_SURFACE_WITH_KNOTS((4,4),(4,1,1,1,1,1,1,1,1,1,1,1,1,1,1,4),(0.,
1.),(0.,0.0565664707614419,0.138737193301063,0.216966583065079,0.292764930742884,
0.367550058790166,0.442396912571936,0.51714275336354,0.591290850026512,
0.664372024038177,0.735878178033487,0.805267355840292,0.8719728304485,0.935407611159442,
0.994981558271123,1.),.UNSPECIFIED.)
GEOMETRIC_REPRESENTATION_ITEM()
RATIONAL_B_SPLINE_SURFACE(((1.117361802752,1.117361802752,1.117361802752,
1.117361802752,1.117361802752,1.117361802752,1.117361802752,1.117361802752,
1.117361802752,1.117361802752,1.117361802752,1.117361802752,1.117361802752,
1.117361802752,1.117361802752,1.117361802752,1.117361802752,1.117361802752),
(0.9608793990826,0.9608793990826,0.9608793990826,0.9608793990826,0.9608793990826,
0.9608793990826,0.9608793990826,0.9608793990826,0.9608793990826,0.9608793990826,
0.9608793990826,0.9608793990826,0.9608793990826,0.9608793990826,0.9608793990826,
0.9608793990826,0.9608793990826,0.9608793990826),(0.9608793990826,0.9608793990826,
0.9608793990826,0.9608793990826,0.9608793990826,0.9608793990826,0.9608793990826,
0.9608793990826,0.9608793990826,0.9608793990826,0.9608793990826,0.9608793990826,
0.9608793990826,0.9608793990826,0.9608793990826,0.9608793990826,0.9608793990826,
0.9608793990826),(1.117361802752,1.117361802752,1.117361802752,1.117361802752,
1.117361802752,1.117361802752,1.117361802752,1.117361802752,1.117361802752,
1.117361802752,1.117361802752,1.117361802752,1.117361802752,1.117361802752,
1.117361802752,1.117361802752,1.117361802752,1.117361802752)))
REPRESENTATION_ITEM('')
SURFACE()
);
#2475=(
BOUNDED_SURFACE()
B_SPLINE_SURFACE(3,3,((#131671,#131672,#131673,#131674,#131675,#131676,
#131677,#131678,#131679,#131680,#131681,#131682,#131683,#131684,#131685),
(#131686,#131687,#131688,#131689,#131690,#131691,#131692,#131693,#131694,
#131695,#131696,#131697,#131698,#131699,#131700),(#131701,#131702,#131703,
#131704,#131705,#131706,#131707,#131708,#131709,#131710,#131711,#131712,
#131713,#131714,#131715),(#131716,#131717,#131718,#131719,#131720,#131721,
#131722,#131723,#131724,#131725,#131726,#131727,#131728,#131729,#131730)),
 .UNSPECIFIED.,.F.,.F.,.F.)
B_SPLINE_SURFACE_WITH_KNOTS((4,4),(4,1,1,1,1,1,1,1,1,1,1,1,4),(0.,1.),(0.,
0.00433344281298221,0.0666934882632817,0.132801776489929,0.205016366496403,
0.284357715917161,0.370665202265106,0.46484948769096,0.568277692564041,
0.682614773264253,0.810064514841178,0.952973196107536,1.),.UNSPECIFIED.)
GEOMETRIC_REPRESENTATION_ITEM()
RATIONAL_B_SPLINE_SURFACE(((1.116717554521,1.116717554521,1.116717554521,
1.116717554521,1.116717554521,1.116717554521,1.116717554521,1.116717554521,
1.116717554521,1.116717554521,1.116717554521,1.116717554521,1.116717554521,
1.116717554521,1.116717554521),(0.9610941484931,0.9610941484931,0.9610941484931,
0.9610941484931,0.9610941484931,0.9610941484931,0.9610941484931,0.9610941484931,
0.9610941484931,0.9610941484931,0.9610941484931,0.9610941484931,0.9610941484931,
0.9610941484931,0.9610941484931),(0.9610941484931,0.9610941484931,0.9610941484931,
0.9610941484931,0.9610941484931,0.9610941484931,0.9610941484931,0.9610941484931,
0.9610941484931,0.9610941484931,0.9610941484931,0.9610941484931,0.9610941484931,
0.9610941484931,0.9610941484931),(1.116717554521,1.116717554521,1.116717554521,
1.116717554521,1.116717554521,1.116717554521,1.116717554521,1.116717554521,
1.116717554521,1.116717554521,1.116717554521,1.116717554521,1.116717554521,
1.116717554521,1.116717554521)))
REPRESENTATION_ITEM('')
SURFACE()
);
#2476=(
BOUNDED_SURFACE()
B_SPLINE_SURFACE(3,3,((#131768,#131769,#131770,#131771),(#131772,#131773,
#131774,#131775),(#131776,#131777,#131778,#131779),(#131780,#131781,#131782,
#131783)),.UNSPECIFIED.,.F.,.F.,.F.)
B_SPLINE_SURFACE_WITH_KNOTS((4,4),(4,4),(0.,1.),(0.,1.),.UNSPECIFIED.)
GEOMETRIC_REPRESENTATION_ITEM()
RATIONAL_B_SPLINE_SURFACE(((1.1173473569,1.1173473569,1.1173473569,1.1173473569),
(0.9608842143667,0.9608842143667,0.9608842143667,0.9608842143667),(0.9608842143667,
0.9608842143667,0.9608842143667,0.9608842143667),(1.1173473569,1.1173473569,
1.1173473569,1.1173473569)))
REPRESENTATION_ITEM('')
SURFACE()
);
#2477=(
BOUNDED_SURFACE()
B_SPLINE_SURFACE(3,3,((#131784,#131785,#131786,#131787,#131788,#131789,
#131790,#131791,#131792,#131793,#131794,#131795,#131796,#131797,#131798,
#131799,#131800,#131801,#131802,#131803),(#131804,#131805,#131806,#131807,
#131808,#131809,#131810,#131811,#131812,#131813,#131814,#131815,#131816,
#131817,#131818,#131819,#131820,#131821,#131822,#131823),(#131824,#131825,
#131826,#131827,#131828,#131829,#131830,#131831,#131832,#131833,#131834,
#131835,#131836,#131837,#131838,#131839,#131840,#131841,#131842,#131843),
(#131844,#131845,#131846,#131847,#131848,#131849,#131850,#131851,#131852,
#131853,#131854,#131855,#131856,#131857,#131858,#131859,#131860,#131861,
#131862,#131863)),.UNSPECIFIED.,.F.,.F.,.F.)
B_SPLINE_SURFACE_WITH_KNOTS((4,4),(4,1,1,1,1,1,1,1,1,1,1,1,1,1,1,1,1,4),
(0.,1.),(0.,0.0634473073458767,0.137474475480583,0.203439315591922,0.266070813426101,
0.333494447777073,0.401437472430427,0.464401084256882,0.51858368764375,
0.569769560865856,0.622221496328389,0.67514181525029,0.727526446084146,
0.778774499915783,0.832231436034466,0.891640084181608,0.951727885385323,
1.),.UNSPECIFIED.)
GEOMETRIC_REPRESENTATION_ITEM()
RATIONAL_B_SPLINE_SURFACE(((1.186029185783,1.186029185783,1.186029185783,
1.186029185783,1.186029185783,1.186029185783,1.186029185783,1.186029185783,
1.186029185783,1.186029185783,1.186029185783,1.186029185783,1.186029185783,
1.186029185783,1.186029185783,1.186029185783,1.186029185783,1.186029185783,
1.186029185783,1.186029185783),(0.9379902714058,0.9379902714058,0.9379902714058,
0.9379902714058,0.9379902714058,0.9379902714058,0.9379902714058,0.9379902714058,
0.9379902714058,0.9379902714058,0.9379902714058,0.9379902714058,0.9379902714058,
0.9379902714058,0.9379902714058,0.9379902714058,0.9379902714058,0.9379902714058,
0.9379902714058,0.9379902714058),(0.9379902714058,0.9379902714058,0.9379902714058,
0.9379902714058,0.9379902714058,0.9379902714058,0.9379902714058,0.9379902714058,
0.9379902714058,0.9379902714058,0.9379902714058,0.9379902714058,0.9379902714058,
0.9379902714058,0.9379902714058,0.9379902714058,0.9379902714058,0.9379902714058,
0.9379902714058,0.9379902714058),(1.186029185783,1.186029185783,1.186029185783,
1.186029185783,1.186029185783,1.186029185783,1.186029185783,1.186029185783,
1.186029185783,1.186029185783,1.186029185783,1.186029185783,1.186029185783,
1.186029185783,1.186029185783,1.186029185783,1.186029185783,1.186029185783,
1.186029185783,1.186029185783)))
REPRESENTATION_ITEM('')
SURFACE()
);
#2478=(
BOUNDED_SURFACE()
B_SPLINE_SURFACE(3,3,((#131894,#131895,#131896,#131897,#131898,#131899,
#131900,#131901,#131902,#131903,#131904,#131905,#131906,#131907),(#131908,
#131909,#131910,#131911,#131912,#131913,#131914,#131915,#131916,#131917,
#131918,#131919,#131920,#131921),(#131922,#131923,#131924,#131925,#131926,
#131927,#131928,#131929,#131930,#131931,#131932,#131933,#131934,#131935),
(#131936,#131937,#131938,#131939,#131940,#131941,#131942,#131943,#131944,
#131945,#131946,#131947,#131948,#131949)),.UNSPECIFIED.,.F.,.F.,.F.)
B_SPLINE_SURFACE_WITH_KNOTS((4,4),(4,1,1,1,1,1,1,1,1,1,1,4),(0.,1.),(0.,
0.025958376473271,0.179859171762141,0.318182203672271,0.441108132212019,
0.551634708740777,0.651710515506557,0.743010369069283,0.826230829945666,
0.901572688650554,0.970015580606343,1.),.UNSPECIFIED.)
GEOMETRIC_REPRESENTATION_ITEM()
RATIONAL_B_SPLINE_SURFACE(((1.116719050321,1.116719050321,1.116719050321,
1.116719050321,1.116719050321,1.116719050321,1.116719050321,1.116719050321,
1.116719050321,1.116719050321,1.116719050321,1.116719050321,1.116719050321,
1.116719050321),(0.961093649893,0.961093649893,0.961093649893,0.961093649893,
0.961093649893,0.961093649893,0.961093649893,0.961093649893,0.961093649893,
0.961093649893,0.961093649893,0.961093649893,0.961093649893,0.961093649893),
(0.961093649893,0.961093649893,0.961093649893,0.961093649893,0.961093649893,
0.961093649893,0.961093649893,0.961093649893,0.961093649893,0.961093649893,
0.961093649893,0.961093649893,0.961093649893,0.961093649893),(1.116719050321,
1.116719050321,1.116719050321,1.116719050321,1.116719050321,1.116719050321,
1.116719050321,1.116719050321,1.116719050321,1.116719050321,1.116719050321,
1.116719050321,1.116719050321,1.116719050321)))
REPRESENTATION_ITEM('')
SURFACE()
);
#2479=(
BOUNDED_SURFACE()
B_SPLINE_SURFACE(3,3,((#131951,#131952,#131953,#131954),(#131955,#131956,
#131957,#131958),(#131959,#131960,#131961,#131962),(#131963,#131964,#131965,
#131966)),.UNSPECIFIED.,.F.,.F.,.F.)
B_SPLINE_SURFACE_WITH_KNOTS((4,4),(4,4),(0.,1.),(0.,1.),.UNSPECIFIED.)
GEOMETRIC_REPRESENTATION_ITEM()
RATIONAL_B_SPLINE_SURFACE(((1.117354081969,1.117354081969,1.117354081969,
1.117354081969),(0.9608819726769,0.9608819726769,0.9608819726769,0.9608819726769),
(0.9608819726769,0.9608819726769,0.9608819726769,0.9608819726769),(1.117354081969,
1.117354081969,1.117354081969,1.117354081969)))
REPRESENTATION_ITEM('')
SURFACE()
);
#2480=(
BOUNDED_SURFACE()
B_SPLINE_SURFACE(3,3,((#131977,#131978,#131979,#131980,#131981,#131982,
#131983,#131984,#131985,#131986,#131987,#131988,#131989,#131990,#131991,
#131992,#131993,#131994),(#131995,#131996,#131997,#131998,#131999,#132000,
#132001,#132002,#132003,#132004,#132005,#132006,#132007,#132008,#132009,
#132010,#132011,#132012),(#132013,#132014,#132015,#132016,#132017,#132018,
#132019,#132020,#132021,#132022,#132023,#132024,#132025,#132026,#132027,
#132028,#132029,#132030),(#132031,#132032,#132033,#132034,#132035,#132036,
#132037,#132038,#132039,#132040,#132041,#132042,#132043,#132044,#132045,
#132046,#132047,#132048)),.UNSPECIFIED.,.F.,.F.,.F.)
B_SPLINE_SURFACE_WITH_KNOTS((4,4),(4,1,1,1,1,1,1,1,1,1,1,1,1,1,1,4),(0.,
1.),(0.,0.000242963129974397,0.0605980029967337,0.126012042753347,0.195352701343378,
0.267486808827858,0.341302963992409,0.415716209072041,0.489674476326956,
0.56246465276733,0.634611827570827,0.706994977225878,0.780514441156784,
0.856110535001656,0.934799701636564,1.),.UNSPECIFIED.)
GEOMETRIC_REPRESENTATION_ITEM()
RATIONAL_B_SPLINE_SURFACE(((1.117353920691,1.117353920691,1.117353920691,
1.117353920691,1.117353920691,1.117353920691,1.117353920691,1.117353920691,
1.117353920691,1.117353920691,1.117353920691,1.117353920691,1.117353920691,
1.117353920691,1.117353920691,1.117353920691,1.117353920691,1.117353920691),
(0.9608820264364,0.9608820264364,0.9608820264364,0.9608820264364,0.9608820264364,
0.9608820264364,0.9608820264364,0.9608820264364,0.9608820264364,0.9608820264364,
0.9608820264364,0.9608820264364,0.9608820264364,0.9608820264364,0.9608820264364,
0.9608820264364,0.9608820264364,0.9608820264364),(0.9608820264364,0.9608820264364,
0.9608820264364,0.9608820264364,0.9608820264364,0.9608820264364,0.9608820264364,
0.9608820264364,0.9608820264364,0.9608820264364,0.9608820264364,0.9608820264364,
0.9608820264364,0.9608820264364,0.9608820264364,0.9608820264364,0.9608820264364,
0.9608820264364),(1.117353920691,1.117353920691,1.117353920691,1.117353920691,
1.117353920691,1.117353920691,1.117353920691,1.117353920691,1.117353920691,
1.117353920691,1.117353920691,1.117353920691,1.117353920691,1.117353920691,
1.117353920691,1.117353920691,1.117353920691,1.117353920691)))
REPRESENTATION_ITEM('')
SURFACE()
);
#2481=(
BOUNDED_SURFACE()
B_SPLINE_SURFACE(3,3,((#132299,#132300,#132301,#132302,#132303,#132304,
#132305,#132306),(#132307,#132308,#132309,#132310,#132311,#132312,#132313,
#132314),(#132315,#132316,#132317,#132318,#132319,#132320,#132321,#132322),
(#132323,#132324,#132325,#132326,#132327,#132328,#132329,#132330)),
 .UNSPECIFIED.,.F.,.F.,.F.)
B_SPLINE_SURFACE_WITH_KNOTS((4,4),(4,1,1,1,1,4),(0.,1.),(0.,0.120712626123964,
0.331920437096621,0.562126515133101,0.816265604424358,1.),.UNSPECIFIED.)
GEOMETRIC_REPRESENTATION_ITEM()
RATIONAL_B_SPLINE_SURFACE(((1.229639485543,1.229639485543,1.229639485543,
1.229639485543,1.229639485543,1.229639485543,1.229639485543,1.229639485543),
(0.9234535048188,0.9234535048188,0.9234535048188,0.9234535048188,0.9234535048188,
0.9234535048188,0.9234535048188,0.9234535048188),(0.9234535048188,0.9234535048188,
0.9234535048188,0.9234535048188,0.9234535048188,0.9234535048188,0.9234535048188,
0.9234535048188),(1.229639485543,1.229639485543,1.229639485543,1.229639485543,
1.229639485543,1.229639485543,1.229639485543,1.229639485543)))
REPRESENTATION_ITEM('')
SURFACE()
);
#2482=(
BOUNDED_SURFACE()
B_SPLINE_SURFACE(3,3,((#132549,#132550,#132551,#132552,#132553,#132554,
#132555,#132556,#132557),(#132558,#132559,#132560,#132561,#132562,#132563,
#132564,#132565,#132566),(#132567,#132568,#132569,#132570,#132571,#132572,
#132573,#132574,#132575),(#132576,#132577,#132578,#132579,#132580,#132581,
#132582,#132583,#132584)),.UNSPECIFIED.,.F.,.F.,.F.)
B_SPLINE_SURFACE_WITH_KNOTS((4,4),(4,1,1,1,1,1,4),(0.,1.),(0.,0.0837316477041681,
0.294311209377657,0.486443539434301,0.667285087674737,0.84576890430481,
1.),.UNSPECIFIED.)
GEOMETRIC_REPRESENTATION_ITEM()
RATIONAL_B_SPLINE_SURFACE(((1.00893514375611,1.00893514375611,1.00893514375611,
1.00893514375611,1.00893514375611,1.00893514375611,1.00893514375611,1.00893514375611,
1.00893514375611),(1.01179069517864,1.01179069517864,1.01179069517864,1.01179069517864,
1.01179069517864,1.01179069517864,1.01179069517864,1.01179069517864,1.01179069517864),
(1.01533069338925,1.01533069338925,1.01533069338925,1.01533069338925,1.01533069338925,
1.01533069338925,1.01533069338925,1.01533069338925,1.01533069338925),(1.01955513838796,
1.01955513838796,1.01955513838796,1.01955513838796,1.01955513838796,1.01955513838796,
1.01955513838796,1.01955513838796,1.01955513838796)))
REPRESENTATION_ITEM('')
SURFACE()
);
#2483=(
BOUNDED_SURFACE()
B_SPLINE_SURFACE(3,3,((#132594,#132595,#132596,#132597,#132598,#132599,
#132600,#132601,#132602),(#132603,#132604,#132605,#132606,#132607,#132608,
#132609,#132610,#132611),(#132612,#132613,#132614,#132615,#132616,#132617,
#132618,#132619,#132620),(#132621,#132622,#132623,#132624,#132625,#132626,
#132627,#132628,#132629)),.UNSPECIFIED.,.F.,.F.,.F.)
B_SPLINE_SURFACE_WITH_KNOTS((4,4),(4,1,1,1,1,1,4),(0.,1.),(0.,0.0837316477041681,
0.294311209377657,0.486443539434301,0.667285087674737,0.84576890430481,
1.),.UNSPECIFIED.)
GEOMETRIC_REPRESENTATION_ITEM()
RATIONAL_B_SPLINE_SURFACE(((1.01955513838796,1.01955513838796,1.01955513838796,
1.01955513838796,1.01955513838796,1.01955513838796,1.01955513838796,1.01955513838796,
1.01955513838796),(1.03766231011378,1.03766231011378,1.03766231011378,1.03766231011378,
1.03766231011378,1.03766231011378,1.03766231011378,1.03766231011378,1.03766231011378),
(1.06834429701362,1.06834429701362,1.06834429701362,1.06834429701362,1.06834429701362,
1.06834429701362,1.06834429701362,1.06834429701362,1.06834429701362),(1.11160109908747,
1.11160109908747,1.11160109908747,1.11160109908747,1.11160109908747,1.11160109908747,
1.11160109908747,1.11160109908747,1.11160109908747)))
REPRESENTATION_ITEM('')
SURFACE()
);
#2484=(
BOUNDED_SURFACE()
B_SPLINE_SURFACE(3,3,((#132643,#132644,#132645,#132646,#132647,#132648,
#132649,#132650,#132651,#132652,#132653,#132654,#132655,#132656,#132657,
#132658,#132659,#132660,#132661,#132662,#132663),(#132664,#132665,#132666,
#132667,#132668,#132669,#132670,#132671,#132672,#132673,#132674,#132675,
#132676,#132677,#132678,#132679,#132680,#132681,#132682,#132683,#132684),
(#132685,#132686,#132687,#132688,#132689,#132690,#132691,#132692,#132693,
#132694,#132695,#132696,#132697,#132698,#132699,#132700,#132701,#132702,
#132703,#132704,#132705),(#132706,#132707,#132708,#132709,#132710,#132711,
#132712,#132713,#132714,#132715,#132716,#132717,#132718,#132719,#132720,
#132721,#132722,#132723,#132724,#132725,#132726)),.UNSPECIFIED.,.F.,.F.,
 .F.)
B_SPLINE_SURFACE_WITH_KNOTS((4,4),(4,1,1,1,1,1,1,1,1,1,1,1,1,1,1,1,1,1,
4),(0.,1.),(0.,0.0546624749950295,0.160757685575355,0.256729617165409,0.343735196321369,
0.422731592898268,0.494638559250071,0.560248549174547,0.620252323655667,
0.6753431121518,0.726138185608107,0.772911121896331,0.815853204906754,0.855219379345603,
0.891312858927466,0.92449329904142,0.955123399607878,0.983429063756098,
1.),.UNSPECIFIED.)
GEOMETRIC_REPRESENTATION_ITEM()
RATIONAL_B_SPLINE_SURFACE(((1.11300250285163,1.11300250285163,1.11300250285163,
1.11300250285163,1.11300250285163,1.11300250285163,1.11300250285163,1.11300250285163,
1.11300250285163,1.11300250285163,1.11300250285163,1.11300250285163,1.11300250285163,
1.11300250285163,1.11300250285163,1.11300250285163,1.11300250285163,1.11300250285163,
1.11300250285163,1.11300250285163,1.11300250285163),(1.04579493402343,1.04579493402343,
1.04579493402343,1.04579493402343,1.04579493402343,1.04579493402343,1.04579493402343,
1.04579493402343,1.04579493402343,1.04579493402343,1.04579493402343,1.04579493402343,
1.04579493402343,1.04579493402343,1.04579493402343,1.04579493402343,1.04579493402343,
1.04579493402343,1.04579493402343,1.04579493402343,1.04579493402343),(1.00856584262147,
1.00856584262147,1.00856584262147,1.00856584262147,1.00856584262147,1.00856584262147,
1.00856584262147,1.00856584262147,1.00856584262147,1.00856584262147,1.00856584262147,
1.00856584262147,1.00856584262147,1.00856584262147,1.00856584262147,1.00856584262147,
1.00856584262147,1.00856584262147,1.00856584262147,1.00856584262147,1.00856584262147),
(1.00131522864575,1.00131522864575,1.00131522864575,1.00131522864575,1.00131522864575,
1.00131522864575,1.00131522864575,1.00131522864575,1.00131522864575,1.00131522864575,
1.00131522864575,1.00131522864575,1.00131522864575,1.00131522864575,1.00131522864575,
1.00131522864575,1.00131522864575,1.00131522864575,1.00131522864575,1.00131522864575,
1.00131522864575)))
REPRESENTATION_ITEM('')
SURFACE()
);
#2485=(
BOUNDED_SURFACE()
B_SPLINE_SURFACE(3,3,((#132823,#132824,#132825,#132826,#132827,#132828),
(#132829,#132830,#132831,#132832,#132833,#132834),(#132835,#132836,#132837,
#132838,#132839,#132840),(#132841,#132842,#132843,#132844,#132845,#132846)),
 .UNSPECIFIED.,.F.,.F.,.F.)
B_SPLINE_SURFACE_WITH_KNOTS((4,4),(4,1,1,4),(0.,1.),(0.,0.0270381251289528,
0.669758370381433,1.),.UNSPECIFIED.)
GEOMETRIC_REPRESENTATION_ITEM()
RATIONAL_B_SPLINE_SURFACE(((1.02521912049085,1.02521912049085,1.02521912049085,
1.02521912049085,1.02521912049085,1.02521912049085),(1.01907532458687,1.01907532458687,
1.01907532458687,1.01907532458687,1.01907532458687,1.01907532458687),(1.0140540765962,
1.0140540765962,1.0140540765962,1.0140540765962,1.0140540765962,1.0140540765962),
(1.01015537651883,1.01015537651883,1.01015537651883,1.01015537651883,1.01015537651883,
1.01015537651883)))
REPRESENTATION_ITEM('')
SURFACE()
);
#2486=(
BOUNDED_SURFACE()
B_SPLINE_SURFACE(3,3,((#132883,#132884,#132885,#132886,#132887,#132888,
#132889,#132890),(#132891,#132892,#132893,#132894,#132895,#132896,#132897,
#132898),(#132899,#132900,#132901,#132902,#132903,#132904,#132905,#132906),
(#132907,#132908,#132909,#132910,#132911,#132912,#132913,#132914)),
 .UNSPECIFIED.,.F.,.F.,.F.)
B_SPLINE_SURFACE_WITH_KNOTS((4,4),(4,1,1,1,1,4),(0.,1.),(0.,0.105738953419075,
0.324437351992926,0.56483220773929,0.829287264033599,1.),.UNSPECIFIED.)
GEOMETRIC_REPRESENTATION_ITEM()
RATIONAL_B_SPLINE_SURFACE(((1.01015537651883,1.01015537651883,1.01015537651883,
1.01015537651883,1.01015537651883,1.01015537651883,1.01015537651883,1.01015537651883),
(1.00780920781131,1.00780920781131,1.00780920781131,1.00780920781131,1.00780920781131,
1.00780920781131,1.00780920781131,1.00780920781131),(1.00586956078178,1.00586956078178,
1.00586956078178,1.00586956078178,1.00586956078178,1.00586956078178,1.00586956078178,
1.00586956078178),(1.00433643543025,1.00433643543025,1.00433643543025,1.00433643543025,
1.00433643543025,1.00433643543025,1.00433643543025,1.00433643543025)))
REPRESENTATION_ITEM('')
SURFACE()
);
#2487=(
BOUNDED_SURFACE()
B_SPLINE_SURFACE(3,3,((#132933,#132934,#132935,#132936,#132937,#132938,
#132939,#132940),(#132941,#132942,#132943,#132944,#132945,#132946,#132947,
#132948),(#132949,#132950,#132951,#132952,#132953,#132954,#132955,#132956),
(#132957,#132958,#132959,#132960,#132961,#132962,#132963,#132964)),
 .UNSPECIFIED.,.F.,.F.,.F.)
B_SPLINE_SURFACE_WITH_KNOTS((4,4),(4,1,1,1,1,4),(0.,1.),(0.,0.105738953419075,
0.324437351992926,0.56483220773929,0.829287264033599,1.),.UNSPECIFIED.)
GEOMETRIC_REPRESENTATION_ITEM()
RATIONAL_B_SPLINE_SURFACE(((1.02521912049085,1.02521912049085,1.02521912049085,
1.02521912049085,1.02521912049085,1.02521912049085,1.02521912049085,1.02521912049085),
(1.01907532458687,1.01907532458687,1.01907532458687,1.01907532458687,1.01907532458687,
1.01907532458687,1.01907532458687,1.01907532458687),(1.0140540765962,1.0140540765962,
1.0140540765962,1.0140540765962,1.0140540765962,1.0140540765962,1.0140540765962,
1.0140540765962),(1.01015537651883,1.01015537651883,1.01015537651883,1.01015537651883,
1.01015537651883,1.01015537651883,1.01015537651883,1.01015537651883)))
REPRESENTATION_ITEM('')
SURFACE()
);
#2488=(
BOUNDED_SURFACE()
B_SPLINE_SURFACE(3,3,((#132996,#132997,#132998,#132999,#133000,#133001,
#133002,#133003,#133004,#133005,#133006,#133007,#133008,#133009,#133010,
#133011),(#133012,#133013,#133014,#133015,#133016,#133017,#133018,#133019,
#133020,#133021,#133022,#133023,#133024,#133025,#133026,#133027),(#133028,
#133029,#133030,#133031,#133032,#133033,#133034,#133035,#133036,#133037,
#133038,#133039,#133040,#133041,#133042,#133043),(#133044,#133045,#133046,
#133047,#133048,#133049,#133050,#133051,#133052,#133053,#133054,#133055,
#133056,#133057,#133058,#133059)),.UNSPECIFIED.,.F.,.F.,.F.)
B_SPLINE_SURFACE_WITH_KNOTS((4,4),(4,1,1,1,1,1,1,1,1,1,1,1,1,4),(0.,1.),
(0.,0.0186503236401621,0.0681861826858635,0.122274864726643,0.181134794327188,
0.244976288689619,0.314185121458223,0.389489559305443,0.47162927932211,
0.561313355930194,0.659220518921088,0.766025144246682,0.882569333512905,
1.),.UNSPECIFIED.)
GEOMETRIC_REPRESENTATION_ITEM()
RATIONAL_B_SPLINE_SURFACE(((1.00001053115096,1.00001053115096,1.00001053115096,
1.00001053115096,1.00001053115096,1.00001053115096,1.00001053115096,1.00001053115096,
1.00001053115096,1.00001053115096,1.00001053115096,1.00001053115096,1.00001053115096,
1.00001053115096,1.00001053115096,1.00001053115096),(0.999657107718199,
0.999657107718199,0.999657107718199,0.999657107718199,0.999657107718199,
0.999657107718199,0.999657107718199,0.999657107718199,0.999657107718199,
0.999657107718199,0.999657107718199,0.999657107718199,0.999657107718199,
0.999657107718199,0.999657107718199,0.999657107718199),(1.0081993019117,
1.0081993019117,1.0081993019117,1.0081993019117,1.0081993019117,1.0081993019117,
1.0081993019117,1.0081993019117,1.0081993019117,1.0081993019117,1.0081993019117,
1.0081993019117,1.0081993019117,1.0081993019117,1.0081993019117,1.0081993019117),
(1.02563711373146,1.02563711373146,1.02563711373146,1.02563711373146,1.02563711373146,
1.02563711373146,1.02563711373146,1.02563711373146,1.02563711373146,1.02563711373146,
1.02563711373146,1.02563711373146,1.02563711373146,1.02563711373146,1.02563711373146,
1.02563711373146)))
REPRESENTATION_ITEM('')
SURFACE()
);
#2489=(
BOUNDED_SURFACE()
B_SPLINE_SURFACE(3,3,((#133129,#133130,#133131,#133132,#133133,#133134),
(#133135,#133136,#133137,#133138,#133139,#133140),(#133141,#133142,#133143,
#133144,#133145,#133146),(#133147,#133148,#133149,#133150,#133151,#133152)),
 .UNSPECIFIED.,.F.,.F.,.F.)
B_SPLINE_SURFACE_WITH_KNOTS((4,4),(4,1,1,4),(0.,1.),(0.,0.0271721067421099,
0.646141430958428,1.),.UNSPECIFIED.)
GEOMETRIC_REPRESENTATION_ITEM()
RATIONAL_B_SPLINE_SURFACE(((1.00945321541545,1.00945321541545,1.00945321541545,
1.00945321541545,1.00945321541545,1.00945321541545),(1.01344341494481,1.01344341494481,
1.01344341494481,1.01344341494481,1.01344341494481,1.01344341494481),(1.01869681103622,
1.01869681103622,1.01869681103622,1.01869681103622,1.01869681103622,1.01869681103622),
(1.02521340368968,1.02521340368968,1.02521340368968,1.02521340368968,1.02521340368968,
1.02521340368968)))
REPRESENTATION_ITEM('')
SURFACE()
);
#2490=(
BOUNDED_SURFACE()
B_SPLINE_SURFACE(3,3,((#133174,#133175,#133176,#133177,#133178,#133179,
#133180,#133181),(#133182,#133183,#133184,#133185,#133186,#133187,#133188,
#133189),(#133190,#133191,#133192,#133193,#133194,#133195,#133196,#133197),
(#133198,#133199,#133200,#133201,#133202,#133203,#133204,#133205)),
 .UNSPECIFIED.,.F.,.F.,.F.)
B_SPLINE_SURFACE_WITH_KNOTS((4,4),(4,1,1,1,1,4),(0.,1.),(-0.00146608837293589,
0.0970814361513046,0.317736262577814,0.559494757859586,0.822645521844187,
1.00146608855681),.UNSPECIFIED.)
GEOMETRIC_REPRESENTATION_ITEM()
RATIONAL_B_SPLINE_SURFACE(((1.00945321541545,1.00945321541545,1.00945321541545,
1.00945321541545,1.00945321541545,1.00945321541545,1.00945321541545,1.00945321541545),
(1.01344341494481,1.01344341494481,1.01344341494481,1.01344341494481,1.01344341494481,
1.01344341494481,1.01344341494481,1.01344341494481),(1.01869681103622,1.01869681103622,
1.01869681103622,1.01869681103622,1.01869681103622,1.01869681103622,1.01869681103622,
1.01869681103622),(1.02521340368968,1.02521340368968,1.02521340368968,1.02521340368968,
1.02521340368968,1.02521340368968,1.02521340368968,1.02521340368968)))
REPRESENTATION_ITEM('')
SURFACE()
);
#2491=(
BOUNDED_SURFACE()
B_SPLINE_SURFACE(3,3,((#133216,#133217,#133218,#133219,#133220,#133221,
#133222,#133223),(#133224,#133225,#133226,#133227,#133228,#133229,#133230,
#133231),(#133232,#133233,#133234,#133235,#133236,#133237,#133238,#133239),
(#133240,#133241,#133242,#133243,#133244,#133245,#133246,#133247)),
 .UNSPECIFIED.,.F.,.F.,.F.)
B_SPLINE_SURFACE_WITH_KNOTS((4,4),(4,1,1,1,1,4),(0.,1.),(0.,0.0970814361513046,
0.317736262577814,0.559494757859586,0.822645521844187,1.),.UNSPECIFIED.)
GEOMETRIC_REPRESENTATION_ITEM()
RATIONAL_B_SPLINE_SURFACE(((1.00417423477067,1.00417423477067,1.00417423477067,
1.00417423477067,1.00417423477067,1.00417423477067,1.00417423477067,1.00417423477067),
(1.00557922143849,1.00557922143849,1.00557922143849,1.00557922143849,1.00557922143849,
1.00557922143849,1.00557922143849,1.00557922143849),(1.00733888165342,1.00733888165342,
1.00733888165342,1.00733888165342,1.00733888165342,1.00733888165342,1.00733888165342,
1.00733888165342),(1.00945321541545,1.00945321541545,1.00945321541545,1.00945321541545,
1.00945321541545,1.00945321541545,1.00945321541545,1.00945321541545)))
REPRESENTATION_ITEM('')
SURFACE()
);
#2492=(
BOUNDED_SURFACE()
B_SPLINE_SURFACE(3,3,((#133254,#133255,#133256,#133257,#133258,#133259,
#133260,#133261,#133262,#133263,#133264,#133265,#133266,#133267,#133268,
#133269,#133270),(#133271,#133272,#133273,#133274,#133275,#133276,#133277,
#133278,#133279,#133280,#133281,#133282,#133283,#133284,#133285,#133286,
#133287),(#133288,#133289,#133290,#133291,#133292,#133293,#133294,#133295,
#133296,#133297,#133298,#133299,#133300,#133301,#133302,#133303,#133304),
(#133305,#133306,#133307,#133308,#133309,#133310,#133311,#133312,#133313,
#133314,#133315,#133316,#133317,#133318,#133319,#133320,#133321)),
 .UNSPECIFIED.,.F.,.F.,.F.)
B_SPLINE_SURFACE_WITH_KNOTS((4,4),(4,1,1,1,1,1,1,1,1,1,1,1,1,1,4),(0.,1.),
(0.,0.0169119460810613,0.0654242130848353,0.118166345404895,0.175802236516308,
0.238929210760529,0.307690566088615,0.381894800562219,0.461375561007429,
0.546721723948187,0.639112945312709,0.739719346812922,0.849650913359874,
0.96995594614347,1.),.UNSPECIFIED.)
GEOMETRIC_REPRESENTATION_ITEM()
RATIONAL_B_SPLINE_SURFACE(((1.00000962163611,1.00000962163611,1.00000962163611,
1.00000962163611,1.00000962163611,1.00000962163611,1.00000962163611,1.00000962163611,
1.00000962163611,1.00000962163611,1.00000962163611,1.00000962163611,1.00000962163611,
1.00000962163611,1.00000962163611,1.00000962163611,1.00000962163611),(1.00033430815833,
1.00033430815833,1.00033430815833,1.00033430815833,1.00033430815833,1.00033430815833,
1.00033430815833,1.00033430815833,1.00033430815833,1.00033430815833,1.00033430815833,
1.00033430815833,1.00033430815833,1.00033430815833,1.00033430815833,1.00033430815833,
1.00033430815833),(1.00887651633456,1.00887651633456,1.00887651633456,1.00887651633456,
1.00887651633456,1.00887651633456,1.00887651633456,1.00887651633456,1.00887651633456,
1.00887651633456,1.00887651633456,1.00887651633456,1.00887651633456,1.00887651633456,
1.00887651633456,1.00887651633456,1.00887651633456),(1.02563624616481,1.02563624616481,
1.02563624616481,1.02563624616481,1.02563624616481,1.02563624616481,1.02563624616481,
1.02563624616481,1.02563624616481,1.02563624616481,1.02563624616481,1.02563624616481,
1.02563624616481,1.02563624616481,1.02563624616481,1.02563624616481,1.02563624616481)))
REPRESENTATION_ITEM('')
SURFACE()
);
#2493=(
BOUNDED_SURFACE()
B_SPLINE_SURFACE(3,3,((#133528,#133529,#133530,#133531,#133532,#133533,
#133534,#133535,#133536,#133537,#133538,#133539,#133540,#133541,#133542,
#133543,#133544,#133545,#133546,#133547),(#133548,#133549,#133550,#133551,
#133552,#133553,#133554,#133555,#133556,#133557,#133558,#133559,#133560,
#133561,#133562,#133563,#133564,#133565,#133566,#133567),(#133568,#133569,
#133570,#133571,#133572,#133573,#133574,#133575,#133576,#133577,#133578,
#133579,#133580,#133581,#133582,#133583,#133584,#133585,#133586,#133587),
(#133588,#133589,#133590,#133591,#133592,#133593,#133594,#133595,#133596,
#133597,#133598,#133599,#133600,#133601,#133602,#133603,#133604,#133605,
#133606,#133607)),.UNSPECIFIED.,.F.,.F.,.F.)
B_SPLINE_SURFACE_WITH_KNOTS((4,4),(4,1,1,1,1,1,1,1,1,1,1,1,1,1,1,1,1,4),
(0.,1.),(0.,0.0396611801962909,0.0991280080993822,0.158967060305227,0.213500355613908,
0.265743805592041,0.31877970559442,0.372320929804579,0.42550049560743,0.477326879186013,
0.531755535132276,0.594383860510548,0.661759309442457,0.728996536779342,
0.791903310438717,0.857857310969531,0.931521029517504,1.),.UNSPECIFIED.)
GEOMETRIC_REPRESENTATION_ITEM()
RATIONAL_B_SPLINE_SURFACE(((1.186027134151,1.186027134151,1.186027134151,
1.186027134151,1.186027134151,1.186027134151,1.186027134151,1.186027134151,
1.186027134151,1.186027134151,1.186027134151,1.186027134151,1.186027134151,
1.186027134151,1.186027134151,1.186027134151,1.186027134151,1.186027134151,
1.186027134151,1.186027134151),(0.9379909552829,0.9379909552829,0.9379909552829,
0.9379909552829,0.9379909552829,0.9379909552829,0.9379909552829,0.9379909552829,
0.9379909552829,0.9379909552829,0.9379909552829,0.9379909552829,0.9379909552829,
0.9379909552829,0.9379909552829,0.9379909552829,0.9379909552829,0.9379909552829,
0.9379909552829,0.9379909552829),(0.9379909552829,0.9379909552829,0.9379909552829,
0.9379909552829,0.9379909552829,0.9379909552829,0.9379909552829,0.9379909552829,
0.9379909552829,0.9379909552829,0.9379909552829,0.9379909552829,0.9379909552829,
0.9379909552829,0.9379909552829,0.9379909552829,0.9379909552829,0.9379909552829,
0.9379909552829,0.9379909552829),(1.186027134151,1.186027134151,1.186027134151,
1.186027134151,1.186027134151,1.186027134151,1.186027134151,1.186027134151,
1.186027134151,1.186027134151,1.186027134151,1.186027134151,1.186027134151,
1.186027134151,1.186027134151,1.186027134151,1.186027134151,1.186027134151,
1.186027134151,1.186027134151)))
REPRESENTATION_ITEM('')
SURFACE()
);
#2494=(
BOUNDED_SURFACE()
B_SPLINE_SURFACE(3,3,((#133731,#133732,#133733,#133734,#133735,#133736,
#133737,#133738,#133739,#133740),(#133741,#133742,#133743,#133744,#133745,
#133746,#133747,#133748,#133749,#133750),(#133751,#133752,#133753,#133754,
#133755,#133756,#133757,#133758,#133759,#133760),(#133761,#133762,#133763,
#133764,#133765,#133766,#133767,#133768,#133769,#133770)),.UNSPECIFIED.,
 .F.,.F.,.F.)
B_SPLINE_SURFACE_WITH_KNOTS((4,4),(4,1,1,1,1,1,1,4),(0.,1.),(0.,0.180483144409011,
0.376627636825192,0.555380925262604,0.717719202974124,0.864187978201653,
0.995189047099047,1.),.UNSPECIFIED.)
GEOMETRIC_REPRESENTATION_ITEM()
RATIONAL_B_SPLINE_SURFACE(((1.543563279584,1.543563279584,1.543563279584,
1.543563279584,1.543563279584,1.543563279584,1.543563279584,1.543563279584,
1.543563279584,1.543563279584),(0.8188122401388,0.8188122401388,0.8188122401388,
0.8188122401388,0.8188122401388,0.8188122401388,0.8188122401388,0.8188122401388,
0.8188122401388,0.8188122401388),(0.8188122401388,0.8188122401388,0.8188122401388,
0.8188122401388,0.8188122401388,0.8188122401388,0.8188122401388,0.8188122401388,
0.8188122401388,0.8188122401388),(1.543563279584,1.543563279584,1.543563279584,
1.543563279584,1.543563279584,1.543563279584,1.543563279584,1.543563279584,
1.543563279584,1.543563279584)))
REPRESENTATION_ITEM('')
SURFACE()
);
#2495=(
BOUNDED_SURFACE()
B_SPLINE_SURFACE(3,3,((#134090,#134091,#134092,#134093,#134094,#134095,
#134096,#134097,#134098,#134099),(#134100,#134101,#134102,#134103,#134104,
#134105,#134106,#134107,#134108,#134109),(#134110,#134111,#134112,#134113,
#134114,#134115,#134116,#134117,#134118,#134119),(#134120,#134121,#134122,
#134123,#134124,#134125,#134126,#134127,#134128,#134129)),.UNSPECIFIED.,
 .F.,.F.,.F.)
B_SPLINE_SURFACE_WITH_KNOTS((4,4),(4,1,1,1,1,1,1,4),(0.,1.),(0.,0.0801033777080447,
0.269947183593058,0.444907444701882,0.606049850917101,0.757247797830559,
0.903019663307709,1.),.UNSPECIFIED.)
GEOMETRIC_REPRESENTATION_ITEM()
RATIONAL_B_SPLINE_SURFACE(((1.289190167752,1.289190167752,1.289190167752,
1.289190167752,1.289190167752,1.289190167752,1.289190167752,1.289190167752,
1.289190167752,1.289190167752),(0.9036032774159,0.9036032774159,0.9036032774159,
0.9036032774159,0.9036032774159,0.9036032774159,0.9036032774159,0.9036032774159,
0.9036032774159,0.9036032774159),(0.9036032774159,0.9036032774159,0.9036032774159,
0.9036032774159,0.9036032774159,0.9036032774159,0.9036032774159,0.9036032774159,
0.9036032774159,0.9036032774159),(1.289190167752,1.289190167752,1.289190167752,
1.289190167752,1.289190167752,1.289190167752,1.289190167752,1.289190167752,
1.289190167752,1.289190167752)))
REPRESENTATION_ITEM('')
SURFACE()
);
#2496=(
BOUNDED_SURFACE()
B_SPLINE_SURFACE(3,3,((#134254,#134255,#134256,#134257,#134258,#134259,
#134260,#134261,#134262,#134263,#134264,#134265,#134266,#134267,#134268,
#134269,#134270,#134271,#134272,#134273,#134274,#134275,#134276),(#134277,
#134278,#134279,#134280,#134281,#134282,#134283,#134284,#134285,#134286,
#134287,#134288,#134289,#134290,#134291,#134292,#134293,#134294,#134295,
#134296,#134297,#134298,#134299),(#134300,#134301,#134302,#134303,#134304,
#134305,#134306,#134307,#134308,#134309,#134310,#134311,#134312,#134313,
#134314,#134315,#134316,#134317,#134318,#134319,#134320,#134321,#134322),
(#134323,#134324,#134325,#134326,#134327,#134328,#134329,#134330,#134331,
#134332,#134333,#134334,#134335,#134336,#134337,#134338,#134339,#134340,
#134341,#134342,#134343,#134344,#134345)),.UNSPECIFIED.,.F.,.F.,.F.)
B_SPLINE_SURFACE_WITH_KNOTS((4,4),(4,3,1,1,1,1,1,1,1,1,1,1,1,1,1,1,1,1,
4),(0.,1.),(-0.0877127999650316,0.,0.0438526529104932,0.0936371717010089,
0.147143943539872,0.203180298908346,0.261023062007613,0.320175420604179,
0.380280116633112,0.441075199270649,0.502372544364654,0.564033875272927,
0.62595494019857,0.68805881886387,0.75029079479597,0.812614800050668,0.875010812287183,
0.937472218801071,1.),.UNSPECIFIED.)
GEOMETRIC_REPRESENTATION_ITEM()
RATIONAL_B_SPLINE_SURFACE(((1.,1.,1.,1.,1.,1.,1.,1.,1.,1.,1.,1.,1.,1.,1.,
1.,1.,1.,1.,1.,1.,1.,1.),(0.776946963780595,0.776946963780595,0.776946963780595,
0.776946963780595,0.776946963780595,0.776946963780595,0.776946963780595,
0.776946963780595,0.776946963780595,0.776946963780595,0.776946963780596,
0.776946963780595,0.776946963780595,0.776946963780595,0.776946963780595,
0.776946963780595,0.776946963780595,0.776946963780595,0.776946963780595,
0.776946963780595,0.776946963780595,0.776946963780595,0.776946963780595),
(0.776946963780595,0.776946963780595,0.776946963780595,0.776946963780595,
0.776946963780595,0.776946963780595,0.776946963780595,0.776946963780595,
0.776946963780595,0.776946963780595,0.776946963780596,0.776946963780595,
0.776946963780595,0.776946963780595,0.776946963780595,0.776946963780595,
0.776946963780595,0.776946963780595,0.776946963780595,0.776946963780595,
0.776946963780595,0.776946963780595,0.776946963780595),(1.,1.,1.,1.,1.,
1.,1.,1.,1.,1.,1.,1.,1.,1.,1.,1.,1.,1.,1.,1.,1.,1.,1.)))
REPRESENTATION_ITEM('')
SURFACE()
);
#2497=(
BOUNDED_SURFACE()
B_SPLINE_SURFACE(3,3,((#134718,#134719,#134720,#134721,#134722,#134723),
(#134724,#134725,#134726,#134727,#134728,#134729),(#134730,#134731,#134732,
#134733,#134734,#134735),(#134736,#134737,#134738,#134739,#134740,#134741)),
 .UNSPECIFIED.,.F.,.F.,.F.)
B_SPLINE_SURFACE_WITH_KNOTS((4,4),(4,1,1,4),(0.,1.),(0.,0.291618855427959,
0.679839163052527,1.),.UNSPECIFIED.)
GEOMETRIC_REPRESENTATION_ITEM()
RATIONAL_B_SPLINE_SURFACE(((1.268105254047,1.268105254047,1.268105254047,
1.268105254047,1.268105254047,1.268105254047),(0.9106315819844,0.9106315819844,
0.9106315819844,0.9106315819844,0.9106315819844,0.9106315819844),(0.9106315819844,
0.9106315819844,0.9106315819844,0.9106315819844,0.9106315819844,0.9106315819844),
(1.268105254047,1.268105254047,1.268105254047,1.268105254047,1.268105254047,
1.268105254047)))
REPRESENTATION_ITEM('')
SURFACE()
);
#2498=(
BOUNDED_SURFACE()
B_SPLINE_SURFACE(3,3,((#134864,#134865,#134866,#134867,#134868,#134869,
#134870,#134871,#134872,#134873),(#134874,#134875,#134876,#134877,#134878,
#134879,#134880,#134881,#134882,#134883),(#134884,#134885,#134886,#134887,
#134888,#134889,#134890,#134891,#134892,#134893),(#134894,#134895,#134896,
#134897,#134898,#134899,#134900,#134901,#134902,#134903)),.UNSPECIFIED.,
 .F.,.F.,.F.)
B_SPLINE_SURFACE_WITH_KNOTS((4,4),(4,1,1,1,1,1,1,4),(0.,1.),(0.,0.0598844757860275,
0.21530560800185,0.388152655537293,0.569077055547832,0.736795344088362,
0.884453290136092,1.),.UNSPECIFIED.)
GEOMETRIC_REPRESENTATION_ITEM()
RATIONAL_B_SPLINE_SURFACE(((1.625548306272,1.625548306272,1.625548306272,
1.625548306272,1.625548306272,1.625548306272,1.625548306272,1.625548306272,
1.625548306272,1.625548306272),(0.7914838979093,0.7914838979093,0.7914838979093,
0.7914838979093,0.7914838979093,0.7914838979093,0.7914838979093,0.7914838979093,
0.7914838979093,0.7914838979093),(0.7914838979093,0.7914838979093,0.7914838979093,
0.7914838979093,0.7914838979093,0.7914838979093,0.7914838979093,0.7914838979093,
0.7914838979093,0.7914838979093),(1.625548306272,1.625548306272,1.625548306272,
1.625548306272,1.625548306272,1.625548306272,1.625548306272,1.625548306272,
1.625548306272,1.625548306272)))
REPRESENTATION_ITEM('')
SURFACE()
);
#2499=(
BOUNDED_SURFACE()
B_SPLINE_SURFACE(3,3,((#134994,#134995,#134996,#134997,#134998,#134999,
#135000,#135001,#135002,#135003),(#135004,#135005,#135006,#135007,#135008,
#135009,#135010,#135011,#135012,#135013),(#135014,#135015,#135016,#135017,
#135018,#135019,#135020,#135021,#135022,#135023),(#135024,#135025,#135026,
#135027,#135028,#135029,#135030,#135031,#135032,#135033)),.UNSPECIFIED.,
 .F.,.F.,.F.)
B_SPLINE_SURFACE_WITH_KNOTS((4,4),(4,1,1,1,1,1,1,4),(0.,1.),(0.,0.118544207568657,
0.266810022823391,0.435219131927487,0.616475909576636,0.78883439689268,
0.943447617027774,1.),.UNSPECIFIED.)
GEOMETRIC_REPRESENTATION_ITEM()
RATIONAL_B_SPLINE_SURFACE(((1.62577582512,1.62577582512,1.62577582512,1.62577582512,
1.62577582512,1.62577582512,1.62577582512,1.62577582512,1.62577582512,1.62577582512),
(0.7914080582935,0.7914080582935,0.7914080582935,0.7914080582935,0.7914080582935,
0.7914080582935,0.7914080582935,0.7914080582935,0.7914080582935,0.7914080582935),
(0.7914080582935,0.7914080582935,0.7914080582935,0.7914080582935,0.7914080582935,
0.7914080582935,0.7914080582935,0.7914080582935,0.7914080582935,0.7914080582935),
(1.62577582512,1.62577582512,1.62577582512,1.62577582512,1.62577582512,
1.62577582512,1.62577582512,1.62577582512,1.62577582512,1.62577582512)))
REPRESENTATION_ITEM('')
SURFACE()
);
#2500=(
BOUNDED_SURFACE()
B_SPLINE_SURFACE(3,3,((#135155,#135156,#135157,#135158,#135159,#135160,
#135161,#135162,#135163,#135164,#135165,#135166,#135167,#135168,#135169),
(#135170,#135171,#135172,#135173,#135174,#135175,#135176,#135177,#135178,
#135179,#135180,#135181,#135182,#135183,#135184),(#135185,#135186,#135187,
#135188,#135189,#135190,#135191,#135192,#135193,#135194,#135195,#135196,
#135197,#135198,#135199),(#135200,#135201,#135202,#135203,#135204,#135205,
#135206,#135207,#135208,#135209,#135210,#135211,#135212,#135213,#135214)),
 .UNSPECIFIED.,.F.,.F.,.F.)
B_SPLINE_SURFACE_WITH_KNOTS((4,4),(4,1,1,1,1,1,1,1,1,1,1,1,4),(0.,1.),(0.,
0.0167135648045114,0.156510702717728,0.290602098832967,0.41291935039186,
0.522243745128064,0.620141294857168,0.708532612403636,0.788779269412781,
0.861957662054057,0.928247897390154,0.98772116750503,1.),.UNSPECIFIED.)
GEOMETRIC_REPRESENTATION_ITEM()
RATIONAL_B_SPLINE_SURFACE(((1.289190114461,1.289190114461,1.289190114461,
1.289190114461,1.289190114461,1.289190114461,1.289190114461,1.289190114461,
1.289190114461,1.289190114461,1.289190114461,1.289190114461,1.289190114461,
1.289190114461,1.289190114461),(0.9036032951798,0.9036032951798,0.9036032951798,
0.9036032951798,0.9036032951798,0.9036032951798,0.9036032951798,0.9036032951798,
0.9036032951798,0.9036032951798,0.9036032951798,0.9036032951798,0.9036032951798,
0.9036032951798,0.9036032951798),(0.9036032951798,0.9036032951798,0.9036032951798,
0.9036032951798,0.9036032951798,0.9036032951798,0.9036032951798,0.9036032951798,
0.9036032951798,0.9036032951798,0.9036032951798,0.9036032951798,0.9036032951798,
0.9036032951798,0.9036032951798),(1.289190114461,1.289190114461,1.289190114461,
1.289190114461,1.289190114461,1.289190114461,1.289190114461,1.289190114461,
1.289190114461,1.289190114461,1.289190114461,1.289190114461,1.289190114461,
1.289190114461,1.289190114461)))
REPRESENTATION_ITEM('')
SURFACE()
);
#2501=(
BOUNDED_SURFACE()
B_SPLINE_SURFACE(3,3,((#135581,#135582,#135583,#135584,#135585,#135586),
(#135587,#135588,#135589,#135590,#135591,#135592),(#135593,#135594,#135595,
#135596,#135597,#135598),(#135599,#135600,#135601,#135602,#135603,#135604)),
 .UNSPECIFIED.,.F.,.F.,.F.)
B_SPLINE_SURFACE_WITH_KNOTS((4,4),(4,1,1,4),(0.,1.),(0.,0.235053155447178,
0.807846173326003,1.),.UNSPECIFIED.)
GEOMETRIC_REPRESENTATION_ITEM()
RATIONAL_B_SPLINE_SURFACE(((1.190144115645,1.190144115645,1.190144115645,
1.190144115645,1.190144115645,1.190144115645),(0.9366186281184,0.9366186281184,
0.9366186281184,0.9366186281184,0.9366186281184,0.9366186281184),(0.9366186281184,
0.9366186281184,0.9366186281184,0.9366186281184,0.9366186281184,0.9366186281184),
(1.190144115645,1.190144115645,1.190144115645,1.190144115645,1.190144115645,
1.190144115645)))
REPRESENTATION_ITEM('')
SURFACE()
);
#2502=(
BOUNDED_SURFACE()
B_SPLINE_SURFACE(3,3,((#135839,#135840,#135841,#135842,#135843,#135844,
#135845,#135846,#135847,#135848,#135849,#135850,#135851,#135852,#135853,
#135854),(#135855,#135856,#135857,#135858,#135859,#135860,#135861,#135862,
#135863,#135864,#135865,#135866,#135867,#135868,#135869,#135870),(#135871,
#135872,#135873,#135874,#135875,#135876,#135877,#135878,#135879,#135880,
#135881,#135882,#135883,#135884,#135885,#135886),(#135887,#135888,#135889,
#135890,#135891,#135892,#135893,#135894,#135895,#135896,#135897,#135898,
#135899,#135900,#135901,#135902),(#135903,#135904,#135905,#135906,#135907,
#135908,#135909,#135910,#135911,#135912,#135913,#135914,#135915,#135916,
#135917,#135918),(#135919,#135920,#135921,#135922,#135923,#135924,#135925,
#135926,#135927,#135928,#135929,#135930,#135931,#135932,#135933,#135934),
(#135935,#135936,#135937,#135938,#135939,#135940,#135941,#135942,#135943,
#135944,#135945,#135946,#135947,#135948,#135949,#135950)),.UNSPECIFIED.,
 .F.,.F.,.F.)
B_SPLINE_SURFACE_WITH_KNOTS((4,3,4),(4,1,1,1,1,1,1,1,1,1,1,1,1,4),(0.,0.5,
1.),(0.,0.0687092176565791,0.148436322486723,0.231002296681117,0.312631644850041,
0.390370677084989,0.463984704679376,0.535797779848878,0.609423921069924,
0.687272621576965,0.769077589534318,0.851644273887414,0.931363117848373,
1.),.UNSPECIFIED.)
GEOMETRIC_REPRESENTATION_ITEM()
RATIONAL_B_SPLINE_SURFACE(((1.308864936088,1.308864936088,1.308864936088,
1.308864936088,1.308864936088,1.308864936088,1.308864936088,1.308864936088,
1.308864936088,1.308864936088,1.308864936088,1.308864936088,1.308864936088,
1.308864936088,1.308864936088,1.308864936088),(0.8970450213041,0.8970450213041,
0.8970450213041,0.8970450213041,0.8970450213041,0.8970450213041,0.8970450213041,
0.8970450213041,0.8970450213041,0.8970450213041,0.8970450213041,0.8970450213041,
0.8970450213041,0.8970450213041,0.8970450213041,0.8970450213041),(0.8970450213041,
0.8970450213041,0.8970450213041,0.8970450213041,0.8970450213041,0.8970450213041,
0.8970450213041,0.8970450213041,0.8970450213041,0.8970450213041,0.8970450213041,
0.8970450213041,0.8970450213041,0.8970450213041,0.8970450213041,0.8970450213041),
(1.308864936088,1.308864936088,1.308864936088,1.308864936088,1.308864936088,
1.308864936088,1.308864936088,1.308864936088,1.308864936088,1.308864936088,
1.308864936088,1.308864936088,1.308864936088,1.308864936088,1.308864936088,
1.308864936088),(0.8970450213041,0.8970450213041,0.8970450213041,0.8970450213041,
0.8970450213041,0.8970450213041,0.8970450213041,0.8970450213041,0.8970450213041,
0.8970450213041,0.8970450213041,0.8970450213041,0.8970450213041,0.8970450213041,
0.8970450213041,0.8970450213041),(0.8970450213041,0.8970450213041,0.8970450213041,
0.8970450213041,0.8970450213041,0.8970450213041,0.8970450213041,0.8970450213041,
0.8970450213041,0.8970450213041,0.8970450213041,0.8970450213041,0.8970450213041,
0.8970450213041,0.8970450213041,0.8970450213041),(1.308864936088,1.308864936088,
1.308864936088,1.308864936088,1.308864936088,1.308864936088,1.308864936088,
1.308864936088,1.308864936088,1.308864936088,1.308864936088,1.308864936088,
1.308864936088,1.308864936088,1.308864936088,1.308864936088)))
REPRESENTATION_ITEM('')
SURFACE()
);
#2503=(
BOUNDED_SURFACE()
B_SPLINE_SURFACE(3,3,((#135952,#135953,#135954,#135955,#135956,#135957),
(#135958,#135959,#135960,#135961,#135962,#135963),(#135964,#135965,#135966,
#135967,#135968,#135969),(#135970,#135971,#135972,#135973,#135974,#135975)),
 .UNSPECIFIED.,.F.,.F.,.F.)
B_SPLINE_SURFACE_WITH_KNOTS((4,4),(4,1,1,4),(0.,1.),(0.,0.0809027375127101,
0.709349370148383,1.),.UNSPECIFIED.)
GEOMETRIC_REPRESENTATION_ITEM()
RATIONAL_B_SPLINE_SURFACE(((1.190145701779,1.190145701779,1.190145701779,
1.190145701779,1.190145701779,1.190145701779),(0.936618099407,0.936618099407,
0.936618099407,0.936618099407,0.936618099407,0.936618099407),(0.936618099407,
0.936618099407,0.936618099407,0.936618099407,0.936618099407,0.936618099407),
(1.190145701779,1.190145701779,1.190145701779,1.190145701779,1.190145701779,
1.190145701779)))
REPRESENTATION_ITEM('')
SURFACE()
);
#2504=(
BOUNDED_SURFACE()
B_SPLINE_SURFACE(3,3,((#135977,#135978,#135979,#135980,#135981,#135982),
(#135983,#135984,#135985,#135986,#135987,#135988),(#135989,#135990,#135991,
#135992,#135993,#135994),(#135995,#135996,#135997,#135998,#135999,#136000),
(#136001,#136002,#136003,#136004,#136005,#136006),(#136007,#136008,#136009,
#136010,#136011,#136012),(#136013,#136014,#136015,#136016,#136017,#136018)),
 .UNSPECIFIED.,.F.,.F.,.F.)
B_SPLINE_SURFACE_WITH_KNOTS((4,3,4),(4,1,1,4),(0.,0.5,1.),(0.,0.274607544356056,
0.733821408099398,1.),.UNSPECIFIED.)
GEOMETRIC_REPRESENTATION_ITEM()
RATIONAL_B_SPLINE_SURFACE(((1.232615246856,1.232615246856,1.232615246856,
1.232615246856,1.232615246856,1.232615246856),(0.9224615843814,0.9224615843814,
0.9224615843814,0.9224615843814,0.9224615843814,0.9224615843814),(0.9224615843814,
0.9224615843814,0.9224615843814,0.9224615843814,0.9224615843814,0.9224615843814),
(1.232615246856,1.232615246856,1.232615246856,1.232615246856,1.232615246856,
1.232615246856),(0.9224615843814,0.9224615843814,0.9224615843814,0.9224615843814,
0.9224615843814,0.9224615843814),(0.9224615843814,0.9224615843814,0.9224615843814,
0.9224615843814,0.9224615843814,0.9224615843814),(1.232615246856,1.232615246856,
1.232615246856,1.232615246856,1.232615246856,1.232615246856)))
REPRESENTATION_ITEM('')
SURFACE()
);
#2505=(
BOUNDED_SURFACE()
B_SPLINE_SURFACE(3,3,((#136020,#136021,#136022,#136023,#136024,#136025),
(#136026,#136027,#136028,#136029,#136030,#136031),(#136032,#136033,#136034,
#136035,#136036,#136037),(#136038,#136039,#136040,#136041,#136042,#136043)),
 .UNSPECIFIED.,.F.,.F.,.F.)
B_SPLINE_SURFACE_WITH_KNOTS((4,4),(4,1,1,4),(0.,1.),(0.,0.0915158091820991,
0.730870545365667,1.),.UNSPECIFIED.)
GEOMETRIC_REPRESENTATION_ITEM()
RATIONAL_B_SPLINE_SURFACE(((1.190145739571,1.190145739571,1.190145739571,
1.190145739571,1.190145739571,1.190145739571),(0.9366180868096,0.9366180868096,
0.9366180868096,0.9366180868096,0.9366180868096,0.9366180868096),(0.9366180868096,
0.9366180868096,0.9366180868096,0.9366180868096,0.9366180868096,0.9366180868096),
(1.190145739571,1.190145739571,1.190145739571,1.190145739571,1.190145739571,
1.190145739571)))
REPRESENTATION_ITEM('')
SURFACE()
);
#2506=(
BOUNDED_SURFACE()
B_SPLINE_SURFACE(3,3,((#136045,#136046,#136047,#136048,#136049,#136050,
#136051,#136052,#136053,#136054,#136055,#136056,#136057,#136058,#136059,
#136060),(#136061,#136062,#136063,#136064,#136065,#136066,#136067,#136068,
#136069,#136070,#136071,#136072,#136073,#136074,#136075,#136076),(#136077,
#136078,#136079,#136080,#136081,#136082,#136083,#136084,#136085,#136086,
#136087,#136088,#136089,#136090,#136091,#136092),(#136093,#136094,#136095,
#136096,#136097,#136098,#136099,#136100,#136101,#136102,#136103,#136104,
#136105,#136106,#136107,#136108),(#136109,#136110,#136111,#136112,#136113,
#136114,#136115,#136116,#136117,#136118,#136119,#136120,#136121,#136122,
#136123,#136124),(#136125,#136126,#136127,#136128,#136129,#136130,#136131,
#136132,#136133,#136134,#136135,#136136,#136137,#136138,#136139,#136140),
(#136141,#136142,#136143,#136144,#136145,#136146,#136147,#136148,#136149,
#136150,#136151,#136152,#136153,#136154,#136155,#136156)),.UNSPECIFIED.,
 .F.,.F.,.F.)
B_SPLINE_SURFACE_WITH_KNOTS((4,3,4),(4,1,1,1,1,1,1,1,1,1,1,1,1,4),(0.,0.5,
1.),(0.,0.0700282448367935,0.149591065260121,0.231957090335842,0.31326843643496,
0.39068316564619,0.464059946408323,0.535688017619035,0.609079764496469,
0.686617012874269,0.768115357612328,0.85048528028637,0.930041884500008,
1.),.UNSPECIFIED.)
GEOMETRIC_REPRESENTATION_ITEM()
RATIONAL_B_SPLINE_SURFACE(((1.308862041161,1.308862041161,1.308862041161,
1.308862041161,1.308862041161,1.308862041161,1.308862041161,1.308862041161,
1.308862041161,1.308862041161,1.308862041161,1.308862041161,1.308862041161,
1.308862041161,1.308862041161,1.308862041161),(0.8970459862798,0.8970459862798,
0.8970459862798,0.8970459862798,0.8970459862798,0.8970459862798,0.8970459862798,
0.8970459862798,0.8970459862798,0.8970459862798,0.8970459862798,0.8970459862798,
0.8970459862798,0.8970459862798,0.8970459862798,0.8970459862798),(0.8970459862798,
0.8970459862798,0.8970459862798,0.8970459862798,0.8970459862798,0.8970459862798,
0.8970459862798,0.8970459862798,0.8970459862798,0.8970459862798,0.8970459862798,
0.8970459862798,0.8970459862798,0.8970459862798,0.8970459862798,0.8970459862798),
(1.308862041161,1.308862041161,1.308862041161,1.308862041161,1.308862041161,
1.308862041161,1.308862041161,1.308862041161,1.308862041161,1.308862041161,
1.308862041161,1.308862041161,1.308862041161,1.308862041161,1.308862041161,
1.308862041161),(0.8970459862798,0.8970459862798,0.8970459862798,0.8970459862798,
0.8970459862798,0.8970459862798,0.8970459862798,0.8970459862798,0.8970459862798,
0.8970459862798,0.8970459862798,0.8970459862798,0.8970459862798,0.8970459862798,
0.8970459862798,0.8970459862798),(0.8970459862798,0.8970459862798,0.8970459862798,
0.8970459862798,0.8970459862798,0.8970459862798,0.8970459862798,0.8970459862798,
0.8970459862798,0.8970459862798,0.8970459862798,0.8970459862798,0.8970459862798,
0.8970459862798,0.8970459862798,0.8970459862798),(1.308862041161,1.308862041161,
1.308862041161,1.308862041161,1.308862041161,1.308862041161,1.308862041161,
1.308862041161,1.308862041161,1.308862041161,1.308862041161,1.308862041161,
1.308862041161,1.308862041161,1.308862041161,1.308862041161)))
REPRESENTATION_ITEM('')
SURFACE()
);
#2507=(
BOUNDED_SURFACE()
B_SPLINE_SURFACE(3,3,((#138377,#138378,#138379,#138380),(#138381,#138382,
#138383,#138384),(#138385,#138386,#138387,#138388),(#138389,#138390,#138391,
#138392)),.UNSPECIFIED.,.F.,.F.,.F.)
B_SPLINE_SURFACE_WITH_KNOTS((4,4),(4,4),(0.,1.),(0.,1.),.UNSPECIFIED.)
GEOMETRIC_REPRESENTATION_ITEM()
RATIONAL_B_SPLINE_SURFACE(((1.008822121122,0.8033151890331,0.8032831812337,
1.008726097724),(1.008912249556,0.8013058203417,0.8012734855446,1.008815245165),
(1.008912321853,0.8013042085275,0.8012718734681,1.008815316675),(1.008822107526,
0.8033154921495,0.8032834843994,1.008726084276)))
REPRESENTATION_ITEM('')
SURFACE()
);
#2508=(
BOUNDED_SURFACE()
B_SPLINE_SURFACE(3,3,((#139238,#139239,#139240,#139241,#139242,#139243,
#139244,#139245,#139246,#139247,#139248,#139249,#139250,#139251,#139252,
#139253,#139254,#139255,#139256,#139257,#139258,#139259,#139260,#139261,
#139262,#139263,#139264,#139265,#139266,#139267,#139268,#139269,#139270,
#139271,#139272,#139273,#139274,#139275,#139276,#139277,#139278,#139279,
#139280,#139281,#139282,#139283,#139284,#139285,#139286,#139287,#139288,
#139289,#139290,#139291,#139292,#139293,#139294),(#139295,#139296,#139297,
#139298,#139299,#139300,#139301,#139302,#139303,#139304,#139305,#139306,
#139307,#139308,#139309,#139310,#139311,#139312,#139313,#139314,#139315,
#139316,#139317,#139318,#139319,#139320,#139321,#139322,#139323,#139324,
#139325,#139326,#139327,#139328,#139329,#139330,#139331,#139332,#139333,
#139334,#139335,#139336,#139337,#139338,#139339,#139340,#139341,#139342,
#139343,#139344,#139345,#139346,#139347,#139348,#139349,#139350,#139351),
(#139352,#139353,#139354,#139355,#139356,#139357,#139358,#139359,#139360,
#139361,#139362,#139363,#139364,#139365,#139366,#139367,#139368,#139369,
#139370,#139371,#139372,#139373,#139374,#139375,#139376,#139377,#139378,
#139379,#139380,#139381,#139382,#139383,#139384,#139385,#139386,#139387,
#139388,#139389,#139390,#139391,#139392,#139393,#139394,#139395,#139396,
#139397,#139398,#139399,#139400,#139401,#139402,#139403,#139404,#139405,
#139406,#139407,#139408),(#139409,#139410,#139411,#139412,#139413,#139414,
#139415,#139416,#139417,#139418,#139419,#139420,#139421,#139422,#139423,
#139424,#139425,#139426,#139427,#139428,#139429,#139430,#139431,#139432,
#139433,#139434,#139435,#139436,#139437,#139438,#139439,#139440,#139441,
#139442,#139443,#139444,#139445,#139446,#139447,#139448,#139449,#139450,
#139451,#139452,#139453,#139454,#139455,#139456,#139457,#139458,#139459,
#139460,#139461,#139462,#139463,#139464,#139465)),.UNSPECIFIED.,.F.,.F.,
 .F.)
B_SPLINE_SURFACE_WITH_KNOTS((4,4),(4,1,1,1,1,1,1,1,1,1,1,1,1,1,1,1,1,1,
1,1,1,1,1,1,1,1,1,1,1,1,1,1,1,1,1,1,1,1,1,1,1,1,1,1,1,1,1,1,1,1,1,1,1,1,
4),(0.,1.),(0.,0.00436594588687658,0.0182600210166181,0.0336361494826213,
0.0506183732771892,0.0693310885947867,0.0898968700401271,0.112502721901119,
0.137670869409112,0.166010055644541,0.197488961679859,0.231803117837838,
0.269453903656424,0.310997004277211,0.356845197598653,0.407613486217267,
0.459741003658159,0.507079603017427,0.548859184651959,0.586033851963287,
0.619338629530692,0.649347424630681,0.676440228532917,0.701038763414989,
0.723416730015481,0.743823676714273,0.762471787524201,0.779541489745329,
0.795189394601638,0.809554049025702,0.822746458983589,0.834875103495141,
0.846051713912006,0.856380231241817,0.865896925803063,0.874602749195169,
0.88252206935229,0.889825047977363,0.896737634924824,0.903485575835366,
0.910246440119728,0.917100212565293,0.923938121747363,0.930419691089745,
0.936750575754955,0.94324323866504,0.949721357335021,0.955738934700183,
0.961744884998761,0.96808108564707,0.974379967180707,0.981030794925491,
0.98771333105686,0.994327233714889,1.),.UNSPECIFIED.)
GEOMETRIC_REPRESENTATION_ITEM()
RATIONAL_B_SPLINE_SURFACE(((1.753204797659,1.753204797659,1.753204797659,
1.753204797659,1.753204797659,1.753204797659,1.753204797659,1.753204797659,
1.753204797659,1.753204797659,1.753204797659,1.753204797659,1.753204797659,
1.753204797659,1.753204797659,1.753204797659,1.753204797659,1.753204797659,
1.753204797659,1.753204797659,1.753204797659,1.753204797659,1.753204797659,
1.753204797659,1.753204797659,1.753204797659,1.753204797659,1.753204797659,
1.753204797659,1.753204797659,1.753204797659,1.753204797659,1.753204797659,
1.753204797659,1.753204797659,1.753204797659,1.753204797659,1.753204797659,
1.753204797659,1.753204797659,1.753204797659,1.753204797659,1.753204797659,
1.753204797659,1.753204797659,1.753204797659,1.753204797659,1.753204797659,
1.753204797659,1.753204797659,1.753204797659,1.753204797659,1.753204797659,
1.753204797659,1.753204797659,1.753204797659,1.753204797659),(0.7489317341138,
0.7489317341138,0.7489317341138,0.7489317341138,0.7489317341138,0.7489317341138,
0.7489317341138,0.7489317341138,0.7489317341138,0.7489317341138,0.7489317341138,
0.7489317341138,0.7489317341138,0.7489317341138,0.7489317341138,0.7489317341138,
0.7489317341138,0.7489317341138,0.7489317341138,0.7489317341138,0.7489317341138,
0.7489317341138,0.7489317341138,0.7489317341138,0.7489317341138,0.7489317341138,
0.7489317341138,0.7489317341138,0.7489317341138,0.7489317341138,0.7489317341138,
0.7489317341138,0.7489317341138,0.7489317341138,0.7489317341138,0.7489317341138,
0.7489317341138,0.7489317341138,0.7489317341138,0.7489317341138,0.7489317341138,
0.7489317341138,0.7489317341138,0.7489317341138,0.7489317341138,0.7489317341138,
0.7489317341138,0.7489317341138,0.7489317341138,0.7489317341138,0.7489317341138,
0.7489317341138,0.7489317341138,0.7489317341138,0.7489317341138,0.7489317341138,
0.7489317341138),(0.7489317341138,0.7489317341138,0.7489317341138,0.7489317341138,
0.7489317341138,0.7489317341138,0.7489317341138,0.7489317341138,0.7489317341138,
0.7489317341138,0.7489317341138,0.7489317341138,0.7489317341138,0.7489317341138,
0.7489317341138,0.7489317341138,0.7489317341138,0.7489317341138,0.7489317341138,
0.7489317341138,0.7489317341138,0.7489317341138,0.7489317341138,0.7489317341138,
0.7489317341138,0.7489317341138,0.7489317341138,0.7489317341138,0.7489317341138,
0.7489317341138,0.7489317341138,0.7489317341138,0.7489317341138,0.7489317341138,
0.7489317341138,0.7489317341138,0.7489317341138,0.7489317341138,0.7489317341138,
0.7489317341138,0.7489317341138,0.7489317341138,0.7489317341138,0.7489317341138,
0.7489317341138,0.7489317341138,0.7489317341138,0.7489317341138,0.7489317341138,
0.7489317341138,0.7489317341138,0.7489317341138,0.7489317341138,0.7489317341138,
0.7489317341138,0.7489317341138,0.7489317341138),(1.753204797659,1.753204797659,
1.753204797659,1.753204797659,1.753204797659,1.753204797659,1.753204797659,
1.753204797659,1.753204797659,1.753204797659,1.753204797659,1.753204797659,
1.753204797659,1.753204797659,1.753204797659,1.753204797659,1.753204797659,
1.753204797659,1.753204797659,1.753204797659,1.753204797659,1.753204797659,
1.753204797659,1.753204797659,1.753204797659,1.753204797659,1.753204797659,
1.753204797659,1.753204797659,1.753204797659,1.753204797659,1.753204797659,
1.753204797659,1.753204797659,1.753204797659,1.753204797659,1.753204797659,
1.753204797659,1.753204797659,1.753204797659,1.753204797659,1.753204797659,
1.753204797659,1.753204797659,1.753204797659,1.753204797659,1.753204797659,
1.753204797659,1.753204797659,1.753204797659,1.753204797659,1.753204797659,
1.753204797659,1.753204797659,1.753204797659,1.753204797659,1.753204797659)))
REPRESENTATION_ITEM('')
SURFACE()
);
#2509=(
BOUNDED_SURFACE()
B_SPLINE_SURFACE(3,3,((#139981,#139982,#139983,#139984,#139985,#139986,
#139987,#139988,#139989,#139990,#139991,#139992,#139993,#139994,#139995,
#139996,#139997),(#139998,#139999,#140000,#140001,#140002,#140003,#140004,
#140005,#140006,#140007,#140008,#140009,#140010,#140011,#140012,#140013,
#140014),(#140015,#140016,#140017,#140018,#140019,#140020,#140021,#140022,
#140023,#140024,#140025,#140026,#140027,#140028,#140029,#140030,#140031),
(#140032,#140033,#140034,#140035,#140036,#140037,#140038,#140039,#140040,
#140041,#140042,#140043,#140044,#140045,#140046,#140047,#140048)),
 .UNSPECIFIED.,.F.,.F.,.F.)
B_SPLINE_SURFACE_WITH_KNOTS((4,4),(4,1,1,1,1,1,1,1,1,1,1,1,1,1,4),(0.,1.),
(0.,0.0309106984649458,0.0767351380515422,0.126422877856924,0.180395940015139,
0.239061834418011,0.302825261448321,0.372125224244129,0.447415877060644,
0.529151218103455,0.61776396940816,0.713738372609746,0.817824498173652,
0.93084881910144,1.),.UNSPECIFIED.)
GEOMETRIC_REPRESENTATION_ITEM()
RATIONAL_B_SPLINE_SURFACE(((1.477765587143,1.477765587143,1.477765587143,
1.477765587143,1.477765587143,1.477765587143,1.477765587143,1.477765587143,
1.477765587143,1.477765587143,1.477765587143,1.477765587143,1.477765587143,
1.477765587143,1.477765587143,1.477765587143,1.477765587143),(0.8407448042857,
0.8407448042857,0.8407448042857,0.8407448042857,0.8407448042857,0.8407448042857,
0.8407448042857,0.8407448042857,0.8407448042857,0.8407448042857,0.8407448042857,
0.8407448042857,0.8407448042857,0.8407448042857,0.8407448042857,0.8407448042857,
0.8407448042857),(0.8407448042857,0.8407448042857,0.8407448042857,0.8407448042857,
0.8407448042857,0.8407448042857,0.8407448042857,0.8407448042857,0.8407448042857,
0.8407448042857,0.8407448042857,0.8407448042857,0.8407448042857,0.8407448042857,
0.8407448042857,0.8407448042857,0.8407448042857),(1.477765587143,1.477765587143,
1.477765587143,1.477765587143,1.477765587143,1.477765587143,1.477765587143,
1.477765587143,1.477765587143,1.477765587143,1.477765587143,1.477765587143,
1.477765587143,1.477765587143,1.477765587143,1.477765587143,1.477765587143)))
REPRESENTATION_ITEM('')
SURFACE()
);
#2510=(
BOUNDED_SURFACE()
B_SPLINE_SURFACE(3,3,((#140136,#140137,#140138,#140139,#140140,#140141,
#140142,#140143,#140144,#140145),(#140146,#140147,#140148,#140149,#140150,
#140151,#140152,#140153,#140154,#140155),(#140156,#140157,#140158,#140159,
#140160,#140161,#140162,#140163,#140164,#140165),(#140166,#140167,#140168,
#140169,#140170,#140171,#140172,#140173,#140174,#140175)),.UNSPECIFIED.,
 .F.,.F.,.F.)
B_SPLINE_SURFACE_WITH_KNOTS((4,4),(4,1,1,1,1,1,1,4),(0.,1.),(0.,0.128230369083995,
0.280285083819611,0.448824676206344,0.626406055676366,0.804550055721658,
0.977970892840894,1.),.UNSPECIFIED.)
GEOMETRIC_REPRESENTATION_ITEM()
RATIONAL_B_SPLINE_SURFACE(((1.391693969077,1.391693969077,1.391693969077,
1.391693969077,1.391693969077,1.391693969077,1.391693969077,1.391693969077,
1.391693969077,1.391693969077),(0.8694353436408,0.8694353436408,0.8694353436408,
0.8694353436408,0.8694353436408,0.8694353436408,0.8694353436408,0.8694353436408,
0.8694353436408,0.8694353436408),(0.8694353436408,0.8694353436408,0.8694353436408,
0.8694353436408,0.8694353436408,0.8694353436408,0.8694353436408,0.8694353436408,
0.8694353436408,0.8694353436408),(1.391693969077,1.391693969077,1.391693969077,
1.391693969077,1.391693969077,1.391693969077,1.391693969077,1.391693969077,
1.391693969077,1.391693969077)))
REPRESENTATION_ITEM('')
SURFACE()
);
#2511=(
BOUNDED_SURFACE()
B_SPLINE_SURFACE(3,3,((#140424,#140425,#140426,#140427),(#140428,#140429,
#140430,#140431),(#140432,#140433,#140434,#140435),(#140436,#140437,#140438,
#140439)),.UNSPECIFIED.,.F.,.F.,.F.)
B_SPLINE_SURFACE_WITH_KNOTS((4,4),(4,4),(0.,1.),(0.,1.),.UNSPECIFIED.)
GEOMETRIC_REPRESENTATION_ITEM()
RATIONAL_B_SPLINE_SURFACE(((1.292957414843,1.292957414843,1.292957414843,
1.292957414843),(0.9023475283856,0.9023475283856,0.9023475283856,0.9023475283856),
(0.9023475283856,0.9023475283856,0.9023475283856,0.9023475283856),(1.292957414843,
1.292957414843,1.292957414843,1.292957414843)))
REPRESENTATION_ITEM('')
SURFACE()
);
#2512=(
BOUNDED_SURFACE()
B_SPLINE_SURFACE(3,3,((#140565,#140566,#140567,#140568,#140569,#140570,
#140571),(#140572,#140573,#140574,#140575,#140576,#140577,#140578),(#140579,
#140580,#140581,#140582,#140583,#140584,#140585),(#140586,#140587,#140588,
#140589,#140590,#140591,#140592)),.UNSPECIFIED.,.F.,.F.,.F.)
B_SPLINE_SURFACE_WITH_KNOTS((4,4),(4,1,1,1,4),(0.,1.),(0.,0.222752526718504,
0.482252641961039,0.73941984056398,1.),.UNSPECIFIED.)
GEOMETRIC_REPRESENTATION_ITEM()
RATIONAL_B_SPLINE_SURFACE(((1.400806786583,1.400806786583,1.400806786583,
1.400806786583,1.400806786583,1.400806786583,1.400806786583),(0.8663977378056,
0.8663977378056,0.8663977378056,0.8663977378056,0.8663977378056,0.8663977378056,
0.8663977378056),(0.8663977378056,0.8663977378056,0.8663977378056,0.8663977378056,
0.8663977378056,0.8663977378056,0.8663977378056),(1.400806786583,1.400806786583,
1.400806786583,1.400806786583,1.400806786583,1.400806786583,1.400806786583)))
REPRESENTATION_ITEM('')
SURFACE()
);
#2513=(
BOUNDED_SURFACE()
B_SPLINE_SURFACE(3,3,((#141054,#141055,#141056,#141057,#141058,#141059,
#141060,#141061,#141062,#141063),(#141064,#141065,#141066,#141067,#141068,
#141069,#141070,#141071,#141072,#141073),(#141074,#141075,#141076,#141077,
#141078,#141079,#141080,#141081,#141082,#141083),(#141084,#141085,#141086,
#141087,#141088,#141089,#141090,#141091,#141092,#141093)),.UNSPECIFIED.,
 .F.,.F.,.F.)
B_SPLINE_SURFACE_WITH_KNOTS((4,4),(4,1,1,1,1,1,1,4),(0.,1.),(0.,0.0210781168668079,
0.19449715108835,0.372688328304436,0.550339588756535,0.718994260976883,
0.87136168298915,1.),.UNSPECIFIED.)
GEOMETRIC_REPRESENTATION_ITEM()
RATIONAL_B_SPLINE_SURFACE(((1.391693714632,1.391693714632,1.391693714632,
1.391693714632,1.391693714632,1.391693714632,1.391693714632,1.391693714632,
1.391693714632,1.391693714632),(0.8694354284561,0.8694354284561,0.8694354284561,
0.8694354284561,0.8694354284561,0.8694354284561,0.8694354284561,0.8694354284561,
0.8694354284561,0.8694354284561),(0.8694354284561,0.8694354284561,0.8694354284561,
0.8694354284561,0.8694354284561,0.8694354284561,0.8694354284561,0.8694354284561,
0.8694354284561,0.8694354284561),(1.391693714632,1.391693714632,1.391693714632,
1.391693714632,1.391693714632,1.391693714632,1.391693714632,1.391693714632,
1.391693714632,1.391693714632)))
REPRESENTATION_ITEM('')
SURFACE()
);
#2514=(
BOUNDED_SURFACE()
B_SPLINE_SURFACE(3,3,((#141536,#141537,#141538,#141539,#141540,#141541,
#141542,#141543,#141544,#141545,#141546,#141547,#141548,#141549,#141550,
#141551,#141552),(#141553,#141554,#141555,#141556,#141557,#141558,#141559,
#141560,#141561,#141562,#141563,#141564,#141565,#141566,#141567,#141568,
#141569),(#141570,#141571,#141572,#141573,#141574,#141575,#141576,#141577,
#141578,#141579,#141580,#141581,#141582,#141583,#141584,#141585,#141586),
(#141587,#141588,#141589,#141590,#141591,#141592,#141593,#141594,#141595,
#141596,#141597,#141598,#141599,#141600,#141601,#141602,#141603)),
 .UNSPECIFIED.,.F.,.F.,.F.)
B_SPLINE_SURFACE_WITH_KNOTS((4,4),(4,1,1,1,1,1,1,1,1,1,1,1,1,1,4),(0.,1.),
(0.,0.069890317865961,0.183519863377166,0.288095357886999,0.384463811683335,
0.473385027678461,0.555345635364338,0.630785683183373,0.700166793190766,
0.763949567937318,0.82257831309593,0.876462900672047,0.926018168114661,
0.971673401817449,1.),.UNSPECIFIED.)
GEOMETRIC_REPRESENTATION_ITEM()
RATIONAL_B_SPLINE_SURFACE(((1.47776666642,1.47776666642,1.47776666642,1.47776666642,
1.47776666642,1.47776666642,1.47776666642,1.47776666642,1.47776666642,1.47776666642,
1.47776666642,1.47776666642,1.47776666642,1.47776666642,1.47776666642,1.47776666642,
1.47776666642),(0.8407444445268,0.8407444445268,0.8407444445268,0.8407444445268,
0.8407444445268,0.8407444445268,0.8407444445268,0.8407444445268,0.8407444445268,
0.8407444445268,0.8407444445268,0.8407444445268,0.8407444445268,0.8407444445268,
0.8407444445268,0.8407444445268,0.8407444445268),(0.8407444445268,0.8407444445268,
0.8407444445268,0.8407444445268,0.8407444445268,0.8407444445268,0.8407444445268,
0.8407444445268,0.8407444445268,0.8407444445268,0.8407444445268,0.8407444445268,
0.8407444445268,0.8407444445268,0.8407444445268,0.8407444445268,0.8407444445268),
(1.47776666642,1.47776666642,1.47776666642,1.47776666642,1.47776666642,
1.47776666642,1.47776666642,1.47776666642,1.47776666642,1.47776666642,1.47776666642,
1.47776666642,1.47776666642,1.47776666642,1.47776666642,1.47776666642,1.47776666642)))
REPRESENTATION_ITEM('')
SURFACE()
);
#2515=(
BOUNDED_SURFACE()
B_SPLINE_SURFACE(3,3,((#141677,#141678,#141679,#141680,#141681,#141682,
#141683,#141684,#141685,#141686,#141687,#141688,#141689,#141690,#141691,
#141692,#141693,#141694,#141695,#141696,#141697,#141698,#141699,#141700,
#141701,#141702,#141703,#141704,#141705,#141706,#141707,#141708,#141709,
#141710,#141711,#141712,#141713,#141714,#141715,#141716,#141717,#141718,
#141719,#141720,#141721,#141722,#141723,#141724,#141725,#141726,#141727,
#141728,#141729,#141730,#141731,#141732,#141733),(#141734,#141735,#141736,
#141737,#141738,#141739,#141740,#141741,#141742,#141743,#141744,#141745,
#141746,#141747,#141748,#141749,#141750,#141751,#141752,#141753,#141754,
#141755,#141756,#141757,#141758,#141759,#141760,#141761,#141762,#141763,
#141764,#141765,#141766,#141767,#141768,#141769,#141770,#141771,#141772,
#141773,#141774,#141775,#141776,#141777,#141778,#141779,#141780,#141781,
#141782,#141783,#141784,#141785,#141786,#141787,#141788,#141789,#141790),
(#141791,#141792,#141793,#141794,#141795,#141796,#141797,#141798,#141799,
#141800,#141801,#141802,#141803,#141804,#141805,#141806,#141807,#141808,
#141809,#141810,#141811,#141812,#141813,#141814,#141815,#141816,#141817,
#141818,#141819,#141820,#141821,#141822,#141823,#141824,#141825,#141826,
#141827,#141828,#141829,#141830,#141831,#141832,#141833,#141834,#141835,
#141836,#141837,#141838,#141839,#141840,#141841,#141842,#141843,#141844,
#141845,#141846,#141847),(#141848,#141849,#141850,#141851,#141852,#141853,
#141854,#141855,#141856,#141857,#141858,#141859,#141860,#141861,#141862,
#141863,#141864,#141865,#141866,#141867,#141868,#141869,#141870,#141871,
#141872,#141873,#141874,#141875,#141876,#141877,#141878,#141879,#141880,
#141881,#141882,#141883,#141884,#141885,#141886,#141887,#141888,#141889,
#141890,#141891,#141892,#141893,#141894,#141895,#141896,#141897,#141898,
#141899,#141900,#141901,#141902,#141903,#141904)),.UNSPECIFIED.,.F.,.F.,
 .F.)
B_SPLINE_SURFACE_WITH_KNOTS((4,4),(4,1,1,1,1,1,1,1,1,1,1,1,1,1,1,1,1,1,
1,1,1,1,1,1,1,1,1,1,1,1,1,1,1,1,1,1,1,1,1,1,1,1,1,1,1,1,1,1,1,1,1,1,1,1,
4),(0.,1.),(0.,0.00102850105811001,0.00759318438410793,0.0139342463721671,
0.0202721319015908,0.0267573495732106,0.0334153340449433,0.0399168198355134,
0.045663172318244,0.0517104759733391,0.0580362016986109,0.0643601149605132,
0.0709346866883761,0.078010969765109,0.0857264910323804,0.0941395929016807,
0.103307185168012,0.113276381440939,0.124079872938569,0.135753629220017,
0.148375964850575,0.162042755872641,0.176849244103508,0.192893057298682,
0.210287271282822,0.229156444467865,0.249639202539587,0.271887793018783,
0.296073149179171,0.322391880247146,0.351041060424109,0.382305717422001,
0.416405241220516,0.453678246748928,0.494467807818825,0.539245592433777,
0.5885590237456,0.638055262903253,0.681623741762806,0.720070723334701,0.754284171425329,
0.784974928394346,0.812861516420407,0.838339911838843,0.861378440096615,
0.882356404231104,0.901543934509106,0.919072351149281,0.935063242320242,
0.949632381127728,0.962891435925974,0.974950552369462,0.985929151039583,
0.995930274056731,1.),.UNSPECIFIED.)
GEOMETRIC_REPRESENTATION_ITEM()
RATIONAL_B_SPLINE_SURFACE(((1.753204347239,1.753204347239,1.753204347239,
1.753204347239,1.753204347239,1.753204347239,1.753204347239,1.753204347239,
1.753204347239,1.753204347239,1.753204347239,1.753204347239,1.753204347239,
1.753204347239,1.753204347239,1.753204347239,1.753204347239,1.753204347239,
1.753204347239,1.753204347239,1.753204347239,1.753204347239,1.753204347239,
1.753204347239,1.753204347239,1.753204347239,1.753204347239,1.753204347239,
1.753204347239,1.753204347239,1.753204347239,1.753204347239,1.753204347239,
1.753204347239,1.753204347239,1.753204347239,1.753204347239,1.753204347239,
1.753204347239,1.753204347239,1.753204347239,1.753204347239,1.753204347239,
1.753204347239,1.753204347239,1.753204347239,1.753204347239,1.753204347239,
1.753204347239,1.753204347239,1.753204347239,1.753204347239,1.753204347239,
1.753204347239,1.753204347239,1.753204347239,1.753204347239),(0.7489318842535,
0.7489318842535,0.7489318842535,0.7489318842535,0.7489318842535,0.7489318842535,
0.7489318842535,0.7489318842535,0.7489318842535,0.7489318842535,0.7489318842535,
0.7489318842535,0.7489318842535,0.7489318842535,0.7489318842535,0.7489318842535,
0.7489318842535,0.7489318842535,0.7489318842535,0.7489318842535,0.7489318842535,
0.7489318842535,0.7489318842535,0.7489318842535,0.7489318842535,0.7489318842535,
0.7489318842535,0.7489318842535,0.7489318842535,0.7489318842535,0.7489318842535,
0.7489318842535,0.7489318842535,0.7489318842535,0.7489318842535,0.7489318842535,
0.7489318842535,0.7489318842535,0.7489318842535,0.7489318842535,0.7489318842535,
0.7489318842535,0.7489318842535,0.7489318842535,0.7489318842535,0.7489318842535,
0.7489318842535,0.7489318842535,0.7489318842535,0.7489318842535,0.7489318842535,
0.7489318842535,0.7489318842535,0.7489318842535,0.7489318842535,0.7489318842535,
0.7489318842535),(0.7489318842535,0.7489318842535,0.7489318842535,0.7489318842535,
0.7489318842535,0.7489318842535,0.7489318842535,0.7489318842535,0.7489318842535,
0.7489318842535,0.7489318842535,0.7489318842535,0.7489318842535,0.7489318842535,
0.7489318842535,0.7489318842535,0.7489318842535,0.7489318842535,0.7489318842535,
0.7489318842535,0.7489318842535,0.7489318842535,0.7489318842535,0.7489318842535,
0.7489318842535,0.7489318842535,0.7489318842535,0.7489318842535,0.7489318842535,
0.7489318842535,0.7489318842535,0.7489318842535,0.7489318842535,0.7489318842535,
0.7489318842535,0.7489318842535,0.7489318842535,0.7489318842535,0.7489318842535,
0.7489318842535,0.7489318842535,0.7489318842535,0.7489318842535,0.7489318842535,
0.7489318842535,0.7489318842535,0.7489318842535,0.7489318842535,0.7489318842535,
0.7489318842535,0.7489318842535,0.7489318842535,0.7489318842535,0.7489318842535,
0.7489318842535,0.7489318842535,0.7489318842535),(1.753204347239,1.753204347239,
1.753204347239,1.753204347239,1.753204347239,1.753204347239,1.753204347239,
1.753204347239,1.753204347239,1.753204347239,1.753204347239,1.753204347239,
1.753204347239,1.753204347239,1.753204347239,1.753204347239,1.753204347239,
1.753204347239,1.753204347239,1.753204347239,1.753204347239,1.753204347239,
1.753204347239,1.753204347239,1.753204347239,1.753204347239,1.753204347239,
1.753204347239,1.753204347239,1.753204347239,1.753204347239,1.753204347239,
1.753204347239,1.753204347239,1.753204347239,1.753204347239,1.753204347239,
1.753204347239,1.753204347239,1.753204347239,1.753204347239,1.753204347239,
1.753204347239,1.753204347239,1.753204347239,1.753204347239,1.753204347239,
1.753204347239,1.753204347239,1.753204347239,1.753204347239,1.753204347239,
1.753204347239,1.753204347239,1.753204347239,1.753204347239,1.753204347239)))
REPRESENTATION_ITEM('')
SURFACE()
);
#2516=(
BOUNDED_SURFACE()
B_SPLINE_SURFACE(3,3,((#143029,#143030,#143031,#143032,#143033,#143034),
(#143035,#143036,#143037,#143038,#143039,#143040),(#143041,#143042,#143043,
#143044,#143045,#143046),(#143047,#143048,#143049,#143050,#143051,#143052)),
 .UNSPECIFIED.,.F.,.F.,.F.)
B_SPLINE_SURFACE_WITH_KNOTS((4,4),(4,1,1,4),(0.,1.),(0.,0.431751876033485,
0.936198433808859,1.),.UNSPECIFIED.)
GEOMETRIC_REPRESENTATION_ITEM()
RATIONAL_B_SPLINE_SURFACE(((1.289342975298,1.289342975298,1.289342975298,
1.289342975298,1.289342975298,1.289342975298),(0.9035523415674,0.9035523415674,
0.9035523415674,0.9035523415674,0.9035523415674,0.9035523415674),(0.9035523415674,
0.9035523415674,0.9035523415674,0.9035523415674,0.9035523415674,0.9035523415674),
(1.289342975298,1.289342975298,1.289342975298,1.289342975298,1.289342975298,
1.289342975298)))
REPRESENTATION_ITEM('')
SURFACE()
);
#2517=(
BOUNDED_SURFACE()
B_SPLINE_SURFACE(3,3,((#143070,#143071,#143072,#143073,#143074,#143075,
#143076,#143077,#143078,#143079),(#143080,#143081,#143082,#143083,#143084,
#143085,#143086,#143087,#143088,#143089),(#143090,#143091,#143092,#143093,
#143094,#143095,#143096,#143097,#143098,#143099),(#143100,#143101,#143102,
#143103,#143104,#143105,#143106,#143107,#143108,#143109)),.UNSPECIFIED.,
 .F.,.F.,.F.)
B_SPLINE_SURFACE_WITH_KNOTS((4,4),(4,1,1,1,1,1,1,4),(0.,1.),(0.,0.0532774375645769,
0.208329877010428,0.378436697484889,0.575701395918878,0.790211251619391,
0.990473980866038,1.),.UNSPECIFIED.)
GEOMETRIC_REPRESENTATION_ITEM()
RATIONAL_B_SPLINE_SURFACE(((1.478656999093,1.478656999093,1.478656999093,
1.478656999093,1.478656999093,1.478656999093,1.478656999093,1.478656999093,
1.478656999093,1.478656999093),(0.8404476669691,0.8404476669691,0.8404476669691,
0.8404476669691,0.8404476669691,0.8404476669691,0.8404476669691,0.8404476669691,
0.8404476669691,0.8404476669691),(0.8404476669691,0.8404476669691,0.8404476669691,
0.8404476669691,0.8404476669691,0.8404476669691,0.8404476669691,0.8404476669691,
0.8404476669691,0.8404476669691),(1.478656999093,1.478656999093,1.478656999093,
1.478656999093,1.478656999093,1.478656999093,1.478656999093,1.478656999093,
1.478656999093,1.478656999093)))
REPRESENTATION_ITEM('')
SURFACE()
);
#2518=(
BOUNDED_SURFACE()
B_SPLINE_SURFACE(3,3,((#143313,#143314,#143315,#143316,#143317,#143318,
#143319,#143320,#143321,#143322),(#143323,#143324,#143325,#143326,#143327,
#143328,#143329,#143330,#143331,#143332),(#143333,#143334,#143335,#143336,
#143337,#143338,#143339,#143340,#143341,#143342),(#143343,#143344,#143345,
#143346,#143347,#143348,#143349,#143350,#143351,#143352)),.UNSPECIFIED.,
 .F.,.F.,.F.)
B_SPLINE_SURFACE_WITH_KNOTS((4,4),(4,1,1,1,1,1,1,4),(0.,1.),(0.,0.0779252083993214,
0.243678133170507,0.415917299399803,0.596243537777757,0.781438784892872,
0.967855482654964,1.),.UNSPECIFIED.)
GEOMETRIC_REPRESENTATION_ITEM()
RATIONAL_B_SPLINE_SURFACE(((1.474156190063,1.474156190063,1.474156190063,
1.474156190063,1.474156190063,1.474156190063,1.474156190063,1.474156190063,
1.474156190063,1.474156190063),(0.8419479366457,0.8419479366457,0.8419479366457,
0.8419479366457,0.8419479366457,0.8419479366457,0.8419479366457,0.8419479366457,
0.8419479366457,0.8419479366457),(0.8419479366457,0.8419479366457,0.8419479366457,
0.8419479366457,0.8419479366457,0.8419479366457,0.8419479366457,0.8419479366457,
0.8419479366457,0.8419479366457),(1.474156190063,1.474156190063,1.474156190063,
1.474156190063,1.474156190063,1.474156190063,1.474156190063,1.474156190063,
1.474156190063,1.474156190063)))
REPRESENTATION_ITEM('')
SURFACE()
);
#2519=(
BOUNDED_SURFACE()
B_SPLINE_SURFACE(3,3,((#143483,#143484,#143485,#143486,#143487,#143488,
#143489,#143490,#143491,#143492),(#143493,#143494,#143495,#143496,#143497,
#143498,#143499,#143500,#143501,#143502),(#143503,#143504,#143505,#143506,
#143507,#143508,#143509,#143510,#143511,#143512),(#143513,#143514,#143515,
#143516,#143517,#143518,#143519,#143520,#143521,#143522)),.UNSPECIFIED.,
 .F.,.F.,.F.)
B_SPLINE_SURFACE_WITH_KNOTS((4,4),(4,1,1,1,1,1,1,4),(0.,1.),(0.,0.0147775451285446,
0.185822509142439,0.356344875612291,0.525759183537156,0.694014694357844,
0.861570783923705,1.),.UNSPECIFIED.)
GEOMETRIC_REPRESENTATION_ITEM()
RATIONAL_B_SPLINE_SURFACE(((1.474127146691,1.474127146691,1.474127146691,
1.474127146691,1.474127146691,1.474127146691,1.474127146691,1.474127146691,
1.474127146691,1.474127146691),(0.8419576177696,0.8419576177696,0.8419576177696,
0.8419576177696,0.8419576177696,0.8419576177696,0.8419576177696,0.8419576177696,
0.8419576177696,0.8419576177696),(0.8419576177696,0.8419576177696,0.8419576177696,
0.8419576177696,0.8419576177696,0.8419576177696,0.8419576177696,0.8419576177696,
0.8419576177696,0.8419576177696),(1.474127146691,1.474127146691,1.474127146691,
1.474127146691,1.474127146691,1.474127146691,1.474127146691,1.474127146691,
1.474127146691,1.474127146691)))
REPRESENTATION_ITEM('')
SURFACE()
);
#2520=(
BOUNDED_SURFACE()
B_SPLINE_SURFACE(3,3,((#143587,#143588,#143589,#143590,#143591,#143592,
#143593,#143594,#143595),(#143596,#143597,#143598,#143599,#143600,#143601,
#143602,#143603,#143604),(#143605,#143606,#143607,#143608,#143609,#143610,
#143611,#143612,#143613),(#143614,#143615,#143616,#143617,#143618,#143619,
#143620,#143621,#143622)),.UNSPECIFIED.,.F.,.F.,.F.)
B_SPLINE_SURFACE_WITH_KNOTS((4,4),(4,1,1,1,1,1,4),(0.,1.),(0.,0.125272810862783,
0.299863569490546,0.48106636157826,0.670112397030726,0.863600947542818,
1.),.UNSPECIFIED.)
GEOMETRIC_REPRESENTATION_ITEM()
RATIONAL_B_SPLINE_SURFACE(((1.30708297461,1.30708297461,1.30708297461,1.30708297461,
1.30708297461,1.30708297461,1.30708297461,1.30708297461,1.30708297461),
(0.8976390084633,0.8976390084633,0.8976390084633,0.8976390084633,0.8976390084633,
0.8976390084633,0.8976390084633,0.8976390084633,0.8976390084633),(0.8976390084633,
0.8976390084633,0.8976390084633,0.8976390084633,0.8976390084633,0.8976390084633,
0.8976390084633,0.8976390084633,0.8976390084633),(1.30708297461,1.30708297461,
1.30708297461,1.30708297461,1.30708297461,1.30708297461,1.30708297461,1.30708297461,
1.30708297461)))
REPRESENTATION_ITEM('')
SURFACE()
);
#2521=(
BOUNDED_SURFACE()
B_SPLINE_SURFACE(3,3,((#143655,#143656,#143657,#143658,#143659,#143660,
#143661,#143662),(#143663,#143664,#143665,#143666,#143667,#143668,#143669,
#143670),(#143671,#143672,#143673,#143674,#143675,#143676,#143677,#143678),
(#143679,#143680,#143681,#143682,#143683,#143684,#143685,#143686)),
 .UNSPECIFIED.,.F.,.F.,.F.)
B_SPLINE_SURFACE_WITH_KNOTS((4,4),(4,1,1,1,1,4),(0.,1.),(0.,0.0104550154603523,
0.283607455569876,0.586586557478444,0.907836751474964,1.),.UNSPECIFIED.)
GEOMETRIC_REPRESENTATION_ITEM()
RATIONAL_B_SPLINE_SURFACE(((1.053280938608,1.053280938608,1.053280938608,
1.053280938608,1.053280938608,1.053280938608,1.053280938608,1.053280938608),
(0.9822396871305,0.9822396871305,0.9822396871305,0.9822396871305,0.9822396871305,
0.9822396871305,0.9822396871305,0.9822396871305),(0.9822396871305,0.9822396871305,
0.9822396871305,0.9822396871305,0.9822396871305,0.9822396871305,0.9822396871305,
0.9822396871305),(1.053280938608,1.053280938608,1.053280938608,1.053280938608,
1.053280938608,1.053280938608,1.053280938608,1.053280938608)))
REPRESENTATION_ITEM('')
SURFACE()
);
#2522=(
BOUNDED_SURFACE()
B_SPLINE_SURFACE(3,3,((#143709,#143710,#143711,#143712,#143713,#143714,
#143715,#143716,#143717),(#143718,#143719,#143720,#143721,#143722,#143723,
#143724,#143725,#143726),(#143727,#143728,#143729,#143730,#143731,#143732,
#143733,#143734,#143735),(#143736,#143737,#143738,#143739,#143740,#143741,
#143742,#143743,#143744)),.UNSPECIFIED.,.F.,.F.,.F.)
B_SPLINE_SURFACE_WITH_KNOTS((4,4),(4,1,1,1,1,1,4),(0.,1.),(0.,0.142766734134771,
0.334374398032124,0.521585124423469,0.701026212149163,0.873921879053949,
1.),.UNSPECIFIED.)
GEOMETRIC_REPRESENTATION_ITEM()
RATIONAL_B_SPLINE_SURFACE(((1.307082945987,1.307082945987,1.307082945987,
1.307082945987,1.307082945987,1.307082945987,1.307082945987,1.307082945987,
1.307082945987),(0.8976390180043,0.8976390180043,0.8976390180043,0.8976390180043,
0.8976390180043,0.8976390180043,0.8976390180043,0.8976390180043,0.8976390180043),
(0.8976390180043,0.8976390180043,0.8976390180043,0.8976390180043,0.8976390180043,
0.8976390180043,0.8976390180043,0.8976390180043,0.8976390180043),(1.307082945987,
1.307082945987,1.307082945987,1.307082945987,1.307082945987,1.307082945987,
1.307082945987,1.307082945987,1.307082945987)))
REPRESENTATION_ITEM('')
SURFACE()
);
#2523=(
BOUNDED_SURFACE()
B_SPLINE_SURFACE(3,3,((#143751,#143752,#143753,#143754,#143755,#143756,
#143757,#143758,#143759,#143760),(#143761,#143762,#143763,#143764,#143765,
#143766,#143767,#143768,#143769,#143770),(#143771,#143772,#143773,#143774,
#143775,#143776,#143777,#143778,#143779,#143780),(#143781,#143782,#143783,
#143784,#143785,#143786,#143787,#143788,#143789,#143790)),.UNSPECIFIED.,
 .F.,.F.,.F.)
B_SPLINE_SURFACE_WITH_KNOTS((4,4),(4,1,1,1,1,1,1,4),(0.,1.),(0.,0.140512983352509,
0.308388853051919,0.476969773176465,0.646706159656357,0.81755755850554,
0.988926783135651,1.),.UNSPECIFIED.)
GEOMETRIC_REPRESENTATION_ITEM()
RATIONAL_B_SPLINE_SURFACE(((1.474127154187,1.474127154187,1.474127154187,
1.474127154187,1.474127154187,1.474127154187,1.474127154187,1.474127154187,
1.474127154187,1.474127154187),(0.8419576152711,0.8419576152711,0.8419576152711,
0.8419576152711,0.8419576152711,0.8419576152711,0.8419576152711,0.8419576152711,
0.8419576152711,0.8419576152711),(0.8419576152711,0.8419576152711,0.8419576152711,
0.8419576152711,0.8419576152711,0.8419576152711,0.8419576152711,0.8419576152711,
0.8419576152711,0.8419576152711),(1.474127154187,1.474127154187,1.474127154187,
1.474127154187,1.474127154187,1.474127154187,1.474127154187,1.474127154187,
1.474127154187,1.474127154187)))
REPRESENTATION_ITEM('')
SURFACE()
);
#2524=(
BOUNDED_SURFACE()
B_SPLINE_SURFACE(3,3,((#143855,#143856,#143857,#143858,#143859,#143860,
#143861,#143862,#143863,#143864),(#143865,#143866,#143867,#143868,#143869,
#143870,#143871,#143872,#143873,#143874),(#143875,#143876,#143877,#143878,
#143879,#143880,#143881,#143882,#143883,#143884),(#143885,#143886,#143887,
#143888,#143889,#143890,#143891,#143892,#143893,#143894)),.UNSPECIFIED.,
 .F.,.F.,.F.)
B_SPLINE_SURFACE_WITH_KNOTS((4,4),(4,1,1,1,1,1,1,4),(0.,1.),(0.,0.0339830500431831,
0.220389385504102,0.405800841682597,0.58634133762222,0.758214941734974,
0.924667979715977,1.),.UNSPECIFIED.)
GEOMETRIC_REPRESENTATION_ITEM()
RATIONAL_B_SPLINE_SURFACE(((1.474147508313,1.474147508313,1.474147508313,
1.474147508313,1.474147508313,1.474147508313,1.474147508313,1.474147508313,
1.474147508313,1.474147508313),(0.8419508305625,0.8419508305625,0.8419508305625,
0.8419508305625,0.8419508305625,0.8419508305625,0.8419508305625,0.8419508305625,
0.8419508305625,0.8419508305625),(0.8419508305625,0.8419508305625,0.8419508305625,
0.8419508305625,0.8419508305625,0.8419508305625,0.8419508305625,0.8419508305625,
0.8419508305625,0.8419508305625),(1.474147508313,1.474147508313,1.474147508313,
1.474147508313,1.474147508313,1.474147508313,1.474147508313,1.474147508313,
1.474147508313,1.474147508313)))
REPRESENTATION_ITEM('')
SURFACE()
);
#2525=(
BOUNDED_SURFACE()
B_SPLINE_SURFACE(3,3,((#144431,#144432,#144433,#144434,#144435,#144436,
#144437,#144438,#144439,#144440,#144441,#144442),(#144443,#144444,#144445,
#144446,#144447,#144448,#144449,#144450,#144451,#144452,#144453,#144454),
(#144455,#144456,#144457,#144458,#144459,#144460,#144461,#144462,#144463,
#144464,#144465,#144466),(#144467,#144468,#144469,#144470,#144471,#144472,
#144473,#144474,#144475,#144476,#144477,#144478)),.UNSPECIFIED.,.F.,.F.,
 .F.)
B_SPLINE_SURFACE_WITH_KNOTS((4,4),(4,1,1,1,1,1,1,1,1,4),(0.,1.),(0.,0.138818488903363,
0.265940452688414,0.381533804843745,0.48830798531101,0.587709442370304,
0.691765681012883,0.798051585674866,0.902466958148731,1.),.UNSPECIFIED.)
GEOMETRIC_REPRESENTATION_ITEM()
RATIONAL_B_SPLINE_SURFACE(((1.438707812053,1.438707812053,1.438707812053,
1.438707812053,1.438707812053,1.438707812053,1.438707812053,1.438707812053,
1.438707812053,1.438707812053,1.438707812053,1.438707812053),(0.853764062649,
0.853764062649,0.853764062649,0.853764062649,0.853764062649,0.853764062649,
0.853764062649,0.853764062649,0.853764062649,0.853764062649,0.853764062649,
0.853764062649),(0.853764062649,0.853764062649,0.853764062649,0.853764062649,
0.853764062649,0.853764062649,0.853764062649,0.853764062649,0.853764062649,
0.853764062649,0.853764062649,0.853764062649),(1.438707812053,1.438707812053,
1.438707812053,1.438707812053,1.438707812053,1.438707812053,1.438707812053,
1.438707812053,1.438707812053,1.438707812053,1.438707812053,1.438707812053)))
REPRESENTATION_ITEM('')
SURFACE()
);
#2526=(
BOUNDED_SURFACE()
B_SPLINE_SURFACE(3,3,((#144481,#144482,#144483,#144484,#144485,#144486,
#144487,#144488,#144489,#144490,#144491,#144492,#144493,#144494,#144495,
#144496),(#144497,#144498,#144499,#144500,#144501,#144502,#144503,#144504,
#144505,#144506,#144507,#144508,#144509,#144510,#144511,#144512),(#144513,
#144514,#144515,#144516,#144517,#144518,#144519,#144520,#144521,#144522,
#144523,#144524,#144525,#144526,#144527,#144528),(#144529,#144530,#144531,
#144532,#144533,#144534,#144535,#144536,#144537,#144538,#144539,#144540,
#144541,#144542,#144543,#144544)),.UNSPECIFIED.,.F.,.F.,.F.)
B_SPLINE_SURFACE_WITH_KNOTS((4,4),(4,1,1,1,1,1,1,1,1,1,1,1,1,4),(0.,1.),
(0.,0.0400287123538256,0.085970757690431,0.136438109413432,0.191920076265951,
0.252892665741402,0.319816049166386,0.393195571222119,0.473564327244262,
0.561361330336151,0.656626165655672,0.760754425605914,0.875598191304292,
1.),.UNSPECIFIED.)
GEOMETRIC_REPRESENTATION_ITEM()
RATIONAL_B_SPLINE_SURFACE(((1.438707901845,1.438707901845,1.438707901845,
1.438707901845,1.438707901845,1.438707901845,1.438707901845,1.438707901845,
1.438707901845,1.438707901845,1.438707901845,1.438707901845,1.438707901845,
1.438707901845,1.438707901845,1.438707901845),(0.8537640327185,0.8537640327185,
0.8537640327185,0.8537640327185,0.8537640327185,0.8537640327185,0.8537640327185,
0.8537640327185,0.8537640327185,0.8537640327185,0.8537640327185,0.8537640327185,
0.8537640327185,0.8537640327185,0.8537640327185,0.8537640327185),(0.8537640327185,
0.8537640327185,0.8537640327185,0.8537640327185,0.8537640327185,0.8537640327185,
0.8537640327185,0.8537640327185,0.8537640327185,0.8537640327185,0.8537640327185,
0.8537640327185,0.8537640327185,0.8537640327185,0.8537640327185,0.8537640327185),
(1.438707901845,1.438707901845,1.438707901845,1.438707901845,1.438707901845,
1.438707901845,1.438707901845,1.438707901845,1.438707901845,1.438707901845,
1.438707901845,1.438707901845,1.438707901845,1.438707901845,1.438707901845,
1.438707901845)))
REPRESENTATION_ITEM('')
SURFACE()
);
#2527=(
BOUNDED_SURFACE()
B_SPLINE_SURFACE(3,3,((#144697,#144698,#144699,#144700,#144701,#144702,
#144703),(#144704,#144705,#144706,#144707,#144708,#144709,#144710),(#144711,
#144712,#144713,#144714,#144715,#144716,#144717),(#144718,#144719,#144720,
#144721,#144722,#144723,#144724)),.UNSPECIFIED.,.F.,.F.,.F.)
B_SPLINE_SURFACE_WITH_KNOTS((4,4),(4,1,1,1,4),(0.,1.),(0.,0.0527467299113482,
0.354834542652793,0.677277799939644,1.),.UNSPECIFIED.)
GEOMETRIC_REPRESENTATION_ITEM()
RATIONAL_B_SPLINE_SURFACE(((1.416282589503,1.416282589503,1.416282589503,
1.416282589503,1.416282589503,1.416282589503,1.416282589503),(0.8612391368322,
0.8612391368322,0.8612391368322,0.8612391368322,0.8612391368322,0.8612391368322,
0.8612391368322),(0.8612391368322,0.8612391368322,0.8612391368322,0.8612391368322,
0.8612391368322,0.8612391368322,0.8612391368322),(1.416282589503,1.416282589503,
1.416282589503,1.416282589503,1.416282589503,1.416282589503,1.416282589503)))
REPRESENTATION_ITEM('')
SURFACE()
);
#2528=(
BOUNDED_SURFACE()
B_SPLINE_SURFACE(3,3,((#144726,#144727,#144728,#144729,#144730,#144731,
#144732,#144733,#144734,#144735,#144736,#144737),(#144738,#144739,#144740,
#144741,#144742,#144743,#144744,#144745,#144746,#144747,#144748,#144749),
(#144750,#144751,#144752,#144753,#144754,#144755,#144756,#144757,#144758,
#144759,#144760,#144761),(#144762,#144763,#144764,#144765,#144766,#144767,
#144768,#144769,#144770,#144771,#144772,#144773)),.UNSPECIFIED.,.F.,.F.,
 .F.)
B_SPLINE_SURFACE_WITH_KNOTS((4,4),(4,1,1,1,1,1,1,1,1,4),(0.,1.),(0.,0.113647120730493,
0.219125808734348,0.329468109271596,0.439978777291567,0.551628244914102,
0.666572223899566,0.781504772087705,0.893407203154914,1.),.UNSPECIFIED.)
GEOMETRIC_REPRESENTATION_ITEM()
RATIONAL_B_SPLINE_SURFACE(((1.411871186478,1.411871186478,1.411871186478,
1.411871186478,1.411871186478,1.411871186478,1.411871186478,1.411871186478,
1.411871186478,1.411871186478,1.411871186478,1.411871186478),(0.8627096045073,
0.8627096045073,0.8627096045073,0.8627096045073,0.8627096045073,0.8627096045073,
0.8627096045073,0.8627096045073,0.8627096045073,0.8627096045073,0.8627096045073,
0.8627096045073),(0.8627096045073,0.8627096045073,0.8627096045073,0.8627096045073,
0.8627096045073,0.8627096045073,0.8627096045073,0.8627096045073,0.8627096045073,
0.8627096045073,0.8627096045073,0.8627096045073),(1.411871186478,1.411871186478,
1.411871186478,1.411871186478,1.411871186478,1.411871186478,1.411871186478,
1.411871186478,1.411871186478,1.411871186478,1.411871186478,1.411871186478)))
REPRESENTATION_ITEM('')
SURFACE()
);
#2529=(
BOUNDED_SURFACE()
B_SPLINE_SURFACE(3,3,((#144849,#144850,#144851,#144852,#144853,#144854),
(#144855,#144856,#144857,#144858,#144859,#144860),(#144861,#144862,#144863,
#144864,#144865,#144866),(#144867,#144868,#144869,#144870,#144871,#144872)),
 .UNSPECIFIED.,.F.,.F.,.F.)
B_SPLINE_SURFACE_WITH_KNOTS((4,4),(4,1,1,4),(0.,1.),(0.,0.373237854628505,
0.718584603248465,1.),.UNSPECIFIED.)
GEOMETRIC_REPRESENTATION_ITEM()
RATIONAL_B_SPLINE_SURFACE(((1.416338033926,1.416338033926,1.416338033926,
1.416338033926,1.416338033926,1.416338033926),(0.861220655358,0.861220655358,
0.861220655358,0.861220655358,0.861220655358,0.861220655358),(0.861220655358,
0.861220655358,0.861220655358,0.861220655358,0.861220655358,0.861220655358),
(1.416338033926,1.416338033926,1.416338033926,1.416338033926,1.416338033926,
1.416338033926)))
REPRESENTATION_ITEM('')
SURFACE()
);
#2530=(
BOUNDED_SURFACE()
B_SPLINE_SURFACE(3,3,((#144894,#144895,#144896,#144897,#144898,#144899,
#144900,#144901,#144902,#144903,#144904,#144905,#144906,#144907),(#144908,
#144909,#144910,#144911,#144912,#144913,#144914,#144915,#144916,#144917,
#144918,#144919,#144920,#144921),(#144922,#144923,#144924,#144925,#144926,
#144927,#144928,#144929,#144930,#144931,#144932,#144933,#144934,#144935),
(#144936,#144937,#144938,#144939,#144940,#144941,#144942,#144943,#144944,
#144945,#144946,#144947,#144948,#144949)),.UNSPECIFIED.,.F.,.F.,.F.)
B_SPLINE_SURFACE_WITH_KNOTS((4,4),(4,1,1,1,1,1,1,1,1,1,1,4),(0.,1.),(0.,
0.0189196969648684,0.123026245101233,0.22799245863482,0.333423755560677,
0.4381783971276,0.543725879883426,0.653238579359784,0.762171136752647,0.869991259904252,
0.976017729140831,1.),.UNSPECIFIED.)
GEOMETRIC_REPRESENTATION_ITEM()
RATIONAL_B_SPLINE_SURFACE(((1.411894266579,1.411894266579,1.411894266579,
1.411894266579,1.411894266579,1.411894266579,1.411894266579,1.411894266579,
1.411894266579,1.411894266579,1.411894266579,1.411894266579,1.411894266579,
1.411894266579),(0.8627019111402,0.8627019111402,0.8627019111402,0.8627019111402,
0.8627019111402,0.8627019111402,0.8627019111402,0.8627019111402,0.8627019111402,
0.8627019111402,0.8627019111402,0.8627019111402,0.8627019111402,0.8627019111402),
(0.8627019111402,0.8627019111402,0.8627019111402,0.8627019111402,0.8627019111402,
0.8627019111402,0.8627019111402,0.8627019111402,0.8627019111402,0.8627019111402,
0.8627019111402,0.8627019111402,0.8627019111402,0.8627019111402),(1.411894266579,
1.411894266579,1.411894266579,1.411894266579,1.411894266579,1.411894266579,
1.411894266579,1.411894266579,1.411894266579,1.411894266579,1.411894266579,
1.411894266579,1.411894266579,1.411894266579)))
REPRESENTATION_ITEM('')
SURFACE()
);
#2531=(
BOUNDED_SURFACE()
B_SPLINE_SURFACE(3,3,((#145190,#145191,#145192,#145193,#145194,#145195,
#145196,#145197),(#145198,#145199,#145200,#145201,#145202,#145203,#145204,
#145205),(#145206,#145207,#145208,#145209,#145210,#145211,#145212,#145213),
(#145214,#145215,#145216,#145217,#145218,#145219,#145220,#145221)),
 .UNSPECIFIED.,.F.,.F.,.F.)
B_SPLINE_SURFACE_WITH_KNOTS((4,4),(4,1,1,1,1,4),(0.,1.),(0.,0.0014184679519637,
0.26748144230672,0.529910202206513,0.793736319541623,1.),.UNSPECIFIED.)
GEOMETRIC_REPRESENTATION_ITEM()
RATIONAL_B_SPLINE_SURFACE(((1.400814311523,1.400814311523,1.400814311523,
1.400814311523,1.400814311523,1.400814311523,1.400814311523,1.400814311523),
(0.8663952294922,0.8663952294922,0.8663952294922,0.8663952294922,0.8663952294922,
0.8663952294922,0.8663952294922,0.8663952294922),(0.8663952294922,0.8663952294922,
0.8663952294922,0.8663952294922,0.8663952294922,0.8663952294922,0.8663952294922,
0.8663952294922),(1.400814311523,1.400814311523,1.400814311523,1.400814311523,
1.400814311523,1.400814311523,1.400814311523,1.400814311523)))
REPRESENTATION_ITEM('')
SURFACE()
);
#2532=(
BOUNDED_SURFACE()
B_SPLINE_SURFACE(3,3,((#145223,#145224,#145225,#145226),(#145227,#145228,
#145229,#145230),(#145231,#145232,#145233,#145234),(#145235,#145236,#145237,
#145238)),.UNSPECIFIED.,.F.,.F.,.F.)
B_SPLINE_SURFACE_WITH_KNOTS((4,4),(4,4),(0.,1.),(0.,1.),.UNSPECIFIED.)
GEOMETRIC_REPRESENTATION_ITEM()
RATIONAL_B_SPLINE_SURFACE(((1.292992000439,1.292992000439,1.292992000439,
1.292992000439),(0.9023359998537,0.9023359998537,0.9023359998537,0.9023359998537),
(0.9023359998537,0.9023359998537,0.9023359998537,0.9023359998537),(1.292992000439,
1.292992000439,1.292992000439,1.292992000439)))
REPRESENTATION_ITEM('')
SURFACE()
);
#2533=(
BOUNDED_SURFACE()
B_SPLINE_SURFACE(3,3,((#145638,#145639,#145640,#145641,#145642,#145643,
#145644,#145645,#145646,#145647,#145648,#145649,#145650,#145651,#145652,
#145653),(#145654,#145655,#145656,#145657,#145658,#145659,#145660,#145661,
#145662,#145663,#145664,#145665,#145666,#145667,#145668,#145669),(#145670,
#145671,#145672,#145673,#145674,#145675,#145676,#145677,#145678,#145679,
#145680,#145681,#145682,#145683,#145684,#145685),(#145686,#145687,#145688,
#145689,#145690,#145691,#145692,#145693,#145694,#145695,#145696,#145697,
#145698,#145699,#145700,#145701)),.UNSPECIFIED.,.F.,.F.,.F.)
B_SPLINE_SURFACE_WITH_KNOTS((4,4),(4,1,1,1,1,1,1,1,1,1,1,1,1,4),(0.,1.),
(0.,0.0559219040610143,0.119566494393519,0.185306102594679,0.252047391027673,
0.319960693178036,0.38890975610616,0.458498614355498,0.530499085950225,
0.608940039864404,0.696077429834816,0.792156237533156,0.898636382678449,
1.),.UNSPECIFIED.)
GEOMETRIC_REPRESENTATION_ITEM()
RATIONAL_B_SPLINE_SURFACE(((1.307002971129,1.307002971129,1.307002971129,
1.307002971129,1.307002971129,1.307002971129,1.307002971129,1.307002971129,
1.307002971129,1.307002971129,1.307002971129,1.307002971129,1.307002971129,
1.307002971129,1.307002971129,1.307002971129),(0.8976656762905,0.8976656762905,
0.8976656762905,0.8976656762905,0.8976656762905,0.8976656762905,0.8976656762905,
0.8976656762905,0.8976656762905,0.8976656762905,0.8976656762905,0.8976656762905,
0.8976656762905,0.8976656762905,0.8976656762905,0.8976656762905),(0.8976656762905,
0.8976656762905,0.8976656762905,0.8976656762905,0.8976656762905,0.8976656762905,
0.8976656762905,0.8976656762905,0.8976656762905,0.8976656762905,0.8976656762905,
0.8976656762905,0.8976656762905,0.8976656762905,0.8976656762905,0.8976656762905),
(1.307002971129,1.307002971129,1.307002971129,1.307002971129,1.307002971129,
1.307002971129,1.307002971129,1.307002971129,1.307002971129,1.307002971129,
1.307002971129,1.307002971129,1.307002971129,1.307002971129,1.307002971129,
1.307002971129)))
REPRESENTATION_ITEM('')
SURFACE()
);
#2534=(
BOUNDED_SURFACE()
B_SPLINE_SURFACE(3,3,((#145952,#145953,#145954,#145955,#145956,#145957,
#145958,#145959,#145960,#145961,#145962,#145963,#145964),(#145965,#145966,
#145967,#145968,#145969,#145970,#145971,#145972,#145973,#145974,#145975,
#145976,#145977),(#145978,#145979,#145980,#145981,#145982,#145983,#145984,
#145985,#145986,#145987,#145988,#145989,#145990),(#145991,#145992,#145993,
#145994,#145995,#145996,#145997,#145998,#145999,#146000,#146001,#146002,
#146003)),.UNSPECIFIED.,.F.,.F.,.F.)
B_SPLINE_SURFACE_WITH_KNOTS((4,4),(4,1,1,1,1,1,1,1,1,1,4),(0.,1.),(0.,0.0361770017020252,
0.110322638446908,0.191341394631034,0.279299595253617,0.374729923390192,
0.478819817310066,0.592531700959653,0.717431194571663,0.855542845896087,
1.),.UNSPECIFIED.)
GEOMETRIC_REPRESENTATION_ITEM()
RATIONAL_B_SPLINE_SURFACE(((1.17157330090261,1.17157330090261,1.17157330090261,
1.17157330090261,1.17157330090261,1.17157330090261,1.17157330090261,1.17157330090261,
1.17157330090261,1.17157330090261,1.17157330090261,1.17157330090261,1.17157330090261),
(0.942808938970757,0.942808938970757,0.942808938970757,0.942808938970757,
0.942808938970757,0.942808938970757,0.942808938970757,0.942808938970757,
0.942808938970757,0.942808938970757,0.942808938970757,0.942808938970757,
0.942808938970757),(0.942808899699103,0.942808899699103,0.942808899699103,
0.942808899699103,0.942808899699103,0.942808899699103,0.942808899699103,
0.942808899699103,0.942808899699103,0.942808899699103,0.942808899699103,
0.942808899699103,0.942808899699103),(1.17157318308765,1.17157318308765,
1.17157318308765,1.17157318308765,1.17157318308765,1.17157318308765,1.17157318308765,
1.17157318308765,1.17157318308765,1.17157318308765,1.17157318308765,1.17157318308765,
1.17157318308765)))
REPRESENTATION_ITEM('')
SURFACE()
);
#2535=(
BOUNDED_SURFACE()
B_SPLINE_SURFACE(3,3,((#146010,#146011,#146012,#146013,#146014,#146015),
(#146016,#146017,#146018,#146019,#146020,#146021),(#146022,#146023,#146024,
#146025,#146026,#146027),(#146028,#146029,#146030,#146031,#146032,#146033)),
 .UNSPECIFIED.,.F.,.F.,.F.)
B_SPLINE_SURFACE_WITH_KNOTS((4,4),(4,1,1,4),(0.,1.),(0.,0.143192077928725,
0.593387555486125,1.),.UNSPECIFIED.)
GEOMETRIC_REPRESENTATION_ITEM()
RATIONAL_B_SPLINE_SURFACE(((1.365448016002,1.365448016002,1.365448016002,
1.365448016002,1.365448016002,1.365448016002),(0.878183994666,0.878183994666,
0.878183994666,0.878183994666,0.878183994666,0.878183994666),(0.878183994666,
0.878183994666,0.878183994666,0.878183994666,0.878183994666,0.878183994666),
(1.365448016002,1.365448016002,1.365448016002,1.365448016002,1.365448016002,
1.365448016002)))
REPRESENTATION_ITEM('')
SURFACE()
);
#2536=(
BOUNDED_SURFACE()
B_SPLINE_SURFACE(3,3,((#146131,#146132,#146133,#146134,#146135,#146136,
#146137,#146138,#146139),(#146140,#146141,#146142,#146143,#146144,#146145,
#146146,#146147,#146148),(#146149,#146150,#146151,#146152,#146153,#146154,
#146155,#146156,#146157),(#146158,#146159,#146160,#146161,#146162,#146163,
#146164,#146165,#146166)),.UNSPECIFIED.,.F.,.F.,.F.)
B_SPLINE_SURFACE_WITH_KNOTS((4,4),(4,1,1,1,1,1,4),(0.,1.),(0.,0.210945365171019,
0.440528327664717,0.642835784013808,0.823409899665082,0.985793689031676,
1.),.UNSPECIFIED.)
GEOMETRIC_REPRESENTATION_ITEM()
RATIONAL_B_SPLINE_SURFACE(((1.289189279229,1.289189279229,1.289189279229,
1.289189279229,1.289189279229,1.289189279229,1.289189279229,1.289189279229,
1.289189279229),(0.9036035735905,0.9036035735905,0.9036035735905,0.9036035735905,
0.9036035735905,0.9036035735905,0.9036035735905,0.9036035735905,0.9036035735905),
(0.9036035735905,0.9036035735905,0.9036035735905,0.9036035735905,0.9036035735905,
0.9036035735905,0.9036035735905,0.9036035735905,0.9036035735905),(1.289189279229,
1.289189279229,1.289189279229,1.289189279229,1.289189279229,1.289189279229,
1.289189279229,1.289189279229,1.289189279229)))
REPRESENTATION_ITEM('')
SURFACE()
);
#2537=(
BOUNDED_SURFACE()
B_SPLINE_SURFACE(3,3,((#146194,#146195,#146196,#146197,#146198,#146199,
#146200,#146201),(#146202,#146203,#146204,#146205,#146206,#146207,#146208,
#146209),(#146210,#146211,#146212,#146213,#146214,#146215,#146216,#146217),
(#146218,#146219,#146220,#146221,#146222,#146223,#146224,#146225)),
 .UNSPECIFIED.,.F.,.F.,.F.)
B_SPLINE_SURFACE_WITH_KNOTS((4,4),(4,1,1,1,1,4),(0.,1.),(0.,0.0487760373381725,
0.313271775641559,0.605696041835668,0.929388134239699,1.),.UNSPECIFIED.)
GEOMETRIC_REPRESENTATION_ITEM()
RATIONAL_B_SPLINE_SURFACE(((1.19718919652,1.19718919652,1.19718919652,1.19718919652,
1.19718919652,1.19718919652,1.19718919652,1.19718919652),(0.9342702678265,
0.9342702678265,0.9342702678265,0.9342702678265,0.9342702678265,0.9342702678265,
0.9342702678265,0.9342702678265),(0.9342702678265,0.9342702678265,0.9342702678265,
0.9342702678265,0.9342702678265,0.9342702678265,0.9342702678265,0.9342702678265),
(1.19718919652,1.19718919652,1.19718919652,1.19718919652,1.19718919652,
1.19718919652,1.19718919652,1.19718919652)))
REPRESENTATION_ITEM('')
SURFACE()
);
#2538=(
BOUNDED_SURFACE()
B_SPLINE_SURFACE(3,3,((#146429,#146430,#146431,#146432,#146433,#146434,
#146435,#146436),(#146437,#146438,#146439,#146440,#146441,#146442,#146443,
#146444),(#146445,#146446,#146447,#146448,#146449,#146450,#146451,#146452),
(#146453,#146454,#146455,#146456,#146457,#146458,#146459,#146460)),
 .UNSPECIFIED.,.F.,.F.,.F.)
B_SPLINE_SURFACE_WITH_KNOTS((4,4),(4,1,1,1,1,4),(0.,1.),(0.,0.218953851268331,
0.474954346235349,0.702206697993898,0.905113568673651,1.),.UNSPECIFIED.)
GEOMETRIC_REPRESENTATION_ITEM()
RATIONAL_B_SPLINE_SURFACE(((1.289211918215,1.289211918215,1.289211918215,
1.289211918215,1.289211918215,1.289211918215,1.289211918215,1.289211918215),
(0.9035960272617,0.9035960272617,0.9035960272617,0.9035960272617,0.9035960272617,
0.9035960272617,0.9035960272617,0.9035960272617),(0.9035960272617,0.9035960272617,
0.9035960272617,0.9035960272617,0.9035960272617,0.9035960272617,0.9035960272617,
0.9035960272617),(1.289211918215,1.289211918215,1.289211918215,1.289211918215,
1.289211918215,1.289211918215,1.289211918215,1.289211918215)))
REPRESENTATION_ITEM('')
SURFACE()
);
#2539=(
BOUNDED_SURFACE()
B_SPLINE_SURFACE(3,3,((#146696,#146697,#146698,#146699,#146700,#146701,
#146702,#146703,#146704,#146705,#146706,#146707,#146708),(#146709,#146710,
#146711,#146712,#146713,#146714,#146715,#146716,#146717,#146718,#146719,
#146720,#146721),(#146722,#146723,#146724,#146725,#146726,#146727,#146728,
#146729,#146730,#146731,#146732,#146733,#146734),(#146735,#146736,#146737,
#146738,#146739,#146740,#146741,#146742,#146743,#146744,#146745,#146746,
#146747)),.UNSPECIFIED.,.F.,.F.,.F.)
B_SPLINE_SURFACE_WITH_KNOTS((4,4),(4,1,1,1,1,1,1,1,1,1,4),(0.,1.),(0.,0.0617308889043711,
0.222967927738356,0.364574399931382,0.491340784341846,0.605251267138888,
0.708180598151713,0.801277211250371,0.885526519088398,0.96089518018748,
1.),.UNSPECIFIED.)
GEOMETRIC_REPRESENTATION_ITEM()
RATIONAL_B_SPLINE_SURFACE(((1.225181244217,1.225181244217,1.225181244217,
1.225181244217,1.225181244217,1.225181244217,1.225181244217,1.225181244217,
1.225181244217,1.225181244217,1.225181244217,1.225181244217,1.225181244217),
(0.9249395852609,0.9249395852609,0.9249395852609,0.9249395852609,0.9249395852609,
0.9249395852609,0.9249395852609,0.9249395852609,0.9249395852609,0.9249395852609,
0.9249395852609,0.9249395852609,0.9249395852609),(0.9249395852609,0.9249395852609,
0.9249395852609,0.9249395852609,0.9249395852609,0.9249395852609,0.9249395852609,
0.9249395852609,0.9249395852609,0.9249395852609,0.9249395852609,0.9249395852609,
0.9249395852609),(1.225181244217,1.225181244217,1.225181244217,1.225181244217,
1.225181244217,1.225181244217,1.225181244217,1.225181244217,1.225181244217,
1.225181244217,1.225181244217,1.225181244217,1.225181244217)))
REPRESENTATION_ITEM('')
SURFACE()
);
#2540=(
BOUNDED_SURFACE()
B_SPLINE_SURFACE(3,3,((#146837,#146838,#146839,#146840,#146841,#146842,
#146843,#146844,#146845,#146846,#146847,#146848,#146849,#146850,#146851,
#146852,#146853),(#146854,#146855,#146856,#146857,#146858,#146859,#146860,
#146861,#146862,#146863,#146864,#146865,#146866,#146867,#146868,#146869,
#146870),(#146871,#146872,#146873,#146874,#146875,#146876,#146877,#146878,
#146879,#146880,#146881,#146882,#146883,#146884,#146885,#146886,#146887),
(#146888,#146889,#146890,#146891,#146892,#146893,#146894,#146895,#146896,
#146897,#146898,#146899,#146900,#146901,#146902,#146903,#146904)),
 .UNSPECIFIED.,.F.,.F.,.F.)
B_SPLINE_SURFACE_WITH_KNOTS((4,4),(4,1,1,1,1,1,1,1,1,1,1,1,1,1,4),(0.,1.),
(0.,0.0169119460810613,0.0654242130848353,0.118166345404895,0.175802236516308,
0.238929210760529,0.307690566088615,0.381894800562219,0.461375561007429,
0.546721723948187,0.639112945312709,0.739719346812922,0.849650913359874,
0.96995594614347,1.),.UNSPECIFIED.)
GEOMETRIC_REPRESENTATION_ITEM()
RATIONAL_B_SPLINE_SURFACE(((1.02563715093864,1.02563715093864,1.02563715093864,
1.02563715093864,1.02563715093864,1.02563715093864,1.02563715093864,1.02563715093864,
1.02563715093864,1.02563715093864,1.02563715093864,1.02563715093864,1.02563715093864,
1.02563715093864,1.02563715093864,1.02563715093864,1.02563715093864),(1.00821461019054,
1.00821461019054,1.00821461019054,1.00821461019054,1.00821461019054,1.00821461019054,
1.00821461019054,1.00821461019054,1.00821461019054,1.00821461019054,1.00821461019054,
1.00821461019054,1.00821461019054,1.00821461019054,1.00821461019054,1.00821461019054,
1.00821461019054),(0.999672100423032,0.999672100423032,0.999672100423032,
0.999672100423032,0.999672100423032,0.999672100423032,0.999672100423032,
0.999672100423032,0.999672100423032,0.999672100423032,0.999672100423032,
0.999672100423032,0.999672100423032,0.999672100423032,0.999672100423032,
0.999672100423032,0.999672100423032),(1.00000962163611,1.00000962163611,
1.00000962163611,1.00000962163611,1.00000962163611,1.00000962163611,1.00000962163611,
1.00000962163611,1.00000962163611,1.00000962163611,1.00000962163611,1.00000962163611,
1.00000962163611,1.00000962163611,1.00000962163611,1.00000962163611,1.00000962163611)))
REPRESENTATION_ITEM('')
SURFACE()
);
#2541=(
BOUNDED_SURFACE()
B_SPLINE_SURFACE(3,3,((#146935,#146936,#146937,#146938,#146939,#146940),
(#146941,#146942,#146943,#146944,#146945,#146946),(#146947,#146948,#146949,
#146950,#146951,#146952),(#146953,#146954,#146955,#146956,#146957,#146958)),
 .UNSPECIFIED.,.F.,.F.,.F.)
B_SPLINE_SURFACE_WITH_KNOTS((4,4),(4,1,1,4),(0.,1.),(0.,0.330743299833935,
0.694013975265241,1.),.UNSPECIFIED.)
GEOMETRIC_REPRESENTATION_ITEM()
RATIONAL_B_SPLINE_SURFACE(((1.289433315103,1.289433315103,1.289433315103,
1.289433315103,1.289433315103,1.289433315103),(0.9035222282991,0.9035222282991,
0.9035222282991,0.9035222282991,0.9035222282991,0.9035222282991),(0.9035222282991,
0.9035222282991,0.9035222282991,0.9035222282991,0.9035222282991,0.9035222282991),
(1.289433315103,1.289433315103,1.289433315103,1.289433315103,1.289433315103,
1.289433315103)))
REPRESENTATION_ITEM('')
SURFACE()
);
#2542=(
BOUNDED_SURFACE()
B_SPLINE_SURFACE(3,3,((#147219,#147220,#147221,#147222,#147223,#147224,
#147225,#147226,#147227,#147228,#147229),(#147230,#147231,#147232,#147233,
#147234,#147235,#147236,#147237,#147238,#147239,#147240),(#147241,#147242,
#147243,#147244,#147245,#147246,#147247,#147248,#147249,#147250,#147251),
(#147252,#147253,#147254,#147255,#147256,#147257,#147258,#147259,#147260,
#147261,#147262)),.UNSPECIFIED.,.F.,.F.,.F.)
B_SPLINE_SURFACE_WITH_KNOTS((4,4),(4,1,1,1,1,1,1,1,4),(0.,1.),(0.,0.09718625494397,
0.209222889679937,0.33412363069135,0.473952091224752,0.627037941696765,
0.768578301480889,0.892964492195342,1.),.UNSPECIFIED.)
GEOMETRIC_REPRESENTATION_ITEM()
RATIONAL_B_SPLINE_SURFACE(((1.155039452605,1.155039452605,1.155039452605,
1.155039452605,1.155039452605,1.155039452605,1.155039452605,1.155039452605,
1.155039452605,1.155039452605,1.155039452605),(0.9483201824649,0.9483201824649,
0.9483201824649,0.9483201824649,0.9483201824649,0.9483201824649,0.9483201824649,
0.9483201824649,0.9483201824649,0.9483201824649,0.9483201824649),(0.9483201824649,
0.9483201824649,0.9483201824649,0.9483201824649,0.9483201824649,0.9483201824649,
0.9483201824649,0.9483201824649,0.9483201824649,0.9483201824649,0.9483201824649),
(1.155039452605,1.155039452605,1.155039452605,1.155039452605,1.155039452605,
1.155039452605,1.155039452605,1.155039452605,1.155039452605,1.155039452605,
1.155039452605)))
REPRESENTATION_ITEM('')
SURFACE()
);
#2543=(
BOUNDED_SURFACE()
B_SPLINE_SURFACE(3,3,((#147376,#147377,#147378,#147379,#147380,#147381),
(#147382,#147383,#147384,#147385,#147386,#147387),(#147388,#147389,#147390,
#147391,#147392,#147393),(#147394,#147395,#147396,#147397,#147398,#147399)),
 .UNSPECIFIED.,.F.,.F.,.F.)
B_SPLINE_SURFACE_WITH_KNOTS((4,4),(4,1,1,4),(0.,1.),(0.,0.335198257973395,
0.677912136352372,1.),.UNSPECIFIED.)
GEOMETRIC_REPRESENTATION_ITEM()
RATIONAL_B_SPLINE_SURFACE(((1.097833560248,1.097833560248,1.097833560248,
1.097833560248,1.097833560248,1.097833560248),(0.9673888132507,0.9673888132507,
0.9673888132507,0.9673888132507,0.9673888132507,0.9673888132507),(0.9673888132507,
0.9673888132507,0.9673888132507,0.9673888132507,0.9673888132507,0.9673888132507),
(1.097833560248,1.097833560248,1.097833560248,1.097833560248,1.097833560248,
1.097833560248)))
REPRESENTATION_ITEM('')
SURFACE()
);
#2544=(
BOUNDED_SURFACE()
B_SPLINE_SURFACE(3,3,((#147427,#147428,#147429,#147430),(#147431,#147432,
#147433,#147434),(#147435,#147436,#147437,#147438),(#147439,#147440,#147441,
#147442)),.UNSPECIFIED.,.F.,.F.,.F.)
B_SPLINE_SURFACE_WITH_KNOTS((4,4),(4,4),(0.,1.),(0.,1.),.UNSPECIFIED.)
GEOMETRIC_REPRESENTATION_ITEM()
RATIONAL_B_SPLINE_SURFACE(((1.007258252712,0.8716678894048,0.857683274695,
0.9653044085823),(1.006827278554,0.879287880805,0.8661336322704,0.9673645329503),
(1.00640304118,0.8867887601249,0.8744518978764,0.9693924544342),(1.006012840932,
0.8936878339527,0.882102778005,0.971257673089)))
REPRESENTATION_ITEM('')
SURFACE()
);
#2545=(
BOUNDED_SURFACE()
B_SPLINE_SURFACE(3,3,((#147485,#147486,#147487,#147488,#147489,#147490,
#147491,#147492,#147493,#147494,#147495,#147496,#147497,#147498,#147499,
#147500,#147501,#147502,#147503,#147504,#147505,#147506),(#147507,#147508,
#147509,#147510,#147511,#147512,#147513,#147514,#147515,#147516,#147517,
#147518,#147519,#147520,#147521,#147522,#147523,#147524,#147525,#147526,
#147527,#147528),(#147529,#147530,#147531,#147532,#147533,#147534,#147535,
#147536,#147537,#147538,#147539,#147540,#147541,#147542,#147543,#147544,
#147545,#147546,#147547,#147548,#147549,#147550),(#147551,#147552,#147553,
#147554,#147555,#147556,#147557,#147558,#147559,#147560,#147561,#147562,
#147563,#147564,#147565,#147566,#147567,#147568,#147569,#147570,#147571,
#147572)),.UNSPECIFIED.,.F.,.F.,.F.)
B_SPLINE_SURFACE_WITH_KNOTS((4,4),(4,1,1,1,1,1,1,1,1,1,1,1,1,1,1,1,1,1,
1,4),(0.,1.),(0.,0.0711383255328258,0.137163359302248,0.195720435393546,
0.247715273019436,0.293698370802659,0.336008737306656,0.380005256943101,
0.425168878602564,0.469947554154179,0.513213820955286,0.55641075188751,
0.604436817371917,0.658671873052936,0.719515049298376,0.788488856663347,
0.862062739446009,0.932266724631227,0.998927768427254,1.),.UNSPECIFIED.)
GEOMETRIC_REPRESENTATION_ITEM()
RATIONAL_B_SPLINE_SURFACE(((1.255321345493,1.255321345493,1.255321345493,
1.255321345493,1.255321345493,1.255321345493,1.255321345493,1.255321345493,
1.255321345493,1.255321345493,1.255321345493,1.255321345493,1.255321345493,
1.255321345493,1.255321345493,1.255321345493,1.255321345493,1.255321345493,
1.255321345493,1.255321345493,1.255321345493,1.255321345493),(0.9148928848357,
0.9148928848357,0.9148928848357,0.9148928848357,0.9148928848357,0.9148928848357,
0.9148928848357,0.9148928848357,0.9148928848357,0.9148928848357,0.9148928848357,
0.9148928848357,0.9148928848357,0.9148928848357,0.9148928848357,0.9148928848357,
0.9148928848357,0.9148928848357,0.9148928848357,0.9148928848357,0.9148928848357,
0.9148928848357),(0.9148928848357,0.9148928848357,0.9148928848357,0.9148928848357,
0.9148928848357,0.9148928848357,0.9148928848357,0.9148928848357,0.9148928848357,
0.9148928848357,0.9148928848357,0.9148928848357,0.9148928848357,0.9148928848357,
0.9148928848357,0.9148928848357,0.9148928848357,0.9148928848357,0.9148928848357,
0.9148928848357,0.9148928848357,0.9148928848357),(1.255321345493,1.255321345493,
1.255321345493,1.255321345493,1.255321345493,1.255321345493,1.255321345493,
1.255321345493,1.255321345493,1.255321345493,1.255321345493,1.255321345493,
1.255321345493,1.255321345493,1.255321345493,1.255321345493,1.255321345493,
1.255321345493,1.255321345493,1.255321345493,1.255321345493,1.255321345493)))
REPRESENTATION_ITEM('')
SURFACE()
);
#2546=(
BOUNDED_SURFACE()
B_SPLINE_SURFACE(3,3,((#147722,#147723,#147724,#147725,#147726,#147727,
#147728,#147729,#147730,#147731,#147732,#147733,#147734,#147735,#147736),
(#147737,#147738,#147739,#147740,#147741,#147742,#147743,#147744,#147745,
#147746,#147747,#147748,#147749,#147750,#147751),(#147752,#147753,#147754,
#147755,#147756,#147757,#147758,#147759,#147760,#147761,#147762,#147763,
#147764,#147765,#147766),(#147767,#147768,#147769,#147770,#147771,#147772,
#147773,#147774,#147775,#147776,#147777,#147778,#147779,#147780,#147781)),
 .UNSPECIFIED.,.F.,.F.,.F.)
B_SPLINE_SURFACE_WITH_KNOTS((4,4),(4,1,1,1,1,1,1,1,1,1,1,1,4),(0.,1.),(0.,
0.00433344281298221,0.0666934882632817,0.132801776489929,0.205016366496403,
0.284357715917161,0.370665202265106,0.46484948769096,0.568277692564041,
0.682614773264253,0.810064514841178,0.952973196107536,1.),.UNSPECIFIED.)
GEOMETRIC_REPRESENTATION_ITEM()
RATIONAL_B_SPLINE_SURFACE(((1.116717554521,1.116717554521,1.116717554521,
1.116717554521,1.116717554521,1.116717554521,1.116717554521,1.116717554521,
1.116717554521,1.116717554521,1.116717554521,1.116717554521,1.116717554521,
1.116717554521,1.116717554521),(0.9610941484931,0.9610941484931,0.9610941484931,
0.9610941484931,0.9610941484931,0.9610941484931,0.9610941484931,0.9610941484931,
0.9610941484931,0.9610941484931,0.9610941484931,0.9610941484931,0.9610941484931,
0.9610941484931,0.9610941484931),(0.9610941484931,0.9610941484931,0.9610941484931,
0.9610941484931,0.9610941484931,0.9610941484931,0.9610941484931,0.9610941484931,
0.9610941484931,0.9610941484931,0.9610941484931,0.9610941484931,0.9610941484931,
0.9610941484931,0.9610941484931),(1.116717554521,1.116717554521,1.116717554521,
1.116717554521,1.116717554521,1.116717554521,1.116717554521,1.116717554521,
1.116717554521,1.116717554521,1.116717554521,1.116717554521,1.116717554521,
1.116717554521,1.116717554521)))
REPRESENTATION_ITEM('')
SURFACE()
);
#2547=(
BOUNDED_SURFACE()
B_SPLINE_SURFACE(3,3,((#147835,#147836,#147837,#147838,#147839,#147840,
#147841,#147842,#147843,#147844,#147845,#147846,#147847,#147848,#147849,
#147850,#147851,#147852,#147853,#147854,#147855,#147856,#147857,#147858,
#147859,#147860,#147861,#147862,#147863,#147864,#147865,#147866),(#147867,
#147868,#147869,#147870,#147871,#147872,#147873,#147874,#147875,#147876,
#147877,#147878,#147879,#147880,#147881,#147882,#147883,#147884,#147885,
#147886,#147887,#147888,#147889,#147890,#147891,#147892,#147893,#147894,
#147895,#147896,#147897,#147898),(#147899,#147900,#147901,#147902,#147903,
#147904,#147905,#147906,#147907,#147908,#147909,#147910,#147911,#147912,
#147913,#147914,#147915,#147916,#147917,#147918,#147919,#147920,#147921,
#147922,#147923,#147924,#147925,#147926,#147927,#147928,#147929,#147930),
(#147931,#147932,#147933,#147934,#147935,#147936,#147937,#147938,#147939,
#147940,#147941,#147942,#147943,#147944,#147945,#147946,#147947,#147948,
#147949,#147950,#147951,#147952,#147953,#147954,#147955,#147956,#147957,
#147958,#147959,#147960,#147961,#147962)),.UNSPECIFIED.,.F.,.F.,.F.)
B_SPLINE_SURFACE_WITH_KNOTS((4,4),(4,1,1,1,1,1,1,1,1,1,1,1,1,1,1,1,1,1,
1,1,1,1,1,1,1,1,1,1,1,4),(0.,1.),(0.,0.00739679806268109,0.0171434919654321,
0.0278671486052808,0.0396906394914082,0.0527364856978208,0.0671005283054457,
0.0828041080432213,0.09991535616353,0.118571172417619,0.13891405612076,
0.161058401251212,0.185059763604759,0.211052408434658,0.23922330365136,
0.269821407003499,0.303084978001006,0.338803301575319,0.377356136968251,
0.419277131157154,0.465109562725025,0.515198516585569,0.569694099550452,
0.628581626647206,0.692308097186769,0.762043150357223,0.838144940217723,
0.913367566845421,0.976864842465518,1.),.UNSPECIFIED.)
GEOMETRIC_REPRESENTATION_ITEM()
RATIONAL_B_SPLINE_SURFACE(((1.778014213746,1.778014213746,1.778014213746,
1.778014213746,1.778014213746,1.778014213746,1.778014213746,1.778014213746,
1.778014213746,1.778014213746,1.778014213746,1.778014213746,1.778014213746,
1.778014213746,1.778014213746,1.778014213746,1.778014213746,1.778014213746,
1.778014213746,1.778014213746,1.778014213746,1.778014213746,1.778014213746,
1.778014213746,1.778014213746,1.778014213746,1.778014213746,1.778014213746,
1.778014213746,1.778014213746,1.778014213746,1.778014213746),(0.7406619287514,
0.7406619287514,0.7406619287514,0.7406619287514,0.7406619287514,0.7406619287514,
0.7406619287514,0.7406619287514,0.7406619287514,0.7406619287514,0.7406619287514,
0.7406619287514,0.7406619287514,0.7406619287514,0.7406619287514,0.7406619287514,
0.7406619287514,0.7406619287514,0.7406619287514,0.7406619287514,0.7406619287514,
0.7406619287514,0.7406619287514,0.7406619287514,0.7406619287514,0.7406619287514,
0.7406619287514,0.7406619287514,0.7406619287514,0.7406619287514,0.7406619287514,
0.7406619287514),(0.7406619287514,0.7406619287514,0.7406619287514,0.7406619287514,
0.7406619287514,0.7406619287514,0.7406619287514,0.7406619287514,0.7406619287514,
0.7406619287514,0.7406619287514,0.7406619287514,0.7406619287514,0.7406619287514,
0.7406619287514,0.7406619287514,0.7406619287514,0.7406619287514,0.7406619287514,
0.7406619287514,0.7406619287514,0.7406619287514,0.7406619287514,0.7406619287514,
0.7406619287514,0.7406619287514,0.7406619287514,0.7406619287514,0.7406619287514,
0.7406619287514,0.7406619287514,0.7406619287514),(1.778014213746,1.778014213746,
1.778014213746,1.778014213746,1.778014213746,1.778014213746,1.778014213746,
1.778014213746,1.778014213746,1.778014213746,1.778014213746,1.778014213746,
1.778014213746,1.778014213746,1.778014213746,1.778014213746,1.778014213746,
1.778014213746,1.778014213746,1.778014213746,1.778014213746,1.778014213746,
1.778014213746,1.778014213746,1.778014213746,1.778014213746,1.778014213746,
1.778014213746,1.778014213746,1.778014213746,1.778014213746,1.778014213746)))
REPRESENTATION_ITEM('')
SURFACE()
);
#2548=(
BOUNDED_SURFACE()
B_SPLINE_SURFACE(3,3,((#147977,#147978,#147979,#147980),(#147981,#147982,
#147983,#147984),(#147985,#147986,#147987,#147988),(#147989,#147990,#147991,
#147992)),.UNSPECIFIED.,.F.,.F.,.F.)
B_SPLINE_SURFACE_WITH_KNOTS((4,4),(4,4),(0.,1.),(0.,1.),.UNSPECIFIED.)
GEOMETRIC_REPRESENTATION_ITEM()
RATIONAL_B_SPLINE_SURFACE(((1.1173473569,1.1173473569,1.1173473569,1.1173473569),
(0.9608842143667,0.9608842143667,0.9608842143667,0.9608842143667),(0.9608842143667,
0.9608842143667,0.9608842143667,0.9608842143667),(1.1173473569,1.1173473569,
1.1173473569,1.1173473569)))
REPRESENTATION_ITEM('')
SURFACE()
);
#2549=(
BOUNDED_SURFACE()
B_SPLINE_SURFACE(3,3,((#147999,#148000,#148001,#148002,#148003,#148004,
#148005,#148006,#148007,#148008,#148009,#148010,#148011,#148012,#148013,
#148014,#148015,#148016,#148017,#148018),(#148019,#148020,#148021,#148022,
#148023,#148024,#148025,#148026,#148027,#148028,#148029,#148030,#148031,
#148032,#148033,#148034,#148035,#148036,#148037,#148038),(#148039,#148040,
#148041,#148042,#148043,#148044,#148045,#148046,#148047,#148048,#148049,
#148050,#148051,#148052,#148053,#148054,#148055,#148056,#148057,#148058),
(#148059,#148060,#148061,#148062,#148063,#148064,#148065,#148066,#148067,
#148068,#148069,#148070,#148071,#148072,#148073,#148074,#148075,#148076,
#148077,#148078)),.UNSPECIFIED.,.F.,.F.,.F.)
B_SPLINE_SURFACE_WITH_KNOTS((4,4),(4,1,1,1,1,1,1,1,1,1,1,1,1,1,1,1,1,4),
(0.,1.),(0.,0.0634473073458767,0.137474475480583,0.203439315591922,0.266070813426101,
0.333494447777073,0.401437472430427,0.464401084256882,0.51858368764375,
0.569769560865856,0.622221496328389,0.67514181525029,0.727526446084146,
0.778774499915783,0.832231436034466,0.891640084181608,0.951727885385323,
1.),.UNSPECIFIED.)
GEOMETRIC_REPRESENTATION_ITEM()
RATIONAL_B_SPLINE_SURFACE(((1.186029185783,1.186029185783,1.186029185783,
1.186029185783,1.186029185783,1.186029185783,1.186029185783,1.186029185783,
1.186029185783,1.186029185783,1.186029185783,1.186029185783,1.186029185783,
1.186029185783,1.186029185783,1.186029185783,1.186029185783,1.186029185783,
1.186029185783,1.186029185783),(0.9379902714058,0.9379902714058,0.9379902714058,
0.9379902714058,0.9379902714058,0.9379902714058,0.9379902714058,0.9379902714058,
0.9379902714058,0.9379902714058,0.9379902714058,0.9379902714058,0.9379902714058,
0.9379902714058,0.9379902714058,0.9379902714058,0.9379902714058,0.9379902714058,
0.9379902714058,0.9379902714058),(0.9379902714058,0.9379902714058,0.9379902714058,
0.9379902714058,0.9379902714058,0.9379902714058,0.9379902714058,0.9379902714058,
0.9379902714058,0.9379902714058,0.9379902714058,0.9379902714058,0.9379902714058,
0.9379902714058,0.9379902714058,0.9379902714058,0.9379902714058,0.9379902714058,
0.9379902714058,0.9379902714058),(1.186029185783,1.186029185783,1.186029185783,
1.186029185783,1.186029185783,1.186029185783,1.186029185783,1.186029185783,
1.186029185783,1.186029185783,1.186029185783,1.186029185783,1.186029185783,
1.186029185783,1.186029185783,1.186029185783,1.186029185783,1.186029185783,
1.186029185783,1.186029185783)))
REPRESENTATION_ITEM('')
SURFACE()
);
#2550=(
BOUNDED_SURFACE()
B_SPLINE_SURFACE(3,3,((#148208,#148209,#148210,#148211,#148212,#148213,
#148214,#148215,#148216,#148217),(#148218,#148219,#148220,#148221,#148222,
#148223,#148224,#148225,#148226,#148227),(#148228,#148229,#148230,#148231,
#148232,#148233,#148234,#148235,#148236,#148237),(#148238,#148239,#148240,
#148241,#148242,#148243,#148244,#148245,#148246,#148247)),.UNSPECIFIED.,
 .F.,.F.,.F.)
B_SPLINE_SURFACE_WITH_KNOTS((4,4),(4,1,1,1,1,1,1,4),(0.,1.),(0.,0.00515718315225492,
0.135375072417774,0.281251016648657,0.443276496267116,0.622074124477441,
0.818604636422717,1.),.UNSPECIFIED.)
GEOMETRIC_REPRESENTATION_ITEM()
RATIONAL_B_SPLINE_SURFACE(((1.54356298079,1.54356298079,1.54356298079,1.54356298079,
1.54356298079,1.54356298079,1.54356298079,1.54356298079,1.54356298079,1.54356298079),
(0.8188123397367,0.8188123397367,0.8188123397367,0.8188123397367,0.8188123397367,
0.8188123397367,0.8188123397367,0.8188123397367,0.8188123397367,0.8188123397367),
(0.8188123397367,0.8188123397367,0.8188123397367,0.8188123397367,0.8188123397367,
0.8188123397367,0.8188123397367,0.8188123397367,0.8188123397367,0.8188123397367),
(1.54356298079,1.54356298079,1.54356298079,1.54356298079,1.54356298079,
1.54356298079,1.54356298079,1.54356298079,1.54356298079,1.54356298079)))
REPRESENTATION_ITEM('')
SURFACE()
);
#2551=(
BOUNDED_SURFACE()
B_SPLINE_SURFACE(3,3,((#148418,#148419,#148420,#148421,#148422,#148423,
#148424,#148425),(#148426,#148427,#148428,#148429,#148430,#148431,#148432,
#148433),(#148434,#148435,#148436,#148437,#148438,#148439,#148440,#148441),
(#148442,#148443,#148444,#148445,#148446,#148447,#148448,#148449)),
 .UNSPECIFIED.,.F.,.F.,.F.)
B_SPLINE_SURFACE_WITH_KNOTS((4,4),(4,1,1,1,1,4),(0.,1.),(0.,0.018056873287542,
0.345151041851993,0.669351068431515,0.992791000152672,1.),.UNSPECIFIED.)
GEOMETRIC_REPRESENTATION_ITEM()
RATIONAL_B_SPLINE_SURFACE(((1.546274274408,1.546274274408,1.546274274408,
1.546274274408,1.546274274408,1.546274274408,1.546274274408,1.546274274408),
(0.8179085751973,0.8179085751973,0.8179085751973,0.8179085751973,0.8179085751973,
0.8179085751973,0.8179085751973,0.8179085751973),(0.8179085751973,0.8179085751973,
0.8179085751973,0.8179085751973,0.8179085751973,0.8179085751973,0.8179085751973,
0.8179085751973),(1.546274274408,1.546274274408,1.546274274408,1.546274274408,
1.546274274408,1.546274274408,1.546274274408,1.546274274408)))
REPRESENTATION_ITEM('')
SURFACE()
);
#2552=(
BOUNDED_SURFACE()
B_SPLINE_SURFACE(3,3,((#148459,#148460,#148461,#148462,#148463,#148464),
(#148465,#148466,#148467,#148468,#148469,#148470),(#148471,#148472,#148473,
#148474,#148475,#148476),(#148477,#148478,#148479,#148480,#148481,#148482)),
 .UNSPECIFIED.,.F.,.F.,.F.)
B_SPLINE_SURFACE_WITH_KNOTS((4,4),(4,1,1,4),(0.,1.),(0.,0.31080225069139,
0.761591972733954,1.),.UNSPECIFIED.)
GEOMETRIC_REPRESENTATION_ITEM()
RATIONAL_B_SPLINE_SURFACE(((1.187262794735,1.187262794735,1.187262794735,
1.187262794735,1.187262794735,1.187262794735),(0.9375790684218,0.9375790684218,
0.9375790684218,0.9375790684218,0.9375790684218,0.9375790684218),(0.9375790684218,
0.9375790684218,0.9375790684218,0.9375790684218,0.9375790684218,0.9375790684218),
(1.187262794735,1.187262794735,1.187262794735,1.187262794735,1.187262794735,
1.187262794735)))
REPRESENTATION_ITEM('')
SURFACE()
);
#2553=(
BOUNDED_SURFACE()
B_SPLINE_SURFACE(3,3,((#148542,#148543,#148544,#148545),(#148546,#148547,
#148548,#148549),(#148550,#148551,#148552,#148553),(#148554,#148555,#148556,
#148557)),.UNSPECIFIED.,.F.,.F.,.F.)
B_SPLINE_SURFACE_WITH_KNOTS((4,4),(4,4),(0.,1.),(0.,1.),.UNSPECIFIED.)
GEOMETRIC_REPRESENTATION_ITEM()
RATIONAL_B_SPLINE_SURFACE(((1.011180720188,0.8618966200521,0.8618556159516,
1.011057707886),(1.011640235655,0.8562207209891,0.8561780316645,1.011512167682),
(1.01213768218,0.8500763004794,0.8500317868227,1.01200414121),(1.012657343954,
0.8436574789567,0.8436110594958,1.012518085571)))
REPRESENTATION_ITEM('')
SURFACE()
);
#2554=(
BOUNDED_SURFACE()
B_SPLINE_SURFACE(3,3,((#148566,#148567,#148568,#148569),(#148570,#148571,
#148572,#148573),(#148574,#148575,#148576,#148577),(#148578,#148579,#148580,
#148581)),.UNSPECIFIED.,.F.,.F.,.F.)
B_SPLINE_SURFACE_WITH_KNOTS((4,4),(4,4),(0.,1.),(0.,1.),.UNSPECIFIED.)
GEOMETRIC_REPRESENTATION_ITEM()
RATIONAL_B_SPLINE_SURFACE(((1.010409839248,0.8769632993351,0.8769431939423,
1.010349523069),(1.01120923021,0.8675150817268,0.8674934324034,1.01114428224),
(1.012237722807,0.8553590500252,0.8553354142881,1.012166815596),(1.013244124764,
0.8434641135782,0.8434385340929,1.013167386308)))
REPRESENTATION_ITEM('')
SURFACE()
);
#2555=(
BOUNDED_SURFACE()
B_SPLINE_SURFACE(3,3,((#148995,#148996,#148997,#148998),(#148999,#149000,
#149001,#149002),(#149003,#149004,#149005,#149006),(#149007,#149008,#149009,
#149010)),.UNSPECIFIED.,.F.,.F.,.F.)
B_SPLINE_SURFACE_WITH_KNOTS((4,4),(4,4),(0.,1.),(0.,1.),.UNSPECIFIED.)
GEOMETRIC_REPRESENTATION_ITEM()
RATIONAL_B_SPLINE_SURFACE(((1.013235612141,0.8434362301637,0.8434372659622,
1.013238719536),(1.012229953762,0.8553321413794,0.8553330984767,1.012232825054),
(1.011193573923,0.867591456086,0.8675923320778,1.011196201899),(1.010402717632,
0.8769464780539,0.8769472921545,1.010405159934)))
REPRESENTATION_ITEM('')
SURFACE()
);
#2556=(
BOUNDED_SURFACE()
B_SPLINE_SURFACE(3,3,((#149118,#149119,#149120,#149121),(#149122,#149123,
#149124,#149125),(#149126,#149127,#149128,#149129),(#149130,#149131,#149132,
#149133)),.UNSPECIFIED.,.F.,.F.,.F.)
B_SPLINE_SURFACE_WITH_KNOTS((4,4),(4,4),(0.,1.),(0.,1.),.UNSPECIFIED.)
GEOMETRIC_REPRESENTATION_ITEM()
RATIONAL_B_SPLINE_SURFACE(((1.010400602958,0.8769605371814,0.8769497680482,
1.010368295558),(1.011189967337,0.8676223315438,0.8676107450762,1.011155207934),
(1.012219596932,0.8554417807797,0.8554291281992,1.012181639191),(1.01323329396,
0.8434497127943,0.8434360105978,1.013192187371)))
REPRESENTATION_ITEM('')
SURFACE()
);
#2557=(
BOUNDED_SURFACE()
B_SPLINE_SURFACE(3,3,((#149564,#149565,#149566,#149567),(#149568,#149569,
#149570,#149571),(#149572,#149573,#149574,#149575),(#149576,#149577,#149578,
#149579)),.UNSPECIFIED.,.F.,.F.,.F.)
B_SPLINE_SURFACE_WITH_KNOTS((4,4),(4,4),(0.,1.),(0.,1.),.UNSPECIFIED.)
GEOMETRIC_REPRESENTATION_ITEM()
RATIONAL_B_SPLINE_SURFACE(((1.013249647536,0.8434881174035,0.8434387387947,
1.01310151171),(1.012238397043,0.8554335459903,0.8553879360963,1.012101567361),
(1.0112206302,0.8674559491715,0.8674141322774,1.011095179517),(1.01041429526,
0.8769808062689,0.876941994413,1.010297859693)))
REPRESENTATION_ITEM('')
SURFACE()
);
#2558=(
BOUNDED_SURFACE()
B_SPLINE_SURFACE(3,3,((#149607,#149608,#149609,#149610),(#149611,#149612,
#149613,#149614),(#149615,#149616,#149617,#149618),(#149619,#149620,#149621,
#149622)),.UNSPECIFIED.,.F.,.F.,.F.)
B_SPLINE_SURFACE_WITH_KNOTS((4,4),(4,4),(0.,1.),(0.,1.),.UNSPECIFIED.)
GEOMETRIC_REPRESENTATION_ITEM()
RATIONAL_B_SPLINE_SURFACE(((1.012658416243,0.843652975638,0.8436063190053,
1.012518446345),(1.012143467457,0.850013227104,0.8499684684794,1.012009191583),
(1.011645124798,0.8561683724535,0.8561254506298,1.011516359326),(1.011180895029,
0.8619021816099,0.8618609708532,1.011057262759)))
REPRESENTATION_ITEM('')
SURFACE()
);
#2559=(
BOUNDED_SURFACE()
B_SPLINE_SURFACE(3,3,((#150260,#150261,#150262,#150263),(#150264,#150265,
#150266,#150267),(#150268,#150269,#150270,#150271),(#150272,#150273,#150274,
#150275)),.UNSPECIFIED.,.F.,.F.,.F.)
B_SPLINE_SURFACE_WITH_KNOTS((4,4),(4,4),(0.,1.),(0.,1.),.UNSPECIFIED.)
GEOMETRIC_REPRESENTATION_ITEM()
RATIONAL_B_SPLINE_SURFACE(((1.013249647536,0.8434881174035,0.8434387387948,
1.01310151171),(1.012238397043,0.8554335459903,0.8553879360964,1.012101567361),
(1.0112206302,0.8674559491716,0.8674141322775,1.011095179517),(1.01041429526,
0.876980806269,0.8769419944131,1.010297859693)))
REPRESENTATION_ITEM('')
SURFACE()
);
#2560=(
BOUNDED_SURFACE()
B_SPLINE_SURFACE(3,3,((#150602,#150603,#150604,#150605),(#150606,#150607,
#150608,#150609),(#150610,#150611,#150612,#150613),(#150614,#150615,#150616,
#150617)),.UNSPECIFIED.,.F.,.F.,.F.)
B_SPLINE_SURFACE_WITH_KNOTS((4,4),(4,4),(0.,1.),(0.,1.),.UNSPECIFIED.)
GEOMETRIC_REPRESENTATION_ITEM()
RATIONAL_B_SPLINE_SURFACE(((1.010400602958,0.8769605371815,0.8769497680483,
1.010368295558),(1.011189967337,0.8676223315439,0.8676107450763,1.011155207934),
(1.012219596932,0.8554417807799,0.8554291281992,1.01218163919),(1.01323329396,
0.8434497127945,0.8434360105979,1.01319218737)))
REPRESENTATION_ITEM('')
SURFACE()
);
#2561=(
BOUNDED_SURFACE()
B_SPLINE_SURFACE(3,3,((#150690,#150691,#150692,#150693),(#150694,#150695,
#150696,#150697),(#150698,#150699,#150700,#150701),(#150702,#150703,#150704,
#150705)),.UNSPECIFIED.,.F.,.F.,.F.)
B_SPLINE_SURFACE_WITH_KNOTS((4,4),(4,4),(0.,1.),(0.,1.),.UNSPECIFIED.)
GEOMETRIC_REPRESENTATION_ITEM()
RATIONAL_B_SPLINE_SURFACE(((1.011180720188,0.8618966200521,0.8618556159514,
1.011057707886),(1.011640235656,0.8562207209891,0.8561780316643,1.011512167682),
(1.012137682181,0.8500763004794,0.8500317868225,1.01200414121),(1.012657343955,
0.8436574789567,0.8436110594956,1.012518085571)))
REPRESENTATION_ITEM('')
SURFACE()
);
#2562=(
BOUNDED_SURFACE()
B_SPLINE_SURFACE(3,3,((#150815,#150816,#150817,#150818),(#150819,#150820,
#150821,#150822),(#150823,#150824,#150825,#150826),(#150827,#150828,#150829,
#150830)),.UNSPECIFIED.,.F.,.F.,.F.)
B_SPLINE_SURFACE_WITH_KNOTS((4,4),(4,4),(0.,1.),(0.,1.),.UNSPECIFIED.)
GEOMETRIC_REPRESENTATION_ITEM()
RATIONAL_B_SPLINE_SURFACE(((1.012658416244,0.8436529756379,0.843606319005,
1.012518446345),(1.012143467457,0.850013227104,0.8499684684792,1.012009191583),
(1.011645124798,0.8561683724535,0.8561254506296,1.011516359326),(1.011180895029,
0.8619021816099,0.861860970853,1.011057262759)))
REPRESENTATION_ITEM('')
SURFACE()
);
#2563=(
BOUNDED_SURFACE()
B_SPLINE_SURFACE(3,3,((#150837,#150838,#150839,#150840),(#150841,#150842,
#150843,#150844),(#150845,#150846,#150847,#150848),(#150849,#150850,#150851,
#150852)),.UNSPECIFIED.,.F.,.F.,.F.)
B_SPLINE_SURFACE_WITH_KNOTS((4,4),(4,4),(0.,1.),(0.,1.),.UNSPECIFIED.)
GEOMETRIC_REPRESENTATION_ITEM()
RATIONAL_B_SPLINE_SURFACE(((1.01323561214,0.8434362301639,0.8434372659623,
1.013238719536),(1.012229953762,0.8553321413796,0.8553330984767,1.012232825053),
(1.011193573923,0.8675914560862,0.8675923320778,1.011196201898),(1.010402717632,
0.8769464780541,0.8769472921545,1.010405159933)))
REPRESENTATION_ITEM('')
SURFACE()
);
#2564=(
BOUNDED_SURFACE()
B_SPLINE_SURFACE(3,3,((#151147,#151148,#151149,#151150),(#151151,#151152,
#151153,#151154),(#151155,#151156,#151157,#151158),(#151159,#151160,#151161,
#151162)),.UNSPECIFIED.,.F.,.F.,.F.)
B_SPLINE_SURFACE_WITH_KNOTS((4,4),(4,4),(0.,1.),(0.,1.),.UNSPECIFIED.)
GEOMETRIC_REPRESENTATION_ITEM()
RATIONAL_B_SPLINE_SURFACE(((1.010409839247,0.8769632993348,0.8769431939425,
1.01034952307),(1.011209230209,0.8675150817265,0.8674934324036,1.01114428224),
(1.012237722807,0.8553590500249,0.8553354142882,1.012166815597),(1.013244124763,
0.8434641135779,0.8434385340931,1.013167386309)))
REPRESENTATION_ITEM('')
SURFACE()
);
#2565=(
BOUNDED_SURFACE()
B_SPLINE_SURFACE(3,3,((#151686,#151687,#151688,#151689),(#151690,#151691,
#151692,#151693),(#151694,#151695,#151696,#151697),(#151698,#151699,#151700,
#151701)),.UNSPECIFIED.,.F.,.F.,.F.)
B_SPLINE_SURFACE_WITH_KNOTS((4,4),(4,4),(0.,1.),(0.,1.),.UNSPECIFIED.)
GEOMETRIC_REPRESENTATION_ITEM()
RATIONAL_B_SPLINE_SURFACE(((1.010417420083,0.8327746891999,0.8327405236387,
1.0103149234),(1.008972082557,0.855975924729,0.8559464993787,1.008883806506),
(1.007744072525,0.8756885174588,0.8756631195597,1.007667878827),(1.007061933964,
0.8866385254159,0.8866153646972,1.006992451808)))
REPRESENTATION_ITEM('')
SURFACE()
);
#2566=(
BOUNDED_SURFACE()
B_SPLINE_SURFACE(3,3,((#151933,#151934,#151935,#151936),(#151937,#151938,
#151939,#151940),(#151941,#151942,#151943,#151944),(#151945,#151946,#151947,
#151948)),.UNSPECIFIED.,.F.,.F.,.F.)
B_SPLINE_SURFACE_WITH_KNOTS((4,4),(4,4),(0.,1.),(0.,1.),.UNSPECIFIED.)
GEOMETRIC_REPRESENTATION_ITEM()
RATIONAL_B_SPLINE_SURFACE(((1.,1.,1.,1.),(0.9999761823555,1.000244831856,
1.000245109353,0.9999770148458),(1.001594007107,0.9836145123668,0.983595940764,
1.001538292299),(1.005023743582,0.9483587695743,0.9483002384861,1.004848150317)))
REPRESENTATION_ITEM('')
SURFACE()
);
#2567=(
BOUNDED_SURFACE()
B_SPLINE_SURFACE(3,3,((#153169,#153170,#153171,#153172),(#153173,#153174,
#153175,#153176),(#153177,#153178,#153179,#153180),(#153181,#153182,#153183,
#153184)),.UNSPECIFIED.,.F.,.F.,.F.)
B_SPLINE_SURFACE_WITH_KNOTS((4,4),(4,4),(0.,1.),(0.,1.),.UNSPECIFIED.)
GEOMETRIC_REPRESENTATION_ITEM()
RATIONAL_B_SPLINE_SURFACE(((1.007042941756,0.8866336160624,0.8866223630418,
1.007009182694),(1.00772434029,0.8756655162888,0.8756531745481,1.007687315068),
(1.008958893915,0.8557935813658,0.8557792670889,1.008915951085),(1.010389488669,
0.832766079544,0.8327494795017,1.010339688542)))
REPRESENTATION_ITEM('')
SURFACE()
);
#2568=(
BOUNDED_SURFACE()
B_SPLINE_SURFACE(3,3,((#153235,#153236,#153237,#153238),(#153239,#153240,
#153241,#153242),(#153243,#153244,#153245,#153246),(#153247,#153248,#153249,
#153250)),.UNSPECIFIED.,.F.,.F.,.F.)
B_SPLINE_SURFACE_WITH_KNOTS((4,4),(4,4),(0.,1.),(0.,1.),.UNSPECIFIED.)
GEOMETRIC_REPRESENTATION_ITEM()
RATIONAL_B_SPLINE_SURFACE(((1.,1.,1.,1.),(0.9999865607556,1.000144735869,
1.000144432799,0.999985651546),(1.001528719443,0.9835362368208,0.9835707111406,
1.001632142403),(1.004804655344,0.9482555755455,0.9483639258552,1.005129706273)))
REPRESENTATION_ITEM('')
SURFACE()
);
#2569=(
BOUNDED_SURFACE()
B_SPLINE_SURFACE(3,3,((#153265,#153266,#153267,#153268),(#153269,#153270,
#153271,#153272),(#153273,#153274,#153275,#153276),(#153277,#153278,#153279,
#153280)),.UNSPECIFIED.,.F.,.F.,.F.)
B_SPLINE_SURFACE_WITH_KNOTS((4,4),(4,4),(0.,1.),(0.,1.),.UNSPECIFIED.)
GEOMETRIC_REPRESENTATION_ITEM()
RATIONAL_B_SPLINE_SURFACE(((1.007751232385,0.8441927077371,0.8441759670975,
1.007701010467),(1.007532711944,0.8485851806412,0.8485689119488,1.007483905867),
(1.00730599456,0.8531424200671,0.8531266410251,1.007258657434),(1.00707431254,
0.8577994534751,0.8577841748059,1.007028476532)))
REPRESENTATION_ITEM('')
SURFACE()
);
#2570=(
BOUNDED_SURFACE()
B_SPLINE_SURFACE(3,3,((#153653,#153654,#153655,#153656),(#153657,#153658,
#153659,#153660),(#153661,#153662,#153663,#153664),(#153665,#153666,#153667,
#153668)),.UNSPECIFIED.,.F.,.F.,.F.)
B_SPLINE_SURFACE_WITH_KNOTS((4,4),(4,4),(0.,1.),(0.,1.),.UNSPECIFIED.)
GEOMETRIC_REPRESENTATION_ITEM()
RATIONAL_B_SPLINE_SURFACE(((1.007074258056,0.8577963970444,0.8577811874664,
1.007028629322),(1.007304418006,0.8531698236429,0.8531541192235,1.007257304748),
(1.007532328373,0.8485884703757,0.8485722759515,1.0074837451),(1.007750873574,
0.8441953715068,0.8441787072129,1.007700880692)))
REPRESENTATION_ITEM('')
SURFACE()
);
#2571=(
BOUNDED_SURFACE()
B_SPLINE_SURFACE(3,3,((#153847,#153848,#153849,#153850),(#153851,#153852,
#153853,#153854),(#153855,#153856,#153857,#153858),(#153859,#153860,#153861,
#153862)),.UNSPECIFIED.,.F.,.F.,.F.)
B_SPLINE_SURFACE_WITH_KNOTS((4,4),(4,4),(0.,1.),(0.,1.),.UNSPECIFIED.)
GEOMETRIC_REPRESENTATION_ITEM()
RATIONAL_B_SPLINE_SURFACE(((1.008509940924,0.8799663128153,0.8799421151717,
1.008437347994),(1.009061509065,0.8721863812946,0.8721606152913,1.008984211055),
(1.009661139189,0.8637285300159,0.8637010589907,1.009578726113),(1.010270334951,
0.8551357543165,0.8551065510698,1.010182725211)))
REPRESENTATION_ITEM('')
SURFACE()
);
#2572=(
BOUNDED_SURFACE()
B_SPLINE_SURFACE(3,3,((#154082,#154083,#154084,#154085),(#154086,#154087,
#154088,#154089),(#154090,#154091,#154092,#154093),(#154094,#154095,#154096,
#154097)),.UNSPECIFIED.,.F.,.F.,.F.)
B_SPLINE_SURFACE_WITH_KNOTS((4,4),(4,4),(0.,1.),(0.,1.),.UNSPECIFIED.)
GEOMETRIC_REPRESENTATION_ITEM()
RATIONAL_B_SPLINE_SURFACE(((1.010270521476,0.855133113183,0.8551039195422,
1.010182940553),(1.009662767308,0.863705555624,0.8636780895057,1.009580368953),
(1.009062759899,0.8721687291531,0.8721429685373,1.008985478052),(1.008509452897,
0.8799731880642,0.8799490002066,1.008436889324)))
REPRESENTATION_ITEM('')
SURFACE()
);
#2573=(
BOUNDED_SURFACE()
B_SPLINE_SURFACE(3,3,((#154178,#154179,#154180,#154181),(#154182,#154183,
#154184,#154185),(#154186,#154187,#154188,#154189),(#154190,#154191,#154192,
#154193)),.UNSPECIFIED.,.F.,.F.,.F.)
B_SPLINE_SURFACE_WITH_KNOTS((4,4),(4,4),(0.,1.),(0.,1.),.UNSPECIFIED.)
GEOMETRIC_REPRESENTATION_ITEM()
RATIONAL_B_SPLINE_SURFACE(((1.010390527686,0.8555764834497,0.8555484358643,
1.01030638493),(1.009638708354,0.8660264235414,0.8660004053733,1.009560653849),
(1.008824865687,0.8773384592094,0.8773146378808,1.008753401701),(1.008356067081,
0.8838545424531,0.8838319865722,1.008288399438)))
REPRESENTATION_ITEM('')
SURFACE()
);
#2574=(
BOUNDED_SURFACE()
B_SPLINE_SURFACE(3,3,((#154234,#154235,#154236,#154237),(#154238,#154239,
#154240,#154241),(#154242,#154243,#154244,#154245),(#154246,#154247,#154248,
#154249)),.UNSPECIFIED.,.F.,.F.,.F.)
B_SPLINE_SURFACE_WITH_KNOTS((4,4),(4,4),(0.,1.),(0.,1.),.UNSPECIFIED.)
GEOMETRIC_REPRESENTATION_ITEM()
RATIONAL_B_SPLINE_SURFACE(((1.008132395777,0.8893233508291,0.8892957763681,
1.008049672393),(1.008118961572,0.8895061816728,0.889478652763,1.008036374842),
(1.008279269408,0.8873244956603,0.8872964231958,1.008195052014),(1.008608872932,
0.8828388047798,0.8828096147308,1.008521302784)))
REPRESENTATION_ITEM('')
SURFACE()
);
#2575=(
BOUNDED_SURFACE()
B_SPLINE_SURFACE(3,3,((#154315,#154316,#154317,#154318),(#154319,#154320,
#154321,#154322),(#154323,#154324,#154325,#154326),(#154327,#154328,#154329,
#154330)),.UNSPECIFIED.,.F.,.F.,.F.)
B_SPLINE_SURFACE_WITH_KNOTS((4,4),(4,4),(0.,1.),(0.,1.),.UNSPECIFIED.)
GEOMETRIC_REPRESENTATION_ITEM()
RATIONAL_B_SPLINE_SURFACE(((1.008356913351,0.8838612339881,0.8838315240827,
1.008267783634),(1.008831957538,0.8772593890908,0.877227990342,1.008737761292),
(1.009633148898,0.8661249699641,0.8660907228766,1.009530407636),(1.010391558546,
0.8555851023152,0.8555481589836,1.010280728551)))
REPRESENTATION_ITEM('')
SURFACE()
);
#2576=(
BOUNDED_SURFACE()
B_SPLINE_SURFACE(3,3,((#154388,#154389,#154390,#154391),(#154392,#154393,
#154394,#154395),(#154396,#154397,#154398,#154399),(#154400,#154401,#154402,
#154403)),.UNSPECIFIED.,.F.,.F.,.F.)
B_SPLINE_SURFACE_WITH_KNOTS((4,4),(4,4),(0.,1.),(0.,1.),.UNSPECIFIED.)
GEOMETRIC_REPRESENTATION_ITEM()
RATIONAL_B_SPLINE_SURFACE(((1.008509940924,0.8799663128153,0.8799421151718,
1.008437347994),(1.009061509065,0.8721863812947,0.8721606152913,1.008984211055),
(1.009661139189,0.863728530016,0.8637010589907,1.009578726113),(1.010270334951,
0.8551357543165,0.8551065510698,1.010182725211)))
REPRESENTATION_ITEM('')
SURFACE()
);
#2577=(
BOUNDED_SURFACE()
B_SPLINE_SURFACE(3,3,((#154612,#154613,#154614,#154615),(#154616,#154617,
#154618,#154619),(#154620,#154621,#154622,#154623),(#154624,#154625,#154626,
#154627)),.UNSPECIFIED.,.F.,.F.,.F.)
B_SPLINE_SURFACE_WITH_KNOTS((4,4),(4,4),(0.,1.),(0.,1.),.UNSPECIFIED.)
GEOMETRIC_REPRESENTATION_ITEM()
RATIONAL_B_SPLINE_SURFACE(((1.010270521476,0.8551331131831,0.8551039195422,
1.010182940553),(1.009662767308,0.863705555624,0.8636780895057,1.009580368953),
(1.009062759899,0.8721687291531,0.8721429685373,1.008985478051),(1.008509452897,
0.8799731880642,0.8799490002065,1.008436889324)))
REPRESENTATION_ITEM('')
SURFACE()
);
#2578=(
BOUNDED_SURFACE()
B_SPLINE_SURFACE(3,3,((#154979,#154980,#154981,#154982,#154983,#154984),
(#154985,#154986,#154987,#154988,#154989,#154990),(#154991,#154992,#154993,
#154994,#154995,#154996),(#154997,#154998,#154999,#155000,#155001,#155002)),
 .UNSPECIFIED.,.F.,.F.,.F.)
B_SPLINE_SURFACE_WITH_KNOTS((4,4),(4,1,1,4),(0.,1.),(0.,0.380343625085213,
0.838543336801836,1.),.UNSPECIFIED.)
GEOMETRIC_REPRESENTATION_ITEM()
RATIONAL_B_SPLINE_SURFACE(((1.097838297065,1.097838297065,1.097838297065,
1.097838297065,1.097838297065,1.097838297065),(0.9673872343117,0.9673872343117,
0.9673872343117,0.9673872343117,0.9673872343117,0.9673872343117),(0.9673872343117,
0.9673872343117,0.9673872343117,0.9673872343117,0.9673872343117,0.9673872343117),
(1.097838297065,1.097838297065,1.097838297065,1.097838297065,1.097838297065,
1.097838297065)))
REPRESENTATION_ITEM('')
SURFACE()
);
#2579=(
BOUNDED_SURFACE()
B_SPLINE_SURFACE(3,3,((#155006,#155007,#155008,#155009),(#155010,#155011,
#155012,#155013),(#155014,#155015,#155016,#155017),(#155018,#155019,#155020,
#155021)),.UNSPECIFIED.,.F.,.F.,.F.)
B_SPLINE_SURFACE_WITH_KNOTS((4,4),(4,4),(0.,1.),(0.,1.),.UNSPECIFIED.)
GEOMETRIC_REPRESENTATION_ITEM()
RATIONAL_B_SPLINE_SURFACE(((1.,0.8932355607724,0.8836489357959,0.9712401250704),
(1.,0.8866507841162,0.8764728968729,0.9694663382699),(1.,0.8795406937193,
0.868724375078,0.9675510440761),(1.,0.8723221998445,0.8608577160073,0.9656065484883)))
REPRESENTATION_ITEM('')
SURFACE()
);
#2580=(
BOUNDED_SURFACE()
B_SPLINE_SURFACE(3,3,((#155029,#155030,#155031,#155032,#155033,#155034),
(#155035,#155036,#155037,#155038,#155039,#155040),(#155041,#155042,#155043,
#155044,#155045,#155046),(#155047,#155048,#155049,#155050,#155051,#155052)),
 .UNSPECIFIED.,.F.,.F.,.F.)
B_SPLINE_SURFACE_WITH_KNOTS((4,4),(4,1,1,4),(0.,1.),(0.,0.048792228532537,
0.607299349828058,1.),.UNSPECIFIED.)
GEOMETRIC_REPRESENTATION_ITEM()
RATIONAL_B_SPLINE_SURFACE(((1.227394348186,1.227394348186,1.227394348186,
1.227394348186,1.227394348186,1.227394348186),(0.9242018839379,0.9242018839379,
0.9242018839379,0.9242018839379,0.9242018839379,0.9242018839379),(0.9242018839379,
0.9242018839379,0.9242018839379,0.9242018839379,0.9242018839379,0.9242018839379),
(1.227394348186,1.227394348186,1.227394348186,1.227394348186,1.227394348186,
1.227394348186)))
REPRESENTATION_ITEM('')
SURFACE()
);
#2581=(
BOUNDED_SURFACE()
B_SPLINE_SURFACE(3,3,((#155055,#155056,#155057,#155058,#155059),(#155060,
#155061,#155062,#155063,#155064),(#155065,#155066,#155067,#155068,#155069),
(#155070,#155071,#155072,#155073,#155074)),.UNSPECIFIED.,.F.,.F.,.F.)
B_SPLINE_SURFACE_WITH_KNOTS((4,4),(4,1,4),(0.,1.),(0.,0.724305737931071,
1.),.UNSPECIFIED.)
GEOMETRIC_REPRESENTATION_ITEM()
RATIONAL_B_SPLINE_SURFACE(((1.071521449038,1.071521449038,1.071521449038,
1.071521449038,1.071521449038),(0.9761595169872,0.9761595169872,0.9761595169872,
0.9761595169872,0.9761595169872),(0.9761595169872,0.9761595169872,0.9761595169872,
0.9761595169872,0.9761595169872),(1.071521449038,1.071521449038,1.071521449038,
1.071521449038,1.071521449038)))
REPRESENTATION_ITEM('')
SURFACE()
);
#2582=(
BOUNDED_SURFACE()
B_SPLINE_SURFACE(3,3,((#155429,#155430,#155431,#155432,#155433),(#155434,
#155435,#155436,#155437,#155438),(#155439,#155440,#155441,#155442,#155443),
(#155444,#155445,#155446,#155447,#155448)),.UNSPECIFIED.,.F.,.F.,.F.)
B_SPLINE_SURFACE_WITH_KNOTS((4,4),(4,1,4),(0.,1.),(0.,0.294824597653245,
1.),.UNSPECIFIED.)
GEOMETRIC_REPRESENTATION_ITEM()
RATIONAL_B_SPLINE_SURFACE(((1.071512049094,1.071512049094,1.071512049094,
1.071512049094,1.071512049094),(0.9761626503021,0.9761626503021,0.9761626503021,
0.9761626503021,0.9761626503021),(0.9761626503021,0.9761626503021,0.9761626503021,
0.9761626503021,0.9761626503021),(1.071512049094,1.071512049094,1.071512049094,
1.071512049094,1.071512049094)))
REPRESENTATION_ITEM('')
SURFACE()
);
#2583=(
BOUNDED_SURFACE()
B_SPLINE_SURFACE(3,3,((#155459,#155460,#155461,#155462,#155463,#155464),
(#155465,#155466,#155467,#155468,#155469,#155470),(#155471,#155472,#155473,
#155474,#155475,#155476),(#155477,#155478,#155479,#155480,#155481,#155482)),
 .UNSPECIFIED.,.F.,.F.,.F.)
B_SPLINE_SURFACE_WITH_KNOTS((4,4),(4,1,1,4),(0.,1.),(0.,0.313954312956168,
0.656504260785239,1.),.UNSPECIFIED.)
GEOMETRIC_REPRESENTATION_ITEM()
RATIONAL_B_SPLINE_SURFACE(((1.097834676065,1.097834676065,1.097834676065,
1.097834676065,1.097834676065,1.097834676065),(0.9673884413118,0.9673884413118,
0.9673884413118,0.9673884413118,0.9673884413118,0.9673884413118),(0.9673884413118,
0.9673884413118,0.9673884413118,0.9673884413118,0.9673884413118,0.9673884413118),
(1.097834676065,1.097834676065,1.097834676065,1.097834676065,1.097834676065,
1.097834676065)))
REPRESENTATION_ITEM('')
SURFACE()
);
#2584=(
BOUNDED_SURFACE()
B_SPLINE_SURFACE(3,3,((#155501,#155502,#155503,#155504),(#155505,#155506,
#155507,#155508),(#155509,#155510,#155511,#155512),(#155513,#155514,#155515,
#155516)),.UNSPECIFIED.,.F.,.F.,.F.)
B_SPLINE_SURFACE_WITH_KNOTS((4,4),(4,4),(0.,1.),(0.,1.),.UNSPECIFIED.)
GEOMETRIC_REPRESENTATION_ITEM()
RATIONAL_B_SPLINE_SURFACE(((1.006012832044,0.8936858019092,0.8821005665622,
0.9712571260029),(1.006404088946,0.8867679030724,0.87442881276,0.9693868180087),
(1.00682837482,0.8792660117647,0.866109427854,0.9673586230877),(1.00725810598,
0.8716678411682,0.8576832719446,0.9653043983088)))
REPRESENTATION_ITEM('')
SURFACE()
);
#2585=(
BOUNDED_SURFACE()
B_SPLINE_SURFACE(3,3,((#155742,#155743,#155744,#155745,#155746,#155747),
(#155748,#155749,#155750,#155751,#155752,#155753),(#155754,#155755,#155756,
#155757,#155758,#155759),(#155760,#155761,#155762,#155763,#155764,#155765)),
 .UNSPECIFIED.,.F.,.F.,.F.)
B_SPLINE_SURFACE_WITH_KNOTS((4,4),(4,1,1,4),(0.,1.),(0.,0.305886131949221,
0.66938588399328,1.),.UNSPECIFIED.)
GEOMETRIC_REPRESENTATION_ITEM()
RATIONAL_B_SPLINE_SURFACE(((1.289432719618,1.289432719618,1.289432719618,
1.289432719618,1.289432719618,1.289432719618),(0.9035224267941,0.9035224267941,
0.9035224267941,0.9035224267941,0.9035224267941,0.9035224267941),(0.9035224267941,
0.9035224267941,0.9035224267941,0.9035224267941,0.9035224267941,0.9035224267941),
(1.289432719618,1.289432719618,1.289432719618,1.289432719618,1.289432719618,
1.289432719618)))
REPRESENTATION_ITEM('')
SURFACE()
);
#2586=(
BOUNDED_SURFACE()
B_SPLINE_SURFACE(3,3,((#155940,#155941,#155942,#155943,#155944,#155945,
#155946,#155947,#155948,#155949),(#155950,#155951,#155952,#155953,#155954,
#155955,#155956,#155957,#155958,#155959),(#155960,#155961,#155962,#155963,
#155964,#155965,#155966,#155967,#155968,#155969),(#155970,#155971,#155972,
#155973,#155974,#155975,#155976,#155977,#155978,#155979)),.UNSPECIFIED.,
 .F.,.F.,.F.)
B_SPLINE_SURFACE_WITH_KNOTS((4,4),(4,1,1,1,1,1,1,4),(0.,1.),(0.,0.00407814944862078,
0.20628932018066,0.424188287120768,0.621485607426675,0.792206769446229,
0.94764413919974,1.),.UNSPECIFIED.)
GEOMETRIC_REPRESENTATION_ITEM()
RATIONAL_B_SPLINE_SURFACE(((1.478660809567,1.478660809567,1.478660809567,
1.478660809567,1.478660809567,1.478660809567,1.478660809567,1.478660809567,
1.478660809567,1.478660809567),(0.840446396811,0.840446396811,0.840446396811,
0.840446396811,0.840446396811,0.840446396811,0.840446396811,0.840446396811,
0.840446396811,0.840446396811),(0.840446396811,0.840446396811,0.840446396811,
0.840446396811,0.840446396811,0.840446396811,0.840446396811,0.840446396811,
0.840446396811,0.840446396811),(1.478660809567,1.478660809567,1.478660809567,
1.478660809567,1.478660809567,1.478660809567,1.478660809567,1.478660809567,
1.478660809567,1.478660809567)))
REPRESENTATION_ITEM('')
SURFACE()
);
#2587=(
BOUNDED_SURFACE()
B_SPLINE_SURFACE(3,3,((#156025,#156026,#156027,#156028,#156029,#156030),
(#156031,#156032,#156033,#156034,#156035,#156036),(#156037,#156038,#156039,
#156040,#156041,#156042),(#156043,#156044,#156045,#156046,#156047,#156048)),
 .UNSPECIFIED.,.F.,.F.,.F.)
B_SPLINE_SURFACE_WITH_KNOTS((4,4),(4,1,1,4),(0.,1.),(0.,0.0564405642465865,
0.555415182027201,1.),.UNSPECIFIED.)
GEOMETRIC_REPRESENTATION_ITEM()
RATIONAL_B_SPLINE_SURFACE(((1.289342804764,1.289342804764,1.289342804764,
1.289342804764,1.289342804764,1.289342804764),(0.9035523984119,0.9035523984119,
0.9035523984119,0.9035523984119,0.9035523984119,0.9035523984119),(0.9035523984119,
0.9035523984119,0.9035523984119,0.9035523984119,0.9035523984119,0.9035523984119),
(1.289342804764,1.289342804764,1.289342804764,1.289342804764,1.289342804764,
1.289342804764)))
REPRESENTATION_ITEM('')
SURFACE()
);
#2588=(
BOUNDED_SURFACE()
B_SPLINE_SURFACE(3,3,((#156100,#156101,#156102,#156103,#156104,#156105,
#156106,#156107,#156108,#156109,#156110,#156111,#156112),(#156113,#156114,
#156115,#156116,#156117,#156118,#156119,#156120,#156121,#156122,#156123,
#156124,#156125),(#156126,#156127,#156128,#156129,#156130,#156131,#156132,
#156133,#156134,#156135,#156136,#156137,#156138),(#156139,#156140,#156141,
#156142,#156143,#156144,#156145,#156146,#156147,#156148,#156149,#156150,
#156151)),.UNSPECIFIED.,.F.,.F.,.F.)
B_SPLINE_SURFACE_WITH_KNOTS((4,4),(4,1,1,1,1,1,1,1,1,1,4),(0.,1.),(0.,0.0392950764212505,
0.11457615782262,0.1986935009597,0.291671866982471,0.394461000807193,0.508210508879651,
0.634800597831141,0.77592091339028,0.937113831440419,1.),.UNSPECIFIED.)
GEOMETRIC_REPRESENTATION_ITEM()
RATIONAL_B_SPLINE_SURFACE(((1.225183392518,1.225183392518,1.225183392518,
1.225183392518,1.225183392518,1.225183392518,1.225183392518,1.225183392518,
1.225183392518,1.225183392518,1.225183392518,1.225183392518,1.225183392518),
(0.9249388691606,0.9249388691606,0.9249388691606,0.9249388691606,0.9249388691606,
0.9249388691606,0.9249388691606,0.9249388691606,0.9249388691606,0.9249388691606,
0.9249388691606,0.9249388691606,0.9249388691606),(0.9249388691606,0.9249388691606,
0.9249388691606,0.9249388691606,0.9249388691606,0.9249388691606,0.9249388691606,
0.9249388691606,0.9249388691606,0.9249388691606,0.9249388691606,0.9249388691606,
0.9249388691606),(1.225183392518,1.225183392518,1.225183392518,1.225183392518,
1.225183392518,1.225183392518,1.225183392518,1.225183392518,1.225183392518,
1.225183392518,1.225183392518,1.225183392518,1.225183392518)))
REPRESENTATION_ITEM('')
SURFACE()
);
#2589=(
BOUNDED_SURFACE()
B_SPLINE_SURFACE(3,3,((#156160,#156161,#156162,#156163,#156164,#156165,
#156166,#156167,#156168,#156169,#156170,#156171,#156172,#156173,#156174,
#156175),(#156176,#156177,#156178,#156179,#156180,#156181,#156182,#156183,
#156184,#156185,#156186,#156187,#156188,#156189,#156190,#156191),(#156192,
#156193,#156194,#156195,#156196,#156197,#156198,#156199,#156200,#156201,
#156202,#156203,#156204,#156205,#156206,#156207),(#156208,#156209,#156210,
#156211,#156212,#156213,#156214,#156215,#156216,#156217,#156218,#156219,
#156220,#156221,#156222,#156223)),.UNSPECIFIED.,.F.,.F.,.F.)
B_SPLINE_SURFACE_WITH_KNOTS((4,4),(4,1,1,1,1,1,1,1,1,1,1,1,1,4),(0.,1.),
(0.,0.0186503236401621,0.0681861826858635,0.122274864726643,0.181134794327188,
0.244976288689619,0.314185121458223,0.389489559305443,0.47162927932211,
0.561313355930194,0.659220518921088,0.766025144246682,0.882569333512905,
1.),.UNSPECIFIED.)
GEOMETRIC_REPRESENTATION_ITEM()
RATIONAL_B_SPLINE_SURFACE(((1.02563369563202,1.02563369563202,1.02563369563202,
1.02563369563202,1.02563369563202,1.02563369563202,1.02563369563202,1.02563369563202,
1.02563369563202,1.02563369563202,1.02563369563202,1.02563369563202,1.02563369563202,
1.02563369563202,1.02563369563202,1.02563369563202),(1.00889094478308,1.00889094478308,
1.00889094478308,1.00889094478308,1.00889094478308,1.00889094478308,1.00889094478308,
1.00889094478308,1.00889094478308,1.00889094478308,1.00889094478308,1.00889094478308,
1.00889094478308,1.00889094478308,1.00889094478308,1.00889094478308),(1.00034988995606,
1.00034988995606,1.00034988995606,1.00034988995606,1.00034988995606,1.00034988995606,
1.00034988995606,1.00034988995606,1.00034988995606,1.00034988995606,1.00034988995606,
1.00034988995606,1.00034988995606,1.00034988995606,1.00034988995606,1.00034988995606),
(1.00001053115096,1.00001053115096,1.00001053115096,1.00001053115096,1.00001053115096,
1.00001053115096,1.00001053115096,1.00001053115096,1.00001053115096,1.00001053115096,
1.00001053115096,1.00001053115096,1.00001053115096,1.00001053115096,1.00001053115096,
1.00001053115096)))
REPRESENTATION_ITEM('')
SURFACE()
);
#2590=(
BOUNDED_SURFACE()
B_SPLINE_SURFACE(3,3,((#156226,#156227,#156228,#156229,#156230,#156231),
(#156232,#156233,#156234,#156235,#156236,#156237),(#156238,#156239,#156240,
#156241,#156242,#156243),(#156244,#156245,#156246,#156247,#156248,#156249)),
 .UNSPECIFIED.,.F.,.F.,.F.)
B_SPLINE_SURFACE_WITH_KNOTS((4,4),(4,1,1,4),(0.,1.),(0.,0.422272978047247,
0.965778076451582,1.),.UNSPECIFIED.)
GEOMETRIC_REPRESENTATION_ITEM()
RATIONAL_B_SPLINE_SURFACE(((1.227394458612,1.227394458612,1.227394458612,
1.227394458612,1.227394458612,1.227394458612),(0.9242018471293,0.9242018471293,
0.9242018471293,0.9242018471293,0.9242018471293,0.9242018471293),(0.9242018471293,
0.9242018471293,0.9242018471293,0.9242018471293,0.9242018471293,0.9242018471293),
(1.227394458612,1.227394458612,1.227394458612,1.227394458612,1.227394458612,
1.227394458612)))
REPRESENTATION_ITEM('')
SURFACE()
);
#2591=(
BOUNDED_SURFACE()
B_SPLINE_SURFACE(3,3,((#156259,#156260,#156261,#156262),(#156263,#156264,
#156265,#156266),(#156267,#156268,#156269,#156270),(#156271,#156272,#156273,
#156274)),.UNSPECIFIED.,.F.,.F.,.F.)
B_SPLINE_SURFACE_WITH_KNOTS((4,4),(4,4),(0.,1.),(0.,1.),.UNSPECIFIED.)
GEOMETRIC_REPRESENTATION_ITEM()
RATIONAL_B_SPLINE_SURFACE(((1.,0.8723221998447,0.8608577160075,0.9656065484883),
(1.,0.8795681296753,0.8687542745717,0.9675584346892),(1.,0.8866850345386,
0.8765102227196,0.9694755645429),(1.,0.8932587951734,0.8836742564673,0.9712463838817)))
REPRESENTATION_ITEM('')
SURFACE()
);
#2592=(
BOUNDED_SURFACE()
B_SPLINE_SURFACE(3,3,((#156276,#156277,#156278,#156279,#156280,#156281),
(#156282,#156283,#156284,#156285,#156286,#156287),(#156288,#156289,#156290,
#156291,#156292,#156293),(#156294,#156295,#156296,#156297,#156298,#156299)),
 .UNSPECIFIED.,.F.,.F.,.F.)
B_SPLINE_SURFACE_WITH_KNOTS((4,4),(4,1,1,4),(0.,1.),(0.,0.148909102857252,
0.594712811487906,1.),.UNSPECIFIED.)
GEOMETRIC_REPRESENTATION_ITEM()
RATIONAL_B_SPLINE_SURFACE(((1.097837209174,1.097837209174,1.097837209174,
1.097837209174,1.097837209174,1.097837209174),(0.9673875969419,0.9673875969419,
0.9673875969419,0.9673875969419,0.9673875969419,0.9673875969419),(0.9673875969419,
0.9673875969419,0.9673875969419,0.9673875969419,0.9673875969419,0.9673875969419),
(1.097837209174,1.097837209174,1.097837209174,1.097837209174,1.097837209174,
1.097837209174)))
REPRESENTATION_ITEM('')
SURFACE()
);
#2593=(
BOUNDED_SURFACE()
B_SPLINE_SURFACE(3,3,((#156303,#156304,#156305,#156306,#156307,#156308,
#156309,#156310,#156311,#156312,#156313),(#156314,#156315,#156316,#156317,
#156318,#156319,#156320,#156321,#156322,#156323,#156324),(#156325,#156326,
#156327,#156328,#156329,#156330,#156331,#156332,#156333,#156334,#156335),
(#156336,#156337,#156338,#156339,#156340,#156341,#156342,#156343,#156344,
#156345,#156346)),.UNSPECIFIED.,.F.,.F.,.F.)
B_SPLINE_SURFACE_WITH_KNOTS((4,4),(4,1,1,1,1,1,1,1,4),(0.,1.),(0.,0.0971862194548168,
0.209222881559132,0.334123661442517,0.473952177526924,0.627038064857414,
0.768578420172363,0.89296459914939,1.),.UNSPECIFIED.)
GEOMETRIC_REPRESENTATION_ITEM()
RATIONAL_B_SPLINE_SURFACE(((1.155039451457,1.155039451457,1.155039451457,
1.155039451457,1.155039451457,1.155039451457,1.155039451457,1.155039451457,
1.155039451457,1.155039451457,1.155039451457),(0.9483201828478,0.9483201828478,
0.9483201828478,0.9483201828478,0.9483201828478,0.9483201828478,0.9483201828478,
0.9483201828478,0.9483201828478,0.9483201828478,0.9483201828478),(0.9483201828478,
0.9483201828478,0.9483201828478,0.9483201828478,0.9483201828478,0.9483201828478,
0.9483201828478,0.9483201828478,0.9483201828478,0.9483201828478,0.9483201828478),
(1.155039451457,1.155039451457,1.155039451457,1.155039451457,1.155039451457,
1.155039451457,1.155039451457,1.155039451457,1.155039451457,1.155039451457,
1.155039451457)))
REPRESENTATION_ITEM('')
SURFACE()
);
#2594=(
BOUNDED_SURFACE()
B_SPLINE_SURFACE(3,3,((#156347,#156348,#156349,#156350,#156351,#156352,
#156353,#156354,#156355,#156356,#156357,#156358,#156359,#156360,#156361,
#156362,#156363,#156364,#156365,#156366,#156367,#156368,#156369,#156370,
#156371,#156372,#156373),(#156374,#156375,#156376,#156377,#156378,#156379,
#156380,#156381,#156382,#156383,#156384,#156385,#156386,#156387,#156388,
#156389,#156390,#156391,#156392,#156393,#156394,#156395,#156396,#156397,
#156398,#156399,#156400),(#156401,#156402,#156403,#156404,#156405,#156406,
#156407,#156408,#156409,#156410,#156411,#156412,#156413,#156414,#156415,
#156416,#156417,#156418,#156419,#156420,#156421,#156422,#156423,#156424,
#156425,#156426,#156427),(#156428,#156429,#156430,#156431,#156432,#156433,
#156434,#156435,#156436,#156437,#156438,#156439,#156440,#156441,#156442,
#156443,#156444,#156445,#156446,#156447,#156448,#156449,#156450,#156451,
#156452,#156453,#156454)),.UNSPECIFIED.,.F.,.F.,.F.)
B_SPLINE_SURFACE_WITH_KNOTS((4,4),(4,1,1,1,1,1,1,1,1,1,1,1,1,1,1,1,1,1,
1,1,1,1,1,1,4),(0.,1.),(0.,0.0133790708609555,0.0453329796627258,0.0807388003454147,
0.119840389730795,0.163002464189262,0.208524978632734,0.255893607883244,
0.304895617468101,0.352488053627177,0.399297953204769,0.44670582741306,
0.495059060800077,0.544318051162291,0.593648529667453,0.642243067504499,
0.69097472016604,0.740534478000938,0.788178737579007,0.834198656035311,
0.878796199450591,0.918860483820039,0.954457386043452,0.986512936409789,
1.),.UNSPECIFIED.)
GEOMETRIC_REPRESENTATION_ITEM()
RATIONAL_B_SPLINE_SURFACE(((1.261104736243,1.261104736243,1.261104736243,
1.261104736243,1.261104736243,1.261104736243,1.261104736243,1.261104736243,
1.261104736243,1.261104736243,1.261104736243,1.261104736243,1.261104736243,
1.261104736243,1.261104736243,1.261104736243,1.261104736243,1.261104736243,
1.261104736243,1.261104736243,1.261104736243,1.261104736243,1.261104736243,
1.261104736243,1.261104736243,1.261104736243,1.261104736243),(0.912965087919,
0.912965087919,0.912965087919,0.912965087919,0.912965087919,0.912965087919,
0.912965087919,0.912965087919,0.912965087919,0.912965087919,0.912965087919,
0.912965087919,0.912965087919,0.912965087919,0.912965087919,0.912965087919,
0.912965087919,0.912965087919,0.912965087919,0.912965087919,0.912965087919,
0.912965087919,0.912965087919,0.912965087919,0.912965087919,0.912965087919,
0.912965087919),(0.912965087919,0.912965087919,0.912965087919,0.912965087919,
0.912965087919,0.912965087919,0.912965087919,0.912965087919,0.912965087919,
0.912965087919,0.912965087919,0.912965087919,0.912965087919,0.912965087919,
0.912965087919,0.912965087919,0.912965087919,0.912965087919,0.912965087919,
0.912965087919,0.912965087919,0.912965087919,0.912965087919,0.912965087919,
0.912965087919,0.912965087919,0.912965087919),(1.261104736243,1.261104736243,
1.261104736243,1.261104736243,1.261104736243,1.261104736243,1.261104736243,
1.261104736243,1.261104736243,1.261104736243,1.261104736243,1.261104736243,
1.261104736243,1.261104736243,1.261104736243,1.261104736243,1.261104736243,
1.261104736243,1.261104736243,1.261104736243,1.261104736243,1.261104736243,
1.261104736243,1.261104736243,1.261104736243,1.261104736243,1.261104736243)))
REPRESENTATION_ITEM('')
SURFACE()
);
#2595=(
BOUNDED_SURFACE()
B_SPLINE_SURFACE(3,3,((#156684,#156685,#156686,#156687,#156688,#156689,
#156690,#156691,#156692,#156693,#156694,#156695,#156696,#156697,#156698,
#156699,#156700,#156701,#156702,#156703,#156704,#156705),(#156706,#156707,
#156708,#156709,#156710,#156711,#156712,#156713,#156714,#156715,#156716,
#156717,#156718,#156719,#156720,#156721,#156722,#156723,#156724,#156725,
#156726,#156727),(#156728,#156729,#156730,#156731,#156732,#156733,#156734,
#156735,#156736,#156737,#156738,#156739,#156740,#156741,#156742,#156743,
#156744,#156745,#156746,#156747,#156748,#156749),(#156750,#156751,#156752,
#156753,#156754,#156755,#156756,#156757,#156758,#156759,#156760,#156761,
#156762,#156763,#156764,#156765,#156766,#156767,#156768,#156769,#156770,
#156771)),.UNSPECIFIED.,.F.,.F.,.F.)
B_SPLINE_SURFACE_WITH_KNOTS((4,4),(4,1,1,1,1,1,1,1,1,1,1,1,1,1,1,1,1,1,
1,4),(0.,1.),(0.,0.00179852648676455,0.0684134361341035,0.138569448512766,
0.212049560253872,0.281023409010827,0.341871044231178,0.39611355557608,
0.444140369343199,0.487339341535663,0.530585789342856,0.575339323721559,
0.620494040055896,0.664485227938823,0.706756351680787,0.752682439877936,
0.80459823145977,0.863065026247903,0.928980423200659,1.),.UNSPECIFIED.)
GEOMETRIC_REPRESENTATION_ITEM()
RATIONAL_B_SPLINE_SURFACE(((1.255321138723,1.255321138723,1.255321138723,
1.255321138723,1.255321138723,1.255321138723,1.255321138723,1.255321138723,
1.255321138723,1.255321138723,1.255321138723,1.255321138723,1.255321138723,
1.255321138723,1.255321138723,1.255321138723,1.255321138723,1.255321138723,
1.255321138723,1.255321138723,1.255321138723,1.255321138723),(0.914892953759,
0.914892953759,0.914892953759,0.914892953759,0.914892953759,0.914892953759,
0.914892953759,0.914892953759,0.914892953759,0.914892953759,0.914892953759,
0.914892953759,0.914892953759,0.914892953759,0.914892953759,0.914892953759,
0.914892953759,0.914892953759,0.914892953759,0.914892953759,0.914892953759,
0.914892953759),(0.914892953759,0.914892953759,0.914892953759,0.914892953759,
0.914892953759,0.914892953759,0.914892953759,0.914892953759,0.914892953759,
0.914892953759,0.914892953759,0.914892953759,0.914892953759,0.914892953759,
0.914892953759,0.914892953759,0.914892953759,0.914892953759,0.914892953759,
0.914892953759,0.914892953759,0.914892953759),(1.255321138723,1.255321138723,
1.255321138723,1.255321138723,1.255321138723,1.255321138723,1.255321138723,
1.255321138723,1.255321138723,1.255321138723,1.255321138723,1.255321138723,
1.255321138723,1.255321138723,1.255321138723,1.255321138723,1.255321138723,
1.255321138723,1.255321138723,1.255321138723,1.255321138723,1.255321138723)))
REPRESENTATION_ITEM('')
SURFACE()
);
#2596=(
BOUNDED_SURFACE()
B_SPLINE_SURFACE(3,3,((#156821,#156822,#156823,#156824,#156825,#156826,
#156827,#156828,#156829,#156830,#156831),(#156832,#156833,#156834,#156835,
#156836,#156837,#156838,#156839,#156840,#156841,#156842),(#156843,#156844,
#156845,#156846,#156847,#156848,#156849,#156850,#156851,#156852,#156853),
(#156854,#156855,#156856,#156857,#156858,#156859,#156860,#156861,#156862,
#156863,#156864)),.UNSPECIFIED.,.F.,.F.,.F.)
B_SPLINE_SURFACE_WITH_KNOTS((4,4),(4,1,1,1,1,1,1,1,4),(0.,1.),(0.,0.0185293626863753,
0.146534230162969,0.288917342557819,0.446398650999111,0.612297392457084,
0.77680939958634,0.936363164269577,1.),.UNSPECIFIED.)
GEOMETRIC_REPRESENTATION_ITEM()
RATIONAL_B_SPLINE_SURFACE(((1.366220667592,1.366220667592,1.366220667592,
1.366220667592,1.366220667592,1.366220667592,1.366220667592,1.366220667592,
1.366220667592,1.366220667592,1.366220667592),(0.8779264441361,0.8779264441361,
0.8779264441361,0.8779264441361,0.8779264441361,0.8779264441361,0.8779264441361,
0.8779264441361,0.8779264441361,0.8779264441361,0.8779264441361),(0.8779264441361,
0.8779264441361,0.8779264441361,0.8779264441361,0.8779264441361,0.8779264441361,
0.8779264441361,0.8779264441361,0.8779264441361,0.8779264441361,0.8779264441361),
(1.366220667592,1.366220667592,1.366220667592,1.366220667592,1.366220667592,
1.366220667592,1.366220667592,1.366220667592,1.366220667592,1.366220667592,
1.366220667592)))
REPRESENTATION_ITEM('')
SURFACE()
);
#2597=(
BOUNDED_SURFACE()
B_SPLINE_SURFACE(2,2,((#157031,#157032,#157033),(#157034,#157035,#157036),
(#157037,#157038,#157039),(#157040,#157041,#157042),(#157043,#157044,#157045)),
 .UNSPECIFIED.,.F.,.F.,.F.)
B_SPLINE_SURFACE_WITH_KNOTS((3,2,3),(3,3),(5.17583184338056E-13,0.78540290201525,
1.57080580402998),(-0.715662500296765,0.715662500296765),.UNSPECIFIED.)
GEOMETRIC_REPRESENTATION_ITEM()
RATIONAL_B_SPLINE_SURFACE(((1.,0.754658728802486,1.),(0.923878625813598,
0.697213069324277,0.923878625813598),(1.,0.754658728802486,1.),(0.923878625813414,
0.697213069324138,0.923878625813414),(1.,0.754658728802486,1.)))
REPRESENTATION_ITEM('')
SURFACE()
);
#2598=(
BOUNDED_SURFACE()
B_SPLINE_SURFACE(3,3,((#157065,#157066,#157067,#157068,#157069,#157070,
#157071,#157072,#157073,#157074),(#157075,#157076,#157077,#157078,#157079,
#157080,#157081,#157082,#157083,#157084),(#157085,#157086,#157087,#157088,
#157089,#157090,#157091,#157092,#157093,#157094),(#157095,#157096,#157097,
#157098,#157099,#157100,#157101,#157102,#157103,#157104)),.UNSPECIFIED.,
 .F.,.F.,.F.)
B_SPLINE_SURFACE_WITH_KNOTS((4,4),(4,1,1,1,1,1,1,4),(0.,1.),(0.,0.0918892366120133,
0.277217977594551,0.468937582524931,0.657129296434973,0.829336528589428,
0.981429132764797,1.),.UNSPECIFIED.)
GEOMETRIC_REPRESENTATION_ITEM()
RATIONAL_B_SPLINE_SURFACE(((1.367123648823,1.367123648823,1.367123648823,
1.367123648823,1.367123648823,1.367123648823,1.367123648823,1.367123648823,
1.367123648823,1.367123648823),(0.8776254503924,0.8776254503924,0.8776254503924,
0.8776254503924,0.8776254503924,0.8776254503924,0.8776254503924,0.8776254503924,
0.8776254503924,0.8776254503924),(0.8776254503924,0.8776254503924,0.8776254503924,
0.8776254503924,0.8776254503924,0.8776254503924,0.8776254503924,0.8776254503924,
0.8776254503924,0.8776254503924),(1.367123648823,1.367123648823,1.367123648823,
1.367123648823,1.367123648823,1.367123648823,1.367123648823,1.367123648823,
1.367123648823,1.367123648823)))
REPRESENTATION_ITEM('')
SURFACE()
);
#2599=(
BOUNDED_SURFACE()
B_SPLINE_SURFACE(2,2,((#157106,#157107,#157108),(#157109,#157110,#157111),
(#157112,#157113,#157114),(#157115,#157116,#157117),(#157118,#157119,#157120)),
 .UNSPECIFIED.,.F.,.F.,.F.)
B_SPLINE_SURFACE_WITH_KNOTS((3,2,3),(3,3),(-1.57080581687637,-0.785402908437997,
3.76899203758591E-13),(-0.715662500299626,0.715662500299626),
 .UNSPECIFIED.)
GEOMETRIC_REPRESENTATION_ITEM()
RATIONAL_B_SPLINE_SURFACE(((1.,0.754658728800609,1.),(0.923878624584496,
0.69721306839499,0.923878624584496),(1.,0.754658728800609,1.),(0.923878624584344,
0.697213068394876,0.923878624584344),(1.,0.754658728800609,1.)))
REPRESENTATION_ITEM('')
SURFACE()
);
#2600=(
BOUNDED_SURFACE()
B_SPLINE_SURFACE(3,3,((#157126,#157127,#157128,#157129,#157130,#157131,
#157132,#157133,#157134,#157135,#157136,#157137,#157138,#157139,#157140,
#157141,#157142,#157143,#157144,#157145,#157146,#157147,#157148,#157149,
#157150,#157151,#157152,#157153,#157154,#157155,#157156,#157157),(#157158,
#157159,#157160,#157161,#157162,#157163,#157164,#157165,#157166,#157167,
#157168,#157169,#157170,#157171,#157172,#157173,#157174,#157175,#157176,
#157177,#157178,#157179,#157180,#157181,#157182,#157183,#157184,#157185,
#157186,#157187,#157188,#157189),(#157190,#157191,#157192,#157193,#157194,
#157195,#157196,#157197,#157198,#157199,#157200,#157201,#157202,#157203,
#157204,#157205,#157206,#157207,#157208,#157209,#157210,#157211,#157212,
#157213,#157214,#157215,#157216,#157217,#157218,#157219,#157220,#157221),
(#157222,#157223,#157224,#157225,#157226,#157227,#157228,#157229,#157230,
#157231,#157232,#157233,#157234,#157235,#157236,#157237,#157238,#157239,
#157240,#157241,#157242,#157243,#157244,#157245,#157246,#157247,#157248,
#157249,#157250,#157251,#157252,#157253)),.UNSPECIFIED.,.F.,.F.,.F.)
B_SPLINE_SURFACE_WITH_KNOTS((4,4),(4,1,1,1,1,1,1,1,1,1,1,1,1,1,1,1,1,1,
1,1,1,1,1,1,1,1,1,1,1,4),(0.,1.),(0.,0.022976135501356,0.0695598229222624,
0.121692586326365,0.178900115493456,0.240694690781884,0.30610330870727,
0.373471747186216,0.440686754218971,0.501942919989092,0.555359583174251,
0.602908392139393,0.6457512695131,0.684704926133708,0.720523567288128,0.753147804956652,
0.782813392672435,0.809944931270991,0.834840676715807,0.857737986813372,
0.878754366287739,0.898008224113769,0.915646640643435,0.931806303451426,
0.946546912483728,0.959896478233652,0.971957268367346,0.982857205461103,
0.992730071740333,1.),.UNSPECIFIED.)
GEOMETRIC_REPRESENTATION_ITEM()
RATIONAL_B_SPLINE_SURFACE(((1.777949029729,1.777949029729,1.777949029729,
1.777949029729,1.777949029729,1.777949029729,1.777949029729,1.777949029729,
1.777949029729,1.777949029729,1.777949029729,1.777949029729,1.777949029729,
1.777949029729,1.777949029729,1.777949029729,1.777949029729,1.777949029729,
1.777949029729,1.777949029729,1.777949029729,1.777949029729,1.777949029729,
1.777949029729,1.777949029729,1.777949029729,1.777949029729,1.777949029729,
1.777949029729,1.777949029729,1.777949029729,1.777949029729),(0.740683656757,
0.740683656757,0.740683656757,0.740683656757,0.740683656757,0.740683656757,
0.740683656757,0.740683656757,0.740683656757,0.740683656757,0.740683656757,
0.740683656757,0.740683656757,0.740683656757,0.740683656757,0.740683656757,
0.740683656757,0.740683656757,0.740683656757,0.740683656757,0.740683656757,
0.740683656757,0.740683656757,0.740683656757,0.740683656757,0.740683656757,
0.740683656757,0.740683656757,0.740683656757,0.740683656757,0.740683656757,
0.740683656757),(0.740683656757,0.740683656757,0.740683656757,0.740683656757,
0.740683656757,0.740683656757,0.740683656757,0.740683656757,0.740683656757,
0.740683656757,0.740683656757,0.740683656757,0.740683656757,0.740683656757,
0.740683656757,0.740683656757,0.740683656757,0.740683656757,0.740683656757,
0.740683656757,0.740683656757,0.740683656757,0.740683656757,0.740683656757,
0.740683656757,0.740683656757,0.740683656757,0.740683656757,0.740683656757,
0.740683656757,0.740683656757,0.740683656757),(1.777949029729,1.777949029729,
1.777949029729,1.777949029729,1.777949029729,1.777949029729,1.777949029729,
1.777949029729,1.777949029729,1.777949029729,1.777949029729,1.777949029729,
1.777949029729,1.777949029729,1.777949029729,1.777949029729,1.777949029729,
1.777949029729,1.777949029729,1.777949029729,1.777949029729,1.777949029729,
1.777949029729,1.777949029729,1.777949029729,1.777949029729,1.777949029729,
1.777949029729,1.777949029729,1.777949029729,1.777949029729,1.777949029729)))
REPRESENTATION_ITEM('')
SURFACE()
);
#2601=(
BOUNDED_SURFACE()
B_SPLINE_SURFACE(3,3,((#157306,#157307,#157308,#157309,#157310,#157311,
#157312,#157313,#157314,#157315,#157316,#157317,#157318,#157319),(#157320,
#157321,#157322,#157323,#157324,#157325,#157326,#157327,#157328,#157329,
#157330,#157331,#157332,#157333),(#157334,#157335,#157336,#157337,#157338,
#157339,#157340,#157341,#157342,#157343,#157344,#157345,#157346,#157347),
(#157348,#157349,#157350,#157351,#157352,#157353,#157354,#157355,#157356,
#157357,#157358,#157359,#157360,#157361)),.UNSPECIFIED.,.F.,.F.,.F.)
B_SPLINE_SURFACE_WITH_KNOTS((4,4),(4,1,1,1,1,1,1,1,1,1,1,4),(0.,1.),(0.,
0.025958376473271,0.179859171762141,0.318182203672271,0.441108132212019,
0.551634708740777,0.651710515506557,0.743010369069283,0.826230829945666,
0.901572688650554,0.970015580606343,1.),.UNSPECIFIED.)
GEOMETRIC_REPRESENTATION_ITEM()
RATIONAL_B_SPLINE_SURFACE(((1.116719050321,1.116719050321,1.116719050321,
1.116719050321,1.116719050321,1.116719050321,1.116719050321,1.116719050321,
1.116719050321,1.116719050321,1.116719050321,1.116719050321,1.116719050321,
1.116719050321),(0.961093649893,0.961093649893,0.961093649893,0.961093649893,
0.961093649893,0.961093649893,0.961093649893,0.961093649893,0.961093649893,
0.961093649893,0.961093649893,0.961093649893,0.961093649893,0.961093649893),
(0.961093649893,0.961093649893,0.961093649893,0.961093649893,0.961093649893,
0.961093649893,0.961093649893,0.961093649893,0.961093649893,0.961093649893,
0.961093649893,0.961093649893,0.961093649893,0.961093649893),(1.116719050321,
1.116719050321,1.116719050321,1.116719050321,1.116719050321,1.116719050321,
1.116719050321,1.116719050321,1.116719050321,1.116719050321,1.116719050321,
1.116719050321,1.116719050321,1.116719050321)))
REPRESENTATION_ITEM('')
SURFACE()
);
#2602=(
BOUNDED_SURFACE()
B_SPLINE_SURFACE(3,3,((#157370,#157371,#157372,#157373),(#157374,#157375,
#157376,#157377),(#157378,#157379,#157380,#157381),(#157382,#157383,#157384,
#157385)),.UNSPECIFIED.,.F.,.F.,.F.)
B_SPLINE_SURFACE_WITH_KNOTS((4,4),(4,4),(0.,1.),(0.,1.),.UNSPECIFIED.)
GEOMETRIC_REPRESENTATION_ITEM()
RATIONAL_B_SPLINE_SURFACE(((1.117354081969,1.117354081969,1.117354081969,
1.117354081969),(0.9608819726769,0.9608819726769,0.9608819726769,0.9608819726769),
(0.9608819726769,0.9608819726769,0.9608819726769,0.9608819726769),(1.117354081969,
1.117354081969,1.117354081969,1.117354081969)))
REPRESENTATION_ITEM('')
SURFACE()
);
#2603=(
BOUNDED_SURFACE()
B_SPLINE_SURFACE(3,3,((#157392,#157393,#157394,#157395,#157396,#157397),
(#157398,#157399,#157400,#157401,#157402,#157403),(#157404,#157405,#157406,
#157407,#157408,#157409),(#157410,#157411,#157412,#157413,#157414,#157415)),
 .UNSPECIFIED.,.F.,.F.,.F.)
B_SPLINE_SURFACE_WITH_KNOTS((4,4),(4,1,1,4),(0.,1.),(0.,0.131075263192113,
0.624369556415442,1.),.UNSPECIFIED.)
GEOMETRIC_REPRESENTATION_ITEM()
RATIONAL_B_SPLINE_SURFACE(((1.187262830589,1.187262830589,1.187262830589,
1.187262830589,1.187262830589,1.187262830589),(0.9375790564704,0.9375790564704,
0.9375790564704,0.9375790564704,0.9375790564704,0.9375790564704),(0.9375790564704,
0.9375790564704,0.9375790564704,0.9375790564704,0.9375790564704,0.9375790564704),
(1.187262830589,1.187262830589,1.187262830589,1.187262830589,1.187262830589,
1.187262830589)))
REPRESENTATION_ITEM('')
SURFACE()
);
#2604=(
BOUNDED_SURFACE()
B_SPLINE_SURFACE(3,3,((#157417,#157418,#157419,#157420,#157421,#157422,
#157423,#157424),(#157425,#157426,#157427,#157428,#157429,#157430,#157431,
#157432),(#157433,#157434,#157435,#157436,#157437,#157438,#157439,#157440),
(#157441,#157442,#157443,#157444,#157445,#157446,#157447,#157448)),
 .UNSPECIFIED.,.F.,.F.,.F.)
B_SPLINE_SURFACE_WITH_KNOTS((4,4),(4,1,1,1,1,4),(0.,1.),(0.,0.0123570293092027,
0.272651924312037,0.542654748910529,0.824134468225905,1.),.UNSPECIFIED.)
GEOMETRIC_REPRESENTATION_ITEM()
RATIONAL_B_SPLINE_SURFACE(((1.546267699181,1.546267699181,1.546267699181,
1.546267699181,1.546267699181,1.546267699181,1.546267699181,1.546267699181),
(0.8179107669398,0.8179107669398,0.8179107669398,0.8179107669398,0.8179107669398,
0.8179107669398,0.8179107669398,0.8179107669398),(0.8179107669398,0.8179107669398,
0.8179107669398,0.8179107669398,0.8179107669398,0.8179107669398,0.8179107669398,
0.8179107669398),(1.546267699181,1.546267699181,1.546267699181,1.546267699181,
1.546267699181,1.546267699181,1.546267699181,1.546267699181)))
REPRESENTATION_ITEM('')
SURFACE()
);
#2605=(
BOUNDED_SURFACE()
B_SPLINE_SURFACE(3,3,((#157456,#157457,#157458,#157459,#157460,#157461,
#157462,#157463,#157464,#157465),(#157466,#157467,#157468,#157469,#157470,
#157471,#157472,#157473,#157474,#157475),(#157476,#157477,#157478,#157479,
#157480,#157481,#157482,#157483,#157484,#157485),(#157486,#157487,#157488,
#157489,#157490,#157491,#157492,#157493,#157494,#157495)),.UNSPECIFIED.,
 .F.,.F.,.F.)
B_SPLINE_SURFACE_WITH_KNOTS((4,4),(4,1,1,1,1,1,1,4),(0.,1.),(0.,0.0912471898348692,
0.237776614561094,0.390267328672513,0.55260360700317,0.728899321816043,
0.920187339345513,1.),.UNSPECIFIED.)
GEOMETRIC_REPRESENTATION_ITEM()
RATIONAL_B_SPLINE_SURFACE(((1.289680320997,1.289680320997,1.289680320997,
1.289680320997,1.289680320997,1.289680320997,1.289680320997,1.289680320997,
1.289680320997,1.289680320997),(0.9034398930009,0.9034398930009,0.9034398930009,
0.9034398930009,0.9034398930009,0.9034398930009,0.9034398930009,0.9034398930009,
0.9034398930009,0.9034398930009),(0.9034398930009,0.9034398930009,0.9034398930009,
0.9034398930009,0.9034398930009,0.9034398930009,0.9034398930009,0.9034398930009,
0.9034398930009,0.9034398930009),(1.289680320997,1.289680320997,1.289680320997,
1.289680320997,1.289680320997,1.289680320997,1.289680320997,1.289680320997,
1.289680320997,1.289680320997)))
REPRESENTATION_ITEM('')
SURFACE()
);
#2606=(
BOUNDED_SURFACE()
B_SPLINE_SURFACE(3,3,((#157621,#157622,#157623,#157624,#157625,#157626,
#157627,#157628,#157629,#157630,#157631,#157632,#157633,#157634,#157635,
#157636,#157637,#157638,#157639,#157640,#157641),(#157642,#157643,#157644,
#157645,#157646,#157647,#157648,#157649,#157650,#157651,#157652,#157653,
#157654,#157655,#157656,#157657,#157658,#157659,#157660,#157661,#157662),
(#157663,#157664,#157665,#157666,#157667,#157668,#157669,#157670,#157671,
#157672,#157673,#157674,#157675,#157676,#157677,#157678,#157679,#157680,
#157681,#157682,#157683),(#157684,#157685,#157686,#157687,#157688,#157689,
#157690,#157691,#157692,#157693,#157694,#157695,#157696,#157697,#157698,
#157699,#157700,#157701,#157702,#157703,#157704)),.UNSPECIFIED.,.F.,.F.,
 .F.)
B_SPLINE_SURFACE_WITH_KNOTS((4,4),(4,1,1,1,1,1,1,1,1,1,1,1,1,1,1,1,1,1,
4),(0.,1.),(0.,0.0546624749950295,0.160757685575355,0.256729617165409,0.343735196321369,
0.422731592898268,0.494638559250071,0.560248549174547,0.620252323655667,
0.6753431121518,0.726138185608107,0.772911121896331,0.815853204906754,0.855219379345603,
0.891312858927466,0.92449329904142,0.955123399607878,0.983429063756098,
1.),.UNSPECIFIED.)
GEOMETRIC_REPRESENTATION_ITEM()
RATIONAL_B_SPLINE_SURFACE(((1.00131522864575,1.00131522864575,1.00131522864575,
1.00131522864575,1.00131522864575,1.00131522864575,1.00131522864575,1.00131522864575,
1.00131522864575,1.00131522864575,1.00131522864575,1.00131522864575,1.00131522864575,
1.00131522864575,1.00131522864575,1.00131522864575,1.00131522864575,1.00131522864575,
1.00131522864575,1.00131522864575,1.00131522864575),(0.992301531113087,
0.992301531113087,0.992301531113087,0.992301531113087,0.992301531113087,
0.992301531113087,0.992301531113087,0.992301531113087,0.992301531113087,
0.992301531113087,0.992301531113087,0.992301531113087,0.992301531113087,
0.992301531113087,0.992301531113087,0.992301531113087,0.992301531113087,
0.992301531113087,0.992301531113087,0.992301531113087,0.992301531113087),
(1.02961822457532,1.02961822457532,1.02961822457532,1.02961822457532,1.02961822457532,
1.02961822457532,1.02961822457532,1.02961822457532,1.02961822457532,1.02961822457532,
1.02961822457532,1.02961822457532,1.02961822457532,1.02961822457532,1.02961822457532,
1.02961822457532,1.02961822457532,1.02961822457532,1.02961822457532,1.02961822457532,
1.02961822457532),(1.11326530903245,1.11326530903245,1.11326530903245,1.11326530903245,
1.11326530903245,1.11326530903245,1.11326530903245,1.11326530903245,1.11326530903245,
1.11326530903245,1.11326530903245,1.11326530903245,1.11326530903245,1.11326530903245,
1.11326530903245,1.11326530903245,1.11326530903245,1.11326530903245,1.11326530903245,
1.11326530903245,1.11326530903245)))
REPRESENTATION_ITEM('')
SURFACE()
);
#2607=(
BOUNDED_SURFACE()
B_SPLINE_SURFACE(3,3,((#157707,#157708,#157709,#157710,#157711,#157712,
#157713,#157714,#157715,#157716),(#157717,#157718,#157719,#157720,#157721,
#157722,#157723,#157724,#157725,#157726),(#157727,#157728,#157729,#157730,
#157731,#157732,#157733,#157734,#157735,#157736),(#157737,#157738,#157739,
#157740,#157741,#157742,#157743,#157744,#157745,#157746)),.UNSPECIFIED.,
 .F.,.F.,.F.)
B_SPLINE_SURFACE_WITH_KNOTS((4,4),(4,1,1,1,1,1,1,4),(0.,1.),(0.,0.100889583131889,
0.31750308787695,0.513050576898124,0.689879175955297,0.85048492065676,0.997565294800237,
1.),.UNSPECIFIED.)
GEOMETRIC_REPRESENTATION_ITEM()
RATIONAL_B_SPLINE_SURFACE(((1.365423084219,1.365423084219,1.365423084219,
1.365423084219,1.365423084219,1.365423084219,1.365423084219,1.365423084219,
1.365423084219,1.365423084219),(0.8781923052603,0.8781923052603,0.8781923052603,
0.8781923052603,0.8781923052603,0.8781923052603,0.8781923052603,0.8781923052603,
0.8781923052603,0.8781923052603),(0.8781923052603,0.8781923052603,0.8781923052603,
0.8781923052603,0.8781923052603,0.8781923052603,0.8781923052603,0.8781923052603,
0.8781923052603,0.8781923052603),(1.365423084219,1.365423084219,1.365423084219,
1.365423084219,1.365423084219,1.365423084219,1.365423084219,1.365423084219,
1.365423084219,1.365423084219)))
REPRESENTATION_ITEM('')
SURFACE()
);
#2608=(
BOUNDED_SURFACE()
B_SPLINE_SURFACE(3,3,((#157765,#157766,#157767,#157768,#157769,#157770,
#157771,#157772),(#157773,#157774,#157775,#157776,#157777,#157778,#157779,
#157780),(#157781,#157782,#157783,#157784,#157785,#157786,#157787,#157788),
(#157789,#157790,#157791,#157792,#157793,#157794,#157795,#157796)),
 .UNSPECIFIED.,.F.,.F.,.F.)
B_SPLINE_SURFACE_WITH_KNOTS((4,4),(4,1,1,1,1,4),(0.,1.),(0.,0.157697040801397,
0.393079047435905,0.650027565804429,0.931370132469644,1.),.UNSPECIFIED.)
GEOMETRIC_REPRESENTATION_ITEM()
RATIONAL_B_SPLINE_SURFACE(((1.197148182303,1.197148182303,1.197148182303,
1.197148182303,1.197148182303,1.197148182303,1.197148182303,1.197148182303),
(0.9342839392322,0.9342839392322,0.9342839392322,0.9342839392322,0.9342839392322,
0.9342839392322,0.9342839392322,0.9342839392322),(0.9342839392322,0.9342839392322,
0.9342839392322,0.9342839392322,0.9342839392322,0.9342839392322,0.9342839392322,
0.9342839392322),(1.197148182303,1.197148182303,1.197148182303,1.197148182303,
1.197148182303,1.197148182303,1.197148182303,1.197148182303)))
REPRESENTATION_ITEM('')
SURFACE()
);
#2609=(
BOUNDED_SURFACE()
B_SPLINE_SURFACE(3,3,((#157809,#157810,#157811,#157812,#157813,#157814,
#157815,#157816),(#157817,#157818,#157819,#157820,#157821,#157822,#157823,
#157824),(#157825,#157826,#157827,#157828,#157829,#157830,#157831,#157832),
(#157833,#157834,#157835,#157836,#157837,#157838,#157839,#157840)),
 .UNSPECIFIED.,.F.,.F.,.F.)
B_SPLINE_SURFACE_WITH_KNOTS((4,4),(4,1,1,1,1,4),(0.,1.),(0.,0.245592378959836,
0.46830203940624,0.669594909978842,0.852727601618965,1.),.UNSPECIFIED.)
GEOMETRIC_REPRESENTATION_ITEM()
RATIONAL_B_SPLINE_SURFACE(((1.57495749403,1.57495749403,1.57495749403,1.57495749403,
1.57495749403,1.57495749403,1.57495749403,1.57495749403),(0.80834750199,
0.80834750199,0.80834750199,0.80834750199,0.80834750199,0.80834750199,0.80834750199,
0.80834750199),(0.80834750199,0.80834750199,0.80834750199,0.80834750199,
0.80834750199,0.80834750199,0.80834750199,0.80834750199),(1.57495749403,
1.57495749403,1.57495749403,1.57495749403,1.57495749403,1.57495749403,1.57495749403,
1.57495749403)))
REPRESENTATION_ITEM('')
SURFACE()
);
#2610=(
BOUNDED_SURFACE()
B_SPLINE_SURFACE(3,3,((#157908,#157909,#157910,#157911,#157912,#157913),
(#157914,#157915,#157916,#157917,#157918,#157919),(#157920,#157921,#157922,
#157923,#157924,#157925),(#157926,#157927,#157928,#157929,#157930,#157931)),
 .UNSPECIFIED.,.F.,.F.,.F.)
B_SPLINE_SURFACE_WITH_KNOTS((4,4),(4,1,1,4),(0.,1.),(0.,0.315996242763536,
0.651612786416777,1.),.UNSPECIFIED.)
GEOMETRIC_REPRESENTATION_ITEM()
RATIONAL_B_SPLINE_SURFACE(((1.618973394811,1.618973394811,1.618973394811,
1.618973394811,1.618973394811,1.618973394811),(0.7936755350628,0.7936755350628,
0.7936755350628,0.7936755350628,0.7936755350628,0.7936755350628),(0.7936755350628,
0.7936755350628,0.7936755350628,0.7936755350628,0.7936755350628,0.7936755350628),
(1.618973394811,1.618973394811,1.618973394811,1.618973394811,1.618973394811,
1.618973394811)))
REPRESENTATION_ITEM('')
SURFACE()
);
#2611=(
BOUNDED_SURFACE()
B_SPLINE_SURFACE(3,3,((#157933,#157934,#157935,#157936,#157937,#157938),
(#157939,#157940,#157941,#157942,#157943,#157944),(#157945,#157946,#157947,
#157948,#157949,#157950),(#157951,#157952,#157953,#157954,#157955,#157956)),
 .UNSPECIFIED.,.F.,.F.,.F.)
B_SPLINE_SURFACE_WITH_KNOTS((4,4),(4,1,1,4),(0.,1.),(0.,0.353278343182746,
0.688996150200427,1.),.UNSPECIFIED.)
GEOMETRIC_REPRESENTATION_ITEM()
RATIONAL_B_SPLINE_SURFACE(((1.61897754235,1.61897754235,1.61897754235,1.61897754235,
1.61897754235,1.61897754235),(0.7936741525501,0.7936741525501,0.7936741525501,
0.7936741525501,0.7936741525501,0.7936741525501),(0.7936741525501,0.7936741525501,
0.7936741525501,0.7936741525501,0.7936741525501,0.7936741525501),(1.61897754235,
1.61897754235,1.61897754235,1.61897754235,1.61897754235,1.61897754235)))
REPRESENTATION_ITEM('')
SURFACE()
);
#2612=(
BOUNDED_SURFACE()
B_SPLINE_SURFACE(3,3,((#158024,#158025,#158026,#158027,#158028,#158029,
#158030),(#158031,#158032,#158033,#158034,#158035,#158036,#158037),(#158038,
#158039,#158040,#158041,#158042,#158043,#158044),(#158045,#158046,#158047,
#158048,#158049,#158050,#158051)),.UNSPECIFIED.,.F.,.F.,.F.)
B_SPLINE_SURFACE_WITH_KNOTS((4,4),(4,1,1,1,4),(0.,1.),(0.,0.238209296182581,
0.514853671561738,0.773063557579565,1.),.UNSPECIFIED.)
GEOMETRIC_REPRESENTATION_ITEM()
RATIONAL_B_SPLINE_SURFACE(((1.574963454954,1.574963454954,1.574963454954,
1.574963454954,1.574963454954,1.574963454954,1.574963454954),(0.8083455150155,
0.8083455150155,0.8083455150155,0.8083455150155,0.8083455150155,0.8083455150155,
0.8083455150155),(0.8083455150155,0.8083455150155,0.8083455150155,0.8083455150155,
0.8083455150155,0.8083455150155,0.8083455150155),(1.574963454954,1.574963454954,
1.574963454954,1.574963454954,1.574963454954,1.574963454954,1.574963454954)))
REPRESENTATION_ITEM('')
SURFACE()
);
#2613=(
BOUNDED_SURFACE()
B_SPLINE_SURFACE(3,3,((#158059,#158060,#158061,#158062,#158063,#158064,
#158065,#158066),(#158067,#158068,#158069,#158070,#158071,#158072,#158073,
#158074),(#158075,#158076,#158077,#158078,#158079,#158080,#158081,#158082),
(#158083,#158084,#158085,#158086,#158087,#158088,#158089,#158090)),
 .UNSPECIFIED.,.F.,.F.,.F.)
B_SPLINE_SURFACE_WITH_KNOTS((4,4),(4,1,1,1,1,4),(0.,1.),(0.,0.0910089094295778,
0.411981715642662,0.714695138546929,0.987601458405524,1.),.UNSPECIFIED.)
GEOMETRIC_REPRESENTATION_ITEM()
RATIONAL_B_SPLINE_SURFACE(((1.053281584436,1.053281584436,1.053281584436,
1.053281584436,1.053281584436,1.053281584436,1.053281584436,1.053281584436),
(0.9822394718546,0.9822394718546,0.9822394718546,0.9822394718546,0.9822394718546,
0.9822394718546,0.9822394718546,0.9822394718546),(0.9822394718546,0.9822394718546,
0.9822394718546,0.9822394718546,0.9822394718546,0.9822394718546,0.9822394718546,
0.9822394718546),(1.053281584436,1.053281584436,1.053281584436,1.053281584436,
1.053281584436,1.053281584436,1.053281584436,1.053281584436)))
REPRESENTATION_ITEM('')
SURFACE()
);
#2614=(
BOUNDED_SURFACE()
B_SPLINE_SURFACE(3,3,((#158092,#158093,#158094,#158095,#158096,#158097,
#158098,#158099,#158100,#158101,#158102,#158103,#158104,#158105,#158106),
(#158107,#158108,#158109,#158110,#158111,#158112,#158113,#158114,#158115,
#158116,#158117,#158118,#158119,#158120,#158121),(#158122,#158123,#158124,
#158125,#158126,#158127,#158128,#158129,#158130,#158131,#158132,#158133,
#158134,#158135,#158136),(#158137,#158138,#158139,#158140,#158141,#158142,
#158143,#158144,#158145,#158146,#158147,#158148,#158149,#158150,#158151)),
 .UNSPECIFIED.,.F.,.F.,.F.)
B_SPLINE_SURFACE_WITH_KNOTS((4,4),(4,1,1,1,1,1,1,1,1,1,1,1,4),(0.,1.),(0.,
0.0156422110548145,0.0753559354221289,0.141207904238176,0.214058894202432,
0.294186759104291,0.382332029305939,0.47906197419899,0.584630248561368,
0.699064662214264,0.825987217014722,0.963692456243815,1.),.UNSPECIFIED.)
GEOMETRIC_REPRESENTATION_ITEM()
RATIONAL_B_SPLINE_SURFACE(((1.289195161833,1.289195161833,1.289195161833,
1.289195161833,1.289195161833,1.289195161833,1.289195161833,1.289195161833,
1.289195161833,1.289195161833,1.289195161833,1.289195161833,1.289195161833,
1.289195161833,1.289195161833),(0.9036016127224,0.9036016127224,0.9036016127224,
0.9036016127224,0.9036016127224,0.9036016127224,0.9036016127224,0.9036016127224,
0.9036016127224,0.9036016127224,0.9036016127224,0.9036016127224,0.9036016127224,
0.9036016127224,0.9036016127224),(0.9036016127224,0.9036016127224,0.9036016127224,
0.9036016127224,0.9036016127224,0.9036016127224,0.9036016127224,0.9036016127224,
0.9036016127224,0.9036016127224,0.9036016127224,0.9036016127224,0.9036016127224,
0.9036016127224,0.9036016127224),(1.289195161833,1.289195161833,1.289195161833,
1.289195161833,1.289195161833,1.289195161833,1.289195161833,1.289195161833,
1.289195161833,1.289195161833,1.289195161833,1.289195161833,1.289195161833,
1.289195161833,1.289195161833)))
REPRESENTATION_ITEM('')
SURFACE()
);
#2634=ELLIPSE('',#79489,7.3350975987285,0.32648194728831);
#2635=ELLIPSE('',#79497,7.83636103876833,0.373161200194601);
#2636=ELLIPSE('',#79579,12.7157342481197,10.9354621733428);
#2637=ELLIPSE('',#79581,12.7157342481197,10.9354621733428);
#2638=ELLIPSE('',#79623,8.41787972385908,7.11051334783377);
#2639=ELLIPSE('',#79624,9.74678054815318,7.6569975264341);
#2640=ELLIPSE('',#79625,8.32808509851651,7.07191618373715);
#2641=ELLIPSE('',#79626,9.18146121407547,7.43010531309855);
#2642=ELLIPSE('',#79642,14.1342891289832,8.17227711305746);
#2643=ELLIPSE('',#79746,0.448239149373515,0.327540749333151);
#2644=ELLIPSE('',#79856,0.537354784288396,0.471561563563283);
#2645=ELLIPSE('',#79960,3.55794038290777,3.09770950143825);
#2646=ELLIPSE('',#79962,3.55430359086793,3.0925288495517);
#2647=ELLIPSE('',#79989,0.230877359575232,0.0439685216321683);
#2648=ELLIPSE('',#79992,0.999999440004323,0.999956206655532);
#2649=ELLIPSE('',#79993,0.58212397125333,0.288222735668278);
#2650=ELLIPSE('',#79994,1.00000913814908,1.00000372087532);
#2651=ELLIPSE('',#79996,0.99999751649857,0.999949952913826);
#2652=ELLIPSE('',#79997,0.461878026571497,0.20445740323273);
#2653=ELLIPSE('',#79999,0.570625652506482,0.279442134038595);
#2654=ELLIPSE('',#80000,1.00000820510229,1.00000324016541);
#2655=ELLIPSE('',#80036,5.77975652153566,1.73376523826803);
#2656=ELLIPSE('',#80037,5.77975702315866,1.73376510670019);
#2657=ELLIPSE('',#80040,7.98766575140942,6.54138279610246);
#2658=ELLIPSE('',#80041,7.89479656652042,6.50286203782701);
#2659=ELLIPSE('',#80048,6.68093268230233,6.48391619812492);
#2660=ELLIPSE('',#80050,17.8204676442288,10.8665310134287);
#2661=ELLIPSE('',#80054,17.8216755759407,10.8669283569276);
#2662=ELLIPSE('',#80055,13.7004973761119,10.3996515308452);
#2663=ELLIPSE('',#80056,17.8213078488318,10.8675975589238);
#2664=ELLIPSE('',#80058,0.300578905254033,0.300169332845296);
#2665=ELLIPSE('',#80061,0.300501638187859,0.300145087153444);
#2666=ELLIPSE('',#80063,26.0448166050072,22.5188326364935);
#2667=ELLIPSE('',#80067,26.0445282577398,22.5188288456468);
#2668=ELLIPSE('',#80075,1.16678567996192,0.984956908240673);
#2669=ELLIPSE('',#80080,2.02790772505133,1.32306037298937);
#2670=ELLIPSE('',#80086,1.50087549620214,1.50024072486622);
#2671=ELLIPSE('',#80109,1.00000429582904,0.999959765461321);
#2672=ELLIPSE('',#80119,7.36743767248193,6.31153366741115);
#2673=ELLIPSE('',#80120,7.3643766184232,6.30732810291296);
#2674=ELLIPSE('',#80121,7.36683820377045,6.30652372661992);
#2675=ELLIPSE('',#80198,6.01936442072139,4.02510096151128);
#2676=ELLIPSE('',#80199,1.50007989461004,1.49835565329252);
#2677=ELLIPSE('',#80201,7.45835235668087,6.38816819337483);
#2678=ELLIPSE('',#80203,14.4207325249774,8.05921542126747);
#2679=ELLIPSE('',#80210,7.92572203798161,6.57522559953783);
#2680=ELLIPSE('',#80324,1.50007991586928,1.49835521240408);
#2681=ELLIPSE('',#80325,6.01990921502876,4.02545539685083);
#2682=ELLIPSE('',#80364,7.9772978335424,6.59922188838911);
#2701=LINE('',#106613,#9768);
#2702=LINE('',#106615,#9769);
#2703=LINE('',#106950,#9770);
#2704=LINE('',#106951,#9771);
#2705=LINE('',#107207,#9772);
#2706=LINE('',#107758,#9773);
#2707=LINE('',#107759,#9774);
#2708=LINE('',#108267,#9775);
#2709=LINE('',#108825,#9776);
#2710=LINE('',#108827,#9777);
#2711=LINE('',#109125,#9778);
#2712=LINE('',#109254,#9779);
#2713=LINE('',#109326,#9780);
#2714=LINE('',#109441,#9781);
#2715=LINE('',#109491,#9782);
#2716=LINE('',#109604,#9783);
#2717=LINE('',#109681,#9784);
#2718=LINE('',#109724,#9785);
#2719=LINE('',#109768,#9786);
#2720=LINE('',#109996,#9787);
#2721=LINE('',#110222,#9788);
#2722=LINE('',#110454,#9789);
#2723=LINE('',#110486,#9790);
#2724=LINE('',#110567,#9791);
#2725=LINE('',#110648,#9792);
#2726=LINE('',#110787,#9793);
#2727=LINE('',#111047,#9794);
#2728=LINE('',#111463,#9795);
#2729=LINE('',#111492,#9796);
#2730=LINE('',#111578,#9797);
#2731=LINE('',#111581,#9798);
#2732=LINE('',#111587,#9799);
#2733=LINE('',#111599,#9800);
#2734=LINE('',#111650,#9801);
#2735=LINE('',#111651,#9802);
#2736=LINE('',#112256,#9803);
#2737=LINE('',#113128,#9804);
#2738=LINE('',#113325,#9805);
#2739=LINE('',#113362,#9806);
#2740=LINE('',#113388,#9807);
#2741=LINE('',#113394,#9808);
#2742=LINE('',#113431,#9809);
#2743=LINE('',#113453,#9810);
#2744=LINE('',#113459,#9811);
#2745=LINE('',#113465,#9812);
#2746=LINE('',#113471,#9813);
#2747=LINE('',#113524,#9814);
#2748=LINE('',#113530,#9815);
#2749=LINE('',#113538,#9816);
#2750=LINE('',#113664,#9817);
#2751=LINE('',#113667,#9818);
#2752=LINE('',#113930,#9819);
#2753=LINE('',#113934,#9820);
#2754=LINE('',#113960,#9821);
#2755=LINE('',#114235,#9822);
#2756=LINE('',#114914,#9823);
#2757=LINE('',#115280,#9824);
#2758=LINE('',#115284,#9825);
#2759=LINE('',#115455,#9826);
#2760=LINE('',#115461,#9827);
#2761=LINE('',#115604,#9828);
#2762=LINE('',#115609,#9829);
#2763=LINE('',#115616,#9830);
#2764=LINE('',#115621,#9831);
#2765=LINE('',#115628,#9832);
#2766=LINE('',#115651,#9833);
#2767=LINE('',#115665,#9834);
#2768=LINE('',#115678,#9835);
#2769=LINE('',#116093,#9836);
#2770=LINE('',#116707,#9837);
#2771=LINE('',#116711,#9838);
#2772=LINE('',#116714,#9839);
#2773=LINE('',#116748,#9840);
#2774=LINE('',#116751,#9841);
#2775=LINE('',#116756,#9842);
#2776=LINE('',#116763,#9843);
#2777=LINE('',#116768,#9844);
#2778=LINE('',#116775,#9845);
#2779=LINE('',#116798,#9846);
#2780=LINE('',#116812,#9847);
#2781=LINE('',#116817,#9848);
#2782=LINE('',#116819,#9849);
#2783=LINE('',#116821,#9850);
#2784=LINE('',#116823,#9851);
#2785=LINE('',#116825,#9852);
#2786=LINE('',#116826,#9853);
#2787=LINE('',#116828,#9854);
#2788=LINE('',#116829,#9855);
#2789=LINE('',#116831,#9856);
#2790=LINE('',#116833,#9857);
#2791=LINE('',#116835,#9858);
#2792=LINE('',#116837,#9859);
#2793=LINE('',#116844,#9860);
#2794=LINE('',#116848,#9861);
#2795=LINE('',#117113,#9862);
#2796=LINE('',#117115,#9863);
#2797=LINE('',#117118,#9864);
#2798=LINE('',#117357,#9865);
#2799=LINE('',#117369,#9866);
#2800=LINE('',#117504,#9867);
#2801=LINE('',#117507,#9868);
#2802=LINE('',#117509,#9869);
#2803=LINE('',#117618,#9870);
#2804=LINE('',#117619,#9871);
#2805=LINE('',#118955,#9872);
#2806=LINE('',#118971,#9873);
#2807=LINE('',#119357,#9874);
#2808=LINE('',#119373,#9875);
#2809=LINE('',#119490,#9876);
#2810=LINE('',#119623,#9877);
#2811=LINE('',#119803,#9878);
#2812=LINE('',#122245,#9879);
#2813=LINE('',#122357,#9880);
#2814=LINE('',#122508,#9881);
#2815=LINE('',#123595,#9882);
#2816=LINE('',#123597,#9883);
#2817=LINE('',#123599,#9884);
#2818=LINE('',#123601,#9885);
#2819=LINE('',#123603,#9886);
#2820=LINE('',#123604,#9887);
#2821=LINE('',#123606,#9888);
#2822=LINE('',#123607,#9889);
#2823=LINE('',#123609,#9890);
#2824=LINE('',#123611,#9891);
#2825=LINE('',#123613,#9892);
#2826=LINE('',#123615,#9893);
#2827=LINE('',#123743,#9894);
#2828=LINE('',#123747,#9895);
#2829=LINE('',#124100,#9896);
#2830=LINE('',#124102,#9897);
#2831=LINE('',#124362,#9898);
#2832=LINE('',#124433,#9899);
#2833=LINE('',#124436,#9900);
#2834=LINE('',#124472,#9901);
#2835=LINE('',#124473,#9902);
#2836=LINE('',#124716,#9903);
#2837=LINE('',#124739,#9904);
#2838=LINE('',#125405,#9905);
#2839=LINE('',#125420,#9906);
#2840=LINE('',#125981,#9907);
#2841=LINE('',#126076,#9908);
#2842=LINE('',#126214,#9909);
#2843=LINE('',#126231,#9910);
#2844=LINE('',#126387,#9911);
#2845=LINE('',#128721,#9912);
#2846=LINE('',#128799,#9913);
#2847=LINE('',#128951,#9914);
#2848=LINE('',#130145,#9915);
#2849=LINE('',#130316,#9916);
#2850=LINE('',#130323,#9917);
#2851=LINE('',#130325,#9918);
#2852=LINE('',#130327,#9919);
#2853=LINE('',#130329,#9920);
#2854=LINE('',#130342,#9921);
#2855=LINE('',#130344,#9922);
#2856=LINE('',#130346,#9923);
#2857=LINE('',#130357,#9924);
#2858=LINE('',#130360,#9925);
#2859=LINE('',#130362,#9926);
#2860=LINE('',#130366,#9927);
#2861=LINE('',#130368,#9928);
#2862=LINE('',#130376,#9929);
#2863=LINE('',#130405,#9930);
#2864=LINE('',#130459,#9931);
#2865=LINE('',#130461,#9932);
#2866=LINE('',#130462,#9933);
#2867=LINE('',#130599,#9934);
#2868=LINE('',#130809,#9935);
#2869=LINE('',#131031,#9936);
#2870=LINE('',#131158,#9937);
#2871=LINE('',#131190,#9938);
#2872=LINE('',#131323,#9939);
#2873=LINE('',#131351,#9940);
#2874=LINE('',#131878,#9941);
#2875=LINE('',#131892,#9942);
#2876=LINE('',#132386,#9943);
#2877=LINE('',#133459,#9944);
#2878=LINE('',#133466,#9945);
#2879=LINE('',#133470,#9946);
#2880=LINE('',#133472,#9947);
#2881=LINE('',#133473,#9948);
#2882=LINE('',#133475,#9949);
#2883=LINE('',#134436,#9950);
#2884=LINE('',#134583,#9951);
#2885=LINE('',#134694,#9952);
#2886=LINE('',#134712,#9953);
#2887=LINE('',#135396,#9954);
#2888=LINE('',#135398,#9955);
#2889=LINE('',#135577,#9956);
#2890=LINE('',#135578,#9957);
#2891=LINE('',#135614,#9958);
#2892=LINE('',#135619,#9959);
#2893=LINE('',#135625,#9960);
#2894=LINE('',#135629,#9961);
#2895=LINE('',#135644,#9962);
#2896=LINE('',#136522,#9963);
#2897=LINE('',#137848,#9964);
#2898=LINE('',#137895,#9965);
#2899=LINE('',#137934,#9966);
#2900=LINE('',#138666,#9967);
#2901=LINE('',#138705,#9968);
#2902=LINE('',#139066,#9969);
#2903=LINE('',#141026,#9970);
#2904=LINE('',#142940,#9971);
#2905=LINE('',#143028,#9972);
#2906=LINE('',#143481,#9973);
#2907=LINE('',#143689,#9974);
#2908=LINE('',#143853,#9975);
#2909=LINE('',#144373,#9976);
#2910=LINE('',#145397,#9977);
#2911=LINE('',#145399,#9978);
#2912=LINE('',#145401,#9979);
#2913=LINE('',#145402,#9980);
#2914=LINE('',#145404,#9981);
#2915=LINE('',#145411,#9982);
#2916=LINE('',#145415,#9983);
#2917=LINE('',#145500,#9984);
#2918=LINE('',#145576,#9985);
#2919=LINE('',#145595,#9986);
#2920=LINE('',#145631,#9987);
#2921=LINE('',#145831,#9988);
#2922=LINE('',#145834,#9989);
#2923=LINE('',#145881,#9990);
#2924=LINE('',#145883,#9991);
#2925=LINE('',#145885,#9992);
#2926=LINE('',#145948,#9993);
#2927=LINE('',#146296,#9994);
#2928=LINE('',#146299,#9995);
#2929=LINE('',#146333,#9996);
#2930=LINE('',#146364,#9997);
#2931=LINE('',#146366,#9998);
#2932=LINE('',#146367,#9999);
#2933=LINE('',#146906,#10000);
#2934=LINE('',#146909,#10001);
#2935=LINE('',#146910,#10002);
#2936=LINE('',#146914,#10003);
#2937=LINE('',#146916,#10004);
#2938=LINE('',#146917,#10005);
#2939=LINE('',#147574,#10006);
#2940=LINE('',#147714,#10007);
#2941=LINE('',#147721,#10008);
#2942=LINE('',#149827,#10009);
#2943=LINE('',#149867,#10010);
#2944=LINE('',#149954,#10011);
#2945=LINE('',#149957,#10012);
#2946=LINE('',#150111,#10013);
#2947=LINE('',#150150,#10014);
#2948=LINE('',#150202,#10015);
#2949=LINE('',#150257,#10016);
#2950=LINE('',#150259,#10017);
#2951=LINE('',#154828,#10018);
#2952=LINE('',#154832,#10019);
#2953=LINE('',#154966,#10020);
#2954=LINE('',#156808,#10021);
#2955=LINE('',#156999,#10022);
#9768=VECTOR('',#86178,1000.);
#9769=VECTOR('',#86179,1000.);
#9770=VECTOR('',#86198,1000.);
#9771=VECTOR('',#86199,1000.);
#9772=VECTOR('',#86208,1000.);
#9773=VECTOR('',#86213,1000.);
#9774=VECTOR('',#86214,1000.);
#9775=VECTOR('',#86225,1000.);
#9776=VECTOR('',#86232,1000.);
#9777=VECTOR('',#86235,1000.);
#9778=VECTOR('',#86242,8.4);
#9779=VECTOR('',#86247,8.4);
#9780=VECTOR('',#86250,8.4);
#9781=VECTOR('',#86253,8.4);
#9782=VECTOR('',#86258,8.4);
#9783=VECTOR('',#86261,8.4);
#9784=VECTOR('',#86266,17.);
#9785=VECTOR('',#86267,1000.);
#9786=VECTOR('',#86270,17.);
#9787=VECTOR('',#86273,17.);
#9788=VECTOR('',#86276,17.);
#9789=VECTOR('',#86279,17.);
#9790=VECTOR('',#86284,16.375);
#9791=VECTOR('',#86285,1000.);
#9792=VECTOR('',#86286,16.375);
#9793=VECTOR('',#86293,16.375);
#9794=VECTOR('',#86296,16.375);
#9795=VECTOR('',#86329,1000.);
#9796=VECTOR('',#86330,1000.);
#9797=VECTOR('',#86343,10.);
#9798=VECTOR('',#86346,10.);
#9799=VECTOR('',#86351,10.5);
#9800=VECTOR('',#86366,11.25);
#9801=VECTOR('',#86389,1000.);
#9802=VECTOR('',#86390,1000.);
#9803=VECTOR('',#86395,21.);
#9804=VECTOR('',#86410,1000.);
#9805=VECTOR('',#86411,1000.);
#9806=VECTOR('',#86428,9.500000000001);
#9807=VECTOR('',#86443,7.75);
#9808=VECTOR('',#86450,6.5);
#9809=VECTOR('',#86461,9.5);
#9810=VECTOR('',#86470,13.5);
#9811=VECTOR('',#86477,13.79977495601);
#9812=VECTOR('',#86484,14.5);
#9813=VECTOR('',#86491,7.25000000000001);
#9814=VECTOR('',#86514,6.5);
#9815=VECTOR('',#86519,5.799851372624);
#9816=VECTOR('',#86530,5.5);
#9817=VECTOR('',#86541,1000.);
#9818=VECTOR('',#86544,1000.);
#9819=VECTOR('',#86551,16.);
#9820=VECTOR('',#86558,16.375);
#9821=VECTOR('',#86563,17.175);
#9822=VECTOR('',#86580,9.49999999999999);
#9823=VECTOR('',#86591,12.);
#9824=VECTOR('',#86598,1000.);
#9825=VECTOR('',#86601,1000.);
#9826=VECTOR('',#86602,1000.);
#9827=VECTOR('',#86607,1000.);
#9828=VECTOR('',#86608,1000.);
#9829=VECTOR('',#86613,10.25);
#9830=VECTOR('',#86620,11.75);
#9831=VECTOR('',#86627,11.25);
#9832=VECTOR('',#86634,7.75000000000001);
#9833=VECTOR('',#86643,7.75000000000001);
#9834=VECTOR('',#86646,7.95);
#9835=VECTOR('',#86663,9.49999999999999);
#9836=VECTOR('',#86674,12.);
#9837=VECTOR('',#86679,1000.);
#9838=VECTOR('',#86682,1000.);
#9839=VECTOR('',#86685,1000.);
#9840=VECTOR('',#86688,1000.);
#9841=VECTOR('',#86691,1000.);
#9842=VECTOR('',#86696,10.25);
#9843=VECTOR('',#86703,11.75);
#9844=VECTOR('',#86710,11.25);
#9845=VECTOR('',#86717,7.75000000000001);
#9846=VECTOR('',#86726,7.75000000000001);
#9847=VECTOR('',#86729,7.95);
#9848=VECTOR('',#86734,1000.);
#9849=VECTOR('',#86735,1000.);
#9850=VECTOR('',#86736,1000.);
#9851=VECTOR('',#86737,1000.);
#9852=VECTOR('',#86738,1000.);
#9853=VECTOR('',#86739,1000.);
#9854=VECTOR('',#86742,1000.);
#9855=VECTOR('',#86743,1000.);
#9856=VECTOR('',#86746,1000.);
#9857=VECTOR('',#86749,1000.);
#9858=VECTOR('',#86752,1000.);
#9859=VECTOR('',#86755,1000.);
#9860=VECTOR('',#86764,1000.);
#9861=VECTOR('',#86767,1000.);
#9862=VECTOR('',#86786,1000.);
#9863=VECTOR('',#86787,1000.);
#9864=VECTOR('',#86790,1000.);
#9865=VECTOR('',#86795,1000.);
#9866=VECTOR('',#86802,1000.);
#9867=VECTOR('',#86807,1000.);
#9868=VECTOR('',#86810,1000.);
#9869=VECTOR('',#86813,1000.);
#9870=VECTOR('',#86820,1000.);
#9871=VECTOR('',#86821,1000.);
#9872=VECTOR('',#86856,1000.);
#9873=VECTOR('',#86879,1000.);
#9874=VECTOR('',#86898,10.);
#9875=VECTOR('',#86921,10.);
#9876=VECTOR('',#86924,1000.);
#9877=VECTOR('',#86939,1000.);
#9878=VECTOR('',#86950,1000.);
#9879=VECTOR('',#86979,10.);
#9880=VECTOR('',#86980,10.);
#9881=VECTOR('',#86981,10.);
#9882=VECTOR('',#86986,1000.);
#9883=VECTOR('',#86987,1000.);
#9884=VECTOR('',#86988,1000.);
#9885=VECTOR('',#86989,1000.);
#9886=VECTOR('',#86990,1000.);
#9887=VECTOR('',#86991,1000.);
#9888=VECTOR('',#86994,1000.);
#9889=VECTOR('',#86995,1000.);
#9890=VECTOR('',#86998,1000.);
#9891=VECTOR('',#87001,1000.);
#9892=VECTOR('',#87004,1000.);
#9893=VECTOR('',#87007,1000.);
#9894=VECTOR('',#87016,1000.);
#9895=VECTOR('',#87019,1000.);
#9896=VECTOR('',#87028,1000.);
#9897=VECTOR('',#87031,1000.);
#9898=VECTOR('',#87034,1000.);
#9899=VECTOR('',#87039,1000.);
#9900=VECTOR('',#87042,1000.);
#9901=VECTOR('',#87049,1000.);
#9902=VECTOR('',#87050,1000.);
#9903=VECTOR('',#87065,1000.);
#9904=VECTOR('',#87070,1000.);
#9905=VECTOR('',#87093,1000.);
#9906=VECTOR('',#87116,1000.);
#9907=VECTOR('',#87145,10.);
#9908=VECTOR('',#87166,1000.);
#9909=VECTOR('',#87169,10.);
#9910=VECTOR('',#87192,1000.);
#9911=VECTOR('',#87195,1000.);
#9912=VECTOR('',#87230,10.);
#9913=VECTOR('',#87231,10.);
#9914=VECTOR('',#87232,10.);
#9915=VECTOR('',#87235,10.);
#9916=VECTOR('',#87236,10.);
#9917=VECTOR('',#87245,1000.);
#9918=VECTOR('',#87246,1000.);
#9919=VECTOR('',#87247,1000.);
#9920=VECTOR('',#87248,1000.);
#9921=VECTOR('',#87261,1000.);
#9922=VECTOR('',#87262,1000.);
#9923=VECTOR('',#87263,1000.);
#9924=VECTOR('',#87274,1000.);
#9925=VECTOR('',#87277,1000.);
#9926=VECTOR('',#87278,1000.);
#9927=VECTOR('',#87283,1000.);
#9928=VECTOR('',#87284,1000.);
#9929=VECTOR('',#87293,10.);
#9930=VECTOR('',#87298,1000.);
#9931=VECTOR('',#87299,10.);
#9932=VECTOR('',#87300,1000.);
#9933=VECTOR('',#87301,1000.);
#9934=VECTOR('',#87306,10.);
#9935=VECTOR('',#87309,1000.);
#9936=VECTOR('',#87314,10.);
#9937=VECTOR('',#87319,1000.);
#9938=VECTOR('',#87322,10.);
#9939=VECTOR('',#87325,10.);
#9940=VECTOR('',#87328,1000.);
#9941=VECTOR('',#87335,1000.);
#9942=VECTOR('',#87338,1000.);
#9943=VECTOR('',#87351,1000.);
#9944=VECTOR('',#87398,1000.);
#9945=VECTOR('',#87411,1000.);
#9946=VECTOR('',#87414,1000.);
#9947=VECTOR('',#87415,1000.);
#9948=VECTOR('',#87416,1000.);
#9949=VECTOR('',#87417,1000.);
#9950=VECTOR('',#87434,1000.);
#9951=VECTOR('',#87437,1000.);
#9952=VECTOR('',#87438,1000.);
#9953=VECTOR('',#87461,1000.);
#9954=VECTOR('',#87472,1000.);
#9955=VECTOR('',#87473,1000.);
#9956=VECTOR('',#87476,1000.);
#9957=VECTOR('',#87477,1000.);
#9958=VECTOR('',#87492,1000.);
#9959=VECTOR('',#87497,1000.);
#9960=VECTOR('',#87502,1000.);
#9961=VECTOR('',#87505,1000.);
#9962=VECTOR('',#87510,1000.);
#9963=VECTOR('',#87521,1000.);
#9964=VECTOR('',#87522,1000.);
#9965=VECTOR('',#87527,1000.);
#9966=VECTOR('',#87528,1000.);
#9967=VECTOR('',#87533,1000.);
#9968=VECTOR('',#87534,1000.);
#9969=VECTOR('',#87545,1000.);
#9970=VECTOR('',#87560,1000.);
#9971=VECTOR('',#87571,1000.);
#9972=VECTOR('',#87574,1000.);
#9973=VECTOR('',#87595,1000.);
#9974=VECTOR('',#87610,1000.);
#9975=VECTOR('',#87625,1000.);
#9976=VECTOR('',#87656,1000.);
#9977=VECTOR('',#87679,1000.);
#9978=VECTOR('',#87682,1000.);
#9979=VECTOR('',#87685,1000.);
#9980=VECTOR('',#87686,1000.);
#9981=VECTOR('',#87689,1000.);
#9982=VECTOR('',#87698,1000.);
#9983=VECTOR('',#87701,1000.);
#9984=VECTOR('',#87702,1000.);
#9985=VECTOR('',#87703,1000.);
#9986=VECTOR('',#87712,1000.);
#9987=VECTOR('',#87727,1000.);
#9988=VECTOR('',#87740,10.);
#9989=VECTOR('',#87743,10.);
#9990=VECTOR('',#87748,1000.);
#9991=VECTOR('',#87751,1000.);
#9992=VECTOR('',#87754,1000.);
#9993=VECTOR('',#87755,1000.);
#9994=VECTOR('',#87776,1000.);
#9995=VECTOR('',#87779,1000.);
#9996=VECTOR('',#87780,1000.);
#9997=VECTOR('',#87781,1000.);
#9998=VECTOR('',#87782,1000.);
#9999=VECTOR('',#87783,1000.);
#10000=VECTOR('',#87810,1000.);
#10001=VECTOR('',#87813,1000.);
#10002=VECTOR('',#87814,1000.);
#10003=VECTOR('',#87817,1000.);
#10004=VECTOR('',#87818,1000.);
#10005=VECTOR('',#87819,1000.);
#10006=VECTOR('',#87844,10.);
#10007=VECTOR('',#87855,10.);
#10008=VECTOR('',#87856,1000.);
#10009=VECTOR('',#87909,1000.);
#10010=VECTOR('',#87914,1000.);
#10011=VECTOR('',#87915,1000.);
#10012=VECTOR('',#87918,1000.);
#10013=VECTOR('',#87935,1000.);
#10014=VECTOR('',#87940,1000.);
#10015=VECTOR('',#87941,1000.);
#10016=VECTOR('',#87942,1000.);
#10017=VECTOR('',#87945,1000.);
#10018=VECTOR('',#88084,1000.);
#10019=VECTOR('',#88089,1000.);
#10020=VECTOR('',#88092,1000.);
#10021=VECTOR('',#88141,1000.);
#10022=VECTOR('',#88150,1000.);
#16835=PLANE('',#79488);
#16836=PLANE('',#79496);
#16837=PLANE('',#79504);
#16838=PLANE('',#79506);
#16839=PLANE('',#79511);
#16840=PLANE('',#79514);
#16841=PLANE('',#79726);
#16842=PLANE('',#79727);
#16843=PLANE('',#79728);
#16844=PLANE('',#79729);
#16845=PLANE('',#79730);
#16846=PLANE('',#79731);
#16847=PLANE('',#79732);
#16848=PLANE('',#79733);
#16849=PLANE('',#79734);
#16850=PLANE('',#79745);
#16851=PLANE('',#79750);
#16852=PLANE('',#79780);
#16853=PLANE('',#79786);
#16854=PLANE('',#79789);
#16855=PLANE('',#79800);
#16856=PLANE('',#79833);
#16857=PLANE('',#79834);
#16858=PLANE('',#79835);
#16859=PLANE('',#79836);
#16860=PLANE('',#79837);
#16861=PLANE('',#79838);
#16862=PLANE('',#79839);
#16863=PLANE('',#79840);
#16864=PLANE('',#79841);
#16865=PLANE('',#79842);
#16866=PLANE('',#79843);
#16867=PLANE('',#79857);
#16868=PLANE('',#79863);
#16869=PLANE('',#79874);
#16870=PLANE('',#79877);
#16871=PLANE('',#79881);
#16872=PLANE('',#79918);
#16873=PLANE('',#79942);
#16874=PLANE('',#79943);
#16875=PLANE('',#79944);
#16876=PLANE('',#79945);
#16877=PLANE('',#79946);
#16878=PLANE('',#79947);
#16879=PLANE('',#79953);
#16880=PLANE('',#79959);
#16881=PLANE('',#79961);
#16882=PLANE('',#79967);
#16883=PLANE('',#80015);
#16884=PLANE('',#80017);
#16885=PLANE('',#80042);
#16886=PLANE('',#80044);
#16887=PLANE('',#80045);
#16888=PLANE('',#80068);
#16889=PLANE('',#80069);
#16890=PLANE('',#80070);
#16891=PLANE('',#80071);
#16892=PLANE('',#80072);
#16893=PLANE('',#80078);
#16894=PLANE('',#80133);
#16895=PLANE('',#80136);
#16896=PLANE('',#80138);
#16897=PLANE('',#80139);
#16898=PLANE('',#80140);
#16899=PLANE('',#80146);
#16900=PLANE('',#80150);
#16901=PLANE('',#80163);
#16902=PLANE('',#80175);
#16903=PLANE('',#80189);
#16904=PLANE('',#80190);
#16905=PLANE('',#80212);
#16906=PLANE('',#80258);
#16907=PLANE('',#80274);
#16908=PLANE('',#80292);
#16909=PLANE('',#80295);
#16910=PLANE('',#80307);
#16911=PLANE('',#80312);
#16912=PLANE('',#80313);
#16913=PLANE('',#80319);
#16914=PLANE('',#80365);
#16915=PLANE('',#80376);
#19873=FACE_OUTER_BOUND('',#23888,.T.);
#19874=FACE_OUTER_BOUND('',#23889,.T.);
#19875=FACE_OUTER_BOUND('',#23890,.T.);
#19876=FACE_OUTER_BOUND('',#23891,.T.);
#19877=FACE_OUTER_BOUND('',#23892,.T.);
#19878=FACE_OUTER_BOUND('',#23893,.T.);
#19879=FACE_OUTER_BOUND('',#23894,.T.);
#19880=FACE_OUTER_BOUND('',#23895,.T.);
#19881=FACE_OUTER_BOUND('',#23896,.T.);
#19882=FACE_OUTER_BOUND('',#23897,.T.);
#19883=FACE_OUTER_BOUND('',#23898,.T.);
#19884=FACE_OUTER_BOUND('',#23899,.T.);
#19885=FACE_OUTER_BOUND('',#23900,.T.);
#19886=FACE_OUTER_BOUND('',#23901,.T.);
#19887=FACE_OUTER_BOUND('',#23902,.T.);
#19888=FACE_OUTER_BOUND('',#23903,.T.);
#19889=FACE_OUTER_BOUND('',#23904,.T.);
#19890=FACE_OUTER_BOUND('',#23905,.T.);
#19891=FACE_OUTER_BOUND('',#23906,.T.);
#19892=FACE_OUTER_BOUND('',#23907,.T.);
#19893=FACE_OUTER_BOUND('',#23908,.T.);
#19894=FACE_OUTER_BOUND('',#23909,.T.);
#19895=FACE_OUTER_BOUND('',#23910,.T.);
#19896=FACE_OUTER_BOUND('',#23911,.T.);
#19897=FACE_OUTER_BOUND('',#23912,.T.);
#19898=FACE_OUTER_BOUND('',#23913,.T.);
#19899=FACE_OUTER_BOUND('',#23914,.T.);
#19900=FACE_OUTER_BOUND('',#23915,.T.);
#19901=FACE_OUTER_BOUND('',#23916,.T.);
#19902=FACE_OUTER_BOUND('',#23917,.T.);
#19903=FACE_OUTER_BOUND('',#23918,.T.);
#19904=FACE_OUTER_BOUND('',#23919,.T.);
#19905=FACE_OUTER_BOUND('',#23920,.T.);
#19906=FACE_OUTER_BOUND('',#23921,.T.);
#19907=FACE_OUTER_BOUND('',#23922,.T.);
#19908=FACE_OUTER_BOUND('',#23923,.T.);
#19909=FACE_OUTER_BOUND('',#23924,.T.);
#19910=FACE_OUTER_BOUND('',#23925,.T.);
#19911=FACE_OUTER_BOUND('',#23926,.T.);
#19912=FACE_OUTER_BOUND('',#23927,.T.);
#19913=FACE_OUTER_BOUND('',#23928,.T.);
#19914=FACE_OUTER_BOUND('',#23929,.T.);
#19915=FACE_OUTER_BOUND('',#23930,.T.);
#19916=FACE_OUTER_BOUND('',#23931,.T.);
#19917=FACE_OUTER_BOUND('',#23932,.T.);
#19918=FACE_OUTER_BOUND('',#23933,.T.);
#19919=FACE_OUTER_BOUND('',#23934,.T.);
#19920=FACE_OUTER_BOUND('',#23935,.T.);
#19921=FACE_OUTER_BOUND('',#23936,.T.);
#19922=FACE_OUTER_BOUND('',#23937,.T.);
#19923=FACE_OUTER_BOUND('',#23938,.T.);
#19924=FACE_OUTER_BOUND('',#23939,.T.);
#19925=FACE_OUTER_BOUND('',#23940,.T.);
#19926=FACE_OUTER_BOUND('',#23941,.T.);
#19927=FACE_OUTER_BOUND('',#23942,.T.);
#19928=FACE_OUTER_BOUND('',#23943,.T.);
#19929=FACE_OUTER_BOUND('',#23944,.T.);
#19930=FACE_OUTER_BOUND('',#23945,.T.);
#19931=FACE_OUTER_BOUND('',#23946,.T.);
#19932=FACE_OUTER_BOUND('',#23947,.T.);
#19933=FACE_OUTER_BOUND('',#23948,.T.);
#19934=FACE_OUTER_BOUND('',#23949,.T.);
#19935=FACE_OUTER_BOUND('',#23950,.T.);
#19936=FACE_OUTER_BOUND('',#23951,.T.);
#19937=FACE_OUTER_BOUND('',#23952,.T.);
#19938=FACE_OUTER_BOUND('',#23953,.T.);
#19939=FACE_OUTER_BOUND('',#23954,.T.);
#19940=FACE_OUTER_BOUND('',#23955,.T.);
#19941=FACE_OUTER_BOUND('',#23956,.T.);
#19942=FACE_OUTER_BOUND('',#23957,.T.);
#19943=FACE_OUTER_BOUND('',#23958,.T.);
#19944=FACE_OUTER_BOUND('',#23959,.T.);
#19945=FACE_OUTER_BOUND('',#23960,.T.);
#19946=FACE_OUTER_BOUND('',#23961,.T.);
#19947=FACE_OUTER_BOUND('',#23962,.T.);
#19948=FACE_OUTER_BOUND('',#23963,.T.);
#19949=FACE_OUTER_BOUND('',#23964,.T.);
#19950=FACE_OUTER_BOUND('',#23965,.T.);
#19951=FACE_OUTER_BOUND('',#23966,.T.);
#19952=FACE_OUTER_BOUND('',#23967,.T.);
#19953=FACE_OUTER_BOUND('',#23968,.T.);
#19954=FACE_OUTER_BOUND('',#23969,.T.);
#19955=FACE_OUTER_BOUND('',#23970,.T.);
#19956=FACE_OUTER_BOUND('',#23971,.T.);
#19957=FACE_OUTER_BOUND('',#23972,.T.);
#19958=FACE_OUTER_BOUND('',#23973,.T.);
#19959=FACE_OUTER_BOUND('',#23974,.T.);
#19960=FACE_OUTER_BOUND('',#23975,.T.);
#19961=FACE_OUTER_BOUND('',#23976,.T.);
#19962=FACE_OUTER_BOUND('',#23977,.T.);
#19963=FACE_OUTER_BOUND('',#23978,.T.);
#19964=FACE_OUTER_BOUND('',#23979,.T.);
#19965=FACE_OUTER_BOUND('',#23980,.T.);
#19966=FACE_OUTER_BOUND('',#23981,.T.);
#19967=FACE_OUTER_BOUND('',#23982,.T.);
#19968=FACE_OUTER_BOUND('',#23983,.T.);
#19969=FACE_OUTER_BOUND('',#23984,.T.);
#19970=FACE_OUTER_BOUND('',#23985,.T.);
#19971=FACE_OUTER_BOUND('',#23986,.T.);
#19972=FACE_OUTER_BOUND('',#23987,.T.);
#19973=FACE_OUTER_BOUND('',#23988,.T.);
#19974=FACE_OUTER_BOUND('',#23989,.T.);
#19975=FACE_OUTER_BOUND('',#23990,.T.);
#19976=FACE_OUTER_BOUND('',#23991,.T.);
#19977=FACE_OUTER_BOUND('',#23992,.T.);
#19978=FACE_OUTER_BOUND('',#23993,.T.);
#19979=FACE_OUTER_BOUND('',#23994,.T.);
#19980=FACE_OUTER_BOUND('',#23995,.T.);
#19981=FACE_OUTER_BOUND('',#23996,.T.);
#19982=FACE_OUTER_BOUND('',#23997,.T.);
#19983=FACE_OUTER_BOUND('',#23998,.T.);
#19984=FACE_OUTER_BOUND('',#24000,.T.);
#19985=FACE_OUTER_BOUND('',#24001,.T.);
#19986=FACE_OUTER_BOUND('',#24002,.T.);
#19987=FACE_OUTER_BOUND('',#24003,.T.);
#19988=FACE_OUTER_BOUND('',#24004,.T.);
#19989=FACE_OUTER_BOUND('',#24005,.T.);
#19990=FACE_OUTER_BOUND('',#24006,.T.);
#19991=FACE_OUTER_BOUND('',#24008,.T.);
#19992=FACE_OUTER_BOUND('',#24010,.T.);
#19993=FACE_OUTER_BOUND('',#24011,.T.);
#19994=FACE_OUTER_BOUND('',#24012,.T.);
#19995=FACE_OUTER_BOUND('',#24013,.T.);
#19996=FACE_OUTER_BOUND('',#24014,.T.);
#19997=FACE_OUTER_BOUND('',#24015,.T.);
#19998=FACE_OUTER_BOUND('',#24016,.T.);
#19999=FACE_OUTER_BOUND('',#24017,.T.);
#20000=FACE_OUTER_BOUND('',#24018,.T.);
#20001=FACE_OUTER_BOUND('',#24019,.T.);
#20002=FACE_OUTER_BOUND('',#24020,.T.);
#20003=FACE_OUTER_BOUND('',#24021,.T.);
#20004=FACE_OUTER_BOUND('',#24022,.T.);
#20005=FACE_OUTER_BOUND('',#24023,.T.);
#20006=FACE_OUTER_BOUND('',#24024,.T.);
#20007=FACE_OUTER_BOUND('',#24025,.T.);
#20008=FACE_OUTER_BOUND('',#24026,.T.);
#20009=FACE_OUTER_BOUND('',#24027,.T.);
#20010=FACE_OUTER_BOUND('',#24028,.T.);
#20011=FACE_OUTER_BOUND('',#24029,.T.);
#20012=FACE_OUTER_BOUND('',#24030,.T.);
#20013=FACE_OUTER_BOUND('',#24031,.T.);
#20014=FACE_OUTER_BOUND('',#24032,.T.);
#20015=FACE_OUTER_BOUND('',#24033,.T.);
#20016=FACE_OUTER_BOUND('',#24034,.T.);
#20017=FACE_OUTER_BOUND('',#24035,.T.);
#20018=FACE_OUTER_BOUND('',#24036,.T.);
#20019=FACE_OUTER_BOUND('',#24037,.T.);
#20020=FACE_OUTER_BOUND('',#24038,.T.);
#20021=FACE_OUTER_BOUND('',#24039,.T.);
#20022=FACE_OUTER_BOUND('',#24040,.T.);
#20023=FACE_OUTER_BOUND('',#24041,.T.);
#20024=FACE_OUTER_BOUND('',#24042,.T.);
#20025=FACE_OUTER_BOUND('',#24043,.T.);
#20026=FACE_OUTER_BOUND('',#24044,.T.);
#20027=FACE_OUTER_BOUND('',#24045,.T.);
#20028=FACE_OUTER_BOUND('',#24046,.T.);
#20029=FACE_OUTER_BOUND('',#24047,.T.);
#20030=FACE_OUTER_BOUND('',#24048,.T.);
#20031=FACE_OUTER_BOUND('',#24049,.T.);
#20032=FACE_OUTER_BOUND('',#24050,.T.);
#20033=FACE_OUTER_BOUND('',#24051,.T.);
#20034=FACE_OUTER_BOUND('',#24052,.T.);
#20035=FACE_OUTER_BOUND('',#24053,.T.);
#20036=FACE_OUTER_BOUND('',#24054,.T.);
#20037=FACE_OUTER_BOUND('',#24055,.T.);
#20038=FACE_OUTER_BOUND('',#24056,.T.);
#20039=FACE_OUTER_BOUND('',#24057,.T.);
#20040=FACE_OUTER_BOUND('',#24058,.T.);
#20041=FACE_OUTER_BOUND('',#24059,.T.);
#20042=FACE_OUTER_BOUND('',#24060,.T.);
#20043=FACE_OUTER_BOUND('',#24061,.T.);
#20044=FACE_OUTER_BOUND('',#24062,.T.);
#20045=FACE_OUTER_BOUND('',#24063,.T.);
#20046=FACE_OUTER_BOUND('',#24064,.T.);
#20047=FACE_OUTER_BOUND('',#24065,.T.);
#20048=FACE_OUTER_BOUND('',#24066,.T.);
#20049=FACE_OUTER_BOUND('',#24067,.T.);
#20050=FACE_OUTER_BOUND('',#24068,.T.);
#20051=FACE_OUTER_BOUND('',#24069,.T.);
#20052=FACE_OUTER_BOUND('',#24070,.T.);
#20053=FACE_OUTER_BOUND('',#24071,.T.);
#20054=FACE_OUTER_BOUND('',#24072,.T.);
#20055=FACE_OUTER_BOUND('',#24073,.T.);
#20056=FACE_OUTER_BOUND('',#24074,.T.);
#20057=FACE_OUTER_BOUND('',#24075,.T.);
#20058=FACE_OUTER_BOUND('',#24076,.T.);
#20059=FACE_OUTER_BOUND('',#24077,.T.);
#20060=FACE_OUTER_BOUND('',#24079,.T.);
#20061=FACE_OUTER_BOUND('',#24080,.T.);
#20062=FACE_OUTER_BOUND('',#24081,.T.);
#20063=FACE_OUTER_BOUND('',#24082,.T.);
#20064=FACE_OUTER_BOUND('',#24083,.T.);
#20065=FACE_OUTER_BOUND('',#24084,.T.);
#20066=FACE_OUTER_BOUND('',#24085,.T.);
#20067=FACE_OUTER_BOUND('',#24087,.T.);
#20068=FACE_OUTER_BOUND('',#24089,.T.);
#20069=FACE_OUTER_BOUND('',#24090,.T.);
#20070=FACE_OUTER_BOUND('',#24091,.T.);
#20071=FACE_OUTER_BOUND('',#24092,.T.);
#20072=FACE_OUTER_BOUND('',#24093,.T.);
#20073=FACE_OUTER_BOUND('',#24094,.T.);
#20074=FACE_OUTER_BOUND('',#24095,.T.);
#20075=FACE_OUTER_BOUND('',#24097,.T.);
#20076=FACE_OUTER_BOUND('',#24099,.T.);
#20077=FACE_OUTER_BOUND('',#24100,.T.);
#20078=FACE_OUTER_BOUND('',#24101,.T.);
#20079=FACE_OUTER_BOUND('',#24102,.T.);
#20080=FACE_OUTER_BOUND('',#24103,.T.);
#20081=FACE_OUTER_BOUND('',#24104,.T.);
#20082=FACE_OUTER_BOUND('',#24105,.T.);
#20083=FACE_OUTER_BOUND('',#24106,.T.);
#20084=FACE_OUTER_BOUND('',#24107,.T.);
#20085=FACE_OUTER_BOUND('',#24108,.T.);
#20086=FACE_OUTER_BOUND('',#24109,.T.);
#20087=FACE_OUTER_BOUND('',#24110,.T.);
#20088=FACE_OUTER_BOUND('',#24111,.T.);
#20089=FACE_OUTER_BOUND('',#24112,.T.);
#20090=FACE_OUTER_BOUND('',#24113,.T.);
#20091=FACE_OUTER_BOUND('',#24114,.T.);
#20092=FACE_OUTER_BOUND('',#24115,.T.);
#20093=FACE_OUTER_BOUND('',#24116,.T.);
#20094=FACE_OUTER_BOUND('',#24117,.T.);
#20095=FACE_OUTER_BOUND('',#24118,.T.);
#20096=FACE_OUTER_BOUND('',#24119,.T.);
#20097=FACE_OUTER_BOUND('',#24120,.T.);
#20098=FACE_OUTER_BOUND('',#24121,.T.);
#20099=FACE_OUTER_BOUND('',#24122,.T.);
#20100=FACE_OUTER_BOUND('',#24123,.T.);
#20101=FACE_OUTER_BOUND('',#24124,.T.);
#20102=FACE_OUTER_BOUND('',#24125,.T.);
#20103=FACE_OUTER_BOUND('',#24126,.T.);
#20104=FACE_OUTER_BOUND('',#24127,.T.);
#20105=FACE_OUTER_BOUND('',#24128,.T.);
#20106=FACE_OUTER_BOUND('',#24129,.T.);
#20107=FACE_OUTER_BOUND('',#24130,.T.);
#20108=FACE_OUTER_BOUND('',#24131,.T.);
#20109=FACE_OUTER_BOUND('',#24132,.T.);
#20110=FACE_OUTER_BOUND('',#24133,.T.);
#20111=FACE_OUTER_BOUND('',#24134,.T.);
#20112=FACE_OUTER_BOUND('',#24135,.T.);
#20113=FACE_OUTER_BOUND('',#24136,.T.);
#20114=FACE_OUTER_BOUND('',#24137,.T.);
#20115=FACE_OUTER_BOUND('',#24138,.T.);
#20116=FACE_OUTER_BOUND('',#24139,.T.);
#20117=FACE_OUTER_BOUND('',#24140,.T.);
#20118=FACE_OUTER_BOUND('',#24141,.T.);
#20119=FACE_OUTER_BOUND('',#24142,.T.);
#20120=FACE_OUTER_BOUND('',#24143,.T.);
#20121=FACE_OUTER_BOUND('',#24144,.T.);
#20122=FACE_OUTER_BOUND('',#24145,.T.);
#20123=FACE_OUTER_BOUND('',#24146,.T.);
#20124=FACE_OUTER_BOUND('',#24147,.T.);
#20125=FACE_OUTER_BOUND('',#24148,.T.);
#20126=FACE_OUTER_BOUND('',#24149,.T.);
#20127=FACE_OUTER_BOUND('',#24150,.T.);
#20128=FACE_OUTER_BOUND('',#24151,.T.);
#20129=FACE_OUTER_BOUND('',#24152,.T.);
#20130=FACE_OUTER_BOUND('',#24153,.T.);
#20131=FACE_OUTER_BOUND('',#24154,.T.);
#20132=FACE_OUTER_BOUND('',#24155,.T.);
#20133=FACE_OUTER_BOUND('',#24156,.T.);
#20134=FACE_OUTER_BOUND('',#24157,.T.);
#20135=FACE_OUTER_BOUND('',#24158,.T.);
#20136=FACE_OUTER_BOUND('',#24159,.T.);
#20137=FACE_OUTER_BOUND('',#24160,.T.);
#20138=FACE_OUTER_BOUND('',#24161,.T.);
#20139=FACE_OUTER_BOUND('',#24162,.T.);
#20140=FACE_OUTER_BOUND('',#24163,.T.);
#20141=FACE_OUTER_BOUND('',#24164,.T.);
#20142=FACE_OUTER_BOUND('',#24165,.T.);
#20143=FACE_OUTER_BOUND('',#24166,.T.);
#20144=FACE_OUTER_BOUND('',#24168,.T.);
#20145=FACE_OUTER_BOUND('',#24169,.T.);
#20146=FACE_OUTER_BOUND('',#24170,.T.);
#20147=FACE_OUTER_BOUND('',#24171,.T.);
#20148=FACE_OUTER_BOUND('',#24172,.T.);
#20149=FACE_OUTER_BOUND('',#24173,.T.);
#20150=FACE_OUTER_BOUND('',#24174,.T.);
#20151=FACE_OUTER_BOUND('',#24176,.T.);
#20152=FACE_OUTER_BOUND('',#24177,.T.);
#20153=FACE_OUTER_BOUND('',#24178,.T.);
#20154=FACE_OUTER_BOUND('',#24179,.T.);
#20155=FACE_OUTER_BOUND('',#24181,.T.);
#20156=FACE_OUTER_BOUND('',#24182,.T.);
#20157=FACE_OUTER_BOUND('',#24183,.T.);
#20158=FACE_OUTER_BOUND('',#24184,.T.);
#20159=FACE_OUTER_BOUND('',#24185,.T.);
#20160=FACE_OUTER_BOUND('',#24186,.T.);
#20161=FACE_OUTER_BOUND('',#24187,.T.);
#20162=FACE_OUTER_BOUND('',#24188,.T.);
#20163=FACE_OUTER_BOUND('',#24189,.T.);
#20164=FACE_OUTER_BOUND('',#24190,.T.);
#20165=FACE_OUTER_BOUND('',#24191,.T.);
#20166=FACE_OUTER_BOUND('',#24192,.T.);
#20167=FACE_OUTER_BOUND('',#24193,.T.);
#20168=FACE_OUTER_BOUND('',#24194,.T.);
#20169=FACE_OUTER_BOUND('',#24195,.T.);
#20170=FACE_OUTER_BOUND('',#24196,.T.);
#20171=FACE_OUTER_BOUND('',#24197,.T.);
#20172=FACE_OUTER_BOUND('',#24198,.T.);
#20173=FACE_OUTER_BOUND('',#24199,.T.);
#20174=FACE_OUTER_BOUND('',#24200,.T.);
#20175=FACE_OUTER_BOUND('',#24201,.T.);
#20176=FACE_OUTER_BOUND('',#24202,.T.);
#20177=FACE_OUTER_BOUND('',#24203,.T.);
#20178=FACE_OUTER_BOUND('',#24204,.T.);
#20179=FACE_OUTER_BOUND('',#24205,.T.);
#20180=FACE_OUTER_BOUND('',#24206,.T.);
#20181=FACE_OUTER_BOUND('',#24207,.T.);
#20182=FACE_OUTER_BOUND('',#24208,.T.);
#20183=FACE_OUTER_BOUND('',#24209,.T.);
#20184=FACE_OUTER_BOUND('',#24210,.T.);
#20185=FACE_OUTER_BOUND('',#24211,.T.);
#20186=FACE_OUTER_BOUND('',#24212,.T.);
#20187=FACE_OUTER_BOUND('',#24213,.T.);
#20188=FACE_OUTER_BOUND('',#24214,.T.);
#20189=FACE_OUTER_BOUND('',#24215,.T.);
#20190=FACE_OUTER_BOUND('',#24216,.T.);
#20191=FACE_OUTER_BOUND('',#24217,.T.);
#20192=FACE_OUTER_BOUND('',#24218,.T.);
#20193=FACE_OUTER_BOUND('',#24219,.T.);
#20194=FACE_OUTER_BOUND('',#24220,.T.);
#20195=FACE_OUTER_BOUND('',#24221,.T.);
#20196=FACE_OUTER_BOUND('',#24222,.T.);
#20197=FACE_OUTER_BOUND('',#24223,.T.);
#20198=FACE_OUTER_BOUND('',#24224,.T.);
#20199=FACE_OUTER_BOUND('',#24225,.T.);
#20200=FACE_OUTER_BOUND('',#24226,.T.);
#20201=FACE_OUTER_BOUND('',#24227,.T.);
#20202=FACE_OUTER_BOUND('',#24228,.T.);
#20203=FACE_OUTER_BOUND('',#24229,.T.);
#20204=FACE_OUTER_BOUND('',#24230,.T.);
#20205=FACE_OUTER_BOUND('',#24231,.T.);
#20206=FACE_OUTER_BOUND('',#24232,.T.);
#20207=FACE_OUTER_BOUND('',#24233,.T.);
#20208=FACE_OUTER_BOUND('',#24234,.T.);
#20209=FACE_OUTER_BOUND('',#24235,.T.);
#20210=FACE_OUTER_BOUND('',#24236,.T.);
#20211=FACE_OUTER_BOUND('',#24237,.T.);
#20212=FACE_OUTER_BOUND('',#24238,.T.);
#20213=FACE_OUTER_BOUND('',#24239,.T.);
#20214=FACE_OUTER_BOUND('',#24240,.T.);
#20215=FACE_OUTER_BOUND('',#24241,.T.);
#20216=FACE_OUTER_BOUND('',#24243,.T.);
#20217=FACE_OUTER_BOUND('',#24245,.T.);
#20218=FACE_OUTER_BOUND('',#24246,.T.);
#20219=FACE_OUTER_BOUND('',#24247,.T.);
#20220=FACE_OUTER_BOUND('',#24248,.T.);
#20221=FACE_OUTER_BOUND('',#24249,.T.);
#20222=FACE_OUTER_BOUND('',#24250,.T.);
#20223=FACE_OUTER_BOUND('',#24251,.T.);
#20224=FACE_OUTER_BOUND('',#24252,.T.);
#20225=FACE_OUTER_BOUND('',#24253,.T.);
#20226=FACE_OUTER_BOUND('',#24254,.T.);
#20227=FACE_OUTER_BOUND('',#24255,.T.);
#20228=FACE_OUTER_BOUND('',#24256,.T.);
#20229=FACE_OUTER_BOUND('',#24257,.T.);
#20230=FACE_OUTER_BOUND('',#24258,.T.);
#20231=FACE_OUTER_BOUND('',#24259,.T.);
#20232=FACE_OUTER_BOUND('',#24260,.T.);
#20233=FACE_OUTER_BOUND('',#24261,.T.);
#20234=FACE_OUTER_BOUND('',#24262,.T.);
#20235=FACE_OUTER_BOUND('',#24263,.T.);
#20236=FACE_OUTER_BOUND('',#24264,.T.);
#20237=FACE_OUTER_BOUND('',#24265,.T.);
#20238=FACE_OUTER_BOUND('',#24266,.T.);
#20239=FACE_OUTER_BOUND('',#24268,.T.);
#20240=FACE_OUTER_BOUND('',#24270,.T.);
#20241=FACE_OUTER_BOUND('',#24272,.T.);
#20242=FACE_OUTER_BOUND('',#24273,.T.);
#20243=FACE_OUTER_BOUND('',#24274,.T.);
#20244=FACE_OUTER_BOUND('',#24275,.T.);
#20245=FACE_OUTER_BOUND('',#24276,.T.);
#20246=FACE_OUTER_BOUND('',#24277,.T.);
#20247=FACE_OUTER_BOUND('',#24278,.T.);
#20248=FACE_OUTER_BOUND('',#24279,.T.);
#20249=FACE_OUTER_BOUND('',#24280,.T.);
#20250=FACE_OUTER_BOUND('',#24281,.T.);
#20251=FACE_OUTER_BOUND('',#24282,.T.);
#20252=FACE_OUTER_BOUND('',#24283,.T.);
#20253=FACE_OUTER_BOUND('',#24284,.T.);
#20254=FACE_OUTER_BOUND('',#24285,.T.);
#20255=FACE_OUTER_BOUND('',#24286,.T.);
#20256=FACE_OUTER_BOUND('',#24287,.T.);
#20257=FACE_OUTER_BOUND('',#24288,.T.);
#20258=FACE_OUTER_BOUND('',#24289,.T.);
#20259=FACE_OUTER_BOUND('',#24290,.T.);
#20260=FACE_OUTER_BOUND('',#24291,.T.);
#20261=FACE_OUTER_BOUND('',#24292,.T.);
#20262=FACE_OUTER_BOUND('',#24293,.T.);
#20263=FACE_OUTER_BOUND('',#24294,.T.);
#20264=FACE_OUTER_BOUND('',#24295,.T.);
#20265=FACE_OUTER_BOUND('',#24296,.T.);
#20266=FACE_OUTER_BOUND('',#24297,.T.);
#20267=FACE_OUTER_BOUND('',#24298,.T.);
#20268=FACE_OUTER_BOUND('',#24299,.T.);
#20269=FACE_OUTER_BOUND('',#24300,.T.);
#20270=FACE_OUTER_BOUND('',#24301,.T.);
#20271=FACE_OUTER_BOUND('',#24302,.T.);
#20272=FACE_OUTER_BOUND('',#24303,.T.);
#20273=FACE_OUTER_BOUND('',#24304,.T.);
#20274=FACE_OUTER_BOUND('',#24305,.T.);
#20275=FACE_OUTER_BOUND('',#24306,.T.);
#20276=FACE_OUTER_BOUND('',#24307,.T.);
#20277=FACE_OUTER_BOUND('',#24308,.T.);
#20278=FACE_OUTER_BOUND('',#24309,.T.);
#20279=FACE_OUTER_BOUND('',#24310,.T.);
#20280=FACE_OUTER_BOUND('',#24311,.T.);
#20281=FACE_OUTER_BOUND('',#24312,.T.);
#20282=FACE_OUTER_BOUND('',#24313,.T.);
#20283=FACE_OUTER_BOUND('',#24314,.T.);
#20284=FACE_OUTER_BOUND('',#24315,.T.);
#20285=FACE_OUTER_BOUND('',#24316,.T.);
#20286=FACE_OUTER_BOUND('',#24317,.T.);
#20287=FACE_OUTER_BOUND('',#24318,.T.);
#20288=FACE_OUTER_BOUND('',#24319,.T.);
#20289=FACE_OUTER_BOUND('',#24320,.T.);
#20290=FACE_OUTER_BOUND('',#24321,.T.);
#20291=FACE_OUTER_BOUND('',#24322,.T.);
#20292=FACE_OUTER_BOUND('',#24323,.T.);
#20293=FACE_OUTER_BOUND('',#24324,.T.);
#20294=FACE_OUTER_BOUND('',#24325,.T.);
#20295=FACE_OUTER_BOUND('',#24326,.T.);
#20296=FACE_OUTER_BOUND('',#24327,.T.);
#20297=FACE_OUTER_BOUND('',#24328,.T.);
#20298=FACE_OUTER_BOUND('',#24329,.T.);
#20299=FACE_OUTER_BOUND('',#24330,.T.);
#20300=FACE_OUTER_BOUND('',#24331,.T.);
#20301=FACE_OUTER_BOUND('',#24332,.T.);
#20302=FACE_OUTER_BOUND('',#24333,.T.);
#20303=FACE_OUTER_BOUND('',#24334,.T.);
#20304=FACE_OUTER_BOUND('',#24335,.T.);
#20305=FACE_OUTER_BOUND('',#24336,.T.);
#20306=FACE_OUTER_BOUND('',#24337,.T.);
#20307=FACE_OUTER_BOUND('',#24338,.T.);
#20308=FACE_OUTER_BOUND('',#24340,.T.);
#20309=FACE_OUTER_BOUND('',#24342,.T.);
#20310=FACE_OUTER_BOUND('',#24343,.T.);
#20311=FACE_OUTER_BOUND('',#24344,.T.);
#20312=FACE_OUTER_BOUND('',#24345,.T.);
#20313=FACE_OUTER_BOUND('',#24346,.T.);
#20314=FACE_OUTER_BOUND('',#24347,.T.);
#20315=FACE_OUTER_BOUND('',#24348,.T.);
#20316=FACE_OUTER_BOUND('',#24349,.T.);
#20317=FACE_OUTER_BOUND('',#24350,.T.);
#20318=FACE_OUTER_BOUND('',#24351,.T.);
#20319=FACE_OUTER_BOUND('',#24352,.T.);
#20320=FACE_OUTER_BOUND('',#24353,.T.);
#20321=FACE_OUTER_BOUND('',#24354,.T.);
#20322=FACE_OUTER_BOUND('',#24355,.T.);
#20323=FACE_OUTER_BOUND('',#24356,.T.);
#20324=FACE_OUTER_BOUND('',#24357,.T.);
#20325=FACE_OUTER_BOUND('',#24358,.T.);
#20326=FACE_OUTER_BOUND('',#24359,.T.);
#20327=FACE_OUTER_BOUND('',#24360,.T.);
#20328=FACE_OUTER_BOUND('',#24361,.T.);
#20329=FACE_OUTER_BOUND('',#24362,.T.);
#20330=FACE_OUTER_BOUND('',#24363,.T.);
#20331=FACE_OUTER_BOUND('',#24364,.T.);
#20332=FACE_OUTER_BOUND('',#24365,.T.);
#20333=FACE_OUTER_BOUND('',#24366,.T.);
#20334=FACE_OUTER_BOUND('',#24367,.T.);
#20335=FACE_OUTER_BOUND('',#24368,.T.);
#20336=FACE_OUTER_BOUND('',#24369,.T.);
#20337=FACE_OUTER_BOUND('',#24370,.T.);
#20338=FACE_OUTER_BOUND('',#24371,.T.);
#20339=FACE_OUTER_BOUND('',#24372,.T.);
#20340=FACE_OUTER_BOUND('',#24373,.T.);
#20341=FACE_OUTER_BOUND('',#24374,.T.);
#20342=FACE_OUTER_BOUND('',#24375,.T.);
#20343=FACE_OUTER_BOUND('',#24376,.T.);
#20344=FACE_OUTER_BOUND('',#24377,.T.);
#20345=FACE_OUTER_BOUND('',#24378,.T.);
#20346=FACE_OUTER_BOUND('',#24379,.T.);
#20347=FACE_OUTER_BOUND('',#24380,.T.);
#20348=FACE_OUTER_BOUND('',#24381,.T.);
#20349=FACE_OUTER_BOUND('',#24382,.T.);
#20350=FACE_OUTER_BOUND('',#24383,.T.);
#20351=FACE_OUTER_BOUND('',#24384,.T.);
#20352=FACE_OUTER_BOUND('',#24385,.T.);
#20353=FACE_OUTER_BOUND('',#24386,.T.);
#20354=FACE_OUTER_BOUND('',#24387,.T.);
#20355=FACE_OUTER_BOUND('',#24388,.T.);
#20356=FACE_OUTER_BOUND('',#24389,.T.);
#20357=FACE_OUTER_BOUND('',#24390,.T.);
#20358=FACE_OUTER_BOUND('',#24391,.T.);
#20359=FACE_OUTER_BOUND('',#24392,.T.);
#20360=FACE_OUTER_BOUND('',#24393,.T.);
#20361=FACE_OUTER_BOUND('',#24395,.T.);
#20362=FACE_OUTER_BOUND('',#24396,.T.);
#20363=FACE_OUTER_BOUND('',#24397,.T.);
#20364=FACE_OUTER_BOUND('',#24398,.T.);
#20365=FACE_OUTER_BOUND('',#24399,.T.);
#20366=FACE_OUTER_BOUND('',#24400,.T.);
#20367=FACE_OUTER_BOUND('',#24401,.T.);
#20368=FACE_OUTER_BOUND('',#24402,.T.);
#20369=FACE_OUTER_BOUND('',#24403,.T.);
#20370=FACE_OUTER_BOUND('',#24404,.T.);
#20371=FACE_OUTER_BOUND('',#24405,.T.);
#20372=FACE_OUTER_BOUND('',#24406,.T.);
#20373=FACE_OUTER_BOUND('',#24407,.T.);
#20374=FACE_OUTER_BOUND('',#24408,.T.);
#20375=FACE_OUTER_BOUND('',#24409,.T.);
#20376=FACE_OUTER_BOUND('',#24410,.T.);
#20377=FACE_OUTER_BOUND('',#24411,.T.);
#20378=FACE_OUTER_BOUND('',#24412,.T.);
#20379=FACE_OUTER_BOUND('',#24413,.T.);
#20380=FACE_OUTER_BOUND('',#24414,.T.);
#20381=FACE_OUTER_BOUND('',#24415,.T.);
#20382=FACE_OUTER_BOUND('',#24416,.T.);
#20383=FACE_OUTER_BOUND('',#24417,.T.);
#20384=FACE_OUTER_BOUND('',#24418,.T.);
#20385=FACE_OUTER_BOUND('',#24419,.T.);
#20386=FACE_OUTER_BOUND('',#24420,.T.);
#20387=FACE_OUTER_BOUND('',#24421,.T.);
#20388=FACE_OUTER_BOUND('',#24422,.T.);
#20389=FACE_OUTER_BOUND('',#24423,.T.);
#20390=FACE_OUTER_BOUND('',#24424,.T.);
#20391=FACE_OUTER_BOUND('',#24426,.T.);
#20392=FACE_OUTER_BOUND('',#24427,.T.);
#20393=FACE_OUTER_BOUND('',#24428,.T.);
#20394=FACE_OUTER_BOUND('',#24429,.T.);
#20395=FACE_OUTER_BOUND('',#24430,.T.);
#20396=FACE_OUTER_BOUND('',#24431,.T.);
#20397=FACE_OUTER_BOUND('',#24432,.T.);
#20398=FACE_OUTER_BOUND('',#24433,.T.);
#20399=FACE_OUTER_BOUND('',#24434,.T.);
#20400=FACE_OUTER_BOUND('',#24435,.T.);
#20401=FACE_OUTER_BOUND('',#24436,.T.);
#20402=FACE_OUTER_BOUND('',#24437,.T.);
#20403=FACE_OUTER_BOUND('',#24438,.T.);
#20404=FACE_OUTER_BOUND('',#24439,.T.);
#20405=FACE_OUTER_BOUND('',#24440,.T.);
#20406=FACE_OUTER_BOUND('',#24441,.T.);
#20407=FACE_OUTER_BOUND('',#24442,.T.);
#20408=FACE_OUTER_BOUND('',#24443,.T.);
#20409=FACE_OUTER_BOUND('',#24444,.T.);
#20410=FACE_OUTER_BOUND('',#24445,.T.);
#20411=FACE_OUTER_BOUND('',#24446,.T.);
#20412=FACE_OUTER_BOUND('',#24447,.T.);
#20413=FACE_OUTER_BOUND('',#24448,.T.);
#20414=FACE_OUTER_BOUND('',#24449,.T.);
#20415=FACE_OUTER_BOUND('',#24450,.T.);
#20416=FACE_OUTER_BOUND('',#24451,.T.);
#20417=FACE_OUTER_BOUND('',#24452,.T.);
#20418=FACE_OUTER_BOUND('',#24453,.T.);
#20419=FACE_OUTER_BOUND('',#24454,.T.);
#20420=FACE_OUTER_BOUND('',#24456,.T.);
#20421=FACE_OUTER_BOUND('',#24457,.T.);
#20422=FACE_OUTER_BOUND('',#24458,.T.);
#20423=FACE_OUTER_BOUND('',#24459,.T.);
#20424=FACE_OUTER_BOUND('',#24460,.T.);
#20425=FACE_OUTER_BOUND('',#24461,.T.);
#20426=FACE_OUTER_BOUND('',#24462,.T.);
#20427=FACE_OUTER_BOUND('',#24463,.T.);
#20428=FACE_OUTER_BOUND('',#24464,.T.);
#20429=FACE_OUTER_BOUND('',#24465,.T.);
#20430=FACE_OUTER_BOUND('',#24466,.T.);
#20431=FACE_OUTER_BOUND('',#24467,.T.);
#20432=FACE_OUTER_BOUND('',#24468,.T.);
#20433=FACE_OUTER_BOUND('',#24469,.T.);
#20434=FACE_OUTER_BOUND('',#24470,.T.);
#20435=FACE_OUTER_BOUND('',#24471,.T.);
#20436=FACE_OUTER_BOUND('',#24472,.T.);
#20437=FACE_OUTER_BOUND('',#24473,.T.);
#20438=FACE_OUTER_BOUND('',#24475,.T.);
#20439=FACE_OUTER_BOUND('',#24476,.T.);
#20440=FACE_OUTER_BOUND('',#24477,.T.);
#20441=FACE_OUTER_BOUND('',#24479,.T.);
#20442=FACE_OUTER_BOUND('',#24481,.T.);
#20443=FACE_OUTER_BOUND('',#24482,.T.);
#20444=FACE_OUTER_BOUND('',#24483,.T.);
#20445=FACE_OUTER_BOUND('',#24484,.T.);
#20446=FACE_OUTER_BOUND('',#24485,.T.);
#20447=FACE_OUTER_BOUND('',#24486,.T.);
#20448=FACE_OUTER_BOUND('',#24487,.T.);
#20449=FACE_OUTER_BOUND('',#24488,.T.);
#20450=FACE_OUTER_BOUND('',#24489,.T.);
#20451=FACE_OUTER_BOUND('',#24490,.T.);
#20452=FACE_OUTER_BOUND('',#24491,.T.);
#20453=FACE_OUTER_BOUND('',#24492,.T.);
#20454=FACE_OUTER_BOUND('',#24493,.T.);
#20455=FACE_OUTER_BOUND('',#24494,.T.);
#20456=FACE_OUTER_BOUND('',#24495,.T.);
#20457=FACE_OUTER_BOUND('',#24496,.T.);
#20458=FACE_OUTER_BOUND('',#24497,.T.);
#20459=FACE_OUTER_BOUND('',#24498,.T.);
#20460=FACE_OUTER_BOUND('',#24499,.T.);
#20461=FACE_OUTER_BOUND('',#24500,.T.);
#20462=FACE_OUTER_BOUND('',#24501,.T.);
#20463=FACE_OUTER_BOUND('',#24502,.T.);
#20464=FACE_OUTER_BOUND('',#24503,.T.);
#20465=FACE_OUTER_BOUND('',#24504,.T.);
#20466=FACE_OUTER_BOUND('',#24505,.T.);
#20467=FACE_OUTER_BOUND('',#24506,.T.);
#20468=FACE_OUTER_BOUND('',#24507,.T.);
#20469=FACE_OUTER_BOUND('',#24508,.T.);
#20470=FACE_OUTER_BOUND('',#24509,.T.);
#20471=FACE_OUTER_BOUND('',#24510,.T.);
#20472=FACE_OUTER_BOUND('',#24511,.T.);
#20473=FACE_OUTER_BOUND('',#24512,.T.);
#20474=FACE_OUTER_BOUND('',#24513,.T.);
#20475=FACE_OUTER_BOUND('',#24514,.T.);
#20476=FACE_OUTER_BOUND('',#24515,.T.);
#20477=FACE_OUTER_BOUND('',#24516,.T.);
#20478=FACE_OUTER_BOUND('',#24517,.T.);
#20479=FACE_OUTER_BOUND('',#24518,.T.);
#20480=FACE_OUTER_BOUND('',#24519,.T.);
#20481=FACE_OUTER_BOUND('',#24520,.T.);
#20482=FACE_OUTER_BOUND('',#24521,.T.);
#20483=FACE_OUTER_BOUND('',#24522,.T.);
#20484=FACE_OUTER_BOUND('',#24523,.T.);
#20485=FACE_OUTER_BOUND('',#24524,.T.);
#20486=FACE_OUTER_BOUND('',#24525,.T.);
#20487=FACE_OUTER_BOUND('',#24526,.T.);
#20488=FACE_OUTER_BOUND('',#24527,.T.);
#20489=FACE_OUTER_BOUND('',#24528,.T.);
#20490=FACE_OUTER_BOUND('',#24529,.T.);
#20491=FACE_OUTER_BOUND('',#24530,.T.);
#20492=FACE_OUTER_BOUND('',#24531,.T.);
#20493=FACE_OUTER_BOUND('',#24532,.T.);
#20494=FACE_OUTER_BOUND('',#24533,.T.);
#20495=FACE_OUTER_BOUND('',#24534,.T.);
#20496=FACE_OUTER_BOUND('',#24535,.T.);
#20497=FACE_OUTER_BOUND('',#24536,.T.);
#20498=FACE_OUTER_BOUND('',#24537,.T.);
#20499=FACE_OUTER_BOUND('',#24538,.T.);
#20500=FACE_OUTER_BOUND('',#24539,.T.);
#20501=FACE_OUTER_BOUND('',#24540,.T.);
#20502=FACE_OUTER_BOUND('',#24541,.T.);
#20503=FACE_OUTER_BOUND('',#24542,.T.);
#20504=FACE_OUTER_BOUND('',#24543,.T.);
#20505=FACE_OUTER_BOUND('',#24544,.T.);
#20506=FACE_OUTER_BOUND('',#24545,.T.);
#20507=FACE_OUTER_BOUND('',#24546,.T.);
#20508=FACE_OUTER_BOUND('',#24547,.T.);
#20509=FACE_OUTER_BOUND('',#24548,.T.);
#20510=FACE_OUTER_BOUND('',#24549,.T.);
#20511=FACE_OUTER_BOUND('',#24550,.T.);
#20512=FACE_OUTER_BOUND('',#24551,.T.);
#20513=FACE_OUTER_BOUND('',#24552,.T.);
#20514=FACE_OUTER_BOUND('',#24553,.T.);
#23888=EDGE_LOOP('',(#52473,#52474,#52475,#52476));
#23889=EDGE_LOOP('',(#52477,#52478,#52479));
#23890=EDGE_LOOP('',(#52480,#52481,#52482));
#23891=EDGE_LOOP('',(#52483,#52484,#52485));
#23892=EDGE_LOOP('',(#52486,#52487,#52488,#52489));
#23893=EDGE_LOOP('',(#52490,#52491,#52492));
#23894=EDGE_LOOP('',(#52493,#52494,#52495,#52496,#52497,#52498));
#23895=EDGE_LOOP('',(#52499,#52500,#52501,#52502));
#23896=EDGE_LOOP('',(#52503,#52504,#52505));
#23897=EDGE_LOOP('',(#52506,#52507,#52508));
#23898=EDGE_LOOP('',(#52509,#52510,#52511,#52512));
#23899=EDGE_LOOP('',(#52513,#52514,#52515));
#23900=EDGE_LOOP('',(#52516,#52517,#52518));
#23901=EDGE_LOOP('',(#52519,#52520,#52521,#52522,#52523,#52524));
#23902=EDGE_LOOP('',(#52525,#52526,#52527,#52528,#52529,#52530,#52531));
#23903=EDGE_LOOP('',(#52532,#52533,#52534,#52535));
#23904=EDGE_LOOP('',(#52536,#52537,#52538));
#23905=EDGE_LOOP('',(#52539,#52540,#52541,#52542));
#23906=EDGE_LOOP('',(#52543,#52544,#52545,#52546));
#23907=EDGE_LOOP('',(#52547,#52548,#52549,#52550));
#23908=EDGE_LOOP('',(#52551,#52552,#52553));
#23909=EDGE_LOOP('',(#52554,#52555,#52556,#52557));
#23910=EDGE_LOOP('',(#52558,#52559,#52560,#52561));
#23911=EDGE_LOOP('',(#52562,#52563,#52564));
#23912=EDGE_LOOP('',(#52565,#52566,#52567,#52568,#52569,#52570,#52571));
#23913=EDGE_LOOP('',(#52572,#52573,#52574));
#23914=EDGE_LOOP('',(#52575,#52576,#52577,#52578));
#23915=EDGE_LOOP('',(#52579,#52580,#52581,#52582));
#23916=EDGE_LOOP('',(#52583,#52584,#52585,#52586));
#23917=EDGE_LOOP('',(#52587,#52588,#52589,#52590));
#23918=EDGE_LOOP('',(#52591,#52592,#52593));
#23919=EDGE_LOOP('',(#52594,#52595,#52596,#52597));
#23920=EDGE_LOOP('',(#52598,#52599,#52600,#52601));
#23921=EDGE_LOOP('',(#52602,#52603,#52604));
#23922=EDGE_LOOP('',(#52605,#52606,#52607,#52608));
#23923=EDGE_LOOP('',(#52609,#52610,#52611,#52612,#52613,#52614));
#23924=EDGE_LOOP('',(#52615,#52616,#52617,#52618,#52619));
#23925=EDGE_LOOP('',(#52620,#52621,#52622,#52623,#52624));
#23926=EDGE_LOOP('',(#52625,#52626,#52627,#52628,#52629));
#23927=EDGE_LOOP('',(#52630,#52631,#52632,#52633));
#23928=EDGE_LOOP('',(#52634,#52635,#52636,#52637));
#23929=EDGE_LOOP('',(#52638,#52639,#52640,#52641));
#23930=EDGE_LOOP('',(#52642,#52643,#52644,#52645));
#23931=EDGE_LOOP('',(#52646,#52647,#52648,#52649));
#23932=EDGE_LOOP('',(#52650,#52651,#52652));
#23933=EDGE_LOOP('',(#52653,#52654,#52655,#52656,#52657,#52658,#52659,#52660,
#52661));
#23934=EDGE_LOOP('',(#52662,#52663,#52664,#52665));
#23935=EDGE_LOOP('',(#52666,#52667,#52668,#52669));
#23936=EDGE_LOOP('',(#52670,#52671,#52672,#52673));
#23937=EDGE_LOOP('',(#52674,#52675,#52676,#52677,#52678,#52679,#52680,#52681,
#52682,#52683,#52684,#52685,#52686,#52687,#52688,#52689,#52690,#52691,#52692,
#52693));
#23938=EDGE_LOOP('',(#52694,#52695,#52696,#52697,#52698,#52699));
#23939=EDGE_LOOP('',(#52700,#52701,#52702,#52703,#52704));
#23940=EDGE_LOOP('',(#52705,#52706,#52707,#52708,#52709));
#23941=EDGE_LOOP('',(#52710,#52711,#52712,#52713));
#23942=EDGE_LOOP('',(#52714,#52715,#52716,#52717,#52718));
#23943=EDGE_LOOP('',(#52719,#52720,#52721,#52722,#52723));
#23944=EDGE_LOOP('',(#52724,#52725,#52726,#52727,#52728));
#23945=EDGE_LOOP('',(#52729,#52730,#52731,#52732,#52733));
#23946=EDGE_LOOP('',(#52734,#52735,#52736,#52737));
#23947=EDGE_LOOP('',(#52738,#52739,#52740,#52741,#52742));
#23948=EDGE_LOOP('',(#52743,#52744,#52745,#52746,#52747,#52748,#52749,#52750,
#52751,#52752,#52753,#52754,#52755,#52756,#52757,#52758,#52759,#52760,#52761,
#52762,#52763));
#23949=EDGE_LOOP('',(#52764,#52765,#52766,#52767));
#23950=EDGE_LOOP('',(#52768,#52769,#52770,#52771,#52772,#52773,#52774,#52775,
#52776,#52777));
#23951=EDGE_LOOP('',(#52778,#52779,#52780,#52781,#52782,#52783));
#23952=EDGE_LOOP('',(#52784,#52785,#52786,#52787,#52788,#52789,#52790));
#23953=EDGE_LOOP('',(#52791,#52792,#52793,#52794,#52795));
#23954=EDGE_LOOP('',(#52796,#52797,#52798,#52799,#52800));
#23955=EDGE_LOOP('',(#52801,#52802,#52803,#52804,#52805,#52806));
#23956=EDGE_LOOP('',(#52807,#52808,#52809,#52810,#52811,#52812,#52813,#52814));
#23957=EDGE_LOOP('',(#52815,#52816,#52817,#52818,#52819));
#23958=EDGE_LOOP('',(#52820,#52821,#52822,#52823,#52824));
#23959=EDGE_LOOP('',(#52825,#52826,#52827,#52828));
#23960=EDGE_LOOP('',(#52829,#52830,#52831,#52832,#52833,#52834,#52835,#52836,
#52837));
#23961=EDGE_LOOP('',(#52838,#52839,#52840,#52841,#52842));
#23962=EDGE_LOOP('',(#52843,#52844,#52845,#52846,#52847));
#23963=EDGE_LOOP('',(#52848,#52849,#52850,#52851,#52852));
#23964=EDGE_LOOP('',(#52853,#52854,#52855,#52856,#52857,#52858));
#23965=EDGE_LOOP('',(#52859,#52860,#52861,#52862));
#23966=EDGE_LOOP('',(#52863,#52864,#52865,#52866));
#23967=EDGE_LOOP('',(#52867,#52868,#52869,#52870));
#23968=EDGE_LOOP('',(#52871,#52872,#52873,#52874,#52875));
#23969=EDGE_LOOP('',(#52876,#52877,#52878,#52879,#52880,#52881));
#23970=EDGE_LOOP('',(#52882,#52883,#52884,#52885,#52886,#52887,#52888,#52889,
#52890));
#23971=EDGE_LOOP('',(#52891,#52892,#52893,#52894,#52895));
#23972=EDGE_LOOP('',(#52896,#52897,#52898,#52899,#52900));
#23973=EDGE_LOOP('',(#52901,#52902,#52903,#52904,#52905));
#23974=EDGE_LOOP('',(#52906,#52907,#52908,#52909,#52910,#52911));
#23975=EDGE_LOOP('',(#52912,#52913,#52914,#52915,#52916,#52917));
#23976=EDGE_LOOP('',(#52918,#52919,#52920,#52921,#52922,#52923,#52924,#52925,
#52926,#52927,#52928,#52929));
#23977=EDGE_LOOP('',(#52930,#52931,#52932,#52933,#52934,#52935,#52936));
#23978=EDGE_LOOP('',(#52937,#52938,#52939,#52940,#52941));
#23979=EDGE_LOOP('',(#52942,#52943,#52944,#52945));
#23980=EDGE_LOOP('',(#52946,#52947,#52948,#52949,#52950));
#23981=EDGE_LOOP('',(#52951,#52952,#52953,#52954,#52955));
#23982=EDGE_LOOP('',(#52956,#52957,#52958,#52959,#52960,#52961));
#23983=EDGE_LOOP('',(#52962,#52963,#52964,#52965,#52966,#52967,#52968,#52969,
#52970,#52971,#52972));
#23984=EDGE_LOOP('',(#52973,#52974,#52975,#52976,#52977));
#23985=EDGE_LOOP('',(#52978,#52979,#52980,#52981,#52982));
#23986=EDGE_LOOP('',(#52983,#52984,#52985,#52986,#52987));
#23987=EDGE_LOOP('',(#52988,#52989,#52990,#52991,#52992,#52993));
#23988=EDGE_LOOP('',(#52994,#52995,#52996,#52997,#52998));
#23989=EDGE_LOOP('',(#52999,#53000,#53001,#53002,#53003,#53004,#53005,#53006,
#53007,#53008,#53009,#53010));
#23990=EDGE_LOOP('',(#53011,#53012,#53013,#53014,#53015,#53016,#53017));
#23991=EDGE_LOOP('',(#53018,#53019,#53020,#53021,#53022));
#23992=EDGE_LOOP('',(#53023,#53024,#53025,#53026));
#23993=EDGE_LOOP('',(#53027,#53028,#53029,#53030,#53031));
#23994=EDGE_LOOP('',(#53032,#53033,#53034,#53035,#53036));
#23995=EDGE_LOOP('',(#53037,#53038,#53039,#53040,#53041,#53042));
#23996=EDGE_LOOP('',(#53043,#53044,#53045,#53046,#53047,#53048,#53049,#53050,
#53051,#53052,#53053));
#23997=EDGE_LOOP('',(#53054,#53055,#53056,#53057,#53058));
#23998=EDGE_LOOP('',(#53059));
#23999=EDGE_LOOP('',(#53060,#53061,#53062,#53063,#53064,#53065));
#24000=EDGE_LOOP('',(#53066,#53067,#53068,#53069));
#24001=EDGE_LOOP('',(#53070,#53071,#53072,#53073));
#24002=EDGE_LOOP('',(#53074,#53075,#53076,#53077));
#24003=EDGE_LOOP('',(#53078,#53079,#53080,#53081));
#24004=EDGE_LOOP('',(#53082,#53083,#53084,#53085,#53086));
#24005=EDGE_LOOP('',(#53087,#53088,#53089,#53090));
#24006=EDGE_LOOP('',(#53091));
#24007=EDGE_LOOP('',(#53092));
#24008=EDGE_LOOP('',(#53093));
#24009=EDGE_LOOP('',(#53094));
#24010=EDGE_LOOP('',(#53095,#53096,#53097,#53098));
#24011=EDGE_LOOP('',(#53099,#53100,#53101));
#24012=EDGE_LOOP('',(#53102,#53103,#53104,#53105,#53106));
#24013=EDGE_LOOP('',(#53107,#53108,#53109,#53110));
#24014=EDGE_LOOP('',(#53111,#53112,#53113));
#24015=EDGE_LOOP('',(#53114,#53115,#53116,#53117,#53118));
#24016=EDGE_LOOP('',(#53119,#53120,#53121));
#24017=EDGE_LOOP('',(#53122,#53123,#53124,#53125));
#24018=EDGE_LOOP('',(#53126,#53127,#53128,#53129));
#24019=EDGE_LOOP('',(#53130,#53131,#53132,#53133,#53134,#53135,#53136));
#24020=EDGE_LOOP('',(#53137,#53138,#53139,#53140));
#24021=EDGE_LOOP('',(#53141,#53142,#53143,#53144));
#24022=EDGE_LOOP('',(#53145,#53146,#53147,#53148,#53149,#53150,#53151,#53152));
#24023=EDGE_LOOP('',(#53153,#53154,#53155,#53156));
#24024=EDGE_LOOP('',(#53157,#53158,#53159,#53160));
#24025=EDGE_LOOP('',(#53161,#53162,#53163,#53164,#53165));
#24026=EDGE_LOOP('',(#53166,#53167,#53168,#53169));
#24027=EDGE_LOOP('',(#53170,#53171,#53172,#53173,#53174,#53175));
#24028=EDGE_LOOP('',(#53176,#53177,#53178,#53179));
#24029=EDGE_LOOP('',(#53180,#53181,#53182,#53183));
#24030=EDGE_LOOP('',(#53184,#53185,#53186,#53187));
#24031=EDGE_LOOP('',(#53188,#53189,#53190,#53191,#53192,#53193));
#24032=EDGE_LOOP('',(#53194,#53195,#53196,#53197));
#24033=EDGE_LOOP('',(#53198,#53199,#53200,#53201,#53202));
#24034=EDGE_LOOP('',(#53203,#53204,#53205,#53206));
#24035=EDGE_LOOP('',(#53207,#53208,#53209,#53210,#53211));
#24036=EDGE_LOOP('',(#53212,#53213,#53214,#53215,#53216,#53217,#53218));
#24037=EDGE_LOOP('',(#53219,#53220,#53221));
#24038=EDGE_LOOP('',(#53222,#53223,#53224,#53225,#53226,#53227,#53228));
#24039=EDGE_LOOP('',(#53229,#53230,#53231,#53232));
#24040=EDGE_LOOP('',(#53233,#53234,#53235,#53236,#53237));
#24041=EDGE_LOOP('',(#53238,#53239,#53240));
#24042=EDGE_LOOP('',(#53241,#53242,#53243,#53244));
#24043=EDGE_LOOP('',(#53245,#53246,#53247));
#24044=EDGE_LOOP('',(#53248,#53249,#53250,#53251));
#24045=EDGE_LOOP('',(#53252,#53253,#53254,#53255));
#24046=EDGE_LOOP('',(#53256,#53257,#53258,#53259,#53260,#53261));
#24047=EDGE_LOOP('',(#53262,#53263,#53264,#53265));
#24048=EDGE_LOOP('',(#53266,#53267,#53268,#53269,#53270));
#24049=EDGE_LOOP('',(#53271,#53272,#53273));
#24050=EDGE_LOOP('',(#53274,#53275,#53276,#53277));
#24051=EDGE_LOOP('',(#53278,#53279,#53280,#53281));
#24052=EDGE_LOOP('',(#53282,#53283,#53284,#53285));
#24053=EDGE_LOOP('',(#53286,#53287,#53288,#53289));
#24054=EDGE_LOOP('',(#53290,#53291,#53292,#53293,#53294));
#24055=EDGE_LOOP('',(#53295,#53296,#53297,#53298,#53299,#53300,#53301));
#24056=EDGE_LOOP('',(#53302,#53303,#53304));
#24057=EDGE_LOOP('',(#53305,#53306,#53307,#53308,#53309,#53310));
#24058=EDGE_LOOP('',(#53311,#53312,#53313));
#24059=EDGE_LOOP('',(#53314,#53315,#53316,#53317,#53318,#53319,#53320,#53321,
#53322));
#24060=EDGE_LOOP('',(#53323,#53324,#53325,#53326,#53327));
#24061=EDGE_LOOP('',(#53328,#53329,#53330,#53331));
#24062=EDGE_LOOP('',(#53332,#53333,#53334,#53335));
#24063=EDGE_LOOP('',(#53336,#53337,#53338,#53339));
#24064=EDGE_LOOP('',(#53340,#53341,#53342,#53343));
#24065=EDGE_LOOP('',(#53344,#53345,#53346,#53347));
#24066=EDGE_LOOP('',(#53348,#53349,#53350,#53351));
#24067=EDGE_LOOP('',(#53352,#53353,#53354,#53355));
#24068=EDGE_LOOP('',(#53356,#53357,#53358,#53359));
#24069=EDGE_LOOP('',(#53360,#53361,#53362,#53363));
#24070=EDGE_LOOP('',(#53364,#53365,#53366,#53367));
#24071=EDGE_LOOP('',(#53368,#53369,#53370,#53371));
#24072=EDGE_LOOP('',(#53372,#53373,#53374,#53375));
#24073=EDGE_LOOP('',(#53376,#53377,#53378,#53379));
#24074=EDGE_LOOP('',(#53380,#53381,#53382,#53383));
#24075=EDGE_LOOP('',(#53384,#53385,#53386,#53387));
#24076=EDGE_LOOP('',(#53388,#53389,#53390,#53391));
#24077=EDGE_LOOP('',(#53392));
#24078=EDGE_LOOP('',(#53393,#53394,#53395,#53396));
#24079=EDGE_LOOP('',(#53397,#53398,#53399,#53400,#53401,#53402));
#24080=EDGE_LOOP('',(#53403,#53404,#53405,#53406));
#24081=EDGE_LOOP('',(#53407,#53408,#53409,#53410,#53411,#53412));
#24082=EDGE_LOOP('',(#53413,#53414,#53415,#53416,#53417,#53418,#53419,#53420));
#24083=EDGE_LOOP('',(#53421,#53422,#53423,#53424));
#24084=EDGE_LOOP('',(#53425,#53426,#53427,#53428,#53429,#53430,#53431,#53432));
#24085=EDGE_LOOP('',(#53433));
#24086=EDGE_LOOP('',(#53434,#53435,#53436,#53437));
#24087=EDGE_LOOP('',(#53438));
#24088=EDGE_LOOP('',(#53439,#53440,#53441,#53442,#53443,#53444));
#24089=EDGE_LOOP('',(#53445,#53446,#53447,#53448));
#24090=EDGE_LOOP('',(#53449,#53450,#53451,#53452));
#24091=EDGE_LOOP('',(#53453,#53454,#53455,#53456));
#24092=EDGE_LOOP('',(#53457,#53458,#53459,#53460));
#24093=EDGE_LOOP('',(#53461,#53462,#53463,#53464,#53465));
#24094=EDGE_LOOP('',(#53466,#53467,#53468,#53469));
#24095=EDGE_LOOP('',(#53470));
#24096=EDGE_LOOP('',(#53471));
#24097=EDGE_LOOP('',(#53472));
#24098=EDGE_LOOP('',(#53473));
#24099=EDGE_LOOP('',(#53474,#53475,#53476));
#24100=EDGE_LOOP('',(#53477,#53478,#53479,#53480));
#24101=EDGE_LOOP('',(#53481,#53482,#53483,#53484,#53485));
#24102=EDGE_LOOP('',(#53486,#53487,#53488,#53489));
#24103=EDGE_LOOP('',(#53490,#53491,#53492,#53493));
#24104=EDGE_LOOP('',(#53494,#53495,#53496,#53497));
#24105=EDGE_LOOP('',(#53498,#53499,#53500,#53501));
#24106=EDGE_LOOP('',(#53502,#53503,#53504,#53505));
#24107=EDGE_LOOP('',(#53506,#53507,#53508,#53509));
#24108=EDGE_LOOP('',(#53510,#53511,#53512,#53513,#53514));
#24109=EDGE_LOOP('',(#53515,#53516,#53517));
#24110=EDGE_LOOP('',(#53518,#53519,#53520));
#24111=EDGE_LOOP('',(#53521,#53522,#53523,#53524));
#24112=EDGE_LOOP('',(#53525,#53526,#53527,#53528,#53529,#53530,#53531));
#24113=EDGE_LOOP('',(#53532,#53533,#53534,#53535,#53536,#53537,#53538,#53539));
#24114=EDGE_LOOP('',(#53540,#53541,#53542,#53543,#53544));
#24115=EDGE_LOOP('',(#53545,#53546,#53547,#53548,#53549,#53550));
#24116=EDGE_LOOP('',(#53551,#53552,#53553,#53554));
#24117=EDGE_LOOP('',(#53555,#53556,#53557,#53558));
#24118=EDGE_LOOP('',(#53559,#53560,#53561,#53562,#53563));
#24119=EDGE_LOOP('',(#53564,#53565,#53566));
#24120=EDGE_LOOP('',(#53567,#53568,#53569,#53570,#53571,#53572,#53573));
#24121=EDGE_LOOP('',(#53574,#53575,#53576));
#24122=EDGE_LOOP('',(#53577,#53578,#53579,#53580,#53581,#53582,#53583));
#24123=EDGE_LOOP('',(#53584,#53585,#53586,#53587,#53588));
#24124=EDGE_LOOP('',(#53589,#53590,#53591,#53592));
#24125=EDGE_LOOP('',(#53593,#53594,#53595,#53596,#53597));
#24126=EDGE_LOOP('',(#53598,#53599,#53600,#53601));
#24127=EDGE_LOOP('',(#53602,#53603,#53604,#53605,#53606,#53607));
#24128=EDGE_LOOP('',(#53608,#53609,#53610,#53611));
#24129=EDGE_LOOP('',(#53612,#53613,#53614,#53615));
#24130=EDGE_LOOP('',(#53616,#53617,#53618,#53619));
#24131=EDGE_LOOP('',(#53620,#53621,#53622,#53623));
#24132=EDGE_LOOP('',(#53624,#53625,#53626));
#24133=EDGE_LOOP('',(#53627,#53628,#53629,#53630));
#24134=EDGE_LOOP('',(#53631,#53632,#53633,#53634,#53635));
#24135=EDGE_LOOP('',(#53636,#53637,#53638,#53639));
#24136=EDGE_LOOP('',(#53640,#53641,#53642,#53643));
#24137=EDGE_LOOP('',(#53644,#53645,#53646,#53647));
#24138=EDGE_LOOP('',(#53648,#53649,#53650,#53651));
#24139=EDGE_LOOP('',(#53652,#53653,#53654));
#24140=EDGE_LOOP('',(#53655,#53656,#53657,#53658,#53659));
#24141=EDGE_LOOP('',(#53660,#53661,#53662,#53663));
#24142=EDGE_LOOP('',(#53664,#53665,#53666,#53667,#53668,#53669));
#24143=EDGE_LOOP('',(#53670,#53671,#53672,#53673));
#24144=EDGE_LOOP('',(#53674,#53675,#53676,#53677,#53678,#53679,#53680));
#24145=EDGE_LOOP('',(#53681,#53682,#53683,#53684,#53685,#53686,#53687,#53688,
#53689));
#24146=EDGE_LOOP('',(#53690,#53691,#53692));
#24147=EDGE_LOOP('',(#53693,#53694,#53695,#53696,#53697,#53698,#53699));
#24148=EDGE_LOOP('',(#53700,#53701,#53702));
#24149=EDGE_LOOP('',(#53703,#53704,#53705,#53706,#53707));
#24150=EDGE_LOOP('',(#53708,#53709,#53710,#53711,#53712));
#24151=EDGE_LOOP('',(#53713,#53714,#53715,#53716));
#24152=EDGE_LOOP('',(#53717,#53718,#53719,#53720));
#24153=EDGE_LOOP('',(#53721,#53722,#53723,#53724));
#24154=EDGE_LOOP('',(#53725,#53726,#53727,#53728));
#24155=EDGE_LOOP('',(#53729,#53730,#53731,#53732));
#24156=EDGE_LOOP('',(#53733,#53734,#53735,#53736));
#24157=EDGE_LOOP('',(#53737,#53738,#53739,#53740));
#24158=EDGE_LOOP('',(#53741,#53742,#53743,#53744));
#24159=EDGE_LOOP('',(#53745,#53746,#53747,#53748));
#24160=EDGE_LOOP('',(#53749,#53750,#53751,#53752));
#24161=EDGE_LOOP('',(#53753,#53754,#53755,#53756));
#24162=EDGE_LOOP('',(#53757,#53758,#53759,#53760));
#24163=EDGE_LOOP('',(#53761,#53762,#53763,#53764));
#24164=EDGE_LOOP('',(#53765,#53766,#53767,#53768));
#24165=EDGE_LOOP('',(#53769,#53770,#53771,#53772));
#24166=EDGE_LOOP('',(#53773));
#24167=EDGE_LOOP('',(#53774,#53775,#53776,#53777));
#24168=EDGE_LOOP('',(#53778,#53779,#53780,#53781,#53782,#53783));
#24169=EDGE_LOOP('',(#53784,#53785,#53786,#53787,#53788,#53789));
#24170=EDGE_LOOP('',(#53790,#53791,#53792,#53793));
#24171=EDGE_LOOP('',(#53794,#53795,#53796,#53797,#53798,#53799,#53800,#53801));
#24172=EDGE_LOOP('',(#53802,#53803,#53804,#53805,#53806,#53807,#53808,#53809));
#24173=EDGE_LOOP('',(#53810,#53811,#53812,#53813));
#24174=EDGE_LOOP('',(#53814));
#24175=EDGE_LOOP('',(#53815,#53816,#53817,#53818));
#24176=EDGE_LOOP('',(#53819,#53820,#53821,#53822,#53823,#53824,#53825,#53826,
#53827,#53828,#53829,#53830));
#24177=EDGE_LOOP('',(#53831,#53832,#53833,#53834,#53835,#53836,#53837,#53838,
#53839,#53840,#53841,#53842,#53843));
#24178=EDGE_LOOP('',(#53844,#53845,#53846,#53847));
#24179=EDGE_LOOP('',(#53848));
#24180=EDGE_LOOP('',(#53849));
#24181=EDGE_LOOP('',(#53850));
#24182=EDGE_LOOP('',(#53851,#53852,#53853,#53854,#53855,#53856,#53857,#53858,
#53859));
#24183=EDGE_LOOP('',(#53860,#53861,#53862,#53863,#53864,#53865,#53866,#53867,
#53868));
#24184=EDGE_LOOP('',(#53869,#53870,#53871,#53872));
#24185=EDGE_LOOP('',(#53873,#53874,#53875,#53876));
#24186=EDGE_LOOP('',(#53877,#53878,#53879,#53880,#53881,#53882));
#24187=EDGE_LOOP('',(#53883,#53884,#53885));
#24188=EDGE_LOOP('',(#53886,#53887,#53888,#53889,#53890));
#24189=EDGE_LOOP('',(#53891,#53892,#53893));
#24190=EDGE_LOOP('',(#53894,#53895,#53896,#53897,#53898,#53899,#53900,#53901,
#53902,#53903));
#24191=EDGE_LOOP('',(#53904,#53905,#53906,#53907,#53908,#53909,#53910,#53911,
#53912,#53913,#53914,#53915));
#24192=EDGE_LOOP('',(#53916,#53917,#53918,#53919,#53920,#53921,#53922,#53923,
#53924));
#24193=EDGE_LOOP('',(#53925,#53926,#53927,#53928,#53929,#53930,#53931,#53932,
#53933));
#24194=EDGE_LOOP('',(#53934,#53935,#53936,#53937,#53938,#53939,#53940));
#24195=EDGE_LOOP('',(#53941,#53942,#53943));
#24196=EDGE_LOOP('',(#53944,#53945,#53946,#53947));
#24197=EDGE_LOOP('',(#53948,#53949,#53950));
#24198=EDGE_LOOP('',(#53951,#53952,#53953,#53954));
#24199=EDGE_LOOP('',(#53955,#53956,#53957,#53958));
#24200=EDGE_LOOP('',(#53959,#53960,#53961));
#24201=EDGE_LOOP('',(#53962,#53963,#53964,#53965));
#24202=EDGE_LOOP('',(#53966,#53967,#53968,#53969,#53970,#53971,#53972));
#24203=EDGE_LOOP('',(#53973,#53974,#53975));
#24204=EDGE_LOOP('',(#53976,#53977,#53978,#53979,#53980));
#24205=EDGE_LOOP('',(#53981,#53982,#53983,#53984,#53985,#53986));
#24206=EDGE_LOOP('',(#53987,#53988,#53989,#53990));
#24207=EDGE_LOOP('',(#53991,#53992,#53993));
#24208=EDGE_LOOP('',(#53994,#53995,#53996,#53997,#53998));
#24209=EDGE_LOOP('',(#53999,#54000,#54001));
#24210=EDGE_LOOP('',(#54002,#54003,#54004));
#24211=EDGE_LOOP('',(#54005,#54006,#54007));
#24212=EDGE_LOOP('',(#54008,#54009,#54010,#54011,#54012));
#24213=EDGE_LOOP('',(#54013,#54014,#54015));
#24214=EDGE_LOOP('',(#54016,#54017,#54018));
#24215=EDGE_LOOP('',(#54019,#54020,#54021,#54022,#54023));
#24216=EDGE_LOOP('',(#54024,#54025,#54026));
#24217=EDGE_LOOP('',(#54027,#54028,#54029,#54030,#54031,#54032));
#24218=EDGE_LOOP('',(#54033,#54034,#54035,#54036));
#24219=EDGE_LOOP('',(#54037,#54038,#54039,#54040));
#24220=EDGE_LOOP('',(#54041,#54042,#54043,#54044));
#24221=EDGE_LOOP('',(#54045,#54046,#54047,#54048));
#24222=EDGE_LOOP('',(#54049,#54050,#54051,#54052));
#24223=EDGE_LOOP('',(#54053,#54054,#54055,#54056));
#24224=EDGE_LOOP('',(#54057,#54058,#54059,#54060,#54061));
#24225=EDGE_LOOP('',(#54062,#54063,#54064,#54065));
#24226=EDGE_LOOP('',(#54066,#54067,#54068));
#24227=EDGE_LOOP('',(#54069,#54070,#54071,#54072));
#24228=EDGE_LOOP('',(#54073,#54074,#54075,#54076,#54077));
#24229=EDGE_LOOP('',(#54078,#54079,#54080,#54081));
#24230=EDGE_LOOP('',(#54082,#54083,#54084,#54085));
#24231=EDGE_LOOP('',(#54086,#54087,#54088,#54089,#54090,#54091,#54092,#54093,
#54094,#54095,#54096));
#24232=EDGE_LOOP('',(#54097,#54098,#54099,#54100));
#24233=EDGE_LOOP('',(#54101,#54102,#54103,#54104));
#24234=EDGE_LOOP('',(#54105,#54106,#54107,#54108,#54109));
#24235=EDGE_LOOP('',(#54110,#54111,#54112,#54113,#54114));
#24236=EDGE_LOOP('',(#54115,#54116,#54117,#54118));
#24237=EDGE_LOOP('',(#54119,#54120,#54121,#54122,#54123));
#24238=EDGE_LOOP('',(#54124,#54125,#54126,#54127,#54128));
#24239=EDGE_LOOP('',(#54129,#54130,#54131,#54132));
#24240=EDGE_LOOP('',(#54133,#54134,#54135,#54136,#54137,#54138,#54139,#54140,
#54141));
#24241=EDGE_LOOP('',(#54142));
#24242=EDGE_LOOP('',(#54143));
#24243=EDGE_LOOP('',(#54144));
#24244=EDGE_LOOP('',(#54145));
#24245=EDGE_LOOP('',(#54146,#54147,#54148,#54149));
#24246=EDGE_LOOP('',(#54150,#54151,#54152,#54153,#54154,#54155));
#24247=EDGE_LOOP('',(#54156,#54157,#54158,#54159,#54160));
#24248=EDGE_LOOP('',(#54161,#54162,#54163,#54164,#54165,#54166));
#24249=EDGE_LOOP('',(#54167,#54168,#54169,#54170));
#24250=EDGE_LOOP('',(#54171,#54172,#54173,#54174));
#24251=EDGE_LOOP('',(#54175,#54176,#54177,#54178));
#24252=EDGE_LOOP('',(#54179,#54180,#54181,#54182));
#24253=EDGE_LOOP('',(#54183,#54184,#54185,#54186));
#24254=EDGE_LOOP('',(#54187,#54188,#54189,#54190,#54191,#54192));
#24255=EDGE_LOOP('',(#54193,#54194,#54195,#54196,#54197));
#24256=EDGE_LOOP('',(#54198,#54199,#54200,#54201,#54202));
#24257=EDGE_LOOP('',(#54203,#54204,#54205,#54206,#54207,#54208));
#24258=EDGE_LOOP('',(#54209,#54210,#54211,#54212,#54213,#54214));
#24259=EDGE_LOOP('',(#54215,#54216,#54217,#54218));
#24260=EDGE_LOOP('',(#54219,#54220,#54221,#54222));
#24261=EDGE_LOOP('',(#54223,#54224,#54225,#54226,#54227));
#24262=EDGE_LOOP('',(#54228,#54229,#54230,#54231));
#24263=EDGE_LOOP('',(#54232,#54233,#54234,#54235));
#24264=EDGE_LOOP('',(#54236,#54237,#54238,#54239,#54240,#54241));
#24265=EDGE_LOOP('',(#54242,#54243,#54244,#54245,#54246,#54247));
#24266=EDGE_LOOP('',(#54248,#54249,#54250,#54251));
#24267=EDGE_LOOP('',(#54252));
#24268=EDGE_LOOP('',(#54253));
#24269=EDGE_LOOP('',(#54254));
#24270=EDGE_LOOP('',(#54255));
#24271=EDGE_LOOP('',(#54256));
#24272=EDGE_LOOP('',(#54257,#54258,#54259,#54260,#54261,#54262,#54263));
#24273=EDGE_LOOP('',(#54264,#54265,#54266));
#24274=EDGE_LOOP('',(#54267,#54268,#54269,#54270,#54271,#54272));
#24275=EDGE_LOOP('',(#54273,#54274,#54275,#54276));
#24276=EDGE_LOOP('',(#54277,#54278,#54279,#54280));
#24277=EDGE_LOOP('',(#54281,#54282,#54283,#54284));
#24278=EDGE_LOOP('',(#54285,#54286,#54287,#54288,#54289));
#24279=EDGE_LOOP('',(#54290,#54291,#54292,#54293));
#24280=EDGE_LOOP('',(#54294,#54295,#54296,#54297,#54298,#54299,#54300,#54301,
#54302));
#24281=EDGE_LOOP('',(#54303,#54304,#54305,#54306,#54307,#54308));
#24282=EDGE_LOOP('',(#54309,#54310,#54311,#54312));
#24283=EDGE_LOOP('',(#54313,#54314,#54315,#54316,#54317,#54318,#54319));
#24284=EDGE_LOOP('',(#54320,#54321,#54322,#54323));
#24285=EDGE_LOOP('',(#54324,#54325,#54326,#54327,#54328,#54329));
#24286=EDGE_LOOP('',(#54330,#54331,#54332));
#24287=EDGE_LOOP('',(#54333,#54334,#54335));
#24288=EDGE_LOOP('',(#54336,#54337,#54338,#54339,#54340,#54341,#54342));
#24289=EDGE_LOOP('',(#54343,#54344,#54345,#54346,#54347,#54348,#54349,#54350,
#54351,#54352,#54353));
#24290=EDGE_LOOP('',(#54354,#54355,#54356,#54357));
#24291=EDGE_LOOP('',(#54358,#54359,#54360,#54361));
#24292=EDGE_LOOP('',(#54362,#54363,#54364,#54365,#54366));
#24293=EDGE_LOOP('',(#54367,#54368,#54369,#54370));
#24294=EDGE_LOOP('',(#54371,#54372,#54373,#54374));
#24295=EDGE_LOOP('',(#54375,#54376,#54377,#54378));
#24296=EDGE_LOOP('',(#54379,#54380,#54381,#54382));
#24297=EDGE_LOOP('',(#54383,#54384,#54385,#54386));
#24298=EDGE_LOOP('',(#54387,#54388,#54389,#54390));
#24299=EDGE_LOOP('',(#54391,#54392,#54393,#54394));
#24300=EDGE_LOOP('',(#54395,#54396,#54397,#54398));
#24301=EDGE_LOOP('',(#54399,#54400,#54401));
#24302=EDGE_LOOP('',(#54402,#54403,#54404,#54405,#54406));
#24303=EDGE_LOOP('',(#54407,#54408,#54409,#54410));
#24304=EDGE_LOOP('',(#54411,#54412,#54413,#54414));
#24305=EDGE_LOOP('',(#54415,#54416,#54417,#54418));
#24306=EDGE_LOOP('',(#54419,#54420,#54421,#54422));
#24307=EDGE_LOOP('',(#54423,#54424,#54425,#54426));
#24308=EDGE_LOOP('',(#54427,#54428,#54429,#54430));
#24309=EDGE_LOOP('',(#54431,#54432,#54433,#54434));
#24310=EDGE_LOOP('',(#54435,#54436,#54437,#54438,#54439));
#24311=EDGE_LOOP('',(#54440,#54441,#54442,#54443,#54444,#54445));
#24312=EDGE_LOOP('',(#54446,#54447,#54448));
#24313=EDGE_LOOP('',(#54449,#54450,#54451,#54452));
#24314=EDGE_LOOP('',(#54453,#54454,#54455,#54456));
#24315=EDGE_LOOP('',(#54457,#54458,#54459));
#24316=EDGE_LOOP('',(#54460,#54461,#54462,#54463,#54464,#54465));
#24317=EDGE_LOOP('',(#54466,#54467,#54468,#54469,#54470));
#24318=EDGE_LOOP('',(#54471,#54472,#54473,#54474));
#24319=EDGE_LOOP('',(#54475,#54476,#54477,#54478));
#24320=EDGE_LOOP('',(#54479,#54480,#54481,#54482,#54483));
#24321=EDGE_LOOP('',(#54484,#54485,#54486,#54487));
#24322=EDGE_LOOP('',(#54488,#54489,#54490,#54491));
#24323=EDGE_LOOP('',(#54492,#54493,#54494,#54495));
#24324=EDGE_LOOP('',(#54496,#54497,#54498,#54499,#54500));
#24325=EDGE_LOOP('',(#54501,#54502,#54503,#54504));
#24326=EDGE_LOOP('',(#54505,#54506,#54507,#54508));
#24327=EDGE_LOOP('',(#54509,#54510,#54511,#54512,#54513));
#24328=EDGE_LOOP('',(#54514,#54515,#54516,#54517,#54518));
#24329=EDGE_LOOP('',(#54519,#54520,#54521,#54522));
#24330=EDGE_LOOP('',(#54523,#54524,#54525,#54526));
#24331=EDGE_LOOP('',(#54527,#54528,#54529,#54530));
#24332=EDGE_LOOP('',(#54531,#54532,#54533,#54534));
#24333=EDGE_LOOP('',(#54535,#54536,#54537,#54538,#54539,#54540,#54541,#54542,
#54543,#54544,#54545));
#24334=EDGE_LOOP('',(#54546,#54547,#54548,#54549));
#24335=EDGE_LOOP('',(#54550,#54551,#54552,#54553,#54554,#54555,#54556));
#24336=EDGE_LOOP('',(#54557,#54558,#54559,#54560,#54561,#54562));
#24337=EDGE_LOOP('',(#54563,#54564,#54565,#54566));
#24338=EDGE_LOOP('',(#54567));
#24339=EDGE_LOOP('',(#54568));
#24340=EDGE_LOOP('',(#54569,#54570));
#24341=EDGE_LOOP('',(#54571));
#24342=EDGE_LOOP('',(#54572,#54573,#54574,#54575,#54576,#54577,#54578,#54579));
#24343=EDGE_LOOP('',(#54580,#54581,#54582,#54583,#54584));
#24344=EDGE_LOOP('',(#54585,#54586,#54587,#54588,#54589,#54590,#54591));
#24345=EDGE_LOOP('',(#54592,#54593,#54594,#54595,#54596,#54597,#54598));
#24346=EDGE_LOOP('',(#54599,#54600,#54601,#54602));
#24347=EDGE_LOOP('',(#54603,#54604,#54605,#54606));
#24348=EDGE_LOOP('',(#54607,#54608,#54609,#54610));
#24349=EDGE_LOOP('',(#54611,#54612,#54613,#54614));
#24350=EDGE_LOOP('',(#54615,#54616,#54617,#54618,#54619));
#24351=EDGE_LOOP('',(#54620,#54621,#54622,#54623,#54624,#54625,#54626,#54627,
#54628,#54629,#54630,#54631,#54632,#54633));
#24352=EDGE_LOOP('',(#54634,#54635,#54636,#54637,#54638));
#24353=EDGE_LOOP('',(#54639,#54640,#54641,#54642));
#24354=EDGE_LOOP('',(#54643,#54644,#54645,#54646));
#24355=EDGE_LOOP('',(#54647,#54648,#54649,#54650));
#24356=EDGE_LOOP('',(#54651,#54652,#54653,#54654));
#24357=EDGE_LOOP('',(#54655,#54656,#54657,#54658));
#24358=EDGE_LOOP('',(#54659,#54660,#54661,#54662));
#24359=EDGE_LOOP('',(#54663,#54664,#54665));
#24360=EDGE_LOOP('',(#54666,#54667,#54668));
#24361=EDGE_LOOP('',(#54669,#54670,#54671,#54672,#54673,#54674,#54675,#54676,
#54677,#54678,#54679,#54680));
#24362=EDGE_LOOP('',(#54681,#54682,#54683,#54684,#54685,#54686,#54687));
#24363=EDGE_LOOP('',(#54688,#54689,#54690,#54691));
#24364=EDGE_LOOP('',(#54692,#54693,#54694,#54695,#54696));
#24365=EDGE_LOOP('',(#54697,#54698,#54699,#54700));
#24366=EDGE_LOOP('',(#54701,#54702,#54703,#54704));
#24367=EDGE_LOOP('',(#54705,#54706,#54707,#54708));
#24368=EDGE_LOOP('',(#54709,#54710,#54711,#54712,#54713,#54714,#54715,#54716,
#54717));
#24369=EDGE_LOOP('',(#54718,#54719,#54720));
#24370=EDGE_LOOP('',(#54721,#54722,#54723,#54724,#54725));
#24371=EDGE_LOOP('',(#54726,#54727,#54728,#54729));
#24372=EDGE_LOOP('',(#54730,#54731,#54732,#54733));
#24373=EDGE_LOOP('',(#54734,#54735,#54736,#54737));
#24374=EDGE_LOOP('',(#54738,#54739,#54740));
#24375=EDGE_LOOP('',(#54741,#54742,#54743,#54744));
#24376=EDGE_LOOP('',(#54745,#54746,#54747,#54748));
#24377=EDGE_LOOP('',(#54749,#54750,#54751,#54752,#54753));
#24378=EDGE_LOOP('',(#54754,#54755,#54756,#54757));
#24379=EDGE_LOOP('',(#54758,#54759,#54760,#54761));
#24380=EDGE_LOOP('',(#54762,#54763,#54764,#54765));
#24381=EDGE_LOOP('',(#54766,#54767,#54768,#54769,#54770,#54771,#54772));
#24382=EDGE_LOOP('',(#54773,#54774,#54775,#54776,#54777,#54778,#54779));
#24383=EDGE_LOOP('',(#54780,#54781,#54782,#54783));
#24384=EDGE_LOOP('',(#54784,#54785,#54786));
#24385=EDGE_LOOP('',(#54787,#54788,#54789));
#24386=EDGE_LOOP('',(#54790,#54791,#54792,#54793));
#24387=EDGE_LOOP('',(#54794,#54795,#54796,#54797));
#24388=EDGE_LOOP('',(#54798,#54799,#54800,#54801));
#24389=EDGE_LOOP('',(#54802,#54803,#54804));
#24390=EDGE_LOOP('',(#54805,#54806,#54807,#54808));
#24391=EDGE_LOOP('',(#54809,#54810,#54811,#54812));
#24392=EDGE_LOOP('',(#54813,#54814,#54815,#54816));
#24393=EDGE_LOOP('',(#54817,#54818,#54819,#54820,#54821,#54822));
#24394=EDGE_LOOP('',(#54823));
#24395=EDGE_LOOP('',(#54824,#54825,#54826,#54827));
#24396=EDGE_LOOP('',(#54828,#54829,#54830,#54831));
#24397=EDGE_LOOP('',(#54832,#54833,#54834,#54835));
#24398=EDGE_LOOP('',(#54836,#54837,#54838,#54839));
#24399=EDGE_LOOP('',(#54840,#54841,#54842,#54843));
#24400=EDGE_LOOP('',(#54844,#54845,#54846,#54847,#54848));
#24401=EDGE_LOOP('',(#54849,#54850,#54851,#54852));
#24402=EDGE_LOOP('',(#54853,#54854,#54855,#54856));
#24403=EDGE_LOOP('',(#54857,#54858,#54859,#54860));
#24404=EDGE_LOOP('',(#54861,#54862,#54863,#54864));
#24405=EDGE_LOOP('',(#54865,#54866,#54867,#54868));
#24406=EDGE_LOOP('',(#54869,#54870,#54871,#54872,#54873));
#24407=EDGE_LOOP('',(#54874,#54875,#54876,#54877,#54878,#54879,#54880));
#24408=EDGE_LOOP('',(#54881,#54882,#54883,#54884));
#24409=EDGE_LOOP('',(#54885,#54886,#54887,#54888,#54889,#54890,#54891,#54892,
#54893,#54894));
#24410=EDGE_LOOP('',(#54895,#54896,#54897,#54898));
#24411=EDGE_LOOP('',(#54899,#54900,#54901,#54902,#54903,#54904,#54905));
#24412=EDGE_LOOP('',(#54906,#54907,#54908,#54909));
#24413=EDGE_LOOP('',(#54910,#54911,#54912,#54913,#54914,#54915,#54916,#54917,
#54918,#54919,#54920,#54921));
#24414=EDGE_LOOP('',(#54922,#54923,#54924,#54925));
#24415=EDGE_LOOP('',(#54926,#54927,#54928,#54929));
#24416=EDGE_LOOP('',(#54930,#54931,#54932,#54933));
#24417=EDGE_LOOP('',(#54934,#54935,#54936,#54937));
#24418=EDGE_LOOP('',(#54938,#54939,#54940,#54941,#54942));
#24419=EDGE_LOOP('',(#54943,#54944,#54945,#54946));
#24420=EDGE_LOOP('',(#54947,#54948,#54949,#54950));
#24421=EDGE_LOOP('',(#54951,#54952,#54953,#54954));
#24422=EDGE_LOOP('',(#54955,#54956,#54957,#54958));
#24423=EDGE_LOOP('',(#54959,#54960,#54961,#54962,#54963));
#24424=EDGE_LOOP('',(#54964,#54965,#54966,#54967,#54968,#54969));
#24425=EDGE_LOOP('',(#54970));
#24426=EDGE_LOOP('',(#54971,#54972,#54973,#54974));
#24427=EDGE_LOOP('',(#54975,#54976,#54977,#54978));
#24428=EDGE_LOOP('',(#54979,#54980,#54981,#54982));
#24429=EDGE_LOOP('',(#54983,#54984,#54985,#54986));
#24430=EDGE_LOOP('',(#54987,#54988,#54989,#54990));
#24431=EDGE_LOOP('',(#54991,#54992,#54993,#54994));
#24432=EDGE_LOOP('',(#54995,#54996,#54997,#54998,#54999,#55000));
#24433=EDGE_LOOP('',(#55001,#55002,#55003,#55004));
#24434=EDGE_LOOP('',(#55005,#55006,#55007,#55008));
#24435=EDGE_LOOP('',(#55009,#55010,#55011,#55012));
#24436=EDGE_LOOP('',(#55013,#55014,#55015,#55016,#55017));
#24437=EDGE_LOOP('',(#55018,#55019,#55020,#55021));
#24438=EDGE_LOOP('',(#55022,#55023,#55024,#55025));
#24439=EDGE_LOOP('',(#55026,#55027,#55028));
#24440=EDGE_LOOP('',(#55029,#55030,#55031,#55032,#55033,#55034,#55035,#55036,
#55037));
#24441=EDGE_LOOP('',(#55038,#55039,#55040,#55041,#55042));
#24442=EDGE_LOOP('',(#55043,#55044,#55045,#55046));
#24443=EDGE_LOOP('',(#55047,#55048,#55049,#55050));
#24444=EDGE_LOOP('',(#55051,#55052,#55053,#55054,#55055));
#24445=EDGE_LOOP('',(#55056,#55057,#55058,#55059));
#24446=EDGE_LOOP('',(#55060,#55061,#55062,#55063));
#24447=EDGE_LOOP('',(#55064,#55065,#55066,#55067,#55068));
#24448=EDGE_LOOP('',(#55069,#55070,#55071));
#24449=EDGE_LOOP('',(#55072,#55073,#55074,#55075));
#24450=EDGE_LOOP('',(#55076,#55077,#55078,#55079));
#24451=EDGE_LOOP('',(#55080,#55081,#55082,#55083));
#24452=EDGE_LOOP('',(#55084,#55085,#55086,#55087,#55088,#55089));
#24453=EDGE_LOOP('',(#55090,#55091,#55092,#55093));
#24454=EDGE_LOOP('',(#55094));
#24455=EDGE_LOOP('',(#55095));
#24456=EDGE_LOOP('',(#55096,#55097,#55098,#55099));
#24457=EDGE_LOOP('',(#55100,#55101,#55102,#55103));
#24458=EDGE_LOOP('',(#55104,#55105,#55106,#55107));
#24459=EDGE_LOOP('',(#55108,#55109,#55110,#55111,#55112,#55113,#55114,#55115));
#24460=EDGE_LOOP('',(#55116,#55117,#55118,#55119));
#24461=EDGE_LOOP('',(#55120,#55121,#55122,#55123));
#24462=EDGE_LOOP('',(#55124,#55125,#55126,#55127));
#24463=EDGE_LOOP('',(#55128,#55129,#55130,#55131));
#24464=EDGE_LOOP('',(#55132,#55133,#55134,#55135));
#24465=EDGE_LOOP('',(#55136,#55137,#55138,#55139));
#24466=EDGE_LOOP('',(#55140,#55141,#55142,#55143));
#24467=EDGE_LOOP('',(#55144,#55145,#55146,#55147));
#24468=EDGE_LOOP('',(#55148,#55149,#55150,#55151));
#24469=EDGE_LOOP('',(#55152,#55153,#55154,#55155));
#24470=EDGE_LOOP('',(#55156,#55157,#55158,#55159));
#24471=EDGE_LOOP('',(#55160,#55161,#55162,#55163));
#24472=EDGE_LOOP('',(#55164,#55165,#55166,#55167));
#24473=EDGE_LOOP('',(#55168,#55169,#55170,#55171,#55172,#55173,#55174));
#24474=EDGE_LOOP('',(#55175));
#24475=EDGE_LOOP('',(#55176,#55177,#55178,#55179));
#24476=EDGE_LOOP('',(#55180,#55181,#55182,#55183));
#24477=EDGE_LOOP('',(#55184));
#24478=EDGE_LOOP('',(#55185));
#24479=EDGE_LOOP('',(#55186));
#24480=EDGE_LOOP('',(#55187,#55188));
#24481=EDGE_LOOP('',(#55189,#55190,#55191,#55192));
#24482=EDGE_LOOP('',(#55193,#55194,#55195,#55196,#55197,#55198,#55199));
#24483=EDGE_LOOP('',(#55200,#55201,#55202,#55203,#55204,#55205,#55206,#55207,
#55208,#55209,#55210,#55211));
#24484=EDGE_LOOP('',(#55212,#55213,#55214,#55215));
#24485=EDGE_LOOP('',(#55216,#55217,#55218));
#24486=EDGE_LOOP('',(#55219,#55220,#55221,#55222));
#24487=EDGE_LOOP('',(#55223,#55224,#55225));
#24488=EDGE_LOOP('',(#55226,#55227,#55228,#55229));
#24489=EDGE_LOOP('',(#55230,#55231,#55232,#55233,#55234,#55235));
#24490=EDGE_LOOP('',(#55236,#55237,#55238,#55239));
#24491=EDGE_LOOP('',(#55240,#55241,#55242,#55243));
#24492=EDGE_LOOP('',(#55244,#55245,#55246,#55247));
#24493=EDGE_LOOP('',(#55248,#55249,#55250,#55251,#55252));
#24494=EDGE_LOOP('',(#55253,#55254,#55255,#55256));
#24495=EDGE_LOOP('',(#55257,#55258,#55259,#55260));
#24496=EDGE_LOOP('',(#55261,#55262,#55263));
#24497=EDGE_LOOP('',(#55264,#55265,#55266,#55267));
#24498=EDGE_LOOP('',(#55268,#55269,#55270,#55271));
#24499=EDGE_LOOP('',(#55272,#55273,#55274,#55275));
#24500=EDGE_LOOP('',(#55276,#55277,#55278,#55279,#55280));
#24501=EDGE_LOOP('',(#55281,#55282,#55283,#55284,#55285,#55286,#55287,#55288,
#55289));
#24502=EDGE_LOOP('',(#55290,#55291,#55292,#55293,#55294,#55295));
#24503=EDGE_LOOP('',(#55296,#55297,#55298,#55299));
#24504=EDGE_LOOP('',(#55300,#55301,#55302,#55303));
#24505=EDGE_LOOP('',(#55304,#55305,#55306,#55307));
#24506=EDGE_LOOP('',(#55308,#55309,#55310));
#24507=EDGE_LOOP('',(#55311,#55312,#55313,#55314));
#24508=EDGE_LOOP('',(#55315,#55316,#55317));
#24509=EDGE_LOOP('',(#55318,#55319,#55320,#55321));
#24510=EDGE_LOOP('',(#55322,#55323,#55324,#55325));
#24511=EDGE_LOOP('',(#55326,#55327));
#24512=EDGE_LOOP('',(#55328,#55329,#55330));
#24513=EDGE_LOOP('',(#55331,#55332,#55333,#55334,#55335));
#24514=EDGE_LOOP('',(#55336,#55337,#55338,#55339,#55340,#55341,#55342));
#24515=EDGE_LOOP('',(#55343,#55344,#55345,#55346));
#24516=EDGE_LOOP('',(#55347,#55348,#55349,#55350));
#24517=EDGE_LOOP('',(#55351,#55352,#55353));
#24518=EDGE_LOOP('',(#55354,#55355,#55356,#55357,#55358,#55359,#55360,#55361,
#55362));
#24519=EDGE_LOOP('',(#55363,#55364,#55365,#55366));
#24520=EDGE_LOOP('',(#55367,#55368,#55369,#55370));
#24521=EDGE_LOOP('',(#55371,#55372,#55373,#55374));
#24522=EDGE_LOOP('',(#55375,#55376,#55377,#55378));
#24523=EDGE_LOOP('',(#55379,#55380,#55381));
#24524=EDGE_LOOP('',(#55382,#55383,#55384,#55385));
#24525=EDGE_LOOP('',(#55386,#55387,#55388,#55389));
#24526=EDGE_LOOP('',(#55390,#55391,#55392,#55393));
#24527=EDGE_LOOP('',(#55394,#55395,#55396,#55397));
#24528=EDGE_LOOP('',(#55398,#55399,#55400,#55401));
#24529=EDGE_LOOP('',(#55402,#55403,#55404,#55405));
#24530=EDGE_LOOP('',(#55406,#55407,#55408,#55409));
#24531=EDGE_LOOP('',(#55410,#55411,#55412,#55413));
#24532=EDGE_LOOP('',(#55414,#55415,#55416,#55417));
#24533=EDGE_LOOP('',(#55418,#55419,#55420,#55421));
#24534=EDGE_LOOP('',(#55422,#55423,#55424,#55425,#55426,#55427,#55428));
#24535=EDGE_LOOP('',(#55429,#55430,#55431,#55432,#55433,#55434,#55435,#55436));
#24536=EDGE_LOOP('',(#55437,#55438,#55439,#55440,#55441,#55442));
#24537=EDGE_LOOP('',(#55443,#55444,#55445,#55446,#55447));
#24538=EDGE_LOOP('',(#55448,#55449,#55450,#55451));
#24539=EDGE_LOOP('',(#55452,#55453,#55454,#55455));
#24540=EDGE_LOOP('',(#55456,#55457,#55458));
#24541=EDGE_LOOP('',(#55459,#55460,#55461));
#24542=EDGE_LOOP('',(#55462,#55463,#55464,#55465));
#24543=EDGE_LOOP('',(#55466,#55467,#55468,#55469));
#24544=EDGE_LOOP('',(#55470,#55471,#55472,#55473));
#24545=EDGE_LOOP('',(#55474,#55475,#55476,#55477));
#24546=EDGE_LOOP('',(#55478,#55479,#55480,#55481));
#24547=EDGE_LOOP('',(#55482,#55483,#55484,#55485));
#24548=EDGE_LOOP('',(#55486,#55487,#55488,#55489));
#24549=EDGE_LOOP('',(#55490,#55491,#55492));
#24550=EDGE_LOOP('',(#55493,#55494,#55495,#55496));
#24551=EDGE_LOOP('',(#55497,#55498,#55499,#55500));
#24552=EDGE_LOOP('',(#55501,#55502,#55503,#55504,#55505,#55506,#55507,#55508,
#55509,#55510,#55511,#55512,#55513,#55514,#55515,#55516));
#24553=EDGE_LOOP('',(#55517,#55518,#55519,#55520,#55521,#55522));
#29387=B_SPLINE_CURVE_WITH_KNOTS('',3,(#106605,#106606,#106607,#106608,
#106609,#106610),.UNSPECIFIED.,.F.,.F.,(4,2,4),(-0.241430299538162,-0.206580137455089,
-0.156109273606686),.UNSPECIFIED.);
#29388=B_SPLINE_CURVE_WITH_KNOTS('',3,(#106654,#106655,#106656,#106657,
#106658,#106659,#106660,#106661,#106662,#106663,#106664,#106665,#106666,
#106667),.UNSPECIFIED.,.F.,.F.,(4,2,2,2,2,2,4),(-0.241853105666202,-0.175836100044282,
-0.122112436673168,-0.0803073887927507,-0.0455467331302326,-0.0227627040768013,
-1.73601080630016E-6),.UNSPECIFIED.);
#29389=B_SPLINE_CURVE_WITH_KNOTS('',3,(#106668,#106669,#106670,#106671),
 .UNSPECIFIED.,.F.,.F.,(4,4),(0.,0.999989990831842),.UNSPECIFIED.);
#29390=B_SPLINE_CURVE_WITH_KNOTS('',3,(#106753,#106754,#106755,#106756,
#106757,#106758,#106759,#106760,#106761,#106762),.UNSPECIFIED.,.F.,.F.,
(4,3,3,4),(0.,0.354579189327693,0.679902554719739,1.),.UNSPECIFIED.);
#29391=B_SPLINE_CURVE_WITH_KNOTS('',3,(#106763,#106764,#106765,#106766,
#106767,#106768),.UNSPECIFIED.,.F.,.F.,(4,2,4),(-0.278077459546498,-0.155434077993828,
-1.73601828061288E-6),.UNSPECIFIED.);
#29392=B_SPLINE_CURVE_WITH_KNOTS('',3,(#106849,#106850,#106851,#106852,
#106853,#106854,#106855,#106856,#106857,#106858,#106859,#106860,#106861,
#106862,#106863,#106864),.UNSPECIFIED.,.F.,.F.,(4,2,2,2,2,2,2,4),(-0.280256489498076,
-0.161862440487671,-0.12787619266535,-0.10766826527807,-0.092664611109678,
-0.0777869012640525,-0.056960032780691,-9.99999003770125E-7),
 .UNSPECIFIED.);
#29393=B_SPLINE_CURVE_WITH_KNOTS('',3,(#106866,#106867,#106868,#106869,
#106870,#106871,#106872,#106873,#106874,#106875),.UNSPECIFIED.,.F.,.F.,
(4,2,2,2,4),(-2.67982627711791E-10,0.0296331580141952,0.0592663162963728,
0.118532632860728,0.223499171284228),.UNSPECIFIED.);
#29394=B_SPLINE_CURVE_WITH_KNOTS('',3,(#106885,#106886,#106887,#106888,
#106889,#106890),.UNSPECIFIED.,.F.,.F.,(4,2,4),(-0.257051044346983,-0.206580142016457,
-0.171729983682942),.UNSPECIFIED.);
#29395=B_SPLINE_CURVE_WITH_KNOTS('',3,(#106928,#106929,#106930,#106931,
#106932,#106933,#106934,#106935,#106936,#106937,#106938,#106939,#106940,
#106941),.UNSPECIFIED.,.F.,.F.,(4,2,2,2,2,2,4),(-0.2438079662112,-0.220869823866369,
-0.197908662602918,-0.162873889664189,-0.1207435672921,-0.0666091518365065,
-1.00053347902397E-6),.UNSPECIFIED.);
#29396=B_SPLINE_CURVE_WITH_KNOTS('',3,(#106942,#106943,#106944,#106945),
 .UNSPECIFIED.,.F.,.F.,(4,4),(0.,0.999999972395555),.UNSPECIFIED.);
#29397=B_SPLINE_CURVE_WITH_KNOTS('',3,(#107029,#107030,#107031,#107032,
#107033,#107034,#107035,#107036,#107037,#107038,#107039,#107040,#107041,
#107042,#107043,#107044),.UNSPECIFIED.,.F.,.F.,(4,2,2,2,2,2,2,4),(-0.442279703755202,
-0.352763675612789,-0.319586925582681,-0.29601592754955,-0.27234102291881,
-0.240616391884951,-0.187314080741787,-9.99999260398177E-7),
 .UNSPECIFIED.);
#29398=B_SPLINE_CURVE_WITH_KNOTS('',3,(#107045,#107046,#107047,#107048,
#107049,#107050,#107051,#107052,#107053,#107054),.UNSPECIFIED.,.F.,.F.,
(4,3,3,4),(2.36937065112853E-5,0.199673744617112,0.681815427418137,1.),
 .UNSPECIFIED.);
#29399=B_SPLINE_CURVE_WITH_KNOTS('',3,(#107135,#107136,#107137,#107138,
#107139,#107140),.UNSPECIFIED.,.F.,.F.,(4,2,4),(-0.278517062048807,-0.122825079395318,
-1.00000141813119E-6),.UNSPECIFIED.);
#29400=B_SPLINE_CURVE_WITH_KNOTS('',3,(#107142,#107143,#107144,#107145,
#107146,#107147,#107148,#107149,#107150,#107151),.UNSPECIFIED.,.F.,.F.,
(4,2,2,2,4),(-0.218420289446346,-0.143529737322937,-0.051830543878608,-0.0259152720267801,
-1.7495224713393E-10),.UNSPECIFIED.);
#29401=B_SPLINE_CURVE_WITH_KNOTS('',3,(#107156,#107157,#107158,#107159,
#107160,#107161,#107162,#107163,#107164,#107165,#107166,#107167),
 .UNSPECIFIED.,.F.,.F.,(4,2,2,2,2,4),(-0.761165579403507,-0.582021759725205,
-0.420760911541275,-0.213198071172165,-0.116802189854271,-7.01180062234323E-6),
 .UNSPECIFIED.);
#29402=B_SPLINE_CURVE_WITH_KNOTS('',3,(#107169,#107170,#107171,#107172,
#107173,#107174,#107175,#107176,#107177,#107178,#107179,#107180,#107181,
#107182,#107183,#107184,#107185,#107186,#107187,#107188,#107189,#107190),
 .UNSPECIFIED.,.F.,.F.,(4,2,2,2,2,2,2,2,2,2,4),(-1.34392737370477,-1.014404550101,
-0.888242703317446,-0.838521487626843,-0.812981145439651,-0.795161744961047,
-0.777218608043124,-0.752854386147025,-0.707252167674362,-0.454372104568619,
-9.99999739524789E-7),.UNSPECIFIED.);
#29403=B_SPLINE_CURVE_WITH_KNOTS('',3,(#107194,#107195,#107196,#107197,
#107198,#107199,#107200,#107201,#107202,#107203,#107204,#107205),
 .UNSPECIFIED.,.F.,.F.,(4,2,2,2,2,4),(0.954693196677972,1.07014467842961,
1.18559616018125,1.24486247667459,1.27449563492126,1.30411858773122),
 .UNSPECIFIED.);
#29404=B_SPLINE_CURVE_WITH_KNOTS('',3,(#107209,#107210,#107211,#107212,
#107213,#107214,#107215,#107216,#107217,#107218,#107219,#107220),
 .UNSPECIFIED.,.F.,.F.,(4,2,2,2,2,4),(-0.109324587965852,-0.0960313413287254,
-0.0826995239600266,-0.0543197165532493,-0.0285691916501081,-1.00000465952576E-6),
 .UNSPECIFIED.);
#29405=B_SPLINE_CURVE_WITH_KNOTS('',3,(#107221,#107222,#107223,#107224,
#107225,#107226),.UNSPECIFIED.,.F.,.F.,(4,2,4),(-0.159987069735286,-0.0797279100080487,
-9.99997231576621E-7),.UNSPECIFIED.);
#29406=B_SPLINE_CURVE_WITH_KNOTS('',3,(#107301,#107302,#107303,#107304,
#107305,#107306,#107307,#107308,#107309,#107310,#107311,#107312,#107313,
#107314,#107315,#107316,#107317,#107318,#107319,#107320,#107321,#107322,
#107323,#107324,#107325,#107326,#107327,#107328,#107329,#107330,#107331),
 .UNSPECIFIED.,.F.,.F.,(4,3,3,3,3,3,3,3,3,3,4),(0.,0.108970225117902,0.218406669395091,
0.328218209138362,0.439039967350302,0.5,0.612445244717792,0.727056478754142,
0.843061292777059,0.961495204479547,1.),.UNSPECIFIED.);
#29407=B_SPLINE_CURVE_WITH_KNOTS('',3,(#107333,#107334,#107335,#107336,
#107337,#107338,#107339,#107340,#107341,#107342,#107343,#107344,#107345,
#107346,#107347,#107348,#107349,#107350,#107351,#107352,#107353,#107354,
#107355,#107356,#107357,#107358,#107359,#107360,#107361,#107362,#107363,
#107364,#107365,#107366,#107367,#107368,#107369,#107370,#107371,#107372,
#107373,#107374,#107375,#107376,#107377,#107378,#107379,#107380,#107381,
#107382,#107383,#107384,#107385,#107386,#107387,#107388,#107389,#107390,
#107391,#107392,#107393,#107394,#107395,#107396,#107397,#107398,#107399,
#107400,#107401,#107402,#107403,#107404,#107405,#107406,#107407,#107408,
#107409,#107410,#107411,#107412,#107413,#107414,#107415,#107416,#107417,
#107418,#107419,#107420,#107421,#107422,#107423,#107424,#107425,#107426,
#107427,#107428,#107429,#107430,#107431,#107432,#107433,#107434,#107435,
#107436,#107437,#107438,#107439,#107440,#107441),.UNSPECIFIED.,.F.,.F.,
(4,3,3,3,3,3,3,3,3,3,3,3,3,3,3,3,3,3,3,3,3,3,3,3,3,3,3,3,3,3,3,3,3,3,3,
3,4),(4.63591186593161E-13,0.0352304133180864,0.0496679699621724,0.07142857142857,
0.116839227155713,0.124882006224014,0.1428571428571,0.179126833876683,0.19987991330948,
0.2142857142857,0.254438827359413,0.275004526555019,0.2857142857143,0.327232537354997,
0.350098755170649,0.3571428571429,0.402277134059596,0.42521990674884,0.4285714285714,
0.479462989405757,0.5,0.500342945580645,0.551400032933508,0.5714285714286,
0.57545998934806,0.630187215511676,0.6428571428571,0.650577761732493,0.7142857142857,
0.725693303545247,0.7857142857143,0.800806742377481,0.8571428571429,0.875935814320093,
0.9285714285714,0.950971031508945,1.),.UNSPECIFIED.);
#29408=B_SPLINE_CURVE_WITH_KNOTS('',3,(#107443,#107444,#107445,#107446,
#107447,#107448,#107449,#107450,#107451,#107452,#107453,#107454,#107455,
#107456,#107457,#107458,#107459,#107460,#107461,#107462,#107463,#107464,
#107465,#107466,#107467,#107468,#107469,#107470,#107471,#107472),
 .UNSPECIFIED.,.F.,.F.,(4,2,2,2,1,1,2,2,2,2,2,1,1,2,2,2,4),(2.30700482817146E-8,
0.124999999999894,0.187499999999842,0.218749999999815,0.2343749999998,0.242187499999795,
0.246093749999791,0.249999999999787,0.374999999999697,0.437499999999653,
0.468749999999625,0.484374999999608,0.492187499999599,0.496093749999589,
0.499999999999578,0.749999999999789,1.),.UNSPECIFIED.);
#29409=B_SPLINE_CURVE_WITH_KNOTS('',3,(#107473,#107474,#107475,#107476,
#107477,#107478,#107479,#107480,#107481,#107482,#107483,#107484,#107485,
#107486,#107487,#107488,#107489,#107490,#107491,#107492,#107493,#107494,
#107495,#107496,#107497,#107498,#107499,#107500,#107501,#107502,#107503,
#107504,#107505,#107506,#107507,#107508,#107509,#107510,#107511,#107512,
#107513,#107514,#107515,#107516,#107517,#107518,#107519,#107520,#107521,
#107522,#107523,#107524,#107525,#107526,#107527,#107528,#107529,#107530,
#107531,#107532,#107533,#107534,#107535,#107536,#107537,#107538,#107539,
#107540,#107541,#107542,#107543,#107544,#107545,#107546,#107547,#107548,
#107549,#107550,#107551,#107552,#107553,#107554,#107555,#107556,#107557,
#107558,#107559,#107560,#107561,#107562,#107563,#107564,#107565,#107566,
#107567,#107568,#107569,#107570,#107571,#107572,#107573,#107574,#107575),
 .UNSPECIFIED.,.F.,.F.,(4,3,3,3,3,3,3,3,3,3,3,3,3,3,3,3,3,3,3,3,3,3,3,3,
3,3,3,3,3,3,3,3,3,3,4),(1.68547190877228E-9,0.04838995602028,0.0978468067776024,
0.118523443707981,0.169551292093508,0.221702103432071,0.249999999999981,
0.280746417338719,0.338633928132514,0.374999999999971,0.434952886602702,
0.437499999999966,0.468749999999964,0.484374999999963,0.492187499999962,
0.496093749999961,0.498046874999961,0.499999999999961,0.56407974531281,
0.624999999999964,0.635959106366061,0.687499999999965,0.718749999999966,
0.734374999999967,0.742187499999967,0.746093749999967,0.748046874999967,
0.749999999999967,0.79840618544373,0.845021640793756,0.88913814197588,0.900369257313181,
0.94302038072256,0.983460917668321,1.),.UNSPECIFIED.);
#29410=B_SPLINE_CURVE_WITH_KNOTS('',3,(#107578,#107579,#107580,#107581,
#107582,#107583,#107584,#107585,#107586,#107587,#107588,#107589,#107590,
#107591,#107592,#107593,#107594,#107595,#107596,#107597,#107598,#107599,
#107600,#107601,#107602,#107603,#107604,#107605,#107606,#107607,#107608,
#107609,#107610,#107611,#107612,#107613,#107614,#107615,#107616,#107617,
#107618,#107619,#107620,#107621,#107622,#107623,#107624,#107625,#107626,
#107627,#107628,#107629,#107630,#107631,#107632,#107633,#107634,#107635,
#107636,#107637,#107638,#107639,#107640,#107641,#107642,#107643,#107644,
#107645,#107646,#107647,#107648,#107649,#107650,#107651,#107652,#107653,
#107654,#107655,#107656,#107657,#107658,#107659,#107660,#107661,#107662,
#107663,#107664,#107665,#107666,#107667,#107668,#107669,#107670,#107671,
#107672,#107673,#107674,#107675,#107676,#107677,#107678,#107679,#107680,
#107681,#107682,#107683),.UNSPECIFIED.,.F.,.F.,(4,3,3,3,3,3,3,3,3,3,3,3,
3,3,3,3,3,3,3,3,3,3,3,3,3,3,3,3,3,3,3,3,3,3,3,4),(0.,0.0764808248342431,
0.152821059018209,0.228907286392826,0.25,0.322571962172829,0.39359505610544,
0.4628389830717,0.5,0.546141355518709,0.591012295465604,0.634660406546386,
0.677861768276641,0.720673067745511,0.75,0.774539320541827,0.79898661610755,
0.823367802660232,0.845152365397452,0.861159832875906,0.87718336701521,
0.893272345997422,0.897541889062698,0.90750437030887,0.91782101386449,0.927979055773836,
0.938396106216881,0.948770944531349,0.96157820839839,0.969207846796616,
0.975863277854313,0.981897458390613,0.987341821099734,0.992436269089802,
0.997046562336808,0.999999999999513),.UNSPECIFIED.);
#29411=B_SPLINE_CURVE_WITH_KNOTS('',3,(#107684,#107685,#107686,#107687,
#107688,#107689,#107690,#107691,#107692,#107693,#107694,#107695,#107696,
#107697,#107698,#107699,#107700,#107701,#107702,#107703,#107704,#107705,
#107706,#107707,#107708,#107709,#107710,#107711,#107712,#107713,#107714,
#107715,#107716,#107717,#107718,#107719,#107720,#107721,#107722,#107723,
#107724,#107725,#107726,#107727,#107728,#107729,#107730,#107731,#107732,
#107733,#107734,#107735,#107736,#107737,#107738,#107739,#107740,#107741,
#107742,#107743,#107744,#107745,#107746,#107747,#107748,#107749,#107750,
#107751,#107752,#107753,#107754,#107755,#107756),.UNSPECIFIED.,.F.,.F.,
(4,3,3,3,3,3,3,3,3,3,3,3,3,3,3,3,3,3,3,3,3,3,3,3,4),(0.,0.0434808822299742,
0.0869588497355593,0.130444807126091,0.173924303377971,0.217408477205238,
0.25,0.293489967069525,0.336977356303322,0.380473012066834,0.423962292814937,
0.467456176409864,0.5,0.543489938002949,0.586977312558548,0.630472970571102,
0.673962260376084,0.717456157789405,0.75,0.793396057067662,0.836788578850184,
0.880190246262028,0.923586689734074,0.966991615126708,1.),.UNSPECIFIED.);
#29412=B_SPLINE_CURVE_WITH_KNOTS('',3,(#107761,#107762,#107763,#107764,
#107765,#107766),.UNSPECIFIED.,.F.,.F.,(4,1,1,4),(0.,0.03448275862069,0.06896551724138,
0.0937639678077082),.UNSPECIFIED.);
#29413=B_SPLINE_CURVE_WITH_KNOTS('',3,(#107899,#107900,#107901,#107902,
#107903,#107904,#107905,#107906,#107907,#107908,#107909,#107910,#107911,
#107912,#107913,#107914),.UNSPECIFIED.,.F.,.F.,(4,3,3,3,3,4),(0.,0.262965024567732,
0.294538946299642,0.575526066696717,0.749091361952922,1.),.UNSPECIFIED.);
#29414=B_SPLINE_CURVE_WITH_KNOTS('',3,(#108082,#108083,#108084,#108085,
#108086,#108087,#108088,#108089,#108090,#108091,#108092,#108093,#108094,
#108095,#108096,#108097,#108098,#108099),.UNSPECIFIED.,.F.,.F.,(4,2,2,1,
1,1,1,2,2,2,4),(6.6564892292755E-9,0.250000000000036,0.375000000000054,
0.437500000000063,0.468750000000068,0.48437500000007,0.492187500000071,
0.499023437500072,0.500000000000072,0.750000000000036,1.),.UNSPECIFIED.);
#29415=B_SPLINE_CURVE_WITH_KNOTS('',3,(#108100,#108101,#108102,#108103,
#108104,#108105,#108106,#108107,#108108,#108109,#108110,#108111,#108112,
#108113,#108114,#108115,#108116,#108117,#108118,#108119,#108120,#108121,
#108122,#108123,#108124,#108125,#108126,#108127,#108128,#108129,#108130,
#108131,#108132,#108133,#108134,#108135,#108136),.UNSPECIFIED.,.F.,.F.,
(4,3,3,3,3,3,3,3,3,3,3,3,4),(0.608849847266439,0.6363636363636,0.685017726170025,
0.7272727272727,0.780361478699975,0.786226863948396,0.8181818181818,0.863485254733718,
0.887113979905965,0.9090909090909,0.952071682476561,0.989449454899762,1.),
 .UNSPECIFIED.);
#29416=B_SPLINE_CURVE_WITH_KNOTS('',3,(#108211,#108212,#108213,#108214,
#108215,#108216,#108217,#108218,#108219,#108220,#108221,#108222,#108223,
#108224,#108225,#108226,#108227,#108228,#108229,#108230,#108231,#108232),
 .UNSPECIFIED.,.F.,.F.,(4,2,2,2,2,2,2,2,2,2,4),(-0.940544117189131,-0.619332516558265,
-0.444109071613271,-0.412240309690337,-0.3952445331146,-0.38272974366006,
-0.370302866822156,-0.352494573845886,-0.317827384886972,-0.229879312811828,
-2.62880783342726E-6),.UNSPECIFIED.);
#29417=B_SPLINE_CURVE_WITH_KNOTS('',3,(#108234,#108235,#108236,#108237,
#108238,#108239,#108240,#108241,#108242,#108243,#108244,#108245),
 .UNSPECIFIED.,.F.,.F.,(4,2,2,2,2,4),(-1.93111365758677,-1.63478602703977,
-1.39013179726251,-0.863381002602519,-0.454372300253159,-2.62886509751779E-6),
 .UNSPECIFIED.);
#29418=B_SPLINE_CURVE_WITH_KNOTS('',3,(#108247,#108248,#108249,#108250,
#108251,#108252),.UNSPECIFIED.,.F.,.F.,(4,2,4),(-0.159887729495531,-0.0801211550522599,
-7.07627439308216E-6),.UNSPECIFIED.);
#29419=B_SPLINE_CURVE_WITH_KNOTS('',3,(#108254,#108255,#108256,#108257,
#108258,#108259,#108260,#108261,#108262,#108263,#108264,#108265),
 .UNSPECIFIED.,.F.,.F.,(4,2,2,2,2,4),(-0.109162067299797,-0.0810886277464997,
-0.0548476741806072,-0.0268518386947001,-0.013401596358416,-1.00000063842087E-6),
 .UNSPECIFIED.);
#29420=B_SPLINE_CURVE_WITH_KNOTS('',3,(#108268,#108269,#108270,#108271,
#108272,#108273,#108274,#108275,#108276,#108277,#108278,#108279),
 .UNSPECIFIED.,.F.,.F.,(4,2,2,2,2,4),(2.14051970094785E-5,0.0296331551158527,
0.0592663102294422,0.118532620456621,0.233984090001705,0.34943555954679),
 .UNSPECIFIED.);
#29421=B_SPLINE_CURVE_WITH_KNOTS('',3,(#108285,#108286,#108287,#108288,
#108289,#108290,#108291,#108292,#108293,#108294,#108295,#108296,#108297,
#108298,#108299,#108300,#108301,#108302,#108303,#108304,#108305,#108306,
#108307,#108308,#108309,#108310,#108311,#108312,#108313,#108314,#108315,
#108316,#108317,#108318,#108319,#108320,#108321,#108322,#108323,#108324,
#108325,#108326,#108327,#108328,#108329,#108330,#108331,#108332,#108333,
#108334,#108335,#108336,#108337,#108338,#108339,#108340,#108341,#108342,
#108343,#108344,#108345,#108346,#108347,#108348,#108349,#108350,#108351,
#108352,#108353,#108354,#108355,#108356,#108357,#108358,#108359,#108360,
#108361,#108362,#108363,#108364,#108365,#108366,#108367,#108368,#108369,
#108370,#108371,#108372,#108373,#108374,#108375,#108376,#108377,#108378,
#108379,#108380,#108381,#108382,#108383,#108384,#108385,#108386,#108387,
#108388,#108389,#108390,#108391,#108392,#108393,#108394,#108395,#108396,
#108397,#108398,#108399,#108400,#108401,#108402,#108403,#108404,#108405,
#108406,#108407,#108408,#108409,#108410,#108411,#108412,#108413,#108414,
#108415,#108416,#108417,#108418,#108419,#108420,#108421,#108422,#108423,
#108424,#108425,#108426,#108427,#108428,#108429,#108430,#108431,#108432,
#108433,#108434,#108435,#108436,#108437,#108438,#108439,#108440,#108441,
#108442,#108443,#108444,#108445,#108446,#108447,#108448,#108449,#108450,
#108451,#108452,#108453,#108454,#108455,#108456,#108457,#108458,#108459,
#108460,#108461,#108462,#108463,#108464,#108465,#108466,#108467,#108468,
#108469,#108470,#108471),.UNSPECIFIED.,.F.,.F.,(4,3,3,3,3,3,3,3,3,3,3,3,
3,3,3,3,3,3,3,3,3,3,3,3,3,3,3,3,3,3,3,3,3,3,3,3,3,3,3,3,3,3,3,3,3,3,3,3,
3,3,3,3,3,3,3,3,3,3,3,3,3,3,4),(0.,0.0329872437640412,0.0654476758840371,
0.0969825963291745,0.124999999999463,0.15624999999933,0.185079449321472,
0.187499999999197,0.215101382804894,0.218749999999062,0.234374999998994,
0.242187499998957,0.24609374999894,0.248046874998929,0.249654188187563,
0.249999999998917,0.281763147934628,0.313158438634503,0.344079219316766,
0.374999999999029,0.406249999999055,0.435043122561979,0.437499999999081,
0.465242747494911,0.468749999999105,0.484374999999117,0.492187499999128,
0.496093749999134,0.498046874999133,0.499630666281772,0.499999999999131,
0.534013529034568,0.567884321792066,0.601244268276834,0.624999999999322,
0.656249999999369,0.687499999999416,0.713991711576831,0.718749999999463,
0.734374999999486,0.742187499999503,0.746739145083346,0.749999999999519,
0.773629762604092,0.797741505499532,0.822215741749771,0.847347843083106,
0.854183532832394,0.87006509986984,0.886169192967915,0.902675549776158,
0.905747160718163,0.91628137237736,0.927109967024123,0.938187604547772,
0.94978201511235,0.952873580359081,0.961664311184405,0.972461163011459,
0.98111395701081,0.988582770586387,0.994957883184895,1.),.UNSPECIFIED.);
#29422=B_SPLINE_CURVE_WITH_KNOTS('',3,(#108472,#108473,#108474,#108475,
#108476,#108477,#108478,#108479,#108480,#108481,#108482,#108483,#108484,
#108485,#108486,#108487,#108488,#108489,#108490,#108491,#108492,#108493,
#108494,#108495,#108496,#108497,#108498,#108499,#108500,#108501,#108502,
#108503,#108504,#108505,#108506,#108507,#108508,#108509,#108510,#108511,
#108512,#108513,#108514,#108515,#108516,#108517,#108518,#108519,#108520,
#108521,#108522,#108523,#108524,#108525,#108526,#108527,#108528,#108529,
#108530,#108531,#108532,#108533,#108534,#108535,#108536,#108537,#108538,
#108539,#108540,#108541,#108542,#108543,#108544),.UNSPECIFIED.,.F.,.F.,
(4,3,3,3,3,3,3,3,3,3,3,3,3,3,3,3,3,3,3,3,3,3,3,3,4),(0.,0.0433422658552247,
0.086676909263646,0.13001585118668,0.173347263402444,0.216684760879611,
0.25,0.293486389657058,0.336970195806956,0.380462253926406,0.423947924714859,
0.46743817868338,0.5,0.543486382048098,0.586970181756904,0.63046223937264,
0.673947914476551,0.717438182744027,0.75,0.793486863123022,0.836971158394904,
0.88046371763125,0.923949893701111,0.967440645880335,0.999992112340553),
 .UNSPECIFIED.);
#29423=B_SPLINE_CURVE_WITH_KNOTS('',3,(#108618,#108619,#108620,#108621,
#108622,#108623,#108624,#108625,#108626,#108627,#108628,#108629,#108630,
#108631,#108632,#108633,#108634),.UNSPECIFIED.,.F.,.F.,(4,1,1,1,1,1,1,1,
1,1,1,1,1,1,4),(0.,0.07142857142857,0.1428571428571,0.2142857142857,0.2857142857143,
0.3571428571429,0.4285714285714,0.5,0.5714285714286,0.6428571428571,0.7142857142857,
0.7857142857143,0.8571428571429,0.9285714285714,0.999986468334629),
 .UNSPECIFIED.);
#29424=B_SPLINE_CURVE_WITH_KNOTS('',3,(#108636,#108637,#108638,#108639,
#108640,#108641,#108642,#108643,#108644,#108645,#108646,#108647,#108648,
#108649,#108650,#108651,#108652,#108653,#108654,#108655,#108656,#108657,
#108658,#108659,#108660,#108661,#108662,#108663,#108664,#108665,#108666),
 .UNSPECIFIED.,.F.,.F.,(4,3,3,3,3,3,3,3,3,3,4),(0.,0.115432015922713,0.229642812946616,
0.343276270183446,0.456483616450404,0.5,0.613381340000953,0.727229291454172,
0.841467570588938,0.956691948556023,1.),.UNSPECIFIED.);
#29425=B_SPLINE_CURVE_WITH_KNOTS('',3,(#108667,#108668,#108669,#108670,
#108671,#108672,#108673,#108674,#108675,#108676,#108677,#108678,#108679,
#108680,#108681,#108682,#108683,#108684,#108685,#108686,#108687,#108688,
#108689,#108690,#108691,#108692,#108693,#108694,#108695,#108696,#108697,
#108698,#108699,#108700,#108701,#108702,#108703,#108704,#108705,#108706,
#108707,#108708,#108709,#108710,#108711,#108712,#108713,#108714,#108715,
#108716,#108717,#108718,#108719,#108720,#108721,#108722,#108723,#108724,
#108725,#108726,#108727,#108728,#108729,#108730,#108731,#108732,#108733,
#108734,#108735,#108736,#108737,#108738,#108739,#108740,#108741,#108742,
#108743,#108744,#108745,#108746,#108747,#108748,#108749,#108750,#108751,
#108752,#108753,#108754,#108755,#108756,#108757,#108758,#108759,#108760),
 .UNSPECIFIED.,.F.,.F.,(4,3,3,3,3,3,3,3,3,3,3,3,3,3,3,3,3,3,3,3,3,3,3,3,
3,3,3,3,3,3,3,4),(0.,0.0345582872736374,0.0929845941816202,0.157419102930535,
0.221550743226399,0.22882816245317,0.24999999999998,0.308202198694642,0.38790552997828,
0.396561948834285,0.437499999999966,0.468749999999965,0.484374999999963,
0.492187499999963,0.494958900481429,0.496093749999963,0.498046874999963,
0.499999999999962,0.545721469363609,0.56291392955358,0.608712744210545,
0.631330920648744,0.678550479743205,0.702223009876759,0.749999999999981,
0.775856937482844,0.824689978755202,0.853522500825404,0.902667675715774,
0.936704266922385,0.986072527972056,1.),.UNSPECIFIED.);
#29426=B_SPLINE_CURVE_WITH_KNOTS('',3,(#108789,#108790,#108791,#108792,
#108793,#108794,#108795,#108796,#108797,#108798,#108799,#108800,#108801,
#108802,#108803,#108804),.UNSPECIFIED.,.F.,.F.,(4,3,3,3,3,4),(0.,0.282010262916946,
0.574348464349707,0.70424617169464,0.982799336161222,1.),.UNSPECIFIED.);
#29427=B_SPLINE_CURVE_WITH_KNOTS('',3,(#108805,#108806,#108807,#108808,
#108809,#108810,#108811,#108812,#108813,#108814,#108815,#108816,#108817,
#108818,#108819,#108820,#108821,#108822,#108823),.UNSPECIFIED.,.F.,.F.,
(4,3,3,3,3,3,4),(0.925378193668854,0.92910797034335,0.9487179487179,0.954912373067182,
0.974358974359,0.980737698040363,1.),.UNSPECIFIED.);
#29428=B_SPLINE_CURVE_WITH_KNOTS('',3,(#108965,#108966,#108967,#108968,
#108969,#108970,#108971,#108972,#108973,#108974,#108975,#108976,#108977,
#108978,#108979,#108980,#108981,#108982),.UNSPECIFIED.,.F.,.F.,(4,2,2,2,
1,1,1,1,2,2,4),(0.,0.124999999999973,0.249999999999946,0.37499999999992,
0.437499999999906,0.4687499999999,0.484374999999896,0.492187499999895,0.499023437499893,
0.499999999999893,1.),.UNSPECIFIED.);
#29429=B_SPLINE_CURVE_WITH_KNOTS('',3,(#109081,#109082,#109083,#109084,
#109085,#109086,#109087,#109088,#109089,#109090,#109091,#109092,#109093,
#109094,#109095,#109096,#109097,#109098,#109099,#109100,#109101,#109102,
#109103,#109104,#109105,#109106,#109107,#109108,#109109,#109110,#109111,
#109112,#109113,#109114,#109115,#109116,#109117,#109118,#109119,#109120),
 .UNSPECIFIED.,.F.,.F.,(4,3,3,3,3,3,3,3,3,3,3,3,3,4),(5.38788773699695E-8,
0.0227676697894301,0.0252326097521616,0.0647859254359117,0.09090909090909,
0.125968648152783,0.1688459408452,0.1818181818182,0.220252907477361,0.225296523956686,
0.2727272727273,0.325087831629694,0.3636363636364,0.379334069832486),
 .UNSPECIFIED.);
#29430=B_SPLINE_CURVE_WITH_KNOTS('',3,(#109127,#109128,#109129,#109130,
#109131,#109132,#109133,#109134,#109135,#109136,#109137,#109138,#109139,
#109140,#109141,#109142,#109143,#109144,#109145,#109146,#109147,#109148,
#109149,#109150,#109151,#109152,#109153,#109154,#109155,#109156,#109157,
#109158,#109159,#109160,#109161,#109162,#109163,#109164,#109165,#109166,
#109167,#109168,#109169,#109170),.UNSPECIFIED.,.F.,.F.,(4,2,2,2,2,2,2,2,
2,2,2,2,2,2,2,2,2,2,2,2,2,4),(2.64508255509259,2.67742444567248,2.83696368675036,
2.91868445378747,3.08595278393744,3.2459923366502,3.56763265862368,3.89772471020104,
4.11625324465983,4.27602450013281,4.44011329228324,4.52179781769355,4.68127923539211,
4.85058653401297,5.01076125898609,5.34010312659572,5.4997579249911,5.65126686288735,
5.80859392641738,6.13704517509721,6.31195283117778,6.49346299030963),
 .UNSPECIFIED.);
#29431=B_SPLINE_CURVE_WITH_KNOTS('',3,(#109173,#109174,#109175,#109176,
#109177,#109178,#109179,#109180,#109181,#109182,#109183,#109184,#109185,
#109186,#109187,#109188,#109189,#109190,#109191,#109192,#109193,#109194,
#109195,#109196),.UNSPECIFIED.,.F.,.F.,(4,2,2,2,2,2,2,2,2,2,2,4),(4.15472255972604E-5,
0.17982649437324,0.358364203739333,0.537917209024395,0.774537605184956,
0.933638986493987,1.09395573577978,1.42368019863028,1.5488568065964,1.88031437861517,
2.03196092149598,2.18921446062996),.UNSPECIFIED.);
#29432=B_SPLINE_CURVE_WITH_KNOTS('',3,(#109199,#109200,#109201,#109202,
#109203,#109204,#109205,#109206,#109207,#109208,#109209,#109210,#109211,
#109212,#109213,#109214,#109215,#109216,#109217,#109218,#109219,#109220,
#109221,#109222,#109223,#109224,#109225,#109226,#109227,#109228,#109229,
#109230,#109231,#109232,#109233,#109234,#109235,#109236,#109237,#109238,
#109239,#109240,#109241,#109242,#109243,#109244,#109245,#109246,#109247,
#109248,#109249,#109250,#109251,#109252),.UNSPECIFIED.,.F.,.F.,(4,2,2,2,
2,2,2,2,2,2,2,2,2,2,2,2,2,2,2,2,2,2,2,2,2,2,4),(1.00000000832767E-6,0.0937993211963754,
0.186006529692417,0.371316915687891,0.51521015489977,0.762878301760565,
0.929855471078699,1.26119411668655,1.38653891902511,1.54201439058365,1.77748339152866,
2.01600554589248,2.21643358592222,2.45329646508949,2.64837263290439,2.94654123765676,
3.13520341574287,3.27613465667508,3.60835599039887,3.77341017939711,3.93955099501437,
4.17631270410318,4.33609163100963,4.67139221186229,4.81889318040861,5.08150161034807,
5.28919429578275),.UNSPECIFIED.);
#29433=B_SPLINE_CURVE_WITH_KNOTS('',3,(#109256,#109257,#109258,#109259,
#109260,#109261,#109262,#109263),.UNSPECIFIED.,.F.,.F.,(4,2,2,4),(3.00455393844332E-5,
0.103997999408186,0.20738927106044,0.414937403627889),.UNSPECIFIED.);
#29434=B_SPLINE_CURVE_WITH_KNOTS('',3,(#109265,#109266,#109267,#109268,
#109269,#109270,#109271,#109272,#109273,#109274,#109275,#109276,#109277,
#109278,#109279,#109280,#109281,#109282,#109283,#109284,#109285,#109286,
#109287,#109288,#109289,#109290,#109291,#109292,#109293,#109294),
 .UNSPECIFIED.,.F.,.F.,(4,2,2,2,2,2,2,2,2,2,2,2,2,2,4),(0.000332275491302904,
0.0840966458402627,0.166687246349549,0.242589704370946,0.456211102935291,
0.570011730232724,0.811990911514058,0.947245253154911,1.11349936008019,
1.2791925587542,1.60988734602343,1.76049112393223,1.97945211479166,2.10332751572814,
2.22822768913076),.UNSPECIFIED.);
#29435=B_SPLINE_CURVE_WITH_KNOTS('',3,(#109295,#109296,#109297,#109298,
#109299,#109300,#109301,#109302,#109303,#109304,#109305,#109306,#109307,
#109308,#109309,#109310,#109311,#109312,#109313,#109314,#109315,#109316,
#109317,#109318,#109319,#109320,#109321,#109322),.UNSPECIFIED.,.F.,.F.,
(4,2,2,2,2,2,2,2,2,2,2,2,2,4),(9.99999997225233E-7,0.316380988376829,0.420339193601812,
0.746639351878567,0.902016774938394,1.06080893086254,1.22053675681677,1.54934292636645,
1.70751623430856,1.85716806248915,2.01680576343376,2.34625710726857,2.50713459399319,
2.64508255509259),.UNSPECIFIED.);
#29436=B_SPLINE_CURVE_WITH_KNOTS('',3,(#109327,#109328,#109329,#109330,
#109331,#109332,#109333,#109334,#109335,#109336,#109337,#109338,#109339,
#109340,#109341,#109342,#109343,#109344,#109345,#109346,#109347,#109348,
#109349,#109350,#109351,#109352,#109353,#109354,#109355,#109356,#109357,
#109358,#109359,#109360,#109361,#109362,#109363,#109364,#109365,#109366,
#109367,#109368,#109369,#109370,#109371,#109372,#109373,#109374,#109375,
#109376,#109377,#109378),.UNSPECIFIED.,.F.,.F.,(4,2,2,2,2,2,2,2,2,2,2,2,
2,2,2,2,2,2,2,2,2,2,2,2,2,4),(1.08729832187199,1.17595088380344,1.33778570454322,
1.61392601185733,1.7757756305946,2.05493223416506,2.21679753879183,2.54025561678765,
2.7026900931946,2.86620583049052,3.18933753411709,3.35213283091687,3.67938788358257,
3.84130843842076,4.17584086404189,4.33859835896819,4.50095601740349,4.66406304349631,
4.99307628290177,5.15514214643947,5.48970140028481,5.57141128126531,5.89662036271308,
6.01657896885547,6.19774098437255,6.37927915487514),.UNSPECIFIED.);
#29437=B_SPLINE_CURVE_WITH_KNOTS('',3,(#109380,#109381,#109382,#109383,
#109384,#109385,#109386,#109387,#109388,#109389,#109390,#109391,#109392,
#109393,#109394,#109395,#109396,#109397,#109398,#109399,#109400,#109401,
#109402,#109403,#109404,#109405,#109406,#109407,#109408,#109409,#109410,
#109411,#109412,#109413,#109414,#109415,#109416,#109417,#109418,#109419,
#109420,#109421,#109422,#109423,#109424,#109425,#109426,#109427,#109428,
#109429,#109430,#109431),.UNSPECIFIED.,.F.,.F.,(4,2,2,2,2,2,2,2,2,2,2,2,
2,2,2,2,2,2,2,2,2,2,2,2,2,4),(5.28919429578275,5.3324848721458,5.49310439715847,
5.73141270289315,5.96292206244042,6.11206963141141,6.25697378422631,6.58716063505421,
6.79605341158305,7.04034155290596,7.19896984076246,7.43590957632683,7.59911565187969,
7.85553254220341,7.99989361468925,8.33497198064668,8.49404727731464,8.73066918018472,
8.90981619304874,9.07479140820227,9.40588960985194,9.55500945800335,9.70146218968651,
9.81681549265543,9.98709458790283,10.1622070063764),.UNSPECIFIED.);
#29438=B_SPLINE_CURVE_WITH_KNOTS('',3,(#109432,#109433,#109434,#109435,
#109436,#109437),.UNSPECIFIED.,.F.,.F.,(4,2,4),(9.84111781119226E-6,0.225748591139482,
0.415214370670141),.UNSPECIFIED.);
#29439=B_SPLINE_CURVE_WITH_KNOTS('',3,(#109443,#109444,#109445,#109446,
#109447,#109448,#109449,#109450,#109451,#109452,#109453,#109454),
 .UNSPECIFIED.,.F.,.F.,(4,2,2,2,2,4),(-1.08694468321814,-0.849318901329702,
-0.686604059603595,-0.524313844518721,-0.264814390599367,-9.9999999880751E-7),
 .UNSPECIFIED.);
#29440=B_SPLINE_CURVE_WITH_KNOTS('',3,(#109458,#109459,#109460,#109461,
#109462,#109463),.UNSPECIFIED.,.F.,.F.,(4,2,4),(4.25996487515901E-5,0.058348665794391,
0.103898374931251),.UNSPECIFIED.);
#29441=B_SPLINE_CURVE_WITH_KNOTS('',3,(#109464,#109465,#109466,#109467,
#109468,#109469,#109470,#109471,#109472,#109473,#109474,#109475,#109476,
#109477,#109478,#109479,#109480,#109481,#109482,#109483,#109484,#109485,
#109486,#109487),.UNSPECIFIED.,.F.,.F.,(4,2,2,2,2,2,2,2,2,2,2,4),(-3.06207312432449,
-2.78609444561215,-2.51065494233778,-2.23496348902561,-1.90651189086599,
-1.69364069136703,-1.53125874524034,-1.36663044472209,-1.04803598247908,
-0.761188827947358,-0.444145659374973,-0.415211727770225),.UNSPECIFIED.);
#29442=B_SPLINE_CURVE_WITH_KNOTS('',3,(#109492,#109493,#109494,#109495,
#109496,#109497,#109498,#109499,#109500,#109501,#109502,#109503,#109504,
#109505,#109506,#109507,#109508,#109509,#109510,#109511,#109512,#109513,
#109514,#109515,#109516,#109517,#109518,#109519,#109520,#109521,#109522,
#109523,#109524,#109525,#109526,#109527,#109528,#109529,#109530,#109531,
#109532,#109533,#109534,#109535,#109536,#109537,#109538,#109539,#109540,
#109541,#109542,#109543),.UNSPECIFIED.,.F.,.F.,(4,2,2,2,2,2,2,2,2,2,2,2,
2,2,2,2,2,2,2,2,2,2,2,2,2,4),(-6.3789533061886,-6.19752540699852,-6.01647535816193,
-5.89659061833356,-5.57148058423157,-5.48976790348919,-5.15521209696545,
-4.99315258417474,-4.66417843590823,-4.50108218501608,-4.33870537818856,
-4.17593333632225,-3.84140152444433,-3.67948513698676,-3.35232154086754,
-3.18953825850364,-2.86636304145829,-2.70286273730807,-2.54041822649752,
-2.21681608328943,-2.05495155736083,-1.77714959629158,-1.61530229675366,
-1.34565532190014,-1.18376871477307,-1.08694468321814),.UNSPECIFIED.);
#29443=B_SPLINE_CURVE_WITH_KNOTS('',3,(#109545,#109546,#109547,#109548,
#109549,#109550),.UNSPECIFIED.,.F.,.F.,(4,2,4),(-0.415211727770225,-0.225749000382965,
-7.22216956189878E-6),.UNSPECIFIED.);
#29444=B_SPLINE_CURVE_WITH_KNOTS('',3,(#109551,#109552,#109553,#109554,
#109555,#109556,#109557,#109558,#109559,#109560,#109561,#109562,#109563,
#109564,#109565,#109566,#109567,#109568,#109569,#109570,#109571,#109572,
#109573,#109574,#109575,#109576,#109577,#109578,#109579,#109580,#109581,
#109582,#109583,#109584,#109585,#109586,#109587,#109588,#109589,#109590,
#109591,#109592,#109593,#109594,#109595,#109596,#109597,#109598,#109599,
#109600),.UNSPECIFIED.,.F.,.F.,(4,2,2,2,2,2,2,2,2,2,2,2,2,2,2,2,2,2,2,2,
2,2,2,2,4),(-10.162288201987,-9.95449044952228,-9.74761344805875,-9.61484561556136,
-9.28928775962058,-9.14607554855514,-8.89667320787399,-8.75278270818488,
-8.5120156150304,-8.30763540975586,-8.07065964378126,-7.91068566964841,
-7.57538438350904,-7.42685701181995,-7.16273754121012,-6.95127001708957,
-6.81320480002116,-6.59034568908175,-6.26098331233411,-6.12764696294493,
-5.97014605611139,-5.73247499024949,-5.49383205799769,-5.33310123773781,
-5.28894858945498),.UNSPECIFIED.);
#29445=B_SPLINE_CURVE_WITH_KNOTS('',3,(#109606,#109607,#109608,#109609,
#109610,#109611,#109612,#109613,#109614,#109615,#109616,#109617,#109618,
#109619,#109620,#109621,#109622,#109623,#109624,#109625,#109626,#109627,
#109628,#109629),.UNSPECIFIED.,.F.,.F.,(4,2,2,2,2,2,2,2,2,2,2,4),(-2.18921446063053,
-2.03196092150216,-1.88031437862538,-1.54885680660905,-1.42368019863116,
-1.09395573578003,-0.93363898649323,-0.774537605184621,-0.537917209023631,
-0.358364203732708,-0.179826494370147,-4.1547225594898E-5),
 .UNSPECIFIED.);
#29446=B_SPLINE_CURVE_WITH_KNOTS('',3,(#109632,#109633,#109634,#109635,
#109636,#109637,#109638,#109639,#109640,#109641,#109642,#109643,#109644,
#109645,#109646,#109647,#109648,#109649,#109650,#109651,#109652,#109653,
#109654,#109655,#109656,#109657,#109658,#109659,#109660,#109661,#109662,
#109663,#109664,#109665,#109666,#109667,#109668,#109669,#109670,#109671,
#109672,#109673,#109674,#109675,#109676,#109677),.UNSPECIFIED.,.F.,.F.,
(4,2,2,2,2,2,2,2,2,2,2,2,2,2,2,2,2,2,2,2,2,2,4),(-6.49276334357195,-6.26669129627648,
-6.04438319173055,-5.89990959341052,-5.74011293729422,-5.41181691433256,
-5.25476581773821,-5.10256055685507,-4.94289957223829,-4.6136056717894,
-4.45367107155358,-4.30712152953011,-4.14751266919742,-3.81785037133824,
-3.65541399409842,-3.48831833314667,-3.32879089951008,-3.24707909133012,
-3.08698762043823,-2.91705494880014,-2.83535718105171,-2.67585877419533,
-2.64509018645311),.UNSPECIFIED.);
#29447=B_SPLINE_CURVE_WITH_KNOTS('',3,(#109683,#109684,#109685,#109686,
#109687,#109688,#109689,#109690,#109691,#109692,#109693,#109694,#109695,
#109696,#109697,#109698,#109699,#109700,#109701,#109702,#109703,#109704,
#109705,#109706,#109707,#109708,#109709,#109710,#109711,#109712,#109713,
#109714,#109715,#109716,#109717,#109718,#109719,#109720,#109721,#109722),
 .UNSPECIFIED.,.F.,.F.,(4,2,2,2,2,2,2,2,2,2,2,2,2,2,2,2,2,2,2,4),(45.1636811624521,
45.1859895775379,45.2909818652286,45.5404043845585,45.7173330695028,45.8583336706336,
46.1022835664149,46.3125310429476,46.5254507861948,46.7755846171368,46.9899008738256,
47.1935127202563,47.4417976479436,47.6581123658742,47.8657808033474,48.1142491024031,
48.3347494994277,48.4289037755271,48.5489428743058,48.7694667551308),
 .UNSPECIFIED.);
#29448=B_SPLINE_CURVE_WITH_KNOTS('',3,(#109725,#109726,#109727,#109728,
#109729,#109730,#109731,#109732,#109733,#109734,#109735,#109736,#109737,
#109738,#109739,#109740,#109741,#109742,#109743,#109744,#109745,#109746,
#109747,#109748,#109749,#109750,#109751,#109752,#109753,#109754,#109755,
#109756,#109757,#109758,#109759,#109760,#109761,#109762,#109763,#109764),
 .UNSPECIFIED.,.F.,.F.,(4,2,2,2,2,2,2,2,2,2,2,2,2,2,2,2,2,2,2,4),(0.,0.2201415667957,
0.339971629687818,0.439268623717367,0.656555209190466,0.904321640813465,
1.10966254441214,1.32710919499732,1.57591624251713,1.7795942888701,1.99387887225677,
2.24400153032728,2.45689921852262,2.66715220225339,2.91106168072629,3.052663104263,
3.22941548161296,3.48018527327844,3.58427704060106,3.60575464092561),
 .UNSPECIFIED.);
#29449=B_SPLINE_CURVE_WITH_KNOTS('',3,(#109769,#109770,#109771,#109772,
#109773,#109774,#109775,#109776,#109777,#109778,#109779,#109780,#109781,
#109782,#109783,#109784,#109785,#109786,#109787,#109788,#109789,#109790,
#109791,#109792,#109793,#109794,#109795,#109796,#109797,#109798,#109799,
#109800,#109801,#109802,#109803,#109804,#109805,#109806,#109807,#109808,
#109809,#109810,#109811,#109812,#109813,#109814,#109815,#109816,#109817,
#109818,#109819,#109820,#109821,#109822,#109823,#109824,#109825,#109826,
#109827,#109828,#109829,#109830,#109831,#109832,#109833,#109834,#109835,
#109836,#109837,#109838,#109839,#109840,#109841,#109842,#109843,#109844,
#109845,#109846,#109847,#109848,#109849,#109850,#109851,#109852,#109853,
#109854,#109855,#109856,#109857,#109858,#109859,#109860,#109861,#109862,
#109863,#109864,#109865,#109866,#109867,#109868,#109869,#109870,#109871,
#109872,#109873,#109874,#109875,#109876,#109877,#109878,#109879,#109880),
 .UNSPECIFIED.,.F.,.F.,(4,2,2,2,2,2,2,2,2,2,2,2,2,2,2,2,2,2,2,2,2,2,2,2,
2,2,2,2,2,2,2,2,2,2,2,2,2,2,2,2,2,2,2,2,2,2,2,2,2,2,2,2,2,2,2,4),(34.4761216253511,
34.4979172951594,34.6023693954826,34.8526887743558,35.0295472782581,35.1709371656285,
35.4189309688937,35.6359352997608,35.8328963334246,35.9362065969497,36.1876018834163,
36.3639547026121,36.5070333217856,36.7546764575407,36.971106225807,37.1692923075338,
37.2730069669589,37.524393883275,37.7010920830533,37.8430292585465,38.0906378467652,
38.3070037787261,38.5053127979877,38.6090676395425,38.8603863189785,39.0370895140391,
39.1789876391809,39.4263179204561,39.6421303069469,39.8416408578658,39.9458004001765,
40.1965152151265,40.3732998895649,40.5148766763876,40.7643540376504,40.9849038360371,
41.1837686424467,41.4322349228299,41.6466582370236,41.8500979980946,42.0970191531081,
42.3106845724003,42.5150805514149,42.6209619147639,42.869039564485,43.0461288157834,
43.1866492687327,43.4306106150213,43.6408570981889,43.8538204907908,44.1039835109216,
44.3183594933174,44.5218709671828,44.7693560633028,44.9840659861086,45.1636811624521),
 .UNSPECIFIED.);
#29450=B_SPLINE_CURVE_WITH_KNOTS('',3,(#109881,#109882,#109883,#109884,
#109885,#109886,#109887,#109888,#109889,#109890,#109891,#109892,#109893,
#109894,#109895,#109896,#109897,#109898,#109899,#109900,#109901,#109902,
#109903,#109904,#109905,#109906,#109907,#109908,#109909,#109910,#109911,
#109912,#109913,#109914,#109915,#109916,#109917,#109918,#109919,#109920,
#109921,#109922,#109923,#109924,#109925,#109926,#109927,#109928,#109929,
#109930,#109931,#109932,#109933,#109934,#109935,#109936,#109937,#109938,
#109939,#109940,#109941,#109942,#109943,#109944,#109945,#109946,#109947,
#109948,#109949,#109950,#109951,#109952,#109953,#109954,#109955,#109956,
#109957,#109958,#109959,#109960,#109961,#109962,#109963,#109964,#109965,
#109966,#109967,#109968,#109969,#109970,#109971,#109972,#109973,#109974,
#109975,#109976,#109977,#109978,#109979,#109980,#109981,#109982,#109983,
#109984,#109985,#109986,#109987,#109988,#109989,#109990,#109991,#109992),
 .UNSPECIFIED.,.F.,.F.,(4,2,2,2,2,2,2,2,2,2,2,2,2,2,2,2,2,2,2,2,2,2,2,2,
2,2,2,2,2,2,2,2,2,2,2,2,2,2,2,2,2,2,2,2,2,2,2,2,2,2,2,2,2,2,2,4),(3.60575464092561,
3.78359886408125,3.99946083484741,4.24708388702773,4.39236370283358,4.56793595394828,
4.8186906336666,4.92138850485364,5.11647310940841,5.33431338911229,5.58259250518372,
5.72459723690218,5.9012529332293,6.15275589785826,6.25635973945805,6.45422443026423,
6.67076629369559,6.91871291519129,7.06376525715824,7.23942224292656,7.49025154511468,
7.59301626702443,7.78830418819424,8.00606241048629,8.25472024889112,8.45938882436026,
8.6732843485801,8.92149695428521,9.12149373452797,9.34120210231813,9.59035578276094,
9.73190774048285,9.90870126959051,10.159367954283,10.2635642219125,10.398281453743,
10.5764045119693,10.807132946455,10.923513855605,11.1373467101536,11.3475658062745,
11.5943089788604,11.8094599884568,12.0189302366049,12.263042231856,12.466391556441,
12.68088166963,12.9311089195156,13.1441582158934,13.3544140888988,13.5983720406559,
13.7397004466345,13.9165747479684,14.1667613476217,14.2713015560327,14.2931793607378),
 .UNSPECIFIED.);
#29451=B_SPLINE_CURVE_WITH_KNOTS('',3,(#109997,#109998,#109999,#110000,
#110001,#110002,#110003,#110004,#110005,#110006,#110007,#110008,#110009,
#110010,#110011,#110012,#110013,#110014,#110015,#110016,#110017,#110018,
#110019,#110020,#110021,#110022,#110023,#110024,#110025,#110026,#110027,
#110028,#110029,#110030,#110031,#110032,#110033,#110034,#110035,#110036,
#110037,#110038,#110039,#110040,#110041,#110042,#110043,#110044,#110045,
#110046,#110047,#110048,#110049,#110050,#110051,#110052,#110053,#110054,
#110055,#110056,#110057,#110058,#110059,#110060,#110061,#110062,#110063,
#110064,#110065,#110066,#110067,#110068,#110069,#110070,#110071,#110072,
#110073,#110074,#110075,#110076,#110077,#110078,#110079,#110080,#110081,
#110082,#110083,#110084,#110085,#110086,#110087,#110088,#110089,#110090,
#110091,#110092,#110093,#110094,#110095,#110096,#110097,#110098,#110099,
#110100,#110101,#110102,#110103,#110104,#110105,#110106,#110107,#110108,
#110109,#110110),.UNSPECIFIED.,.F.,.F.,(4,2,2,2,2,2,2,2,2,2,2,2,2,2,2,2,
2,2,2,2,2,2,2,2,2,2,2,2,2,2,2,2,2,2,2,2,2,2,2,2,2,2,2,2,2,2,2,2,2,2,2,2,
2,2,2,2,4),(23.7864907164679,23.8600639976838,24.0542846994271,24.3840968250959,
24.4971715165633,24.6330208701138,24.8469376514058,25.0346122986433,25.1606329989249,
25.2855425024337,25.5042341007853,25.6834576792019,25.8267691843993,25.9520184150769,
26.1697796229055,26.3490328893123,26.481026560496,26.5857283218547,26.835737628172,
27.0126691422952,27.1539259336804,27.4033991467519,27.6237508415675,27.8230105963696,
28.0714965084728,28.2858833510739,28.4895842322703,28.7380762425912,28.9547166091719,
29.1525471320625,29.2561491615275,29.50776076928,29.6844576808734,29.8265266170278,
30.0751049001722,30.2935384751636,30.4932806994328,30.6019456262967,30.845689151055,
31.0231916363084,31.1626154796419,31.4119757064893,31.6321290211168,31.8316181013685,
32.0800461296406,32.2943364330095,32.4982050554351,32.7422107336455,32.9517436244225,
33.1667909413486,33.4109673000422,33.6180184359698,33.8403444537529,33.9603314256126,
34.1855282423232,34.3640236325502,34.4761216253511),.UNSPECIFIED.);
#29452=B_SPLINE_CURVE_WITH_KNOTS('',3,(#110111,#110112,#110113,#110114,
#110115,#110116,#110117,#110118,#110119,#110120,#110121,#110122,#110123,
#110124,#110125,#110126,#110127,#110128,#110129,#110130,#110131,#110132,
#110133,#110134,#110135,#110136,#110137,#110138,#110139,#110140,#110141,
#110142,#110143,#110144,#110145,#110146,#110147,#110148,#110149,#110150,
#110151,#110152,#110153,#110154,#110155,#110156,#110157,#110158,#110159,
#110160,#110161,#110162,#110163,#110164,#110165,#110166,#110167,#110168,
#110169,#110170,#110171,#110172,#110173,#110174,#110175,#110176,#110177,
#110178,#110179,#110180,#110181,#110182,#110183,#110184,#110185,#110186,
#110187,#110188,#110189,#110190,#110191,#110192,#110193,#110194,#110195,
#110196,#110197,#110198,#110199,#110200,#110201,#110202,#110203,#110204,
#110205,#110206,#110207,#110208,#110209,#110210,#110211,#110212,#110213,
#110214,#110215,#110216,#110217,#110218),.UNSPECIFIED.,.F.,.F.,(4,2,2,2,
2,2,2,2,2,2,2,2,2,2,2,2,2,2,2,2,2,2,2,2,2,2,2,2,2,2,2,2,2,2,2,2,2,2,2,2,
2,2,2,2,2,2,2,2,2,2,2,2,2,4),(14.2931793607378,14.4719098425484,14.6872583759001,
14.9351026692841,15.1386971335507,15.3530966410328,15.6033037705098,15.8162964769165,
16.0265891038553,16.2706031058181,16.4112504626503,16.5883428601802,16.8367703417248,
16.9424796939961,17.1463839003186,17.3603166283152,17.6074137217094,17.8109118097724,
18.0253695011367,18.2738820176566,18.4728078227829,18.6933852905092,18.941885950872,
19.1507625149527,19.3629700308906,19.6117464009867,19.8250974060452,20.035279940003,
20.2791833581233,20.4206775644385,20.5975340742559,20.8480724242665,20.9524141261965,
21.0868029155594,21.2651217691753,21.4932588084231,21.6113526553399,21.8291758340079,
22.0379331058812,22.2817432043622,22.5020467265233,22.7097652725934,22.9539842354375,
23.0867579418792,23.3199522342735,23.4885961536804,23.6723009005603,23.916471372828,
24.1224173322998,24.3480071497465,24.4694211502622,24.6925614637182,24.8712489134122,
24.9828701266438),.UNSPECIFIED.);
#29453=B_SPLINE_CURVE_WITH_KNOTS('',3,(#110223,#110224,#110225,#110226,
#110227,#110228,#110229,#110230,#110231,#110232,#110233,#110234,#110235,
#110236,#110237,#110238,#110239,#110240,#110241,#110242,#110243,#110244,
#110245,#110246,#110247,#110248,#110249,#110250,#110251,#110252,#110253,
#110254,#110255,#110256,#110257,#110258,#110259,#110260,#110261,#110262,
#110263,#110264,#110265,#110266,#110267,#110268,#110269,#110270,#110271,
#110272,#110273,#110274,#110275,#110276,#110277,#110278,#110279,#110280,
#110281,#110282,#110283,#110284,#110285,#110286,#110287,#110288,#110289,
#110290,#110291,#110292,#110293,#110294,#110295,#110296,#110297,#110298,
#110299,#110300,#110301,#110302,#110303,#110304,#110305,#110306,#110307,
#110308,#110309,#110310,#110311,#110312,#110313,#110314,#110315,#110316,
#110317,#110318,#110319,#110320,#110321,#110322,#110323,#110324,#110325,
#110326,#110327,#110328,#110329,#110330,#110331,#110332,#110333,#110334,
#110335,#110336,#110337,#110338),.UNSPECIFIED.,.F.,.F.,(4,2,2,2,2,2,2,2,
2,2,2,2,2,2,2,2,2,2,2,2,2,2,2,2,2,2,2,2,2,2,2,2,2,2,2,2,2,2,2,2,2,2,2,2,
2,2,2,2,2,2,2,2,2,2,2,2,2,4),(13.0972599015927,13.2088828109584,13.3875334083998,
13.6107174250379,13.7320572875133,13.9574866046717,14.1634411494772,14.4074934721232,
14.6198640778286,14.830385732743,15.0744021000641,15.2121076743174,15.3901968600944,
15.6232620182162,15.7384871167831,15.9428362432387,16.1617584586995,16.4106155859748,
16.552127272608,16.7289621853694,16.9795405830886,17.0838343658739,17.2183386710432,
17.3965893870818,17.6255881568458,17.7431067818442,17.9442863416335,18.1631905505658,
18.4147148656307,18.6302600478368,18.8396270523619,19.0836785105287,19.2870272477183,
19.5015598569899,19.7501128405144,19.9487018496239,20.1695396125155,20.4190495433896,
20.5567802222878,20.7348844425986,20.9680455918345,21.0832382004914,21.2873872231948,
21.5064642813777,21.7554244536792,21.8966798707429,22.0736115378505,22.3236200606198,
22.4283237575531,22.5602905911023,22.7395532376602,22.9572385707407,23.0825455561075,
23.2257497280802,23.4050230633458,23.5985515058283,23.7392262097004,23.7864907164679),
 .UNSPECIFIED.);
#29454=B_SPLINE_CURVE_WITH_KNOTS('',3,(#110339,#110340,#110341,#110342,
#110343,#110344,#110345,#110346,#110347,#110348,#110349,#110350,#110351,
#110352,#110353,#110354,#110355,#110356,#110357,#110358,#110359,#110360,
#110361,#110362,#110363,#110364,#110365,#110366,#110367,#110368,#110369,
#110370,#110371,#110372,#110373,#110374,#110375,#110376,#110377,#110378,
#110379,#110380,#110381,#110382,#110383,#110384,#110385,#110386,#110387,
#110388,#110389,#110390,#110391,#110392,#110393,#110394,#110395,#110396,
#110397,#110398,#110399,#110400,#110401,#110402,#110403,#110404,#110405,
#110406,#110407,#110408,#110409,#110410,#110411,#110412,#110413,#110414,
#110415,#110416,#110417,#110418,#110419,#110420,#110421,#110422,#110423,
#110424,#110425,#110426,#110427,#110428,#110429,#110430,#110431,#110432,
#110433,#110434,#110435,#110436,#110437,#110438,#110439,#110440,#110441,
#110442,#110443,#110444,#110445,#110446,#110447,#110448,#110449,#110450),
 .UNSPECIFIED.,.F.,.F.,(4,2,2,2,2,2,2,2,2,2,2,2,2,2,2,2,2,2,2,2,2,2,2,2,
2,2,2,2,2,2,2,2,2,2,2,2,2,2,2,2,2,2,2,2,2,2,2,2,2,2,2,2,2,2,2,4),(24.9828701266438,
25.0047437426501,25.1092917244477,25.3595256298742,25.536425165321,25.6777802263797,
25.9269916394664,26.146704044784,26.3467271041175,26.5945217846717,26.8075316126368,
27.0144611916814,27.2623182684099,27.479834605962,27.6757810316877,27.7787657608995,
28.0298495783055,28.2057922252096,28.3501372639755,28.5941240660552,28.804267754094,
29.0176912708963,29.1270790527437,29.3696427046905,29.5472215910744,29.6864116441914,
29.9338935621333,30.1498971464094,30.3490772925246,30.4531295853532,30.7040580372953,
30.8808418343143,31.0225290299326,31.2706128526426,31.4878561599192,31.6843333167744,
31.7874871124857,32.0387306114881,32.2148840736119,32.3585605441454,32.6073592275527,
32.8260861401882,33.0307434417365,33.1460277507439,33.3789808560992,33.5570691230152,
33.6947547740834,33.944640995557,34.1665970254851,34.3635944165894,34.6121184634748,
34.8266361796678,35.0299201573721,35.2739093239344,35.4831982054315,35.6719042779843),
 .UNSPECIFIED.);
#29455=B_SPLINE_CURVE_WITH_KNOTS('',3,(#110457,#110458,#110459,#110460,
#110461,#110462,#110463,#110464,#110465,#110466,#110467,#110468,#110469,
#110470,#110471,#110472,#110473,#110474,#110475,#110476,#110477,#110478,
#110479,#110480,#110481,#110482),.UNSPECIFIED.,.F.,.F.,(4,2,2,2,2,2,2,2,
2,2,2,2,4),(1.0000000086885E-6,0.368005088305128,0.597205559032035,0.80384623486168,
1.04823515581348,1.26147811522057,1.47159759188732,1.71543402139935,1.85674376816772,
2.03357552274096,2.28373478672066,2.38823344563787,2.41008863111305),
 .UNSPECIFIED.);
#29456=B_SPLINE_CURVE_WITH_KNOTS('',3,(#110488,#110489,#110490,#110491,
#110492,#110493,#110494,#110495,#110496,#110497,#110498,#110499,#110500,
#110501,#110502,#110503,#110504,#110505,#110506,#110507,#110508,#110509,
#110510,#110511,#110512,#110513,#110514,#110515,#110516,#110517,#110518,
#110519,#110520,#110521,#110522,#110523,#110524,#110525,#110526,#110527,
#110528,#110529,#110530,#110531,#110532,#110533,#110534,#110535,#110536,
#110537,#110538,#110539,#110540,#110541,#110542,#110543,#110544,#110545,
#110546,#110547,#110548,#110549,#110550,#110551,#110552,#110553,#110554,
#110555,#110556,#110557,#110558,#110559,#110560,#110561,#110562,#110563,
#110564,#110565),.UNSPECIFIED.,.F.,.F.,(4,2,2,2,2,2,2,2,2,2,2,2,2,2,2,2,
2,2,2,2,2,2,2,2,2,2,2,2,2,2,2,2,2,2,2,2,2,2,4),(-6.04591668252116,-6.00476951035527,
-5.87222595335921,-5.67235526281456,-5.48950750851185,-5.36878304006732,
-5.24465029945799,-5.03006846521196,-4.84621171253538,-4.71821442823858,
-4.58567217775998,-4.38580592098932,-4.20296115284965,-4.08223804754818,
-3.95810761088525,-3.74352838666824,-3.55967449478355,-3.43167889162868,
-3.29913885159351,-3.09927498044057,-2.91643280631889,-2.79571164775362,
-2.67158286570741,-2.45700702974226,-2.27315580075226,-2.14516217087974,
-2.0126239935607,-1.8127632957672,-1.6299238664427,-1.50920443010279,-1.38507755238952,
-1.17050480527998,-0.986656315246761,-0.858664546249773,-0.72612836535116,
-0.518106196771695,-0.329531023944945,-0.208588893485145,0.),
 .UNSPECIFIED.);
#29457=B_SPLINE_CURVE_WITH_KNOTS('',3,(#110569,#110570,#110571,#110572,
#110573,#110574,#110575,#110576,#110577,#110578,#110579,#110580,#110581,
#110582,#110583,#110584,#110585,#110586,#110587,#110588,#110589,#110590,
#110591,#110592,#110593,#110594,#110595,#110596,#110597,#110598,#110599,
#110600,#110601,#110602,#110603,#110604,#110605,#110606,#110607,#110608,
#110609,#110610,#110611,#110612,#110613,#110614,#110615,#110616,#110617,
#110618,#110619,#110620,#110621,#110622,#110623,#110624,#110625,#110626,
#110627,#110628,#110629,#110630,#110631,#110632,#110633,#110634,#110635,
#110636,#110637,#110638,#110639,#110640,#110641,#110642,#110643,#110644,
#110645,#110646),.UNSPECIFIED.,.F.,.F.,(4,2,2,2,2,2,2,2,2,2,2,2,2,2,2,2,
2,2,2,2,2,2,2,2,2,2,2,2,2,2,2,2,2,2,2,2,2,2,4),(-44.7046953009418,-44.4961174550277,
-44.3751813824112,-44.1866150987334,-43.9786034224711,-43.8460746896715,
-43.7180893074422,-43.5342494045959,-43.319687980552,-43.1955677260083,
-43.0748545558397,-42.8920235107033,-42.6921725900386,-42.5596418820413,
-42.4316545870372,-42.2478119418575,-42.0332473087007,-41.9091252070089,
-41.7884102301501,-41.6055764593785,-41.4057225730062,-41.2731898792282,
-41.145200680294,-40.9613552867331,-40.7467874680579,-40.6226634994675,
-40.5019467336222,-40.3191102252629,-40.1192533109191,-39.9867186587913,
-39.8587275328118,-39.674879406461,-39.4603083407335,-39.3361825565139,
-39.2154639555481,-39.0326247405373,-38.8327649599833,-38.7002282780622,
-38.6590831067128),.UNSPECIFIED.);
#29458=B_SPLINE_CURVE_WITH_KNOTS('',3,(#110652,#110653,#110654,#110655,
#110656,#110657,#110658,#110659,#110660,#110661,#110662,#110663,#110664,
#110665,#110666,#110667,#110668,#110669,#110670,#110671,#110672,#110673,
#110674,#110675,#110676,#110677,#110678,#110679,#110680,#110681,#110682,
#110683,#110684,#110685,#110686,#110687,#110688,#110689,#110690,#110691,
#110692,#110693,#110694,#110695,#110696,#110697,#110698,#110699,#110700,
#110701,#110702,#110703,#110704,#110705,#110706,#110707,#110708,#110709,
#110710,#110711,#110712,#110713,#110714,#110715,#110716,#110717,#110718,
#110719,#110720,#110721,#110722,#110723,#110724,#110725,#110726,#110727,
#110728,#110729,#110730,#110731,#110732,#110733,#110734,#110735,#110736,
#110737,#110738,#110739,#110740,#110741,#110742,#110743,#110744,#110745,
#110746,#110747,#110748,#110749,#110750,#110751,#110752,#110753,#110754,
#110755,#110756,#110757,#110758,#110759,#110760,#110761,#110762,#110763,
#110764,#110765,#110766,#110767,#110768,#110769,#110770,#110771,#110772,
#110773,#110774,#110775,#110776,#110777,#110778,#110779,#110780,#110781,
#110782,#110783),.UNSPECIFIED.,.F.,.F.,(4,2,2,2,2,2,2,2,2,2,2,2,2,2,2,2,
2,2,2,2,2,2,2,2,2,2,2,2,2,2,2,2,2,2,2,2,2,2,2,2,2,2,2,2,2,2,2,2,2,2,2,2,
2,2,2,2,2,2,2,2,2,2,2,2,2,4),(-38.6590831067128,-38.5722352850204,-38.3883843851979,
-38.1738102322154,-38.0496824989805,-37.9289621827312,-37.7461201804974,
-37.5462571130413,-37.4137185869527,-37.2857235708196,-37.1018700031292,
-36.8872923472881,-36.7631630117032,-36.6424406685207,-36.4595960883871,
-36.2597308275695,-36.1271899746231,-35.9991933409473,-35.8153368306907,
-35.6007567523108,-35.47662491301,-35.3559013530122,-35.1730536506359,-34.9731833533706,
-34.8406414283239,-34.7126421226622,-34.5287833838445,-34.314198074117,
-34.190066074372,-34.0693391912543,-33.886489781691,-33.6866218396677,-33.5540755800713,
-33.426076343729,-33.2422135198448,-33.0276302806854,-32.9034920284243,
-32.7827672974878,-32.5999125019413,-32.4000277011298,-32.2674855869042,
-32.1394792934867,-31.9556172102756,-31.7410170567801,-31.6168883901235,
-31.496151573051,-31.3133009567084,-31.1134492691578,-30.9808892431195,
-30.8528944231952,-30.6690205303196,-30.4544528103358,-30.3302925542304,
-30.2095806433422,-30.0267093469457,-29.8267609886913,-29.6942403203475,
-29.5662088219705,-29.3823557187603,-29.1676920783934,-29.0436072853419,
-28.9228239434374,-28.7399966527432,-28.5402899448457,-28.4076592357397,
-28.3664636591338),.UNSPECIFIED.);
#29459=B_SPLINE_CURVE_WITH_KNOTS('',3,(#110788,#110789,#110790,#110791,
#110792,#110793,#110794,#110795,#110796,#110797,#110798,#110799,#110800,
#110801,#110802,#110803,#110804,#110805,#110806,#110807,#110808,#110809,
#110810,#110811,#110812,#110813,#110814,#110815,#110816,#110817,#110818,
#110819,#110820,#110821,#110822,#110823,#110824,#110825,#110826,#110827,
#110828,#110829,#110830,#110831,#110832,#110833,#110834,#110835,#110836,
#110837,#110838,#110839,#110840,#110841,#110842,#110843,#110844,#110845,
#110846,#110847,#110848,#110849,#110850,#110851,#110852,#110853,#110854,
#110855,#110856,#110857,#110858,#110859,#110860,#110861,#110862,#110863,
#110864,#110865,#110866,#110867,#110868,#110869,#110870,#110871,#110872,
#110873,#110874,#110875,#110876,#110877,#110878,#110879,#110880,#110881,
#110882,#110883,#110884,#110885,#110886,#110887,#110888,#110889,#110890,
#110891,#110892,#110893,#110894,#110895,#110896,#110897,#110898,#110899,
#110900,#110901,#110902,#110903,#110904,#110905,#110906,#110907,#110908,
#110909,#110910,#110911,#110912,#110913,#110914,#110915,#110916,#110917,
#110918,#110919),.UNSPECIFIED.,.F.,.F.,(4,2,2,2,2,2,2,2,2,2,2,2,2,2,2,2,
2,2,2,2,2,2,2,2,2,2,2,2,2,2,2,2,2,2,2,2,2,2,2,2,2,2,2,2,2,2,2,2,2,2,2,2,
2,2,2,2,2,2,2,2,2,2,2,2,2,4),(-16.3390445012698,-16.298426200689,-16.166778655205,
-15.9647852229255,-15.7814976184508,-15.6613692539658,-15.5365156611228,
-15.3227464875177,-15.1386478417236,-15.0109573811329,-14.8780085731732,
-14.6789982417746,-14.4962973493348,-14.3753117150272,-14.251438549892,
-14.0365067439024,-13.8527132572171,-13.7245807727206,-13.5921688649728,
-13.3919547030279,-13.2090279708675,-13.0883859304888,-12.9641379473126,
-12.7496618317777,-12.5657569020848,-12.4377952576735,-12.3051851627858,
-12.1054281309303,-11.9225913885721,-11.8018214480026,-11.6777201024695,
-11.4630737509824,-11.279215755038,-11.151190767859,-11.0186604052744,-10.8187302245468,
-10.6358625226298,-10.5151445065074,-10.390989291289,-10.1764129045308,
-9.99254066580108,-9.86454262459124,-9.73198442629992,-9.53212472352012,
-9.34927265927946,-9.22853718096996,-9.10440522551202,-8.88980633429332,
-8.70594334413277,-8.57793755307151,-8.44539279197424,-8.24551004092596,
-8.0626557027428,-7.94192941787983,-7.81779105664513,-7.60320521590703,
-7.41934243289807,-7.29134224194124,-7.15879502810392,-6.95892522880392,
-6.77607550773787,-6.65534815874714,-6.53121480227879,-6.31662833452605,
-6.13276923541242,-6.04591668252116),.UNSPECIFIED.);
#29460=B_SPLINE_CURVE_WITH_KNOTS('',3,(#110920,#110921,#110922,#110923,
#110924,#110925,#110926,#110927,#110928,#110929,#110930,#110931,#110932,
#110933,#110934,#110935,#110936,#110937,#110938,#110939,#110940,#110941,
#110942,#110943,#110944,#110945,#110946,#110947,#110948,#110949,#110950,
#110951,#110952,#110953,#110954,#110955,#110956,#110957,#110958,#110959,
#110960,#110961,#110962,#110963,#110964,#110965,#110966,#110967,#110968,
#110969,#110970,#110971,#110972,#110973,#110974,#110975,#110976,#110977,
#110978,#110979,#110980,#110981,#110982,#110983,#110984,#110985,#110986,
#110987,#110988,#110989,#110990,#110991,#110992,#110993,#110994,#110995,
#110996,#110997,#110998,#110999,#111000,#111001,#111002,#111003,#111004,
#111005,#111006,#111007,#111008,#111009,#111010,#111011,#111012,#111013,
#111014,#111015,#111016,#111017,#111018,#111019,#111020,#111021,#111022,
#111023,#111024,#111025,#111026,#111027,#111028,#111029,#111030,#111031,
#111032,#111033,#111034,#111035,#111036,#111037,#111038,#111039,#111040,
#111041,#111042,#111043),.UNSPECIFIED.,.F.,.F.,(4,2,2,2,2,2,2,2,2,2,2,2,
2,2,2,2,2,2,2,2,2,2,2,2,2,2,2,2,2,2,2,2,2,2,2,2,2,2,2,2,2,2,2,2,2,2,2,2,
2,2,2,2,2,2,2,2,2,2,2,2,2,4),(-28.3664636591338,-28.2797164067546,-28.0957991446076,
-27.8813728801688,-27.7570852714097,-27.6364798580693,-27.4535287823062,
-27.2531901316938,-27.1208344506832,-26.9926554760349,-26.8088936135346,
-26.5938354358871,-26.4700688114316,-26.3489853264082,-26.166349363524,
-25.9676936590255,-25.8345873150101,-25.7070245448486,-25.5228377739724,
-25.309390712311,-25.1842638792361,-25.0643606619124,-24.880914873015,-24.678168502708,
-24.5468424897756,-24.4177225832527,-24.2345671466329,-24.0167535315306,
-23.8951880884269,-23.7717293855261,-23.5905460589239,-23.3579655954052,
-23.2465264208019,-23.0825156762046,-22.865983031935,-22.6737097020076,
-22.5350681654638,-22.3527744370753,-22.1566459550718,-21.9799356327157,
-21.8558264126631,-21.5279549309628,-21.3734881578538,-21.2542705816141,
-21.1282476137618,-20.9158238967757,-20.7313360509443,-20.604194473977,
-20.4705375834989,-20.2581262018923,-20.0645349087967,-19.9518595706235,
-19.7964644208917,-19.6067510181749,-19.4027874754777,-19.2759433238808,
-18.9596269287533,-18.7693531702309,-18.6425637212898,-18.3115867582224,
-18.1333371708877,-18.0721778794789),.UNSPECIFIED.);
#29461=B_SPLINE_CURVE_WITH_KNOTS('',3,(#111049,#111050,#111051,#111052,
#111053,#111054,#111055,#111056,#111057,#111058,#111059,#111060,#111061,
#111062,#111063,#111064,#111065,#111066,#111067,#111068,#111069,#111070,
#111071,#111072,#111073,#111074,#111075,#111076,#111077,#111078,#111079,
#111080,#111081,#111082,#111083,#111084,#111085,#111086,#111087,#111088,
#111089,#111090,#111091,#111092,#111093,#111094,#111095,#111096,#111097,
#111098,#111099,#111100,#111101,#111102,#111103,#111104,#111105,#111106,
#111107,#111108,#111109,#111110,#111111,#111112,#111113,#111114,#111115,
#111116,#111117,#111118,#111119,#111120,#111121,#111122,#111123,#111124,
#111125,#111126,#111127,#111128,#111129,#111130,#111131,#111132,#111133,
#111134,#111135,#111136,#111137,#111138,#111139,#111140,#111141,#111142,
#111143,#111144,#111145,#111146,#111147,#111148,#111149,#111150),
 .UNSPECIFIED.,.F.,.F.,(4,2,2,2,2,2,2,2,2,2,2,2,2,2,2,2,2,2,2,2,2,2,2,2,
2,2,2,2,2,2,2,2,2,2,2,2,2,2,2,2,2,2,2,2,2,2,2,2,2,2,4),(-7.77890601744087,
-7.73775952422739,-7.60521657566241,-7.40533999301184,-7.22248980594114,
-7.10176541325388,-6.97763025612404,-6.76304803944614,-6.57918923266191,
-6.45119137673529,-6.31864723598035,-6.11878074870569,-5.93593463178674,
-5.81520998891301,-5.69107893079637,-5.47649717261703,-5.29264177366034,
-5.16464479115933,-5.03210382215314,-4.83223754253986,-4.64939360270815,
-4.52867152720027,-4.40454143327114,-4.18996389096452,-4.006110944537,-3.87811624601041,
-3.74557677001655,-3.54571450147723,-3.3628734668396,-3.2421528748727,-3.11802495086557,
-2.90345017912367,-2.71960005260632,-2.59160709546981,-2.45906975813039,
-2.25921003770872,-2.0763716281537,-1.95565293656456,-1.83152671866895,
-1.61695527334596,-1.43310782537051,-1.3051168182877,-1.1725813712171,-0.972724761576554,
-0.789889084794008,-0.66917213320999,-0.545047799792159,-0.338165976073822,
-0.171332043416279,-0.0714908710089851,-1.00000000013978E-6),
 .UNSPECIFIED.);
#29462=B_SPLINE_CURVE_WITH_KNOTS('',3,(#111153,#111154,#111155,#111156,
#111157,#111158,#111159,#111160,#111161,#111162,#111163,#111164,#111165,
#111166,#111167,#111168,#111169,#111170,#111171,#111172,#111173,#111174,
#111175,#111176,#111177,#111178,#111179,#111180,#111181,#111182,#111183,
#111184,#111185,#111186,#111187,#111188,#111189,#111190,#111191,#111192,
#111193,#111194,#111195,#111196,#111197,#111198,#111199,#111200,#111201,
#111202,#111203,#111204,#111205,#111206,#111207,#111208,#111209,#111210,
#111211,#111212,#111213,#111214,#111215,#111216,#111217,#111218,#111219,
#111220,#111221,#111222,#111223,#111224,#111225,#111226,#111227,#111228,
#111229,#111230,#111231,#111232,#111233,#111234,#111235,#111236,#111237,
#111238,#111239,#111240,#111241,#111242,#111243,#111244,#111245,#111246,
#111247,#111248,#111249,#111250,#111251,#111252,#111253,#111254,#111255,
#111256,#111257,#111258,#111259,#111260,#111261,#111262,#111263,#111264,
#111265,#111266,#111267,#111268,#111269,#111270),.UNSPECIFIED.,.F.,.F.,
(4,2,2,2,2,2,2,2,2,2,2,2,2,2,2,2,2,2,2,2,2,2,2,2,2,2,2,2,2,2,2,2,2,2,2,
2,2,2,2,2,2,2,2,2,2,2,2,2,2,2,2,2,2,2,2,2,2,2,4),(-36.0129143984966,-35.6654593228707,
-35.537072950901,-35.3588637813898,-35.1538708028347,-35.029741652255,-34.9090199548459,
-34.7261758635798,-34.5263105162429,-34.3937704731966,-34.265773995761,
-34.0819183254459,-33.8673382214782,-33.7432074632986,-33.6224837436366,
-33.4396370712807,-33.2397695140582,-33.1072271514087,-32.9792290502946,
-32.7953704415222,-32.5807878986877,-32.4566546503621,-32.335929701651,
-32.1530799152275,-31.9532073643807,-31.8206639106931,-31.6926631534603,
-31.508802305335,-31.2942145734511,-31.1700811293413,-31.0493528892366,
-30.8665013742659,-30.6666310672203,-30.5340833281315,-30.4060825988881,
-30.2222176936415,-30.0076319222705,-29.8834923174173,-29.7627661469876,
-29.5799093014275,-29.3800224249991,-29.2474787035248,-29.1194710245465,
-28.9356067872445,-28.7210043875804,-28.5968741296704,-28.4761360877002,
-28.2932832771621,-28.0934287605428,-27.9608674598407,-27.8328709750455,
-27.6489951172486,-27.4344244077396,-27.3102631807291,-27.1895494881339,
-27.0066763718689,-26.8067271367829,-26.6742043326556,-26.6330714141515),
 .UNSPECIFIED.);
#29463=B_SPLINE_CURVE_WITH_KNOTS('',3,(#111308,#111309,#111310,#111311,
#111312,#111313),.UNSPECIFIED.,.F.,.F.,(4,2,4),(-0.363774153394201,-0.193995614301166,
-9.9999999492173E-7),.UNSPECIFIED.);
#29464=B_SPLINE_CURVE_WITH_KNOTS('',3,(#111315,#111316,#111317,#111318,
#111319,#111320),.UNSPECIFIED.,.F.,.F.,(4,2,4),(-0.0532370215568508,-0.0266540826832716,
-6.04251272476367E-5),.UNSPECIFIED.);
#29465=B_SPLINE_CURVE_WITH_KNOTS('',3,(#111322,#111323,#111324,#111325,
#111326,#111327,#111328,#111329),.UNSPECIFIED.,.F.,.F.,(4,2,2,4),(-0.97744616972974,
-0.755136975405854,-0.488475539962772,-4.97420921147455E-6),
 .UNSPECIFIED.);
#29466=B_SPLINE_CURVE_WITH_KNOTS('',3,(#111331,#111332,#111333,#111334,
#111335,#111336),.UNSPECIFIED.,.F.,.F.,(4,2,4),(-1.85769505606768,-1.79339407393835,
-1.78591587085069),.UNSPECIFIED.);
#29467=B_SPLINE_CURVE_WITH_KNOTS('',3,(#111338,#111339,#111340,#111341),
 .UNSPECIFIED.,.F.,.F.,(4,4),(-4.93178416469503,-4.7947631910491),
 .UNSPECIFIED.);
#29468=B_SPLINE_CURVE_WITH_KNOTS('',3,(#111343,#111344,#111345,#111346,
#111347,#111348),.UNSPECIFIED.,.F.,.F.,(4,2,4),(-0.283103945271065,-0.141864378167519,
-2.13228232499812E-5),.UNSPECIFIED.);
#29469=B_SPLINE_CURVE_WITH_KNOTS('',3,(#111350,#111351,#111352,#111353,
#111354,#111355,#111356,#111357,#111358,#111359),.UNSPECIFIED.,.F.,.F.,
(4,2,2,2,4),(-0.201081696163703,-0.163457552386683,-0.100078064474262,-0.0500222454439804,
-9.99999075795843E-7),.UNSPECIFIED.);
#29470=B_SPLINE_CURVE_WITH_KNOTS('',3,(#111361,#111362,#111363,#111364),
 .UNSPECIFIED.,.F.,.F.,(4,4),(-0.298447768546908,-0.255015273222757),
 .UNSPECIFIED.);
#29471=B_SPLINE_CURVE_WITH_KNOTS('',3,(#111368,#111369,#111370,#111371,
#111372,#111373,#111374,#111375,#111376,#111377,#111378,#111379,#111380,
#111381,#111382,#111383,#111384,#111385,#111386),.UNSPECIFIED.,.F.,.F.,
(4,2,2,2,3,2,2,2,4),(-0.610180623927036,-0.587175612996075,-0.39145040866405,
-0.195725204332025,0.,0.195725204332025,0.39145040866405,0.587175612996075,
0.610180623930912),.UNSPECIFIED.);
#29472=B_SPLINE_CURVE_WITH_KNOTS('',3,(#111390,#111391,#111392,#111393),
 .UNSPECIFIED.,.F.,.F.,(4,4),(0.255015307744493,0.298443104215235),
 .UNSPECIFIED.);
#29473=B_SPLINE_CURVE_WITH_KNOTS('',3,(#111395,#111396,#111397,#111398,
#111399,#111400,#111401,#111402,#111403,#111404),.UNSPECIFIED.,.F.,.F.,
(4,2,2,2,4),(-0.199687815022838,-0.149974116571578,-0.100216949852256,-0.0373389572995741,
-7.28195441159246E-6),.UNSPECIFIED.);
#29474=B_SPLINE_CURVE_WITH_KNOTS('',3,(#111406,#111407,#111408,#111409,
#111410,#111411),.UNSPECIFIED.,.F.,.F.,(4,2,4),(-0.282640897342865,-0.141106701828136,
-7.28089112813694E-6),.UNSPECIFIED.);
#29475=B_SPLINE_CURVE_WITH_KNOTS('',3,(#111413,#111414,#111415,#111416),
 .UNSPECIFIED.,.F.,.F.,(4,4),(-0.15813773249332,-0.0210839373106531),
 .UNSPECIFIED.);
#29476=B_SPLINE_CURVE_WITH_KNOTS('',3,(#111418,#111419,#111420,#111421,
#111422,#111423,#111424),.UNSPECIFIED.,.F.,.F.,(4,3,4),(3.57860390370164,
3.58607926747234,3.65058765243316),.UNSPECIFIED.);
#29477=B_SPLINE_CURVE_WITH_KNOTS('',3,(#111426,#111427,#111428,#111429,
#111430,#111431,#111432,#111433),.UNSPECIFIED.,.F.,.F.,(4,2,2,4),(-0.854961148274419,
-0.437424717360482,-0.208632467898837,-1.3315846961078E-6),
 .UNSPECIFIED.);
#29478=B_SPLINE_CURVE_WITH_KNOTS('',3,(#111435,#111436,#111437,#111438,
#111439,#111440),.UNSPECIFIED.,.F.,.F.,(4,2,4),(-0.0532242538119046,-0.0266129661743925,
-9.99979108816385E-7),.UNSPECIFIED.);
#29479=B_SPLINE_CURVE_WITH_KNOTS('',3,(#111441,#111442,#111443,#111444,
#111445,#111446),.UNSPECIFIED.,.F.,.F.,(4,2,4),(-0.366235065052103,-0.18359159279208,
-6.68175113310375E-5),.UNSPECIFIED.);
#29480=B_SPLINE_CURVE_WITH_KNOTS('',3,(#111465,#111466,#111467,#111468,
#111469,#111470,#111471,#111472,#111473,#111474,#111475,#111476,#111477,
#111478,#111479,#111480),.UNSPECIFIED.,.F.,.F.,(4,3,3,3,3,4),(0.502459200378718,
0.620190407064421,0.733279471434336,0.843062918436606,0.948007554888288,
1.),.UNSPECIFIED.);
#29481=B_SPLINE_CURVE_WITH_KNOTS('',3,(#111482,#111483,#111484,#111485,
#111486,#111487,#111488,#111489,#111490,#111491),.UNSPECIFIED.,.F.,.F.,
(4,3,3,4),(0.,0.250000032895274,0.500000001353585,0.502459200168118),
 .UNSPECIFIED.);
#29482=B_SPLINE_CURVE_WITH_KNOTS('',3,(#111498,#111499,#111500,#111501,
#111502,#111503,#111504,#111505,#111506,#111507,#111508,#111509,#111510,
#111511,#111512,#111513,#111514,#111515,#111516,#111517,#111518,#111519,
#111520,#111521,#111522,#111523,#111524,#111525,#111526,#111527,#111528),
 .UNSPECIFIED.,.F.,.F.,(4,3,3,3,3,3,3,3,3,3,4),(2.2999675379427E-5,0.107908156121774,
0.216746941279355,0.325262700986818,0.432143196947118,0.5,0.625,0.740855777232924,
0.853585574556454,0.962004883925567,1.),.UNSPECIFIED.);
#29483=B_SPLINE_CURVE_WITH_KNOTS('',3,(#111530,#111531,#111532,#111533,
#111534,#111535,#111536,#111537,#111538,#111539,#111540,#111541,#111542,
#111543,#111544,#111545,#111546,#111547,#111548,#111549,#111550,#111551,
#111552,#111553,#111554,#111555,#111556,#111557,#111558,#111559,#111560,
#111561,#111562,#111563,#111564,#111565,#111566,#111567,#111568,#111569),
 .UNSPECIFIED.,.F.,.F.,(4,3,3,3,3,3,3,3,3,3,3,3,3,4),(0.,0.0652545873447945,
0.130565334251207,0.195328617575902,0.259486956805454,0.323171822834989,
0.386813145579456,0.450743489197714,0.5,0.596291449745224,0.697218586866101,
0.798920501895149,0.903698189064629,0.999999998228732),.UNSPECIFIED.);
#29484=B_SPLINE_CURVE_WITH_KNOTS('',3,(#111618,#111619,#111620,#111621,
#111622,#111623),.UNSPECIFIED.,.F.,.F.,(4,2,4),(0.498212563703856,0.749106281851928,
1.),.UNSPECIFIED.);
#29485=B_SPLINE_CURVE_WITH_KNOTS('',3,(#111625,#111626,#111627,#111628,
#111629,#111630,#111631,#111632,#111633,#111634,#111635,#111636,#111637,
#111638,#111639,#111640,#111641,#111642,#111643,#111644,#111645,#111646,
#111647,#111648,#111649),.UNSPECIFIED.,.F.,.F.,(4,3,3,3,3,3,3,3,4),(0.,
0.0689055252943441,0.137761127810044,0.206585336728476,0.249106281851928,
0.323525151579527,0.397954655315057,0.472431765057328,0.498212563703856),
 .UNSPECIFIED.);
#29486=B_SPLINE_CURVE_WITH_KNOTS('',3,(#111655,#111656,#111657,#111658,
#111659,#111660,#111661,#111662,#111663,#111664,#111665,#111666,#111667,
#111668,#111669,#111670,#111671,#111672,#111673,#111674,#111675,#111676,
#111677,#111678,#111679,#111680,#111681,#111682,#111683,#111684,#111685,
#111686,#111687,#111688,#111689,#111690,#111691,#111692,#111693,#111694,
#111695,#111696,#111697,#111698,#111699,#111700,#111701,#111702,#111703,
#111704,#111705,#111706,#111707,#111708,#111709,#111710,#111711,#111712,
#111713,#111714,#111715),.UNSPECIFIED.,.F.,.F.,(4,2,1,1,1,2,2,2,2,1,1,1,
2,2,2,2,2,1,1,1,2,2,2,2,2,2,2,2,2,2,2,1,1,2,2,4),(0.,0.0624999999999867,
0.09374999999998,0.109374999999977,0.117187499999975,0.121093749999974,
0.124999999999974,0.18749999999996,0.218749999999953,0.234374999999949,
0.242187499999947,0.246093749999946,0.248046874999946,0.249999999999946,
0.312499999999934,0.343749999999927,0.359374999999924,0.367187499999923,
0.371093749999922,0.373046874999922,0.374023437499922,0.374999999999922,
0.406249999999926,0.437499999999929,0.499999999999936,0.562499999999943,
0.593749999999947,0.609374999999949,0.62499999999995,0.687499999999957,
0.718749999999961,0.734374999999963,0.742187499999963,0.746093749999964,
0.749999999999964,1.),.UNSPECIFIED.);
#29487=B_SPLINE_CURVE_WITH_KNOTS('',3,(#111717,#111718,#111719,#111720,
#111721,#111722,#111723,#111724,#111725,#111726,#111727,#111728,#111729,
#111730,#111731,#111732,#111733,#111734,#111735,#111736,#111737,#111738,
#111739,#111740,#111741,#111742,#111743,#111744,#111745,#111746,#111747,
#111748,#111749,#111750,#111751,#111752,#111753,#111754,#111755,#111756,
#111757,#111758,#111759,#111760,#111761,#111762,#111763,#111764,#111765,
#111766,#111767,#111768,#111769,#111770,#111771,#111772,#111773,#111774,
#111775,#111776,#111777,#111778,#111779,#111780,#111781,#111782,#111783,
#111784,#111785,#111786,#111787,#111788,#111789,#111790,#111791,#111792,
#111793,#111794,#111795,#111796,#111797,#111798,#111799,#111800,#111801,
#111802,#111803,#111804,#111805,#111806,#111807,#111808,#111809,#111810,
#111811,#111812,#111813,#111814,#111815,#111816,#111817,#111818,#111819,
#111820,#111821,#111822,#111823,#111824,#111825,#111826,#111827,#111828,
#111829,#111830,#111831,#111832,#111833,#111834,#111835,#111836,#111837,
#111838,#111839,#111840,#111841,#111842,#111843,#111844,#111845,#111846,
#111847,#111848,#111849,#111850,#111851,#111852,#111853,#111854,#111855,
#111856,#111857,#111858,#111859,#111860,#111861,#111862,#111863,#111864,
#111865,#111866,#111867,#111868,#111869,#111870,#111871,#111872,#111873,
#111874,#111875,#111876,#111877,#111878,#111879,#111880,#111881,#111882,
#111883,#111884,#111885,#111886,#111887,#111888,#111889,#111890,#111891,
#111892,#111893,#111894,#111895,#111896,#111897),.UNSPECIFIED.,.F.,.F.,
(4,3,3,3,3,3,3,3,3,3,3,3,3,3,3,3,3,3,3,3,3,3,3,3,3,3,3,3,3,3,3,3,3,3,3,
3,3,3,3,3,3,3,3,3,3,3,3,3,3,3,3,3,3,3,3,3,3,3,3,3,4),(0.,0.0262353854799647,
0.0513882004402501,0.0760178707878943,0.100508935393731,0.124999999999569,
0.146668664871975,0.167619212130507,0.187499999999353,0.206963439919906,
0.218749999999244,0.23437499999919,0.242187499999164,0.246093749999151,
0.248046874999144,0.249023437499141,0.249755859374139,0.249999999999139,
0.27775990491465,0.304665955204806,0.331126738408159,0.356935472854795,
0.374999999999302,0.399714190734549,0.423855306551184,0.437499999999384,
0.460793596117878,0.468749999999425,0.484374999999445,0.492187499999455,
0.496093749999461,0.498046874999463,0.499023437499464,0.499999999999465,
0.536295573395747,0.572992063007457,0.610419270902384,0.624999999999589,
0.663936021974758,0.687499999999651,0.718749999999682,0.734374999999698,
0.742187499999706,0.746093749999709,0.749999999999712,0.778491977107122,
0.806509853673822,0.812499999999779,0.839780690346737,0.843749999999813,
0.85937499999983,0.867187499999838,0.871093749999843,0.874558700595564,
0.874999999999847,0.900177168816563,0.925224410427566,0.937499999999923,
0.962146915143125,0.986446671485073,1.),.UNSPECIFIED.);
#29488=B_SPLINE_CURVE_WITH_KNOTS('',3,(#111899,#111900,#111901,#111902,
#111903,#111904,#111905,#111906,#111907,#111908,#111909,#111910,#111911,
#111912,#111913,#111914,#111915,#111916,#111917,#111918,#111919,#111920,
#111921,#111922,#111923,#111924,#111925,#111926,#111927,#111928,#111929,
#111930,#111931,#111932,#111933,#111934,#111935,#111936,#111937,#111938,
#111939,#111940,#111941,#111942,#111943,#111944,#111945,#111946,#111947,
#111948,#111949,#111950,#111951,#111952,#111953,#111954,#111955,#111956,
#111957,#111958,#111959,#111960,#111961,#111962,#111963,#111964,#111965,
#111966,#111967,#111968,#111969,#111970,#111971,#111972,#111973,#111974,
#111975,#111976,#111977),.UNSPECIFIED.,.F.,.F.,(4,3,3,3,3,3,3,3,3,3,3,3,
3,3,3,3,3,3,3,3,3,3,3,3,3,3,4),(0.,0.052534295743839,0.106576781307671,
0.161234944024884,0.216296509746233,0.245421908055237,0.250000000000013,
0.305725650220763,0.362692703373066,0.37500000000002,0.431487410462525,
0.437500000000023,0.468750000000026,0.484375000000029,0.49218750000003,
0.49726975938631,0.500000000000032,0.562069345831075,0.622388694423505,
0.685333038873855,0.748277383324204,0.750000000000016,0.812500000000012,
0.872426273840813,0.932272985466431,0.991740773404511,1.),.UNSPECIFIED.);
#29489=B_SPLINE_CURVE_WITH_KNOTS('',3,(#111979,#111980,#111981,#111982,
#111983,#111984,#111985,#111986,#111987,#111988,#111989,#111990,#111991,
#111992,#111993,#111994,#111995,#111996,#111997,#111998,#111999,#112000,
#112001,#112002,#112003),.UNSPECIFIED.,.F.,.F.,(4,3,3,3,3,3,3,3,4),(7.26160252641012E-16,
0.131689505404652,0.260452970173316,0.385904363725134,0.5,0.645695716670177,
0.792716448908783,0.939175390751928,0.999999995177892),.UNSPECIFIED.);
#29490=B_SPLINE_CURVE_WITH_KNOTS('',3,(#112005,#112006,#112007,#112008,
#112009,#112010,#112011,#112012,#112013,#112014,#112015,#112016,#112017,
#112018,#112019,#112020,#112021,#112022,#112023,#112024,#112025,#112026,
#112027,#112028,#112029,#112030,#112031,#112032,#112033,#112034,#112035,
#112036,#112037,#112038,#112039,#112040,#112041,#112042,#112043,#112044,
#112045,#112046),.UNSPECIFIED.,.F.,.F.,(4,2,2,1,1,1,1,2,2,2,2,2,1,1,2,2,
2,2,2,1,1,1,1,2,2,4),(3.3708601358344E-9,0.125000000000098,0.187500000000147,
0.218750000000172,0.234375000000184,0.24218750000019,0.246093750000193,
0.249511718750197,0.250000000000197,0.375000000000224,0.437500000000236,
0.468750000000243,0.484375000000246,0.492187500000248,0.496093750000249,
0.50000000000025,0.625000000000263,0.68750000000027,0.718750000000273,0.734375000000275,
0.742187500000275,0.746093750000276,0.748046875000276,0.749511718750276,
0.750000000000276,1.),.UNSPECIFIED.);
#29491=B_SPLINE_CURVE_WITH_KNOTS('',3,(#112048,#112049,#112050,#112051,
#112052,#112053,#112054),.UNSPECIFIED.,.F.,.F.,(4,3,4),(4.999036296921E-14,
0.550250096230919,1.),.UNSPECIFIED.);
#29492=B_SPLINE_CURVE_WITH_KNOTS('',3,(#112056,#112057,#112058,#112059,
#112060,#112061,#112062,#112063,#112064,#112065,#112066,#112067,#112068,
#112069,#112070,#112071,#112072,#112073,#112074,#112075,#112076,#112077,
#112078,#112079,#112080,#112081,#112082,#112083,#112084,#112085,#112086,
#112087,#112088,#112089,#112090,#112091,#112092,#112093,#112094,#112095,
#112096,#112097,#112098,#112099,#112100,#112101,#112102,#112103,#112104,
#112105,#112106,#112107,#112108,#112109,#112110,#112111,#112112,#112113,
#112114,#112115,#112116,#112117,#112118,#112119,#112120,#112121,#112122,
#112123,#112124,#112125,#112126,#112127,#112128,#112129,#112130,#112131,
#112132,#112133,#112134,#112135,#112136,#112137,#112138,#112139,#112140,
#112141,#112142,#112143,#112144,#112145,#112146,#112147,#112148,#112149,
#112150,#112151,#112152,#112153,#112154,#112155,#112156,#112157,#112158,
#112159,#112160,#112161,#112162,#112163,#112164,#112165,#112166,#112167,
#112168,#112169,#112170,#112171,#112172,#112173,#112174,#112175,#112176,
#112177,#112178,#112179,#112180,#112181,#112182,#112183,#112184,#112185,
#112186,#112187,#112188,#112189,#112190,#112191,#112192,#112193,#112194,
#112195,#112196,#112197,#112198,#112199,#112200,#112201,#112202,#112203,
#112204,#112205,#112206,#112207,#112208,#112209,#112210,#112211,#112212,
#112213,#112214,#112215,#112216,#112217,#112218,#112219,#112220,#112221,
#112222,#112223,#112224,#112225,#112226,#112227,#112228,#112229,#112230,
#112231,#112232,#112233),.UNSPECIFIED.,.F.,.F.,(4,3,3,3,3,3,3,3,3,3,3,3,
3,3,3,3,3,3,3,3,3,3,3,3,3,3,3,3,3,3,3,3,3,3,3,3,3,3,3,3,3,3,3,3,3,3,3,3,
3,3,3,3,3,3,3,3,3,3,3,4),(0.,0.14352010892212,0.157701972276987,0.187500000000143,
0.218750000000166,0.234375000000178,0.242187500000183,0.246093750000185,
0.249659449839678,0.250000000000188,0.281779335707362,0.312823317660577,
0.317344564634756,0.349964665468181,0.381768385729566,0.392730548659543,
0.429582778946505,0.462987101572329,0.468750000000182,0.484375000000181,
0.49218750000018,0.49609375000018,0.498046875000181,0.499511718750183,0.500000000000183,
0.520007430934713,0.564789698817782,0.593750000000083,0.609375000000066,
0.617187500000057,0.624023437500051,0.62500000000005,0.663088784225902,
0.702110465150732,0.718750000000061,0.734375000000064,0.742187500000065,
0.746093750000066,0.749023437500067,0.750000000000069,0.771164208394432,
0.792032424081969,0.797583188711953,0.817998066584681,0.838686533292382,
0.859375000000083,0.867187500000084,0.871093750000085,0.873046875000085,
0.874023437500085,0.874511718750085,0.875000000000085,0.892460570687305,
0.909577023073872,0.926237545524542,0.937500000000042,0.953627291503346,
0.96958168681015,0.98530977827609,1.),.UNSPECIFIED.);
#29493=B_SPLINE_CURVE_WITH_KNOTS('',3,(#112235,#112236,#112237,#112238,
#112239,#112240,#112241,#112242,#112243,#112244,#112245,#112246,#112247,
#112248,#112249,#112250,#112251,#112252),.UNSPECIFIED.,.F.,.F.,(4,1,2,1,
2,2,2,1,1,1,1,4),(0.,0.125,0.25,0.3125,0.375,0.5,0.625,0.6875,0.75,0.8125,
0.874999999999999,1.),.UNSPECIFIED.);
#29494=B_SPLINE_CURVE_WITH_KNOTS('',3,(#112261,#112262,#112263,#112264,
#112265,#112266,#112267,#112268,#112269,#112270,#112271,#112272,#112273,
#112274,#112275,#112276,#112277,#112278,#112279,#112280,#112281,#112282,
#112283,#112284,#112285,#112286,#112287,#112288,#112289,#112290,#112291,
#112292,#112293,#112294,#112295,#112296,#112297,#112298,#112299,#112300,
#112301,#112302,#112303,#112304,#112305,#112306,#112307,#112308,#112309,
#112310,#112311,#112312,#112313,#112314,#112315,#112316,#112317,#112318,
#112319,#112320,#112321,#112322,#112323,#112324,#112325,#112326,#112327,
#112328,#112329,#112330,#112331,#112332,#112333,#112334,#112335,#112336,
#112337,#112338,#112339,#112340,#112341,#112342,#112343,#112344,#112345,
#112346,#112347,#112348,#112349,#112350,#112351,#112352,#112353,#112354,
#112355,#112356,#112357,#112358,#112359,#112360,#112361,#112362,#112363,
#112364,#112365,#112366,#112367,#112368,#112369),.UNSPECIFIED.,.F.,.F.,
(4,3,3,3,3,3,3,3,3,3,3,3,3,3,3,3,3,3,3,3,3,3,3,3,3,3,3,3,3,3,3,3,3,3,3,
3,4),(0.,0.0221285907803649,0.0457146490130174,0.0624999316519651,0.0936982528543991,
0.124999863304009,0.156249829130032,0.183271416696792,0.187499794956055,
0.220371047068795,0.249999726608099,0.281249692434121,0.310392278499468,
0.338981017787981,0.3669802812056,0.374999589912188,0.410712814329141,0.445935995865815,
0.480427395075885,0.499999453216277,0.532474023028728,0.564651000993001,
0.596435510326097,0.624999316520367,0.659415128053142,0.693382150709312,
0.726649798606273,0.749999179824455,0.778823340006754,0.807383283604156,
0.835813998348854,0.864094537414675,0.874999043128545,0.910273598518763,
0.945062381131166,0.979104413886319,1.),.UNSPECIFIED.);
#29495=B_SPLINE_CURVE_WITH_KNOTS('',3,(#112371,#112372,#112373,#112374,
#112375,#112376,#112377,#112378,#112379,#112380,#112381,#112382,#112383,
#112384,#112385,#112386,#112387,#112388,#112389,#112390,#112391,#112392,
#112393,#112394,#112395,#112396,#112397,#112398,#112399,#112400,#112401,
#112402,#112403,#112404,#112405,#112406,#112407,#112408,#112409,#112410,
#112411,#112412,#112413,#112414,#112415,#112416,#112417,#112418,#112419,
#112420,#112421,#112422,#112423,#112424,#112425,#112426,#112427,#112428,
#112429,#112430,#112431,#112432,#112433,#112434,#112435,#112436,#112437,
#112438,#112439,#112440,#112441,#112442,#112443,#112444,#112445,#112446,
#112447,#112448,#112449,#112450),.UNSPECIFIED.,.F.,.F.,(4,2,2,1,2,2,1,2,
2,1,1,2,2,1,2,2,2,1,2,2,1,1,1,2,2,2,2,1,2,2,2,2,2,1,1,2,2,2,2,2,2,1,2,2,
1,2,4),(0.,0.1249999999995,0.249999999999001,0.281249999998876,0.285156249998862,
0.289062499998847,0.296874999998818,0.31249999999876,0.374999999998527,
0.406249999998409,0.421874999998351,0.427734374998332,0.428710937498328,
0.429687499998324,0.437499999998293,0.499999999998021,0.562499999997748,
0.570312499997713,0.571289062497709,0.571777343747708,0.572265624997707,
0.574218749997718,0.578124999997741,0.593749999997826,0.624999999998001,
0.687499999998352,0.718749999998528,0.734374999998614,0.742187499998659,
0.746093749998681,0.749999999998703,0.812499999999069,0.843749999999253,
0.859374999999346,0.867187499999392,0.871093749999416,0.873046874999426,
0.874999999999437,0.906249999999573,0.921874999999641,0.929687499999675,
0.933593749999692,0.935546874999701,0.936523437499705,0.937499999999709,
0.968749999999855,1.),.UNSPECIFIED.);
#29496=B_SPLINE_CURVE_WITH_KNOTS('',3,(#112452,#112453,#112454,#112455,
#112456,#112457,#112458),.UNSPECIFIED.,.F.,.F.,(4,3,4),(0.,0.552168243797124,
0.99999996236639),.UNSPECIFIED.);
#29497=B_SPLINE_CURVE_WITH_KNOTS('',3,(#112460,#112461,#112462,#112463,
#112464,#112465,#112466,#112467,#112468,#112469,#112470,#112471,#112472,
#112473,#112474,#112475,#112476,#112477,#112478,#112479,#112480,#112481,
#112482,#112483,#112484,#112485,#112486,#112487,#112488,#112489,#112490,
#112491,#112492,#112493,#112494,#112495,#112496,#112497,#112498,#112499,
#112500,#112501,#112502,#112503,#112504,#112505,#112506,#112507,#112508,
#112509,#112510,#112511,#112512,#112513,#112514,#112515,#112516,#112517,
#112518,#112519,#112520,#112521,#112522,#112523,#112524,#112525,#112526,
#112527,#112528,#112529,#112530,#112531,#112532,#112533,#112534,#112535,
#112536,#112537,#112538,#112539,#112540,#112541,#112542,#112543,#112544,
#112545,#112546,#112547,#112548,#112549,#112550,#112551,#112552,#112553,
#112554,#112555,#112556,#112557,#112558,#112559,#112560,#112561,#112562,
#112563,#112564,#112565,#112566,#112567,#112568,#112569,#112570,#112571,
#112572,#112573,#112574,#112575,#112576,#112577,#112578,#112579,#112580,
#112581,#112582,#112583,#112584,#112585,#112586,#112587,#112588,#112589,
#112590,#112591,#112592,#112593,#112594,#112595,#112596,#112597,#112598,
#112599,#112600,#112601,#112602,#112603,#112604,#112605,#112606,#112607,
#112608,#112609,#112610,#112611,#112612,#112613,#112614,#112615,#112616,
#112617,#112618,#112619,#112620,#112621,#112622,#112623,#112624,#112625,
#112626,#112627,#112628,#112629,#112630,#112631,#112632,#112633,#112634,
#112635,#112636,#112637,#112638,#112639,#112640,#112641,#112642,#112643,
#112644,#112645,#112646,#112647,#112648,#112649,#112650,#112651,#112652,
#112653,#112654,#112655,#112656,#112657,#112658,#112659,#112660,#112661,
#112662,#112663,#112664,#112665,#112666,#112667,#112668,#112669,#112670,
#112671,#112672,#112673),.UNSPECIFIED.,.F.,.F.,(4,3,3,3,3,3,3,3,3,3,3,3,
3,3,3,3,3,3,3,3,3,3,3,3,3,3,3,3,3,3,3,3,3,3,3,3,3,3,3,3,3,3,3,3,3,3,3,3,
3,3,3,3,3,3,3,3,3,3,3,3,3,3,3,3,3,3,3,3,3,3,3,4),(1.72563345367939E-9,0.0251902887445909,
0.0431288153335098,0.0624999999999211,0.0895200409842773,0.0937499999998817,
0.109374999999862,0.117187499999852,0.121093749999847,0.123046874999844,
0.124999999999842,0.144918719463055,0.165108115533264,0.176831133963176,
0.197350519867584,0.218134806338091,0.234374999999699,0.242187499999689,
0.246093749999683,0.248046874999681,0.249755859374679,0.249877929687179,
0.249999999999679,0.273529672022163,0.297668999478059,0.317227671725171,
0.342520462487478,0.368140297657527,0.394182158920048,0.420410072964651,
0.446860880515511,0.468749999999632,0.484374999999629,0.492187499999627,
0.496093749999626,0.498046874999626,0.499511718749626,0.499755859374627,
0.499999999999627,0.53315145702459,0.566804203446233,0.601247768565495,
0.630326335104507,0.664700120223858,0.699891114094579,0.718749999999988,
0.734375000000014,0.742187500000027,0.746093750000033,0.748046875000036,
0.749511718750039,0.75000000000004,0.763329402270841,0.776642772728383,
0.789909749239645,0.803137903948878,0.816279431179592,0.825842999740232,
0.838787243962379,0.85158256388443,0.859375000000014,0.867187500000012,
0.871093750000011,0.87304687500001,0.87402343750001,0.87451171875001,0.87500000000001,
0.902182619157957,0.929229736943535,0.94702964207556,0.974458771224453,
0.999999996801779),.UNSPECIFIED.);
#29498=B_SPLINE_CURVE_WITH_KNOTS('',3,(#112675,#112676,#112677,#112678,
#112679,#112680,#112681,#112682,#112683,#112684,#112685,#112686,#112687,
#112688,#112689,#112690,#112691,#112692,#112693,#112694,#112695,#112696,
#112697,#112698,#112699,#112700,#112701,#112702),.UNSPECIFIED.,.F.,.F.,
(4,3,3,3,3,3,3,3,3,4),(4.84983446249765E-9,0.132630715103507,0.268748748725146,
0.409090067082655,0.5,0.612453315498843,0.727402227633262,0.843933478268945,
0.963413781542886,1.),.UNSPECIFIED.);
#29499=B_SPLINE_CURVE_WITH_KNOTS('',3,(#112704,#112705,#112706,#112707,
#112708,#112709,#112710,#112711,#112712,#112713,#112714,#112715,#112716,
#112717,#112718,#112719,#112720,#112721,#112722,#112723,#112724,#112725),
 .UNSPECIFIED.,.F.,.F.,(4,2,2,2,2,2,2,2,2,2,4),(0.,0.125000000000008,0.187500000000011,
0.218750000000013,0.250000000000016,0.375000000000019,0.437500000000019,
0.468750000000018,0.500000000000016,0.750000000000008,1.),.UNSPECIFIED.);
#29500=B_SPLINE_CURVE_WITH_KNOTS('',3,(#112727,#112728,#112729,#112730,
#112731,#112732,#112733,#112734,#112735,#112736,#112737,#112738,#112739,
#112740,#112741,#112742,#112743,#112744,#112745,#112746,#112747,#112748,
#112749,#112750,#112751,#112752,#112753,#112754,#112755,#112756,#112757,
#112758,#112759,#112760,#112761,#112762,#112763,#112764,#112765,#112766,
#112767,#112768,#112769,#112770,#112771,#112772,#112773,#112774,#112775,
#112776,#112777,#112778,#112779,#112780,#112781,#112782,#112783,#112784,
#112785,#112786,#112787,#112788,#112789,#112790,#112791,#112792,#112793,
#112794,#112795,#112796,#112797,#112798,#112799,#112800,#112801,#112802,
#112803,#112804,#112805,#112806,#112807,#112808,#112809,#112810,#112811,
#112812,#112813,#112814,#112815,#112816,#112817,#112818,#112819,#112820,
#112821,#112822,#112823,#112824,#112825,#112826,#112827,#112828,#112829,
#112830,#112831,#112832,#112833,#112834,#112835,#112836,#112837,#112838,
#112839,#112840,#112841,#112842,#112843,#112844,#112845,#112846,#112847,
#112848,#112849,#112850,#112851,#112852,#112853),.UNSPECIFIED.,.F.,.F.,
(4,3,3,3,3,3,3,3,3,3,3,3,3,3,3,3,3,3,3,3,3,3,3,3,3,3,3,3,3,3,3,3,3,3,3,
3,3,3,3,3,3,3,4),(0.,0.021047851700448,0.0420641562918161,0.0625000000000671,
0.0834215117481714,0.104231039484499,0.109375000000118,0.117187500000127,
0.121093750000131,0.124211568697334,0.125000000000136,0.143426311945488,
0.170178097660854,0.197400256138289,0.218750000000252,0.234375000000271,
0.24218750000028,0.246093750000284,0.248046875000286,0.250000000000288,
0.275019250919516,0.296988168551031,0.322708916352598,0.34790789542466,
0.372156990324995,0.395828889732673,0.418651543771118,0.430683726473005,
0.456873584251504,0.468750000000375,0.484375000000381,0.492187500000384,
0.496093750000386,0.498046875000388,0.499023437500388,0.500000000000389,
0.536638842599964,0.630613966148358,0.652479703862573,0.75633333254645,
0.768320183847596,0.877828717397992,1.),.UNSPECIFIED.);
#29501=B_SPLINE_CURVE_WITH_KNOTS('',3,(#112854,#112855,#112856,#112857,
#112858,#112859,#112860,#112861,#112862,#112863,#112864,#112865,#112866,
#112867,#112868,#112869,#112870,#112871,#112872,#112873,#112874,#112875,
#112876,#112877,#112878,#112879,#112880,#112881,#112882,#112883,#112884,
#112885,#112886,#112887,#112888,#112889,#112890,#112891,#112892,#112893,
#112894,#112895,#112896,#112897,#112898,#112899,#112900,#112901,#112902,
#112903,#112904,#112905,#112906,#112907,#112908,#112909,#112910,#112911,
#112912,#112913,#112914,#112915,#112916,#112917,#112918,#112919,#112920,
#112921,#112922,#112923,#112924,#112925,#112926,#112927,#112928,#112929,
#112930,#112931,#112932),.UNSPECIFIED.,.F.,.F.,(4,2,2,2,1,1,1,1,2,2,2,2,
1,1,1,1,2,2,2,2,1,1,1,1,2,2,2,2,2,1,1,1,1,2,2,2,2,1,1,1,1,2,2,2,2,1,1,1,
2,2,4),(0.,0.124999999999979,0.187499999999968,0.218749999999963,0.23437499999996,
0.242187499999958,0.246093749999958,0.248046874999957,0.249023437499957,
0.249999999999957,0.312499999999942,0.343749999999934,0.35937499999993,
0.367187499999928,0.371093749999927,0.373046874999927,0.374023437499926,
0.374999999999926,0.437499999999906,0.468749999999896,0.484374999999891,
0.492187499999889,0.496093749999888,0.498046874999887,0.499755859374888,
0.499999999999888,0.562499999999828,0.593749999999799,0.609374999999784,
0.617187499999776,0.621093749999773,0.623046874999771,0.62402343749977,
0.62475585937477,0.62499999999977,0.687499999999799,0.718749999999813,0.73437499999982,
0.742187499999824,0.746093749999826,0.748046874999826,0.749511718749826,
0.749999999999826,0.812499999999865,0.843749999999885,0.859374999999894,
0.867187499999899,0.871093749999902,0.873046874999903,0.874999999999905,
1.),.UNSPECIFIED.);
#29502=B_SPLINE_CURVE_WITH_KNOTS('',3,(#112942,#112943,#112944,#112945,
#112946,#112947,#112948,#112949,#112950,#112951,#112952,#112953,#112954,
#112955,#112956,#112957,#112958,#112959,#112960,#112961,#112962,#112963,
#112964,#112965,#112966,#112967,#112968,#112969,#112970,#112971,#112972,
#112973,#112974,#112975,#112976,#112977,#112978,#112979,#112980,#112981,
#112982,#112983,#112984,#112985,#112986,#112987,#112988,#112989,#112990,
#112991,#112992,#112993,#112994,#112995,#112996,#112997,#112998,#112999),
 .UNSPECIFIED.,.F.,.F.,(4,3,3,3,3,3,3,3,3,3,3,3,3,3,3,3,3,3,3,4),(0.,0.0832713098445368,
0.165797375546863,0.187499999999976,0.218749999999971,0.23437499999997,
0.247637083347011,0.249999999999968,0.367385209176164,0.374999999999965,
0.437499999999964,0.468749999999964,0.484374999999965,0.499182128881398,
0.499999999999967,0.618394583046436,0.734930438524368,0.850408746057064,
0.964416460208876,0.999999999999995),.UNSPECIFIED.);
#29503=B_SPLINE_CURVE_WITH_KNOTS('',3,(#113001,#113002,#113003,#113004,
#113005,#113006,#113007,#113008,#113009,#113010,#113011,#113012,#113013,
#113014,#113015,#113016,#113017,#113018,#113019,#113020,#113021,#113022,
#113023,#113024,#113025,#113026,#113027,#113028,#113029,#113030,#113031,
#113032,#113033,#113034,#113035,#113036,#113037,#113038,#113039,#113040,
#113041,#113042,#113043,#113044,#113045,#113046,#113047,#113048,#113049,
#113050,#113051,#113052,#113053,#113054,#113055,#113056,#113057,#113058,
#113059,#113060,#113061,#113062,#113063,#113064,#113065,#113066,#113067,
#113068,#113069,#113070,#113071,#113072,#113073,#113074,#113075,#113076,
#113077,#113078,#113079,#113080,#113081,#113082,#113083,#113084,#113085,
#113086,#113087,#113088,#113089,#113090,#113091,#113092,#113093,#113094,
#113095,#113096,#113097,#113098,#113099,#113100),.UNSPECIFIED.,.F.,.F.,
(4,3,3,3,3,3,3,3,3,3,3,3,3,3,3,3,3,3,3,3,3,3,3,3,3,3,3,3,3,3,3,3,3,4),(0.,
0.00157583922411374,0.0826938458291058,0.124999999999998,0.12541626163461,
0.169971053142697,0.214255800133528,0.249510415781629,0.249999999999996,
0.306480976121043,0.363470399754044,0.374207181925756,0.374999999999994,
0.437499999999993,0.468749999999993,0.484374999999994,0.492187499999995,
0.498780286635775,0.499999999999996,0.500783062716376,0.57069940241407,
0.624281140924415,0.624999999999999,0.674699886918992,0.6875,0.71875,0.73649200577412,
0.748843590324373,0.750000000000001,0.801976158225286,0.854862646973396,
0.907963524134435,0.960913180138766,1.),.UNSPECIFIED.);
#29504=B_SPLINE_CURVE_WITH_KNOTS('',3,(#113102,#113103,#113104,#113105,
#113106,#113107,#113108,#113109,#113110,#113111,#113112,#113113,#113114,
#113115,#113116,#113117,#113118,#113119,#113120,#113121,#113122,#113123,
#113124,#113125,#113126),.UNSPECIFIED.,.F.,.F.,(4,3,3,3,3,3,3,3,4),(0.,
0.195180208056074,0.250000000000001,0.375,0.4375,0.5,0.682692739872639,
0.866396142559968,1.),.UNSPECIFIED.);
#29505=B_SPLINE_CURVE_WITH_KNOTS('',3,(#113130,#113131,#113132,#113133,
#113134,#113135,#113136,#113137,#113138,#113139,#113140,#113141,#113142,
#113143,#113144,#113145,#113146,#113147,#113148,#113149,#113150,#113151),
 .UNSPECIFIED.,.F.,.F.,(4,3,3,3,3,3,3,4),(0.,0.180290242506945,0.25,0.43116946893496,
0.5,0.702896747154662,0.903673086907349,1.),.UNSPECIFIED.);
#29506=B_SPLINE_CURVE_WITH_KNOTS('',3,(#113153,#113154,#113155,#113156,
#113157,#113158,#113159,#113160,#113161,#113162,#113163,#113164,#113165,
#113166,#113167,#113168,#113169,#113170,#113171,#113172,#113173,#113174,
#113175,#113176,#113177,#113178,#113179,#113180,#113181,#113182,#113183,
#113184,#113185,#113186,#113187,#113188,#113189,#113190,#113191,#113192,
#113193,#113194,#113195,#113196,#113197,#113198,#113199,#113200,#113201,
#113202,#113203,#113204,#113205,#113206,#113207,#113208,#113209,#113210),
 .UNSPECIFIED.,.F.,.F.,(4,3,3,3,3,3,3,3,3,3,3,3,3,3,3,3,3,3,3,4),(0.,0.0832713098165828,
0.165797375467783,0.187500000000001,0.218750000000002,0.234375000000003,
0.247637083317996,0.250000000000004,0.367385208916902,0.375000000000004,
0.437500000000006,0.468750000000006,0.484375000000006,0.499182128806393,
0.500000000000005,0.61839458300907,0.734930438447227,0.850408745939979,
0.964416460051457,0.999999999999995),.UNSPECIFIED.);
#29507=B_SPLINE_CURVE_WITH_KNOTS('',3,(#113212,#113213,#113214,#113215,
#113216,#113217,#113218,#113219,#113220,#113221,#113222,#113223,#113224,
#113225,#113226,#113227,#113228,#113229,#113230,#113231,#113232,#113233,
#113234,#113235,#113236,#113237,#113238,#113239,#113240,#113241,#113242,
#113243,#113244,#113245,#113246,#113247,#113248,#113249,#113250,#113251,
#113252,#113253,#113254,#113255,#113256,#113257,#113258,#113259,#113260,
#113261,#113262,#113263,#113264,#113265,#113266,#113267,#113268,#113269,
#113270,#113271,#113272,#113273,#113274,#113275,#113276,#113277,#113278,
#113279,#113280,#113281,#113282,#113283,#113284,#113285,#113286,#113287,
#113288,#113289,#113290,#113291,#113292,#113293,#113294,#113295,#113296,
#113297,#113298,#113299,#113300,#113301,#113302,#113303,#113304,#113305,
#113306,#113307,#113308,#113309,#113310,#113311),.UNSPECIFIED.,.F.,.F.,
(4,3,3,3,3,3,3,3,3,3,3,3,3,3,3,3,3,3,3,3,3,3,3,3,3,3,3,3,3,3,3,3,3,4),(0.,
0.00157583922263862,0.0826938457606489,0.124999999999983,0.125416261644559,
0.169971053528897,0.214255800893783,0.249510415781452,0.249999999999966,
0.30648097610305,0.363470399718357,0.374207181925786,0.37499999999995,0.437499999999941,
0.468749999999939,0.484374999999937,0.492187499999937,0.498780286636739,
0.499999999999938,0.500783062713993,0.570699402452992,0.624281140920161,
0.624999999999953,0.674699886914206,0.687499999999959,0.718749999999964,
0.736492005804936,0.748843590315732,0.749999999999968,0.80197615821585,
0.854862646954884,0.907963524106764,0.960913180101409,1.),.UNSPECIFIED.);
#29508=B_SPLINE_CURVE_WITH_KNOTS('',3,(#113313,#113314,#113315,#113316,
#113317,#113318,#113319,#113320,#113321,#113322,#113323),.UNSPECIFIED.,
 .F.,.F.,(4,2,1,2,2,4),(0.,0.250000000000001,0.375000000000002,0.437500000000001,
0.500000000000001,1.),.UNSPECIFIED.);
#29509=B_SPLINE_CURVE_WITH_KNOTS('',3,(#113326,#113327,#113328,#113329,
#113330,#113331,#113332,#113333,#113334,#113335,#113336,#113337,#113338,
#113339,#113340,#113341,#113342,#113343,#113344,#113345,#113346,#113347),
 .UNSPECIFIED.,.F.,.F.,(4,3,3,3,3,3,3,4),(0.,0.187500000000001,0.375000000000002,
0.465350260778303,0.500000000000003,0.702064785007046,0.902038946571831,
1.),.UNSPECIFIED.);
#29510=B_SPLINE_CURVE_WITH_KNOTS('',3,(#113364,#113365,#113366,#113367,
#113368,#113369),.UNSPECIFIED.,.F.,.F.,(4,2,4),(0.659245462660571,0.848526904814134,
0.950302518199856),.UNSPECIFIED.);
#29511=B_SPLINE_CURVE_WITH_KNOTS('',3,(#113372,#113373,#113374,#113375,
#113376,#113377),.UNSPECIFIED.,.F.,.F.,(4,2,4),(0.368188407121287,0.469964020507009,
0.659245462660571),.UNSPECIFIED.);
#29512=B_SPLINE_CURVE_WITH_KNOTS('',3,(#113398,#113399,#113400,#113401,
#113402,#113403,#113404,#113405,#113406,#113407),.UNSPECIFIED.,.F.,.F.,
(4,2,2,2,4),(-0.989948967812353,-0.817116807788299,-0.638223028190753,-0.459329248593207,
-0.286497088569423),.UNSPECIFIED.);
#29513=B_SPLINE_CURVE_WITH_KNOTS('',3,(#113414,#113415,#113416,#113417,
#113418,#113419,#113420,#113421,#113422,#113423,#113424,#113425,#113426,
#113427),.UNSPECIFIED.,.F.,.F.,(4,2,2,2,2,2,4),(9.999995437339E-7,0.259748030405366,
0.508379521897915,0.568189856021016,0.593019351884581,0.603881938758307,
0.614169443343448),.UNSPECIFIED.);
#29514=B_SPLINE_CURVE_WITH_KNOTS('',3,(#113435,#113436,#113437,#113438,
#113439,#113440,#113441,#113442,#113443,#113444,#113445,#113446,#113447,
#113448),.UNSPECIFIED.,.F.,.F.,(4,2,2,2,2,2,4),(1.00000361513827E-6,0.00712177767761689,
0.0148839153232921,0.032515583953615,0.0900479458768181,0.184553013873431,
0.25295173128519),.UNSPECIFIED.);
#29515=B_SPLINE_CURVE_WITH_KNOTS('',3,(#113544,#113545,#113546,#113547,
#113548,#113549,#113550,#113551,#113552,#113553,#113554,#113555,#113556,
#113557,#113558,#113559,#113560,#113561,#113562,#113563,#113564,#113565,
#113566,#113567,#113568,#113569,#113570,#113571,#113572,#113573,#113574,
#113575,#113576,#113577,#113578,#113579,#113580,#113581,#113582,#113583,
#113584,#113585,#113586,#113587,#113588,#113589,#113590,#113591,#113592,
#113593,#113594,#113595,#113596,#113597,#113598),.UNSPECIFIED.,.F.,.F.,
(4,3,3,3,3,3,3,3,3,3,3,3,3,3,3,3,3,3,4),(0.,0.0969544955629047,0.192024794958463,
0.229538341359698,0.249999999999967,0.35554605419242,0.374999999999951,
0.437499999999944,0.46874999999994,0.484374999999939,0.494786925416321,
0.499999999999939,0.53995794249682,0.622741542029251,0.703614813184483,
0.781706215824503,0.84330713965756,0.92367183712412,0.999998921631664),
 .UNSPECIFIED.);
#29516=B_SPLINE_CURVE_WITH_KNOTS('',3,(#113601,#113602,#113603,#113604,
#113605,#113606,#113607,#113608,#113609,#113610,#113611,#113612,#113613,
#113614,#113615,#113616,#113617,#113618,#113619,#113620,#113621,#113622,
#113623,#113624,#113625,#113626,#113627,#113628,#113629,#113630,#113631,
#113632,#113633,#113634,#113635,#113636,#113637,#113638,#113639,#113640,
#113641,#113642,#113643,#113644,#113645,#113646,#113647,#113648,#113649,
#113650,#113651,#113652,#113653,#113654,#113655,#113656,#113657,#113658),
 .UNSPECIFIED.,.F.,.F.,(4,3,3,3,3,3,3,3,3,3,3,3,3,3,3,3,3,3,3,4),(1.22754616606188E-6,
0.077127828978588,0.155720459280002,0.164018043179436,0.238669858928981,
0.25000000000002,0.33192992133946,0.375000000000029,0.437500000000033,0.466959333266612,
0.468750000000036,0.484375000000037,0.494691856545788,0.500000000000039,
0.603437310447197,0.709278989321924,0.777007528128708,0.876123815416302,
0.97719726753376,1.),.UNSPECIFIED.);
#29517=B_SPLINE_CURVE_WITH_KNOTS('',3,(#113669,#113670,#113671,#113672,
#113673,#113674,#113675,#113676,#113677,#113678,#113679,#113680,#113681,
#113682,#113683,#113684,#113685,#113686,#113687,#113688,#113689,#113690,
#113691,#113692,#113693,#113694,#113695,#113696,#113697,#113698,#113699,
#113700,#113701,#113702,#113703,#113704,#113705,#113706,#113707,#113708,
#113709,#113710,#113711,#113712,#113713,#113714,#113715,#113716,#113717,
#113718,#113719,#113720,#113721,#113722,#113723,#113724,#113725,#113726,
#113727,#113728,#113729,#113730,#113731,#113732,#113733,#113734,#113735,
#113736,#113737,#113738,#113739,#113740,#113741,#113742,#113743,#113744,
#113745,#113746,#113747,#113748,#113749,#113750,#113751,#113752,#113753,
#113754,#113755,#113756,#113757,#113758,#113759,#113760,#113761,#113762,
#113763,#113764,#113765,#113766,#113767,#113768,#113769,#113770,#113771,
#113772,#113773,#113774,#113775,#113776,#113777,#113778,#113779,#113780,
#113781,#113782,#113783,#113784,#113785,#113786,#113787,#113788,#113789,
#113790,#113791,#113792,#113793,#113794),.UNSPECIFIED.,.F.,.F.,(4,2,2,2,
2,2,2,2,2,2,2,2,2,2,2,2,2,2,2,2,2,2,2,2,2,2,2,2,2,2,2,2,2,2,2,2,2,2,2,2,
2,2,2,2,2,2,2,2,2,2,2,2,2,2,2,2,2,2,2,2,2,2,4),(-26.6330714141515,-26.5461718850615,
-26.3623163068096,-26.1476515893506,-26.0235641990265,-25.9027805180327,
-25.7199504119376,-25.52023768622,-25.3876070905798,-25.2596614153778,-25.075742962878,
-24.8613106090056,-24.7370245950165,-24.6164151116154,-24.4334637395033,
-24.2331320927081,-24.1007708017898,-23.9725938499412,-23.7888275193191,
-23.5737764190362,-23.4500004740476,-23.328922994976,-23.146280056007,-22.9475953530379,
-22.8144994884482,-22.6869256936087,-22.5027434433308,-22.2892700348955,
-22.1641622465145,-22.0442410956717,-21.8608049283298,-21.6581114786105,
-21.5267605884321,-21.3976615518945,-21.2144897688346,-20.9967439736818,
-20.8751222092299,-20.7517296234012,-20.5705052234198,-20.3382869277355,
-20.2266059298047,-20.0233423698298,-19.8491553360417,-19.6541417125856,
-19.5151391277833,-19.3112475069076,-18.9971860038498,-18.8697053091383,
-18.6654013868218,-18.4761495657214,-18.3202149817156,-18.1926036175017,
-18.0055480775392,-17.7772911355014,-17.5965622030943,-17.4820501552149,
-17.254067231833,-17.0723774292265,-16.9497776930168,-16.8274806751369,
-16.6105938804691,-16.42724496372,-16.3390445012698),.UNSPECIFIED.);
#29518=B_SPLINE_CURVE_WITH_KNOTS('',3,(#113795,#113796,#113797,#113798,
#113799,#113800,#113801,#113802,#113803,#113804,#113805,#113806,#113807,
#113808,#113809,#113810,#113811,#113812,#113813,#113814,#113815,#113816,
#113817,#113818,#113819,#113820,#113821,#113822,#113823,#113824,#113825,
#113826,#113827,#113828,#113829,#113830,#113831,#113832,#113833,#113834,
#113835,#113836,#113837,#113838,#113839,#113840,#113841,#113842,#113843,
#113844,#113845,#113846,#113847,#113848,#113849,#113850,#113851,#113852,
#113853,#113854,#113855,#113856,#113857,#113858,#113859,#113860,#113861,
#113862,#113863,#113864,#113865,#113866,#113867,#113868,#113869,#113870,
#113871,#113872,#113873,#113874,#113875,#113876,#113877,#113878,#113879,
#113880,#113881,#113882,#113883,#113884,#113885,#113886,#113887,#113888,
#113889,#113890,#113891,#113892,#113893,#113894,#113895,#113896,#113897,
#113898,#113899,#113900,#113901,#113902,#113903,#113904,#113905,#113906,
#113907,#113908,#113909,#113910,#113911,#113912,#113913,#113914,#113915,
#113916,#113917,#113918,#113919,#113920,#113921,#113922,#113923,#113924),
 .UNSPECIFIED.,.F.,.F.,(4,2,2,2,2,2,2,2,2,2,2,2,2,2,2,2,2,2,2,2,2,2,2,2,
2,2,2,2,2,2,2,2,2,2,2,2,2,2,2,2,2,2,2,2,2,2,2,2,2,2,2,2,2,2,2,2,2,2,2,2,
2,2,2,2,4),(-18.0721778794789,-18.0147391790313,-17.848488462182,-17.6523618007567,
-17.4700564061978,-17.3315069833901,-17.1399140645343,-16.9510607065254,
-16.7547238024059,-16.6382243763846,-16.4131310110674,-16.2310907448218,
-16.1090716764663,-15.9862441360979,-15.7700282293703,-15.5865362500968,
-15.4579456815901,-15.3260537827938,-15.1246399336788,-14.9414739734795,
-14.8211784252922,-14.6965292288557,-14.4825265993111,-14.2984956615897,
-14.1707149237915,-14.0378832037766,-13.8386208210009,-13.6558760636882,
-13.5349646836358,-13.4110162700538,-13.196182681518,-13.012369598465,-12.8842744198052,
-12.7518244552662,-12.5517071320015,-12.3688020842637,-12.2481359237797,
-12.1239203513428,-11.9094128952947,-11.7255208756108,-11.5975483555581,
-11.4649570988441,-11.2651676578925,-11.0823276922443,-10.9615705901044,
-10.8374602821415,-10.6228321046749,-10.4389743666522,-10.3109571588975,
-10.1784233654973,-9.97851117792921,-9.79564987665335,-9.67493035708778,
-9.55078209715648,-9.33620479360897,-9.15233765659768,-9.02434023802163,
-8.89178711592832,-8.69192612399274,-8.50907676515503,-8.38834528084005,
-8.26421415879336,-8.04962168685307,-7.86576193192956,-7.77890601744087),
 .UNSPECIFIED.);
#29519=B_SPLINE_CURVE_WITH_KNOTS('',3,(#113939,#113940,#113941,#113942,
#113943,#113944,#113945,#113946,#113947,#113948,#113949,#113950,#113951,
#113952,#113953,#113954,#113955,#113956,#113957,#113958),.UNSPECIFIED.,
 .F.,.F.,(4,2,2,2,2,2,2,2,2,4),(-8.47209184883771,-8.00048983906625,-7.52055114659877,
-6.8722219354319,-6.22309965668783,-5.57315017673749,-4.92241575243503,
-4.27087199654946,-3.61860418547544,-3.49997929625738),.UNSPECIFIED.);
#29520=B_SPLINE_CURVE_WITH_KNOTS('',3,(#113962,#113963,#113964,#113965,
#113966,#113967,#113968,#113969,#113970,#113971,#113972,#113973,#113974,
#113975,#113976,#113977,#113978,#113979,#113980,#113981),.UNSPECIFIED.,
 .F.,.F.,(4,2,2,2,2,2,2,2,2,4),(-3.49997929625738,-2.96555708180064,-2.63548584285813,
-2.32891559001148,-1.67589454653547,-1.34607632565228,-1.03948591871613,
-0.517021270138503,-0.266082667592821,-9.99999997031153E-7),
 .UNSPECIFIED.);
#29521=B_SPLINE_CURVE_WITH_KNOTS('',3,(#113982,#113983,#113984,#113985,
#113986,#113987,#113988,#113989,#113990,#113991,#113992,#113993,#113994,
#113995,#113996,#113997),.UNSPECIFIED.,.F.,.F.,(4,2,2,2,2,2,2,4),(1.00000001422647E-6,
0.289657184683206,0.584406985012342,1.32553765774545,1.87661181724534,2.26478053342409,
2.87644457082816,3.45555001571885),.UNSPECIFIED.);
#29522=B_SPLINE_CURVE_WITH_KNOTS('',3,(#113999,#114000,#114001,#114002,
#114003,#114004,#114005,#114006,#114007,#114008,#114009,#114010,#114011,
#114012,#114013,#114014,#114015,#114016,#114017,#114018,#114019,#114020,
#114021,#114022,#114023,#114024,#114025,#114026,#114027,#114028,#114029,
#114030,#114031,#114032,#114033,#114034,#114035,#114036,#114037,#114038,
#114039,#114040,#114041,#114042,#114043,#114044,#114045,#114046,#114047,
#114048,#114049,#114050,#114051,#114052,#114053,#114054,#114055,#114056,
#114057,#114058,#114059,#114060,#114061,#114062,#114063,#114064,#114065,
#114066,#114067,#114068,#114069,#114070,#114071,#114072,#114073,#114074,
#114075,#114076,#114077,#114078,#114079,#114080,#114081,#114082,#114083,
#114084,#114085,#114086,#114087,#114088,#114089,#114090,#114091,#114092,
#114093,#114094,#114095,#114096,#114097,#114098,#114099,#114100,#114101,
#114102,#114103,#114104,#114105,#114106,#114107,#114108,#114109,#114110,
#114111,#114112),.UNSPECIFIED.,.F.,.F.,(4,2,2,2,2,2,2,2,2,2,2,2,2,2,2,2,
2,2,2,2,2,2,2,2,2,2,2,2,2,2,2,2,2,2,2,2,2,2,2,2,2,2,2,2,2,2,2,2,2,2,2,2,
2,2,2,2,4),(2.41008863111305,2.52174442163098,2.70033972549205,2.92369762280168,
3.04486262995073,3.2699058204366,3.47593555345123,3.71971767488146,3.93301751394918,
4.14313038398822,4.38696718236632,4.52827216930786,4.70511631179351,4.95526170895235,
5.05978336461602,5.19319665811648,5.37184186831745,5.59474028269326,5.7162341072511,
5.94201868468735,6.14780793011872,6.39208756826504,6.59175960584656,6.81006046539538,
7.05854698653331,7.20057922269586,7.37723602770402,7.62878532831887,7.73236772863619,
7.93016354412659,8.14674889545556,8.39450091527641,8.53613198848105,8.71290018477586,
8.96372521774679,9.06781001094518,9.2027827813947,9.3807836127047,9.61369745721821,
9.72870340636482,9.93943009685857,10.150844445182,10.3980528363782,10.61427984803,
10.8233562392541,11.0673155262955,11.2701613800128,11.4848671499499,11.735161198995,
11.9483525425192,12.1585505827427,12.4024637528689,12.5437967955747,12.7206663052054,
12.9708642740141,13.075392587722,13.0972599015927),.UNSPECIFIED.);
#29523=B_SPLINE_CURVE_WITH_KNOTS('',3,(#114113,#114114,#114115,#114116,
#114117,#114118,#114119,#114120,#114121,#114122,#114123,#114124,#114125,
#114126,#114127,#114128,#114129,#114130,#114131,#114132,#114133,#114134,
#114135,#114136,#114137,#114138,#114139,#114140,#114141,#114142,#114143,
#114144,#114145,#114146,#114147,#114148,#114149,#114150,#114151,#114152,
#114153,#114154,#114155,#114156,#114157,#114158,#114159,#114160,#114161,
#114162,#114163,#114164,#114165,#114166,#114167,#114168,#114169,#114170,
#114171,#114172,#114173,#114174,#114175,#114176,#114177,#114178,#114179,
#114180,#114181,#114182,#114183,#114184,#114185,#114186,#114187,#114188,
#114189,#114190,#114191,#114192,#114193,#114194,#114195,#114196,#114197,
#114198,#114199,#114200,#114201,#114202,#114203,#114204,#114205,#114206,
#114207,#114208,#114209,#114210,#114211,#114212,#114213,#114214,#114215,
#114216,#114217,#114218,#114219,#114220,#114221,#114222,#114223,#114224),
 .UNSPECIFIED.,.F.,.F.,(4,2,2,2,2,2,2,2,2,2,2,2,2,2,2,2,2,2,2,2,2,2,2,2,
2,2,2,2,2,2,2,2,2,2,2,2,2,2,2,2,2,2,2,2,2,2,2,2,2,2,2,2,2,2,2,4),(35.6719042779843,
35.698846252975,35.9456358690002,36.1561600266645,36.3691876752439,36.4852065366329,
36.7165059103028,36.8945968142958,37.0293842265218,37.1335515931008,37.3842580697099,
37.5610455870247,37.7026183581998,37.9465483670245,38.156808619327,38.3697830199319,
38.6199604238591,38.8343464422794,39.0378777959768,39.2854304033603,39.5002526882164,
39.7019618265655,39.8068806810891,40.0564398533407,40.2333648418571,40.374422708839,
40.6183598224011,40.828585309869,41.0416113215738,41.2918064614692,41.5062756580261,
41.7095792835508,41.9536140589348,42.1629930736033,42.3782883405402,42.6224005275956,
42.8295076043742,43.0515020881796,43.1713412678411,43.396670626196,43.5751131440329,
43.7090103891009,43.8134320109559,44.0637072404468,44.240525253567,44.3818890339293,
44.6299725742976,44.8472345963081,45.0435004559988,45.1465753469289,45.4038401488928,
45.5827799938148,45.7182660506219,45.8319348150512,46.018095320874,46.173488535676),
 .UNSPECIFIED.);
#29524=B_SPLINE_CURVE_WITH_KNOTS('',3,(#114240,#114241,#114242,#114243,
#114244,#114245,#114246,#114247,#114248,#114249,#114250,#114251,#114252,
#114253,#114254,#114255,#114256,#114257),.UNSPECIFIED.,.F.,.F.,(4,2,2,2,
2,2,2,2,4),(0.000255302998063218,0.246325831779527,0.49141476805784,0.65921643818013,
0.997718736921762,1.17390964291707,1.34739888243814,1.62418200982642,1.88073156156305),
 .UNSPECIFIED.);
#29525=B_SPLINE_CURVE_WITH_KNOTS('',3,(#114258,#114259,#114260,#114261,
#114262,#114263,#114264,#114265,#114266,#114267,#114268,#114269,#114270,
#114271,#114272,#114273),.UNSPECIFIED.,.F.,.F.,(4,2,2,2,2,2,2,4),(4.9144922740773E-5,
0.142815688788647,0.281124699864451,0.565337366058049,0.730491337491295,
0.901589879048025,1.18024330277771,1.46497496578543),.UNSPECIFIED.);
#29526=B_SPLINE_CURVE_WITH_KNOTS('',3,(#114275,#114276,#114277,#114278,
#114279,#114280),.UNSPECIFIED.,.F.,.F.,(4,2,4),(0.490673357805338,0.745336678902669,
0.999999351274048),.UNSPECIFIED.);
#29527=B_SPLINE_CURVE_WITH_KNOTS('',3,(#114282,#114283,#114284,#114285,
#114286,#114287),.UNSPECIFIED.,.F.,.F.,(4,2,4),(0.000935847610688105,0.245336678902669,
0.490673357805338),.UNSPECIFIED.);
#29528=B_SPLINE_CURVE_WITH_KNOTS('',3,(#114291,#114292,#114293,#114294,
#114295,#114296,#114297,#114298,#114299,#114300,#114301,#114302,#114303,
#114304,#114305,#114306,#114307,#114308,#114309,#114310,#114311,#114312,
#114313,#114314,#114315,#114316,#114317,#114318),.UNSPECIFIED.,.F.,.F.,
(4,2,2,2,2,2,2,2,2,2,2,2,2,4),(-2.64509018645311,-2.50816004857991,-2.34671657830517,
-2.01718588845666,-1.85756130276746,-1.70918083912142,-1.55034169509354,
-1.22132434868371,-1.06162752878633,-0.905703863111212,-0.749839080353907,
-0.422524714244554,-0.31803881392449,-9.99999997919332E-7),
 .UNSPECIFIED.);
#29529=B_SPLINE_CURVE_WITH_KNOTS('',3,(#114320,#114321,#114322,#114323,
#114324,#114325,#114326,#114327,#114328,#114329,#114330,#114331,#114332,
#114333,#114334,#114335,#114336,#114337,#114338,#114339,#114340,#114341,
#114342,#114343,#114344,#114345,#114346,#114347,#114348,#114349),
 .UNSPECIFIED.,.F.,.F.,(4,2,2,2,2,2,2,2,2,2,2,2,2,2,4),(-2.22830115735267,
-2.10423539530511,-1.98117528854211,-1.76090462968372,-1.61039047033868,
-1.27976081955513,-1.11407105510081,-0.947815483327209,-0.811106554685308,
-0.570211254781244,-0.456895349287952,-0.242344900393441,-0.166499094513352,
-0.0837880375494301,-0.00040012110997669),.UNSPECIFIED.);
#29530=B_SPLINE_CURVE_WITH_KNOTS('',3,(#114350,#114351,#114352,#114353,
#114354,#114355,#114356,#114357),.UNSPECIFIED.,.F.,.F.,(4,2,2,4),(-0.414938412676938,
-0.20738927105766,-0.103997999406809,-3.00555698333633E-5),
 .UNSPECIFIED.);
#29531=B_SPLINE_CURVE_WITH_KNOTS('',3,(#114358,#114359,#114360,#114361,
#114362,#114363,#114364,#114365,#114366,#114367,#114368,#114369,#114370,
#114371,#114372,#114373,#114374,#114375,#114376,#114377,#114378,#114379,
#114380,#114381,#114382,#114383,#114384,#114385,#114386,#114387,#114388,
#114389,#114390,#114391,#114392,#114393,#114394,#114395,#114396,#114397,
#114398,#114399,#114400,#114401,#114402,#114403,#114404,#114405,#114406,
#114407,#114408,#114409,#114410,#114411),.UNSPECIFIED.,.F.,.F.,(4,2,2,2,
2,2,2,2,2,2,2,2,2,2,2,2,2,2,2,2,2,2,2,2,2,2,4),(-5.28894858945498,-5.08167259374315,
-4.81846912921226,-4.67057708951716,-4.33526508630831,-4.17540607219834,
-3.93856667323282,-3.73878662711519,-3.50054599788927,-3.27019447785332,
-3.12273109480938,-2.97074609410328,-2.64130975684182,-2.41922687895394,
-2.28199475627433,-2.06266818806845,-1.80663906162605,-1.6623990385579,
-1.32730358543026,-1.16824509313182,-0.931652725510682,-0.768974340438366,
-0.515348342954449,-0.371740570718675,-0.186227377844307,-0.093912563896873,
-1.00000000813338E-6),.UNSPECIFIED.);
#29532=B_SPLINE_CURVE_WITH_KNOTS('',3,(#114415,#114416,#114417,#114418,
#114419,#114420,#114421,#114422,#114423,#114424,#114425,#114426,#114427,
#114428,#114429,#114430,#114431,#114432,#114433,#114434,#114435,#114436,
#114437,#114438,#114439,#114440,#114441,#114442,#114443,#114444,#114445,
#114446,#114447,#114448,#114449,#114450,#114451,#114452,#114453,#114454,
#114455,#114456,#114457,#114458,#114459,#114460),.UNSPECIFIED.,.F.,.F.,
(4,2,2,1,1,1,2,2,2,2,1,1,1,1,2,2,2,2,2,2,2,2,1,1,1,2,2,4),(0.,0.124999999999551,
0.187499999999329,0.21874999999922,0.234374999999166,0.242187499999141,
0.248046874999122,0.249999999999116,0.374999999998904,0.437499999998797,
0.468749999998741,0.484374999998712,0.492187499998699,0.496093749998692,
0.499023437498686,0.499999999998685,0.562499999998843,0.593749999998923,
0.609374999998965,0.624999999999006,0.687499999999173,0.718749999999255,
0.734374999999296,0.742187499999314,0.746093749999326,0.748046874999334,
0.749999999999342,0.999999681575655),.UNSPECIFIED.);
#29533=B_SPLINE_CURVE_WITH_KNOTS('',3,(#114462,#114463,#114464,#114465,
#114466,#114467,#114468,#114469,#114470,#114471,#114472,#114473,#114474,
#114475,#114476,#114477,#114478,#114479,#114480,#114481,#114482,#114483,
#114484,#114485,#114486,#114487,#114488,#114489,#114490,#114491,#114492,
#114493,#114494,#114495,#114496,#114497,#114498,#114499,#114500,#114501,
#114502,#114503,#114504),.UNSPECIFIED.,.F.,.F.,(4,3,3,3,3,3,3,3,3,3,3,3,
3,3,4),(0.,0.0851829461708695,0.125,0.222485710899397,0.25,0.359792863725203,
0.375,0.5,0.625,0.634408323454812,0.75,0.771715737793405,0.875,0.909019034253072,
1.),.UNSPECIFIED.);
#29534=B_SPLINE_CURVE_WITH_KNOTS('',3,(#114506,#114507,#114508,#114509,
#114510,#114511,#114512,#114513,#114514,#114515,#114516,#114517,#114518,
#114519,#114520,#114521,#114522,#114523,#114524,#114525,#114526,#114527,
#114528,#114529,#114530,#114531,#114532,#114533,#114534,#114535,#114536,
#114537,#114538,#114539,#114540,#114541,#114542,#114543,#114544,#114545,
#114546,#114547,#114548,#114549,#114550,#114551,#114552,#114553,#114554,
#114555,#114556,#114557,#114558,#114559,#114560,#114561,#114562,#114563,
#114564,#114565,#114566,#114567,#114568,#114569,#114570,#114571,#114572,
#114573,#114574,#114575,#114576,#114577,#114578,#114579,#114580,#114581,
#114582,#114583,#114584,#114585,#114586,#114587,#114588,#114589,#114590,
#114591,#114592,#114593,#114594,#114595,#114596,#114597,#114598,#114599,
#114600,#114601,#114602,#114603,#114604,#114605,#114606,#114607,#114608,
#114609,#114610,#114611,#114612,#114613,#114614,#114615,#114616,#114617,
#114618,#114619,#114620,#114621,#114622,#114623,#114624,#114625,#114626,
#114627,#114628,#114629,#114630,#114631,#114632,#114633,#114634,#114635,
#114636,#114637,#114638,#114639,#114640,#114641,#114642,#114643,#114644,
#114645,#114646,#114647,#114648,#114649,#114650,#114651,#114652,#114653,
#114654,#114655,#114656,#114657,#114658,#114659,#114660,#114661,#114662,
#114663,#114664,#114665,#114666,#114667,#114668,#114669,#114670,#114671),
 .UNSPECIFIED.,.F.,.F.,(4,3,3,3,3,3,3,3,3,3,3,3,3,3,3,3,3,3,3,3,3,3,3,3,
3,3,3,3,3,3,3,3,3,3,3,3,3,3,3,3,3,3,3,3,3,3,3,3,3,3,3,3,3,3,3,4),(0.,0.0502845361710956,
0.0994669690397177,0.126508894795659,0.177997127033869,0.202535883941732,
0.250000000000155,0.275210682027024,0.336732694395824,0.343185824135615,
0.375000000000234,0.407090352173637,0.437500000000274,0.468541360955746,
0.468750000000296,0.484375000000307,0.492187500000312,0.496093750000314,
0.500000000000316,0.533182600914947,0.562500000000305,0.593750000000299,
0.602610758708892,0.609375000000297,0.617187500000295,0.621093750000294,
0.623046875000291,0.625000000000289,0.646711254898203,0.668295817163414,
0.683216765640327,0.687500000000225,0.708161347198757,0.718750000000194,
0.73437500000018,0.742187500000173,0.743753663871175,0.74609375000017,0.74975032942102,
0.750000000000166,0.773417459328957,0.797812834268651,0.804484657939817,
0.812500000000111,0.839850659045814,0.843750000000082,0.859375000000067,
0.867187500000061,0.87109375000006,0.873046875000058,0.875000000000055,
0.880771660675667,0.92555749543768,0.951439720715529,0.994584358314706,
1.),.UNSPECIFIED.);
#29535=B_SPLINE_CURVE_WITH_KNOTS('',3,(#114673,#114674,#114675,#114676,
#114677,#114678,#114679,#114680,#114681,#114682,#114683,#114684,#114685,
#114686,#114687,#114688,#114689,#114690,#114691,#114692,#114693,#114694,
#114695,#114696,#114697,#114698,#114699,#114700,#114701,#114702,#114703,
#114704,#114705,#114706,#114707,#114708,#114709,#114710,#114711,#114712,
#114713,#114714,#114715,#114716,#114717,#114718,#114719,#114720,#114721,
#114722,#114723,#114724,#114725,#114726,#114727,#114728,#114729,#114730,
#114731,#114732,#114733,#114734,#114735,#114736,#114737,#114738,#114739,
#114740,#114741,#114742,#114743,#114744,#114745,#114746,#114747,#114748,
#114749,#114750,#114751,#114752,#114753,#114754,#114755,#114756,#114757,
#114758,#114759,#114760,#114761,#114762,#114763,#114764,#114765,#114766,
#114767,#114768,#114769,#114770,#114771,#114772,#114773,#114774,#114775,
#114776,#114777,#114778,#114779,#114780,#114781,#114782,#114783,#114784,
#114785,#114786,#114787,#114788,#114789,#114790,#114791,#114792,#114793,
#114794,#114795,#114796,#114797,#114798,#114799,#114800,#114801,#114802,
#114803,#114804,#114805,#114806,#114807,#114808,#114809,#114810,#114811),
 .UNSPECIFIED.,.F.,.F.,(4,3,3,3,3,3,3,3,3,3,3,3,3,3,3,3,3,3,3,3,3,3,3,3,
3,3,3,3,3,3,3,3,3,3,3,3,3,3,3,3,3,3,3,3,3,3,4),(0.,0.0387804699265066,0.0942195402664754,
0.102869907782688,0.124999999999886,0.168539308649517,0.187499999999826,
0.218749999999794,0.234374999999778,0.236283397554344,0.242187499999772,
0.24609374999977,0.249718717532596,0.249999999999769,0.301433219361833,
0.312499999999771,0.343749999999771,0.359374999999769,0.367187499999768,
0.368285161567645,0.373965193564266,0.374999999999768,0.4186575976671,0.43658151927549,
0.437499999999769,0.468749999999769,0.484374999999771,0.492187499999769,
0.496093749999768,0.498046874999767,0.499600428894499,0.499999999999766,
0.552876401003889,0.572979629602993,0.627644747305819,0.644937199235735,
0.698789788204271,0.71444928382849,0.749999999999883,0.781357579985869,
0.833170646642696,0.845560939644304,0.896652264821656,0.906911855988006,
0.955116861547587,0.965240055383411,1.),.UNSPECIFIED.);
#29536=B_SPLINE_CURVE_WITH_KNOTS('',3,(#114813,#114814,#114815,#114816,
#114817,#114818,#114819,#114820,#114821,#114822,#114823,#114824,#114825,
#114826,#114827,#114828,#114829,#114830,#114831,#114832,#114833,#114834,
#114835,#114836,#114837,#114838,#114839,#114840,#114841,#114842,#114843,
#114844,#114845,#114846,#114847,#114848,#114849,#114850,#114851,#114852,
#114853,#114854,#114855),.UNSPECIFIED.,.F.,.F.,(4,3,3,3,3,3,3,3,3,3,3,3,
3,3,4),(0.,0.0891026163983255,0.125,0.226410788650375,0.25,0.363723238331853,
0.375,0.5,0.625,0.638348932643424,0.75,0.775661264039743,0.875,0.912969309651361,
1.),.UNSPECIFIED.);
#29537=B_SPLINE_CURVE_WITH_KNOTS('',3,(#114857,#114858,#114859,#114860,
#114861,#114862,#114863,#114864,#114865,#114866,#114867,#114868,#114869,
#114870,#114871,#114872,#114873,#114874,#114875,#114876,#114877,#114878,
#114879,#114880,#114881,#114882,#114883,#114884,#114885,#114886,#114887,
#114888,#114889,#114890,#114891,#114892,#114893,#114894,#114895,#114896,
#114897,#114898,#114899,#114900,#114901,#114902,#114903,#114904,#114905,
#114906,#114907,#114908,#114909,#114910,#114911,#114912),.UNSPECIFIED.,
 .F.,.F.,(4,2,2,1,1,1,1,2,2,2,2,2,2,2,2,1,1,1,1,2,2,2,1,1,1,1,2,2,2,1,1,
1,1,2,2,4),(0.,0.124999999999216,0.187499999998822,0.218749999998626,0.234374999998527,
0.242187499998475,0.246093749998447,0.248046874998435,0.249999999998424,
0.312499999998387,0.343749999998366,0.359374999998357,0.374999999998348,
0.437499999998312,0.468749999998293,0.484374999998284,0.492187499998276,
0.496093749998271,0.498046874998268,0.499023437498271,0.499999999998274,
0.562499999998525,0.593749999998648,0.609374999998706,0.617187499998738,
0.621093749998754,0.623046874998761,0.624999999998768,0.687499999998984,
0.71874999999909,0.734374999999143,0.742187499999172,0.746093749999189,
0.748046874999198,0.749999999999207,1.),.UNSPECIFIED.);
#29538=B_SPLINE_CURVE_WITH_KNOTS('',3,(#114917,#114918,#114919,#114920,
#114921,#114922,#114923,#114924,#114925,#114926,#114927,#114928,#114929,
#114930,#114931,#114932,#114933,#114934,#114935,#114936,#114937,#114938,
#114939,#114940,#114941,#114942,#114943,#114944,#114945,#114946,#114947,
#114948,#114949,#114950,#114951,#114952,#114953,#114954,#114955,#114956,
#114957,#114958,#114959,#114960,#114961,#114962,#114963,#114964,#114965,
#114966,#114967,#114968,#114969,#114970,#114971,#114972,#114973,#114974,
#114975,#114976,#114977,#114978,#114979,#114980,#114981,#114982,#114983,
#114984,#114985,#114986,#114987,#114988,#114989,#114990,#114991,#114992,
#114993,#114994,#114995,#114996,#114997,#114998,#114999,#115000,#115001,
#115002,#115003,#115004,#115005,#115006,#115007,#115008,#115009,#115010,
#115011,#115012,#115013,#115014,#115015,#115016,#115017,#115018,#115019,
#115020,#115021,#115022,#115023,#115024,#115025,#115026,#115027,#115028,
#115029,#115030,#115031,#115032,#115033,#115034,#115035,#115036,#115037,
#115038,#115039,#115040,#115041,#115042,#115043,#115044,#115045,#115046,
#115047,#115048,#115049,#115050,#115051,#115052,#115053,#115054,#115055,
#115056,#115057,#115058,#115059,#115060,#115061,#115062,#115063,#115064,
#115065,#115066,#115067),.UNSPECIFIED.,.F.,.F.,(4,3,3,3,3,3,3,3,3,3,3,3,
3,3,3,3,3,3,3,3,3,3,3,3,3,3,3,3,3,3,3,3,3,3,3,3,3,3,3,3,3,3,3,3,3,3,3,3,
3,3,4),(0.,0.062500000000062,0.121231089415165,0.125000000000124,0.163221664701878,
0.187500000000186,0.218750000000215,0.234375000000229,0.242187500000236,
0.24804687500024,0.250000000000239,0.304896813849926,0.312500000000136,
0.332752681627818,0.343750000000084,0.35937500000006,0.367187500000049,
0.371093750000046,0.373046875000042,0.375000000000038,0.416499412144631,
0.437500000000003,0.468749999999986,0.48437499999998,0.492187499999977,
0.496093749999974,0.498046874999974,0.499999999999975,0.505620037612421,
0.542493516498535,0.562500000000078,0.59375000000013,0.609375000000156,
0.617187500000171,0.624056075689695,0.625000000000187,0.652859210405975,
0.667499665105052,0.687500000000334,0.716973604152224,0.718750000000407,
0.734375000000444,0.742187500000462,0.746093750000471,0.748046875000471,
0.750000000000471,0.80654618724685,0.848568566521544,0.91466210797078,0.984037448506897,
1.),.UNSPECIFIED.);
#29539=B_SPLINE_CURVE_WITH_KNOTS('',3,(#115069,#115070,#115071,#115072,
#115073,#115074,#115075,#115076,#115077,#115078,#115079,#115080,#115081,
#115082,#115083,#115084,#115085,#115086,#115087,#115088,#115089,#115090,
#115091,#115092,#115093,#115094,#115095,#115096,#115097,#115098,#115099,
#115100,#115101,#115102,#115103,#115104,#115105,#115106,#115107,#115108,
#115109,#115110,#115111,#115112,#115113,#115114,#115115,#115116,#115117,
#115118,#115119,#115120,#115121,#115122,#115123,#115124,#115125,#115126,
#115127,#115128,#115129,#115130,#115131,#115132,#115133,#115134,#115135,
#115136,#115137,#115138,#115139,#115140,#115141,#115142,#115143,#115144,
#115145,#115146,#115147,#115148,#115149,#115150,#115151,#115152,#115153,
#115154,#115155,#115156,#115157,#115158,#115159,#115160,#115161,#115162,
#115163,#115164,#115165,#115166,#115167,#115168,#115169,#115170,#115171,
#115172,#115173,#115174,#115175,#115176,#115177,#115178,#115179,#115180,
#115181,#115182,#115183,#115184,#115185,#115186,#115187,#115188,#115189,
#115190,#115191,#115192,#115193,#115194,#115195,#115196,#115197,#115198,
#115199,#115200,#115201,#115202,#115203,#115204,#115205,#115206,#115207,
#115208,#115209,#115210,#115211,#115212,#115213,#115214,#115215,#115216,
#115217,#115218,#115219),.UNSPECIFIED.,.F.,.F.,(4,3,3,3,3,3,3,3,3,3,3,3,
3,3,3,3,3,3,3,3,3,3,3,3,3,3,3,3,3,3,3,3,3,3,3,3,3,3,3,3,3,3,3,3,3,3,3,3,
3,3,4),(1.72657252367726E-14,0.0313585598533987,0.0630900598213949,0.0954643376068659,
0.124999999999572,0.158293445510127,0.192289017368953,0.218749999999252,
0.234374999999199,0.242187499999174,0.246093749999162,0.248046874999155,
0.249511718749151,0.249999999999149,0.277343749999143,0.303223001372441,
0.328859577421254,0.354258958240136,0.379426422600146,0.404255272733001,
0.42889482456838,0.453251627638804,0.468749999999104,0.484374999999102,
0.492187499999101,0.496093749999101,0.499126022146931,0.499999999999101,
0.523490792672927,0.547898193588698,0.571926688005287,0.596161788289904,
0.620607891014182,0.64539693871608,0.670375825827579,0.695677573208496,
0.718749999999088,0.734374999999086,0.742187499999085,0.746093749999085,
0.748046874999085,0.749511718749087,0.749999999999087,0.784171524212072,
0.81788730066329,0.850916982531674,0.874999999999544,0.907027947890119,
0.938664708227929,0.969685288090575,1.),.UNSPECIFIED.);
#29540=B_SPLINE_CURVE_WITH_KNOTS('',3,(#115220,#115221,#115222,#115223,
#115224,#115225,#115226,#115227,#115228,#115229,#115230,#115231,#115232,
#115233,#115234,#115235,#115236,#115237,#115238,#115239,#115240,#115241,
#115242,#115243,#115244,#115245,#115246,#115247,#115248,#115249,#115250,
#115251,#115252,#115253,#115254,#115255,#115256,#115257,#115258,#115259,
#115260,#115261,#115262,#115263,#115264,#115265,#115266,#115267,#115268,
#115269,#115270,#115271,#115272,#115273,#115274),.UNSPECIFIED.,.F.,.F.,
(4,2,2,1,1,1,1,2,2,2,2,1,2,2,2,2,1,1,1,2,2,2,1,1,1,1,2,2,2,1,1,1,2,2,4),
(0.,0.12500000000011,0.187500000000167,0.218750000000197,0.234375000000212,
0.242187500000223,0.246093750000225,0.248046875000223,0.250000000000222,
0.312500000000213,0.343750000000213,0.35937500000021,0.367187500000211,
0.375000000000212,0.437500000000193,0.468750000000179,0.484375000000175,
0.492187500000171,0.496093750000168,0.498046875000166,0.500000000000165,
0.562500000000093,0.593750000000061,0.609375000000042,0.617187500000036,
0.621093750000036,0.623046875000033,0.62500000000003,0.687500000000018,
0.718750000000013,0.734375000000011,0.74218750000001,0.746093750000013,
0.750000000000015,1.),.UNSPECIFIED.);
#29541=B_SPLINE_CURVE_WITH_KNOTS('',3,(#115286,#115287,#115288,#115289,
#115290,#115291,#115292,#115293,#115294,#115295,#115296,#115297,#115298,
#115299,#115300,#115301,#115302,#115303,#115304,#115305,#115306,#115307,
#115308,#115309,#115310,#115311,#115312,#115313,#115314,#115315,#115316,
#115317,#115318,#115319,#115320,#115321,#115322,#115323,#115324,#115325,
#115326,#115327,#115328,#115329,#115330,#115331,#115332,#115333,#115334,
#115335,#115336,#115337,#115338,#115339,#115340,#115341,#115342,#115343,
#115344,#115345,#115346,#115347,#115348,#115349,#115350,#115351,#115352,
#115353,#115354,#115355,#115356,#115357,#115358,#115359,#115360,#115361,
#115362,#115363,#115364,#115365,#115366,#115367,#115368,#115369,#115370,
#115371,#115372,#115373,#115374,#115375,#115376,#115377,#115378,#115379,
#115380,#115381,#115382,#115383,#115384,#115385,#115386,#115387,#115388,
#115389,#115390,#115391,#115392,#115393,#115394,#115395,#115396,#115397,
#115398,#115399,#115400,#115401,#115402,#115403,#115404,#115405,#115406,
#115407,#115408,#115409,#115410,#115411,#115412,#115413,#115414,#115415),
 .UNSPECIFIED.,.F.,.F.,(4,3,3,3,3,3,3,3,3,3,3,3,3,3,3,3,3,3,3,3,3,3,3,3,
3,3,3,3,3,3,3,3,3,3,3,3,3,3,3,3,3,3,3,4),(0.,0.0155305327960008,0.0311496512367539,
0.0467827647740799,0.0524931088100301,0.0681787493894734,0.0835455441413793,
0.0993906076345913,0.115235671127803,0.120656007198578,0.124426507423533,
0.125369132479772,0.126311757536011,0.128197007648489,0.135738008098405,
0.150820008998236,0.170300375377521,0.1809840107979,0.18297180671857,0.202416974502378,
0.221864494449803,0.241312014397229,0.243677276861593,0.248853014847146,
0.249795639903385,0.250738264959625,0.252623515072105,0.256394015297065,
0.271476016196905,0.297137858146395,0.301640017996586,0.310841253760449,
0.336445877357579,0.361968021595948,0.365738521820908,0.36831758881443,
0.369509022045868,0.371220548011419,0.377050022495787,0.392132023395624,
0.422296025195297,0.434902671324438,0.463575489153042,0.482624028794642),
 .UNSPECIFIED.);
#29542=B_SPLINE_CURVE_WITH_KNOTS('',3,(#115417,#115418,#115419,#115420,
#115421,#115422,#115423,#115424,#115425,#115426,#115427,#115428,#115429,
#115430,#115431,#115432,#115433,#115434,#115435,#115436,#115437,#115438,
#115439,#115440,#115441,#115442,#115443,#115444,#115445,#115446,#115447,
#115448,#115449,#115450,#115451,#115452,#115453,#115454),.UNSPECIFIED.,
 .F.,.F.,(4,2,2,1,2,2,2,2,2,1,1,1,1,2,2,2,2,1,1,1,2,2,4),(0.482624028794642,
0.498792027894815,0.514960026994988,0.547296025195333,0.611968021596022,
0.676640017996712,0.741312014397401,0.749396013947487,0.750406513891247,
0.751417013835008,0.753438013722528,0.757480013497569,0.77364801259773,
0.805984010798051,0.870656007198694,0.874698006973734,0.875708506917494,
0.876719006861254,0.878740006748774,0.886824006298856,0.902992005399019,
0.935328003599346,1.),.UNSPECIFIED.);
#29543=B_SPLINE_CURVE_WITH_KNOTS('',3,(#115463,#115464,#115465,#115466,
#115467,#115468,#115469,#115470,#115471,#115472,#115473,#115474,#115475,
#115476,#115477,#115478,#115479,#115480,#115481,#115482,#115483,#115484,
#115485,#115486,#115487,#115488,#115489,#115490,#115491,#115492,#115493,
#115494,#115495,#115496,#115497,#115498,#115499,#115500,#115501,#115502,
#115503,#115504,#115505,#115506,#115507,#115508,#115509,#115510,#115511,
#115512,#115513,#115514,#115515,#115516,#115517,#115518,#115519,#115520,
#115521,#115522,#115523,#115524,#115525,#115526,#115527,#115528,#115529),
 .UNSPECIFIED.,.F.,.F.,(4,3,3,3,3,3,3,3,3,3,3,3,3,3,3,3,3,3,3,3,3,3,4),
(0.51166377080594,0.527494550556984,0.543364644919874,0.559320212793699,
0.572705799393256,0.588776327230632,0.590143328248497,0.606753705472004,
0.618487320886823,0.622302447677953,0.624210011073519,0.626117574469085,
0.63374782805135,0.665558992312902,0.694789856709447,0.725310871038494,
0.740571378203017,0.748201631785278,0.754270747493039,0.755831885367539,
0.800644721001023,0.970898896272127,1.),.UNSPECIFIED.);
#29544=B_SPLINE_CURVE_WITH_KNOTS('',3,(#115531,#115532,#115533,#115534,
#115535,#115536,#115537,#115538,#115539,#115540,#115541,#115542,#115543,
#115544,#115545,#115546,#115547,#115548,#115549,#115550,#115551,#115552,
#115553,#115554,#115555,#115556,#115557,#115558,#115559,#115560,#115561,
#115562,#115563,#115564,#115565,#115566,#115567,#115568,#115569,#115570,
#115571,#115572,#115573,#115574,#115575,#115576,#115577,#115578,#115579,
#115580,#115581,#115582,#115583,#115584,#115585,#115586,#115587,#115588,
#115589,#115590,#115591,#115592,#115593,#115594,#115595,#115596,#115597,
#115598,#115599,#115600,#115601,#115602,#115603),.UNSPECIFIED.,.F.,.F.,
(4,3,3,3,3,3,3,3,3,3,3,3,3,3,3,3,3,3,3,3,3,3,3,3,4),(3.53787488667062E-13,
0.0213362951863518,0.0426471332641246,0.0639579713418974,0.0845324772100754,
0.104712953249514,0.111926449848326,0.119921196266065,0.123918569474935,
0.127076608691764,0.127915942683804,0.141403650168183,0.20292737719542,
0.223852899696638,0.239842392532111,0.255831885367583,0.352228943328355,
0.38374782805135,0.447705799393233,0.479684785064172,0.495674277899644,
0.499671651108512,0.501670337712947,0.503669024317381,0.511663770735164),
 .UNSPECIFIED.);
#29545=B_SPLINE_CURVE_WITH_KNOTS('',3,(#115681,#115682,#115683,#115684,
#115685,#115686,#115687,#115688,#115689,#115690,#115691,#115692,#115693,
#115694,#115695,#115696),.UNSPECIFIED.,.F.,.F.,(4,2,2,2,2,2,2,4),(-1.46479957099081,
-1.1805105246837,-0.90257725733764,-0.731520481211716,-0.566447433224417,
-0.281660671194902,-0.143091894881949,-4.91448849857019E-5),
 .UNSPECIFIED.);
#29546=B_SPLINE_CURVE_WITH_KNOTS('',3,(#115698,#115699,#115700,#115701,
#115702,#115703,#115704,#115705,#115706,#115707,#115708,#115709,#115710,
#115711,#115712,#115713,#115714,#115715),.UNSPECIFIED.,.F.,.F.,(4,2,2,2,
2,2,2,2,4),(-1.88059535984106,-1.62418108159893,-1.34742306272744,-1.17391543699637,
-0.99773934830901,-0.659269873371318,-0.49144696425701,-0.246353941888789,
-1.00000001190814E-6),.UNSPECIFIED.);
#29547=B_SPLINE_CURVE_WITH_KNOTS('',3,(#115719,#115720,#115721,#115722,
#115723,#115724),.UNSPECIFIED.,.F.,.F.,(4,2,4),(0.509326642194732,0.754663321097366,
0.999997368427725),.UNSPECIFIED.);
#29548=B_SPLINE_CURVE_WITH_KNOTS('',3,(#115725,#115726,#115727,#115728,
#115729,#115730),.UNSPECIFIED.,.F.,.F.,(4,2,4),(6.48725954440461E-7,0.254663321097366,
0.509326642194732),.UNSPECIFIED.);
#29549=B_SPLINE_CURVE_WITH_KNOTS('',3,(#115733,#115734,#115735,#115736,
#115737,#115738,#115739,#115740,#115741,#115742,#115743,#115744,#115745,
#115746,#115747,#115748,#115749,#115750,#115751,#115752,#115753,#115754,
#115755,#115756),.UNSPECIFIED.,.F.,.F.,(4,2,2,2,2,2,2,2,2,2,2,4),(0.415214370670141,
0.44414492098826,0.761187688701984,1.04803781412441,1.36663216176434,1.53126048254232,
1.69364240787812,1.9065115824004,2.23496333776899,2.51066490402767,2.78610480852283,
3.06208402115945),.UNSPECIFIED.);
#29550=B_SPLINE_CURVE_WITH_KNOTS('',3,(#115758,#115759,#115760,#115761,
#115762,#115763),.UNSPECIFIED.,.F.,.F.,(4,2,4),(-0.103830434024033,-0.0610640491738462,
-5.68668496666812E-5),.UNSPECIFIED.);
#29551=B_SPLINE_CURVE_WITH_KNOTS('',3,(#115766,#115767,#115768,#115769,
#115770,#115771,#115772,#115773,#115774,#115775,#115776,#115777),
 .UNSPECIFIED.,.F.,.F.,(4,2,2,2,2,4),(1.00000003078193E-6,0.31287663257672,
0.416307716745341,0.750817151791374,0.912809059863007,1.08729832187199),
 .UNSPECIFIED.);
#29552=B_SPLINE_CURVE_WITH_KNOTS('',3,(#115781,#115782,#115783,#115784,
#115785,#115786,#115787,#115788,#115789,#115790,#115791,#115792,#115793,
#115794,#115795,#115796,#115797,#115798,#115799,#115800,#115801,#115802,
#115803,#115804,#115805,#115806,#115807,#115808,#115809,#115810,#115811,
#115812,#115813,#115814,#115815,#115816,#115817,#115818,#115819,#115820,
#115821,#115822,#115823,#115824,#115825,#115826),.UNSPECIFIED.,.F.,.F.,
(4,2,2,1,1,1,2,2,2,2,1,1,1,1,2,2,2,2,2,2,2,2,1,1,1,2,2,4),(0.,0.124999999999755,
0.187499999999633,0.218749999999572,0.234374999999541,0.242187499999528,
0.248046874999513,0.249999999999507,0.374999999998963,0.437499999998691,
0.468749999998555,0.484374999998485,0.492187499998451,0.496093749998433,
0.499023437498418,0.499999999998412,0.562499999998579,0.593749999998663,
0.609374999998708,0.624999999998753,0.687499999998917,0.718749999999002,
0.734374999999047,0.742187499999073,0.746093749999086,0.748046874999093,
0.7499999999991,1.),.UNSPECIFIED.);
#29553=B_SPLINE_CURVE_WITH_KNOTS('',3,(#115828,#115829,#115830,#115831,
#115832,#115833,#115834,#115835,#115836,#115837,#115838,#115839,#115840,
#115841,#115842,#115843,#115844,#115845,#115846,#115847,#115848,#115849,
#115850,#115851,#115852,#115853,#115854,#115855,#115856,#115857,#115858,
#115859,#115860,#115861,#115862,#115863,#115864,#115865,#115866,#115867,
#115868,#115869,#115870,#115871,#115872,#115873,#115874,#115875,#115876,
#115877,#115878,#115879,#115880,#115881,#115882,#115883,#115884,#115885,
#115886,#115887,#115888,#115889,#115890,#115891,#115892,#115893,#115894,
#115895,#115896,#115897,#115898,#115899,#115900,#115901,#115902,#115903,
#115904,#115905,#115906,#115907,#115908,#115909,#115910,#115911,#115912,
#115913,#115914,#115915,#115916,#115917,#115918,#115919,#115920,#115921,
#115922,#115923,#115924,#115925,#115926,#115927,#115928,#115929,#115930,
#115931,#115932,#115933),.UNSPECIFIED.,.F.,.F.,(4,3,3,3,3,3,3,3,3,3,3,3,
3,3,3,3,3,3,3,3,3,3,3,3,3,3,3,3,3,3,3,3,3,3,3,4),(0.,0.0349290761455846,
0.0707303823045988,0.095011048545903,0.124999999999988,0.166181057698321,
0.187499999999982,0.218749999999978,0.234374999999977,0.240157824751891,
0.242187499999976,0.246093749999979,0.24902343749998,0.249999999999982,
0.31267456409958,0.372848667033719,0.375000000000061,0.432592797080129,
0.4375000000001,0.468750000000121,0.484375000000131,0.492187500000136,0.496093750000137,
0.499023437500137,0.500000000000137,0.500974800543195,0.574225292197682,
0.646387457364885,0.657372771579407,0.728223741866551,0.750000000000069,
0.792392860831951,0.863966896072285,0.909141464253675,0.975114473482201,
0.999999999977459),.UNSPECIFIED.);
#29554=B_SPLINE_CURVE_WITH_KNOTS('',3,(#115935,#115936,#115937,#115938,
#115939,#115940,#115941,#115942,#115943,#115944,#115945,#115946,#115947,
#115948,#115949,#115950,#115951,#115952,#115953,#115954,#115955,#115956,
#115957,#115958,#115959,#115960,#115961,#115962,#115963,#115964,#115965,
#115966,#115967,#115968,#115969,#115970,#115971,#115972,#115973,#115974,
#115975,#115976,#115977,#115978,#115979,#115980,#115981,#115982,#115983,
#115984,#115985,#115986,#115987,#115988,#115989,#115990,#115991,#115992,
#115993,#115994,#115995,#115996,#115997,#115998,#115999,#116000,#116001,
#116002,#116003,#116004,#116005,#116006,#116007,#116008,#116009,#116010,
#116011,#116012,#116013,#116014,#116015,#116016,#116017,#116018,#116019,
#116020,#116021,#116022,#116023,#116024,#116025,#116026,#116027,#116028,
#116029,#116030,#116031,#116032,#116033,#116034),.UNSPECIFIED.,.F.,.F.,
(4,3,3,3,3,3,3,3,3,3,3,3,3,3,3,3,3,3,3,3,3,3,3,3,3,3,3,3,3,3,3,3,3,4),(1.29149088468994E-15,
0.0582680136424074,0.11778957915424,0.132355339703123,0.195189423730358,
0.2499999999999,0.301027172061525,0.364795158597509,0.374999999999851,0.437499999999827,
0.468749999999815,0.484374999999807,0.492187499999803,0.496093749999802,
0.4980468749998,0.49993495296673,0.499999999999798,0.562499999999693,0.624999999999588,
0.675813194782976,0.687499999999484,0.718749999999429,0.734374999999402,
0.74218749999939,0.746093749999385,0.749023437499379,0.749999999999377,
0.794477594674165,0.837925486107252,0.859170308090223,0.898790378500282,
0.937526932086563,0.975001831172104,1.),.UNSPECIFIED.);
#29555=B_SPLINE_CURVE_WITH_KNOTS('',3,(#116036,#116037,#116038,#116039,
#116040,#116041,#116042,#116043,#116044,#116045,#116046,#116047,#116048,
#116049,#116050,#116051,#116052,#116053,#116054,#116055,#116056,#116057,
#116058,#116059,#116060,#116061,#116062,#116063,#116064,#116065,#116066,
#116067,#116068,#116069,#116070,#116071,#116072,#116073,#116074,#116075,
#116076,#116077,#116078,#116079,#116080,#116081,#116082,#116083,#116084,
#116085,#116086,#116087,#116088,#116089,#116090,#116091),.UNSPECIFIED.,
 .F.,.F.,(4,2,2,1,1,1,1,2,2,2,2,2,2,2,2,1,1,1,1,2,2,2,1,1,1,1,2,2,2,1,1,
1,1,2,2,4),(0.,0.125000000000341,0.187500000000507,0.218750000000587,0.234375000000627,
0.242187500000643,0.246093750000651,0.248046875000653,0.250000000000654,
0.312500000000671,0.343750000000679,0.359375000000681,0.375000000000683,
0.43750000000069,0.468750000000697,0.484375000000704,0.492187500000707,
0.496093750000704,0.498046875000703,0.499023437500703,0.500000000000703,
0.562500000000648,0.593750000000621,0.609375000000607,0.617187500000603,
0.621093750000601,0.6230468750006,0.625000000000599,0.687500000000444,0.718750000000368,
0.734375000000333,0.742187500000316,0.746093750000307,0.748046875000303,
0.750000000000299,1.),.UNSPECIFIED.);
#29556=B_SPLINE_CURVE_WITH_KNOTS('',3,(#116096,#116097,#116098,#116099,
#116100,#116101,#116102,#116103,#116104,#116105,#116106,#116107,#116108,
#116109,#116110,#116111,#116112,#116113,#116114,#116115,#116116,#116117,
#116118,#116119,#116120,#116121,#116122,#116123,#116124,#116125,#116126,
#116127,#116128,#116129,#116130,#116131,#116132,#116133,#116134,#116135,
#116136,#116137,#116138,#116139,#116140,#116141,#116142,#116143,#116144,
#116145,#116146,#116147,#116148,#116149,#116150,#116151,#116152,#116153,
#116154,#116155,#116156,#116157,#116158,#116159,#116160,#116161,#116162,
#116163,#116164,#116165,#116166,#116167,#116168,#116169,#116170,#116171,
#116172,#116173,#116174,#116175,#116176,#116177,#116178,#116179,#116180,
#116181,#116182,#116183,#116184,#116185,#116186,#116187,#116188,#116189,
#116190,#116191,#116192,#116193,#116194,#116195,#116196,#116197,#116198,
#116199,#116200,#116201,#116202,#116203,#116204,#116205,#116206,#116207,
#116208,#116209,#116210,#116211,#116212,#116213,#116214,#116215,#116216,
#116217,#116218,#116219,#116220,#116221,#116222,#116223,#116224,#116225,
#116226,#116227,#116228,#116229,#116230,#116231,#116232,#116233,#116234,
#116235,#116236,#116237,#116238,#116239,#116240,#116241,#116242,#116243,
#116244,#116245,#116246),.UNSPECIFIED.,.F.,.F.,(4,3,3,3,3,3,3,3,3,3,3,3,
3,3,3,3,3,3,3,3,3,3,3,3,3,3,3,3,3,3,3,3,3,3,3,3,3,3,3,3,3,3,3,3,3,3,3,3,
3,3,4),(0.,0.0624999999998672,0.121231102053757,0.124999999999734,0.163221688707204,
0.187499999999604,0.218749999999539,0.234374999999508,0.242187499999495,
0.248046874999491,0.249999999999491,0.304896852417071,0.312499999999486,
0.332752736514499,0.343749999999486,0.359374999999489,0.36718749999949,
0.371093749999491,0.373046874999494,0.374999999999496,0.416499783200529,
0.437499999999609,0.468749999999662,0.484374999999692,0.492187499999707,
0.496093749999711,0.498046874999714,0.499999999999717,0.505620558654761,
0.542490554879664,0.562499999999747,0.593749999999762,0.609374999999769,
0.617187499999773,0.624061796612807,0.624999999999776,0.652866429296472,
0.66750585984053,0.687499999999818,0.716981488664328,0.718749999999839,
0.734374999999854,0.742187499999857,0.746093749999853,0.748046874999851,
0.74999999999985,0.806521545396385,0.848556247067743,0.914625004658987,
0.983976194844835,1.),.UNSPECIFIED.);
#29557=B_SPLINE_CURVE_WITH_KNOTS('',3,(#116248,#116249,#116250,#116251,
#116252,#116253,#116254,#116255,#116256,#116257,#116258,#116259,#116260,
#116261,#116262,#116263,#116264,#116265,#116266,#116267,#116268,#116269,
#116270,#116271,#116272),.UNSPECIFIED.,.F.,.F.,(4,3,3,3,3,3,3,3,4),(0.,
0.125,0.25,0.375,0.5,0.625,0.75,0.875,1.),.UNSPECIFIED.);
#29558=B_SPLINE_CURVE_WITH_KNOTS('',3,(#116274,#116275,#116276,#116277,
#116278,#116279,#116280,#116281,#116282,#116283,#116284,#116285,#116286,
#116287,#116288,#116289,#116290,#116291,#116292,#116293,#116294,#116295,
#116296,#116297,#116298,#116299,#116300,#116301,#116302,#116303,#116304,
#116305,#116306,#116307,#116308,#116309,#116310,#116311,#116312,#116313,
#116314,#116315,#116316,#116317,#116318,#116319,#116320,#116321,#116322,
#116323,#116324,#116325,#116326,#116327,#116328,#116329,#116330,#116331,
#116332,#116333,#116334,#116335,#116336,#116337,#116338,#116339,#116340,
#116341,#116342,#116343,#116344,#116345,#116346,#116347,#116348,#116349,
#116350,#116351,#116352,#116353,#116354,#116355,#116356,#116357,#116358,
#116359,#116360,#116361,#116362,#116363,#116364,#116365,#116366,#116367,
#116368,#116369,#116370,#116371,#116372,#116373,#116374,#116375,#116376,
#116377,#116378,#116379,#116380,#116381,#116382,#116383,#116384,#116385,
#116386,#116387,#116388,#116389,#116390,#116391,#116392,#116393,#116394,
#116395,#116396,#116397,#116398,#116399,#116400,#116401,#116402,#116403,
#116404,#116405,#116406,#116407,#116408,#116409,#116410,#116411,#116412,
#116413,#116414,#116415,#116416,#116417,#116418,#116419,#116420,#116421,
#116422,#116423,#116424,#116425,#116426,#116427,#116428,#116429,#116430,
#116431,#116432,#116433,#116434,#116435,#116436,#116437,#116438,#116439,
#116440,#116441,#116442,#116443,#116444,#116445,#116446,#116447,#116448,
#116449,#116450,#116451,#116452,#116453,#116454,#116455,#116456,#116457,
#116458,#116459,#116460,#116461,#116462,#116463,#116464,#116465,#116466,
#116467,#116468,#116469,#116470,#116471,#116472,#116473,#116474,#116475,
#116476,#116477,#116478,#116479,#116480,#116481,#116482,#116483,#116484,
#116485,#116486,#116487,#116488,#116489,#116490,#116491,#116492,#116493,
#116494,#116495,#116496,#116497,#116498,#116499,#116500,#116501,#116502,
#116503,#116504,#116505,#116506,#116507,#116508,#116509,#116510,#116511,
#116512,#116513,#116514,#116515,#116516,#116517,#116518,#116519,#116520,
#116521,#116522,#116523,#116524,#116525,#116526,#116527,#116528,#116529,
#116530,#116531,#116532,#116533,#116534,#116535,#116536,#116537,#116538,
#116539,#116540,#116541,#116542,#116543,#116544,#116545,#116546,#116547,
#116548,#116549,#116550,#116551,#116552,#116553,#116554,#116555,#116556),
 .UNSPECIFIED.,.F.,.F.,(4,3,3,3,3,3,3,3,3,3,3,3,3,3,3,3,3,3,3,3,3,3,3,3,
3,3,3,3,3,3,3,3,3,3,3,3,3,3,3,3,3,3,3,3,3,3,3,3,3,3,3,3,3,3,3,3,3,3,3,3,
3,3,3,3,3,3,3,3,3,3,3,3,3,3,3,3,3,3,3,3,3,3,3,3,3,3,3,3,3,3,3,3,3,3,4),
(0.,0.0218553192416152,0.0239909676408461,0.047404899596648,0.0576150789306258,
0.0817019507604128,0.0923175822312087,0.11725378633643,0.125000000000385,
0.12782188704429,0.153315965606252,0.163932697097646,0.187500000000578,
0.200455026760637,0.218750000000674,0.234375000000722,0.236703243244336,
0.242187500000746,0.246093750000759,0.248046875000764,0.249750884846123,
0.25000000000077,0.266748876337169,0.274607654122715,0.281250000000843,
0.296875000000879,0.304687500000897,0.307933981749264,0.308593750000907,
0.310546875000913,0.311523437500915,0.312500000000917,0.342097572559386,
0.34375000000095,0.359375000000966,0.367558307807294,0.375000000000983,
0.377517642532591,0.403712695856758,0.413666303605555,0.437500000001046,
0.448741255419369,0.468750000001077,0.483155469156573,0.484375000001092,
0.492187500001098,0.496093750001103,0.498046875001104,0.499818401517535,
0.500000000001105,0.520741585243092,0.542287513872453,0.557662955585771,
0.562500000001145,0.581759226316266,0.591897962726741,0.593750000001166,
0.609375000001177,0.617187500001182,0.621093750001185,0.623046875001185,
0.623651136778459,0.624023437501185,0.625000000001186,0.637497695748092,
0.648624211071175,0.661971401128478,0.675806858384994,0.678364062535773,
0.687500000001248,0.702496729367031,0.717149250528625,0.718750000001278,
0.734375000001294,0.742187500001303,0.746093750001308,0.74804687500131,
0.74902343750131,0.749511718751307,0.750000000001304,0.764878648076392,
0.791680428121145,0.802651410975554,0.829731221647044,0.840058129334189,
0.867079580400336,0.875000000000652,0.876521389536748,0.902828525497309,
0.911862695096826,0.937111114145424,0.945833175269185,0.970733896748208,
0.978118639161034,1.),.UNSPECIFIED.);
#29559=B_SPLINE_CURVE_WITH_KNOTS('',3,(#116558,#116559,#116560,#116561,
#116562,#116563,#116564,#116565,#116566,#116567,#116568,#116569,#116570,
#116571,#116572,#116573,#116574,#116575,#116576,#116577,#116578,#116579,
#116580,#116581,#116582),.UNSPECIFIED.,.F.,.F.,(4,3,3,3,3,3,3,3,4),(0.,
0.125,0.25,0.375,0.5,0.625,0.75,0.875,0.999999873942638),.UNSPECIFIED.);
#29560=B_SPLINE_CURVE_WITH_KNOTS('',3,(#116583,#116584,#116585,#116586,
#116587,#116588,#116589,#116590,#116591,#116592,#116593,#116594,#116595,
#116596,#116597,#116598,#116599,#116600,#116601,#116602,#116603,#116604,
#116605,#116606,#116607,#116608,#116609,#116610,#116611,#116612,#116613,
#116614,#116615,#116616,#116617,#116618,#116619,#116620,#116621,#116622,
#116623,#116624,#116625,#116626,#116627,#116628,#116629,#116630,#116631,
#116632,#116633,#116634,#116635,#116636,#116637),.UNSPECIFIED.,.F.,.F.,
(4,2,2,1,1,1,1,2,2,2,2,1,2,2,2,2,1,1,1,2,2,2,1,1,1,1,2,2,2,1,1,1,2,2,4),
(0.,0.124999999999915,0.187499999999874,0.218749999999858,0.23437499999985,
0.242187499999846,0.24609374999984,0.248046874999841,0.249999999999842,
0.312499999999878,0.343749999999894,0.359374999999902,0.367187499999908,
0.374999999999913,0.437499999999939,0.468749999999949,0.484374999999953,
0.492187499999951,0.49609374999995,0.498046874999954,0.499999999999959,
0.562500000000051,0.593750000000098,0.609375000000121,0.617187500000129,
0.621093750000132,0.623046875000133,0.625000000000134,0.687500000000118,
0.718750000000112,0.73437500000011,0.742187500000109,0.746093750000106,
0.750000000000103,1.),.UNSPECIFIED.);
#29561=B_SPLINE_CURVE_WITH_KNOTS('',3,(#116641,#116642,#116643,#116644,
#116645,#116646,#116647,#116648,#116649,#116650,#116651,#116652,#116653,
#116654,#116655,#116656,#116657,#116658,#116659,#116660,#116661,#116662,
#116663,#116664,#116665,#116666,#116667,#116668),.UNSPECIFIED.,.F.,.F.,
(4,2,2,1,2,2,2,2,2,2,2,1,2,2,4),(0.,0.125000000000002,0.187500000000005,
0.218750000000006,0.234375000000007,0.250000000000008,0.375000000000012,
0.437500000000012,0.500000000000012,0.625000000000009,0.687500000000007,
0.718750000000006,0.734375000000006,0.750000000000007,1.),.UNSPECIFIED.);
#29562=B_SPLINE_CURVE_WITH_KNOTS('',3,(#116670,#116671,#116672,#116673,
#116674,#116675,#116676,#116677,#116678,#116679,#116680,#116681,#116682,
#116683,#116684,#116685,#116686,#116687,#116688,#116689,#116690,#116691,
#116692,#116693,#116694,#116695,#116696,#116697,#116698,#116699,#116700,
#116701,#116702,#116703,#116704,#116705),.UNSPECIFIED.,.F.,.F.,(4,2,1,1,
1,1,2,2,2,2,1,2,2,2,1,2,2,2,2,2,4),(0.,0.124999999999964,0.187499999999947,
0.218749999999938,0.234374999999932,0.242187499999929,0.246093749999927,
0.249999999999926,0.37499999999994,0.437499999999946,0.46874999999995,0.484374999999953,
0.499999999999956,0.562499999999969,0.593749999999976,0.609374999999978,
0.624999999999981,0.687499999999985,0.718749999999986,0.749999999999987,
1.),.UNSPECIFIED.);
#29563=B_SPLINE_CURVE_WITH_KNOTS('',3,(#116728,#116729,#116730,#116731,
#116732,#116733,#116734,#116735,#116736,#116737,#116738,#116739,#116740,
#116741,#116742,#116743,#116744,#116745,#116746),.UNSPECIFIED.,.F.,.F.,
(4,3,3,3,3,3,4),(0.,0.0815195060317968,0.185640530775494,0.274473694370806,
0.363855401859883,0.461632447753659,0.498245638802628),.UNSPECIFIED.);
#29564=B_SPLINE_CURVE_WITH_KNOTS('',3,(#116884,#116885,#116886,#116887,
#116888,#116889,#116890,#116891,#116892,#116893,#116894,#116895,#116896,
#116897,#116898,#116899,#116900,#116901,#116902,#116903,#116904,#116905,
#116906,#116907,#116908,#116909,#116910,#116911,#116912,#116913,#116914,
#116915,#116916,#116917,#116918,#116919,#116920,#116921,#116922,#116923,
#116924,#116925,#116926,#116927,#116928,#116929,#116930,#116931,#116932,
#116933,#116934,#116935,#116936,#116937,#116938,#116939,#116940,#116941,
#116942,#116943,#116944),.UNSPECIFIED.,.F.,.F.,(4,3,3,3,3,3,3,3,3,3,3,3,
3,3,3,3,3,3,3,3,4),(0.,0.0927792530957532,0.181143034095441,0.250000000000402,
0.302029203004749,0.375000000000606,0.437500000000711,0.468750000000757,
0.484375000000779,0.492187500000791,0.496093750000796,0.500000000000801,
0.569042640114168,0.636907417646122,0.691184957664156,0.750000000000401,
0.8125000000003,0.870058800372124,0.925905746294812,0.980241350328491,1.),
 .UNSPECIFIED.);
#29565=B_SPLINE_CURVE_WITH_KNOTS('',3,(#116946,#116947,#116948,#116949,
#116950,#116951,#116952,#116953,#116954,#116955,#116956,#116957,#116958,
#116959,#116960,#116961,#116962,#116963,#116964,#116965,#116966,#116967,
#116968,#116969,#116970,#116971,#116972,#116973,#116974,#116975,#116976),
 .UNSPECIFIED.,.F.,.F.,(4,3,3,3,3,3,3,3,3,3,4),(2.46560854681056E-10,0.113253207042464,
0.225068571246234,0.336211172061686,0.446873791004117,0.5,0.610600731635704,
0.721861535753223,0.833640664344923,0.946719460130871,0.99999999991526),
 .UNSPECIFIED.);
#29566=B_SPLINE_CURVE_WITH_KNOTS('',3,(#116977,#116978,#116979,#116980,
#116981,#116982,#116983,#116984,#116985,#116986,#116987,#116988,#116989,
#116990,#116991,#116992),.UNSPECIFIED.,.F.,.F.,(4,2,2,1,1,2,2,2,4),(0.,
0.249999999999911,0.374999999999873,0.437499999999854,0.468749999999844,
0.484374999999845,0.499999999999846,0.749999999999923,1.),.UNSPECIFIED.);
#29567=B_SPLINE_CURVE_WITH_KNOTS('',3,(#117052,#117053,#117054,#117055,
#117056,#117057),.UNSPECIFIED.,.F.,.F.,(4,2,4),(-0.918590950811215,-0.473516281042627,
-9.99999057782475E-7),.UNSPECIFIED.);
#29568=B_SPLINE_CURVE_WITH_KNOTS('',3,(#117063,#117064,#117065,#117066,
#117067,#117068,#117069,#117070,#117071,#117072,#117073,#117074,#117075,
#117076,#117077,#117078,#117079,#117080,#117081,#117082,#117083,#117084,
#117085,#117086,#117087),.UNSPECIFIED.,.F.,.F.,(4,3,3,3,3,3,3,3,4),(0.,
0.131958835404557,0.26974144616476,0.407524056924964,0.545524898370289,
0.683735650569008,0.821345328537211,0.953680929508149,1.),.UNSPECIFIED.);
#29569=B_SPLINE_CURVE_WITH_KNOTS('',3,(#117088,#117089,#117090,#117091,
#117092,#117093,#117094,#117095,#117096,#117097,#117098,#117099,#117100,
#117101,#117102,#117103,#117104,#117105,#117106),.UNSPECIFIED.,.F.,.F.,
(4,3,3,3,3,3,4),(4.45019463169606E-7,0.162711821023231,0.327779237456247,
0.496643240664868,0.667586333454032,0.841952576666844,1.),.UNSPECIFIED.);
#29570=B_SPLINE_CURVE_WITH_KNOTS('',3,(#117172,#117173,#117174,#117175,
#117176,#117177,#117178,#117179,#117180,#117181,#117182,#117183,#117184,
#117185,#117186,#117187,#117188,#117189,#117190,#117191,#117192,#117193,
#117194,#117195,#117196,#117197,#117198,#117199,#117200,#117201,#117202,
#117203,#117204,#117205,#117206,#117207,#117208,#117209,#117210,#117211,
#117212,#117213,#117214,#117215,#117216,#117217,#117218,#117219,#117220,
#117221,#117222,#117223,#117224,#117225,#117226,#117227,#117228,#117229),
 .UNSPECIFIED.,.F.,.F.,(4,3,3,3,3,3,3,3,3,3,3,3,3,3,3,3,3,3,3,4),(0.,0.0619432161112905,
0.124508308999197,0.142068526750139,0.205837696787764,0.249999999999997,
0.279531917274151,0.346849139134802,0.413029519231283,0.483936394515832,
0.499999999999994,0.543184869644407,0.614814399058056,0.671122191652417,
0.743062292031408,0.79701922190678,0.867896471689319,0.922141629836563,
0.991397233405132,0.999997239496597),.UNSPECIFIED.);
#29571=B_SPLINE_CURVE_WITH_KNOTS('',3,(#117231,#117232,#117233,#117234,
#117235,#117236,#117237,#117238,#117239,#117240,#117241,#117242,#117243,
#117244,#117245,#117246,#117247,#117248,#117249,#117250,#117251,#117252,
#117253,#117254,#117255,#117256,#117257,#117258,#117259,#117260,#117261,
#117262,#117263,#117264,#117265,#117266,#117267,#117268,#117269,#117270,
#117271,#117272,#117273),.UNSPECIFIED.,.F.,.F.,(4,3,3,3,3,3,3,3,3,3,3,3,
3,3,4),(0.,0.0937334144157132,0.185189062989018,0.273500600704511,0.360125764759083,
0.444327725505443,0.5,0.581147963193658,0.66094496171836,0.738987112431448,
0.75,0.825900760301095,0.900636141668165,0.973772467019908,1.),
 .UNSPECIFIED.);
#29572=B_SPLINE_CURVE_WITH_KNOTS('',3,(#117300,#117301,#117302,#117303,
#117304,#117305),.UNSPECIFIED.,.F.,.F.,(4,2,4),(0.,0.5,1.),
 .UNSPECIFIED.);
#29573=B_SPLINE_CURVE_WITH_KNOTS('',3,(#117306,#117307,#117308,#117309,
#117310,#117311,#117312,#117313,#117314,#117315,#117316,#117317,#117318,
#117319,#117320,#117321,#117322,#117323,#117324,#117325,#117326,#117327,
#117328,#117329,#117330,#117331,#117332,#117333,#117334,#117335,#117336,
#117337,#117338,#117339,#117340,#117341,#117342,#117343,#117344,#117345,
#117346,#117347,#117348,#117349,#117350,#117351,#117352,#117353,#117354),
 .UNSPECIFIED.,.F.,.F.,(4,3,3,3,3,3,3,3,3,3,3,3,3,3,3,3,4),(0.,0.0659495801766569,
0.1308373231871,0.19438095135116,0.25,0.3125,0.374042589957,0.435265209100815,
0.496321655486699,0.559741241615024,0.621102771689104,0.685551385844552,
0.75,0.813619167758251,0.87800524330354,0.944005251946419,1.),
 .UNSPECIFIED.);
#29574=B_SPLINE_CURVE_WITH_KNOTS('',3,(#117363,#117364,#117365,#117366,
#117367,#117368),.UNSPECIFIED.,.F.,.F.,(4,2,4),(1.00000000968122E-6,0.267925099545075,
0.535347184622059),.UNSPECIFIED.);
#29575=B_SPLINE_CURVE_WITH_KNOTS('',3,(#117418,#117419,#117420,#117421,
#117422,#117423,#117424,#117425,#117426,#117427,#117428,#117429,#117430,
#117431,#117432,#117433,#117434,#117435,#117436,#117437,#117438,#117439,
#117440,#117441,#117442,#117443,#117444,#117445,#117446,#117447,#117448,
#117449,#117450,#117451,#117452,#117453,#117454,#117455,#117456,#117457,
#117458,#117459,#117460,#117461,#117462,#117463,#117464,#117465,#117466,
#117467,#117468,#117469,#117470,#117471,#117472,#117473,#117474,#117475,
#117476,#117477,#117478,#117479,#117480,#117481,#117482,#117483,#117484,
#117485,#117486,#117487),.UNSPECIFIED.,.F.,.F.,(4,3,3,3,3,3,3,3,3,3,3,3,
3,3,3,3,3,3,3,3,3,3,3,4),(0.,0.11048788577789,0.124999999999995,0.201428248706923,
0.218749999999992,0.235851895407793,0.249999999999992,0.312861916977878,
0.386450511607397,0.437499999999996,0.464170261187618,0.490703896049709,
0.499999999999997,0.514209169182011,0.578362302765488,0.624999999999998,
0.673321561493809,0.714910737311328,0.749999999999999,0.807840811261223,
0.869314910339536,0.914553166950376,0.969583186255868,0.999999999703888),
 .UNSPECIFIED.);
#29576=B_SPLINE_CURVE_WITH_KNOTS('',3,(#117491,#117492,#117493,#117494,
#117495,#117496,#117497,#117498,#117499,#117500,#117501,#117502),
 .UNSPECIFIED.,.F.,.F.,(4,2,2,2,2,4),(-0.486148537655684,-0.486124291092022,
-0.428314815488407,-0.370505339884792,-0.308168734459638,-0.245832129034485),
 .UNSPECIFIED.);
#29577=B_SPLINE_CURVE_WITH_KNOTS('',3,(#117513,#117514,#117515,#117516,
#117517,#117518,#117519,#117520,#117521,#117522),.UNSPECIFIED.,.F.,.F.,
(4,2,2,2,4),(-0.231634949000231,-0.17437767996901,-0.115937607104994,-0.0533819428831184,
-9.99999772544058E-7),.UNSPECIFIED.);
#29578=B_SPLINE_CURVE_WITH_KNOTS('',3,(#117523,#117524,#117525,#117526,
#117527,#117528,#117529,#117530,#117531,#117532),.UNSPECIFIED.,.F.,.F.,
(4,3,3,4),(3.09320682459972E-12,0.485988696847241,0.738935319808724,1.),
 .UNSPECIFIED.);
#29579=B_SPLINE_CURVE_WITH_KNOTS('',3,(#117533,#117534,#117535,#117536,
#117537,#117538,#117539),.UNSPECIFIED.,.F.,.F.,(4,3,4),(0.,0.734307685730172,
1.),.UNSPECIFIED.);
#29580=B_SPLINE_CURVE_WITH_KNOTS('',3,(#117600,#117601,#117602,#117603,
#117604,#117605,#117606),.UNSPECIFIED.,.F.,.F.,(4,3,4),(0.,0.1,0.126954494999424),
 .UNSPECIFIED.);
#29581=B_SPLINE_CURVE_WITH_KNOTS('',3,(#117681,#117682,#117683,#117684,
#117685,#117686,#117687,#117688,#117689,#117690,#117691,#117692,#117693,
#117694,#117695,#117696,#117697,#117698,#117699,#117700,#117701,#117702,
#117703,#117704,#117705,#117706,#117707,#117708,#117709,#117710,#117711,
#117712,#117713,#117714,#117715,#117716,#117717,#117718,#117719,#117720,
#117721,#117722,#117723,#117724,#117725,#117726,#117727,#117728,#117729,
#117730,#117731,#117732,#117733,#117734,#117735,#117736,#117737,#117738,
#117739,#117740,#117741,#117742,#117743,#117744,#117745,#117746,#117747,
#117748,#117749,#117750,#117751,#117752,#117753,#117754,#117755,#117756,
#117757,#117758,#117759,#117760,#117761,#117762,#117763,#117764,#117765,
#117766,#117767,#117768,#117769,#117770,#117771,#117772,#117773,#117774),
 .UNSPECIFIED.,.F.,.F.,(4,3,3,3,3,3,3,3,3,3,3,3,3,3,3,3,3,3,3,3,3,3,3,3,
3,3,3,3,3,3,3,4),(0.,0.0434329855669776,0.08907548745578,0.0992782405803121,
0.1111111111111,0.150652206158072,0.189763811698692,0.216719719165669,0.2222222222222,
0.27777777777775,0.328951791908699,0.3333333333333,0.33411341030855,0.367911781436324,
0.401192650050171,0.43352701848881,0.4444444444444,0.451268763306688,0.494769905150912,
0.536743026897841,0.5555555555556,0.568707898163555,0.617687282415127,0.6666666666667,
0.686226797860462,0.73658037633076,0.7777777777778,0.803542347385094,0.85501524701251,
0.8888888888889,0.920843304974927,0.999999999998517),.UNSPECIFIED.);
#29582=B_SPLINE_CURVE_WITH_KNOTS('',3,(#117777,#117778,#117779,#117780,
#117781,#117782,#117783,#117784,#117785,#117786,#117787,#117788,#117789,
#117790,#117791,#117792,#117793,#117794,#117795,#117796,#117797,#117798,
#117799,#117800,#117801,#117802,#117803,#117804,#117805,#117806,#117807,
#117808,#117809,#117810,#117811,#117812,#117813,#117814,#117815,#117816,
#117817,#117818,#117819,#117820,#117821,#117822,#117823,#117824,#117825,
#117826,#117827,#117828,#117829,#117830,#117831,#117832,#117833,#117834,
#117835,#117836,#117837,#117838,#117839,#117840,#117841,#117842,#117843,
#117844,#117845,#117846,#117847,#117848,#117849,#117850,#117851,#117852,
#117853,#117854,#117855,#117856,#117857,#117858,#117859,#117860,#117861,
#117862,#117863,#117864,#117865,#117866,#117867,#117868,#117869,#117870,
#117871,#117872,#117873,#117874,#117875,#117876),.UNSPECIFIED.,.F.,.F.,
(4,3,3,3,3,3,3,3,3,3,3,3,3,3,3,3,3,3,3,3,3,3,3,3,3,3,3,3,3,3,3,3,3,4),(0.,
0.0482896592338093,0.102692540909445,0.136650408423194,0.190645379027607,
0.225179914594825,0.25000000000002,0.304085285007251,0.313864436259833,
0.365917320127364,0.375000000000032,0.402681143263378,0.437500000000037,
0.468750000000041,0.484375000000044,0.492187500000046,0.492692625002022,
0.496093750000046,0.498046875000046,0.500000000000047,0.536325374785433,
0.569651731954972,0.606130649818242,0.644147897050678,0.647285809980453,
0.686930286977043,0.724488661589305,0.750000000000023,0.802797594861853,
0.809964462253265,0.867077701254393,0.908266360714621,0.975423950021811,
0.99999999995535),.UNSPECIFIED.);
#29583=B_SPLINE_CURVE_WITH_KNOTS('',3,(#117914,#117915,#117916,#117917,
#117918,#117919,#117920,#117921),.UNSPECIFIED.,.F.,.F.,(4,1,1,1,1,4),(2.28402671907889E-6,
0.2,0.4,0.6,0.8,1.),.UNSPECIFIED.);
#29584=B_SPLINE_CURVE_WITH_KNOTS('',3,(#117924,#117925,#117926,#117927,
#117928,#117929,#117930,#117931,#117932,#117933,#117934,#117935,#117936,
#117937,#117938,#117939,#117940,#117941,#117942,#117943,#117944,#117945,
#117946,#117947,#117948),.UNSPECIFIED.,.F.,.F.,(4,3,3,3,3,3,3,3,4),(2.23348816774046E-5,
0.0628477441748189,0.220194717015139,0.373526365176584,0.524161382659806,
0.670551898649584,0.744053228789804,0.90146949799915,1.),.UNSPECIFIED.);
#29585=B_SPLINE_CURVE_WITH_KNOTS('',3,(#118019,#118020,#118021,#118022,
#118023,#118024,#118025,#118026,#118027,#118028,#118029,#118030,#118031,
#118032,#118033,#118034,#118035,#118036,#118037,#118038,#118039,#118040,
#118041,#118042,#118043,#118044,#118045,#118046,#118047,#118048,#118049,
#118050,#118051,#118052,#118053,#118054,#118055,#118056,#118057,#118058,
#118059,#118060,#118061,#118062,#118063,#118064,#118065,#118066,#118067,
#118068,#118069,#118070,#118071,#118072,#118073,#118074,#118075,#118076,
#118077,#118078,#118079,#118080,#118081,#118082,#118083,#118084,#118085,
#118086,#118087,#118088,#118089,#118090,#118091,#118092,#118093,#118094,
#118095,#118096,#118097,#118098,#118099,#118100,#118101,#118102,#118103,
#118104,#118105,#118106,#118107,#118108,#118109,#118110,#118111,#118112,
#118113,#118114,#118115,#118116,#118117,#118118,#118119,#118120,#118121,
#118122,#118123,#118124,#118125,#118126,#118127,#118128,#118129,#118130,
#118131,#118132,#118133,#118134,#118135,#118136,#118137,#118138,#118139,
#118140,#118141,#118142,#118143,#118144,#118145,#118146,#118147,#118148,
#118149,#118150,#118151,#118152,#118153,#118154,#118155,#118156,#118157,
#118158,#118159,#118160,#118161,#118162,#118163,#118164,#118165,#118166,
#118167,#118168,#118169,#118170,#118171,#118172,#118173,#118174,#118175,
#118176,#118177,#118178,#118179,#118180,#118181,#118182,#118183,#118184,
#118185,#118186,#118187,#118188,#118189,#118190,#118191,#118192,#118193,
#118194,#118195,#118196),.UNSPECIFIED.,.F.,.F.,(4,3,3,3,3,3,3,3,3,3,3,3,
3,3,3,3,3,3,3,3,3,3,3,3,3,3,3,3,3,3,3,3,3,3,3,3,3,3,3,3,3,3,3,3,3,3,3,3,
3,3,3,3,3,3,3,3,3,3,3,4),(0.,0.0488641282796294,0.104159161587302,0.123022321598326,
0.124999999999995,0.179678682731705,0.187499999999992,0.197853928883569,
0.21874999999999,0.234374999999989,0.242187499999989,0.248089771096223,
0.249999999999988,0.274414806619095,0.332705726838955,0.351483832875215,
0.410368538967155,0.425145513293437,0.437499999999992,0.468749999999993,
0.484374999999992,0.492187499999991,0.496093749999991,0.496290295252264,
0.499999999999991,0.543327592310242,0.570763138693585,0.613636521352308,
0.644189079608782,0.685332797437125,0.68749999999999,0.718749999999989,
0.718953363471053,0.73437499999999,0.742187499999989,0.746093749999989,
0.748046874999988,0.749023437499988,0.749999999999988,0.769489339732673,
0.789169556834021,0.801427018275548,0.821475974402478,0.841466221066801,
0.859375000000003,0.867187500000004,0.869582291779894,0.871093750000004,
0.873046875000005,0.874023437500005,0.875000000000005,0.890106498209821,
0.905512726506942,0.921370222932082,0.930397372833373,0.937500000000002,
0.954034229226621,0.970837951409062,0.988025978151,1.),.UNSPECIFIED.);
#29586=B_SPLINE_CURVE_WITH_KNOTS('',3,(#118240,#118241,#118242,#118243,
#118244,#118245,#118246,#118247,#118248,#118249,#118250,#118251,#118252,
#118253,#118254,#118255,#118256,#118257,#118258,#118259,#118260,#118261,
#118262,#118263,#118264,#118265,#118266,#118267,#118268,#118269,#118270,
#118271,#118272,#118273,#118274,#118275,#118276,#118277,#118278,#118279,
#118280,#118281,#118282,#118283,#118284,#118285,#118286,#118287,#118288,
#118289,#118290,#118291,#118292,#118293,#118294,#118295,#118296,#118297,
#118298,#118299,#118300,#118301,#118302,#118303,#118304,#118305,#118306,
#118307,#118308,#118309),.UNSPECIFIED.,.F.,.F.,(4,3,3,3,3,3,3,3,3,3,3,3,
3,3,3,3,3,3,3,3,3,3,3,4),(2.33665370772347E-6,0.0496371691506646,0.0994512751400878,
0.12500000000005,0.17474957176903,0.187500000000073,0.218750000000083,0.234375000000087,
0.24218750000009,0.249493988611268,0.250000000000093,0.304451733242835,
0.359731547709945,0.416068672295921,0.43224145509044,0.437500000000231,
0.468750000000251,0.484375000000263,0.492187500000273,0.496093750000274,
0.498046875000272,0.50000000000027,0.956286239664588,0.999999847835327),
 .UNSPECIFIED.);
#29587=B_SPLINE_CURVE_WITH_KNOTS('',3,(#118364,#118365,#118366,#118367,
#118368,#118369,#118370,#118371,#118372,#118373,#118374,#118375,#118376,
#118377,#118378,#118379,#118380,#118381,#118382,#118383,#118384,#118385,
#118386,#118387,#118388,#118389,#118390,#118391,#118392,#118393,#118394,
#118395,#118396,#118397,#118398,#118399,#118400,#118401,#118402,#118403,
#118404,#118405,#118406,#118407,#118408,#118409,#118410,#118411,#118412,
#118413,#118414,#118415,#118416,#118417,#118418,#118419,#118420,#118421,
#118422,#118423,#118424,#118425,#118426,#118427,#118428,#118429,#118430,
#118431,#118432,#118433,#118434,#118435,#118436,#118437,#118438,#118439,
#118440,#118441,#118442,#118443,#118444,#118445,#118446,#118447,#118448,
#118449,#118450,#118451,#118452,#118453,#118454,#118455,#118456,#118457,
#118458,#118459,#118460,#118461,#118462,#118463,#118464,#118465,#118466,
#118467,#118468,#118469,#118470,#118471,#118472,#118473,#118474,#118475,
#118476,#118477,#118478,#118479,#118480,#118481,#118482,#118483,#118484,
#118485,#118486,#118487,#118488,#118489,#118490,#118491,#118492,#118493,
#118494,#118495,#118496,#118497,#118498,#118499,#118500,#118501,#118502,
#118503,#118504,#118505,#118506,#118507,#118508,#118509,#118510,#118511,
#118512,#118513,#118514,#118515,#118516,#118517,#118518,#118519,#118520,
#118521,#118522,#118523,#118524,#118525,#118526,#118527,#118528,#118529,
#118530,#118531,#118532,#118533,#118534,#118535,#118536,#118537,#118538),
 .UNSPECIFIED.,.F.,.F.,(4,3,3,3,3,3,3,3,3,3,3,3,3,3,3,3,3,3,3,3,3,3,3,3,
3,3,3,3,3,3,3,3,3,3,3,3,3,3,3,3,3,3,3,3,3,3,3,3,3,3,3,3,3,3,3,3,3,3,4),
(0.,0.0555382977619952,0.0624999999999407,0.0692575826362369,0.0937499999999123,
0.109374999999899,0.117187499999892,0.121093749999889,0.124023437499886,
0.124999999999885,0.144081499360291,0.163253233995527,0.171874999999873,
0.179028327204326,0.179687499999871,0.185657163721033,0.187499999999869,
0.211416108967977,0.218749999999859,0.234374999999853,0.24218749999985,
0.246093749999849,0.248046874999848,0.249999999999847,0.283186761764929,
0.322905151422521,0.343749999999848,0.359374999999848,0.367187499999848,
0.373100637420652,0.374999999999848,0.394064544065694,0.437499999999848,
0.468749999999848,0.484374999999849,0.492187499999849,0.49609374999985,
0.499384498321497,0.49999999999985,0.501066362102164,0.554831394622692,
0.608443932593253,0.659742424080655,0.709573207920356,0.716593188313347,
0.718749999999909,0.734374999999914,0.742187499999916,0.746093749999917,
0.748046874999918,0.749999999999918,0.793255601342627,0.81956640435806,
0.858098769840019,0.897160626316328,0.929164183156927,0.961210686803325,
0.993512835337006,1.),.UNSPECIFIED.);
#29588=B_SPLINE_CURVE_WITH_KNOTS('',3,(#118544,#118545,#118546,#118547,
#118548,#118549,#118550,#118551,#118552,#118553,#118554,#118555,#118556,
#118557,#118558,#118559,#118560,#118561,#118562,#118563,#118564,#118565,
#118566,#118567,#118568,#118569,#118570,#118571,#118572,#118573,#118574,
#118575,#118576,#118577,#118578,#118579,#118580,#118581,#118582,#118583,
#118584,#118585,#118586,#118587,#118588,#118589,#118590,#118591,#118592,
#118593,#118594,#118595,#118596,#118597,#118598,#118599,#118600,#118601,
#118602,#118603,#118604,#118605,#118606,#118607,#118608,#118609,#118610,
#118611,#118612,#118613,#118614,#118615,#118616,#118617,#118618,#118619,
#118620,#118621,#118622,#118623,#118624,#118625,#118626,#118627,#118628,
#118629,#118630,#118631),.UNSPECIFIED.,.F.,.F.,(4,3,3,3,3,3,3,3,3,3,3,3,
3,3,3,3,3,3,3,3,3,3,3,3,3,3,3,3,3,4),(3.36783202418071E-7,0.0704310134426517,
0.154324908618331,0.178703893197204,0.250000000000081,0.291512562001931,
0.375000000000122,0.399673169085418,0.437500000000142,0.468750000000152,
0.484375000000157,0.492187500000159,0.499023437500161,0.500000000000161,
0.501549258011091,0.5461457214218,0.59050184840333,0.63104355844614,0.67441742482806,
0.717108969540505,0.739637705241223,0.75000000000008,0.791454313031361,
0.832044716531103,0.843349397267229,0.87500000000004,0.916301019532102,
0.942758457577564,0.976122915483621,1.),.UNSPECIFIED.);
#29589=B_SPLINE_CURVE_WITH_KNOTS('',3,(#118721,#118722,#118723,#118724,
#118725,#118726,#118727,#118728,#118729,#118730,#118731,#118732,#118733,
#118734,#118735,#118736,#118737,#118738,#118739,#118740,#118741,#118742,
#118743,#118744,#118745,#118746,#118747,#118748,#118749,#118750,#118751,
#118752,#118753,#118754,#118755,#118756,#118757,#118758,#118759,#118760,
#118761,#118762,#118763,#118764,#118765,#118766,#118767,#118768,#118769,
#118770,#118771,#118772,#118773,#118774,#118775),.UNSPECIFIED.,.F.,.F.,
(4,3,3,3,3,3,3,3,3,3,3,3,3,3,3,3,3,3,4),(0.,0.0682759325374089,0.154250463005588,
0.238795938723332,0.250000000000005,0.332839120626675,0.346908656220202,
0.430143950681296,0.437500000000009,0.46875000000001,0.48437500000001,0.49218750000001,
0.498046875000011,0.500000000000011,0.634899028144559,0.670690163863966,
0.802255340146405,0.929676150621539,1.),.UNSPECIFIED.);
#29590=B_SPLINE_CURVE_WITH_KNOTS('',3,(#118776,#118777,#118778,#118779,
#118780,#118781,#118782,#118783,#118784,#118785,#118786,#118787,#118788,
#118789,#118790,#118791,#118792,#118793,#118794,#118795,#118796,#118797,
#118798,#118799,#118800,#118801,#118802,#118803,#118804,#118805,#118806,
#118807,#118808,#118809,#118810,#118811,#118812,#118813,#118814,#118815,
#118816,#118817,#118818,#118819,#118820,#118821,#118822,#118823,#118824,
#118825,#118826,#118827,#118828,#118829,#118830,#118831,#118832,#118833,
#118834,#118835,#118836,#118837,#118838,#118839,#118840,#118841,#118842,
#118843,#118844,#118845,#118846,#118847,#118848,#118849,#118850,#118851,
#118852,#118853,#118854,#118855,#118856,#118857,#118858,#118859,#118860,
#118861,#118862,#118863,#118864,#118865,#118866,#118867,#118868,#118869,
#118870,#118871,#118872,#118873,#118874,#118875,#118876,#118877,#118878,
#118879,#118880,#118881,#118882,#118883,#118884,#118885,#118886,#118887,
#118888,#118889,#118890,#118891,#118892,#118893,#118894,#118895,#118896,
#118897,#118898,#118899,#118900,#118901,#118902,#118903,#118904,#118905,
#118906,#118907,#118908,#118909,#118910,#118911,#118912,#118913,#118914,
#118915,#118916,#118917,#118918,#118919,#118920,#118921,#118922,#118923,
#118924,#118925,#118926,#118927,#118928,#118929,#118930,#118931,#118932,
#118933,#118934,#118935,#118936,#118937,#118938,#118939,#118940,#118941,
#118942,#118943,#118944,#118945,#118946,#118947,#118948,#118949,#118950,
#118951,#118952,#118953),.UNSPECIFIED.,.F.,.F.,(4,3,3,3,3,3,3,3,3,3,3,3,
3,3,3,3,3,3,3,3,3,3,3,3,3,3,3,3,3,3,3,3,3,3,3,3,3,3,3,3,3,3,3,3,3,3,3,3,
3,3,3,3,3,3,3,3,3,3,3,4),(0.,0.0457546736928399,0.0595877683597098,0.0625000000000001,
0.0937500000000003,0.109375,0.1171875,0.123526663010336,0.125,0.154802074788136,
0.192739789732303,0.230157223808861,0.249999999999998,0.251214518677982,
0.294717106205779,0.33793097163504,0.347765493387925,0.374999999999996,
0.390624999999996,0.398926310167048,0.406249999999995,0.437499999999994,
0.443749474057719,0.468749999999993,0.484374999999993,0.492187499999993,
0.497995340860155,0.499999999999993,0.535787989099162,0.56249999999999,
0.593749999999989,0.609374999999989,0.617187499999989,0.624023437499989,
0.624999999999989,0.632640348092497,0.667465916356947,0.687499999999993,
0.718749999999994,0.727500196920872,0.734374999999995,0.742187499999996,
0.749023437499996,0.749999999999996,0.779007516334961,0.808104573985199,
0.812499999999994,0.822012805932175,0.843749999999993,0.859374999999993,
0.867187499999992,0.871093749999992,0.874023437499992,0.874999999999992,
0.899004394474957,0.917844380165313,0.941858795920938,0.965884596741871,
0.989772975332555,1.),.UNSPECIFIED.);
#29591=B_SPLINE_CURVE_WITH_KNOTS('',3,(#118972,#118973,#118974,#118975),
 .UNSPECIFIED.,.F.,.F.,(4,4),(0.,1.),.UNSPECIFIED.);
#29592=B_SPLINE_CURVE_WITH_KNOTS('',3,(#119063,#119064,#119065,#119066,
#119067,#119068,#119069,#119070,#119071,#119072,#119073,#119074,#119075,
#119076,#119077,#119078,#119079,#119080,#119081,#119082,#119083,#119084,
#119085,#119086,#119087,#119088,#119089,#119090,#119091,#119092,#119093,
#119094,#119095,#119096,#119097,#119098,#119099,#119100,#119101,#119102,
#119103,#119104,#119105,#119106,#119107,#119108,#119109,#119110,#119111,
#119112,#119113,#119114,#119115,#119116,#119117,#119118,#119119,#119120,
#119121,#119122,#119123,#119124,#119125,#119126,#119127,#119128,#119129,
#119130,#119131,#119132,#119133,#119134,#119135,#119136,#119137,#119138,
#119139,#119140,#119141,#119142,#119143,#119144,#119145,#119146,#119147,
#119148,#119149,#119150,#119151,#119152,#119153,#119154,#119155,#119156,
#119157,#119158,#119159,#119160,#119161,#119162,#119163,#119164,#119165),
 .UNSPECIFIED.,.F.,.F.,(4,3,3,3,3,3,3,3,3,3,3,3,3,3,3,3,3,3,3,3,3,3,3,3,
3,3,3,3,3,3,3,3,3,3,4),(0.,0.067563816995275,0.130591467722512,0.181054213924464,
0.236634402691202,0.288380007132738,0.306370007127845,0.354266716525829,
0.399092160822195,0.402163425923814,0.44373159496594,0.468750000000269,
0.478404816342543,0.484375000000277,0.492187500000285,0.496093750000291,
0.498046875000291,0.500000000000291,0.544044020950823,0.564564733044594,
0.605001389397497,0.642763780545731,0.680551013373682,0.687500000000175,
0.706851062819798,0.71038379496846,0.730191897484299,0.750000000000139,
0.783679309806148,0.837365834608666,0.863499857353213,0.912275470648177,
0.95177477806762,0.995440622620178,1.),.UNSPECIFIED.);
#29593=B_SPLINE_CURVE_WITH_KNOTS('',3,(#119166,#119167,#119168,#119169,
#119170,#119171,#119172,#119173,#119174,#119175,#119176,#119177,#119178,
#119179,#119180,#119181,#119182,#119183,#119184,#119185,#119186,#119187,
#119188,#119189,#119190,#119191,#119192,#119193,#119194,#119195,#119196,
#119197,#119198,#119199,#119200,#119201,#119202,#119203,#119204,#119205,
#119206,#119207,#119208,#119209,#119210,#119211,#119212,#119213,#119214,
#119215,#119216,#119217,#119218,#119219,#119220,#119221,#119222,#119223,
#119224,#119225,#119226,#119227,#119228,#119229,#119230,#119231,#119232,
#119233,#119234,#119235,#119236,#119237,#119238,#119239,#119240,#119241,
#119242,#119243,#119244,#119245,#119246,#119247,#119248,#119249,#119250,
#119251,#119252,#119253,#119254,#119255,#119256,#119257,#119258,#119259,
#119260,#119261,#119262,#119263,#119264,#119265,#119266,#119267,#119268),
 .UNSPECIFIED.,.F.,.F.,(4,3,3,3,3,3,3,3,3,3,3,3,3,3,3,3,3,3,3,3,3,3,3,3,
3,3,3,3,3,3,3,3,3,3,4),(0.,0.0501535530149427,0.0843408069737685,0.125000000000027,
0.16757754732749,0.179135824507627,0.187500000000039,0.218750000000045,
0.234375000000044,0.242187500000042,0.248359381055688,0.250000000000041,
0.285533837129323,0.346076131737884,0.374999999999979,0.380522902976463,
0.437499999999947,0.468749999999931,0.474795911141055,0.484374999999925,
0.492187499999923,0.496093749999925,0.499999999999927,0.553255897370739,
0.603065113704012,0.627088768202908,0.675665818704117,0.707465524125276,
0.749999999999963,0.80466568180373,0.85475077335072,0.910734288428706,0.926422203511138,
0.978719943194182,1.),.UNSPECIFIED.);
#29594=B_SPLINE_CURVE_WITH_KNOTS('',3,(#119340,#119341,#119342,#119343,
#119344,#119345,#119346,#119347,#119348,#119349,#119350,#119351,#119352,
#119353,#119354,#119355),.UNSPECIFIED.,.F.,.F.,(4,3,3,3,3,4),(1.44815538111642E-5,
0.210256084640174,0.423632741635552,0.639251052850045,0.859563807440021,
0.999999999994534),.UNSPECIFIED.);
#29595=B_SPLINE_CURVE_WITH_KNOTS('',3,(#119422,#119423,#119424,#119425,
#119426,#119427,#119428,#119429,#119430,#119431,#119432,#119433,#119434,
#119435,#119436,#119437,#119438,#119439,#119440,#119441,#119442,#119443,
#119444,#119445,#119446,#119447,#119448,#119449,#119450,#119451,#119452,
#119453,#119454,#119455,#119456,#119457,#119458,#119459,#119460,#119461,
#119462,#119463,#119464,#119465,#119466,#119467,#119468,#119469,#119470,
#119471,#119472,#119473,#119474,#119475,#119476,#119477,#119478,#119479,
#119480,#119481,#119482,#119483,#119484,#119485,#119486,#119487,#119488),
 .UNSPECIFIED.,.F.,.F.,(4,3,3,3,3,3,3,3,3,3,3,3,3,3,3,3,3,3,3,3,3,3,4),
(2.0903552712953E-10,0.0302476823861621,0.0946324368287587,0.162216233220878,
0.18810280752984,0.250000000000002,0.328856575995871,0.390941197142464,
0.453025818289058,0.468750000000002,0.484375000000002,0.492187500000003,
0.496093750000003,0.498046875000003,0.500000000000004,0.585458270036095,
0.655183530447372,0.72490879085865,0.750000000000002,0.861552612219485,
0.906217681176828,0.953108840588414,1.),.UNSPECIFIED.);
#29596=B_SPLINE_CURVE_WITH_KNOTS('',3,(#119499,#119500,#119501,#119502,
#119503,#119504,#119505,#119506,#119507,#119508,#119509,#119510,#119511,
#119512,#119513,#119514,#119515,#119516,#119517,#119518,#119519,#119520,
#119521,#119522,#119523,#119524,#119525,#119526,#119527,#119528,#119529,
#119530,#119531,#119532,#119533,#119534,#119535,#119536,#119537,#119538,
#119539,#119540,#119541,#119542,#119543,#119544,#119545,#119546,#119547,
#119548,#119549,#119550,#119551,#119552,#119553,#119554,#119555,#119556,
#119557,#119558,#119559,#119560,#119561,#119562,#119563,#119564,#119565,
#119566,#119567,#119568,#119569,#119570,#119571,#119572,#119573,#119574,
#119575,#119576,#119577,#119578,#119579,#119580,#119581,#119582,#119583,
#119584,#119585,#119586,#119587,#119588,#119589,#119590,#119591,#119592,
#119593,#119594,#119595,#119596,#119597,#119598,#119599,#119600,#119601,
#119602,#119603,#119604,#119605,#119606,#119607,#119608,#119609,#119610,
#119611,#119612,#119613,#119614,#119615,#119616,#119617,#119618,#119619,
#119620,#119621,#119622),.UNSPECIFIED.,.F.,.F.,(4,3,3,3,3,3,3,3,3,3,3,3,
3,3,3,3,3,3,3,3,3,3,3,3,3,3,3,3,3,3,3,3,3,3,3,3,3,3,3,3,3,4),(1.06186481877749E-15,
0.0340851358066496,0.0691999299672166,0.105785020111385,0.117362581696846,
0.125000000000004,0.160169392187649,0.187500000000007,0.218750000000008,
0.234375000000009,0.242187500000011,0.246093750000011,0.250000000000011,
0.285437709422724,0.309021567011856,0.343532732159649,0.37857221360227,
0.413947095861862,0.449222909696327,0.483968840156166,0.500000000000016,
0.500003316435609,0.534824037905456,0.570002504688142,0.605300892498013,
0.625000000000019,0.659693858326166,0.68750000000002,0.691017683145083,
0.718750000000021,0.734375000000022,0.742187500000022,0.746093750000022,
0.750000000000022,0.787161509091454,0.823722624830958,0.859049261837564,
0.882626506205646,0.918399913913295,0.953209132777543,0.986561655878065,
1.),.UNSPECIFIED.);
#29597=B_SPLINE_CURVE_WITH_KNOTS('',3,(#119626,#119627,#119628,#119629,
#119630,#119631,#119632,#119633,#119634,#119635,#119636,#119637,#119638,
#119639,#119640,#119641,#119642,#119643,#119644,#119645,#119646,#119647),
 .UNSPECIFIED.,.F.,.F.,(4,3,3,3,3,3,3,4),(4.08364197003503E-10,0.250000000000007,
0.375000000000007,0.437500000000006,0.496331466076166,0.500000000000005,
0.753785934071933,0.999999999974308),.UNSPECIFIED.);
#29598=B_SPLINE_CURVE_WITH_KNOTS('',3,(#119651,#119652,#119653,#119654,
#119655,#119656,#119657,#119658,#119659,#119660,#119661,#119662,#119663,
#119664,#119665,#119666,#119667,#119668,#119669,#119670,#119671,#119672,
#119673,#119674,#119675,#119676,#119677,#119678,#119679,#119680,#119681,
#119682,#119683,#119684,#119685,#119686,#119687,#119688,#119689,#119690,
#119691,#119692,#119693,#119694,#119695,#119696,#119697,#119698,#119699,
#119700,#119701,#119702,#119703,#119704,#119705,#119706,#119707,#119708,
#119709,#119710,#119711,#119712,#119713,#119714,#119715,#119716,#119717,
#119718,#119719,#119720,#119721,#119722,#119723,#119724,#119725,#119726,
#119727,#119728,#119729,#119730,#119731,#119732,#119733,#119734,#119735,
#119736,#119737,#119738,#119739,#119740,#119741,#119742,#119743,#119744,
#119745,#119746,#119747,#119748,#119749,#119750,#119751,#119752,#119753,
#119754,#119755,#119756,#119757,#119758,#119759,#119760,#119761,#119762,
#119763,#119764,#119765,#119766,#119767,#119768),.UNSPECIFIED.,.F.,.F.,
(4,3,3,3,3,3,3,3,3,3,3,3,3,3,3,3,3,3,3,3,3,3,3,3,3,3,3,3,3,3,3,3,3,3,3,
3,3,3,3,4),(0.,0.0271623998492999,0.0553322026502384,0.0841874376300376,
0.113763564313068,0.144091135811689,0.175190924106879,0.207067488782461,
0.240096712177752,0.273752683323411,0.30795455313194,0.342604883632704,
0.377744298735794,0.413067078246304,0.448574733468898,0.468749999999997,
0.484374999999999,0.492187499999999,0.49883613893283,0.5,0.537434732927738,
0.574951049695804,0.611904861516709,0.649702430758356,0.687500000000003,
0.697178248398173,0.703125000000003,0.718750000000002,0.750000000000002,
0.784381124832368,0.81809272813315,0.850771307730581,0.875000000000004,
0.890625000000004,0.898437500000004,0.904724710564298,0.906250000000003,
0.937500000000002,0.980487098276565,1.),.UNSPECIFIED.);
#29599=B_SPLINE_CURVE_WITH_KNOTS('',3,(#119772,#119773,#119774,#119775,
#119776,#119777,#119778,#119779,#119780,#119781,#119782,#119783,#119784,
#119785,#119786,#119787,#119788,#119789,#119790,#119791,#119792,#119793,
#119794,#119795,#119796,#119797,#119798,#119799,#119800,#119801,#119802),
 .UNSPECIFIED.,.F.,.F.,(4,3,3,3,3,3,3,3,3,3,4),(1.10824284158061E-6,0.249999999999966,
0.374999999999952,0.43749999999995,0.468749999999949,0.484374999999949,
0.496093749999949,0.499999999999948,0.719932202069709,0.941144134881108,
1.),.UNSPECIFIED.);
#29600=B_SPLINE_CURVE_WITH_KNOTS('',3,(#119806,#119807,#119808,#119809,
#119810,#119811,#119812,#119813,#119814,#119815,#119816,#119817,#119818,
#119819),.UNSPECIFIED.,.F.,.F.,(4,2,2,1,1,2,2,4),(0.,0.250000000000008,
0.375000000000012,0.437500000000012,0.468750000000011,0.484375000000011,
0.500000000000012,0.999999993863129),.UNSPECIFIED.);
#29601=B_SPLINE_CURVE_WITH_KNOTS('',3,(#119820,#119821,#119822,#119823,
#119824,#119825,#119826,#119827,#119828,#119829,#119830,#119831,#119832,
#119833),.UNSPECIFIED.,.F.,.F.,(4,2,2,1,1,2,2,4),(0.,0.249999999999992,
0.374999999999991,0.43749999999999,0.468749999999991,0.484374999999992,
0.499999999999993,1.),.UNSPECIFIED.);
#29602=B_SPLINE_CURVE_WITH_KNOTS('',3,(#119873,#119874,#119875,#119876,
#119877,#119878,#119879,#119880,#119881,#119882,#119883,#119884,#119885,
#119886,#119887,#119888,#119889,#119890,#119891,#119892,#119893,#119894,
#119895,#119896,#119897,#119898,#119899,#119900,#119901,#119902,#119903,
#119904,#119905,#119906,#119907,#119908,#119909,#119910,#119911,#119912),
 .UNSPECIFIED.,.F.,.F.,(4,3,3,3,3,3,3,3,3,3,3,3,3,4),(0.,0.0829435186321783,
0.16544324384915,0.247585715556801,0.329456585306884,0.413274512143524,
0.494872951961396,0.576482179278369,0.65817673585635,0.743632551892263,
0.825892623948683,0.908430785310346,0.991464788229984,1.),.UNSPECIFIED.);
#29603=B_SPLINE_CURVE_WITH_KNOTS('',3,(#119914,#119915,#119916,#119917,
#119918,#119919,#119920,#119921,#119922,#119923),.UNSPECIFIED.,.F.,.F.,
(4,2,2,2,4),(0.,0.25,0.5,0.75,1.),.UNSPECIFIED.);
#29604=B_SPLINE_CURVE_WITH_KNOTS('',3,(#119924,#119925,#119926,#119927,
#119928,#119929,#119930,#119931,#119932,#119933,#119934,#119935,#119936,
#119937,#119938,#119939,#119940,#119941,#119942,#119943,#119944,#119945,
#119946,#119947,#119948),.UNSPECIFIED.,.F.,.F.,(4,2,2,2,2,2,2,1,1,1,2,2,
2,4),(1.36445938018877E-7,0.124999999999883,0.187499999999825,0.249999999999766,
0.374999999999658,0.437499999999601,0.468749999999574,0.484374999999559,
0.492187499999552,0.496093749999551,0.498046874999548,0.499999999999545,
0.749999999999773,1.),.UNSPECIFIED.);
#29605=B_SPLINE_CURVE_WITH_KNOTS('',3,(#119975,#119976,#119977,#119978,
#119979,#119980,#119981,#119982,#119983,#119984,#119985),.UNSPECIFIED.,
 .F.,.F.,(4,1,1,1,1,1,1,1,4),(0.,0.125,0.25,0.375,0.5,0.625,0.75,0.875,
1.),.UNSPECIFIED.);
#29606=B_SPLINE_CURVE_WITH_KNOTS('',3,(#120092,#120093,#120094,#120095,
#120096,#120097,#120098,#120099,#120100,#120101,#120102,#120103,#120104,
#120105,#120106,#120107,#120108,#120109,#120110,#120111,#120112,#120113,
#120114,#120115,#120116,#120117,#120118,#120119,#120120,#120121,#120122,
#120123,#120124,#120125,#120126,#120127,#120128,#120129,#120130,#120131,
#120132,#120133,#120134,#120135,#120136,#120137,#120138,#120139,#120140,
#120141,#120142,#120143,#120144,#120145,#120146,#120147,#120148,#120149,
#120150,#120151,#120152,#120153,#120154,#120155,#120156,#120157,#120158,
#120159,#120160,#120161,#120162,#120163,#120164,#120165,#120166,#120167,
#120168,#120169,#120170,#120171,#120172,#120173,#120174,#120175,#120176,
#120177,#120178,#120179,#120180,#120181,#120182,#120183,#120184,#120185,
#120186,#120187,#120188,#120189,#120190,#120191,#120192,#120193,#120194,
#120195,#120196,#120197,#120198,#120199,#120200,#120201,#120202,#120203,
#120204,#120205,#120206,#120207,#120208,#120209,#120210,#120211,#120212,
#120213,#120214,#120215,#120216,#120217,#120218,#120219,#120220,#120221,
#120222,#120223,#120224,#120225,#120226,#120227,#120228,#120229,#120230,
#120231,#120232,#120233,#120234,#120235,#120236,#120237,#120238,#120239,
#120240,#120241,#120242,#120243,#120244,#120245,#120246,#120247,#120248,
#120249,#120250,#120251,#120252,#120253,#120254,#120255,#120256,#120257,
#120258,#120259,#120260,#120261,#120262,#120263,#120264,#120265,#120266,
#120267,#120268,#120269,#120270,#120271,#120272,#120273,#120274,#120275,
#120276,#120277,#120278,#120279,#120280,#120281,#120282,#120283,#120284,
#120285,#120286,#120287,#120288,#120289,#120290,#120291,#120292,#120293,
#120294,#120295,#120296,#120297,#120298,#120299,#120300,#120301,#120302,
#120303,#120304,#120305,#120306,#120307,#120308,#120309,#120310,#120311,
#120312,#120313,#120314,#120315,#120316,#120317,#120318,#120319,#120320,
#120321,#120322,#120323,#120324,#120325,#120326,#120327,#120328,#120329,
#120330,#120331,#120332,#120333,#120334,#120335,#120336,#120337,#120338,
#120339,#120340,#120341,#120342,#120343,#120344,#120345,#120346,#120347,
#120348,#120349,#120350,#120351,#120352,#120353),.UNSPECIFIED.,.F.,.F.,
(4,3,3,3,3,3,3,3,3,3,3,3,3,3,3,3,3,3,3,3,3,3,3,3,3,3,3,3,3,3,3,3,3,3,3,
3,3,3,3,3,3,3,3,3,3,3,3,3,3,3,3,3,3,3,3,3,3,3,3,3,3,3,3,3,3,3,3,3,3,3,3,
3,3,3,3,3,3,3,3,3,3,3,3,3,3,3,3,4),(0.,0.0238209341068048,0.0467771592652955,
0.0716124027086975,0.0960789029123286,0.121297615955388,0.124999999999497,
0.1448631456153,0.177264818887828,0.187499999999245,0.192104350528002,0.218749999999119,
0.234374999999057,0.236532403911906,0.242187499999027,0.246093749999012,
0.248046874999006,0.249999999999,0.277130585388565,0.306461178729683,0.312499999998764,
0.31866267267183,0.343749999998647,0.357129683416764,0.359374999998589,
0.367187499998561,0.371093749998547,0.374023437498536,0.374999999998531,
0.396143077643392,0.397799905177464,0.417649952587889,0.437499999998313,
0.438016277914377,0.455310479258491,0.468749999998204,0.474778249992469,
0.484374999998149,0.492187499998122,0.496093749998109,0.498046874998102,
0.499511718748098,0.499999999998097,0.512502904327935,0.531852979385863,
0.550582392521049,0.555525187566182,0.562499999997784,0.581209522793947,
0.593412137124177,0.593749999997628,0.609374999997549,0.61718749999751,
0.621093749997491,0.623046874997481,0.624023437497476,0.624755859372473,
0.624999999997473,0.626485940845937,0.637328140931271,0.64811722289407,
0.656249999997412,0.667544912414052,0.6778997253239,0.687499999997352,0.698454072030051,
0.709299235852108,0.718749999997292,0.729412231271347,0.734374999997263,
0.742187499997248,0.742996539894464,0.746093749997245,0.748046874997241,
0.749023437497239,0.749755859372251,0.749999999997255,0.787581559332529,
0.80494092963963,0.845391786652635,0.868911827543509,0.874999999998627,
0.901163899253755,0.926976316555449,0.941952390352306,0.966830975600087,
0.990868090258758,1.),.UNSPECIFIED.);
#29607=B_SPLINE_CURVE_WITH_KNOTS('',3,(#120391,#120392,#120393,#120394,
#120395,#120396,#120397,#120398,#120399,#120400,#120401,#120402,#120403,
#120404,#120405,#120406,#120407,#120408,#120409,#120410,#120411,#120412,
#120413,#120414,#120415,#120416,#120417,#120418,#120419,#120420,#120421,
#120422,#120423,#120424,#120425,#120426,#120427),.UNSPECIFIED.,.F.,.F.,
(4,3,3,3,3,3,3,3,3,3,3,3,4),(0.,0.125,0.159379704574452,0.25,0.375,0.442772260766343,
0.5,0.625,0.695069700307422,0.75,0.875,0.9182517730451,1.),
 .UNSPECIFIED.);
#29608=B_SPLINE_CURVE_WITH_KNOTS('',3,(#120454,#120455,#120456,#120457,
#120458,#120459,#120460,#120461,#120462,#120463,#120464,#120465,#120466,
#120467,#120468,#120469,#120470,#120471,#120472,#120473,#120474,#120475,
#120476,#120477,#120478,#120479,#120480,#120481,#120482,#120483,#120484,
#120485,#120486,#120487,#120488,#120489,#120490,#120491,#120492,#120493,
#120494,#120495,#120496,#120497,#120498,#120499,#120500,#120501,#120502,
#120503,#120504,#120505,#120506,#120507,#120508,#120509,#120510,#120511),
 .UNSPECIFIED.,.F.,.F.,(4,3,3,3,3,3,3,3,3,3,3,3,3,3,3,3,3,3,3,4),(2.46869136895203E-9,
0.0537338962153679,0.107904863661443,0.162436722894872,0.217699031243316,
0.25,0.304279076375914,0.325891175570963,0.382268789223474,0.441134394611737,
0.5,0.565029224088735,0.631574437929143,0.701211809658827,0.727527916786862,
0.75,0.829316881692732,0.908964210246409,0.988920295930411,1.),
 .UNSPECIFIED.);
#29609=B_SPLINE_CURVE_WITH_KNOTS('',3,(#120538,#120539,#120540,#120541,
#120542,#120543,#120544,#120545,#120546,#120547,#120548,#120549,#120550,
#120551,#120552,#120553,#120554,#120555,#120556,#120557,#120558,#120559,
#120560,#120561,#120562,#120563,#120564,#120565,#120566,#120567,#120568,
#120569,#120570,#120571,#120572,#120573,#120574,#120575,#120576,#120577,
#120578,#120579,#120580,#120581,#120582,#120583,#120584,#120585,#120586,
#120587,#120588,#120589,#120590,#120591,#120592,#120593,#120594,#120595,
#120596,#120597,#120598),.UNSPECIFIED.,.F.,.F.,(4,3,3,3,3,3,3,3,3,3,3,3,
3,3,3,3,3,3,3,3,4),(3.09719472403435E-11,0.0796519720589834,0.159046227126963,
0.237897866026407,0.25,0.280661606842029,0.349436459717617,0.416021534400952,
0.480361119054478,0.5,0.557540612918763,0.614138830092457,0.669699825343428,
0.689729105407977,0.743459053446208,0.75,0.805600763210536,0.860275880253665,
0.91452354817423,0.96831217149722,1.),.UNSPECIFIED.);
#29610=B_SPLINE_CURVE_WITH_KNOTS('',3,(#120637,#120638,#120639,#120640,
#120641,#120642,#120643,#120644,#120645,#120646,#120647,#120648,#120649,
#120650,#120651,#120652,#120653,#120654,#120655,#120656,#120657,#120658,
#120659,#120660,#120661,#120662,#120663,#120664,#120665,#120666,#120667,
#120668,#120669,#120670,#120671,#120672,#120673,#120674,#120675,#120676,
#120677,#120678,#120679,#120680,#120681,#120682,#120683,#120684,#120685,
#120686,#120687,#120688,#120689,#120690,#120691,#120692,#120693,#120694,
#120695,#120696,#120697,#120698,#120699,#120700,#120701,#120702,#120703,
#120704,#120705,#120706,#120707,#120708,#120709,#120710,#120711,#120712,
#120713,#120714,#120715,#120716,#120717,#120718,#120719,#120720,#120721,
#120722,#120723,#120724,#120725,#120726,#120727,#120728,#120729,#120730,
#120731,#120732,#120733,#120734,#120735,#120736,#120737,#120738,#120739,
#120740,#120741,#120742,#120743,#120744,#120745,#120746,#120747,#120748),
 .UNSPECIFIED.,.F.,.F.,(4,3,3,3,3,3,3,3,3,3,3,3,3,3,3,3,3,3,3,3,3,3,3,3,
3,3,3,3,3,3,3,3,3,3,3,3,3,4),(1.35859990185527E-10,0.0470443616163219,0.0914258222496483,
0.134880138091579,0.177094202045214,0.188177446057708,0.232586222210198,
0.249999999999647,0.292935299290597,0.334529543417577,0.370069482793404,
0.374999999999471,0.419953636131847,0.437499999999383,0.468749999999339,
0.484374999999316,0.492187499999305,0.497503839155331,0.499999999999294,
0.527504839471645,0.586107358467935,0.624999999999114,0.680623224833669,
0.687499999999023,0.718749999998977,0.734374999998954,0.742187499998943,
0.746093749998938,0.749023437498937,0.749999999998938,0.790947953022685,
0.831969774017496,0.866381434603491,0.87499999999947,0.917111533151109,
0.958555766575555,0.997597822520349,1.),.UNSPECIFIED.);
#29611=B_SPLINE_CURVE_WITH_KNOTS('',3,(#120785,#120786,#120787,#120788,
#120789,#120790,#120791,#120792,#120793,#120794,#120795,#120796,#120797,
#120798,#120799,#120800,#120801,#120802,#120803,#120804,#120805,#120806,
#120807,#120808,#120809,#120810,#120811,#120812,#120813,#120814,#120815,
#120816,#120817,#120818,#120819,#120820,#120821,#120822,#120823,#120824,
#120825,#120826,#120827,#120828,#120829,#120830,#120831,#120832,#120833,
#120834,#120835,#120836,#120837,#120838,#120839,#120840,#120841,#120842,
#120843,#120844,#120845,#120846,#120847,#120848,#120849,#120850,#120851,
#120852,#120853,#120854,#120855,#120856,#120857,#120858,#120859,#120860,
#120861,#120862,#120863,#120864,#120865,#120866,#120867,#120868,#120869,
#120870,#120871,#120872,#120873,#120874,#120875,#120876,#120877,#120878),
 .UNSPECIFIED.,.F.,.F.,(4,3,3,3,3,3,3,3,3,3,3,3,3,3,3,3,3,3,3,3,3,3,3,3,
3,3,3,3,3,3,3,4),(1.82471863577943E-15,0.0480765556136813,0.0950049750541619,
0.109486100629603,0.125000000000092,0.17303730245179,0.187500000000138,
0.218750000000161,0.234375000000174,0.242187500000179,0.242327475881498,
0.246093750000182,0.249352229155617,0.250000000000186,0.333497092429205,
0.371351184332586,0.375000000000239,0.437500000000266,0.46875000000028,
0.484375000000287,0.492187500000291,0.499023437500293,0.500000000000293,
0.500924792082816,0.597383972836421,0.652289628044168,0.743514330544788,
0.750000000000146,0.786603976412445,0.885125481150069,0.905550136399524,
1.),.UNSPECIFIED.);
#29612=B_SPLINE_CURVE_WITH_KNOTS('',3,(#120950,#120951,#120952,#120953,
#120954,#120955,#120956,#120957,#120958,#120959,#120960,#120961,#120962,
#120963,#120964,#120965,#120966,#120967,#120968,#120969,#120970,#120971,
#120972,#120973,#120974,#120975,#120976,#120977,#120978,#120979,#120980,
#120981,#120982,#120983,#120984,#120985,#120986,#120987,#120988,#120989,
#120990,#120991,#120992,#120993,#120994,#120995,#120996,#120997,#120998,
#120999,#121000,#121001,#121002,#121003,#121004,#121005,#121006,#121007,
#121008,#121009,#121010,#121011,#121012,#121013,#121014,#121015,#121016,
#121017,#121018,#121019,#121020,#121021,#121022,#121023,#121024,#121025,
#121026,#121027,#121028,#121029,#121030,#121031,#121032,#121033,#121034),
 .UNSPECIFIED.,.F.,.F.,(4,3,3,3,3,3,3,3,3,3,3,3,3,3,3,3,3,3,3,3,3,3,3,3,
3,3,3,3,4),(0.,0.0377356474345836,0.0750359183060471,0.112014973382577,
0.148784553462237,0.185454708791299,0.222134505688996,0.259084364534882,
0.296281779749553,0.333825646040157,0.37181660829074,0.410693571798126,
0.450151209829126,0.490604164911084,0.49999988363958,0.540309510289047,
0.579736856800743,0.618411911999495,0.656459211910049,0.69399873229563,
0.732248890758676,0.769066832853226,0.805766270351344,0.842443980675107,
0.87919658146079,0.916274247721778,0.953595787796437,0.99142322355931,1.),
 .UNSPECIFIED.);
#29613=B_SPLINE_CURVE_WITH_KNOTS('',3,(#121585,#121586,#121587,#121588,
#121589,#121590,#121591,#121592,#121593,#121594,#121595,#121596,#121597,
#121598,#121599,#121600,#121601,#121602),.UNSPECIFIED.,.F.,.F.,(4,2,2,2,
2,2,2,2,4),(0.,0.125,0.25,0.375,0.5,0.625,0.75,0.875,1.),.UNSPECIFIED.);
#29614=B_SPLINE_CURVE_WITH_KNOTS('',3,(#121744,#121745,#121746,#121747,
#121748,#121749,#121750,#121751,#121752,#121753,#121754,#121755,#121756,
#121757,#121758,#121759,#121760,#121761,#121762,#121763,#121764,#121765,
#121766,#121767,#121768,#121769,#121770,#121771,#121772,#121773,#121774,
#121775,#121776,#121777,#121778,#121779,#121780,#121781,#121782,#121783,
#121784,#121785,#121786,#121787,#121788,#121789,#121790,#121791,#121792,
#121793,#121794,#121795,#121796,#121797,#121798,#121799,#121800,#121801,
#121802,#121803,#121804,#121805,#121806,#121807,#121808,#121809,#121810,
#121811,#121812,#121813,#121814,#121815,#121816,#121817,#121818,#121819),
 .UNSPECIFIED.,.F.,.F.,(4,3,3,3,3,3,3,3,3,3,3,3,3,3,3,3,3,3,3,3,3,3,3,3,
3,4),(0.,0.0425596242447764,0.0850361814342877,0.127671390328244,0.170444375881725,
0.213698376037449,0.25,0.294181213942584,0.339346412338439,0.375,0.421689901291409,
0.433453762242374,0.480051410417501,0.5,0.545161817254489,0.589577224406666,
0.633151386249373,0.676316383684887,0.719082658493756,0.75,0.792498951096667,
0.835001497275773,0.877796290208396,0.920803849450017,0.964410339796297,
1.),.UNSPECIFIED.);
#29615=B_SPLINE_CURVE_WITH_KNOTS('',3,(#121907,#121908,#121909,#121910,
#121911,#121912,#121913,#121914,#121915,#121916),.UNSPECIFIED.,.F.,.F.,
(4,2,2,2,4),(0.000307180223244836,0.23813963987228,0.403654270152061,0.532445083611112,
0.661208903651667),.UNSPECIFIED.);
#29616=B_SPLINE_CURVE_WITH_KNOTS('',3,(#121917,#121918,#121919,#121920,
#121921,#121922,#121923,#121924,#121925,#121926,#121927,#121928,#121929,
#121930),.UNSPECIFIED.,.F.,.F.,(4,2,2,2,2,2,4),(0.000330903451301007,0.188084532547518,
0.374775943028081,0.612257137717574,0.795567417884798,0.901363102744604,
1.00443306905523),.UNSPECIFIED.);
#29617=B_SPLINE_CURVE_WITH_KNOTS('',3,(#121931,#121932,#121933,#121934,
#121935,#121936,#121937,#121938,#121939,#121940,#121941,#121942,#121943,
#121944,#121945,#121946,#121947,#121948,#121949,#121950,#121951,#121952,
#121953,#121954,#121955,#121956,#121957,#121958,#121959,#121960,#121961,
#121962,#121963,#121964,#121965,#121966,#121967,#121968,#121969,#121970,
#121971,#121972,#121973,#121974,#121975,#121976,#121977,#121978,#121979,
#121980,#121981,#121982,#121983,#121984,#121985,#121986,#121987,#121988,
#121989,#121990,#121991,#121992,#121993,#121994,#121995,#121996,#121997,
#121998,#121999,#122000,#122001,#122002,#122003,#122004,#122005,#122006,
#122007,#122008,#122009,#122010,#122011,#122012,#122013,#122014,#122015,
#122016,#122017,#122018,#122019,#122020,#122021,#122022,#122023,#122024,
#122025,#122026,#122027,#122028,#122029,#122030,#122031,#122032,#122033,
#122034,#122035,#122036,#122037,#122038,#122039),.UNSPECIFIED.,.F.,.F.,
(4,3,3,3,3,3,3,3,3,3,3,3,3,3,3,3,3,3,3,3,3,3,3,3,3,3,3,3,3,3,3,3,3,3,3,
3,4),(5.49757971508832E-5,0.0323764919258928,0.0647628196246539,0.0969949948714976,
0.124999999999994,0.157798122778746,0.189882334389919,0.201607571319194,
0.234374999999991,0.243938228638234,0.249999999999991,0.281697673924662,
0.313958065309001,0.346679963238968,0.379829992946779,0.413050745110431,
0.446112843622199,0.468749999999984,0.484374999999984,0.499999999999983,
0.533983406046698,0.56790148030433,0.601435499225249,0.629514094834484,
0.663266314189443,0.687499999999991,0.715194727768877,0.743005238070075,
0.749999999999992,0.782919512243476,0.816298218352298,0.850005157037389,
0.883880530988718,0.917676982175652,0.951261736544021,0.984338012747187,
0.999964300005559),.UNSPECIFIED.);
#29618=B_SPLINE_CURVE_WITH_KNOTS('',3,(#122085,#122086,#122087,#122088,
#122089,#122090,#122091,#122092,#122093,#122094,#122095,#122096,#122097,
#122098,#122099,#122100,#122101,#122102,#122103,#122104,#122105,#122106,
#122107,#122108,#122109,#122110,#122111,#122112,#122113,#122114,#122115,
#122116,#122117,#122118,#122119,#122120,#122121,#122122,#122123,#122124,
#122125,#122126,#122127,#122128,#122129,#122130,#122131,#122132,#122133,
#122134,#122135,#122136,#122137,#122138,#122139,#122140,#122141,#122142,
#122143,#122144,#122145,#122146,#122147,#122148,#122149,#122150,#122151,
#122152,#122153,#122154,#122155,#122156,#122157,#122158,#122159,#122160,
#122161,#122162,#122163,#122164,#122165,#122166,#122167,#122168,#122169,
#122170,#122171,#122172,#122173,#122174,#122175,#122176,#122177,#122178,
#122179,#122180,#122181,#122182,#122183,#122184,#122185,#122186,#122187,
#122188,#122189,#122190,#122191,#122192,#122193,#122194,#122195,#122196,
#122197,#122198,#122199,#122200,#122201,#122202,#122203,#122204,#122205,
#122206,#122207,#122208,#122209,#122210,#122211,#122212,#122213,#122214,
#122215,#122216,#122217,#122218,#122219,#122220,#122221,#122222,#122223,
#122224,#122225,#122226,#122227,#122228,#122229,#122230,#122231,#122232,
#122233,#122234,#122235,#122236,#122237,#122238,#122239,#122240,#122241,
#122242,#122243,#122244),.UNSPECIFIED.,.F.,.F.,(4,3,3,3,3,3,3,3,3,3,3,3,
3,3,3,3,3,3,3,3,3,3,3,3,3,3,3,3,3,3,3,3,3,3,3,3,3,3,3,3,3,3,3,3,3,3,3,3,
3,3,3,3,3,4),(0.,0.033129419996528,0.0625,0.082406368093979,0.101976381960474,
0.120919538933606,0.125,0.131399088166994,0.155178211525652,0.180376994852815,
0.206264449066017,0.23253290097541,0.25,0.269300260094727,0.286686870246049,
0.305558168739884,0.324831549147336,0.344082508667133,0.362955762961432,
0.375,0.39250067506772,0.41010515685722,0.42757262063518,0.441864639561154,
0.459372727734466,0.476982526010831,0.494482045172937,0.5,0.520230351612384,
0.541125772179517,0.562132098769343,0.582818980361532,0.597074992568842,
0.61807026910004,0.625,0.648247295937558,0.671966741455924,0.695535554643394,
0.718590663848995,0.740681955330333,0.75,0.752375849440358,0.775477859920143,
0.800358394940107,0.825273162437448,0.850161922207706,0.874999999999999,
0.893484411102079,0.907662745170859,0.925963795076234,0.9375,0.958867940339968,
0.981119642099533,0.999990983828168),.UNSPECIFIED.);
#29619=B_SPLINE_CURVE_WITH_KNOTS('',3,(#122358,#122359,#122360,#122361,
#122362,#122363,#122364,#122365,#122366,#122367,#122368,#122369,#122370,
#122371,#122372,#122373,#122374,#122375,#122376,#122377,#122378,#122379,
#122380,#122381,#122382,#122383,#122384,#122385,#122386,#122387,#122388,
#122389,#122390,#122391,#122392,#122393,#122394,#122395,#122396,#122397,
#122398,#122399,#122400,#122401,#122402,#122403,#122404,#122405,#122406,
#122407,#122408,#122409,#122410,#122411,#122412,#122413,#122414,#122415,
#122416,#122417,#122418,#122419,#122420,#122421,#122422,#122423,#122424,
#122425,#122426,#122427,#122428,#122429,#122430,#122431),.UNSPECIFIED.,
 .F.,.F.,(4,2,2,2,2,2,2,2,2,2,2,2,2,2,2,2,2,2,2,2,2,2,2,2,2,2,2,2,2,2,2,
2,2,2,2,2,4),(0.000380014155147578,0.245400900644386,0.378255056806249,
0.463178941729333,0.615939968604413,0.712651720402226,0.856256025420663,
0.962182568221084,1.24868208289919,1.37004830733658,1.46833903165977,1.67247354457994,
1.76813658054073,1.98089867447481,2.11019670522888,2.24182819113389,2.50529938263797,
2.70189252294529,2.80669898539374,2.94035387038927,3.05860534802554,3.30159424022801,
3.45351780809231,3.71018557888163,3.82068057363443,4.00827847738079,4.09333004173814,
4.25652959393851,4.3142784495563,4.44522754595014,4.62073300232603,4.82402568991634,
4.90519387006344,5.0009249225532,5.14395581948815,5.28962261426793,5.35030271608699),
 .UNSPECIFIED.);
#29620=B_SPLINE_CURVE_WITH_KNOTS('',3,(#122650,#122651,#122652,#122653,
#122654,#122655),.UNSPECIFIED.,.F.,.F.,(4,2,4),(-0.164978192357391,-0.0826598660794179,
-6.1266948559559E-5),.UNSPECIFIED.);
#29621=B_SPLINE_CURVE_WITH_KNOTS('',3,(#122656,#122657,#122658,#122659,
#122660,#122661,#122662,#122663,#122664,#122665,#122666,#122667,#122668,
#122669,#122670,#122671,#122672,#122673,#122674,#122675,#122676,#122677,
#122678,#122679,#122680,#122681,#122682,#122683,#122684,#122685,#122686,
#122687,#122688,#122689,#122690,#122691,#122692,#122693,#122694,#122695,
#122696,#122697,#122698,#122699,#122700,#122701,#122702,#122703,#122704,
#122705,#122706,#122707,#122708,#122709,#122710,#122711,#122712,#122713,
#122714,#122715,#122716,#122717,#122718,#122719,#122720,#122721,#122722,
#122723,#122724,#122725,#122726,#122727,#122728,#122729,#122730,#122731,
#122732,#122733,#122734,#122735,#122736,#122737,#122738,#122739,#122740,
#122741,#122742,#122743,#122744,#122745,#122746,#122747,#122748,#122749,
#122750,#122751,#122752,#122753,#122754,#122755,#122756,#122757,#122758,
#122759,#122760,#122761,#122762,#122763,#122764,#122765,#122766,#122767,
#122768,#122769,#122770,#122771,#122772,#122773,#122774,#122775,#122776,
#122777,#122778,#122779,#122780,#122781,#122782,#122783,#122784,#122785,
#122786,#122787,#122788,#122789,#122790,#122791,#122792,#122793,#122794,
#122795,#122796,#122797,#122798,#122799,#122800,#122801,#122802,#122803,
#122804,#122805,#122806,#122807,#122808,#122809,#122810,#122811,#122812,
#122813,#122814,#122815,#122816,#122817,#122818,#122819,#122820,#122821,
#122822,#122823,#122824,#122825,#122826,#122827,#122828,#122829,#122830,
#122831,#122832,#122833,#122834,#122835,#122836,#122837,#122838,#122839,
#122840,#122841,#122842,#122843,#122844,#122845,#122846,#122847,#122848,
#122849,#122850,#122851,#122852,#122853,#122854,#122855,#122856,#122857,
#122858,#122859,#122860,#122861,#122862,#122863,#122864,#122865,#122866,
#122867,#122868,#122869,#122870,#122871,#122872,#122873,#122874,#122875,
#122876,#122877,#122878,#122879,#122880,#122881,#122882,#122883,#122884,
#122885,#122886,#122887,#122888,#122889,#122890,#122891,#122892,#122893,
#122894,#122895,#122896,#122897,#122898,#122899,#122900,#122901,#122902,
#122903,#122904,#122905,#122906,#122907,#122908,#122909,#122910,#122911,
#122912,#122913,#122914,#122915,#122916,#122917,#122918,#122919,#122920,
#122921,#122922,#122923,#122924,#122925,#122926,#122927,#122928,#122929),
 .UNSPECIFIED.,.F.,.F.,(4,2,2,2,2,2,2,2,2,2,2,2,2,2,2,2,2,2,2,2,2,2,2,2,
2,2,2,2,2,2,2,2,2,2,2,2,2,2,2,2,2,2,2,2,2,2,2,2,2,2,2,2,2,2,2,2,2,2,2,2,
2,2,2,2,2,2,2,2,2,2,2,2,2,2,2,2,2,2,2,2,2,2,2,2,2,2,2,2,2,2,2,2,2,2,2,2,
2,2,2,2,2,2,2,2,2,2,2,2,2,2,2,2,2,2,2,2,2,2,2,2,2,2,2,2,2,2,2,2,2,2,2,2,
2,2,2,2,4),(0.000107512992587567,0.0307029019400883,0.100674212329956,0.180228075751325,
0.223629579703032,0.323919845537183,0.427401544199471,0.471224803865406,
0.583011397883141,0.626400339262408,0.66873184127474,0.737215545709424,
0.845622646823796,0.911171121611078,0.953287896144272,1.02549345955771,
1.09680105460438,1.14185700300284,1.25541675409781,1.35851753679182,1.40299698368004,
1.47702838572308,1.5551977984083,1.60115722077726,1.71873749126671,1.81817866078206,
1.86436795535943,1.93730809028004,2.01368613423001,2.06088763331795,2.20020985446626,
2.26468915413711,2.31672947233915,2.4246770501876,2.46671363402353,2.51411350596787,
2.65381332413122,2.72275435940137,2.777342380313,2.88426525387493,2.92678175415279,
2.97615763886728,3.10740549087446,3.180980377387,3.23815711434674,3.34215362263346,
3.38601797756853,3.43741188267961,3.54467777649841,3.63171848251686,3.69481537016392,
3.75212879385147,3.82275558517828,3.87612962526921,3.95177424416194,4.07393090099034,
4.13172841019533,4.18351479411174,4.2705764461913,4.31912584057365,4.38250782077004,
4.5251978320351,4.60817147112523,4.66273098314723,4.75271255076504,4.80889116540233,
4.90294295753267,5.00850630294855,5.08083401316878,5.15285202196741,5.20910477165492,
5.26759899494988,5.36663118994816,5.47251101319393,5.54617039862718,5.63257611663657,
5.6862460524546,5.75288766489232,5.90524576359981,5.99823452074483,6.0990762014458,
6.17136776695553,6.35777567918109,6.46014851823537,6.55091370704972,6.61114640499581,
6.69291504150126,6.84207985177244,6.91279980483302,6.98265522377385,7.0445092411034,
7.11723125794406,7.20271918433045,7.38789940501584,7.4583079712193,7.55592669346919,
7.69308787750945,7.84085311941344,7.92076956771712,8.01940122147781,8.10637205006814,
8.32606194523382,8.39803835772438,8.4817437542093,8.57639856983484,8.7850038869388,
8.86453348834936,8.95410792023663,9.06348271921736,9.25315373748551,9.33890568952937,
9.44906848541356,9.60176037303482,9.72921770001139,9.81940238786216,9.97563038872898,
10.2009413300206,10.2906338093867,10.479299785875,10.6556209495947,10.7576154833082,
10.8890151810613,11.0616734096201,11.2444507251959,11.4132342709487,11.5897230164771,
11.7152242220242,11.9303380425397,12.2870964789061,12.4637943364461,12.7344749369786,
12.9129627166077,13.0899098943205,13.4398693363585,13.613254539275,13.8661682772203,
14.1207718959965),.UNSPECIFIED.);
#29622=B_SPLINE_CURVE_WITH_KNOTS('',3,(#123071,#123072,#123073,#123074,
#123075,#123076,#123077,#123078,#123079,#123080,#123081,#123082,#123083,
#123084,#123085,#123086,#123087,#123088,#123089,#123090,#123091,#123092,
#123093,#123094,#123095,#123096,#123097,#123098,#123099,#123100,#123101,
#123102,#123103,#123104,#123105,#123106,#123107,#123108,#123109,#123110,
#123111,#123112,#123113,#123114,#123115,#123116,#123117,#123118,#123119,
#123120,#123121,#123122,#123123,#123124,#123125,#123126,#123127,#123128,
#123129,#123130,#123131,#123132,#123133,#123134,#123135,#123136,#123137,
#123138,#123139,#123140),.UNSPECIFIED.,.F.,.F.,(4,3,3,3,3,3,3,3,3,3,3,3,
3,3,3,3,3,3,3,3,3,3,3,4),(0.000487461485702938,0.0513587634045652,0.102739521495275,
0.154402996931755,0.206009843163793,0.25733899970698,0.30794881997648,0.334407148518828,
0.385559996521794,0.436202598467051,0.483282059114614,0.493580691131268,
0.498350316792659,0.502179951010243,0.551475747420326,0.601611641439809,
0.654418301991745,0.705919568722183,0.759378926184868,0.812838283647554,
0.864463775759805,0.916113864982514,0.967433679917503,1.),.UNSPECIFIED.);
#29623=B_SPLINE_CURVE_WITH_KNOTS('',3,(#123141,#123142,#123143,#123144,
#123145,#123146,#123147,#123148,#123149,#123150,#123151,#123152,#123153,
#123154,#123155,#123156,#123157,#123158,#123159,#123160,#123161,#123162,
#123163,#123164,#123165,#123166,#123167,#123168,#123169,#123170,#123171,
#123172,#123173,#123174,#123175,#123176,#123177,#123178,#123179,#123180,
#123181,#123182,#123183,#123184,#123185,#123186,#123187,#123188,#123189,
#123190,#123191,#123192,#123193,#123194,#123195,#123196,#123197,#123198,
#123199,#123200,#123201,#123202,#123203,#123204,#123205,#123206,#123207,
#123208,#123209,#123210,#123211,#123212,#123213,#123214,#123215,#123216,
#123217,#123218,#123219,#123220,#123221,#123222,#123223,#123224,#123225,
#123226,#123227,#123228,#123229,#123230,#123231,#123232,#123233,#123234,
#123235,#123236,#123237,#123238,#123239,#123240,#123241,#123242,#123243,
#123244,#123245,#123246,#123247,#123248,#123249,#123250,#123251,#123252,
#123253,#123254,#123255,#123256,#123257,#123258,#123259,#123260,#123261,
#123262,#123263,#123264,#123265,#123266,#123267,#123268,#123269,#123270,
#123271,#123272,#123273,#123274,#123275,#123276,#123277,#123278,#123279,
#123280,#123281,#123282,#123283,#123284,#123285,#123286,#123287,#123288,
#123289,#123290,#123291,#123292,#123293,#123294,#123295,#123296,#123297,
#123298,#123299,#123300,#123301,#123302,#123303,#123304,#123305,#123306,
#123307,#123308,#123309,#123310,#123311,#123312,#123313,#123314,#123315,
#123316,#123317,#123318,#123319,#123320,#123321,#123322,#123323,#123324,
#123325,#123326,#123327,#123328,#123329,#123330,#123331,#123332,#123333,
#123334,#123335,#123336,#123337,#123338,#123339,#123340,#123341,#123342,
#123343,#123344,#123345,#123346,#123347,#123348,#123349,#123350,#123351,
#123352,#123353,#123354,#123355,#123356,#123357,#123358,#123359,#123360,
#123361,#123362,#123363,#123364,#123365,#123366,#123367,#123368,#123369,
#123370,#123371,#123372,#123373,#123374,#123375,#123376,#123377,#123378,
#123379,#123380,#123381,#123382,#123383,#123384,#123385,#123386,#123387,
#123388,#123389,#123390,#123391,#123392,#123393,#123394,#123395,#123396,
#123397,#123398,#123399,#123400,#123401,#123402,#123403,#123404,#123405,
#123406,#123407,#123408,#123409,#123410,#123411,#123412,#123413,#123414,
#123415,#123416,#123417,#123418,#123419,#123420,#123421,#123422,#123423,
#123424,#123425,#123426,#123427,#123428,#123429,#123430,#123431,#123432,
#123433,#123434,#123435,#123436,#123437,#123438,#123439,#123440,#123441,
#123442,#123443,#123444,#123445,#123446,#123447,#123448,#123449,#123450,
#123451,#123452),.UNSPECIFIED.,.F.,.F.,(4,2,2,2,2,2,2,2,2,2,2,2,2,2,2,2,
2,2,2,2,2,2,2,2,2,2,2,2,2,2,2,2,2,2,2,2,2,2,2,2,2,2,2,2,2,2,2,2,2,2,2,2,
2,2,2,2,2,2,2,2,2,2,2,2,2,2,2,2,2,2,2,2,2,2,2,2,2,2,2,2,2,2,2,2,2,2,2,2,
2,2,2,2,2,2,2,2,2,2,2,2,2,2,2,2,2,2,2,2,2,2,2,2,2,2,2,2,2,2,2,2,2,2,2,2,
2,2,2,2,2,2,2,2,2,2,2,2,2,2,2,2,2,2,2,2,2,2,2,2,2,2,2,2,2,2,2,4),(-18.5336227826717,
-18.4514448464926,-18.3192192351927,-18.2650075335487,-18.2296714748852,
-18.1936764844934,-18.1398332323042,-17.9787567624792,-17.6074573856008,
-17.4091261341456,-17.2859748498613,-17.1486066700017,-16.8265679635732,
-16.6714026169584,-16.5369101371266,-16.3635946951212,-16.1449777165132,
-15.976591588593,-15.850232744328,-15.719410379549,-15.4335967644799,-15.3021203406268,
-15.0737477187498,-14.9686633592023,-14.6821199003543,-14.5166018440642,
-14.4190871127192,-14.2365688695425,-14.1549985867376,-14.0094123223151,
-13.8390819603086,-13.7262967303264,-13.6376584314877,-13.4760226296493,
-13.3832983618377,-13.2972446525463,-13.0899731981048,-12.9983742927356,
-12.920788894281,-12.7456562217242,-12.6050338049676,-12.5359590214847,
-12.3689141170616,-12.2113297245226,-12.1394297703413,-12.0218491054587,
-11.8753788793851,-11.7807108351215,-11.7066713015056,-11.523302821056,
-11.4412051755254,-11.3676144563314,-11.1253926001387,-11.0293198021,-10.9504792860078,
-10.7430838491658,-10.6623854411574,-10.5829348304118,-10.4242381587643,
-10.2707780527122,-10.1645906166968,-10.0761279647731,-9.89450227377428,
-9.80277984150293,-9.64601940897569,-9.47027339843058,-9.34923892594618,
-9.18181695131492,-9.0807999609014,-8.94229176178927,-8.68557879400708,
-8.56254906259355,-8.44364973517209,-8.30539798661457,-7.89871833726101,
-7.73145721019517,-7.45916760741117,-6.83025432997125,-6.52534187991016,
-6.07249570523818,-5.89165241152614,-5.79714214963211,-5.63598606556114,
-5.52969354225683,-5.3423835033615,-5.25759186065315,-5.18724048257733,
-5.1175100810236,-4.96593366239356,-4.89035567654671,-4.83259928305064,
-4.75029160524615,-4.6849317220865,-4.59312652184032,-4.49460001409083,
-4.44161946958288,-4.33894081785888,-4.28905965363311,-4.22808891227909,
-4.13686583498971,-4.05095250786917,-4.00560939785189,-3.95669382763748,
-3.85483321893934,-3.81312267865046,-3.71393955714425,-3.62374250053462,
-3.58177584901668,-3.50096552738975,-3.40620773382679,-3.36751847198954,
-3.32526910970592,-3.2327219323547,-3.17161730698468,-3.12911420654313,
-3.07675136756009,-2.95087046426691,-2.91184371074789,-2.82377441762149,
-2.74097048134806,-2.69835381872593,-2.64854468976623,-2.53188028518126,
-2.48203230616119,-2.4328648000492,-2.35512837158407,-2.29536984943275,
-2.24180082960586,-2.17243444539022,-2.04973933686738,-2.00344232911898,
-1.95639296462131,-1.85954692193472,-1.79502549613509,-1.70634293710404,
-1.59827660739526,-1.54298367544123,-1.48200932828646,-1.41686546373561,
-1.33260166363418,-1.19565746731822,-1.12254945361788,-1.04777428960563,
-0.945985362306715,-0.782164001502387,-0.679764347521197,-0.600110757961878,
-0.517945998215963,-0.330531509823378,-0.233428033688739,-0.204144318222011,
-0.185289377988479,-0.166925413601217,-0.13677198850432,-0.0618204439494522,
-0.000371176546537626),.UNSPECIFIED.);
#29624=B_SPLINE_CURVE_WITH_KNOTS('',3,(#123585,#123586,#123587,#123588,
#123589,#123590),.UNSPECIFIED.,.F.,.F.,(4,2,4),(-0.164574081374655,-0.0827307715189429,
0.),.UNSPECIFIED.);
#29625=B_SPLINE_CURVE_WITH_KNOTS('',3,(#123653,#123654,#123655,#123656,
#123657,#123658,#123659,#123660,#123661,#123662,#123663,#123664,#123665,
#123666,#123667,#123668,#123669,#123670,#123671,#123672,#123673,#123674,
#123675,#123676,#123677,#123678,#123679,#123680,#123681,#123682,#123683,
#123684,#123685,#123686,#123687,#123688,#123689,#123690,#123691,#123692,
#123693,#123694,#123695,#123696,#123697,#123698,#123699,#123700,#123701),
 .UNSPECIFIED.,.F.,.F.,(4,3,3,3,3,3,3,3,3,3,3,3,3,3,3,3,4),(0.,0.0904233751484227,
0.178899056629695,0.24999999999995,0.336290310678144,0.374999999999928,
0.398831360155259,0.437499999999918,0.468749999999913,0.487949724956403,
0.499999999999908,0.586414266141055,0.67420168428988,0.764518735858738,
0.856393583171992,0.950989960497635,1.),.UNSPECIFIED.);
#29626=B_SPLINE_CURVE_WITH_KNOTS('',3,(#123703,#123704,#123705,#123706,
#123707,#123708,#123709,#123710,#123711,#123712,#123713,#123714,#123715,
#123716,#123717,#123718,#123719,#123720,#123721,#123722,#123723,#123724,
#123725,#123726,#123727,#123728,#123729,#123730,#123731,#123732,#123733),
 .UNSPECIFIED.,.F.,.F.,(4,3,3,3,3,3,3,3,3,3,4),(3.51711785548937E-10,0.113284432153487,
0.225129807988068,0.336301994397872,0.446993881464188,0.5,0.610566778230462,
0.721794516243209,0.833540970047342,0.946588755238846,1.),.UNSPECIFIED.);
#29627=B_SPLINE_CURVE_WITH_KNOTS('',3,(#123734,#123735,#123736,#123737,
#123738,#123739),.UNSPECIFIED.,.F.,.F.,(4,2,4),(0.,0.5,1.),
 .UNSPECIFIED.);
#29628=B_SPLINE_CURVE_WITH_KNOTS('',3,(#123810,#123811,#123812,#123813,
#123814,#123815,#123816,#123817,#123818,#123819,#123820,#123821,#123822,
#123823,#123824,#123825,#123826,#123827,#123828,#123829,#123830,#123831,
#123832,#123833,#123834,#123835,#123836,#123837,#123838,#123839,#123840,
#123841,#123842,#123843,#123844,#123845,#123846,#123847,#123848,#123849,
#123850,#123851,#123852,#123853,#123854,#123855,#123856,#123857,#123858,
#123859,#123860,#123861,#123862,#123863,#123864,#123865,#123866,#123867,
#123868,#123869,#123870,#123871,#123872,#123873,#123874,#123875,#123876,
#123877,#123878,#123879,#123880,#123881,#123882,#123883,#123884,#123885,
#123886,#123887,#123888,#123889,#123890,#123891,#123892,#123893,#123894,
#123895,#123896,#123897,#123898,#123899,#123900,#123901,#123902,#123903,
#123904,#123905,#123906,#123907,#123908,#123909),.UNSPECIFIED.,.F.,.F.,
(4,3,3,3,3,3,3,3,3,3,3,3,3,3,3,3,3,3,3,3,3,3,3,3,3,3,3,3,3,3,3,3,3,4),(0.,
0.0675516705121917,0.085904273434277,0.143599051494154,0.180074662513404,
0.232991527865125,0.25000000000006,0.263677503500483,0.304234548981259,
0.340135041073349,0.37500000000009,0.411897079421141,0.417227647478623,
0.437500000000106,0.468750000000114,0.484375000000117,0.492187500000118,
0.49283408507591,0.496093750000118,0.498046875000118,0.500000000000118,
0.549453116060544,0.580671458879676,0.630985226919279,0.669322200424887,
0.721053052147648,0.750000000000059,0.75885720396782,0.812757172953105,
0.849107112554098,0.90344480954754,0.939801610670112,0.995535258890343,
1.),.UNSPECIFIED.);
#29629=B_SPLINE_CURVE_WITH_KNOTS('',3,(#123913,#123914,#123915,#123916,
#123917,#123918,#123919,#123920,#123921,#123922,#123923,#123924,#123925,
#123926,#123927,#123928,#123929,#123930,#123931,#123932,#123933,#123934,
#123935,#123936,#123937,#123938,#123939,#123940,#123941,#123942,#123943,
#123944,#123945,#123946,#123947,#123948,#123949,#123950,#123951,#123952,
#123953,#123954,#123955,#123956,#123957,#123958,#123959,#123960,#123961,
#123962,#123963,#123964,#123965,#123966,#123967,#123968,#123969,#123970,
#123971,#123972,#123973,#123974,#123975,#123976,#123977,#123978,#123979,
#123980,#123981,#123982,#123983,#123984,#123985,#123986,#123987,#123988,
#123989,#123990,#123991,#123992,#123993,#123994,#123995,#123996,#123997,
#123998,#123999,#124000,#124001,#124002,#124003,#124004,#124005,#124006,
#124007,#124008,#124009),.UNSPECIFIED.,.F.,.F.,(4,3,3,3,3,3,3,3,3,3,3,3,
3,3,3,3,3,3,3,3,3,3,3,3,3,3,3,3,3,3,3,3,4),(1.13242242768556E-6,0.0650063186321231,
0.0987043254187582,0.1,0.146470218313343,0.192972087340009,0.2,0.213812109012698,
0.259692574051291,0.3,0.328657232220735,0.382282662717156,0.4,0.444122225894707,
0.488445076783722,0.5,0.549055659943903,0.559727753542975,0.6,0.634781863006224,
0.670535134136114,0.67404569477506,0.7,0.773428608298956,0.789454090675106,
0.8,0.8448500120543,0.888980980115078,0.9,0.904688768249668,0.949235840745,
0.992552407694861,1.),.UNSPECIFIED.);
#29630=B_SPLINE_CURVE_WITH_KNOTS('',3,(#124010,#124011,#124012,#124013,
#124014,#124015,#124016,#124017,#124018,#124019,#124020,#124021,#124022,
#124023,#124024,#124025,#124026,#124027,#124028,#124029,#124030,#124031,
#124032,#124033,#124034,#124035,#124036,#124037,#124038,#124039,#124040,
#124041,#124042,#124043,#124044,#124045,#124046,#124047,#124048,#124049,
#124050,#124051,#124052,#124053,#124054,#124055,#124056,#124057,#124058,
#124059,#124060,#124061,#124062,#124063,#124064,#124065,#124066,#124067,
#124068,#124069,#124070,#124071,#124072,#124073,#124074,#124075,#124076,
#124077,#124078,#124079,#124080,#124081,#124082,#124083,#124084,#124085,
#124086,#124087,#124088,#124089,#124090,#124091,#124092,#124093,#124094),
 .UNSPECIFIED.,.F.,.F.,(4,3,3,3,3,3,3,3,3,3,3,3,3,3,3,3,3,3,3,3,3,3,3,3,
3,3,3,3,4),(0.,0.0464234475031527,0.0972394848002348,0.124999999999925,
0.18293996388668,0.187499999999885,0.218749999999865,0.234374999999855,
0.242187499999853,0.246093749999855,0.249999999999857,0.312499999999872,
0.374999999999887,0.394398921641171,0.437499999999902,0.468749999999906,
0.484374999999908,0.495923412975398,0.49999999999991,0.569072679957118,
0.596914948823617,0.659857187217588,0.72408610632743,0.749999999999955,
0.79535387639268,0.860907736963063,0.93010399676668,0.998673877112228,0.999999999665933),
 .UNSPECIFIED.);
#29631=B_SPLINE_CURVE_WITH_KNOTS('',3,(#124143,#124144,#124145,#124146,
#124147,#124148,#124149,#124150,#124151,#124152,#124153,#124154,#124155,
#124156,#124157,#124158,#124159,#124160,#124161,#124162,#124163,#124164,
#124165,#124166,#124167,#124168,#124169,#124170,#124171,#124172,#124173,
#124174,#124175,#124176,#124177,#124178,#124179,#124180,#124181,#124182,
#124183,#124184,#124185,#124186,#124187,#124188,#124189,#124190,#124191,
#124192,#124193,#124194,#124195,#124196,#124197,#124198,#124199,#124200),
 .UNSPECIFIED.,.F.,.F.,(4,2,2,2,2,2,2,2,2,1,1,2,2,2,2,2,1,2,2,2,2,1,1,1,
2,2,2,2,2,2,2,4),(4.03773831338313E-9,0.125000000000036,0.187500000000054,
0.218750000000064,0.234375000000069,0.250000000000074,0.375000000000128,
0.437500000000155,0.468750000000169,0.484375000000176,0.492187500000179,
0.49609375000018,0.500000000000181,0.562500000000179,0.59375000000018,0.60156250000018,
0.609375000000181,0.62500000000018,0.656250000000178,0.671875000000176,
0.687500000000174,0.718750000000168,0.734375000000164,0.74218750000016,
0.746093750000158,0.750000000000155,0.812500000000121,0.820312500000117,
0.828125000000113,0.843750000000102,0.875000000000082,1.),.UNSPECIFIED.);
#29632=B_SPLINE_CURVE_WITH_KNOTS('',3,(#124263,#124264,#124265,#124266,
#124267,#124268,#124269,#124270,#124271,#124272),.UNSPECIFIED.,.F.,.F.,
(4,2,2,2,4),(-0.23344982273972,-0.179647450786024,-0.11659637991489,-0.0577031790998955,
-9.99999849621291E-7),.UNSPECIFIED.);
#29633=B_SPLINE_CURVE_WITH_KNOTS('',3,(#124273,#124274,#124275,#124276,
#124277,#124278,#124279,#124280,#124281,#124282,#124283,#124284,#124285,
#124286,#124287,#124288,#124289,#124290,#124291,#124292,#124293,#124294,
#124295,#124296,#124297,#124298,#124299,#124300,#124301,#124302,#124303,
#124304,#124305,#124306,#124307,#124308,#124309,#124310,#124311,#124312,
#124313,#124314,#124315,#124316,#124317,#124318,#124319,#124320,#124321,
#124322,#124323,#124324,#124325,#124326,#124327,#124328,#124329,#124330,
#124331,#124332,#124333,#124334,#124335,#124336,#124337,#124338,#124339,
#124340,#124341,#124342,#124343,#124344,#124345),.UNSPECIFIED.,.F.,.F.,
(4,3,3,3,3,3,3,3,3,3,3,3,3,3,3,3,3,3,3,3,3,3,3,3,4),(0.,0.12757222074774,
0.25000000000007,0.29760660917728,0.375000000000104,0.437500000000121,0.468750000000129,
0.484375000000132,0.492187500000134,0.496093750000137,0.500000000000139,
0.555888236349678,0.62500000000008,0.687500000000052,0.718750000000038,
0.734375000000033,0.742187500000031,0.74609375000003,0.750000000000029,
0.777889116176992,0.822699163900004,0.868116122275604,0.913783777296168,
0.959719246544919,1.),.UNSPECIFIED.);
#29634=B_SPLINE_CURVE_WITH_KNOTS('',3,(#124346,#124347,#124348,#124349,
#124350,#124351,#124352,#124353,#124354,#124355,#124356,#124357,#124358),
 .UNSPECIFIED.,.F.,.F.,(4,3,3,3,4),(0.,0.0494576143635624,0.0970068022307913,
0.1,0.12449382449223),.UNSPECIFIED.);
#29635=B_SPLINE_CURVE_WITH_KNOTS('',3,(#124366,#124367,#124368,#124369),
 .UNSPECIFIED.,.F.,.F.,(4,4),(0.,1.),.UNSPECIFIED.);
#29636=B_SPLINE_CURVE_WITH_KNOTS('',3,(#124370,#124371,#124372,#124373,
#124374,#124375,#124376,#124377,#124378,#124379,#124380,#124381,#124382,
#124383,#124384,#124385,#124386,#124387,#124388,#124389,#124390,#124391,
#124392,#124393,#124394,#124395,#124396,#124397,#124398,#124399,#124400,
#124401,#124402,#124403,#124404,#124405,#124406,#124407,#124408,#124409,
#124410,#124411,#124412,#124413,#124414,#124415,#124416,#124417,#124418),
 .UNSPECIFIED.,.F.,.F.,(4,3,3,3,3,3,3,3,3,3,3,3,3,3,3,3,4),(1.46675811174605E-9,
0.0686791264152932,0.136755536608584,0.20412240032792,0.25,0.3125,0.374509470854035,
0.437254735427017,0.5,0.5625,0.624427008921756,0.687213504460878,0.75,0.817395177031026,
0.885212462891086,0.953912866973348,1.),.UNSPECIFIED.);
#29637=B_SPLINE_CURVE_WITH_KNOTS('',3,(#124422,#124423,#124424,#124425,
#124426,#124427,#124428,#124429,#124430,#124431),.UNSPECIFIED.,.F.,.F.,
(4,2,2,2,4),(-0.726405805381144,-0.662305272963298,-0.598204740545452,-0.542164515818623,
-0.486124291091795),.UNSPECIFIED.);
#29638=B_SPLINE_CURVE_WITH_KNOTS('',3,(#124462,#124463,#124464,#124465,
#124466,#124467),.UNSPECIFIED.,.F.,.F.,(4,2,4),(0.,0.5,1.),
 .UNSPECIFIED.);
#29639=B_SPLINE_CURVE_WITH_KNOTS('',3,(#124535,#124536,#124537,#124538,
#124539,#124540,#124541,#124542,#124543,#124544,#124545,#124546,#124547,
#124548,#124549,#124550,#124551,#124552,#124553,#124554,#124555,#124556,
#124557,#124558,#124559,#124560,#124561,#124562,#124563,#124564,#124565,
#124566,#124567,#124568,#124569,#124570,#124571,#124572,#124573,#124574,
#124575,#124576,#124577,#124578,#124579,#124580),.UNSPECIFIED.,.F.,.F.,
(4,3,3,3,3,3,3,3,3,3,3,3,3,3,3,4),(0.,0.0589597084867831,0.119779732984347,
0.184889866492172,0.249999999999997,0.315933256860396,0.384199006139739,
0.437499999999991,0.466976182919735,0.496747691491063,0.499999999999988,
0.60353311268981,0.709573998306953,0.817048051970079,0.926891247804535,
0.999999998760338),.UNSPECIFIED.);
#29640=B_SPLINE_CURVE_WITH_KNOTS('',3,(#124581,#124582,#124583,#124584,
#124585,#124586,#124587,#124588,#124589,#124590,#124591,#124592,#124593,
#124594,#124595,#124596,#124597,#124598,#124599,#124600,#124601,#124602,
#124603,#124604,#124605,#124606,#124607,#124608,#124609,#124610,#124611,
#124612,#124613,#124614,#124615,#124616,#124617,#124618,#124619,#124620,
#124621,#124622,#124623,#124624,#124625,#124626,#124627,#124628,#124629,
#124630,#124631,#124632,#124633,#124634,#124635,#124636,#124637,#124638,
#124639,#124640,#124641,#124642,#124643,#124644,#124645,#124646,#124647,
#124648,#124649,#124650,#124651,#124652,#124653),.UNSPECIFIED.,.F.,.F.,
(4,3,3,3,3,3,3,3,3,3,3,3,3,3,3,3,3,3,3,3,3,3,3,3,4),(0.,0.0711144888714902,
0.0945275596457417,0.167636396974067,0.208716067427079,0.249999999999987,
0.320184542884328,0.374999999999986,0.431373619662498,0.437499999999988,
0.466325239000227,0.495576657133584,0.499999999999989,0.547812431517224,
0.611883700119326,0.663674500140904,0.722930038864494,0.749999999999994,
0.776562960482692,0.832323559435951,0.88400805595098,0.888084158389211,
0.939713999835979,0.99090756022988,1.),.UNSPECIFIED.);
#29641=B_SPLINE_CURVE_WITH_KNOTS('',3,(#124661,#124662,#124663,#124664,
#124665,#124666,#124667,#124668,#124669,#124670,#124671,#124672,#124673,
#124674,#124675,#124676,#124677,#124678,#124679,#124680,#124681,#124682,
#124683,#124684,#124685),.UNSPECIFIED.,.F.,.F.,(4,3,3,3,3,3,3,3,4),(0.,
0.0465847089982569,0.184218794802992,0.322341777280543,0.460351258074531,
0.592494069563406,0.725479240786321,0.862739620393161,1.),.UNSPECIFIED.);
#29642=B_SPLINE_CURVE_WITH_KNOTS('',3,(#124687,#124688,#124689,#124690,
#124691,#124692,#124693,#124694,#124695,#124696,#124697,#124698,#124699,
#124700,#124701,#124702,#124703,#124704,#124705),.UNSPECIFIED.,.F.,.F.,
(4,3,3,3,3,3,4),(3.48947356593272E-12,0.174977590683796,0.347502183077061,
0.516223131647767,0.682841488005358,0.846077647659188,1.),.UNSPECIFIED.);
#29643=B_SPLINE_CURVE_WITH_KNOTS('',3,(#124708,#124709,#124710,#124711,
#124712,#124713),.UNSPECIFIED.,.F.,.F.,(4,2,4),(2.51526495094515E-6,0.266858815172523,
0.535468336387855),.UNSPECIFIED.);
#29644=B_SPLINE_CURVE_WITH_KNOTS('',3,(#124719,#124720,#124721,#124722,
#124723,#124724),.UNSPECIFIED.,.F.,.F.,(4,2,4),(-0.194540442929235,-0.0972716515835901,
-9.99999999418133E-7),.UNSPECIFIED.);
#29645=B_SPLINE_CURVE_WITH_KNOTS('',3,(#124726,#124727,#124728,#124729,
#124730,#124731),.UNSPECIFIED.,.F.,.F.,(4,2,4),(-1.07453211284631,-0.509989083706148,
-4.22263312715382E-6),.UNSPECIFIED.);
#29646=B_SPLINE_CURVE_WITH_KNOTS('',3,(#124732,#124733,#124734,#124735,
#124736,#124737),.UNSPECIFIED.,.F.,.F.,(4,2,4),(-0.252023834669692,-0.127427092192949,
-2.00386101438639E-6),.UNSPECIFIED.);
#29647=B_SPLINE_CURVE_WITH_KNOTS('',3,(#124843,#124844,#124845,#124846,
#124847,#124848,#124849,#124850,#124851,#124852,#124853,#124854,#124855,
#124856,#124857,#124858,#124859,#124860,#124861,#124862,#124863,#124864,
#124865,#124866,#124867,#124868,#124869,#124870,#124871,#124872,#124873,
#124874,#124875,#124876,#124877,#124878,#124879,#124880,#124881,#124882,
#124883,#124884,#124885,#124886,#124887,#124888,#124889,#124890,#124891,
#124892,#124893,#124894,#124895,#124896,#124897,#124898,#124899,#124900,
#124901,#124902,#124903,#124904,#124905,#124906,#124907,#124908,#124909,
#124910,#124911,#124912,#124913,#124914,#124915,#124916,#124917,#124918,
#124919,#124920,#124921,#124922,#124923,#124924,#124925,#124926,#124927,
#124928,#124929,#124930,#124931,#124932,#124933,#124934,#124935,#124936,
#124937,#124938,#124939,#124940,#124941,#124942,#124943,#124944,#124945,
#124946,#124947,#124948,#124949,#124950,#124951,#124952,#124953,#124954,
#124955,#124956,#124957,#124958,#124959,#124960,#124961,#124962,#124963,
#124964,#124965,#124966,#124967,#124968,#124969,#124970,#124971,#124972,
#124973,#124974,#124975,#124976,#124977,#124978,#124979,#124980,#124981,
#124982,#124983,#124984,#124985,#124986,#124987,#124988,#124989,#124990,
#124991,#124992,#124993,#124994,#124995,#124996,#124997,#124998,#124999,
#125000,#125001,#125002,#125003,#125004,#125005),.UNSPECIFIED.,.F.,.F.,
(4,3,3,3,3,3,3,3,3,3,3,3,3,3,3,3,3,3,3,3,3,3,3,3,3,3,3,3,3,3,3,3,3,3,3,
3,3,3,3,3,3,3,3,3,3,3,3,3,3,3,3,3,3,3,4),(5.06083412936115E-12,0.0171539559720731,
0.0340650402423521,0.0505541415213171,0.0624999999999573,0.0696180872669653,
0.0855236320894016,0.100975672650675,0.109374999999926,0.117187499999921,
0.121093749999919,0.123046874999918,0.124023437499918,0.124999999999917,
0.13042801320028,0.15034045199903,0.17036742202076,0.190437495147897,0.198613274729677,
0.218301764397597,0.234374999999947,0.242187499999948,0.24609374999995,
0.248046874999951,0.249023437499951,0.24999999999995,0.28107801214436,0.322352060126167,
0.355872213215164,0.398801088383518,0.429267293437837,0.468749999999988,
0.48437499999999,0.49218749999999,0.49609374999999,0.499733967514589,0.499999999999991,
0.50367996751005,0.562817552938163,0.57466735513887,0.633872953101113,0.648359273799131,
0.687499999999987,0.718749999999986,0.725680974454021,0.734374999999985,
0.742187499999985,0.746093749999985,0.749999999999985,0.802396398205991,
0.856875204425067,0.877172016234362,0.932464864793394,0.951194936350549,
1.),.UNSPECIFIED.);
#29648=B_SPLINE_CURVE_WITH_KNOTS('',3,(#125050,#125051,#125052,#125053,
#125054,#125055,#125056,#125057),.UNSPECIFIED.,.F.,.F.,(4,1,1,1,1,4),(0.,
0.2,0.4,0.6,0.8,1.),.UNSPECIFIED.);
#29649=B_SPLINE_CURVE_WITH_KNOTS('',3,(#125058,#125059,#125060,#125061,
#125062,#125063,#125064,#125065,#125066,#125067,#125068,#125069,#125070,
#125071,#125072,#125073,#125074,#125075,#125076,#125077,#125078,#125079,
#125080,#125081,#125082,#125083,#125084,#125085,#125086,#125087,#125088),
 .UNSPECIFIED.,.F.,.F.,(4,3,3,3,3,3,3,3,3,3,4),(0.,0.136431436038453,0.269177825084775,
0.340888348203681,0.486556920879233,0.552216379427244,0.703562789808188,
0.762705775705736,0.91923339399344,0.967149486305342,0.999969191797008),
 .UNSPECIFIED.);
#29650=B_SPLINE_CURVE_WITH_KNOTS('',3,(#125198,#125199,#125200,#125201,
#125202,#125203,#125204,#125205,#125206,#125207,#125208,#125209,#125210,
#125211,#125212,#125213,#125214,#125215,#125216,#125217,#125218,#125219,
#125220,#125221,#125222,#125223,#125224,#125225,#125226,#125227,#125228,
#125229,#125230,#125231,#125232,#125233,#125234,#125235,#125236,#125237,
#125238,#125239,#125240,#125241,#125242,#125243,#125244,#125245,#125246,
#125247,#125248,#125249,#125250,#125251,#125252,#125253,#125254,#125255,
#125256,#125257,#125258,#125259,#125260,#125261,#125262,#125263,#125264,
#125265,#125266,#125267,#125268,#125269,#125270,#125271,#125272,#125273,
#125274,#125275,#125276,#125277,#125278,#125279,#125280,#125281,#125282,
#125283,#125284,#125285,#125286,#125287,#125288,#125289,#125290,#125291,
#125292,#125293,#125294,#125295,#125296,#125297,#125298,#125299,#125300),
 .UNSPECIFIED.,.F.,.F.,(4,3,3,3,3,3,3,3,3,3,3,3,3,3,3,3,3,3,3,3,3,3,3,3,
3,3,3,3,3,3,3,3,3,3,4),(0.,0.0548361818126014,0.06666666666667,0.069441502424314,
0.114564908225941,0.1333333333333,0.138885271670704,0.189448418695147,0.2,
0.208327253730071,0.259706436177619,0.2666666666667,0.277771362672896,0.330517828067452,
0.3333333333333,0.347212826950769,0.4,0.416644409960725,0.4666666666667,
0.486092163022652,0.5333333333333,0.555533216886878,0.6,0.624946427182303,
0.6666666666667,0.694406514328659,0.7333333333333,0.763870816800353,0.8,
0.833291783351506,0.8666666666667,0.902746432778773,0.9333333333333,0.9720818174012,
0.99999998908041),.UNSPECIFIED.);
#29651=B_SPLINE_CURVE_WITH_KNOTS('',3,(#125301,#125302,#125303,#125304,
#125305,#125306,#125307,#125308,#125309,#125310,#125311,#125312,#125313,
#125314,#125315,#125316,#125317,#125318,#125319,#125320,#125321,#125322,
#125323,#125324,#125325,#125326,#125327,#125328,#125329,#125330,#125331,
#125332,#125333,#125334,#125335,#125336,#125337,#125338,#125339,#125340,
#125341,#125342,#125343,#125344,#125345,#125346,#125347,#125348,#125349,
#125350,#125351,#125352,#125353,#125354,#125355,#125356,#125357,#125358,
#125359,#125360,#125361,#125362,#125363,#125364,#125365,#125366,#125367,
#125368,#125369,#125370,#125371,#125372,#125373,#125374,#125375,#125376,
#125377,#125378,#125379,#125380,#125381,#125382,#125383,#125384,#125385,
#125386,#125387,#125388,#125389,#125390,#125391,#125392,#125393,#125394,
#125395,#125396,#125397,#125398,#125399,#125400,#125401,#125402,#125403),
 .UNSPECIFIED.,.F.,.F.,(4,3,3,3,3,3,3,3,3,3,3,3,3,3,3,3,3,3,3,3,3,3,3,3,
3,3,3,3,3,3,3,3,3,3,4),(0.,0.0355393849942929,0.06666666666667,0.0694416969043181,
0.107940146958524,0.1333333333333,0.138885647269038,0.181937310148047,0.2,
0.208327299984056,0.254737431641626,0.2666666666667,0.277771268979535,0.326713057347023,
0.3333333333333,0.347212653366961,0.4,0.416644220166199,0.4666666666667,
0.486091967689304,0.5333333333333,0.555533081355431,0.6,0.624946070796763,
0.6666666666667,0.694405739054948,0.7333333333333,0.763869845720447,0.8,
0.833290765384722,0.8666666666667,0.902745177151871,0.9333333333333,0.972081604890996,
1.),.UNSPECIFIED.);
#29652=B_SPLINE_CURVE_WITH_KNOTS('',3,(#125510,#125511,#125512,#125513,
#125514,#125515,#125516,#125517,#125518,#125519,#125520,#125521,#125522,
#125523,#125524,#125525,#125526,#125527,#125528,#125529,#125530,#125531,
#125532,#125533,#125534,#125535,#125536,#125537,#125538,#125539,#125540,
#125541,#125542,#125543,#125544,#125545,#125546,#125547,#125548,#125549,
#125550,#125551,#125552,#125553,#125554,#125555,#125556,#125557,#125558,
#125559,#125560,#125561,#125562,#125563,#125564,#125565,#125566,#125567,
#125568,#125569,#125570,#125571,#125572,#125573,#125574,#125575,#125576,
#125577,#125578,#125579,#125580,#125581,#125582,#125583,#125584,#125585,
#125586,#125587,#125588,#125589,#125590,#125591,#125592,#125593,#125594,
#125595,#125596,#125597,#125598,#125599,#125600,#125601,#125602,#125603,
#125604,#125605,#125606,#125607,#125608,#125609,#125610,#125611,#125612,
#125613,#125614,#125615,#125616,#125617,#125618,#125619,#125620,#125621,
#125622,#125623,#125624,#125625,#125626,#125627,#125628,#125629,#125630,
#125631,#125632,#125633,#125634,#125635,#125636,#125637,#125638,#125639,
#125640,#125641,#125642,#125643,#125644,#125645,#125646,#125647,#125648,
#125649,#125650,#125651,#125652,#125653,#125654,#125655,#125656,#125657,
#125658,#125659,#125660,#125661,#125662,#125663,#125664,#125665,#125666,
#125667,#125668,#125669,#125670,#125671,#125672,#125673,#125674,#125675,
#125676,#125677,#125678,#125679,#125680,#125681,#125682,#125683,#125684),
 .UNSPECIFIED.,.F.,.F.,(4,3,3,3,3,3,3,3,3,3,3,3,3,3,3,3,3,3,3,3,3,3,3,3,
3,3,3,3,3,3,3,3,3,3,3,3,3,3,3,3,3,3,3,3,3,3,3,3,3,3,3,3,3,3,3,3,3,3,4),
(0.,0.0235492679861395,0.0472137911635587,0.0625000000000093,0.0822518681564539,
0.093750000000014,0.109375000000016,0.117187500000018,0.121093750000018,
0.124023437500019,0.125000000000019,0.154178375199939,0.178178863460657,
0.187500000000026,0.216538644948386,0.218750000000029,0.234375000000031,
0.242187500000032,0.246093750000032,0.249023437500033,0.250000000000033,
0.272786625660294,0.307326218844534,0.312500000000031,0.34375000000003,
0.359375000000029,0.367187500000029,0.367684567420504,0.374023437500029,
0.375000000000029,0.406250000000027,0.421875000000026,0.4310209687631,0.437500000000026,
0.464080358294731,0.500000000000023,0.531250000000021,0.54687500000002,
0.556871877293205,0.557630128037314,0.56250000000002,0.593750000000018,
0.610383926884643,0.625000000000017,0.653411097831424,0.687500000000013,
0.718750000000012,0.734375000000011,0.74218750000001,0.748042269832564,
0.749392484289949,0.75000000000001,0.795146546828096,0.840684774852451,
0.847431192599437,0.894737435067752,0.942043677536068,0.987527628774997,
0.999999716407811),.UNSPECIFIED.);
#29653=B_SPLINE_CURVE_WITH_KNOTS('',3,(#125686,#125687,#125688,#125689,
#125690,#125691,#125692,#125693,#125694,#125695,#125696,#125697,#125698,
#125699,#125700,#125701,#125702,#125703,#125704,#125705,#125706,#125707,
#125708,#125709,#125710,#125711,#125712,#125713,#125714,#125715,#125716,
#125717,#125718,#125719,#125720,#125721,#125722,#125723,#125724,#125725,
#125726,#125727,#125728,#125729,#125730,#125731,#125732,#125733,#125734,
#125735,#125736,#125737),.UNSPECIFIED.,.F.,.F.,(4,3,3,3,3,3,3,3,3,3,3,3,
3,3,3,3,3,4),(2.99130189936697E-13,0.126968394289133,0.249999999999985,
0.329706325480795,0.374999999999978,0.437499999999975,0.468749999999973,
0.484374999999973,0.492187499999972,0.498046874999972,0.499999999999971,
0.582586360741502,0.654012877805904,0.737251808022353,0.821597889449064,
0.907434469096319,0.933231048795402,1.),.UNSPECIFIED.);
#29654=B_SPLINE_CURVE_WITH_KNOTS('',3,(#125738,#125739,#125740,#125741,
#125742,#125743,#125744,#125745,#125746,#125747,#125748,#125749,#125750,
#125751,#125752,#125753,#125754,#125755,#125756,#125757,#125758,#125759,
#125760,#125761,#125762,#125763,#125764,#125765,#125766,#125767,#125768,
#125769,#125770,#125771,#125772,#125773,#125774,#125775,#125776,#125777,
#125778,#125779,#125780,#125781,#125782,#125783,#125784,#125785,#125786,
#125787,#125788,#125789,#125790,#125791,#125792,#125793,#125794,#125795,
#125796,#125797,#125798,#125799,#125800,#125801,#125802,#125803,#125804,
#125805,#125806,#125807,#125808,#125809,#125810,#125811,#125812,#125813,
#125814,#125815,#125816,#125817,#125818,#125819,#125820,#125821,#125822,
#125823,#125824,#125825,#125826,#125827,#125828,#125829,#125830,#125831,
#125832,#125833,#125834,#125835,#125836,#125837,#125838,#125839,#125840),
 .UNSPECIFIED.,.F.,.F.,(4,3,3,3,3,3,3,3,3,3,3,3,3,3,3,3,3,3,3,3,3,3,3,3,
3,3,3,3,3,3,3,3,3,3,4),(0.,0.0624999999999969,0.0937499999999951,0.109374999999994,
0.117187499999994,0.121093749999994,0.123046874999994,0.123242106419626,
0.124999999999993,0.163746701278836,0.20166480609802,0.218750000000004,
0.234375000000005,0.242187500000006,0.246093750000006,0.248046875000006,
0.250000000000006,0.290663556421084,0.352736974639709,0.415434775032593,
0.4375,0.468749999999998,0.478234768091092,0.484374999999998,0.492187499999998,
0.496093749999998,0.499999999999998,0.579044129469348,0.657254873091502,
0.674737829808071,0.749999999999999,0.828546295365536,0.889501455477367,
0.968672694605542,1.),.UNSPECIFIED.);
#29655=B_SPLINE_CURVE_WITH_KNOTS('',3,(#125899,#125900,#125901,#125902,
#125903,#125904,#125905,#125906,#125907,#125908,#125909,#125910,#125911,
#125912,#125913,#125914,#125915,#125916,#125917,#125918,#125919,#125920,
#125921,#125922,#125923,#125924,#125925,#125926,#125927,#125928,#125929,
#125930),.UNSPECIFIED.,.F.,.F.,(4,1,1,1,1,1,1,1,1,1,1,1,1,1,1,1,1,1,1,1,
1,1,1,1,1,1,1,1,1,4),(0.,0.0268581202847227,0.053576525889946,0.0801578745940373,
0.106606641707507,0.132924195530782,0.159110310690199,0.185166065577177,
0.211093744297133,0.236896651377879,0.262577255427033,0.288136464224189,
0.313575794895345,0.338897466804712,0.364104280017708,0.389198781870568,
0.414183265290867,0.439060365533827,0.463833043802139,0.495403201210392,
0.587316390229939,0.642835451771974,0.704686515759081,0.772883347569249,
0.814032578447846,0.853827591278796,0.892297474609331,0.929469891075696,
0.965365253976918,1.),.UNSPECIFIED.);
#29656=B_SPLINE_CURVE_WITH_KNOTS('',3,(#126050,#126051,#126052,#126053,
#126054,#126055,#126056,#126057,#126058,#126059,#126060,#126061,#126062,
#126063,#126064,#126065),.UNSPECIFIED.,.F.,.F.,(4,3,3,3,3,4),(0.,0.221610690796373,
0.437664957226359,0.651285519899787,0.862133513064776,0.999985703601229),
 .UNSPECIFIED.);
#29657=B_SPLINE_CURVE_WITH_KNOTS('',3,(#126125,#126126,#126127,#126128,
#126129,#126130,#126131,#126132,#126133,#126134,#126135,#126136,#126137,
#126138,#126139,#126140,#126141,#126142,#126143,#126144,#126145,#126146,
#126147,#126148,#126149,#126150,#126151,#126152,#126153,#126154,#126155,
#126156,#126157,#126158,#126159,#126160,#126161,#126162,#126163,#126164,
#126165,#126166,#126167,#126168,#126169,#126170,#126171,#126172,#126173,
#126174,#126175,#126176,#126177,#126178,#126179,#126180,#126181,#126182,
#126183,#126184,#126185,#126186,#126187,#126188,#126189,#126190,#126191,
#126192,#126193,#126194,#126195,#126196,#126197,#126198,#126199,#126200,
#126201,#126202,#126203,#126204,#126205,#126206,#126207,#126208,#126209,
#126210,#126211,#126212),.UNSPECIFIED.,.F.,.F.,(4,3,3,3,3,3,3,3,3,3,3,3,
3,3,3,3,3,3,3,3,3,3,3,3,3,3,3,3,3,4),(0.,1.36955922228348E-5,0.0462209864660522,
0.0923085477371591,0.138396109008266,0.249999999999993,0.275014435602624,
0.344752712976046,0.414490990349467,0.437499999999987,0.468749999999986,
0.484374999999986,0.492187499999986,0.496093749999986,0.499999999999987,
0.552744721211975,0.620122360605994,0.687500000000013,0.691683644659851,
0.718750000000017,0.73437500000002,0.742187500000021,0.748046875000022,
0.750000000000022,0.813958948873022,0.829406161009669,0.895045917261246,
0.957116251376177,0.972386509597121,0.999999999927525),.UNSPECIFIED.);
#29658=B_SPLINE_CURVE_WITH_KNOTS('',3,(#126232,#126233,#126234,#126235,
#126236,#126237,#126238,#126239,#126240,#126241,#126242,#126243,#126244,
#126245,#126246,#126247,#126248,#126249,#126250,#126251,#126252,#126253,
#126254,#126255,#126256,#126257,#126258,#126259,#126260,#126261,#126262,
#126263,#126264,#126265,#126266,#126267,#126268,#126269,#126270,#126271,
#126272,#126273,#126274,#126275,#126276,#126277,#126278,#126279,#126280,
#126281,#126282,#126283,#126284,#126285,#126286,#126287,#126288,#126289,
#126290,#126291,#126292,#126293,#126294,#126295,#126296,#126297,#126298,
#126299,#126300,#126301,#126302,#126303,#126304,#126305,#126306,#126307,
#126308,#126309,#126310,#126311,#126312,#126313,#126314,#126315,#126316,
#126317,#126318,#126319,#126320,#126321,#126322,#126323,#126324,#126325,
#126326,#126327,#126328,#126329,#126330,#126331,#126332,#126333,#126334,
#126335,#126336,#126337,#126338,#126339,#126340,#126341,#126342,#126343,
#126344,#126345,#126346,#126347,#126348,#126349,#126350,#126351,#126352,
#126353,#126354,#126355),.UNSPECIFIED.,.F.,.F.,(4,3,3,3,3,3,3,3,3,3,3,3,
3,3,3,3,3,3,3,3,3,3,3,3,3,3,3,3,3,3,3,3,3,3,3,3,3,3,3,3,3,4),(0.,0.0340829424126167,
0.0691949614776787,0.105776364582913,0.117363353323133,0.125000000000056,
0.160169501196136,0.187500000000084,0.218750000000098,0.234375000000105,
0.242187500000108,0.246093750000108,0.250000000000108,0.285436053496591,
0.309021515795873,0.343531233663922,0.378569260057507,0.413942671359278,
0.44921700327509,0.483961412343902,0.500000000000092,0.500003316427969,
0.534823892860835,0.570002258034842,0.605300618146352,0.625000000000085,
0.659693928278741,0.68750000000008,0.691017580435165,0.718750000000077,
0.734375000000075,0.742187500000074,0.746093750000073,0.750000000000071,
0.787162851469644,0.823724950689069,0.8590520932407,0.882627289955567,0.918401461247141,
0.953211128280996,0.986563735801074,1.),.UNSPECIFIED.);
#29659=B_SPLINE_CURVE_WITH_KNOTS('',3,(#126358,#126359,#126360,#126361,
#126362,#126363,#126364,#126365,#126366,#126367,#126368,#126369,#126370,
#126371),.UNSPECIFIED.,.F.,.F.,(4,2,2,1,1,2,2,4),(0.,0.249999999999985,
0.37499999999998,0.437499999999977,0.468749999999975,0.484374999999977,
0.499999999999978,0.999999993863134),.UNSPECIFIED.);
#29660=B_SPLINE_CURVE_WITH_KNOTS('',3,(#126373,#126374,#126375,#126376,
#126377,#126378,#126379,#126380,#126381,#126382,#126383,#126384,#126385,
#126386),.UNSPECIFIED.,.F.,.F.,(4,2,2,1,1,2,2,4),(0.,0.249999999999981,
0.37499999999997,0.437499999999966,0.468749999999966,0.484374999999966,
0.499999999999966,1.),.UNSPECIFIED.);
#29661=B_SPLINE_CURVE_WITH_KNOTS('',3,(#126390,#126391,#126392,#126393,
#126394,#126395,#126396,#126397,#126398,#126399,#126400,#126401,#126402,
#126403,#126404,#126405,#126406,#126407,#126408),.UNSPECIFIED.,.F.,.F.,
(4,3,3,3,3,3,4),(0.,0.250000000000009,0.375000000000016,0.437500000000016,
0.500000000000016,0.753487667768314,1.),.UNSPECIFIED.);
#29662=B_SPLINE_CURVE_WITH_KNOTS('',3,(#126412,#126413,#126414,#126415,
#126416,#126417,#126418,#126419,#126420,#126421,#126422,#126423,#126424,
#126425,#126426,#126427,#126428,#126429,#126430,#126431,#126432,#126433,
#126434,#126435,#126436,#126437,#126438,#126439,#126440,#126441,#126442,
#126443,#126444,#126445,#126446,#126447,#126448,#126449,#126450,#126451,
#126452,#126453,#126454,#126455,#126456,#126457,#126458,#126459,#126460,
#126461,#126462,#126463,#126464,#126465,#126466,#126467,#126468,#126469,
#126470,#126471,#126472,#126473,#126474,#126475,#126476,#126477,#126478,
#126479,#126480,#126481,#126482,#126483,#126484,#126485,#126486,#126487,
#126488,#126489,#126490,#126491,#126492,#126493,#126494,#126495,#126496,
#126497,#126498,#126499,#126500,#126501,#126502,#126503,#126504,#126505,
#126506,#126507,#126508,#126509,#126510,#126511,#126512,#126513,#126514,
#126515,#126516,#126517,#126518,#126519,#126520,#126521,#126522,#126523,
#126524,#126525,#126526,#126527,#126528,#126529,#126530,#126531,#126532),
 .UNSPECIFIED.,.F.,.F.,(4,3,3,3,3,3,3,3,3,3,3,3,3,3,3,3,3,3,3,3,3,3,3,3,
3,3,3,3,3,3,3,3,3,3,3,3,3,3,3,3,4),(1.35350574291754E-11,0.0307091849465562,
0.0778545924732743,0.124999999999992,0.155534322638056,0.18749999999999,
0.218749999999991,0.234374999999991,0.2452894568283,0.249999999999992,0.280109082038762,
0.327554541019382,0.375000000000003,0.40543633558073,0.437500000000006,
0.468750000000008,0.48437500000001,0.492187500000014,0.496093750000014,
0.498046875000011,0.500000000000009,0.525870094542647,0.579929503357328,
0.624999999999902,0.644130534816122,0.687499999999847,0.718749999999819,
0.734374999999805,0.742187499999796,0.74609374999979,0.749023437499785,
0.749999999999784,0.77607790488667,0.805973888385761,0.836642472345653,
0.868991593120488,0.895661838883031,0.927139320876192,0.960297481709551,
0.995806785180928,0.999999984939203),.UNSPECIFIED.);
#29663=B_SPLINE_CURVE_WITH_KNOTS('',3,(#126534,#126535,#126536,#126537,
#126538,#126539,#126540,#126541,#126542,#126543,#126544,#126545,#126546,
#126547,#126548,#126549,#126550,#126551,#126552,#126553),.UNSPECIFIED.,
 .F.,.F.,(4,2,2,2,1,1,1,1,2,2,2,4),(0.,0.249999999999962,0.374999999999941,
0.437499999999932,0.468749999999929,0.484374999999928,0.492187499999926,
0.496093749999923,0.49804687499992,0.499999999999918,0.749999999999959,
1.),.UNSPECIFIED.);
#29664=B_SPLINE_CURVE_WITH_KNOTS('',3,(#126556,#126557,#126558,#126559,
#126560,#126561,#126562,#126563,#126564,#126565,#126566,#126567,#126568,
#126569,#126570,#126571,#126572,#126573,#126574),.UNSPECIFIED.,.F.,.F.,
(4,3,3,3,3,3,4),(0.,0.249999999999981,0.374999999999971,0.43749999999997,
0.499999999999968,0.749999999760635,0.999999999521302),.UNSPECIFIED.);
#29665=B_SPLINE_CURVE_WITH_KNOTS('',3,(#126619,#126620,#126621,#126622,
#126623,#126624,#126625,#126626,#126627,#126628),.UNSPECIFIED.,.F.,.F.,
(4,2,2,2,4),(0.,0.25,0.5,0.75,1.),.UNSPECIFIED.);
#29666=B_SPLINE_CURVE_WITH_KNOTS('',3,(#126629,#126630,#126631,#126632,
#126633,#126634,#126635,#126636,#126637,#126638,#126639,#126640,#126641,
#126642,#126643,#126644,#126645,#126646,#126647,#126648,#126649,#126650,
#126651,#126652,#126653),.UNSPECIFIED.,.F.,.F.,(4,2,2,2,2,2,2,1,1,1,2,2,
2,4),(0.,0.125000000000013,0.187500000000021,0.250000000000029,0.375000000000041,
0.437500000000047,0.468750000000048,0.48437500000005,0.492187500000048,
0.49609375000005,0.498046875000053,0.500000000000057,0.750000000000028,
1.),.UNSPECIFIED.);
#29667=B_SPLINE_CURVE_WITH_KNOTS('',3,(#126735,#126736,#126737,#126738,
#126739,#126740,#126741,#126742,#126743,#126744,#126745,#126746,#126747,
#126748,#126749,#126750,#126751,#126752,#126753,#126754,#126755,#126756,
#126757,#126758,#126759,#126760,#126761,#126762,#126763,#126764,#126765,
#126766,#126767,#126768,#126769,#126770,#126771,#126772,#126773,#126774,
#126775,#126776,#126777,#126778,#126779,#126780,#126781,#126782,#126783,
#126784,#126785,#126786,#126787,#126788,#126789,#126790,#126791,#126792,
#126793,#126794,#126795,#126796,#126797,#126798,#126799,#126800,#126801,
#126802,#126803,#126804,#126805,#126806,#126807,#126808,#126809,#126810,
#126811,#126812,#126813,#126814,#126815,#126816,#126817,#126818,#126819,
#126820,#126821,#126822,#126823,#126824,#126825,#126826,#126827,#126828,
#126829,#126830,#126831,#126832,#126833,#126834,#126835,#126836,#126837,
#126838,#126839,#126840,#126841,#126842,#126843,#126844,#126845,#126846,
#126847,#126848,#126849,#126850,#126851,#126852,#126853,#126854,#126855,
#126856,#126857,#126858,#126859,#126860,#126861,#126862,#126863,#126864,
#126865,#126866,#126867,#126868,#126869,#126870,#126871,#126872,#126873,
#126874,#126875,#126876,#126877,#126878,#126879,#126880,#126881,#126882,
#126883,#126884,#126885,#126886,#126887,#126888,#126889,#126890,#126891,
#126892,#126893,#126894,#126895,#126896,#126897,#126898,#126899,#126900,
#126901,#126902,#126903,#126904,#126905,#126906,#126907,#126908,#126909,
#126910,#126911,#126912,#126913,#126914,#126915,#126916,#126917,#126918,
#126919,#126920,#126921,#126922,#126923,#126924,#126925,#126926,#126927,
#126928,#126929,#126930,#126931,#126932,#126933,#126934,#126935,#126936,
#126937,#126938,#126939,#126940,#126941,#126942,#126943,#126944,#126945,
#126946,#126947,#126948),.UNSPECIFIED.,.F.,.F.,(4,3,3,3,3,3,3,3,3,3,3,3,
3,3,3,3,3,3,3,3,3,3,3,3,3,3,3,3,3,3,3,3,3,3,3,3,3,3,3,3,3,3,3,3,3,3,3,3,
3,3,3,3,3,3,3,3,3,3,3,3,3,3,3,3,3,3,3,3,3,3,3,4),(0.,0.0282178331377545,
0.0561330259963789,0.0834964584640116,0.105856518636603,0.124999999999945,
0.157071974609684,0.187499999999919,0.203569253523847,0.218749999999905,
0.234374999999898,0.242187499999895,0.246093749999893,0.248046874999891,
0.249755859374893,0.249999999999893,0.267047585275722,0.284291037965404,
0.30185817244769,0.308180029008359,0.31249999999989,0.328204075134219,0.344328892806464,
0.348280256700363,0.364286610611002,0.374999999999886,0.388280152658778,
0.404495028033477,0.421258823707265,0.435513775269351,0.437499999999883,
0.454742790478908,0.468749999999881,0.484374999999881,0.490871007459825,
0.492187499999882,0.496093749999883,0.49909253482406,0.499999999999883,
0.518016063137528,0.535457441797552,0.545566661066867,0.562499999999891,
0.579018449955007,0.5921657794438,0.608582889721849,0.624999999999898,0.635193611489272,
0.651282564283057,0.666884015919654,0.679131883867457,0.687499999999906,
0.704012137647359,0.71874999999991,0.724717457344516,0.734374999999912,
0.742187499999913,0.746093749999914,0.748046874999915,0.749023437499915,
0.749755859374914,0.749999999999914,0.776532649485828,0.78835186737661,
0.818021368597962,0.848252842493185,0.874999999999957,0.891177430866168,
0.918383073149626,0.945148095559187,0.972574047779593,0.999999999999999),
 .UNSPECIFIED.);
#29668=B_SPLINE_CURVE_WITH_KNOTS('',3,(#126975,#126976,#126977,#126978,
#126979,#126980,#126981,#126982,#126983,#126984,#126985,#126986,#126987,
#126988,#126989,#126990,#126991,#126992,#126993,#126994,#126995,#126996,
#126997,#126998,#126999,#127000,#127001,#127002,#127003,#127004,#127005,
#127006,#127007,#127008,#127009,#127010,#127011,#127012,#127013,#127014,
#127015,#127016,#127017,#127018,#127019,#127020,#127021,#127022,#127023,
#127024,#127025,#127026,#127027,#127028,#127029,#127030,#127031,#127032),
 .UNSPECIFIED.,.F.,.F.,(4,3,3,3,3,3,3,3,3,3,3,3,3,3,3,3,3,3,3,4),(2.46876960649128E-9,
0.0537367748554289,0.107910543359844,0.162445165998166,0.217710133013511,
0.25,0.304280929502245,0.325898769308603,0.382277994389015,0.441138997194507,
0.5,0.565029573834012,0.631575019684094,0.701212572652556,0.727536024996926,
0.75,0.829317054604299,0.908964390223096,0.988919926273896,1.),
 .UNSPECIFIED.);
#29669=B_SPLINE_CURVE_WITH_KNOTS('',3,(#127059,#127060,#127061,#127062,
#127063,#127064,#127065,#127066,#127067,#127068,#127069,#127070,#127071,
#127072,#127073,#127074,#127075,#127076,#127077,#127078,#127079,#127080,
#127081,#127082,#127083,#127084,#127085,#127086,#127087,#127088,#127089,
#127090,#127091,#127092,#127093,#127094,#127095,#127096,#127097,#127098,
#127099,#127100,#127101,#127102,#127103,#127104,#127105,#127106,#127107,
#127108,#127109,#127110,#127111,#127112,#127113,#127114,#127115,#127116,
#127117,#127118,#127119),.UNSPECIFIED.,.F.,.F.,(4,3,3,3,3,3,3,3,3,3,3,3,
3,3,3,3,3,3,3,3,4),(0.,0.0796513800767319,0.159044881296861,0.237895722259121,
0.25,0.280665700157712,0.349440429576461,0.416025348655478,0.480364738776273,
0.5,0.557540039378102,0.614137632699517,0.669697924521297,0.689732568620921,
0.743461700114881,0.75,0.805599575422341,0.860273458499742,0.914519873462587,
0.968307205903025,1.),.UNSPECIFIED.);
#29670=B_SPLINE_CURVE_WITH_KNOTS('',3,(#127146,#127147,#127148,#127149,
#127150,#127151,#127152,#127153,#127154,#127155,#127156),.UNSPECIFIED.,
 .F.,.F.,(4,1,1,1,1,1,1,1,4),(0.,0.125,0.25,0.375,0.5,0.625,0.75,0.875,
1.),.UNSPECIFIED.);
#29671=B_SPLINE_CURVE_WITH_KNOTS('',3,(#127207,#127208,#127209,#127210,
#127211,#127212,#127213,#127214,#127215,#127216,#127217,#127218,#127219,
#127220,#127221,#127222,#127223,#127224,#127225,#127226,#127227,#127228,
#127229,#127230,#127231,#127232,#127233,#127234,#127235,#127236,#127237,
#127238,#127239,#127240,#127241,#127242,#127243,#127244,#127245,#127246,
#127247,#127248,#127249,#127250,#127251,#127252,#127253,#127254,#127255,
#127256,#127257,#127258,#127259,#127260,#127261,#127262,#127263,#127264,
#127265,#127266,#127267,#127268,#127269,#127270,#127271,#127272,#127273,
#127274,#127275,#127276,#127277,#127278,#127279,#127280,#127281,#127282,
#127283,#127284,#127285,#127286,#127287,#127288,#127289,#127290,#127291,
#127292,#127293,#127294,#127295,#127296,#127297,#127298,#127299,#127300,
#127301,#127302,#127303,#127304,#127305,#127306,#127307,#127308,#127309,
#127310,#127311,#127312,#127313,#127314,#127315,#127316,#127317,#127318,
#127319,#127320,#127321,#127322,#127323,#127324,#127325,#127326,#127327,
#127328,#127329,#127330,#127331,#127332,#127333,#127334,#127335,#127336,
#127337,#127338,#127339,#127340,#127341,#127342,#127343,#127344,#127345,
#127346,#127347,#127348,#127349,#127350,#127351,#127352,#127353,#127354,
#127355,#127356,#127357),.UNSPECIFIED.,.F.,.F.,(4,3,3,3,3,3,3,3,3,3,3,3,
3,3,3,3,3,3,3,3,3,3,3,3,3,3,3,3,3,3,3,3,3,3,3,3,3,3,3,3,3,3,3,3,3,3,3,3,
3,3,4),(3.37531681360733E-8,0.017205386283455,0.0344007668864576,0.0514925949099461,
0.0625000000003226,0.0788325765450556,0.093750000000486,0.109375000000568,
0.117187500000608,0.121093750000628,0.123046875000637,0.124023437500642,
0.124511718750645,0.125000000000647,0.132155380101528,0.154901536392429,
0.177338716362301,0.187500000000683,0.209154443768504,0.218750000000699,
0.234375000000707,0.242187500000711,0.246093750000714,0.248046875000715,
0.250000000000715,0.275941425824807,0.321226396871429,0.367758215452313,
0.375000000000597,0.401097960541236,0.437500000000536,0.468750000000505,
0.484375000000489,0.494714665161877,0.500000000000472,0.532447775598141,
0.586688269433701,0.638600054374137,0.652704130622242,0.701352065311238,
0.750000000000234,0.769959744739266,0.808596168225151,0.845577084750668,
0.875000000000117,0.879285832015869,0.909685991152717,0.939197353512371,
0.96748243414976,0.977540640360751,1.),.UNSPECIFIED.);
#29672=B_SPLINE_CURVE_WITH_KNOTS('',3,(#127392,#127393,#127394,#127395,
#127396,#127397,#127398,#127399,#127400,#127401,#127402,#127403,#127404,
#127405,#127406,#127407,#127408,#127409,#127410,#127411,#127412,#127413,
#127414,#127415,#127416,#127417,#127418,#127419,#127420,#127421,#127422,
#127423,#127424),.UNSPECIFIED.,.F.,.F.,(4,2,2,2,1,1,1,1,2,2,2,2,2,1,1,1,
2,2,2,4),(0.,0.250000000000239,0.375000000000361,0.437500000000424,0.468750000000454,
0.484375000000468,0.492187500000475,0.49609375000048,0.499023437500488,
0.500000000000492,0.625000000000438,0.687500000000413,0.7187500000004,0.734375000000394,
0.742187500000391,0.746093750000391,0.748046875000389,0.750000000000388,
0.875000000000194,1.),.UNSPECIFIED.);
#29673=B_SPLINE_CURVE_WITH_KNOTS('',3,(#127449,#127450,#127451,#127452,
#127453,#127454,#127455,#127456,#127457,#127458,#127459,#127460,#127461,
#127462,#127463,#127464,#127465,#127466,#127467,#127468,#127469,#127470,
#127471,#127472,#127473,#127474,#127475,#127476,#127477,#127478,#127479,
#127480,#127481,#127482,#127483,#127484,#127485,#127486,#127487,#127488),
 .UNSPECIFIED.,.F.,.F.,(4,3,3,3,3,3,3,3,3,3,3,3,3,4),(6.02213740706731E-7,
0.18780417571379,0.250000000000018,0.279295317709131,0.375000000000028,
0.437500000000024,0.468750000000018,0.493606973159941,0.500000000000012,
0.628564160145021,0.732916122017548,0.858621496952094,0.982199270722659,
1.),.UNSPECIFIED.);
#29674=B_SPLINE_CURVE_WITH_KNOTS('',3,(#127560,#127561,#127562,#127563,
#127564,#127565,#127566,#127567,#127568,#127569,#127570,#127571,#127572,
#127573,#127574,#127575,#127576,#127577,#127578,#127579,#127580,#127581,
#127582,#127583,#127584,#127585,#127586,#127587,#127588,#127589,#127590,
#127591,#127592,#127593,#127594,#127595,#127596,#127597,#127598,#127599,
#127600,#127601,#127602,#127603,#127604,#127605,#127606,#127607,#127608,
#127609,#127610,#127611,#127612,#127613,#127614,#127615,#127616,#127617,
#127618,#127619,#127620,#127621,#127622,#127623,#127624,#127625,#127626,
#127627,#127628,#127629,#127630,#127631,#127632,#127633,#127634,#127635,
#127636,#127637,#127638,#127639,#127640,#127641,#127642,#127643,#127644),
 .UNSPECIFIED.,.F.,.F.,(4,3,3,3,3,3,3,3,3,3,3,3,3,3,3,3,3,3,3,3,3,3,3,3,
3,3,3,3,4),(4.27405454084845E-15,0.0377356474346085,0.0750359183061167,
0.112014973382717,0.148784553462517,0.185454708791789,0.222134505689713,
0.259084364535886,0.296281779750846,0.333825646041853,0.371816608292509,
0.410693571800077,0.450151209830871,0.490604164912764,0.499999883639221,
0.540309510288622,0.579736856800223,0.618411911999041,0.656459211909535,
0.693998732295002,0.732248890758127,0.769066832852564,0.805766270350655,
0.842443980674244,0.879196581460098,0.916274247721184,0.953595787795862,
0.991423223558937,1.),.UNSPECIFIED.);
#29675=B_SPLINE_CURVE_WITH_KNOTS('',3,(#127969,#127970,#127971,#127972,
#127973,#127974,#127975,#127976,#127977,#127978,#127979,#127980,#127981,
#127982,#127983,#127984,#127985,#127986),.UNSPECIFIED.,.F.,.F.,(4,2,2,2,
2,2,2,2,4),(0.,0.125,0.25,0.375,0.5,0.625,0.75,0.875,1.),.UNSPECIFIED.);
#29676=B_SPLINE_CURVE_WITH_KNOTS('',3,(#128290,#128291,#128292,#128293,
#128294,#128295,#128296,#128297,#128298,#128299,#128300,#128301,#128302,
#128303,#128304,#128305,#128306,#128307),.UNSPECIFIED.,.F.,.F.,(4,2,2,2,
2,2,2,2,4),(0.,0.125,0.25,0.375,0.5,0.625,0.75,0.875,1.),.UNSPECIFIED.);
#29677=B_SPLINE_CURVE_WITH_KNOTS('',3,(#128441,#128442,#128443,#128444,
#128445,#128446,#128447,#128448,#128449,#128450,#128451,#128452,#128453,
#128454,#128455,#128456,#128457,#128458,#128459,#128460,#128461,#128462,
#128463,#128464,#128465,#128466,#128467,#128468,#128469,#128470,#128471,
#128472,#128473,#128474,#128475,#128476,#128477,#128478,#128479,#128480,
#128481,#128482,#128483,#128484,#128485,#128486,#128487,#128488,#128489,
#128490,#128491,#128492,#128493,#128494,#128495,#128496,#128497,#128498,
#128499,#128500,#128501,#128502,#128503,#128504,#128505,#128506,#128507,
#128508,#128509,#128510,#128511,#128512,#128513,#128514,#128515,#128516,
#128517,#128518,#128519,#128520,#128521,#128522),.UNSPECIFIED.,.F.,.F.,
(4,3,3,3,3,3,3,3,3,3,3,3,3,3,3,3,3,3,3,3,3,3,3,3,3,3,3,4),(0.,0.0394358656769841,
0.0785691055717362,0.11744545980691,0.125,0.163728602867978,0.203692449020046,
0.242758028571359,0.282103574403945,0.321833855203582,0.362445642816848,
0.403594461611848,0.445876068134623,0.483439372084522,0.52606025705519,
0.569677724923291,0.610226588911753,0.650200831769538,0.689710220697424,
0.728861943519438,0.767724842093286,0.806475376386791,0.84527239412539,
0.875,0.914134277322075,0.953517865253058,0.993412874544988,1.),
 .UNSPECIFIED.);
#29678=B_SPLINE_CURVE_WITH_KNOTS('',3,(#128609,#128610,#128611,#128612,
#128613,#128614,#128615,#128616,#128617,#128618,#128619,#128620,#128621,
#128622),.UNSPECIFIED.,.F.,.F.,(4,2,2,2,2,2,4),(-1.00304124093577,-0.900314725496988,
-0.794873156144138,-0.612050855402291,-0.374992741653492,-0.188195460796421,
-0.000330903306112853),.UNSPECIFIED.);
#29679=B_SPLINE_CURVE_WITH_KNOTS('',3,(#128624,#128625,#128626,#128627,
#128628,#128629,#128630,#128631,#128632,#128633),.UNSPECIFIED.,.F.,.F.,
(4,2,2,2,4),(-0.66037468527763,-0.531312380184094,-0.402225004171424,-0.237342302443342,
-0.00010611583071703),.UNSPECIFIED.);
#29680=B_SPLINE_CURVE_WITH_KNOTS('',3,(#128634,#128635,#128636,#128637,
#128638,#128639,#128640,#128641,#128642,#128643,#128644,#128645,#128646,
#128647),.UNSPECIFIED.,.F.,.F.,(4,2,2,2,2,2,4),(-1.42617023783195,-1.24379379176015,
-1.06262174742879,-0.713770494942383,-0.373736089754977,-0.185591640376111,
-0.00031726611114529),.UNSPECIFIED.);
#29681=B_SPLINE_CURVE_WITH_KNOTS('',3,(#128693,#128694,#128695,#128696,
#128697,#128698,#128699,#128700,#128701,#128702,#128703,#128704,#128705,
#128706,#128707,#128708,#128709,#128710,#128711,#128712,#128713,#128714,
#128715,#128716,#128717,#128718,#128719,#128720),.UNSPECIFIED.,.F.,.F.,
(4,2,2,2,2,2,2,2,2,2,2,2,2,4),(2.58033318348083E-7,0.125000000000001,0.250000000000002,
0.281250000000002,0.312500000000001,0.437499999999999,0.499999999999998,
0.593749999999996,0.624999999999996,0.749999999999997,0.874999999999998,
0.906249999999999,0.937499999999999,0.999953591056302),.UNSPECIFIED.);
#29682=B_SPLINE_CURVE_WITH_KNOTS('',3,(#128800,#128801,#128802,#128803,
#128804,#128805,#128806,#128807,#128808,#128809,#128810,#128811,#128812,
#128813,#128814,#128815,#128816,#128817,#128818,#128819,#128820,#128821,
#128822,#128823,#128824,#128825,#128826,#128827,#128828,#128829,#128830,
#128831,#128832,#128833,#128834,#128835,#128836,#128837,#128838,#128839,
#128840,#128841,#128842,#128843,#128844,#128845,#128846,#128847,#128848,
#128849,#128850,#128851,#128852,#128853,#128854,#128855,#128856,#128857,
#128858,#128859,#128860,#128861,#128862,#128863,#128864,#128865,#128866,
#128867,#128868,#128869,#128870,#128871,#128872,#128873),.UNSPECIFIED.,
 .F.,.F.,(4,2,2,2,2,2,2,2,2,2,2,2,2,2,2,2,2,2,2,2,2,2,2,2,2,2,2,2,2,2,2,
2,2,2,2,2,4),(-5.75143272123174,-5.51425389802513,-5.38581494958568,-5.30282096642187,
-5.15632832998793,-5.0625607905497,-4.92381637402678,-4.8214199017456,-4.54353032383151,
-4.42739783573035,-4.3324600201362,-4.13063478019986,-4.0342164491489,-3.82372116145262,
-3.70528204848231,-3.57327965413493,-3.32474231832744,-3.13615410152035,
-3.02764808010997,-2.90892832901364,-2.79616302940586,-2.55643264429745,
-2.40818598215869,-2.11545935413461,-1.9712552015513,-1.7324587016481,-1.62232234512572,
-1.41548413105099,-1.33888975016641,-1.17684236228568,-0.952280572602755,
-0.698170153676864,-0.594739755733359,-0.489501749629593,-0.294699430069487,
-0.149216263156714,-0.000229344986775188),.UNSPECIFIED.);
#29683=B_SPLINE_CURVE_WITH_KNOTS('',3,(#129093,#129094,#129095,#129096,
#129097,#129098,#129099,#129100,#129101,#129102,#129103,#129104,#129105,
#129106,#129107,#129108,#129109,#129110,#129111,#129112,#129113,#129114,
#129115,#129116,#129117,#129118,#129119,#129120,#129121,#129122,#129123,
#129124,#129125,#129126,#129127,#129128,#129129,#129130,#129131,#129132,
#129133,#129134,#129135,#129136,#129137,#129138,#129139,#129140,#129141,
#129142,#129143,#129144,#129145,#129146,#129147,#129148,#129149,#129150,
#129151,#129152,#129153,#129154,#129155,#129156,#129157,#129158,#129159,
#129160,#129161,#129162,#129163,#129164,#129165,#129166,#129167,#129168,
#129169,#129170,#129171,#129172,#129173,#129174,#129175,#129176,#129177,
#129178,#129179,#129180,#129181,#129182,#129183,#129184,#129185,#129186,
#129187,#129188,#129189,#129190,#129191,#129192,#129193,#129194,#129195,
#129196,#129197,#129198,#129199,#129200,#129201,#129202,#129203,#129204,
#129205,#129206,#129207,#129208,#129209,#129210,#129211,#129212,#129213,
#129214,#129215,#129216,#129217,#129218,#129219,#129220,#129221,#129222,
#129223,#129224,#129225,#129226,#129227,#129228,#129229,#129230,#129231,
#129232,#129233,#129234,#129235,#129236,#129237,#129238,#129239,#129240,
#129241,#129242,#129243,#129244,#129245,#129246,#129247,#129248,#129249,
#129250,#129251,#129252,#129253,#129254,#129255,#129256,#129257,#129258,
#129259,#129260,#129261,#129262,#129263,#129264,#129265,#129266,#129267,
#129268,#129269,#129270,#129271,#129272,#129273,#129274,#129275,#129276,
#129277,#129278,#129279,#129280,#129281,#129282,#129283,#129284,#129285,
#129286,#129287,#129288,#129289,#129290,#129291,#129292,#129293,#129294,
#129295,#129296,#129297,#129298,#129299,#129300,#129301,#129302,#129303,
#129304,#129305,#129306,#129307,#129308,#129309,#129310,#129311,#129312,
#129313,#129314,#129315,#129316,#129317,#129318,#129319,#129320,#129321,
#129322,#129323,#129324,#129325,#129326,#129327,#129328,#129329,#129330,
#129331,#129332,#129333,#129334,#129335,#129336,#129337,#129338,#129339,
#129340,#129341,#129342,#129343,#129344,#129345,#129346,#129347,#129348,
#129349,#129350,#129351,#129352,#129353,#129354,#129355,#129356,#129357,
#129358,#129359,#129360,#129361,#129362,#129363,#129364),.UNSPECIFIED.,
 .F.,.F.,(4,2,2,2,2,2,2,2,2,2,2,2,2,2,2,2,2,2,2,2,2,2,2,2,2,2,2,2,2,2,2,
2,2,2,2,2,2,2,2,2,2,2,2,2,2,2,2,2,2,2,2,2,2,2,2,2,2,2,2,2,2,2,2,2,2,2,2,
2,2,2,2,2,2,2,2,2,2,2,2,2,2,2,2,2,2,2,2,2,2,2,2,2,2,2,2,2,2,2,2,2,2,2,2,
2,2,2,2,2,2,2,2,2,2,2,2,2,2,2,2,2,2,2,2,2,2,2,2,2,2,2,2,2,2,2,2,4),(-13.9545132561037,
-13.9243030347878,-13.8575170995572,-13.7785668713752,-13.7363373288312,
-13.6253227823618,-13.5243077460179,-13.4833877659198,-13.4030198483249,
-13.3284452205562,-13.2858020755448,-13.189303459552,-13.1074519173399,
-13.0504571298454,-13.0076680275537,-12.9176522169789,-12.87866620077,-12.8355501446248,
-12.6930731819753,-12.6321432772867,-12.5829931309723,-12.5301482343459,
-12.4529024056035,-12.403313338851,-12.3494336337027,-12.2225984085807,
-12.1670628471684,-12.1199144497519,-12.0484147414705,-11.9693330995282,
-11.9229510002117,-11.7841889511872,-11.72065110925,-11.6693287546292,-11.5631721644431,
-11.5215261585167,-11.4747646633081,-11.336582485301,-11.2685496843921,
-11.2146703139058,-11.1091993946513,-11.0672227875629,-11.0184919885405,
-10.8868200257123,-10.8151746930919,-10.7591366586285,-10.6594788673485,
-10.6160890886625,-10.5659061606284,-10.4336417282592,-10.3600070767517,
-10.3024464292213,-10.2309151663927,-10.1747020296126,-10.123457696155,
-10.0440113070302,-9.93064217307638,-9.85860877432813,-9.8050648596685,
-9.71297606393378,-9.65914341719085,-9.5404548514819,-9.42480737878252,
-9.37094702494681,-9.28398853774682,-9.224575986282,-9.14504171662432,-9.02074473675671,
-8.9434072201311,-8.83429935998517,-8.77068589316592,-8.68763185293676,
-8.56247735742417,-8.48355843939953,-8.39498619186753,-8.34209848688848,
-8.27644926478958,-8.12312435399313,-8.03114001084608,-7.93136637309668,
-7.85989734033156,-7.67560598889003,-7.57433200921146,-7.48453368081615,
-7.42496102203331,-7.34406973953897,-7.19659109542607,-7.12665726422423,
-7.05756427926115,-6.99640672785181,-6.92448537424654,-6.83993498028912,
-6.65681728040653,-6.5872013227692,-6.49064247711442,-6.35498028494421,
-6.20884708319934,-6.12963523553158,-6.03237383964925,-5.94640062904513,
-5.7289825886956,-5.65781097228224,-5.57515679238814,-5.48160063377645,
-5.27541159940625,-5.19666533043402,-5.10815835870751,-5.00016934485196,
-4.81195237411132,-4.72722527119558,-4.61820771918028,-4.46691676878017,
-4.34057070962386,-4.25166078773298,-4.09537792947731,-3.87430507429907,
-3.78572847737797,-3.5977727605266,-3.42324722260386,-3.32305025872687,
-3.19251305750451,-3.02160159678814,-2.84379246729926,-2.67766870850884,
-2.50316178137508,-2.37785241780002,-2.1660464726187,-1.8128682400176,-1.63820944838796,
-1.36589316898249,-1.18932485818936,-1.01455646022611,-0.6682097331427,
-0.582399699183827,-0.292247528397441,-0.000240302142428214),
 .UNSPECIFIED.);
#29684=B_SPLINE_CURVE_WITH_KNOTS('',3,(#129365,#129366,#129367,#129368,
#129369,#129370),.UNSPECIFIED.,.F.,.F.,(4,2,4),(-0.164149603932805,-0.0824424404676746,
-0.000154614832286251),.UNSPECIFIED.);
#29685=B_SPLINE_CURVE_WITH_KNOTS('',3,(#129504,#129505,#129506,#129507,
#129508,#129509,#129510,#129511,#129512,#129513,#129514,#129515,#129516,
#129517,#129518,#129519,#129520,#129521,#129522,#129523,#129524,#129525,
#129526,#129527,#129528,#129529,#129530,#129531,#129532,#129533,#129534,
#129535,#129536,#129537,#129538,#129539,#129540,#129541,#129542,#129543,
#129544,#129545,#129546,#129547,#129548,#129549,#129550,#129551,#129552,
#129553,#129554,#129555,#129556,#129557,#129558,#129559,#129560,#129561,
#129562,#129563,#129564,#129565,#129566,#129567,#129568,#129569,#129570,
#129571,#129572,#129573,#129574,#129575,#129576,#129577,#129578,#129579,
#129580,#129581,#129582,#129583,#129584,#129585,#129586,#129587,#129588,
#129589,#129590,#129591,#129592,#129593,#129594,#129595,#129596,#129597,
#129598,#129599,#129600,#129601,#129602,#129603,#129604,#129605,#129606,
#129607,#129608,#129609,#129610,#129611,#129612,#129613,#129614,#129615,
#129616,#129617,#129618,#129619,#129620,#129621,#129622,#129623,#129624,
#129625,#129626,#129627,#129628,#129629,#129630,#129631,#129632,#129633,
#129634,#129635,#129636,#129637,#129638,#129639,#129640,#129641,#129642,
#129643,#129644,#129645,#129646,#129647,#129648,#129649,#129650,#129651,
#129652,#129653,#129654,#129655,#129656,#129657,#129658,#129659,#129660,
#129661,#129662,#129663,#129664,#129665,#129666,#129667,#129668,#129669,
#129670,#129671,#129672,#129673,#129674,#129675,#129676,#129677,#129678,
#129679,#129680,#129681,#129682,#129683,#129684,#129685,#129686,#129687,
#129688,#129689,#129690,#129691,#129692,#129693,#129694,#129695,#129696,
#129697,#129698,#129699,#129700,#129701,#129702,#129703,#129704,#129705,
#129706,#129707,#129708,#129709,#129710,#129711,#129712,#129713,#129714,
#129715,#129716,#129717,#129718,#129719,#129720,#129721,#129722,#129723,
#129724,#129725,#129726,#129727,#129728,#129729,#129730,#129731,#129732,
#129733,#129734,#129735,#129736,#129737,#129738,#129739,#129740,#129741,
#129742,#129743,#129744,#129745,#129746,#129747,#129748,#129749,#129750,
#129751,#129752,#129753,#129754,#129755,#129756,#129757,#129758,#129759,
#129760,#129761,#129762,#129763,#129764,#129765,#129766,#129767,#129768,
#129769,#129770,#129771,#129772,#129773,#129774,#129775,#129776,#129777,
#129778,#129779,#129780,#129781,#129782,#129783,#129784,#129785,#129786,
#129787,#129788,#129789,#129790,#129791,#129792,#129793,#129794,#129795,
#129796,#129797,#129798,#129799,#129800,#129801,#129802,#129803,#129804,
#129805,#129806,#129807,#129808,#129809,#129810,#129811,#129812,#129813,
#129814,#129815,#129816,#129817),.UNSPECIFIED.,.F.,.F.,(4,2,2,2,2,2,2,2,
2,2,2,2,2,2,2,2,2,2,2,2,2,2,2,2,2,2,2,2,2,2,2,2,2,2,2,2,2,2,2,2,2,2,2,2,
2,2,2,2,2,2,2,2,2,2,2,2,2,2,2,2,2,2,2,2,2,2,2,2,2,2,2,2,2,2,2,2,2,2,2,2,
2,2,2,2,2,2,2,2,2,2,2,2,2,2,2,2,2,2,2,2,2,2,2,2,2,2,2,2,2,2,2,2,2,2,2,2,
2,2,2,2,2,2,2,2,2,2,2,2,2,2,2,2,2,2,2,2,2,2,2,2,2,2,2,2,2,2,2,2,2,2,2,2,
2,2,2,2,4),(0.,0.032292413384482,0.11338718692391,0.148040637360976,0.168457618704367,
0.188241267176605,0.216038652259134,0.284641193115187,0.516477879067667,
0.628828996864852,0.698718093436911,0.774482230614078,1.01964708834714,
1.08748899446127,1.28277707866717,1.3781384951923,1.46460487362281,1.50518672809182,
1.57800422200734,1.73771378462538,1.81311152286536,1.88176895350014,1.95404514404598,
2.00976777043747,2.09658527865148,2.19998313419955,2.27067456521156,2.37364567285775,
2.41997691965579,2.46564898784514,2.58691325670246,2.65712644782479,2.71143601938331,
2.82794621827374,2.87254740263902,2.91367632676383,2.98020888418034,3.0753799403036,
3.13535568618203,3.17968681150426,3.28186089602486,3.32557799525498,3.36461674882526,
3.49176004613578,3.5441977239118,3.58686713316643,3.64812307506937,3.73946558923753,
3.78172916415125,3.82042537563761,3.88402172937341,3.96156672397072,4.01204824266024,
4.06119724607902,4.17634788817974,4.24269266121792,4.28380509965422,4.38055741765955,
4.42537444493737,4.46996733633555,4.59727073297398,4.66224549973719,4.71375714915893,
4.78346138227071,4.84676247744024,4.89890054546601,4.98583850473261,5.09036543444882,
5.16016149181101,5.23257607886221,5.31344437235388,5.3920060656924,5.53474468458556,
5.60359021446961,5.67281256216165,5.75141742025346,5.96539223474982,6.0626546923424,
6.24539619154649,6.41562405879438,6.58288154350623,6.93438230015164,7.10968814663871,
7.41650283228968,7.48753766525244,7.60660749658937,7.79833043443923,7.90069890178098,
7.9918943868596,8.12012415913234,8.25291457596143,8.32075540014824,8.40878778808261,
8.46337012536212,8.52754771413151,8.69630599603858,8.75047744326148,8.82021519340532,
8.87981752418822,8.93185513408938,8.99843303084257,9.12503452987674,9.17054070891333,
9.2160938364855,9.33101367297571,9.37508646137077,9.4289483232484,9.56648674393166,
9.60816961500189,9.65398813669105,9.75702981795865,9.79873482965581,9.85217651583745,
9.93589798757444,10.0047129824676,10.0455924923016,10.0926323646473,10.2020178262266,
10.2475433702179,10.2955529207173,10.3673739495341,10.4414644234633,10.4843910944375,
10.5350239462422,10.6516584989123,10.7006690121429,10.7511670411831,10.8342347958694,
10.890001742534,10.9464695831528,11.0231499654804,11.1290376384701,11.1756073459244,
11.2201404018214,11.3276326418953,11.397372897746,11.5017623038629,11.5870601969509,
11.6427638139526,11.7103971351646,11.7750294377741,11.8800807922603,12.0379343848749,
12.0936733175175,12.1497862113955,12.3415494616393,12.4613597357732,12.5535607266093,
12.6245905782894,12.7178066948602,12.9154555835334,12.9619081589602,12.9841322280929,
13.001682382259,13.0233152594812,13.0726241508325,13.1773028203083),
 .UNSPECIFIED.);
#29686=B_SPLINE_CURVE_WITH_KNOTS('',3,(#129818,#129819,#129820,#129821,
#129822,#129823),.UNSPECIFIED.,.F.,.F.,(4,2,4),(-0.166256920440251,-0.0836095578472467,
-0.00165050313143913),.UNSPECIFIED.);
#29687=B_SPLINE_CURVE_WITH_KNOTS('',3,(#129964,#129965,#129966,#129967,
#129968,#129969,#129970,#129971,#129972,#129973),.UNSPECIFIED.,.F.,.F.,
(4,2,2,2,4),(-0.95725541846645,-0.716501478982729,-0.477123522853866,-0.237827282638415,
-0.000965045394558864),.UNSPECIFIED.);
#29688=B_SPLINE_CURVE_WITH_KNOTS('',3,(#130398,#130399,#130400,#130401),
 .UNSPECIFIED.,.F.,.F.,(4,4),(0.,1.),.UNSPECIFIED.);
#29689=B_SPLINE_CURVE_WITH_KNOTS('',3,(#130407,#130408,#130409,#130410,
#130411,#130412,#130413,#130414,#130415,#130416,#130417,#130418,#130419,
#130420,#130421,#130422,#130423,#130424,#130425,#130426,#130427,#130428,
#130429,#130430,#130431,#130432,#130433,#130434,#130435,#130436,#130437,
#130438,#130439,#130440,#130441,#130442,#130443,#130444,#130445,#130446,
#130447,#130448,#130449,#130450,#130451,#130452,#130453,#130454,#130455,
#130456,#130457,#130458),.UNSPECIFIED.,.F.,.F.,(4,3,3,3,3,3,3,3,3,3,3,3,
3,3,3,3,3,4),(0.850540505530354,0.8518518518519,0.869052332122078,0.878364846193632,
0.8888888888889,0.902430518835671,0.914652441047175,0.915972148782441,0.9259259259259,
0.935258076282245,0.944312112201459,0.953366148120672,0.962155996387792,
0.962962962963,0.976212027251997,0.989052760382921,0.991448955688734,0.999999999999999),
 .UNSPECIFIED.);
#29690=B_SPLINE_CURVE_WITH_KNOTS('',3,(#130544,#130545,#130546,#130547,
#130548,#130549,#130550,#130551,#130552,#130553,#130554,#130555,#130556,
#130557,#130558,#130559),.UNSPECIFIED.,.F.,.F.,(4,3,3,3,3,4),(1.4363549744475E-5,
0.234649898876813,0.25,0.410893410472241,0.5,0.590850967488242),
 .UNSPECIFIED.);
#29691=B_SPLINE_CURVE_WITH_KNOTS('',3,(#130560,#130561,#130562,#130563,
#130564,#130565,#130566,#130567,#130568,#130569,#130570,#130571,#130572,
#130573,#130574,#130575),.UNSPECIFIED.,.F.,.F.,(4,3,3,3,3,4),(6.08869750723345E-5,
0.237050635026911,0.475427842837836,0.5,0.768673980783898,0.999995089856074),
 .UNSPECIFIED.);
#29692=B_SPLINE_CURVE_WITH_KNOTS('',3,(#130578,#130579,#130580,#130581),
 .UNSPECIFIED.,.F.,.F.,(4,4),(0.,1.),.UNSPECIFIED.);
#29693=B_SPLINE_CURVE_WITH_KNOTS('',3,(#130583,#130584,#130585,#130586,
#130587,#130588,#130589,#130590,#130591,#130592,#130593,#130594,#130595),
 .UNSPECIFIED.,.F.,.F.,(4,3,3,3,4),(0.,0.249999996691539,0.495025461485148,
0.747512724125653,0.999999986766158),.UNSPECIFIED.);
#29694=B_SPLINE_CURVE_WITH_KNOTS('',3,(#130601,#130602,#130603,#130604,
#130605,#130606,#130607,#130608,#130609,#130610,#130611,#130612),
 .UNSPECIFIED.,.F.,.F.,(4,2,2,2,2,4),(5.38437140579657E-7,0.25,0.5,0.75,
0.875,1.),.UNSPECIFIED.);
#29695=B_SPLINE_CURVE_WITH_KNOTS('',3,(#130616,#130617,#130618,#130619,
#130620,#130621,#130622,#130623,#130624,#130625,#130626,#130627,#130628,
#130629,#130630,#130631,#130632,#130633,#130634,#130635,#130636,#130637,
#130638,#130639,#130640,#130641,#130642,#130643,#130644,#130645,#130646,
#130647,#130648,#130649,#130650,#130651,#130652,#130653,#130654,#130655,
#130656,#130657,#130658,#130659,#130660,#130661,#130662,#130663,#130664,
#130665,#130666,#130667,#130668,#130669,#130670,#130671,#130672,#130673,
#130674,#130675,#130676,#130677,#130678,#130679,#130680,#130681,#130682,
#130683,#130684,#130685,#130686,#130687,#130688,#130689,#130690,#130691,
#130692,#130693,#130694,#130695,#130696,#130697,#130698,#130699,#130700,
#130701,#130702,#130703,#130704,#130705,#130706,#130707,#130708,#130709,
#130710,#130711,#130712,#130713,#130714,#130715,#130716,#130717,#130718,
#130719,#130720,#130721,#130722,#130723,#130724,#130725,#130726,#130727,
#130728,#130729,#130730,#130731,#130732,#130733,#130734,#130735,#130736,
#130737,#130738,#130739,#130740,#130741,#130742,#130743,#130744,#130745,
#130746,#130747,#130748,#130749,#130750,#130751,#130752,#130753,#130754,
#130755,#130756,#130757,#130758,#130759,#130760,#130761,#130762,#130763,
#130764,#130765,#130766,#130767,#130768,#130769,#130770,#130771,#130772,
#130773,#130774,#130775,#130776,#130777,#130778,#130779,#130780,#130781,
#130782,#130783,#130784,#130785,#130786,#130787,#130788,#130789,#130790,
#130791,#130792,#130793,#130794,#130795,#130796,#130797,#130798,#130799,
#130800,#130801,#130802,#130803,#130804,#130805,#130806,#130807,#130808),
 .UNSPECIFIED.,.F.,.F.,(4,3,3,3,3,3,3,3,3,3,3,3,3,3,3,3,3,3,3,3,3,3,3,3,
3,3,3,3,3,3,3,3,3,3,3,3,3,3,3,3,3,3,3,3,3,3,3,3,3,3,3,3,3,3,3,3,3,3,3,3,
3,3,3,3,4),(2.74350323131394E-5,0.0624999999997235,0.0937499999995802,0.109374999999565,
0.117187499999557,0.121093749999553,0.124999999999549,0.187499999999655,
0.218749999999689,0.234374999999707,0.249111998385219,0.249999999999725,
0.312499999999783,0.3546748106784,0.374999999999841,0.406249999999865,0.422838753251247,
0.437499999999889,0.454769316094528,0.460746878832215,0.468749999999913,
0.484374999999921,0.49218749999992,0.496898696477359,0.499999999999918,
0.517209260150661,0.529730256140993,0.562499999999972,0.570312499999985,
0.575426028661125,0.578124999999998,0.593750000000013,0.594551426193997,
0.623324356174083,0.625000000000046,0.642774596457414,0.644014348734208,
0.662522111460604,0.681015861169127,0.687500000000103,0.688469968606538,
0.718750000000133,0.732476180168218,0.73437500000015,0.742187500000159,
0.74804687500016,0.750000000000159,0.76909300821462,0.80116220296322,0.812500000000106,
0.833321748262734,0.843750000000081,0.859375000000067,0.865392429488015,
0.86718750000006,0.871093750000055,0.873046875000055,0.874658875118369,
0.875000000000055,0.890541952448512,0.913010890352078,0.935653276704301,
0.958350383364628,0.980987301333187,1.),.UNSPECIFIED.);
#29696=B_SPLINE_CURVE_WITH_KNOTS('',3,(#130811,#130812,#130813,#130814,
#130815,#130816,#130817,#130818,#130819,#130820,#130821,#130822,#130823,
#130824,#130825,#130826),.UNSPECIFIED.,.F.,.F.,(4,3,3,3,3,4),(0.,0.272018137403932,
0.5,0.733225822333112,0.965046929604712,0.999871379634594),
 .UNSPECIFIED.);
#29697=B_SPLINE_CURVE_WITH_KNOTS('',3,(#130828,#130829,#130830,#130831,
#130832,#130833,#130834,#130835,#130836,#130837,#130838,#130839,#130840,
#130841,#130842,#130843,#130844,#130845,#130846,#130847,#130848,#130849,
#130850,#130851,#130852,#130853,#130854,#130855,#130856,#130857,#130858,
#130859,#130860,#130861,#130862,#130863,#130864,#130865,#130866,#130867,
#130868,#130869,#130870,#130871,#130872,#130873,#130874,#130875,#130876,
#130877,#130878,#130879,#130880,#130881,#130882,#130883,#130884,#130885,
#130886,#130887,#130888,#130889,#130890,#130891,#130892,#130893,#130894,
#130895,#130896,#130897,#130898,#130899,#130900,#130901,#130902,#130903,
#130904,#130905,#130906,#130907,#130908,#130909,#130910,#130911,#130912,
#130913,#130914,#130915,#130916,#130917,#130918,#130919,#130920,#130921,
#130922,#130923,#130924,#130925,#130926,#130927,#130928,#130929,#130930,
#130931,#130932,#130933,#130934,#130935,#130936,#130937,#130938,#130939,
#130940,#130941,#130942,#130943,#130944,#130945,#130946,#130947,#130948,
#130949,#130950,#130951,#130952,#130953,#130954,#130955,#130956,#130957,
#130958,#130959,#130960,#130961,#130962,#130963,#130964,#130965,#130966,
#130967,#130968,#130969,#130970,#130971,#130972,#130973,#130974,#130975,
#130976,#130977,#130978,#130979,#130980,#130981,#130982,#130983,#130984,
#130985,#130986,#130987,#130988,#130989,#130990,#130991,#130992,#130993,
#130994,#130995,#130996,#130997,#130998,#130999),.UNSPECIFIED.,.F.,.F.,
(4,3,3,3,3,3,3,3,3,3,3,3,3,3,3,3,3,3,3,3,3,3,3,3,3,3,3,3,3,3,3,3,3,3,3,
3,3,3,3,3,3,3,3,3,3,3,3,3,3,3,3,3,3,3,3,3,3,4),(0.,0.027175431995618,0.0625000000000007,
0.0880630432418482,0.0937500000000011,0.109375000000001,0.1171875,0.121093749999997,
0.124350215203792,0.124999999999995,0.146206578525037,0.18750000000001,
0.204900747761968,0.218750000000018,0.234375000000023,0.242187500000027,
0.246093750000027,0.249409409547392,0.250000000000028,0.259834344000549,
0.29426179667726,0.312500000000027,0.314402755346343,0.320312500000027,
0.325489425754323,0.328125000000026,0.343750000000025,0.373866631016789,
0.375000000000014,0.406250000000002,0.437499999999991,0.439137004609811,
0.468749999999979,0.484374999999977,0.494881653599767,0.499999999999974,
0.502112536539499,0.551112506283609,0.562382890212236,0.562499999999971,
0.593749999999965,0.609374999999967,0.612898884207516,0.617187499999969,
0.623058384348781,0.624999999999971,0.66474708209181,0.687499999999985,
0.718749999999986,0.720444473291107,0.73437499999999,0.744928262125903,
0.749999999999993,0.783323050751545,0.848613134581319,0.90975816302401,
0.966654952023228,1.),.UNSPECIFIED.);
#29698=B_SPLINE_CURVE_WITH_KNOTS('',3,(#131001,#131002,#131003,#131004,
#131005,#131006,#131007,#131008,#131009),.UNSPECIFIED.,.F.,.F.,(4,1,2,2,
4),(0.,0.250000000000002,0.37500000000002,0.500000000000039,0.999998122610419),
 .UNSPECIFIED.);
#29699=B_SPLINE_CURVE_WITH_KNOTS('',3,(#131011,#131012,#131013,#131014),
 .UNSPECIFIED.,.F.,.F.,(4,4),(0.,0.987417625481105),.UNSPECIFIED.);
#29700=B_SPLINE_CURVE_WITH_KNOTS('',3,(#131018,#131019,#131020,#131021,
#131022,#131023,#131024,#131025,#131026,#131027,#131028,#131029),
 .UNSPECIFIED.,.F.,.F.,(4,2,2,2,2,4),(0.,0.125,0.25,0.5,0.75,0.999999414381818),
 .UNSPECIFIED.);
#29701=B_SPLINE_CURVE_WITH_KNOTS('',3,(#131035,#131036,#131037,#131038,
#131039,#131040,#131041,#131042,#131043,#131044,#131045,#131046,#131047),
 .UNSPECIFIED.,.F.,.F.,(4,3,3,3,4),(1.05547686689035E-8,0.250000007878098,
0.495573600746854,0.74778680029747,0.999999999848086),.UNSPECIFIED.);
#29702=B_SPLINE_CURVE_WITH_KNOTS('',3,(#131048,#131049,#131050,#131051),
 .UNSPECIFIED.,.F.,.F.,(4,4),(0.,1.),.UNSPECIFIED.);
#29703=B_SPLINE_CURVE_WITH_KNOTS('',3,(#131054,#131055,#131056,#131057,
#131058,#131059,#131060,#131061,#131062,#131063,#131064,#131065,#131066,
#131067,#131068,#131069,#131070,#131071,#131072,#131073,#131074,#131075,
#131076,#131077,#131078,#131079,#131080,#131081,#131082,#131083,#131084,
#131085,#131086,#131087,#131088,#131089,#131090,#131091,#131092,#131093,
#131094,#131095,#131096,#131097,#131098,#131099,#131100,#131101,#131102,
#131103,#131104,#131105,#131106,#131107,#131108,#131109,#131110,#131111,
#131112,#131113,#131114,#131115,#131116,#131117,#131118,#131119,#131120,
#131121,#131122,#131123,#131124,#131125,#131126,#131127,#131128,#131129,
#131130,#131131,#131132,#131133,#131134,#131135,#131136,#131137,#131138,
#131139,#131140,#131141,#131142,#131143,#131144,#131145,#131146,#131147,
#131148,#131149,#131150,#131151,#131152,#131153,#131154,#131155,#131156),
 .UNSPECIFIED.,.F.,.F.,(4,3,3,3,3,3,3,3,3,3,3,3,3,3,3,3,3,3,3,3,3,3,3,3,
3,3,3,3,3,3,3,3,3,3,4),(0.,0.0723506085258293,0.125000000000116,0.18750000000018,
0.218750000000209,0.234375000000217,0.242187500000227,0.250000000000237,
0.299895474419656,0.345551114878514,0.375000000000126,0.41500361137732,
0.437500000000074,0.468750000000044,0.48437500000003,0.492187500000022,
0.499388887162804,0.500000000000015,0.562499999999964,0.593749999999936,
0.609374999999922,0.617187499999912,0.624999999999901,0.665272339956595,
0.687499999999829,0.718749999999794,0.734374999999776,0.742187499999767,
0.746093749999763,0.749999999999758,0.80362415793811,0.855431431549843,
0.874999999999879,0.93749999999994,1.),.UNSPECIFIED.);
#29704=B_SPLINE_CURVE_WITH_KNOTS('',3,(#131162,#131163,#131164,#131165,
#131166,#131167,#131168,#131169,#131170,#131171,#131172,#131173,#131174,
#131175,#131176,#131177,#131178,#131179,#131180,#131181,#131182,#131183,
#131184,#131185,#131186,#131187,#131188),.UNSPECIFIED.,.F.,.F.,(4,2,2,2,
2,2,2,2,2,1,1,1,2,2,4),(0.,0.124999999999985,0.249999999999971,0.374999999999956,
0.437499999999948,0.468749999999943,0.499999999999939,0.62499999999992,
0.687499999999912,0.718749999999909,0.734374999999908,0.742187499999908,
0.746093749999909,0.74999999999991,1.),.UNSPECIFIED.);
#29705=B_SPLINE_CURVE_WITH_KNOTS('',3,(#131192,#131193,#131194,#131195,
#131196,#131197,#131198,#131199,#131200,#131201),.UNSPECIFIED.,.F.,.F.,
(4,3,3,4),(0.,0.343291977175944,0.694006915258001,1.),.UNSPECIFIED.);
#29706=B_SPLINE_CURVE_WITH_KNOTS('',3,(#131202,#131203,#131204,#131205,
#131206,#131207,#131208,#131209,#131210,#131211,#131212,#131213,#131214,
#131215,#131216,#131217,#131218,#131219,#131220,#131221,#131222,#131223,
#131224,#131225,#131226,#131227,#131228,#131229,#131230,#131231,#131232,
#131233,#131234,#131235,#131236,#131237,#131238,#131239,#131240,#131241,
#131242,#131243,#131244,#131245,#131246,#131247,#131248,#131249,#131250,
#131251,#131252,#131253,#131254,#131255,#131256),.UNSPECIFIED.,.F.,.F.,
(4,3,3,3,3,3,3,3,3,3,3,3,3,3,3,3,3,3,4),(5.35764201986684E-7,0.0626028178933704,
0.125,0.183946083050093,0.244293768613518,0.25,0.309271075467163,0.369561477217816,
0.374999999999999,0.439386734520521,0.499999999999999,0.570406759789097,
0.640766647615167,0.710632672526661,0.75,0.820183692041351,0.889379411738386,
0.956887378896293,1.),.UNSPECIFIED.);
#29707=B_SPLINE_CURVE_WITH_KNOTS('',3,(#131259,#131260,#131261,#131262,
#131263,#131264,#131265,#131266,#131267,#131268,#131269,#131270,#131271,
#131272,#131273,#131274,#131275,#131276,#131277,#131278,#131279,#131280,
#131281,#131282,#131283,#131284,#131285,#131286,#131287,#131288,#131289,
#131290,#131291,#131292,#131293,#131294,#131295,#131296,#131297,#131298,
#131299,#131300,#131301,#131302,#131303,#131304,#131305,#131306,#131307,
#131308,#131309,#131310,#131311,#131312,#131313),.UNSPECIFIED.,.F.,.F.,
(4,3,3,3,3,3,3,3,3,3,3,3,3,3,3,3,3,3,4),(0.,0.0675500997162986,0.136181197824484,
0.20632392252024,0.25,0.319906911503152,0.390159163770846,0.460517396300711,
0.5,0.564174428820622,0.625,0.6875,0.746428238623813,0.75,0.8125,0.870495037255567,
0.875,0.937499678080067,0.999999356160134),.UNSPECIFIED.);
#29708=B_SPLINE_CURVE_WITH_KNOTS('',3,(#131315,#131316,#131317,#131318,
#131319,#131320,#131321),.UNSPECIFIED.,.F.,.F.,(4,3,4),(3.32652296912383E-8,
0.56832246895326,0.999999998771275),.UNSPECIFIED.);
#29709=B_SPLINE_CURVE_WITH_KNOTS('',3,(#131325,#131326,#131327,#131328,
#131329,#131330,#131331,#131332,#131333,#131334,#131335,#131336,#131337,
#131338,#131339,#131340,#131341,#131342,#131343,#131344,#131345,#131346,
#131347),.UNSPECIFIED.,.F.,.F.,(4,2,2,1,1,1,2,2,2,2,2,2,4),(0.,0.125000000000061,
0.187500000000091,0.218750000000105,0.234375000000112,0.242187500000114,
0.246093750000114,0.250000000000115,0.375000000000096,0.437500000000086,
0.500000000000076,0.750000000000038,1.),.UNSPECIFIED.);
#29710=B_SPLINE_CURVE_WITH_KNOTS('',3,(#131352,#131353,#131354,#131355,
#131356,#131357,#131358,#131359,#131360,#131361,#131362,#131363,#131364,
#131365,#131366,#131367,#131368,#131369,#131370,#131371,#131372,#131373,
#131374,#131375,#131376,#131377,#131378,#131379,#131380,#131381,#131382,
#131383,#131384,#131385,#131386,#131387,#131388,#131389,#131390,#131391,
#131392,#131393,#131394,#131395,#131396,#131397,#131398,#131399,#131400,
#131401,#131402,#131403,#131404,#131405,#131406,#131407,#131408,#131409,
#131410,#131411,#131412,#131413,#131414,#131415,#131416,#131417,#131418,
#131419,#131420,#131421,#131422,#131423,#131424,#131425,#131426,#131427,
#131428,#131429,#131430,#131431,#131432,#131433,#131434,#131435,#131436,
#131437,#131438,#131439,#131440,#131441,#131442,#131443,#131444,#131445,
#131446,#131447,#131448,#131449,#131450,#131451),.UNSPECIFIED.,.F.,.F.,
(4,3,3,3,3,3,3,3,3,3,3,3,3,3,3,3,3,3,3,3,3,3,3,3,3,3,3,3,3,3,3,3,3,4),(0.,
0.0508232102907746,0.0999610534001555,0.124999999999707,0.156249999999633,
0.164062499999615,0.167968749999606,0.171874999999596,0.187499999999589,
0.249999999999539,0.298872692796552,0.343285506562304,0.374999999999437,
0.413686183409598,0.437499999999392,0.468749999999367,0.484374999999355,
0.492187499999351,0.496093749999351,0.499999999999351,0.535775879334486,
0.572857181333828,0.612180962308859,0.624999999999508,0.668969590894529,
0.687499999999586,0.71874999999963,0.734374999999642,0.742187499999655,
0.749999999999668,0.833516144219682,0.912374151136646,0.986436512705714,
1.),.UNSPECIFIED.);
#29711=B_SPLINE_CURVE_WITH_KNOTS('',3,(#131525,#131526,#131527,#131528,
#131529,#131530),.UNSPECIFIED.,.F.,.F.,(4,2,4),(1.00000001544255E-6,0.194540681199865,
0.386597804410077),.UNSPECIFIED.);
#29712=B_SPLINE_CURVE_WITH_KNOTS('',3,(#131536,#131537,#131538,#131539,
#131540,#131541,#131542,#131543,#131544,#131545,#131546,#131547,#131548,
#131549,#131550,#131551,#131552,#131553,#131554,#131555,#131556,#131557,
#131558,#131559,#131560,#131561,#131562,#131563,#131564,#131565,#131566,
#131567,#131568,#131569,#131570,#131571,#131572,#131573,#131574,#131575,
#131576,#131577,#131578,#131579,#131580,#131581),.UNSPECIFIED.,.F.,.F.,
(4,3,3,3,3,3,3,3,3,3,3,3,3,3,3,4),(0.,0.0415381079537162,0.126736790018611,
0.207848081378628,0.25,0.286439332862369,0.363980210205771,0.441585087808742,
0.519085230204526,0.595965602261323,0.671739736746559,0.745880813468968,
0.817826906179531,0.886990404412328,0.952762686580257,1.),.UNSPECIFIED.);
#29713=B_SPLINE_CURVE_WITH_KNOTS('',3,(#131585,#131586,#131587,#131588,
#131589,#131590,#131591,#131592,#131593,#131594,#131595,#131596,#131597,
#131598,#131599,#131600,#131601,#131602,#131603,#131604,#131605,#131606,
#131607,#131608,#131609,#131610,#131611,#131612,#131613,#131614,#131615,
#131616,#131617,#131618,#131619,#131620,#131621,#131622,#131623,#131624,
#131625,#131626,#131627,#131628,#131629,#131630,#131631,#131632,#131633,
#131634,#131635,#131636,#131637,#131638,#131639,#131640,#131641,#131642,
#131643,#131644,#131645,#131646,#131647,#131648,#131649,#131650,#131651,
#131652,#131653,#131654,#131655,#131656,#131657,#131658,#131659,#131660,
#131661,#131662,#131663,#131664,#131665,#131666),.UNSPECIFIED.,.F.,.F.,
(4,3,3,3,3,3,3,3,3,3,3,3,3,3,3,3,3,3,3,3,3,3,3,3,3,3,3,4),(0.,0.0334067132104181,
0.0951069985116222,0.103593870574672,0.160292573944682,0.172810003123751,
0.225452114130447,0.242418205893516,0.25,0.298890317737418,0.313853438307388,
0.362302570675681,0.388221306904702,0.436699311471132,0.465433186831388,
0.5,0.544971053720226,0.590222923525372,0.626161235508926,0.671327272640816,
0.707999949658858,0.75,0.789293973450788,0.837497575175666,0.868788214041699,
0.922151731283876,0.94510500688402,0.99999771126323),.UNSPECIFIED.);
#29714=B_SPLINE_CURVE_WITH_KNOTS('',3,(#131731,#131732,#131733,#131734,
#131735,#131736,#131737,#131738,#131739,#131740,#131741,#131742,#131743,
#131744,#131745,#131746,#131747,#131748,#131749,#131750,#131751,#131752,
#131753,#131754,#131755,#131756,#131757,#131758,#131759,#131760,#131761,
#131762,#131763,#131764,#131765,#131766,#131767),.UNSPECIFIED.,.F.,.F.,
(4,3,3,3,3,3,3,3,3,3,3,3,4),(4.74817631795029E-11,0.0827291018525572,0.166364550926279,
0.25,0.333157078619199,0.416730922791078,0.499999999999999,0.584300894672092,
0.669074900194399,0.754752782585889,0.840964366055479,0.928186520372598,
1.),.UNSPECIFIED.);
#29715=B_SPLINE_CURVE_WITH_KNOTS('',3,(#131866,#131867,#131868,#131869,
#131870,#131871,#131872,#131873,#131874,#131875),.UNSPECIFIED.,.F.,.F.,
(4,2,2,2,4),(-0.612259894639514,-0.574621721277036,-0.536983547914558,-0.497876710714951,
-0.458769873515343),.UNSPECIFIED.);
#29716=B_SPLINE_CURVE_WITH_KNOTS('',3,(#131881,#131882,#131883,#131884,
#131885,#131886,#131887,#131888,#131889,#131890),.UNSPECIFIED.,.F.,.F.,
(4,2,2,2,4),(-0.153491378099786,-0.114756863309896,-0.0760223485200071,
-0.038011174259927,1.52988732793347E-13),.UNSPECIFIED.);
#29717=B_SPLINE_CURVE_WITH_KNOTS('',3,(#131967,#131968,#131969,#131970,
#131971,#131972,#131973,#131974,#131975,#131976),.UNSPECIFIED.,.F.,.F.,
(4,2,2,2,4),(1.40619031198242E-8,0.250000000000001,0.500000000000001,0.75,
0.999999870300648),.UNSPECIFIED.);
#29718=B_SPLINE_CURVE_WITH_KNOTS('',3,(#132050,#132051,#132052,#132053,
#132054,#132055),.UNSPECIFIED.,.F.,.F.,(4,2,4),(4.58324947990726E-5,0.192154614647802,
0.386590702245323),.UNSPECIFIED.);
#29719=B_SPLINE_CURVE_WITH_KNOTS('',3,(#132057,#132058,#132059,#132060,
#132061,#132062),.UNSPECIFIED.,.F.,.F.,(4,2,4),(0.,0.500000000000002,1.),
 .UNSPECIFIED.);
#29720=B_SPLINE_CURVE_WITH_KNOTS('',3,(#132063,#132064,#132065,#132066,
#132067,#132068,#132069,#132070,#132071,#132072,#132073,#132074,#132075,
#132076,#132077,#132078,#132079,#132080,#132081,#132082,#132083,#132084,
#132085,#132086,#132087,#132088,#132089,#132090,#132091,#132092,#132093,
#132094,#132095,#132096,#132097,#132098,#132099,#132100,#132101,#132102,
#132103,#132104,#132105,#132106,#132107,#132108,#132109,#132110,#132111,
#132112,#132113,#132114,#132115,#132116,#132117,#132118,#132119,#132120,
#132121,#132122,#132123,#132124,#132125,#132126,#132127,#132128,#132129,
#132130,#132131,#132132,#132133,#132134,#132135),.UNSPECIFIED.,.F.,.F.,
(4,3,3,3,3,3,3,3,3,3,3,3,3,3,3,3,3,3,3,3,3,3,3,3,4),(0.,0.0694189172578119,
0.141890572965811,0.210576021946684,0.21436222867381,0.249999999999992,
0.315883055493651,0.380615641482329,0.443499936334932,0.468749999999985,
0.4748539020741,0.484374999999985,0.492187499999985,0.496093749999985,0.498046874999985,
0.499999999999985,0.568648136554788,0.63598650772398,0.701417617452483,
0.749999999999993,0.793695925425306,0.856370695328245,0.918075299204161,
0.978538384319356,1.),.UNSPECIFIED.);
#29721=B_SPLINE_CURVE_WITH_KNOTS('',3,(#132136,#132137,#132138,#132139,
#132140,#132141,#132142,#132143,#132144,#132145,#132146,#132147,#132148,
#132149,#132150,#132151,#132152,#132153,#132154,#132155,#132156,#132157,
#132158,#132159,#132160,#132161,#132162,#132163,#132164,#132165,#132166,
#132167,#132168,#132169,#132170,#132171,#132172,#132173,#132174,#132175,
#132176,#132177,#132178,#132179,#132180,#132181,#132182,#132183,#132184,
#132185,#132186,#132187,#132188,#132189,#132190,#132191,#132192,#132193,
#132194,#132195,#132196,#132197,#132198,#132199,#132200,#132201,#132202,
#132203,#132204,#132205,#132206,#132207,#132208,#132209,#132210,#132211,
#132212,#132213,#132214,#132215,#132216,#132217,#132218,#132219,#132220,
#132221,#132222,#132223,#132224,#132225,#132226,#132227,#132228,#132229,
#132230,#132231,#132232,#132233,#132234,#132235,#132236,#132237,#132238,
#132239,#132240,#132241,#132242,#132243,#132244,#132245,#132246,#132247,
#132248,#132249,#132250,#132251,#132252,#132253,#132254,#132255,#132256,
#132257,#132258,#132259,#132260,#132261,#132262,#132263,#132264,#132265,
#132266,#132267,#132268,#132269,#132270,#132271,#132272,#132273,#132274,
#132275,#132276,#132277,#132278,#132279,#132280,#132281,#132282,#132283,
#132284,#132285,#132286,#132287,#132288,#132289,#132290,#132291,#132292,
#132293,#132294,#132295,#132296,#132297,#132298),.UNSPECIFIED.,.F.,.F.,
(4,3,3,3,3,3,3,3,3,3,3,3,3,3,3,3,3,3,3,3,3,3,3,3,3,3,3,3,3,3,3,3,3,3,3,
3,3,3,3,3,3,3,3,3,3,3,3,3,3,3,3,3,3,3,4),(3.40946049943408E-6,0.054842748741813,
0.106432016312161,0.125000000000608,0.129350108745852,0.178571945306471,
0.205765448657295,0.218750000001064,0.23437500000114,0.242187500001178,
0.246093750001197,0.248046875001207,0.250000000001216,0.288792477778297,
0.332542876341043,0.370249106745186,0.411741696022687,0.441542507192826,
0.468750000002289,0.484375000002366,0.492187500002404,0.496093750002423,
0.498046875002432,0.49975585937744,0.500000000002441,0.514416732036424,
0.522335100169526,0.536786245068709,0.551261014077162,0.565758932084681,
0.580251982159897,0.594687007165219,0.599198235475945,0.609375000001889,
0.61718750000185,0.62109375000183,0.62304687500182,0.624023437501815,0.624511718751812,
0.62500000000181,0.652077693741378,0.685413846871352,0.718750000001327,
0.72732126050095,0.734375000001246,0.742187500001204,0.746093750001184,
0.748046875001174,0.750000000001164,0.802585370019843,0.854434672410697,
0.875607568098376,0.929894244795768,0.951979590739165,1.),.UNSPECIFIED.);
#29722=B_SPLINE_CURVE_WITH_KNOTS('',3,(#132333,#132334,#132335,#132336,
#132337,#132338,#132339,#132340,#132341,#132342,#132343,#132344,#132345,
#132346,#132347,#132348,#132349,#132350,#132351,#132352,#132353,#132354,
#132355,#132356,#132357,#132358,#132359,#132360,#132361,#132362,#132363,
#132364,#132365,#132366,#132367,#132368,#132369,#132370,#132371,#132372,
#132373,#132374,#132375,#132376,#132377,#132378,#132379,#132380,#132381),
 .UNSPECIFIED.,.F.,.F.,(4,3,3,3,3,3,3,3,3,3,3,3,3,3,3,3,4),(0.,0.0744307467764002,
0.148427940845822,0.221954288050944,0.25,0.319609640865989,0.389063697351913,
0.458416657409939,0.5,0.569367807722475,0.638779849028523,0.708396453691038,
0.75,0.823587544912622,0.897476995603493,0.971968625959274,0.999999999975216),
 .UNSPECIFIED.);
#29723=B_SPLINE_CURVE_WITH_KNOTS('',3,(#132387,#132388,#132389,#132390,
#132391,#132392,#132393,#132394,#132395,#132396,#132397,#132398,#132399,
#132400,#132401,#132402,#132403,#132404,#132405,#132406,#132407,#132408,
#132409,#132410,#132411,#132412,#132413,#132414,#132415,#132416,#132417,
#132418,#132419,#132420,#132421,#132422,#132423,#132424,#132425,#132426,
#132427,#132428,#132429,#132430,#132431,#132432),.UNSPECIFIED.,.F.,.F.,
(4,3,3,3,3,3,3,3,3,3,3,3,3,3,3,4),(2.64815152994146E-6,0.0765183545169465,
0.153024457583502,0.229532776872433,0.25,0.326519104574361,0.403032996572845,
0.479542540666675,0.55606478721308,0.632576548147086,0.70909348482205,0.75,
0.826508908783698,0.903008250114437,0.97950997539458,1.),.UNSPECIFIED.);
#29724=B_SPLINE_CURVE_WITH_KNOTS('',3,(#132490,#132491,#132492,#132493,
#132494,#132495,#132496,#132497,#132498,#132499,#132500,#132501,#132502,
#132503,#132504,#132505,#132506,#132507,#132508,#132509,#132510,#132511,
#132512,#132513,#132514,#132515,#132516,#132517,#132518,#132519,#132520,
#132521,#132522,#132523,#132524,#132525,#132526,#132527,#132528,#132529,
#132530,#132531,#132532,#132533,#132534,#132535,#132536,#132537,#132538,
#132539,#132540,#132541,#132542,#132543,#132544),.UNSPECIFIED.,.F.,.F.,
(4,3,3,3,3,3,3,3,3,3,3,3,3,3,3,3,3,3,4),(0.0078125,0.0332755574502296,0.065666662832044,
0.10663681473059,0.131835937499996,0.193847656249995,0.229850852495821,
0.255859374999993,0.28686523437499,0.305008654602828,0.317871093749986,
0.348876953124983,0.366851135809689,0.37988281249998,0.433610794258693,
0.476339196060823,0.503906250000037,0.564135200036142,0.625021704863166),
 .UNSPECIFIED.);
#29725=B_SPLINE_CURVE_WITH_KNOTS('',3,(#132545,#132546,#132547,#132548),
 .UNSPECIFIED.,.F.,.F.,(4,4),(-0.0351695698157893,0.),.UNSPECIFIED.);
#29726=B_SPLINE_CURVE_WITH_KNOTS('',3,(#132590,#132591,#132592,#132593),
 .UNSPECIFIED.,.F.,.F.,(4,4),(1.45270373485029E-10,1.),.UNSPECIFIED.);
#29727=B_SPLINE_CURVE_WITH_KNOTS('',3,(#132630,#132631,#132632,#132633,
#132634,#132635,#132636,#132637,#132638,#132639,#132640,#132641),
 .UNSPECIFIED.,.F.,.F.,(4,2,2,2,2,4),(0.,0.249999999999838,0.374999999999759,
0.437499999999719,0.499999999999679,1.),.UNSPECIFIED.);
#29728=B_SPLINE_CURVE_WITH_KNOTS('',3,(#132728,#132729,#132730,#132731,
#132732,#132733,#132734,#132735,#132736,#132737,#132738,#132739,#132740,
#132741,#132742,#132743,#132744,#132745,#132746,#132747,#132748,#132749,
#132750,#132751,#132752,#132753,#132754,#132755,#132756,#132757,#132758,
#132759,#132760,#132761,#132762,#132763,#132764,#132765,#132766,#132767),
 .UNSPECIFIED.,.F.,.F.,(4,3,3,3,3,3,3,3,3,3,3,3,3,4),(0.00704145220077311,
0.0546624749950295,0.160757685575355,0.256729617165409,0.343735196321369,
0.422731592898268,0.494638559250071,0.560248549174547,0.620252323655667,
0.6753431121518,0.726138185608107,0.772911121896331,0.815853204906754,0.818639731362567),
 .UNSPECIFIED.);
#29729=B_SPLINE_CURVE_WITH_KNOTS('',3,(#132768,#132769,#132770,#132771,
#132772,#132773,#132774,#132775,#132776,#132777,#132778,#132779,#132780,
#132781,#132782,#132783,#132784,#132785,#132786,#132787,#132788,#132789,
#132790,#132791,#132792,#132793,#132794,#132795,#132796,#132797,#132798,
#132799,#132800,#132801,#132802,#132803,#132804,#132805,#132806,#132807,
#132808,#132809,#132810,#132811,#132812,#132813,#132814,#132815,#132816,
#132817,#132818,#132819,#132820,#132821,#132822),.UNSPECIFIED.,.F.,.F.,
(4,3,3,3,3,3,3,3,3,3,3,3,3,3,3,3,3,3,4),(3.4986814498593E-6,0.0718168524834047,
0.144450116073449,0.218617782422917,0.250000000000133,0.324851340463086,
0.3750000000002,0.437500000000237,0.46875000000026,0.484375000000269,0.492187500000267,
0.498371542815579,0.500000000000264,0.550121069632035,0.64802203477807,
0.748418884904067,0.850267541208494,0.954333458676404,1.),.UNSPECIFIED.);
#29730=B_SPLINE_CURVE_WITH_KNOTS('',3,(#132851,#132852,#132853,#132854,
#132855,#132856,#132857,#132858,#132859,#132860,#132861,#132862,#132863),
 .UNSPECIFIED.,.F.,.F.,(4,3,3,3,4),(2.27623555205564E-8,0.250485617068881,
0.495662151858339,0.697586558037137,1.),.UNSPECIFIED.);
#29731=B_SPLINE_CURVE_WITH_KNOTS('',3,(#132864,#132865,#132866,#132867,
#132868,#132869,#132870,#132871,#132872,#132873,#132874,#132875,#132876,
#132877,#132878,#132879,#132880,#132881,#132882),.UNSPECIFIED.,.F.,.F.,
(4,3,3,3,3,3,4),(3.83662521257097E-8,0.190570751481294,0.368121042182241,
0.56520196650433,0.694927749154686,0.76228289082642,1.),.UNSPECIFIED.);
#29732=B_SPLINE_CURVE_WITH_KNOTS('',3,(#132919,#132920,#132921,#132922,
#132923,#132924,#132925,#132926,#132927,#132928,#132929,#132930,#132931),
 .UNSPECIFIED.,.F.,.F.,(4,2,1,2,2,2,4),(0.,0.500000000000364,0.625000000000329,
0.687500000000449,0.750000000000568,0.875000000000284,0.996873152388077),
 .UNSPECIFIED.);
#29733=B_SPLINE_CURVE_WITH_KNOTS('',3,(#132966,#132967,#132968,#132969,
#132970,#132971,#132972,#132973,#132974,#132975,#132976,#132977,#132978,
#132979,#132980,#132981,#132982,#132983,#132984,#132985,#132986,#132987,
#132988,#132989,#132990),.UNSPECIFIED.,.F.,.F.,(4,3,3,3,3,3,3,3,4),(4.68314545443848E-6,
0.126309882651852,0.341277948136751,0.371917171174264,0.592944537541651,
0.616839507849623,0.837854929064512,0.858095091419386,0.999999798284643),
 .UNSPECIFIED.);
#29734=B_SPLINE_CURVE_WITH_KNOTS('',3,(#132991,#132992,#132993,#132994),
 .UNSPECIFIED.,.F.,.F.,(4,4),(0.,0.999997220816645),.UNSPECIFIED.);
#29735=B_SPLINE_CURVE_WITH_KNOTS('',3,(#133062,#133063,#133064,#133065,
#133066,#133067,#133068,#133069,#133070,#133071,#133072,#133073,#133074,
#133075,#133076,#133077,#133078,#133079,#133080,#133081,#133082,#133083,
#133084,#133085,#133086,#133087,#133088,#133089),.UNSPECIFIED.,.F.,.F.,
(4,3,3,3,3,3,3,3,3,4),(0.214741457420206,0.244976288689619,0.314185121458223,
0.389489559305443,0.47162927932211,0.561313355930194,0.659220518921088,
0.766025144246682,0.882569333512905,0.992703055040362),.UNSPECIFIED.);
#29736=B_SPLINE_CURVE_WITH_KNOTS('',3,(#133091,#133092,#133093,#133094,
#133095,#133096,#133097,#133098,#133099,#133100,#133101,#133102,#133103,
#133104,#133105,#133106,#133107,#133108,#133109,#133110,#133111,#133112,
#133113,#133114,#133115,#133116,#133117,#133118),.UNSPECIFIED.,.F.,.F.,
(4,2,2,1,2,2,2,2,1,2,2,2,2,2,4),(0.00114265111152173,0.031250000000139,
0.0625000000002779,0.0937500000004169,0.109375000000459,0.125000000000502,
0.187500000000573,0.218750000000609,0.23437500000061,0.24218750000061,0.250000000000609,
0.375000000000563,0.437500000000518,0.500000000000472,1.),.UNSPECIFIED.);
#29737=B_SPLINE_CURVE_WITH_KNOTS('',3,(#133119,#133120,#133121,#133122,
#133123,#133124,#133125,#133126,#133127,#133128),.UNSPECIFIED.,.F.,.F.,
(4,3,3,4),(0.,0.419606594749395,0.828176819914611,1.),.UNSPECIFIED.);
#29738=B_SPLINE_CURVE_WITH_KNOTS('',3,(#133157,#133158,#133159,#133160),
 .UNSPECIFIED.,.F.,.F.,(4,4),(0.,1.),.UNSPECIFIED.);
#29739=B_SPLINE_CURVE_WITH_KNOTS('',3,(#133161,#133162,#133163,#133164,
#133165,#133166,#133167,#133168,#133169,#133170,#133171,#133172,#133173),
 .UNSPECIFIED.,.F.,.F.,(4,3,3,3,4),(1.30992509567256E-8,0.000738091185335242,
0.604572500785313,0.636544025568632,1.),.UNSPECIFIED.);
#29740=B_SPLINE_CURVE_WITH_KNOTS('',3,(#133207,#133208,#133209,#133210),
 .UNSPECIFIED.,.F.,.F.,(4,4),(0.,0.999998862998874),.UNSPECIFIED.);
#29741=B_SPLINE_CURVE_WITH_KNOTS('',3,(#133249,#133250,#133251,#133252),
 .UNSPECIFIED.,.F.,.F.,(4,4),(0.,0.9999560856806),.UNSPECIFIED.);
#29742=B_SPLINE_CURVE_WITH_KNOTS('',3,(#133323,#133324,#133325,#133326,
#133327,#133328,#133329,#133330,#133331,#133332),.UNSPECIFIED.,.F.,.F.,
(4,2,2,2,4),(0.,0.249999999999965,0.374999999999948,0.499999999999931,1.),
 .UNSPECIFIED.);
#29743=B_SPLINE_CURVE_WITH_KNOTS('',3,(#133334,#133335,#133336,#133337,
#133338,#133339,#133340,#133341,#133342,#133343,#133344,#133345,#133346,
#133347,#133348,#133349,#133350,#133351,#133352,#133353,#133354,#133355,
#133356,#133357,#133358,#133359,#133360,#133361,#133362,#133363,#133364,
#133365,#133366,#133367,#133368,#133369,#133370,#133371,#133372,#133373,
#133374,#133375,#133376),.UNSPECIFIED.,.F.,.F.,(4,3,3,3,3,3,3,3,3,3,3,3,
3,3,4),(0.,0.0170350126721402,0.0659003937260698,0.119026578604631,0.177082319856503,
0.240669318325304,0.309931937354791,0.384677289941797,0.464737806725433,
0.550706641745405,0.643772022188173,0.745112545500137,0.855846190868192,
0.977028739045804,1.),.UNSPECIFIED.);
#29744=B_SPLINE_CURVE_WITH_KNOTS('',3,(#133379,#133380,#133381,#133382,
#133383,#133384,#133385,#133386,#133387,#133388,#133389,#133390,#133391,
#133392,#133393,#133394,#133395,#133396,#133397,#133398,#133399,#133400,
#133401,#133402,#133403,#133404,#133405,#133406,#133407,#133408,#133409),
 .UNSPECIFIED.,.F.,.F.,(4,3,3,3,3,3,3,3,3,3,4),(0.212527788159309,0.238929210760529,
0.307690566088615,0.381894800562219,0.461375561007429,0.546721723948187,
0.639112945312709,0.739719346812922,0.849650913359874,0.96995594614347,
0.992688397423917),.UNSPECIFIED.);
#29745=B_SPLINE_CURVE_WITH_KNOTS('',3,(#133415,#133416,#133417,#133418,
#133419,#133420,#133421,#133422,#133423,#133424,#133425,#133426,#133427,
#133428,#133429,#133430,#133431,#133432,#133433,#133434,#133435,#133436,
#133437,#133438,#133439,#133440,#133441,#133442,#133443,#133444,#133445,
#133446,#133447,#133448,#133449,#133450,#133451),.UNSPECIFIED.,.F.,.F.,
(4,3,3,3,3,3,3,3,3,3,3,3,4),(1.05070778171511E-6,0.0846709690617889,0.169333918564356,
0.254017969883459,0.338685915870495,0.423368260937166,0.5,0.584710646576704,
0.669415319125059,0.754141291593392,0.838850899372478,0.923573259875887,
0.999999999818943),.UNSPECIFIED.);
#29746=B_SPLINE_CURVE_WITH_KNOTS('',3,(#133476,#133477,#133478,#133479,
#133480,#133481,#133482,#133483,#133484,#133485,#133486,#133487,#133488,
#133489,#133490,#133491,#133492,#133493,#133494,#133495,#133496,#133497,
#133498,#133499,#133500,#133501,#133502,#133503,#133504,#133505,#133506,
#133507,#133508,#133509,#133510,#133511,#133512,#133513,#133514,#133515,
#133516,#133517,#133518,#133519,#133520,#133521,#133522,#133523,#133524),
 .UNSPECIFIED.,.F.,.F.,(4,3,3,3,3,3,3,3,3,3,3,3,3,3,3,3,4),(4.14194216132566E-7,
0.0104023161409394,0.032404745883467,0.03703703703704,0.0478687762215131,
0.064929592738566,0.07407407407407,0.0852992481295061,0.103435575750171,
0.1111111111111,0.122727871410933,0.140785542467441,0.1481481481481,0.160147068559508,
0.178135173528707,0.1851851851852,0.188788270697576),.UNSPECIFIED.);
#29747=B_SPLINE_CURVE_WITH_KNOTS('',3,(#133610,#133611,#133612,#133613,
#133614,#133615,#133616,#133617,#133618,#133619,#133620,#133621,#133622,
#133623,#133624,#133625,#133626,#133627,#133628,#133629,#133630,#133631,
#133632,#133633,#133634,#133635,#133636,#133637,#133638,#133639,#133640,
#133641,#133642,#133643,#133644,#133645,#133646,#133647,#133648,#133649,
#133650,#133651,#133652,#133653,#133654,#133655,#133656,#133657,#133658,
#133659,#133660,#133661,#133662,#133663,#133664,#133665,#133666,#133667,
#133668,#133669,#133670,#133671,#133672,#133673,#133674,#133675,#133676,
#133677,#133678,#133679,#133680,#133681,#133682,#133683,#133684,#133685,
#133686,#133687,#133688,#133689,#133690,#133691,#133692,#133693,#133694,
#133695,#133696,#133697,#133698,#133699,#133700,#133701,#133702,#133703,
#133704,#133705,#133706,#133707,#133708,#133709,#133710,#133711,#133712,
#133713,#133714,#133715,#133716,#133717,#133718,#133719,#133720,#133721,
#133722,#133723,#133724,#133725,#133726,#133727,#133728,#133729,#133730),
 .UNSPECIFIED.,.F.,.F.,(4,3,3,3,3,3,3,3,3,3,3,3,3,3,3,3,3,3,3,3,3,3,3,3,
3,3,3,3,3,3,3,3,3,3,3,3,3,3,3,3,4),(1.53023996016127E-7,0.0538427975473875,
0.106014120122847,0.138416004234508,0.188613008991339,0.237253646912087,
0.249999999999905,0.29089575167527,0.332947875837564,0.374999999999858,
0.412763016597034,0.430211822807126,0.437499999999834,0.468749999999821,
0.484374999999816,0.492187499999813,0.496093749999812,0.498046874999813,
0.499999999999813,0.530073715669157,0.545349746812652,0.577232219491959,
0.612722550574342,0.624999999999838,0.667651696788102,0.6854298162725,0.687499999999852,
0.718749999999858,0.734374999999862,0.742187499999864,0.746093749999865,
0.748046874999865,0.749023437499864,0.749999999999864,0.788119952138273,
0.826960318898607,0.861440854495596,0.874999999999932,0.916050892639579,
0.958617696487004,1.),.UNSPECIFIED.);
#29748=B_SPLINE_CURVE_WITH_KNOTS('',3,(#133772,#133773,#133774,#133775,
#133776,#133777,#133778,#133779,#133780,#133781,#133782,#133783,#133784,
#133785,#133786,#133787,#133788,#133789,#133790,#133791,#133792,#133793,
#133794,#133795,#133796,#133797,#133798,#133799,#133800,#133801,#133802,
#133803,#133804,#133805,#133806,#133807,#133808,#133809,#133810,#133811,
#133812,#133813,#133814,#133815,#133816,#133817,#133818,#133819,#133820,
#133821,#133822,#133823,#133824,#133825,#133826,#133827,#133828,#133829,
#133830,#133831,#133832,#133833,#133834,#133835,#133836,#133837,#133838,
#133839,#133840,#133841,#133842,#133843,#133844,#133845,#133846,#133847),
 .UNSPECIFIED.,.F.,.F.,(4,3,3,3,3,3,3,3,3,3,3,3,3,3,3,3,3,3,3,3,3,3,3,3,
3,4),(0.,0.0456119370812063,0.0901169024201462,0.133174944288965,0.175489150215472,
0.21680962027251,0.249999999999996,0.290181447017008,0.329860550964997,
0.369132815094579,0.408091464900065,0.446827929532484,0.485444282452249,
0.524050417570924,0.562725051494045,0.601547160582328,0.640796170375351,
0.680321689677691,0.720459842891237,0.749999999999995,0.79120051762038,
0.833087720599072,0.876268031681826,0.920221939306363,0.965605219388956,
1.),.UNSPECIFIED.);
#29749=B_SPLINE_CURVE_WITH_KNOTS('',3,(#133849,#133850,#133851,#133852,
#133853,#133854,#133855,#133856,#133857,#133858,#133859,#133860,#133861,
#133862,#133863,#133864,#133865,#133866,#133867,#133868,#133869,#133870,
#133871,#133872,#133873,#133874,#133875,#133876,#133877,#133878,#133879,
#133880,#133881,#133882,#133883,#133884,#133885,#133886,#133887,#133888,
#133889,#133890,#133891,#133892,#133893,#133894,#133895,#133896,#133897,
#133898,#133899,#133900,#133901,#133902,#133903,#133904,#133905,#133906,
#133907,#133908,#133909,#133910,#133911,#133912,#133913,#133914,#133915,
#133916,#133917,#133918,#133919,#133920,#133921,#133922,#133923,#133924,
#133925,#133926,#133927),.UNSPECIFIED.,.F.,.F.,(4,3,3,3,3,3,3,3,3,3,3,3,
3,3,3,3,3,3,3,3,3,3,3,3,3,3,4),(0.,0.0579592582826019,0.117537310561431,
0.137605588686488,0.1666666666667,0.221698698493835,0.278959935509025,0.312671189889294,
0.3333333333333,0.384068668956614,0.436358111426463,0.48775592023987,0.5,
0.548139419643831,0.597217471856499,0.647741698863853,0.662828277240584,
0.6666666666667,0.710131267633883,0.753817884952815,0.797986207280148,0.8333333333333,
0.837876903054292,0.884001153291541,0.930724356583334,0.977764846540732,
1.),.UNSPECIFIED.);
#29750=B_SPLINE_CURVE_WITH_KNOTS('',3,(#133928,#133929,#133930,#133931,
#133932,#133933,#133934,#133935,#133936,#133937,#133938,#133939,#133940,
#133941,#133942,#133943,#133944,#133945,#133946,#133947,#133948,#133949,
#133950,#133951,#133952,#133953,#133954,#133955,#133956,#133957,#133958,
#133959,#133960,#133961,#133962,#133963,#133964,#133965,#133966,#133967,
#133968,#133969,#133970,#133971,#133972,#133973,#133974,#133975,#133976),
 .UNSPECIFIED.,.F.,.F.,(4,3,3,3,3,3,3,3,3,3,3,3,3,3,3,3,4),(0.,0.0730059574833017,
0.148337817232831,0.227137820373852,0.25,0.327004186947971,0.403735606439391,
0.478795951017224,0.5,0.578287285905121,0.652570479575901,0.722752191628911,
0.75,0.821415096305571,0.889388191525017,0.953935905694943,1.),
 .UNSPECIFIED.);
#29751=B_SPLINE_CURVE_WITH_KNOTS('',3,(#133980,#133981,#133982,#133983,
#133984,#133985,#133986,#133987,#133988,#133989,#133990,#133991,#133992,
#133993,#133994,#133995,#133996,#133997,#133998,#133999,#134000,#134001,
#134002,#134003,#134004,#134005,#134006,#134007,#134008,#134009,#134010,
#134011,#134012,#134013,#134014,#134015,#134016,#134017,#134018,#134019,
#134020,#134021,#134022,#134023,#134024,#134025),.UNSPECIFIED.,.F.,.F.,
(4,3,3,3,3,3,3,3,3,3,3,3,3,3,3,4),(0.,0.0690009757230223,0.139000969046554,
0.210540625571563,0.250000000000003,0.323645213950312,0.375000000000004,
0.420107205654051,0.465619287340062,0.500000000000005,0.580484011806695,
0.660881352942184,0.74112761125252,0.750000000000003,0.830053892628388,
0.87579096992742),.UNSPECIFIED.);
#29752=B_SPLINE_CURVE_WITH_KNOTS('',3,(#134026,#134027,#134028,#134029,
#134030,#134031,#134032,#134033,#134034,#134035,#134036,#134037,#134038,
#134039,#134040,#134041,#134042,#134043,#134044,#134045,#134046,#134047,
#134048,#134049,#134050,#134051,#134052,#134053,#134054,#134055,#134056,
#134057,#134058,#134059,#134060,#134061,#134062,#134063,#134064,#134065,
#134066,#134067,#134068,#134069,#134070,#134071,#134072,#134073,#134074,
#134075,#134076,#134077,#134078,#134079,#134080,#134081,#134082,#134083,
#134084,#134085,#134086,#134087,#134088,#134089),.UNSPECIFIED.,.F.,.F.,
(4,3,3,3,3,3,3,3,3,3,3,3,3,3,3,3,3,3,3,3,3,4),(9.24012471371765E-5,0.00781249999997771,
0.0123214344920132,0.0156249999999554,0.0252180688217443,0.0312499999999034,
0.0468749999998515,0.0546874999998286,0.0567075535144753,0.0616623599061952,
0.0624999999998058,0.0781249999997706,0.0859374999997557,0.0916222253068236,
0.0937499999997409,0.104842993274865,0.109374999999727,0.11718749999972,
0.121093749999716,0.123667271168975,0.124999999999712,0.125769234561334),
 .UNSPECIFIED.);
#29753=B_SPLINE_CURVE_WITH_KNOTS('',3,(#134130,#134131,#134132,#134133,
#134134,#134135,#134136,#134137,#134138,#134139,#134140,#134141,#134142,
#134143,#134144,#134145,#134146,#134147,#134148,#134149,#134150,#134151,
#134152,#134153,#134154,#134155,#134156,#134157,#134158,#134159,#134160,
#134161,#134162,#134163,#134164,#134165,#134166,#134167,#134168,#134169,
#134170,#134171,#134172,#134173,#134174,#134175,#134176,#134177,#134178,
#134179,#134180,#134181,#134182,#134183,#134184,#134185,#134186,#134187,
#134188,#134189,#134190,#134191,#134192,#134193,#134194,#134195,#134196,
#134197,#134198,#134199,#134200,#134201,#134202,#134203,#134204,#134205,
#134206,#134207,#134208,#134209,#134210,#134211,#134212,#134213,#134214,
#134215,#134216,#134217,#134218,#134219,#134220,#134221,#134222,#134223,
#134224,#134225,#134226,#134227,#134228,#134229,#134230,#134231,#134232,
#134233,#134234,#134235,#134236,#134237,#134238,#134239,#134240,#134241,
#134242,#134243,#134244,#134245,#134246,#134247,#134248,#134249,#134250,
#134251,#134252,#134253),.UNSPECIFIED.,.F.,.F.,(4,3,3,3,3,3,3,3,3,3,3,3,
3,3,3,3,3,3,3,3,3,3,3,3,3,3,3,3,3,3,3,3,3,3,3,3,3,3,3,3,3,4),(0.125769234561334,
0.156249999999699,0.171874999999696,0.179687499999699,0.18510387473411,
0.187499999999701,0.20993433329871,0.218749999999721,0.234374999999732,
0.236573630102243,0.242187499999737,0.247339650344557,0.249999999999742,
0.292365467774003,0.312499999999742,0.343749999999746,0.359374999999748,
0.368677766486324,0.37499999999975,0.407840430019361,0.441178081221039,
0.449378570186183,0.482419525033026,0.499999999999794,0.541113598173256,
0.583056799086548,0.621560046995617,0.624999999999839,0.662035042781543,
0.687499999999861,0.707481972235775,0.718749999999871,0.734701024419774,
0.749999999999882,0.785989295627372,0.821188223681543,0.855344319121138,
0.874999999999941,0.907317639185196,0.939018051031254,0.969895301305895,
1.),.UNSPECIFIED.);
#29754=B_SPLINE_CURVE_WITH_KNOTS('',3,(#134349,#134350,#134351,#134352,
#134353,#134354,#134355,#134356,#134357,#134358,#134359,#134360,#134361,
#134362,#134363,#134364,#134365,#134366,#134367,#134368,#134369,#134370,
#134371,#134372,#134373,#134374,#134375,#134376,#134377,#134378,#134379,
#134380,#134381,#134382,#134383,#134384,#134385,#134386,#134387,#134388,
#134389,#134390,#134391,#134392,#134393,#134394,#134395,#134396,#134397,
#134398,#134399,#134400,#134401,#134402,#134403,#134404,#134405,#134406,
#134407,#134408,#134409),.UNSPECIFIED.,.F.,.F.,(4,3,3,3,3,3,3,3,3,3,3,3,
3,3,3,3,3,3,3,3,4),(4.41879037505324E-7,0.00293416295367035,0.0671893044344527,
0.133594652217226,0.2,0.23548216482957,0.317741082414785,0.395209823031483,
0.4,0.468144568890046,0.571815881128029,0.6,0.682012670063369,0.700986784537182,
0.782354872297676,0.8,0.86055647464313,0.919767494757683,0.935528803203491,
0.994611937942401,1.),.UNSPECIFIED.);
#29755=B_SPLINE_CURVE_WITH_KNOTS('',3,(#134413,#134414,#134415,#134416,
#134417,#134418,#134419,#134420,#134421,#134422,#134423,#134424,#134425,
#134426,#134427,#134428,#134429,#134430,#134431,#134432,#134433,#134434),
 .UNSPECIFIED.,.F.,.F.,(4,3,3,3,3,3,3,4),(1.50238356842823E-7,0.174712592830832,
0.2,0.4,0.6,0.757840534374447,0.8,0.999999999914443),.UNSPECIFIED.);
#29756=B_SPLINE_CURVE_WITH_KNOTS('',3,(#134438,#134439,#134440,#134441,
#134442,#134443,#134444,#134445,#134446,#134447,#134448,#134449,#134450,
#134451,#134452,#134453,#134454,#134455,#134456,#134457,#134458,#134459,
#134460,#134461,#134462,#134463,#134464,#134465,#134466,#134467,#134468,
#134469,#134470,#134471,#134472,#134473,#134474,#134475,#134476,#134477,
#134478,#134479,#134480,#134481,#134482,#134483,#134484,#134485,#134486,
#134487,#134488,#134489,#134490,#134491,#134492,#134493,#134494,#134495,
#134496,#134497,#134498,#134499,#134500,#134501,#134502,#134503,#134504,
#134505,#134506,#134507,#134508,#134509,#134510,#134511,#134512,#134513,
#134514,#134515,#134516,#134517,#134518,#134519,#134520,#134521,#134522,
#134523,#134524,#134525,#134526,#134527,#134528,#134529,#134530,#134531,
#134532,#134533,#134534,#134535,#134536,#134537,#134538,#134539,#134540,
#134541,#134542,#134543,#134544,#134545,#134546,#134547,#134548,#134549,
#134550,#134551,#134552,#134553,#134554,#134555,#134556,#134557,#134558,
#134559,#134560,#134561),.UNSPECIFIED.,.F.,.F.,(4,3,3,3,3,3,3,3,3,3,3,3,
3,3,3,3,3,3,3,3,3,3,3,3,3,3,3,3,3,3,3,3,3,3,3,3,3,3,3,3,3,4),(0.,0.0279278080041807,
0.0557827086768811,0.0625000000001052,0.0899713451083436,0.11793110647808,
0.12500000000021,0.14062500000023,0.142578125000225,0.144531250000221,0.148437500000221,
0.15625000000021,0.18750000000016,0.250000000000059,0.312499999999954,0.37499999999985,
0.437499999999747,0.468749999999689,0.484374999999664,0.492187499999655,
0.498046874999639,0.499999999999631,0.535126545335568,0.562499999999678,
0.593749999999709,0.609374999999727,0.617187499999733,0.621093749999737,
0.62304687499974,0.624999999999744,0.676210940457145,0.687499999999654,
0.71874999999961,0.734374999999588,0.742187499999573,0.746093749999566,
0.748046874999562,0.749999999999559,0.82786552888256,0.874999999999779,
0.938760612897857,0.999999999913687),.UNSPECIFIED.);
#29757=B_SPLINE_CURVE_WITH_KNOTS('',3,(#134565,#134566,#134567,#134568),
 .UNSPECIFIED.,.F.,.F.,(4,4),(0.,1.),.UNSPECIFIED.);
#29758=B_SPLINE_CURVE_WITH_KNOTS('',3,(#134570,#134571,#134572,#134573,
#134574,#134575,#134576,#134577,#134578,#134579,#134580,#134581),
 .UNSPECIFIED.,.F.,.F.,(4,1,1,1,1,1,1,1,1,4),(7.9860235734547E-5,0.0276758837216907,
0.0924977068314539,0.157319299200597,0.22214089156974,0.351784076308025,
0.481427261046311,0.740713630522883,0.870356815261168,0.999999999137475),
 .UNSPECIFIED.);
#29759=B_SPLINE_CURVE_WITH_KNOTS('',3,(#134585,#134586,#134587,#134588,
#134589,#134590,#134591,#134592,#134593,#134594,#134595,#134596,#134597,
#134598,#134599,#134600,#134601,#134602,#134603,#134604,#134605,#134606,
#134607,#134608,#134609,#134610,#134611,#134612,#134613,#134614,#134615,
#134616,#134617,#134618,#134619,#134620,#134621,#134622,#134623,#134624,
#134625,#134626,#134627,#134628,#134629,#134630,#134631,#134632,#134633,
#134634,#134635,#134636,#134637,#134638,#134639,#134640,#134641,#134642,
#134643,#134644,#134645,#134646,#134647,#134648,#134649,#134650,#134651,
#134652,#134653,#134654,#134655,#134656,#134657,#134658,#134659,#134660,
#134661,#134662,#134663,#134664,#134665,#134666,#134667,#134668,#134669,
#134670,#134671,#134672,#134673,#134674,#134675,#134676,#134677,#134678,
#134679,#134680,#134681,#134682,#134683,#134684,#134685,#134686,#134687,
#134688,#134689,#134690,#134691,#134692,#134693),.UNSPECIFIED.,.F.,.F.,
(4,3,3,3,3,3,3,3,3,3,3,3,3,3,3,3,3,3,3,3,3,3,3,3,3,3,3,3,3,3,3,3,3,3,3,
3,4),(9.49981110155694E-5,0.0439079474192139,0.0874336360946032,0.122157576242435,
0.16721492818219,0.212076568275687,0.250000000000103,0.295096146098991,
0.344309653086449,0.375000000000154,0.422725953413255,0.437500000000179,
0.468750000000191,0.482012101196372,0.484375000000197,0.4921875000002,0.496093750000201,
0.499589070935268,0.500000000000202,0.551495839462826,0.601713414256964,
0.625000000000169,0.657972729458139,0.687500000000153,0.718750000000144,
0.73437500000014,0.742187500000137,0.748177025422295,0.750000000000133,
0.791495676503256,0.814047913622898,0.85483988042624,0.896403261494273,
0.939242980538536,0.956354100682218,0.99563199192476,0.999999999985943),
 .UNSPECIFIED.);
#29760=B_SPLINE_CURVE_WITH_KNOTS('',3,(#134742,#134743,#134744,#134745,
#134746,#134747,#134748,#134749,#134750,#134751,#134752,#134753,#134754,
#134755,#134756,#134757,#134758,#134759,#134760,#134761,#134762,#134763,
#134764,#134765,#134766,#134767,#134768,#134769,#134770,#134771,#134772,
#134773,#134774,#134775,#134776,#134777,#134778,#134779,#134780,#134781,
#134782,#134783,#134784,#134785,#134786,#134787,#134788,#134789,#134790,
#134791,#134792,#134793,#134794,#134795,#134796,#134797,#134798,#134799,
#134800,#134801,#134802),.UNSPECIFIED.,.F.,.F.,(4,3,3,3,3,3,3,3,3,3,3,3,
3,3,3,3,3,3,3,3,4),(0.,0.0573467126579996,0.113335897514098,0.168615343495432,
0.223030306420361,0.25,0.303580319758419,0.359382779788616,0.412115475219052,
0.464689063753643,0.517201688167575,0.569751228579584,0.622581475411049,
0.675624819261524,0.729158060796906,0.75,0.804273166293312,0.859584359029149,
0.915547401796053,0.972684308211155,0.999999999999995),.UNSPECIFIED.);
#29761=B_SPLINE_CURVE_WITH_KNOTS('',3,(#134803,#134804,#134805,#134806,
#134807,#134808,#134809,#134810,#134811,#134812,#134813,#134814,#134815,
#134816,#134817,#134818,#134819,#134820,#134821,#134822,#134823,#134824,
#134825,#134826,#134827,#134828,#134829,#134830,#134831,#134832,#134833,
#134834,#134835,#134836,#134837,#134838,#134839,#134840,#134841,#134842,
#134843,#134844,#134845,#134846,#134847,#134848,#134849,#134850,#134851,
#134852,#134853,#134854,#134855,#134856,#134857,#134858,#134859,#134860,
#134861,#134862,#134863),.UNSPECIFIED.,.F.,.F.,(4,3,3,3,3,3,3,3,3,3,3,3,
3,3,3,3,3,3,3,3,4),(7.44116098701117E-15,0.0512371487041215,0.101989469318509,
0.152519576430421,0.202910903303978,0.25,0.300261981465075,0.350846320516069,
0.40164929578049,0.453037776867762,0.5,0.552205879476937,0.605524420566545,
0.659525200433921,0.714793533787152,0.75,0.806897139877591,0.865686533687191,
0.925670351357924,0.98752344482043,1.),.UNSPECIFIED.);
#29762=B_SPLINE_CURVE_WITH_KNOTS('',3,(#134905,#134906,#134907,#134908,
#134909,#134910,#134911,#134912,#134913,#134914,#134915,#134916,#134917,
#134918,#134919,#134920,#134921,#134922,#134923,#134924,#134925,#134926,
#134927,#134928,#134929,#134930,#134931,#134932,#134933,#134934,#134935,
#134936,#134937,#134938,#134939,#134940,#134941,#134942,#134943,#134944,
#134945,#134946,#134947,#134948,#134949,#134950,#134951,#134952,#134953,
#134954,#134955,#134956,#134957,#134958,#134959,#134960,#134961,#134962,
#134963,#134964,#134965,#134966,#134967,#134968,#134969,#134970,#134971,
#134972,#134973,#134974,#134975,#134976,#134977,#134978,#134979,#134980),
 .UNSPECIFIED.,.F.,.F.,(4,3,3,3,3,3,3,3,3,3,3,3,3,3,3,3,3,3,3,3,3,3,3,3,
3,4),(0.,0.0240095347924936,0.0480575330575472,0.0624999999999994,0.0939199229640899,
0.124999999999999,0.156695647248868,0.189726142714701,0.223167127401312,
0.249999999999999,0.288838755939898,0.32816014520085,0.368106946620112,
0.374999999999999,0.422671007495536,0.471592059303987,0.499999999999999,
0.517768565868439,0.578191826686414,0.640220818655331,0.704885773476388,
0.749999999999999,0.823691392983596,0.852261955107439,0.928556327574316,
1.),.UNSPECIFIED.);
#29763=B_SPLINE_CURVE_WITH_KNOTS('',3,(#134981,#134982,#134983,#134984,
#134985,#134986,#134987,#134988,#134989,#134990,#134991,#134992,#134993),
 .UNSPECIFIED.,.F.,.F.,(4,3,3,3,4),(0.,0.392244811655611,0.5,0.76234491070066,
1.),.UNSPECIFIED.);
#29764=B_SPLINE_CURVE_WITH_KNOTS('',3,(#135035,#135036,#135037,#135038,
#135039,#135040,#135041,#135042,#135043,#135044,#135045,#135046,#135047,
#135048,#135049,#135050,#135051,#135052,#135053,#135054,#135055,#135056,
#135057,#135058,#135059,#135060,#135061),.UNSPECIFIED.,.F.,.F.,(4,2,2,1,
1,2,2,2,2,1,1,1,2,2,2,4),(0.,0.125000000000001,0.187500000000001,0.218750000000002,
0.234375000000002,0.242187500000002,0.250000000000002,0.37499999999999,
0.437499999999985,0.468749999999982,0.48437499999998,0.492187499999979,
0.496093749999979,0.49999999999998,0.74999999999999,0.999906678651906),
 .UNSPECIFIED.);
#29765=B_SPLINE_CURVE_WITH_KNOTS('',3,(#135063,#135064,#135065,#135066,
#135067,#135068,#135069,#135070,#135071,#135072,#135073,#135074,#135075),
 .UNSPECIFIED.,.F.,.F.,(4,3,3,3,4),(7.78289278789026E-10,0.237624182551005,
0.5,0.607655001033738,0.999999999858253),.UNSPECIFIED.);
#29766=B_SPLINE_CURVE_WITH_KNOTS('',3,(#135076,#135077,#135078,#135079,
#135080,#135081,#135082,#135083,#135084,#135085,#135086,#135087,#135088,
#135089,#135090,#135091,#135092,#135093,#135094,#135095,#135096,#135097,
#135098,#135099,#135100,#135101,#135102,#135103,#135104,#135105,#135106,
#135107,#135108,#135109,#135110,#135111,#135112,#135113,#135114,#135115,
#135116,#135117,#135118,#135119,#135120,#135121,#135122,#135123,#135124,
#135125,#135126,#135127,#135128,#135129,#135130,#135131,#135132,#135133,
#135134,#135135,#135136,#135137,#135138,#135139,#135140,#135141,#135142,
#135143,#135144,#135145,#135146,#135147,#135148,#135149,#135150,#135151,
#135152,#135153,#135154),.UNSPECIFIED.,.F.,.F.,(4,3,3,3,3,3,3,3,3,3,3,3,
3,3,3,3,3,3,3,3,3,3,3,3,3,3,4),(0.,0.0781417538335214,0.156283507667043,
0.229903094289744,0.25,0.314389271872266,0.377077783281621,0.43711271294967,
0.490712794158447,0.499999999999999,0.549101400831195,0.596959248933236,
0.624999999999999,0.664843799387995,0.704220170720158,0.742896099962853,
0.75,0.783424128120187,0.816659225360256,0.849374153129844,0.853956214206258,
0.875,0.906271016403279,0.9375,0.961323616750085,0.985107754960295,1.),
 .UNSPECIFIED.);
#29767=B_SPLINE_CURVE_WITH_KNOTS('',3,(#135221,#135222,#135223,#135224,
#135225,#135226,#135227,#135228,#135229,#135230,#135231,#135232,#135233,
#135234,#135235,#135236,#135237,#135238,#135239),.UNSPECIFIED.,.F.,.F.,
(4,3,3,3,3,3,4),(0.,0.181519090760199,0.362120636613677,0.542234912997426,
0.72225841896039,0.902871075785579,1.),.UNSPECIFIED.);
#29768=B_SPLINE_CURVE_WITH_KNOTS('',3,(#135240,#135241,#135242,#135243,
#135244,#135245,#135246,#135247,#135248,#135249,#135250,#135251,#135252,
#135253,#135254,#135255,#135256,#135257,#135258,#135259,#135260,#135261,
#135262,#135263,#135264,#135265,#135266,#135267,#135268,#135269,#135270,
#135271,#135272,#135273,#135274,#135275,#135276,#135277,#135278,#135279,
#135280,#135281,#135282,#135283,#135284,#135285,#135286,#135287,#135288,
#135289,#135290,#135291,#135292,#135293,#135294,#135295,#135296,#135297,
#135298,#135299,#135300,#135301,#135302,#135303,#135304,#135305,#135306,
#135307,#135308,#135309,#135310,#135311,#135312,#135313,#135314,#135315,
#135316,#135317,#135318,#135319,#135320,#135321,#135322,#135323,#135324,
#135325,#135326,#135327,#135328,#135329,#135330,#135331,#135332,#135333,
#135334,#135335,#135336,#135337,#135338,#135339,#135340,#135341,#135342,
#135343,#135344,#135345,#135346,#135347,#135348,#135349,#135350,#135351,
#135352,#135353,#135354,#135355,#135356,#135357,#135358,#135359,#135360,
#135361,#135362,#135363,#135364,#135365,#135366,#135367,#135368,#135369,
#135370,#135371,#135372,#135373,#135374,#135375,#135376,#135377,#135378,
#135379,#135380,#135381,#135382,#135383,#135384,#135385,#135386,#135387,
#135388,#135389,#135390,#135391,#135392,#135393),.UNSPECIFIED.,.F.,.F.,
(4,3,3,3,3,3,3,3,3,3,3,3,3,3,3,3,3,3,3,3,3,3,3,3,3,3,3,3,3,3,3,3,3,3,3,
3,3,3,3,3,3,3,3,3,3,3,3,3,3,3,3,4),(2.73322965884126E-10,0.0264549111194651,
0.0485516362526499,0.062499999999984,0.0850151135779835,0.0867625902511057,
0.116275778153569,0.124023437499972,0.124999999999974,0.160063595048907,
0.189301312632248,0.223901320758205,0.248046875000073,0.250000000000073,
0.28653488326189,0.292550069720856,0.326377468207769,0.364655941592613,
0.367187500000048,0.374510310049938,0.375000000000045,0.397544446166902,
0.434809267245017,0.474466284754075,0.492187500000022,0.498183594972155,
0.500000000000021,0.527222702158733,0.55616511346704,0.588322976640463,
0.596116434011651,0.609375000000011,0.618910390786312,0.62500000000001,
0.658201936263826,0.694362627592558,0.700819345682431,0.718750000000008,
0.732543917215725,0.745471055817449,0.750000000000008,0.779429696038487,
0.80209682307013,0.824435228005092,0.848926685652495,0.874561887630016,
0.900806883711232,0.905330311691599,0.927606641474703,0.951122356025715,
0.975561177979689,0.999999999933663),.UNSPECIFIED.);
#29769=B_SPLINE_CURVE_WITH_KNOTS('',3,(#135400,#135401,#135402,#135403,
#135404,#135405,#135406,#135407,#135408,#135409,#135410,#135411,#135412,
#135413,#135414,#135415,#135416,#135417,#135418,#135419,#135420,#135421,
#135422,#135423,#135424,#135425,#135426,#135427,#135428,#135429,#135430,
#135431,#135432,#135433,#135434,#135435,#135436,#135437,#135438,#135439,
#135440,#135441,#135442,#135443,#135444,#135445,#135446,#135447,#135448,
#135449,#135450,#135451,#135452,#135453,#135454,#135455,#135456,#135457,
#135458,#135459,#135460,#135461,#135462,#135463,#135464,#135465,#135466,
#135467,#135468,#135469,#135470,#135471,#135472,#135473,#135474,#135475,
#135476,#135477,#135478,#135479,#135480,#135481,#135482,#135483,#135484,
#135485,#135486,#135487,#135488,#135489,#135490,#135491,#135492,#135493,
#135494,#135495,#135496,#135497,#135498,#135499,#135500,#135501,#135502,
#135503,#135504,#135505,#135506,#135507,#135508,#135509,#135510,#135511,
#135512,#135513,#135514,#135515,#135516,#135517,#135518,#135519,#135520,
#135521,#135522,#135523,#135524,#135525,#135526,#135527,#135528,#135529,
#135530,#135531,#135532,#135533,#135534,#135535,#135536,#135537,#135538,
#135539,#135540,#135541,#135542,#135543,#135544,#135545,#135546,#135547,
#135548,#135549,#135550,#135551,#135552,#135553,#135554,#135555,#135556,
#135557,#135558,#135559,#135560,#135561,#135562,#135563,#135564,#135565,
#135566,#135567,#135568,#135569,#135570,#135571,#135572,#135573,#135574),
 .UNSPECIFIED.,.F.,.F.,(4,3,3,3,3,3,3,3,3,3,3,3,3,3,3,3,3,3,3,3,3,3,3,3,
3,3,3,3,3,3,3,3,3,3,3,3,3,3,3,3,3,3,3,3,3,3,3,3,3,3,3,3,3,3,3,3,3,3,4),
(8.96765241561959E-11,0.0241198469644619,0.0474038529016274,0.0625000000000184,
0.0836216493288717,0.0973629920783003,0.109375000000032,0.116503694188718,
0.123844299441502,0.125000000000036,0.147610163784958,0.170591682874619,
0.193590311413262,0.196215774040552,0.218750000000064,0.231600729773752,
0.245051809224319,0.250000000000072,0.277441233902207,0.301886806087822,
0.338443403043965,0.368343375402564,0.375000000000108,0.394858108367889,
0.401874435804676,0.424366897198985,0.437500000000125,0.475573217952329,
0.492187500000139,0.497520504312495,0.50000000000014,0.534667154153412,
0.546875000000145,0.557645435349896,0.562500000000147,0.59375000000015,
0.596577244630875,0.61546646504238,0.625000000000153,0.66314840319689,0.698751804371271,
0.737883241891824,0.746093750000162,0.750000000000161,0.785934144325005,
0.800108539909645,0.837065988704875,0.871303163694748,0.874023437500105,
0.875000000000105,0.898592058160894,0.9047087781261,0.92187500000007,0.936535331259133,
0.937500000000057,0.955831751877182,0.976381324473505,0.992332357317893,
0.999999999999997),.UNSPECIFIED.);
#29770=B_SPLINE_CURVE_WITH_KNOTS('',3,(#135633,#135634,#135635,#135636,
#135637,#135638,#135639,#135640,#135641,#135642),.UNSPECIFIED.,.F.,.F.,
(4,2,2,2,4),(0.,0.25,0.5,0.75,1.),.UNSPECIFIED.);
#29771=B_SPLINE_CURVE_WITH_KNOTS('',3,(#135645,#135646,#135647,#135648,
#135649,#135650,#135651,#135652,#135653,#135654,#135655,#135656,#135657,
#135658,#135659,#135660,#135661,#135662,#135663,#135664,#135665,#135666,
#135667,#135668,#135669,#135670,#135671,#135672,#135673,#135674,#135675),
 .UNSPECIFIED.,.F.,.F.,(4,3,3,3,3,3,3,3,3,3,4),(0.,0.125000017210984,0.250000014806018,
0.375000012401051,0.500000009996085,0.62500000759112,0.750000005186153,
0.812500003983669,0.875000002781187,0.937500001578704,1.),.UNSPECIFIED.);
#29772=B_SPLINE_CURVE_WITH_KNOTS('',3,(#135676,#135677,#135678,#135679,
#135680,#135681,#135682,#135683,#135684,#135685,#135686,#135687,#135688,
#135689,#135690,#135691,#135692,#135693,#135694,#135695,#135696,#135697,
#135698,#135699,#135700,#135701,#135702,#135703,#135704,#135705,#135706,
#135707,#135708,#135709,#135710,#135711,#135712,#135713,#135714,#135715,
#135716,#135717,#135718,#135719,#135720,#135721,#135722,#135723,#135724,
#135725,#135726,#135727,#135728,#135729,#135730,#135731,#135732,#135733,
#135734,#135735,#135736,#135737,#135738,#135739,#135740,#135741,#135742,
#135743,#135744,#135745,#135746,#135747,#135748,#135749,#135750,#135751,
#135752,#135753,#135754,#135755,#135756,#135757,#135758,#135759,#135760,
#135761,#135762,#135763,#135764,#135765,#135766,#135767,#135768,#135769,
#135770,#135771,#135772,#135773,#135774,#135775,#135776,#135777,#135778,
#135779,#135780,#135781,#135782,#135783,#135784,#135785,#135786,#135787,
#135788,#135789,#135790,#135791,#135792,#135793,#135794,#135795,#135796,
#135797,#135798,#135799,#135800,#135801,#135802,#135803,#135804,#135805,
#135806,#135807,#135808,#135809,#135810,#135811,#135812,#135813,#135814,
#135815,#135816,#135817,#135818,#135819,#135820,#135821,#135822,#135823,
#135824,#135825,#135826,#135827,#135828,#135829,#135830,#135831,#135832,
#135833,#135834,#135835,#135836,#135837,#135838),.UNSPECIFIED.,.F.,.F.,
(4,3,3,3,3,3,3,3,3,3,3,3,3,3,3,3,3,3,3,3,3,3,3,3,3,3,3,3,3,3,3,3,3,3,3,
3,3,3,3,3,3,3,3,3,3,3,3,3,3,3,3,3,3,3,4),(4.48981150760254E-9,0.0393536153485956,
0.0624999999999912,0.0937499999999866,0.109374999999985,0.117187499999983,
0.121093749999983,0.124999999999982,0.154799793759501,0.184939633053664,
0.215527805974844,0.218749999999966,0.234374999999964,0.242187499999962,
0.248759787824685,0.249999999999961,0.276843317058182,0.303796959875753,
0.330874054305417,0.343749999999956,0.359374999999956,0.367187499999956,
0.374999999999956,0.400813537045637,0.426642884048751,0.452475164185863,
0.478308677755654,0.499999999999977,0.525829006322467,0.551657601353355,
0.577482865841678,0.593749999999991,0.609374999999993,0.617187499999993,
0.624999999999994,0.651988603271001,0.67892648510348,0.705754490984526,
0.718749999999989,0.734374999999988,0.742187499999988,0.749108314032712,
0.749999999999988,0.780820961713403,0.812285480856701,0.84375,0.859375000000001,
0.867187500000002,0.871093750000002,0.874779879052441,0.875000000000003,
0.91517837097112,0.954934021116031,0.994126825971164,0.999999999998253),
 .UNSPECIFIED.);
#29773=B_SPLINE_CURVE_WITH_KNOTS('',3,(#136157,#136158,#136159,#136160,
#136161,#136162,#136163,#136164,#136165,#136166,#136167,#136168,#136169,
#136170,#136171,#136172,#136173,#136174,#136175,#136176,#136177,#136178,
#136179,#136180,#136181,#136182,#136183,#136184,#136185,#136186,#136187,
#136188,#136189,#136190,#136191,#136192,#136193,#136194,#136195,#136196,
#136197,#136198,#136199,#136200,#136201,#136202,#136203,#136204,#136205,
#136206,#136207,#136208,#136209,#136210,#136211,#136212,#136213,#136214,
#136215,#136216,#136217,#136218,#136219,#136220,#136221,#136222,#136223,
#136224,#136225,#136226,#136227,#136228,#136229,#136230,#136231,#136232,
#136233,#136234,#136235,#136236,#136237,#136238,#136239,#136240,#136241,
#136242,#136243,#136244,#136245,#136246,#136247,#136248,#136249,#136250,
#136251,#136252,#136253,#136254,#136255,#136256,#136257,#136258,#136259,
#136260,#136261,#136262,#136263,#136264,#136265,#136266,#136267,#136268,
#136269,#136270,#136271,#136272,#136273,#136274,#136275,#136276,#136277,
#136278,#136279,#136280,#136281,#136282,#136283,#136284,#136285,#136286,
#136287,#136288,#136289,#136290,#136291,#136292,#136293,#136294,#136295,
#136296,#136297,#136298,#136299,#136300,#136301,#136302,#136303,#136304,
#136305,#136306,#136307,#136308,#136309,#136310,#136311,#136312,#136313,
#136314,#136315,#136316,#136317,#136318,#136319,#136320,#136321,#136322,
#136323,#136324,#136325,#136326,#136327,#136328,#136329,#136330,#136331,
#136332,#136333,#136334,#136335,#136336,#136337,#136338,#136339,#136340,
#136341,#136342,#136343,#136344,#136345,#136346,#136347,#136348,#136349,
#136350,#136351,#136352,#136353,#136354,#136355,#136356,#136357,#136358,
#136359,#136360,#136361,#136362,#136363,#136364,#136365,#136366,#136367,
#136368,#136369,#136370,#136371,#136372,#136373,#136374,#136375,#136376,
#136377,#136378,#136379,#136380,#136381,#136382,#136383,#136384,#136385,
#136386,#136387,#136388,#136389,#136390,#136391,#136392,#136393,#136394,
#136395,#136396,#136397,#136398,#136399,#136400,#136401,#136402,#136403),
 .UNSPECIFIED.,.F.,.F.,(4,3,3,3,3,3,3,3,3,3,3,3,3,3,3,3,3,3,3,3,3,3,3,3,
3,3,3,3,3,3,3,3,3,3,3,3,3,3,3,3,3,3,3,3,3,3,3,3,3,3,3,3,3,3,3,3,3,3,3,3,
3,3,3,3,3,3,3,3,3,3,3,3,3,3,3,3,3,3,3,3,3,3,4),(0.,0.0182036326055988,0.0365586805154091,
0.0549664507454061,0.0618630850421433,0.0625000000000037,0.082871203764013,
0.0937500000000058,0.109375000000006,0.117187500000006,0.121093750000007,
0.123955543489655,0.125000000000008,0.141772636856682,0.160701514674118,
0.179933095227437,0.187500000000012,0.206742027831368,0.218750000000015,
0.221802188213591,0.234375000000016,0.242187500000016,0.246587970153079,
0.250000000000015,0.269649006232186,0.289649551960229,0.302311004851823,
0.312500000000011,0.331828586949002,0.34375000000001,0.359375000000009,
0.367187500000009,0.371839982042231,0.375000000000009,0.381564892865856,
0.401351920256644,0.420725587216239,0.440719294822623,0.460713002429007,
0.480356501214506,0.500000000000005,0.519655374734875,0.539310749469746,
0.55873928442422,0.562500000000005,0.582101419253175,0.593750000000003,
0.609375000000003,0.617187500000004,0.618517773284973,0.623131725816646,
0.625000000000005,0.643925066155593,0.663072701417495,0.682366749879823,
0.687500000000011,0.697796532795641,0.717621058411164,0.718750000000013,
0.734375000000014,0.742187500000014,0.746829629420927,0.750000000000014,
0.769077781416545,0.778274111050064,0.79759938395752,0.812500000000014,
0.831723467455908,0.843750000000013,0.858266019020329,0.859375000000013,
0.867187500000012,0.871093750000012,0.873908642882608,0.875000000000011,
0.894275615001603,0.913642445688952,0.932986570725005,0.93820730918229,
0.957307698559546,0.97634626547438,0.995134148476193,0.999999998885172),
 .UNSPECIFIED.);
#29774=B_SPLINE_CURVE_WITH_KNOTS('',3,(#136406,#136407,#136408,#136409,
#136410,#136411,#136412,#136413,#136414,#136415,#136416,#136417,#136418,
#136419,#136420,#136421,#136422,#136423,#136424,#136425,#136426,#136427,
#136428,#136429,#136430,#136431,#136432,#136433,#136434,#136435,#136436,
#136437,#136438,#136439,#136440,#136441,#136442,#136443,#136444,#136445,
#136446,#136447,#136448,#136449,#136450,#136451,#136452,#136453,#136454,
#136455,#136456,#136457,#136458,#136459,#136460,#136461,#136462,#136463,
#136464,#136465,#136466,#136467,#136468,#136469,#136470,#136471,#136472,
#136473,#136474,#136475,#136476,#136477,#136478,#136479,#136480,#136481,
#136482,#136483,#136484,#136485,#136486,#136487,#136488,#136489,#136490,
#136491,#136492,#136493,#136494,#136495,#136496,#136497,#136498,#136499,
#136500,#136501,#136502,#136503,#136504,#136505,#136506,#136507,#136508,
#136509,#136510,#136511,#136512,#136513,#136514,#136515,#136516,#136517,
#136518,#136519,#136520),.UNSPECIFIED.,.F.,.F.,(4,3,3,3,3,3,3,3,3,3,3,3,
3,3,3,3,3,3,3,3,3,3,3,3,3,3,3,3,3,3,3,3,3,3,3,3,3,3,4),(0.,0.0312499994700485,
0.0620396289050024,0.0935803778640139,0.124999997880194,0.159516816915742,
0.187499996904519,0.215676877869275,0.244239375088295,0.249999995928844,
0.276585162517748,0.303351488571435,0.312499994953169,0.36324402498958,
0.374999993977494,0.418857054128309,0.437499993001819,0.466980128711126,
0.496376788249355,0.499999992026143,0.533828245823419,0.562499991050468,
0.601187995873233,0.624999990074793,0.662802044869547,0.687499989099118,
0.715357883472307,0.742917981241798,0.749999988123444,0.776876675242584,
0.803610334516972,0.830278666812802,0.856879045765974,0.874999986172094,
0.903656784953601,0.932051835173095,0.960238948507373,0.988060471740437,
1.),.UNSPECIFIED.);
#29775=B_SPLINE_CURVE_WITH_KNOTS('',3,(#136523,#136524,#136525,#136526,
#136527,#136528,#136529,#136530,#136531,#136532),.UNSPECIFIED.,.F.,.F.,
(4,2,2,2,4),(0.,0.25,0.5,0.75,1.),.UNSPECIFIED.);
#29776=B_SPLINE_CURVE_WITH_KNOTS('',3,(#136820,#136821,#136822,#136823,
#136824,#136825,#136826,#136827,#136828,#136829,#136830,#136831,#136832,
#136833),.UNSPECIFIED.,.F.,.F.,(4,1,1,1,1,1,1,1,1,1,1,4),(2.16135430569987E-6,
0.0624986405827758,0.124998731210682,0.187498821838588,0.249998912466494,
0.3124990030944,0.374999093722306,0.499999274978118,0.624999456233931,0.749999637489742,
0.874999818745554,1.),.UNSPECIFIED.);
#29777=B_SPLINE_CURVE_WITH_KNOTS('',3,(#136835,#136836,#136837,#136838,
#136839,#136840,#136841,#136842,#136843,#136844,#136845,#136846),
 .UNSPECIFIED.,.F.,.F.,(4,2,2,2,2,4),(1.00000004342141E-6,0.403419775728668,
0.804091688335629,1.59898592457929,2.38592377386386,3.42850354275929),
 .UNSPECIFIED.);
#29778=B_SPLINE_CURVE_WITH_KNOTS('',3,(#136847,#136848,#136849,#136850,
#136851,#136852,#136853,#136854,#136855,#136856,#136857,#136858,#136859,
#136860,#136861,#136862,#136863,#136864,#136865,#136866,#136867,#136868,
#136869,#136870,#136871,#136872,#136873,#136874,#136875,#136876,#136877,
#136878,#136879,#136880,#136881,#136882,#136883,#136884,#136885,#136886,
#136887,#136888,#136889,#136890,#136891,#136892,#136893,#136894,#136895,
#136896,#136897,#136898,#136899,#136900,#136901),.UNSPECIFIED.,.F.,.F.,
(4,3,3,3,3,3,3,3,3,3,3,3,3,3,3,3,3,3,4),(0.,0.1249992580603,0.2499985161206,
0.3124981451508,0.3437479596658,0.3515604132946,0.355466640109,0.3593728669234,
0.3671853205522,0.3749977741809,0.4374974032111,0.4999970322412,0.6249962903015,
0.6874959193317,0.7499955483619,0.812495177392,0.8749948064222,0.9374944354523,
0.999997046746475),.UNSPECIFIED.);
#29779=B_SPLINE_CURVE_WITH_KNOTS('',3,(#137189,#137190,#137191,#137192,
#137193,#137194,#137195,#137196,#137197,#137198,#137199,#137200),
 .UNSPECIFIED.,.F.,.F.,(4,2,2,2,2,4),(-3.42848865728252,-2.38586959064534,
-1.59889051136132,-0.80404245339222,-0.403394192455397,-1.00000004321643E-6),
 .UNSPECIFIED.);
#29780=B_SPLINE_CURVE_WITH_KNOTS('',3,(#137201,#137202,#137203,#137204,
#137205,#137206,#137207,#137208,#137209,#137210,#137211,#137212,#137213,
#137214,#137215,#137216,#137217,#137218,#137219,#137220,#137221,#137222,
#137223,#137224,#137225,#137226,#137227,#137228,#137229,#137230,#137231,
#137232,#137233,#137234,#137235,#137236,#137237,#137238,#137239,#137240,
#137241,#137242,#137243,#137244,#137245,#137246,#137247,#137248,#137249,
#137250,#137251,#137252,#137253,#137254,#137255,#137256,#137257,#137258,
#137259,#137260,#137261,#137262,#137263,#137264,#137265,#137266,#137267,
#137268,#137269,#137270,#137271,#137272,#137273,#137274,#137275,#137276,
#137277,#137278,#137279,#137280,#137281,#137282,#137283,#137284,#137285,
#137286,#137287,#137288,#137289,#137290,#137291,#137292,#137293,#137294,
#137295,#137296,#137297,#137298,#137299,#137300,#137301,#137302,#137303,
#137304,#137305,#137306,#137307,#137308,#137309,#137310,#137311,#137312,
#137313,#137314,#137315,#137316,#137317,#137318,#137319,#137320,#137321,
#137322,#137323,#137324,#137325,#137326,#137327,#137328,#137329,#137330,
#137331,#137332,#137333,#137334,#137335,#137336,#137337,#137338,#137339,
#137340,#137341,#137342,#137343,#137344,#137345,#137346,#137347,#137348,
#137349,#137350,#137351,#137352,#137353,#137354,#137355,#137356,#137357,
#137358,#137359,#137360,#137361,#137362,#137363,#137364,#137365,#137366,
#137367,#137368,#137369,#137370,#137371,#137372,#137373,#137374,#137375,
#137376,#137377,#137378,#137379,#137380,#137381,#137382,#137383,#137384,
#137385,#137386,#137387,#137388,#137389,#137390,#137391,#137392,#137393,
#137394,#137395,#137396,#137397,#137398,#137399,#137400,#137401,#137402,
#137403,#137404,#137405,#137406,#137407,#137408,#137409,#137410,#137411,
#137412,#137413,#137414,#137415,#137416,#137417,#137418,#137419,#137420,
#137421,#137422,#137423,#137424,#137425,#137426,#137427,#137428,#137429,
#137430,#137431,#137432,#137433,#137434,#137435,#137436,#137437,#137438,
#137439,#137440,#137441,#137442,#137443,#137444,#137445,#137446,#137447,
#137448,#137449,#137450,#137451,#137452,#137453,#137454,#137455,#137456,
#137457,#137458,#137459,#137460,#137461,#137462,#137463,#137464,#137465,
#137466,#137467,#137468,#137469,#137470,#137471,#137472,#137473,#137474,
#137475,#137476,#137477,#137478,#137479,#137480,#137481,#137482,#137483,
#137484,#137485,#137486,#137487,#137488,#137489,#137490,#137491,#137492,
#137493,#137494,#137495,#137496,#137497,#137498,#137499,#137500,#137501,
#137502,#137503,#137504,#137505,#137506,#137507,#137508,#137509,#137510,
#137511,#137512,#137513,#137514,#137515,#137516,#137517,#137518,#137519,
#137520,#137521,#137522,#137523,#137524,#137525,#137526,#137527,#137528,
#137529,#137530,#137531,#137532,#137533,#137534,#137535,#137536,#137537,
#137538,#137539,#137540,#137541,#137542,#137543,#137544,#137545,#137546,
#137547,#137548,#137549,#137550,#137551,#137552,#137553,#137554,#137555,
#137556,#137557,#137558,#137559,#137560,#137561,#137562,#137563,#137564,
#137565,#137566,#137567,#137568,#137569,#137570,#137571,#137572,#137573,
#137574,#137575,#137576,#137577,#137578,#137579,#137580,#137581,#137582,
#137583,#137584,#137585,#137586,#137587,#137588,#137589,#137590,#137591,
#137592,#137593,#137594,#137595,#137596,#137597,#137598,#137599,#137600,
#137601,#137602,#137603,#137604,#137605,#137606,#137607,#137608,#137609),
 .UNSPECIFIED.,.F.,.F.,(4,3,3,3,3,3,3,3,3,3,3,3,3,3,3,3,3,3,3,3,3,3,3,3,
3,3,3,3,3,3,3,3,3,3,3,3,3,3,3,3,3,3,3,3,3,3,3,3,3,3,3,3,3,3,3,3,3,3,3,3,
3,3,3,3,3,3,3,3,3,3,3,3,3,3,3,3,3,3,3,3,3,3,3,3,3,3,3,3,3,3,3,3,3,3,3,3,
3,3,3,3,3,3,3,3,3,3,3,3,3,3,3,3,3,3,3,3,3,3,3,3,3,3,3,3,3,3,3,3,3,3,3,3,
3,3,3,3,4),(6.47368976766051E-6,0.00725838257496969,0.0141323813951552,
0.0156249999999179,0.0221230041052499,0.0234374999998775,0.0278231632375317,
0.0312499999998371,0.0412979481287643,0.0515362268175401,0.0546874999997163,
0.0585937499996962,0.0614614635536616,0.0624225099282763,0.0624999999996762,
0.0692488858490118,0.0759171946668936,0.0824400660205615,0.0859374999995616,
0.0898437499995427,0.0917968749995329,0.093362181664774,0.0937499999995232,
0.101619833110208,0.109489660904306,0.1171874999994,0.121093749999379,0.12304687499937,
0.124023437499365,0.124511718749363,0.124999999999361,0.125000421843579,
0.156249999999298,0.171874999999267,0.179687499999252,0.183593749999245,
0.187255859374237,0.187499999999235,0.187812734412932,0.193285114515677,
0.198943721724235,0.204940610861751,0.210937499999267,0.214843749999272,
0.216796874999274,0.217773437499276,0.21864351577971,0.218749999999278,
0.224777092603502,0.230968753176944,0.237434536816778,0.242187499999301,
0.246093749999304,0.248046874999305,0.249023437499305,0.249999999999305,
0.250000896937272,0.258949631909927,0.26861453161126,0.279019268751896,
0.291936888674985,0.296874999999176,0.304687499999154,0.308593749999144,
0.310546874999139,0.311523437499137,0.312011718749137,0.312438123073067,
0.312499999999136,0.327192126832278,0.342180569775975,0.357615807070226,
0.35937499999909,0.367187499999082,0.371093749999079,0.373046874999077,
0.374023437499076,0.374511718749076,0.37486588780349,0.374999999999077,
0.389541902170744,0.405702934607373,0.421874999999136,0.429687499999146,
0.433593749999152,0.435546874999154,0.437499999999156,0.450421377890763,
0.4637608580172,0.477821333311977,0.484374999999216,0.492187499999226,0.496093749999231,
0.498046874999233,0.499023437499234,0.499511718749235,0.499999999999237,
0.50000061815793,0.518844646217501,0.539458313992307,0.563321627450737,
0.580035098181879,0.599659339325083,0.609374999999321,0.617187499999327,
0.621093749999329,0.623046874999331,0.624023437499331,0.62475585937433,
0.624912515890386,0.62499999999933,0.632203687527198,0.639579179896025,
0.643289262967552,0.647014480029964,0.654511066905249,0.685142110349945,
0.718749999999486,0.734374999999512,0.742187499999524,0.74609374999953,
0.749023437499535,0.749862397068581,0.749999999999536,0.796874999999623,
0.833576459585674,0.843749999999709,0.859374999999738,0.867187499999752,
0.871093749999759,0.873046874999763,0.874991355581291,0.874999999999767,
0.902852656589029,0.932807157055022,0.964284959295619,1.),.UNSPECIFIED.);
#29781=B_SPLINE_CURVE_WITH_KNOTS('',3,(#137835,#137836,#137837,#137838,
#137839,#137840,#137841,#137842,#137843,#137844,#137845,#137846),
 .UNSPECIFIED.,.F.,.F.,(4,2,2,2,2,4),(5.39127788108557E-6,0.702745616718545,
1.35698856532349,2.35941555843787,3.02455033620795,3.69163212190561),
 .UNSPECIFIED.);
#29782=B_SPLINE_CURVE_WITH_KNOTS('',3,(#137850,#137851,#137852,#137853,
#137854,#137855,#137856,#137857,#137858,#137859,#137860,#137861,#137862,
#137863,#137864,#137865,#137866,#137867,#137868,#137869,#137870,#137871,
#137872,#137873,#137874,#137875,#137876,#137877,#137878,#137879,#137880),
 .UNSPECIFIED.,.F.,.F.,(4,3,3,3,3,3,3,3,3,3,4),(0.,0.149815463957079,0.25,
0.402389145397824,0.4375,0.481435618988557,0.5,0.638702449716338,0.775917053246462,
0.911161507515076,1.),.UNSPECIFIED.);
#29783=B_SPLINE_CURVE_WITH_KNOTS('',3,(#137883,#137884,#137885,#137886,
#137887,#137888,#137889,#137890,#137891,#137892),.UNSPECIFIED.,.F.,.F.,
(4,2,2,2,4),(0.,0.25,0.5,0.75,1.),.UNSPECIFIED.);
#29784=B_SPLINE_CURVE_WITH_KNOTS('',3,(#137897,#137898,#137899,#137900,
#137901,#137902,#137903,#137904,#137905,#137906,#137907,#137908,#137909,
#137910,#137911,#137912,#137913,#137914,#137915,#137916,#137917,#137918,
#137919,#137920,#137921,#137922,#137923,#137924,#137925,#137926,#137927,
#137928,#137929,#137930,#137931,#137932),.UNSPECIFIED.,.F.,.F.,(4,2,2,2,
1,1,1,2,2,2,2,2,2,2,1,1,1,2,2,2,4),(0.,0.124999999999928,0.187499999999891,
0.218749999999872,0.234374999999863,0.242187499999859,0.246093749999857,
0.248046874999856,0.249999999999856,0.374999999999863,0.499999999999871,
0.624999999999879,0.687499999999884,0.718749999999886,0.734374999999888,
0.742187499999889,0.746093749999889,0.74804687499989,0.74999999999989,0.874999999999945,
1.),.UNSPECIFIED.);
#29785=B_SPLINE_CURVE_WITH_KNOTS('',3,(#137935,#137936,#137937,#137938,
#137939,#137940,#137941,#137942,#137943,#137944,#137945,#137946,#137947,
#137948,#137949,#137950,#137951,#137952,#137953,#137954,#137955,#137956,
#137957,#137958,#137959,#137960,#137961,#137962,#137963,#137964,#137965,
#137966,#137967,#137968,#137969,#137970,#137971,#137972,#137973,#137974,
#137975,#137976,#137977,#137978,#137979,#137980,#137981,#137982,#137983,
#137984,#137985,#137986,#137987,#137988,#137989,#137990,#137991,#137992,
#137993,#137994,#137995,#137996,#137997,#137998,#137999,#138000,#138001,
#138002,#138003,#138004,#138005,#138006,#138007,#138008,#138009,#138010,
#138011,#138012,#138013,#138014,#138015,#138016,#138017,#138018,#138019,
#138020,#138021,#138022,#138023,#138024,#138025,#138026,#138027,#138028,
#138029,#138030,#138031,#138032,#138033,#138034,#138035,#138036,#138037,
#138038,#138039,#138040,#138041,#138042,#138043,#138044,#138045,#138046,
#138047,#138048,#138049,#138050,#138051,#138052,#138053,#138054,#138055,
#138056,#138057,#138058,#138059,#138060,#138061,#138062,#138063,#138064,
#138065,#138066,#138067,#138068,#138069,#138070,#138071,#138072,#138073,
#138074,#138075,#138076,#138077,#138078,#138079,#138080,#138081,#138082,
#138083,#138084,#138085,#138086,#138087,#138088,#138089,#138090,#138091,
#138092,#138093,#138094,#138095,#138096,#138097,#138098,#138099,#138100,
#138101,#138102,#138103,#138104,#138105,#138106,#138107,#138108,#138109,
#138110,#138111,#138112,#138113,#138114,#138115,#138116,#138117,#138118,
#138119,#138120,#138121,#138122,#138123,#138124),.UNSPECIFIED.,.F.,.F.,
(4,3,3,3,3,3,3,3,3,3,3,3,3,3,3,3,3,3,3,3,3,3,3,3,3,3,3,3,3,3,3,3,3,3,3,
3,3,3,3,3,3,3,3,3,3,3,3,3,3,3,3,3,3,3,3,3,3,3,3,3,3,3,3,4),(7.48046056638122E-14,
0.0567206634532088,0.062499999999308,0.0937499999989595,0.109374999998785,
0.117187499998698,0.121093749998655,0.123046874998633,0.124023437498624,
0.124999999998615,0.136819606049853,0.148727050045804,0.156249999998778,
0.168434086306113,0.17187499999886,0.179687499998901,0.183593749998921,
0.185546874998933,0.186523437498939,0.187499999998944,0.212520418034415,
0.218749999999069,0.234374999999131,0.242187499999162,0.246093749999176,
0.249793570825364,0.249999999999189,0.292343721475176,0.312499999999426,
0.343749999999545,0.359374999999606,0.367187499999637,0.371093749999655,
0.374511718749671,0.374999999999672,0.391450481329379,0.408065573550668,
0.424947768379996,0.437499999999929,0.455064117344876,0.468750000000057,
0.484375000000121,0.492187500000154,0.49609375000017,0.498046875000178,
0.499023437500183,0.499511718750185,0.500000000000188,0.543812045995623,
0.587944303750082,0.625000000000253,0.687500000000286,0.718750000000301,
0.734375000000308,0.742187500000312,0.749023437500313,0.750000000000313,
0.792697234305152,0.835164563984767,0.875000000000156,0.910161204145841,
0.944986000859805,0.979192521511994,1.),.UNSPECIFIED.);
#29786=B_SPLINE_CURVE_WITH_KNOTS('',3,(#138233,#138234,#138235,#138236,
#138237,#138238,#138239,#138240,#138241),.UNSPECIFIED.,.F.,.F.,(4,1,1,1,
1,1,4),(0.,0.249667236143351,0.375008055254049,0.500348874364846,0.625689693475543,
0.75103051258624,1.),.UNSPECIFIED.);
#29787=B_SPLINE_CURVE_WITH_KNOTS('',3,(#138242,#138243,#138244,#138245,
#138246,#138247,#138248,#138249,#138250),.UNSPECIFIED.,.F.,.F.,(4,1,1,1,
1,1,4),(0.,0.2489687868754,0.3743093060332,0.499649825191,0.6249903443489,
0.7503308635067,1.),.UNSPECIFIED.);
#29788=B_SPLINE_CURVE_WITH_KNOTS('',3,(#138368,#138369,#138370,#138371,
#138372,#138373,#138374,#138375,#138376),.UNSPECIFIED.,.F.,.F.,(4,1,1,1,
1,1,4),(0.,0.249612957690097,0.37469441872057,0.499775879751044,0.624857340781618,
0.749938801812092,1.),.UNSPECIFIED.);
#29789=B_SPLINE_CURVE_WITH_KNOTS('',3,(#138393,#138394,#138395,#138396,
#138397,#138398,#138399,#138400,#138401,#138402,#138403,#138404,#138405,
#138406,#138407,#138408,#138409,#138410,#138411),.UNSPECIFIED.,.F.,.F.,
(4,3,3,3,3,3,4),(0.,0.249979519116017,0.3749906021302,0.500001685144484,
0.625012768158668,0.750023851172851,1.),.UNSPECIFIED.);
#29790=B_SPLINE_CURVE_WITH_KNOTS('',3,(#138556,#138557,#138558,#138559,
#138560,#138561,#138562,#138563,#138564),.UNSPECIFIED.,.F.,.F.,(4,1,1,1,
1,1,4),(0.,0.249978015946122,0.374989466361611,0.500000916777201,0.62501236719269,
0.750023817608178,1.),.UNSPECIFIED.);
#29791=B_SPLINE_CURVE_WITH_KNOTS('',3,(#138651,#138652,#138653,#138654,
#138655,#138656,#138657,#138658,#138659,#138660,#138661,#138662,#138663),
 .UNSPECIFIED.,.F.,.F.,(4,2,2,2,2,1,4),(0.,0.250000000000001,0.500000000000002,
0.625000000000002,0.750000000000001,0.875000000000001,1.),.UNSPECIFIED.);
#29792=B_SPLINE_CURVE_WITH_KNOTS('',3,(#138668,#138669,#138670,#138671,
#138672,#138673,#138674,#138675,#138676,#138677,#138678,#138679,#138680,
#138681,#138682,#138683,#138684,#138685,#138686,#138687,#138688,#138689,
#138690,#138691,#138692,#138693,#138694,#138695,#138696,#138697,#138698,
#138699,#138700,#138701,#138702,#138703),.UNSPECIFIED.,.F.,.F.,(4,2,2,2,
1,1,1,2,2,2,2,2,2,2,1,1,1,2,2,2,4),(0.,0.124999999999949,0.187499999999923,
0.218749999999911,0.234374999999906,0.242187499999904,0.246093749999903,
0.248046874999902,0.249999999999901,0.374999999999893,0.499999999999885,
0.624999999999877,0.687499999999873,0.718749999999871,0.73437499999987,
0.74218749999987,0.746093749999869,0.748046874999869,0.749999999999869,
0.874999999999935,1.),.UNSPECIFIED.);
#29793=B_SPLINE_CURVE_WITH_KNOTS('',3,(#138706,#138707,#138708,#138709,
#138710,#138711,#138712,#138713,#138714,#138715),.UNSPECIFIED.,.F.,.F.,
(4,2,2,2,4),(0.,0.25,0.5,0.75,1.),.UNSPECIFIED.);
#29794=B_SPLINE_CURVE_WITH_KNOTS('',3,(#138942,#138943,#138944,#138945,
#138946,#138947,#138948,#138949,#138950,#138951,#138952,#138953,#138954,
#138955,#138956,#138957,#138958,#138959,#138960,#138961,#138962,#138963,
#138964,#138965,#138966,#138967,#138968,#138969),.UNSPECIFIED.,.F.,.F.,
(4,3,3,3,3,3,3,3,3,4),(0.,0.117080806693866,0.233583246000496,0.348303590725999,
0.46135301553334,0.5,0.625,0.744908083513982,0.872454041756991,1.),
 .UNSPECIFIED.);
#29795=B_SPLINE_CURVE_WITH_KNOTS('',3,(#138970,#138971,#138972,#138973,
#138974,#138975,#138976,#138977,#138978,#138979,#138980,#138981),
 .UNSPECIFIED.,.F.,.F.,(4,2,2,2,2,4),(-3.42420775850897,-2.83987518299694,
-2.25725819870026,-1.34987067298873,-0.707053266798169,-5.39057101361098E-6),
 .UNSPECIFIED.);
#29796=B_SPLINE_CURVE_WITH_KNOTS('',3,(#138987,#138988,#138989,#138990,
#138991,#138992,#138993,#138994,#138995,#138996,#138997,#138998,#138999,
#139000,#139001,#139002,#139003,#139004,#139005,#139006,#139007,#139008,
#139009,#139010,#139011,#139012,#139013,#139014,#139015,#139016,#139017,
#139018,#139019,#139020,#139021,#139022,#139023),.UNSPECIFIED.,.F.,.F.,
(4,1,1,1,1,1,1,1,1,1,1,1,1,1,1,1,1,1,1,1,1,1,1,1,1,1,1,1,1,1,1,1,1,1,4),
(0.,0.02941176470588,0.05882352941176,0.08823529411765,0.1176470588235,
0.1470588235294,0.1764705882353,0.2058823529412,0.2352941176471,0.2647058823529,
0.2941176470588,0.3235294117647,0.3529411764706,0.3823529411765,0.4117647058824,
0.4411764705882,0.4705882352941,0.5,0.5294117647059,0.5588235294118,0.5882352941176,
0.6176470588235,0.6470588235294,0.6764705882353,0.7058823529412,0.7352941176471,
0.7647058823529,0.7941176470588,0.8235294117647,0.8529411764706,0.8823529411765,
0.9117647058824,0.9411764705882,0.9705882352941,0.999994374858691),
 .UNSPECIFIED.);
#29797=B_SPLINE_CURVE_WITH_KNOTS('',3,(#139025,#139026,#139027,#139028,
#139029,#139030,#139031,#139032,#139033,#139034,#139035,#139036,#139037,
#139038,#139039,#139040,#139041,#139042,#139043,#139044,#139045,#139046,
#139047,#139048,#139049,#139050,#139051,#139052,#139053,#139054,#139055,
#139056,#139057,#139058,#139059,#139060,#139061,#139062,#139063,#139064),
 .UNSPECIFIED.,.F.,.F.,(4,3,3,3,3,3,3,3,3,3,3,3,3,4),(0.,0.07692307692308,
0.1538461538462,0.2307692307692,0.3076923076923,0.3846153846154,0.4615384615385,
0.5384615384615,0.6153846153846,0.6923076923077,0.7692307692308,0.8461538461538,
0.9230769230769,1.),.UNSPECIFIED.);
#29798=B_SPLINE_CURVE_WITH_KNOTS('',3,(#139068,#139069,#139070,#139071,
#139072,#139073,#139074,#139075,#139076,#139077,#139078,#139079,#139080,
#139081,#139082,#139083,#139084,#139085,#139086,#139087,#139088,#139089,
#139090,#139091,#139092,#139093,#139094,#139095,#139096,#139097,#139098,
#139099,#139100,#139101,#139102,#139103,#139104,#139105,#139106,#139107),
 .UNSPECIFIED.,.F.,.F.,(4,3,3,3,3,3,3,3,3,3,3,3,3,4),(0.,0.07692307692308,
0.1538461538462,0.2307692307692,0.3076923076923,0.3846153846154,0.4615384615385,
0.5384615384615,0.6153846153846,0.6923076923077,0.7692307692308,0.8461538461538,
0.9230769230769,0.999990181765799),.UNSPECIFIED.);
#29799=B_SPLINE_CURVE_WITH_KNOTS('',3,(#139108,#139109,#139110,#139111,
#139112,#139113,#139114,#139115,#139116,#139117,#139118,#139119,#139120,
#139121,#139122,#139123,#139124,#139125,#139126,#139127,#139128,#139129,
#139130,#139131,#139132,#139133,#139134,#139135,#139136,#139137,#139138,
#139139,#139140),.UNSPECIFIED.,.F.,.F.,(4,1,1,1,1,1,1,1,1,1,1,1,1,1,1,1,
1,1,1,1,1,1,1,1,1,1,1,1,1,1,4),(0.,0.03333333333333,0.06666666666667,0.1,
0.1333333333333,0.1666666666667,0.2,0.2333333333333,0.2666666666667,0.3,
0.3333333333333,0.3666666666667,0.4,0.4333333333333,0.4666666666667,0.5,
0.5333333333333,0.5666666666667,0.6,0.6333333333333,0.6666666666667,0.7,
0.7333333333333,0.7666666666667,0.8,0.8333333333333,0.8666666666667,0.9,
0.9333333333333,0.9666666666667,1.),.UNSPECIFIED.);
#29800=B_SPLINE_CURVE_WITH_KNOTS('',3,(#139143,#139144,#139145,#139146,
#139147,#139148,#139149,#139150,#139151,#139152,#139153,#139154,#139155,
#139156,#139157,#139158,#139159,#139160,#139161,#139162,#139163,#139164,
#139165,#139166,#139167,#139168,#139169,#139170,#139171,#139172,#139173,
#139174,#139175,#139176,#139177,#139178,#139179,#139180,#139181,#139182,
#139183,#139184,#139185,#139186,#139187,#139188,#139189,#139190,#139191,
#139192,#139193,#139194),.UNSPECIFIED.,.F.,.F.,(4,3,3,3,3,3,3,3,3,3,3,3,
3,3,3,3,3,4),(0.,0.0104300641450095,0.0403038134976636,0.0731177483969922,
0.109196822930784,0.148840753280782,0.192353399031002,0.240049789161611,
0.292260775959177,0.349343693489284,0.412033590379295,0.481362584134171,
0.557244485460841,0.640756781399926,0.733854635093322,0.838472312208226,
0.95702604171734,1.),.UNSPECIFIED.);
#29801=B_SPLINE_CURVE_WITH_KNOTS('',3,(#139195,#139196,#139197,#139198,
#139199,#139200,#139201,#139202,#139203,#139204,#139205,#139206,#139207,
#139208,#139209,#139210,#139211,#139212,#139213,#139214,#139215,#139216,
#139217,#139218,#139219,#139220,#139221,#139222,#139223,#139224,#139225,
#139226,#139227,#139228,#139229,#139230,#139231,#139232,#139233,#139234,
#139235,#139236,#139237),.UNSPECIFIED.,.F.,.F.,(4,3,3,3,3,3,3,3,3,3,3,3,
3,3,4),(0.,0.0569254788267774,0.181698225622002,0.29475495478262,0.397219013347534,
0.490602660719935,0.576270367287962,0.653393539486814,0.721886944980528,
0.78340723675226,0.83937561533012,0.890301000193252,0.936516969810281,0.978362059982727,
1.),.UNSPECIFIED.);
#29802=B_SPLINE_CURVE_WITH_KNOTS('',3,(#139469,#139470,#139471,#139472,
#139473,#139474,#139475,#139476,#139477,#139478,#139479,#139480,#139481,
#139482,#139483,#139484,#139485,#139486,#139487,#139488,#139489,#139490,
#139491,#139492,#139493,#139494,#139495,#139496,#139497,#139498,#139499,
#139500,#139501,#139502,#139503,#139504,#139505,#139506,#139507,#139508,
#139509,#139510,#139511,#139512,#139513,#139514,#139515,#139516,#139517,
#139518,#139519,#139520,#139521,#139522,#139523,#139524,#139525,#139526,
#139527,#139528,#139529,#139530,#139531,#139532,#139533,#139534,#139535,
#139536,#139537,#139538,#139539,#139540,#139541,#139542,#139543,#139544,
#139545,#139546,#139547,#139548,#139549,#139550,#139551,#139552,#139553,
#139554,#139555,#139556,#139557,#139558,#139559,#139560,#139561,#139562,
#139563,#139564,#139565,#139566,#139567,#139568,#139569,#139570,#139571,
#139572,#139573,#139574,#139575,#139576,#139577,#139578,#139579,#139580,
#139581,#139582,#139583,#139584,#139585,#139586,#139587,#139588,#139589,
#139590,#139591,#139592,#139593,#139594,#139595,#139596,#139597,#139598,
#139599,#139600,#139601,#139602,#139603,#139604,#139605,#139606,#139607,
#139608,#139609,#139610,#139611,#139612,#139613,#139614,#139615,#139616,
#139617,#139618,#139619,#139620,#139621,#139622,#139623,#139624,#139625,
#139626,#139627,#139628,#139629,#139630,#139631,#139632,#139633,#139634,
#139635,#139636,#139637,#139638,#139639,#139640,#139641,#139642,#139643,
#139644,#139645,#139646,#139647,#139648,#139649,#139650,#139651,#139652,
#139653,#139654,#139655,#139656,#139657,#139658,#139659,#139660,#139661,
#139662,#139663,#139664,#139665,#139666,#139667,#139668,#139669,#139670,
#139671,#139672,#139673,#139674,#139675,#139676,#139677,#139678,#139679,
#139680,#139681,#139682,#139683,#139684,#139685,#139686,#139687,#139688,
#139689,#139690,#139691,#139692,#139693,#139694,#139695,#139696,#139697,
#139698,#139699,#139700,#139701,#139702,#139703,#139704,#139705,#139706,
#139707,#139708,#139709,#139710,#139711,#139712,#139713,#139714,#139715,
#139716,#139717,#139718,#139719,#139720,#139721,#139722,#139723,#139724,
#139725,#139726,#139727,#139728,#139729,#139730,#139731,#139732,#139733,
#139734,#139735,#139736,#139737,#139738,#139739,#139740,#139741,#139742,
#139743,#139744,#139745,#139746,#139747,#139748,#139749,#139750,#139751,
#139752,#139753,#139754,#139755,#139756,#139757,#139758,#139759,#139760,
#139761,#139762,#139763,#139764,#139765,#139766,#139767,#139768,#139769,
#139770,#139771,#139772,#139773,#139774,#139775,#139776,#139777,#139778,
#139779,#139780,#139781,#139782,#139783,#139784,#139785,#139786,#139787,
#139788,#139789,#139790,#139791,#139792,#139793,#139794,#139795,#139796,
#139797,#139798,#139799,#139800,#139801,#139802,#139803,#139804,#139805,
#139806,#139807,#139808,#139809,#139810,#139811,#139812,#139813,#139814,
#139815,#139816,#139817,#139818,#139819,#139820,#139821,#139822,#139823,
#139824,#139825,#139826,#139827,#139828,#139829,#139830,#139831,#139832,
#139833,#139834,#139835,#139836,#139837,#139838,#139839,#139840,#139841,
#139842,#139843,#139844,#139845,#139846,#139847,#139848,#139849,#139850,
#139851,#139852,#139853,#139854,#139855,#139856,#139857,#139858,#139859,
#139860,#139861,#139862,#139863,#139864,#139865,#139866,#139867,#139868,
#139869,#139870,#139871,#139872,#139873,#139874,#139875,#139876,#139877,
#139878,#139879,#139880,#139881,#139882,#139883,#139884,#139885,#139886,
#139887,#139888,#139889,#139890,#139891,#139892,#139893,#139894,#139895,
#139896,#139897,#139898,#139899,#139900,#139901,#139902,#139903,#139904,
#139905,#139906,#139907,#139908,#139909,#139910,#139911,#139912,#139913,
#139914,#139915,#139916,#139917,#139918,#139919,#139920,#139921,#139922,
#139923,#139924,#139925,#139926,#139927,#139928,#139929,#139930,#139931,
#139932,#139933,#139934,#139935,#139936,#139937,#139938,#139939,#139940,
#139941,#139942,#139943,#139944,#139945,#139946,#139947,#139948,#139949,
#139950,#139951,#139952,#139953,#139954,#139955,#139956,#139957,#139958,
#139959,#139960,#139961,#139962,#139963,#139964,#139965,#139966,#139967,
#139968,#139969,#139970,#139971,#139972,#139973,#139974,#139975,#139976),
 .UNSPECIFIED.,.F.,.F.,(4,3,3,3,3,3,3,3,3,3,3,3,3,3,3,3,3,3,3,3,3,3,3,3,
3,3,3,3,3,3,3,3,3,3,3,3,3,3,3,3,3,3,3,3,3,3,3,3,3,3,3,3,3,3,3,3,3,3,3,3,
3,3,3,3,3,3,3,3,3,3,3,3,3,3,3,3,3,3,3,3,3,3,3,3,3,3,3,3,3,3,3,3,3,3,3,3,
3,3,3,3,3,3,3,3,3,3,3,3,3,3,3,3,3,3,3,3,3,3,3,3,3,3,3,3,3,3,3,3,3,3,3,3,
3,3,3,3,3,3,3,3,3,3,3,3,3,3,3,3,3,3,3,3,3,3,3,3,3,3,3,3,3,3,3,3,3,3,3,3,
3,4),(5.26314413123426E-7,0.0113155790796151,0.0251388647517376,0.0310479652170974,
0.0312499999999604,0.0453461316134197,0.0504424803060528,0.0546874999999304,
0.0585937499999254,0.060546874999923,0.0615234374999218,0.0624999999999207,
0.068812174829043,0.0868926240447748,0.106944947332055,0.109374999999864,
0.117316441901434,0.124999999999845,0.129323876863945,0.138802102939861,
0.147918081323925,0.150435171341309,0.160121428953758,0.169646632060944,
0.17968749999978,0.183593749999775,0.185546874999773,0.186523437499772,
0.187356316568156,0.18749999999977,0.187612433563859,0.19852836668657,0.207386871759649,
0.210937499999736,0.214843749999731,0.216796874999728,0.217773437499727,
0.218261718749726,0.218627929687226,0.218749999999725,0.222280520679915,
0.223685847591065,0.22735827302368,0.231153270031486,0.235015757477918,
0.238982945278941,0.242461789679081,0.246093749999737,0.248046874999738,
0.249023437499738,0.249511718749739,0.249755859374739,0.249877929687239,
0.249999999999739,0.26375570429153,0.272081592566711,0.286146390012587,
0.297869928440458,0.312213441963219,0.319939108622709,0.334363175203937,
0.338507769117277,0.353008489557291,0.354400873634069,0.359374999999608,
0.367187499999598,0.368187520310837,0.371093749999594,0.373046874999591,
0.37402343749959,0.374877929687089,0.374999999999589,0.386016201521818,
0.408995234585906,0.430287360079277,0.450033444879799,0.468370688663691,
0.468749999999059,0.484374999998971,0.485418078837636,0.492187499998926,
0.496093749998902,0.498046874998891,0.499511718748883,0.499999999998881,
0.502215778241268,0.527808479215655,0.551648453387262,0.573847489919669,
0.594524368852247,0.613814210682214,0.63184891774307,0.648649582659718,
0.664177872392781,0.678439363988811,0.687499999998774,0.691709046355161,
0.69531249999877,0.699218749998768,0.703124999998766,0.7070337496537,0.718749999998772,
0.726954573406456,0.746903046788504,0.749999999998779,0.765624999998783,
0.767111069151479,0.779817712431221,0.781249999998786,0.788479240017865,
0.79687499999879,0.804687499998791,0.808593749998796,0.810546874998799,
0.812499999998802,0.816347726587709,0.825122186626889,0.828124999998883,
0.832031249998907,0.834060327467434,0.83593749999893,0.841284161873138,
0.843749999998977,0.847656249999001,0.849609374999007,0.851562499999012,
0.855274741365915,0.859374999999035,0.865479004774198,0.867187499999057,
0.86836688933082,0.869140624999062,0.871093749999068,0.87314150143147,0.874999999999078,
0.876834002406975,0.878906249999089,0.882812499999099,0.886466989130165,
0.886718749999109,0.889851811247551,0.89062499999912,0.893182462397039,
0.898437499999135,0.902343749999146,0.904296874999155,0.905864048581422,
0.906249999999164,0.912210533917316,0.915434747904591,0.920209721935489,
0.921874999999294,0.924080465062891,0.925781249999328,0.929687499999361,
0.936091306260822,0.943409695495072,0.949693108201396,0.953124999999578,
0.953429994527388,0.958676452650152,0.964971871567472,0.968749999999721,
0.972942846958018,0.976562499999789,0.980800250809871,0.984374999999857,
0.991373939213844,0.993657578315312,1.),.UNSPECIFIED.);
#29803=B_SPLINE_CURVE_WITH_KNOTS('',3,(#140050,#140051,#140052,#140053,
#140054,#140055,#140056,#140057,#140058,#140059,#140060,#140061,#140062,
#140063,#140064,#140065,#140066,#140067,#140068,#140069,#140070,#140071,
#140072,#140073,#140074,#140075,#140076,#140077,#140078,#140079,#140080,
#140081,#140082,#140083,#140084,#140085,#140086,#140087,#140088,#140089,
#140090,#140091,#140092,#140093,#140094,#140095,#140096,#140097,#140098,
#140099,#140100,#140101,#140102,#140103,#140104,#140105,#140106,#140107,
#140108,#140109,#140110,#140111,#140112,#140113,#140114,#140115,#140116,
#140117,#140118,#140119,#140120,#140121,#140122,#140123,#140124,#140125,
#140126,#140127,#140128,#140129,#140130,#140131,#140132,#140133,#140134),
 .UNSPECIFIED.,.F.,.F.,(4,3,3,3,3,3,3,3,3,3,3,3,3,3,3,3,3,3,3,3,3,3,3,3,
3,3,3,3,4),(1.46586088669429E-9,0.0147856209054546,0.0788187793390021,0.148252710563286,
0.223677641753622,0.249999999999859,0.305663645075048,0.374999999999792,
0.394777161192625,0.437499999999753,0.468749999999731,0.484374999999723,
0.491632695048001,0.492187499999724,0.499999999999724,0.565831577623568,
0.589741931466674,0.65688948573569,0.669154414594773,0.687499999999827,
0.718749999999843,0.734374999999853,0.739649768105247,0.74218749999986,
0.749999999999866,0.806188103222823,0.879930291384157,0.963019849159479,
1.),.UNSPECIFIED.);
#29804=B_SPLINE_CURVE_WITH_KNOTS('',3,(#140177,#140178,#140179,#140180,
#140181,#140182,#140183,#140184,#140185,#140186,#140187,#140188,#140189,
#140190,#140191,#140192,#140193,#140194,#140195,#140196,#140197,#140198,
#140199,#140200,#140201,#140202,#140203,#140204,#140205,#140206,#140207,
#140208,#140209,#140210,#140211,#140212,#140213,#140214,#140215,#140216,
#140217,#140218,#140219,#140220,#140221,#140222,#140223,#140224,#140225,
#140226,#140227,#140228,#140229,#140230,#140231,#140232,#140233,#140234,
#140235,#140236,#140237,#140238,#140239,#140240,#140241,#140242,#140243),
 .UNSPECIFIED.,.F.,.F.,(4,3,3,3,3,3,3,3,3,3,3,3,3,3,3,3,3,3,3,3,3,3,4),
(0.,0.0624999999999875,0.124999999999975,0.182979972803975,0.187499999999971,
0.215193239530195,0.242577553898054,0.249999999999967,0.329473835291726,
0.40895094369529,0.437499999999961,0.468749999999968,0.483425128960071,
0.497765120795587,0.499999999999974,0.572711351548969,0.645848264911811,
0.719643398937141,0.749999999999987,0.824765188414245,0.899992548619747,
0.975917224544569,1.),.UNSPECIFIED.);
#29805=B_SPLINE_CURVE_WITH_KNOTS('',3,(#140245,#140246,#140247,#140248,
#140249,#140250,#140251,#140252,#140253,#140254,#140255,#140256,#140257,
#140258,#140259,#140260,#140261,#140262,#140263,#140264,#140265,#140266,
#140267,#140268,#140269,#140270,#140271,#140272,#140273,#140274,#140275,
#140276,#140277,#140278,#140279,#140280,#140281,#140282,#140283,#140284,
#140285,#140286,#140287,#140288,#140289,#140290,#140291,#140292,#140293,
#140294,#140295,#140296,#140297,#140298,#140299,#140300,#140301,#140302,
#140303,#140304,#140305,#140306,#140307,#140308,#140309,#140310,#140311,
#140312,#140313,#140314,#140315,#140316,#140317,#140318,#140319,#140320,
#140321,#140322,#140323,#140324,#140325,#140326,#140327,#140328,#140329,
#140330,#140331,#140332,#140333,#140334,#140335,#140336,#140337,#140338,
#140339,#140340,#140341,#140342,#140343,#140344,#140345,#140346,#140347,
#140348,#140349,#140350,#140351,#140352,#140353,#140354,#140355,#140356,
#140357,#140358,#140359,#140360,#140361,#140362,#140363,#140364,#140365),
 .UNSPECIFIED.,.F.,.F.,(4,3,3,3,3,3,3,3,3,3,3,3,3,3,3,3,3,3,3,3,3,3,3,3,
3,3,3,3,3,3,3,3,3,3,3,3,3,3,3,3,4),(4.84503357369714E-12,0.0625000000038769,
0.119886196849213,0.125000000002909,0.179080353524112,0.187500000004363,
0.218750000005092,0.234375000005453,0.242187500005639,0.250000000005825,
0.312500000007308,0.343750000008051,0.359375000008415,0.367187500008598,
0.374023437508775,0.375000000008799,0.392863091523399,0.40625000000836,
0.421875000008141,0.429687500008027,0.433593750007968,0.435546875007939,
0.437500000007909,0.440114549658553,0.472413623124356,0.500000000007027,
0.547747027865969,0.592672173262821,0.625000000005261,0.665016457000979,
0.687500000004373,0.718750000003932,0.734375000003712,0.746910733725364,
0.750000000003492,0.791768980893818,0.83477727983257,0.875000000001746,
0.92207412377465,0.972243230788792,1.),.UNSPECIFIED.);
#29806=B_SPLINE_CURVE_WITH_KNOTS('',3,(#140366,#140367,#140368,#140369,
#140370,#140371,#140372,#140373,#140374,#140375,#140376,#140377,#140378,
#140379,#140380,#140381,#140382,#140383,#140384,#140385,#140386,#140387,
#140388,#140389,#140390,#140391,#140392,#140393,#140394,#140395,#140396,
#140397,#140398,#140399,#140400,#140401,#140402,#140403,#140404,#140405,
#140406,#140407,#140408,#140409,#140410,#140411,#140412,#140413,#140414,
#140415,#140416,#140417,#140418,#140419,#140420,#140421,#140422,#140423),
 .UNSPECIFIED.,.F.,.F.,(4,3,3,3,3,3,3,3,3,3,3,3,3,3,3,3,3,3,3,4),(1.2576115163105E-9,
0.0582372114102846,0.115345099826069,0.171871515531986,0.227755575554621,
0.25,0.30535089973337,0.360932037266699,0.415956126690006,0.471025812356985,
0.526253513839453,0.58219013537959,0.638316250545109,0.695300688824847,
0.75,0.808269975267283,0.867972281236829,0.928599616214729,0.990708785988877,
1.),.UNSPECIFIED.);
#29807=B_SPLINE_CURVE_WITH_KNOTS('',3,(#140442,#140443,#140444,#140445,
#140446,#140447,#140448,#140449,#140450,#140451,#140452,#140453,#140454,
#140455,#140456,#140457,#140458,#140459,#140460,#140461,#140462,#140463,
#140464,#140465,#140466,#140467,#140468,#140469,#140470,#140471,#140472,
#140473,#140474,#140475,#140476,#140477,#140478,#140479,#140480,#140481,
#140482,#140483,#140484,#140485,#140486,#140487,#140488,#140489,#140490,
#140491,#140492,#140493,#140494,#140495,#140496,#140497,#140498,#140499),
 .UNSPECIFIED.,.F.,.F.,(4,3,3,3,3,3,3,3,3,3,3,3,3,3,3,3,3,3,3,4),(5.75195662416378E-12,
0.062500000004314,0.120799294736565,0.178331807923707,0.234974821688961,
0.25,0.305845453226057,0.3613647715728,0.416311125147688,0.471089488762509,
0.525811881558363,0.581858911168772,0.636959838781275,0.693479919390638,
0.75,0.806575787009208,0.864269428679939,0.922683317676143,0.982337040140753,
1.),.UNSPECIFIED.);
#29808=B_SPLINE_CURVE_WITH_KNOTS('',3,(#140532,#140533,#140534,#140535),
 .UNSPECIFIED.,.F.,.F.,(4,4),(0.,1.),.UNSPECIFIED.);
#29809=B_SPLINE_CURVE_WITH_KNOTS('',3,(#140537,#140538,#140539,#140540,
#140541,#140542,#140543,#140544,#140545,#140546),.UNSPECIFIED.,.F.,.F.,
(4,2,2,2,4),(1.0680348650496E-8,0.25,0.5,0.75,1.),.UNSPECIFIED.);
#29810=B_SPLINE_CURVE_WITH_KNOTS('',3,(#140548,#140549,#140550,#140551,
#140552,#140553,#140554),.UNSPECIFIED.,.F.,.F.,(4,3,4),(0.,0.362128916600015,
1.),.UNSPECIFIED.);
#29811=B_SPLINE_CURVE_WITH_KNOTS('',3,(#140555,#140556,#140557,#140558,
#140559,#140560,#140561,#140562,#140563,#140564),.UNSPECIFIED.,.F.,.F.,
(4,2,2,2,4),(0.,0.25,0.5,0.75,1.),.UNSPECIFIED.);
#29812=B_SPLINE_CURVE_WITH_KNOTS('',3,(#140595,#140596,#140597,#140598,
#140599,#140600,#140601,#140602,#140603,#140604,#140605,#140606,#140607,
#140608,#140609,#140610,#140611,#140612,#140613,#140614,#140615,#140616,
#140617,#140618,#140619,#140620,#140621,#140622,#140623,#140624,#140625,
#140626,#140627,#140628,#140629,#140630,#140631,#140632,#140633,#140634,
#140635,#140636,#140637,#140638,#140639,#140640,#140641,#140642,#140643,
#140644,#140645,#140646),.UNSPECIFIED.,.F.,.F.,(4,3,3,3,3,3,3,3,3,3,3,3,
3,3,3,3,3,4),(0.,0.0606123631499776,0.121810480050351,0.183182706218067,
0.200869175620174,0.25,0.328361933407609,0.406263651642803,0.479625687786031,
0.5,0.59129802050641,0.682804917911111,0.75,0.757779334258463,0.821554838527955,
0.885141851778926,0.947606732206778,1.),.UNSPECIFIED.);
#29813=B_SPLINE_CURVE_WITH_KNOTS('',3,(#140649,#140650,#140651,#140652,
#140653,#140654,#140655,#140656,#140657,#140658,#140659,#140660,#140661,
#140662,#140663,#140664,#140665,#140666,#140667,#140668,#140669,#140670,
#140671,#140672,#140673,#140674,#140675,#140676,#140677,#140678,#140679,
#140680,#140681,#140682,#140683,#140684,#140685,#140686,#140687,#140688,
#140689,#140690,#140691,#140692,#140693,#140694,#140695,#140696,#140697),
 .UNSPECIFIED.,.F.,.F.,(4,3,3,3,3,3,3,3,3,3,3,3,3,3,3,3,4),(0.,0.101045004834656,
0.1428571428571,0.247561218121864,0.255765081058048,0.2857142857143,0.409190479713353,
0.4285714285714,0.519960169066042,0.56339195277172,0.5714285714286,0.657014403441729,
0.7142857142857,0.717414049033271,0.8571428571429,0.871468788702833,1.),
 .UNSPECIFIED.);
#29814=B_SPLINE_CURVE_WITH_KNOTS('',3,(#140699,#140700,#140701,#140702,
#140703,#140704),.UNSPECIFIED.,.F.,.F.,(4,1,1,4),(0.,0.3333333333333,0.6666666666667,
1.),.UNSPECIFIED.);
#29815=B_SPLINE_CURVE_WITH_KNOTS('',3,(#140706,#140707,#140708,#140709,
#140710,#140711,#140712,#140713,#140714,#140715,#140716,#140717,#140718,
#140719,#140720,#140721,#140722,#140723,#140724,#140725,#140726,#140727,
#140728,#140729,#140730,#140731,#140732,#140733,#140734,#140735,#140736,
#140737,#140738,#140739,#140740,#140741,#140742,#140743,#140744,#140745,
#140746,#140747,#140748,#140749,#140750,#140751,#140752,#140753,#140754,
#140755,#140756,#140757,#140758,#140759,#140760,#140761,#140762,#140763,
#140764,#140765,#140766,#140767,#140768,#140769,#140770,#140771,#140772,
#140773,#140774,#140775,#140776,#140777,#140778,#140779,#140780,#140781,
#140782,#140783,#140784,#140785,#140786,#140787,#140788,#140789,#140790,
#140791,#140792,#140793,#140794,#140795,#140796,#140797,#140798,#140799,
#140800,#140801,#140802,#140803,#140804,#140805),.UNSPECIFIED.,.F.,.F.,
(4,3,3,3,3,3,3,3,3,3,3,3,3,3,3,3,3,3,3,3,3,3,3,3,3,3,3,3,3,3,3,3,3,4),(1.42536501268589E-7,
0.0477654802612144,0.07692307692308,0.12794560731773,0.1538461538462,0.208199907711091,
0.2307692307692,0.288440067990146,0.3076923076923,0.368684577671203,0.3846153846154,
0.440455527634295,0.448926709032301,0.4615384615385,0.515233835999228,0.529168651732405,
0.5384615384615,0.587702308433438,0.609417787020049,0.6153846153846,0.689658855316415,
0.6923076923077,0.733559153082206,0.7692307692308,0.76990413797734,0.809524173197566,
0.8461538461538,0.850154012702905,0.886615467889903,0.921164890063805,0.9230769230769,
0.930386224751045,0.970178482045245,0.999999996823438),.UNSPECIFIED.);
#29816=B_SPLINE_CURVE_WITH_KNOTS('',3,(#140807,#140808,#140809,#140810,
#140811,#140812,#140813,#140814,#140815,#140816,#140817,#140818,#140819,
#140820,#140821,#140822,#140823,#140824,#140825,#140826,#140827,#140828,
#140829,#140830,#140831,#140832,#140833,#140834,#140835,#140836,#140837,
#140838,#140839,#140840,#140841,#140842,#140843,#140844,#140845,#140846,
#140847,#140848,#140849,#140850,#140851,#140852,#140853,#140854,#140855,
#140856,#140857,#140858,#140859,#140860,#140861,#140862,#140863,#140864,
#140865,#140866,#140867,#140868,#140869,#140870,#140871,#140872,#140873,
#140874,#140875,#140876,#140877,#140878,#140879,#140880,#140881,#140882,
#140883,#140884,#140885,#140886,#140887,#140888,#140889,#140890,#140891,
#140892,#140893,#140894,#140895,#140896,#140897,#140898,#140899,#140900,
#140901,#140902,#140903),.UNSPECIFIED.,.F.,.F.,(4,3,3,3,3,3,3,3,3,3,3,3,
3,3,3,3,3,3,3,3,3,3,3,3,3,3,3,3,3,3,3,3,4),(0.,0.0528043674744117,0.101411794382289,
0.1111111111111,0.15644763557432,0.203145303458736,0.216184392620985,0.2222222222222,
0.268327215607274,0.315677403819418,0.331009546931535,0.3333333333333,0.383603126000518,
0.435467618888511,0.4444444444444,0.445827374170425,0.479865806193693,0.514265446278494,
0.548751475142092,0.5555555555556,0.560638706485747,0.604765726042025,0.64872763385938,
0.6666666666667,0.675334559394413,0.731216324970566,0.7777777777778,0.79015606296775,
0.842285728432088,0.8888888888889,0.905015646757144,0.971815255624162,1.),
 .UNSPECIFIED.);
#29817=B_SPLINE_CURVE_WITH_KNOTS('',3,(#140905,#140906,#140907,#140908,
#140909,#140910),.UNSPECIFIED.,.F.,.F.,(4,1,1,4),(2.01511427487787E-6,0.3333333333333,
0.6666666666667,1.),.UNSPECIFIED.);
#29818=B_SPLINE_CURVE_WITH_KNOTS('',3,(#140912,#140913,#140914,#140915,
#140916,#140917,#140918,#140919,#140920,#140921,#140922,#140923,#140924,
#140925,#140926,#140927,#140928,#140929,#140930,#140931,#140932,#140933,
#140934,#140935,#140936,#140937,#140938,#140939,#140940,#140941,#140942,
#140943,#140944,#140945,#140946,#140947,#140948,#140949,#140950,#140951,
#140952,#140953,#140954,#140955,#140956,#140957,#140958,#140959,#140960,
#140961,#140962,#140963),.UNSPECIFIED.,.F.,.F.,(4,3,3,3,3,3,3,3,3,3,3,3,
3,3,3,3,3,4),(2.54841849385267E-8,0.142339474713401,0.1428571428571,0.2857142857143,
0.2872008613377,0.4285714285714,0.432100905493033,0.534601452193607,0.5714285714286,
0.576982678559165,0.664494236306334,0.7142857142857,0.721781321793795,0.836816076392738,
0.8571428571429,0.866672992875378,0.98528256580256,1.),.UNSPECIFIED.);
#29819=B_SPLINE_CURVE_WITH_KNOTS('',3,(#140965,#140966,#140967,#140968,
#140969,#140970,#140971,#140972,#140973,#140974,#140975,#140976,#140977,
#140978,#140979,#140980,#140981,#140982,#140983,#140984,#140985,#140986,
#140987,#140988,#140989,#140990,#140991,#140992,#140993,#140994,#140995,
#140996,#140997,#140998,#140999,#141000,#141001,#141002,#141003,#141004,
#141005,#141006,#141007,#141008,#141009,#141010,#141011,#141012,#141013,
#141014,#141015,#141016,#141017,#141018,#141019,#141020,#141021,#141022,
#141023,#141024,#141025),.UNSPECIFIED.,.F.,.F.,(4,3,3,3,3,3,3,3,3,3,3,3,
3,3,3,3,3,3,3,3,4),(0.,0.0630782732840507,0.127042279284709,0.191683536836724,
0.245591759692709,0.25,0.318849375572925,0.387799611033952,0.456438644994925,
0.5,0.524717413166611,0.577360244871049,0.630453687094251,0.683820373655777,
0.73762295854436,0.75,0.805440391682254,0.860809675952561,0.916874810401688,
0.973450529840081,1.),.UNSPECIFIED.);
#29820=B_SPLINE_CURVE_WITH_KNOTS('',3,(#141030,#141031,#141032,#141033,
#141034,#141035,#141036,#141037,#141038,#141039,#141040,#141041,#141042,
#141043,#141044,#141045,#141046,#141047,#141048,#141049,#141050,#141051,
#141052,#141053),.UNSPECIFIED.,.F.,.F.,(4,2,2,2,1,2,2,2,2,1,2,2,4),(0.,
0.249999999999934,0.374999999999892,0.437499999999875,0.46874999999986,
0.484374999999857,0.499999999999854,0.624999999999859,0.68749999999986,
0.718749999999861,0.734374999999859,0.749999999999857,1.),.UNSPECIFIED.);
#29821=B_SPLINE_CURVE_WITH_KNOTS('',3,(#141097,#141098,#141099,#141100,
#141101,#141102,#141103,#141104,#141105,#141106,#141107,#141108,#141109,
#141110,#141111,#141112,#141113,#141114,#141115,#141116,#141117,#141118,
#141119,#141120,#141121,#141122,#141123,#141124,#141125,#141126,#141127,
#141128,#141129,#141130,#141131,#141132,#141133,#141134,#141135,#141136,
#141137,#141138,#141139,#141140,#141141,#141142,#141143,#141144,#141145,
#141146,#141147,#141148,#141149,#141150,#141151,#141152,#141153,#141154,
#141155,#141156,#141157),.UNSPECIFIED.,.F.,.F.,(4,3,3,3,3,3,3,3,3,3,3,3,
3,3,3,3,3,3,3,3,4),(9.41833711872304E-10,0.0625000007063753,0.121242456281344,
0.179227817213172,0.236342485654817,0.25,0.306333949112938,0.362097082496164,
0.4175941270922,0.472908213704477,0.5,0.555299901063676,0.610886228909014,
0.666693722114869,0.723046964424233,0.75,0.807180637358659,0.865491041455086,
0.924532986353485,0.984817318215386,1.),.UNSPECIFIED.);
#29822=B_SPLINE_CURVE_WITH_KNOTS('',3,(#141158,#141159,#141160,#141161,
#141162,#141163,#141164,#141165,#141166,#141167,#141168,#141169,#141170,
#141171,#141172,#141173,#141174,#141175,#141176,#141177,#141178,#141179,
#141180,#141181,#141182,#141183,#141184,#141185,#141186,#141187,#141188,
#141189,#141190,#141191,#141192,#141193,#141194,#141195,#141196,#141197,
#141198,#141199,#141200,#141201,#141202,#141203,#141204,#141205,#141206,
#141207,#141208,#141209,#141210,#141211,#141212,#141213,#141214,#141215,
#141216,#141217,#141218,#141219,#141220,#141221,#141222,#141223,#141224,
#141225,#141226,#141227,#141228,#141229,#141230,#141231,#141232,#141233,
#141234,#141235,#141236,#141237,#141238,#141239,#141240,#141241,#141242,
#141243,#141244,#141245,#141246,#141247,#141248,#141249,#141250,#141251,
#141252,#141253,#141254,#141255,#141256,#141257,#141258,#141259,#141260,
#141261,#141262,#141263,#141264,#141265,#141266,#141267,#141268,#141269,
#141270,#141271,#141272,#141273,#141274,#141275,#141276,#141277,#141278,
#141279,#141280,#141281,#141282,#141283,#141284,#141285,#141286,#141287,
#141288,#141289,#141290,#141291,#141292,#141293,#141294,#141295,#141296,
#141297,#141298,#141299,#141300,#141301,#141302,#141303,#141304,#141305),
 .UNSPECIFIED.,.F.,.F.,(4,3,3,3,3,3,3,3,3,3,3,3,3,3,3,3,3,3,3,3,3,3,3,3,
3,3,3,3,3,3,3,3,3,3,3,3,3,3,3,3,3,3,3,3,3,3,3,3,3,4),(0.,0.0264084774457084,
0.0540004211451316,0.0624999999999468,0.0915694128606951,0.0937499999999201,
0.109374999999903,0.119184263010084,0.124999999999885,0.145880152879992,
0.177607617245252,0.187499999999834,0.218749999999808,0.234374999999798,
0.24218749999979,0.246093749999782,0.249087826771642,0.249999999999775,
0.293126079918406,0.334757157073219,0.342577256663599,0.386121644454048,
0.427849055909688,0.468749999999184,0.484374999999145,0.492187499999127,
0.496093749999121,0.498046874999117,0.499836436232448,0.499999999999114,
0.531787217869695,0.541498700431291,0.574411422832711,0.606759999982205,
0.63772744515156,0.667782336245535,0.696377557994492,0.718749999999466,
0.726270401674991,0.734374999999495,0.742187499999505,0.746093749999508,
0.748046874999507,0.749999999999506,0.794307853808405,0.839179251836691,
0.884989399471881,0.897490307255218,0.948745153627609,1.),.UNSPECIFIED.);
#29823=B_SPLINE_CURVE_WITH_KNOTS('',3,(#141403,#141404,#141405,#141406,
#141407,#141408,#141409,#141410,#141411,#141412,#141413,#141414,#141415,
#141416,#141417,#141418,#141419,#141420,#141421,#141422,#141423,#141424,
#141425,#141426,#141427,#141428,#141429,#141430,#141431,#141432,#141433,
#141434,#141435,#141436,#141437,#141438,#141439,#141440,#141441,#141442,
#141443,#141444,#141445,#141446,#141447,#141448),.UNSPECIFIED.,.F.,.F.,
(4,3,3,3,3,3,3,3,3,3,3,3,3,3,3,4),(0.,0.0871565653129833,0.124999999999222,
0.187499999998834,0.218749999998644,0.230568207164711,0.234374999998548,
0.242187499998501,0.249023437498464,0.249999999998459,0.374999999998704,
0.437499999998831,0.468749999998894,0.484374999998931,0.499999999998967,
0.999999999995782),.UNSPECIFIED.);
#29824=B_SPLINE_CURVE_WITH_KNOTS('',3,(#141449,#141450,#141451,#141452,
#141453,#141454,#141455,#141456,#141457,#141458,#141459,#141460),
 .UNSPECIFIED.,.F.,.F.,(4,1,1,1,1,1,1,1,1,4),(8.62526419816179E-10,0.129643184459891,
0.259286368919425,0.518572737838491,0.648215922298025,0.777859106757558,
0.842680698987325,0.907502291217091,0.972323883446858,0.999920136454838),
 .UNSPECIFIED.);
#29825=B_SPLINE_CURVE_WITH_KNOTS('',3,(#141462,#141463,#141464,#141465,
#141466,#141467,#141468,#141469,#141470,#141471,#141472,#141473,#141474,
#141475,#141476,#141477),.UNSPECIFIED.,.F.,.F.,(4,3,3,3,3,4),(0.,0.36363630059361,
0.727272601186151,0.818181676334287,0.909090751482421,1.),.UNSPECIFIED.);
#29826=B_SPLINE_CURVE_WITH_KNOTS('',3,(#141479,#141480,#141481,#141482,
#141483,#141484,#141485,#141486,#141487,#141488,#141489),.UNSPECIFIED.,
 .F.,.F.,(4,1,1,1,1,1,1,1,4),(0.,0.0812515846062436,0.265002401744267,0.448753218882289,
0.632504036020311,0.724379444589322,0.816254853158334,0.90813274562238,
1.),.UNSPECIFIED.);
#29827=B_SPLINE_CURVE_WITH_KNOTS('',3,(#141490,#141491,#141492,#141493,
#141494,#141495,#141496,#141497,#141498,#141499,#141500,#141501,#141502,
#141503,#141504,#141505,#141506,#141507,#141508,#141509,#141510,#141511,
#141512,#141513,#141514,#141515,#141516,#141517,#141518,#141519,#141520,
#141521,#141522,#141523,#141524,#141525,#141526,#141527,#141528,#141529,
#141530,#141531,#141532,#141533,#141534,#141535),.UNSPECIFIED.,.F.,.F.,
(4,3,3,3,3,3,3,3,3,3,3,3,3,3,3,4),(0.,0.0570300637188032,0.185099460109903,
0.299971203046531,0.403465598063635,0.497076472649179,0.5,0.581844924036565,
0.658648191461615,0.728294917113762,0.791519404429945,0.848980821447152,
0.901257474787093,0.948894557413619,0.992419572443448,1.),.UNSPECIFIED.);
#29828=B_SPLINE_CURVE_WITH_KNOTS('',3,(#141604,#141605,#141606,#141607,
#141608,#141609,#141610,#141611,#141612,#141613,#141614,#141615,#141616,
#141617,#141618,#141619,#141620,#141621,#141622,#141623,#141624,#141625,
#141626,#141627,#141628,#141629,#141630,#141631,#141632,#141633,#141634,
#141635,#141636,#141637,#141638,#141639,#141640,#141641,#141642,#141643,
#141644,#141645,#141646,#141647,#141648,#141649,#141650,#141651,#141652,
#141653,#141654,#141655,#141656,#141657,#141658,#141659,#141660,#141661,
#141662,#141663,#141664,#141665,#141666,#141667,#141668,#141669,#141670,
#141671,#141672,#141673,#141674,#141675,#141676),.UNSPECIFIED.,.F.,.F.,
(4,3,3,3,3,3,3,3,3,3,3,3,3,3,3,3,3,3,3,3,3,3,3,3,4),(0.,0.0480603990646371,
0.0950212146263362,0.140589379788711,0.185423925913468,0.229341106002203,
0.25,0.292898936761959,0.335299629910999,0.377303576459375,0.419010031839926,
0.460499854771804,0.501925680604814,0.543371999439227,0.584923371415726,
0.626860203634118,0.669047367421796,0.711846231343259,0.75,0.793852299612026,
0.838391808404164,0.884188277214604,0.930765244414424,0.978681703509444,
0.999999999999208),.UNSPECIFIED.);
#29829=B_SPLINE_CURVE_WITH_KNOTS('',3,(#141905,#141906,#141907,#141908,
#141909,#141910,#141911,#141912,#141913,#141914,#141915,#141916,#141917,
#141918,#141919,#141920,#141921,#141922,#141923,#141924,#141925,#141926,
#141927,#141928,#141929,#141930,#141931,#141932,#141933,#141934,#141935,
#141936,#141937,#141938,#141939,#141940,#141941,#141942,#141943,#141944,
#141945,#141946,#141947,#141948,#141949,#141950,#141951,#141952,#141953,
#141954,#141955,#141956,#141957,#141958,#141959,#141960,#141961,#141962,
#141963,#141964,#141965,#141966,#141967,#141968,#141969,#141970,#141971,
#141972,#141973,#141974,#141975,#141976,#141977,#141978,#141979,#141980,
#141981,#141982,#141983,#141984,#141985,#141986,#141987,#141988,#141989,
#141990,#141991,#141992,#141993,#141994,#141995,#141996,#141997,#141998,
#141999,#142000,#142001,#142002,#142003,#142004,#142005,#142006,#142007,
#142008,#142009,#142010,#142011,#142012,#142013,#142014,#142015,#142016,
#142017,#142018,#142019,#142020,#142021,#142022,#142023,#142024,#142025,
#142026,#142027,#142028,#142029,#142030,#142031,#142032,#142033,#142034,
#142035,#142036,#142037,#142038,#142039,#142040,#142041,#142042,#142043,
#142044,#142045,#142046,#142047,#142048,#142049,#142050,#142051,#142052,
#142053,#142054,#142055,#142056,#142057,#142058,#142059,#142060,#142061,
#142062,#142063,#142064,#142065,#142066,#142067,#142068,#142069,#142070,
#142071,#142072,#142073,#142074,#142075,#142076,#142077,#142078,#142079,
#142080,#142081,#142082,#142083,#142084,#142085,#142086,#142087,#142088,
#142089,#142090,#142091,#142092,#142093,#142094,#142095,#142096,#142097,
#142098,#142099,#142100,#142101,#142102,#142103,#142104,#142105,#142106,
#142107,#142108,#142109,#142110,#142111,#142112,#142113,#142114,#142115,
#142116,#142117,#142118,#142119,#142120,#142121,#142122,#142123,#142124,
#142125,#142126,#142127,#142128,#142129,#142130,#142131,#142132,#142133,
#142134,#142135,#142136,#142137,#142138,#142139,#142140,#142141,#142142,
#142143,#142144,#142145,#142146,#142147,#142148,#142149,#142150,#142151,
#142152,#142153,#142154,#142155,#142156,#142157,#142158,#142159,#142160,
#142161,#142162,#142163,#142164,#142165,#142166,#142167,#142168,#142169,
#142170,#142171,#142172,#142173,#142174,#142175,#142176,#142177,#142178,
#142179,#142180,#142181,#142182,#142183,#142184,#142185,#142186,#142187,
#142188,#142189,#142190,#142191,#142192,#142193,#142194,#142195,#142196,
#142197,#142198,#142199,#142200,#142201,#142202,#142203,#142204,#142205,
#142206,#142207,#142208,#142209,#142210,#142211,#142212,#142213,#142214,
#142215,#142216,#142217,#142218,#142219,#142220,#142221,#142222,#142223,
#142224,#142225,#142226,#142227,#142228,#142229,#142230,#142231,#142232,
#142233,#142234,#142235,#142236,#142237,#142238,#142239,#142240,#142241,
#142242,#142243,#142244,#142245,#142246,#142247,#142248,#142249,#142250,
#142251,#142252,#142253,#142254,#142255,#142256,#142257,#142258,#142259,
#142260,#142261,#142262,#142263,#142264,#142265,#142266,#142267,#142268,
#142269,#142270,#142271,#142272,#142273,#142274,#142275,#142276,#142277,
#142278,#142279,#142280,#142281,#142282,#142283,#142284,#142285,#142286,
#142287,#142288,#142289),.UNSPECIFIED.,.F.,.F.,(4,3,3,3,3,3,3,3,3,3,3,3,
3,3,3,3,3,3,3,3,3,3,3,3,3,3,3,3,3,3,3,3,3,3,3,3,3,3,3,3,3,3,3,3,3,3,3,3,
3,3,3,3,3,3,3,3,3,3,3,3,3,3,3,3,3,3,3,3,3,3,3,3,3,3,3,3,3,3,3,3,3,3,3,3,
3,3,3,3,3,3,3,3,3,3,3,3,3,3,3,3,3,3,3,3,3,3,3,3,3,3,3,3,3,3,3,3,3,3,3,3,
3,3,3,3,3,3,3,3,4),(0.,0.00521449698044272,0.0113488205456387,0.0178358694463679,
0.0234650279830911,0.0243229183470971,0.0292986400166019,0.0312499999989362,
0.0382626231936421,0.0497978180709293,0.0564051787566613,0.0618583024771885,
0.0624999999978725,0.0689925129920575,0.0703124999976079,0.0712890624975725,
0.0722656249975372,0.0742187499974694,0.0766934911129652,0.0781249999973303,
0.0820312499971913,0.0839843749971273,0.0857099042925744,0.0859374999970634,
0.0894444052754588,0.0926142549496846,0.0937499999968183,0.0959369608234018,
0.0978509239991937,0.0987752323809756,0.101358853034054,0.101562499996573,
0.103648949249782,0.105468749996451,0.106220025523178,0.106783782019121,
0.107421874996389,0.108664772469553,0.109374999996328,0.110500918498203,
0.110828843478205,0.112253795390214,0.113861390132636,0.115696843465077,
0.11718749999609,0.119800214430568,0.121093749995968,0.123046874995902,
0.124498774121639,0.124999999995837,0.135004728902792,0.140624999995255,
0.145085768584857,0.148437499994964,0.156249999994673,0.164069778087939,
0.187499999993506,0.203124999992923,0.210937499992628,0.212890624992553,
0.214843749992478,0.218749999992334,0.22735411870143,0.234374999991791,
0.242187499991519,0.246093749991382,0.248046874991314,0.249023437491279,
0.249511718741263,0.249755859366256,0.249999999991249,0.269690675432299,
0.281249999991643,0.285156249991687,0.285644531241691,0.286132812491694,
0.287109374991704,0.289062499991721,0.296874999991792,0.306919225954505,
0.312499999991936,0.321016191980661,0.353149448606746,0.374999999992511,
0.432000932161343,0.437499999993086,0.455335442631984,0.468749999993373,
0.484374999993516,0.492187499993586,0.496093749993623,0.498046874993641,
0.499755859368656,0.499999999993659,0.525196633496263,0.542217052572066,
0.563483502376743,0.584129658100889,0.591456271900779,0.611541339049758,
0.624999999995042,0.64356144097782,0.661716660603838,0.679380722824786,
0.687499999995734,0.705132772898844,0.71874999999608,0.730587760228015,
0.734374999996252,0.742187499996338,0.746093749996381,0.748046874996403,
0.749755859371422,0.749999999996425,0.770904489841411,0.782034308694622,
0.802645260226518,0.812499999997319,0.833204988474798,0.847304939070212,
0.865266431846127,0.874999999998213,0.89362961551321,0.913178662494567,
0.919532052425721,0.937499999999106,0.95788376607959,0.979974477596612,
1.),.UNSPECIFIED.);
#29830=B_SPLINE_CURVE_WITH_KNOTS('',3,(#142477,#142478,#142479,#142480,
#142481,#142482,#142483,#142484,#142485,#142486,#142487,#142488,#142489,
#142490,#142491,#142492,#142493),.UNSPECIFIED.,.F.,.F.,(4,1,1,1,1,1,1,1,
1,1,1,1,1,1,4),(0.,0.0171470494701,0.0342940989402,0.04286762367525,0.0514411484103,
0.06001467314535,0.0685881978804,0.0857352473505,0.1028822968206,0.1371763957608,
0.2057645936412,0.2743527915216,0.4115291872824,0.685881978804,1.),
 .UNSPECIFIED.);
#29831=B_SPLINE_CURVE_WITH_KNOTS('',3,(#142681,#142682,#142683,#142684,
#142685,#142686,#142687,#142688,#142689,#142690,#142691),.UNSPECIFIED.,
 .F.,.F.,(4,1,1,1,1,1,1,1,4),(0.,0.0918420543167816,0.183748190378033,0.275623105346068,
0.367498020314102,0.55124785025017,0.734997680186239,0.918747510122307,
1.),.UNSPECIFIED.);
#29832=B_SPLINE_CURVE_WITH_KNOTS('',3,(#142790,#142791,#142792,#142793),
 .UNSPECIFIED.,.F.,.F.,(4,4),(0.,1.),.UNSPECIFIED.);
#29833=B_SPLINE_CURVE_WITH_KNOTS('',3,(#142797,#142798,#142799,#142800,
#142801,#142802,#142803,#142804,#142805,#142806,#142807,#142808,#142809,
#142810,#142811,#142812,#142813,#142814,#142815,#142816,#142817,#142818,
#142819,#142820,#142821,#142822,#142823,#142824,#142825,#142826,#142827,
#142828,#142829,#142830,#142831,#142832,#142833,#142834,#142835,#142836,
#142837,#142838,#142839,#142840,#142841,#142842,#142843,#142844,#142845,
#142846,#142847,#142848,#142849,#142850,#142851,#142852,#142853,#142854,
#142855,#142856,#142857,#142858,#142859,#142860,#142861,#142862,#142863,
#142864,#142865,#142866,#142867,#142868,#142869,#142870,#142871,#142872,
#142873,#142874,#142875,#142876,#142877,#142878,#142879,#142880,#142881,
#142882,#142883,#142884,#142885,#142886,#142887,#142888,#142889,#142890,
#142891,#142892,#142893,#142894,#142895,#142896,#142897,#142898,#142899,
#142900,#142901,#142902,#142903,#142904,#142905,#142906,#142907,#142908,
#142909,#142910,#142911,#142912,#142913,#142914,#142915,#142916,#142917,
#142918,#142919,#142920,#142921,#142922,#142923,#142924,#142925,#142926,
#142927,#142928,#142929,#142930,#142931,#142932,#142933,#142934,#142935,
#142936,#142937,#142938),.UNSPECIFIED.,.F.,.F.,(4,3,3,3,3,3,3,3,3,3,3,3,
3,3,3,3,3,3,3,3,3,3,3,3,3,3,3,3,3,3,3,3,3,3,3,3,3,3,3,3,3,3,3,3,3,3,3,4),
(1.73463430039571E-9,0.0335107622719545,0.0886020995752468,0.143100924356775,
0.196889311633565,0.2500000000009,0.254017552135438,0.302432649453191,0.350353609669106,
0.397676447026696,0.437500000001574,0.437860949912641,0.46875000000169,
0.484375000001741,0.49218750000177,0.496093750001781,0.498914845875728,
0.500000000001793,0.525979626844155,0.552783114604028,0.580825272327736,
0.593673938705637,0.620738510610158,0.649058596437683,0.677973658530814,
0.707468186587495,0.718750000002402,0.734375000002449,0.74218750000248,
0.746093750002493,0.74804687500251,0.749023437502518,0.750000000002527,
0.825232812730111,0.843750000003066,0.859375000003151,0.867187500003194,
0.874023437503235,0.875000000003245,0.891046614145269,0.907083150610724,
0.923049256526572,0.937500000001623,0.953124999998386,0.968447616826583,
0.984223808407629,0.998753350832935,0.999999999988675),.UNSPECIFIED.);
#29834=B_SPLINE_CURVE_WITH_KNOTS('',3,(#142942,#142943,#142944,#142945,
#142946,#142947,#142948,#142949,#142950,#142951,#142952,#142953,#142954,
#142955,#142956,#142957,#142958,#142959,#142960,#142961,#142962,#142963),
 .UNSPECIFIED.,.F.,.F.,(4,3,3,3,3,3,3,4),(8.55806068908103E-11,0.2,0.357842525431517,
0.4,0.6,0.8,0.974718041105161,1.),.UNSPECIFIED.);
#29835=B_SPLINE_CURVE_WITH_KNOTS('',3,(#142967,#142968,#142969,#142970,
#142971,#142972,#142973,#142974,#142975,#142976,#142977,#142978,#142979,
#142980,#142981,#142982,#142983,#142984,#142985,#142986,#142987,#142988,
#142989,#142990,#142991,#142992,#142993,#142994,#142995,#142996,#142997,
#142998,#142999,#143000,#143001,#143002,#143003,#143004,#143005,#143006,
#143007,#143008,#143009,#143010,#143011,#143012,#143013,#143014,#143015,
#143016,#143017,#143018,#143019,#143020,#143021,#143022,#143023,#143024,
#143025,#143026,#143027),.UNSPECIFIED.,.F.,.F.,(4,3,3,3,3,3,3,3,3,3,3,3,
3,3,3,3,3,3,3,3,4),(2.95674022625425E-11,0.0590835197265977,0.0644729979353127,
0.123579051781818,0.184080539447088,0.2,0.281365249285575,0.299014851252803,
0.381024531865931,0.4,0.503697847279184,0.5318585389134,0.6,0.677481482895928,
0.757900617461102,0.764520989067543,0.8,0.866123989598734,0.931596831446147,
0.99706967329356,1.),.UNSPECIFIED.);
#29836=B_SPLINE_CURVE_WITH_KNOTS('',3,(#143056,#143057,#143058,#143059,
#143060,#143061,#143062,#143063,#143064,#143065,#143066,#143067,#143068),
 .UNSPECIFIED.,.F.,.F.,(4,3,3,3,4),(0.,0.258977222641322,0.520864720696312,
0.787686771689713,1.),.UNSPECIFIED.);
#29837=B_SPLINE_CURVE_WITH_KNOTS('',3,(#143111,#143112,#143113,#143114,
#143115,#143116,#143117,#143118,#143119,#143120,#143121,#143122,#143123,
#143124,#143125,#143126,#143127,#143128,#143129,#143130,#143131,#143132,
#143133,#143134,#143135,#143136,#143137,#143138,#143139,#143140,#143141,
#143142,#143143,#143144,#143145,#143146,#143147,#143148,#143149,#143150,
#143151,#143152,#143153,#143154,#143155,#143156,#143157,#143158,#143159,
#143160,#143161,#143162,#143163,#143164,#143165,#143166,#143167,#143168,
#143169,#143170,#143171,#143172,#143173,#143174,#143175,#143176,#143177),
 .UNSPECIFIED.,.F.,.F.,(4,3,3,3,3,3,3,3,3,3,3,3,3,3,3,3,3,3,3,3,3,3,4),
(0.,0.08027036975129,0.15868466085864,0.23464894294463,0.250000000000064,
0.323297303695469,0.394307113162551,0.437500000000121,0.468750000000125,
0.484375000000122,0.49218750000012,0.497768800090433,0.500000000000119,
0.551027785102183,0.604025486376891,0.65818398549835,0.714271007151812,
0.750000000000059,0.808455080078342,0.869171922711029,0.931152591310257,
0.994693264380135,1.),.UNSPECIFIED.);
#29838=B_SPLINE_CURVE_WITH_KNOTS('',3,(#143178,#143179,#143180,#143181,
#143182,#143183,#143184,#143185,#143186,#143187,#143188,#143189,#143190,
#143191,#143192,#143193,#143194,#143195,#143196,#143197,#143198,#143199,
#143200,#143201,#143202,#143203,#143204,#143205,#143206,#143207,#143208,
#143209,#143210,#143211,#143212,#143213,#143214,#143215,#143216,#143217,
#143218,#143219,#143220,#143221,#143222,#143223,#143224,#143225,#143226,
#143227,#143228,#143229,#143230,#143231,#143232,#143233,#143234,#143235,
#143236,#143237,#143238),.UNSPECIFIED.,.F.,.F.,(4,3,3,3,3,3,3,3,3,3,3,3,
3,3,3,3,3,3,3,3,4),(0.,0.0500140916140122,0.102810472433336,0.157768197269118,
0.218317721152486,0.25,0.305665021786033,0.364108822971698,0.424270070064475,
0.486191448667807,0.5,0.5625,0.622367801824673,0.680496857852398,0.736297030446486,
0.75,0.8125,0.867577176507066,0.920267714681305,0.970593913147975,1.),
 .UNSPECIFIED.);
#29839=B_SPLINE_CURVE_WITH_KNOTS('',3,(#143241,#143242,#143243,#143244,
#143245,#143246,#143247,#143248,#143249,#143250),.UNSPECIFIED.,.F.,.F.,
(4,2,2,2,4),(0.,0.25,0.5,0.75,0.999999989319756),.UNSPECIFIED.);
#29840=B_SPLINE_CURVE_WITH_KNOTS('',3,(#143252,#143253,#143254,#143255),
 .UNSPECIFIED.,.F.,.F.,(4,4),(0.,0.999980732155484),.UNSPECIFIED.);
#29841=B_SPLINE_CURVE_WITH_KNOTS('',3,(#143257,#143258,#143259,#143260),
 .UNSPECIFIED.,.F.,.F.,(4,4),(0.,1.),.UNSPECIFIED.);
#29842=B_SPLINE_CURVE_WITH_KNOTS('',3,(#143264,#143265,#143266,#143267,
#143268,#143269,#143270,#143271,#143272,#143273,#143274,#143275,#143276,
#143277,#143278,#143279,#143280,#143281,#143282,#143283,#143284,#143285,
#143286,#143287,#143288,#143289,#143290,#143291,#143292,#143293,#143294,
#143295,#143296,#143297,#143298,#143299,#143300),.UNSPECIFIED.,.F.,.F.,
(4,3,3,3,3,3,3,3,3,3,3,3,4),(2.99246483692683E-10,0.0840858906723014,0.168136003243227,
0.252183926484771,0.336208591087671,0.420255785707517,0.5,0.584777283150557,
0.669548215185025,0.75434071751584,0.839117300724285,0.923908041707433,
1.),.UNSPECIFIED.);
#29843=B_SPLINE_CURVE_WITH_KNOTS('',3,(#143303,#143304,#143305,#143306,
#143307,#143308),.UNSPECIFIED.,.F.,.F.,(4,2,4),(0.,0.5,0.999484898490112),
 .UNSPECIFIED.);
#29844=B_SPLINE_CURVE_WITH_KNOTS('',3,(#143354,#143355,#143356,#143357,
#143358,#143359,#143360,#143361,#143362,#143363,#143364,#143365,#143366,
#143367,#143368,#143369,#143370,#143371,#143372,#143373,#143374,#143375,
#143376,#143377,#143378,#143379,#143380,#143381,#143382,#143383,#143384,
#143385,#143386,#143387,#143388,#143389,#143390,#143391,#143392,#143393,
#143394,#143395,#143396,#143397,#143398,#143399,#143400,#143401,#143402,
#143403,#143404,#143405,#143406,#143407,#143408,#143409,#143410,#143411,
#143412,#143413,#143414,#143415,#143416,#143417,#143418,#143419,#143420,
#143421,#143422,#143423,#143424,#143425,#143426,#143427,#143428,#143429),
 .UNSPECIFIED.,.F.,.F.,(4,3,3,3,3,3,3,3,3,3,3,3,3,3,3,3,3,3,3,3,3,3,3,3,
3,4),(1.88018170531242E-9,0.0645057624885224,0.127700538116555,0.188893270247744,
0.250000000000156,0.30857082095324,0.366124740049286,0.422323360922472,
0.437500000000273,0.468750000000288,0.484375000000291,0.492187500000292,
0.496930650753609,0.500000000000293,0.538964511246705,0.578808443724839,
0.621606332793664,0.663892028395619,0.707754775287589,0.750000000000138,
0.796133698674557,0.843505573269289,0.892672648356596,0.942812405953015,
0.994119325581967,0.99999999896473),.UNSPECIFIED.);
#29845=B_SPLINE_CURVE_WITH_KNOTS('',3,(#143430,#143431,#143432,#143433,
#143434,#143435,#143436,#143437,#143438,#143439,#143440,#143441,#143442,
#143443,#143444,#143445,#143446,#143447,#143448,#143449,#143450,#143451,
#143452,#143453,#143454,#143455,#143456,#143457,#143458,#143459,#143460,
#143461,#143462,#143463,#143464,#143465,#143466,#143467,#143468,#143469,
#143470,#143471,#143472,#143473,#143474,#143475,#143476,#143477,#143478),
 .UNSPECIFIED.,.F.,.F.,(4,3,3,3,3,3,3,3,3,3,3,3,3,3,3,3,4),(1.15239154642677E-10,
0.0649165563113629,0.132403698407869,0.206726934240605,0.25,0.320782786022654,
0.393717759036282,0.469211508163737,0.5,0.575238128201483,0.648757748742531,
0.719054838158213,0.75,0.82388280728322,0.892741770995936,0.95719031445221,
1.),.UNSPECIFIED.);
#29846=B_SPLINE_CURVE_WITH_KNOTS('',3,(#143524,#143525,#143526,#143527,
#143528,#143529,#143530,#143531,#143532,#143533,#143534,#143535,#143536,
#143537,#143538,#143539,#143540,#143541,#143542,#143543,#143544,#143545,
#143546,#143547,#143548,#143549,#143550,#143551,#143552,#143553,#143554,
#143555,#143556,#143557,#143558,#143559,#143560,#143561,#143562,#143563,
#143564,#143565,#143566,#143567,#143568,#143569,#143570,#143571,#143572,
#143573,#143574,#143575,#143576,#143577,#143578,#143579,#143580,#143581),
 .UNSPECIFIED.,.F.,.F.,(4,3,3,3,3,3,3,3,3,3,3,3,3,3,3,3,3,3,3,4),(0.,0.0591362138677374,
0.120878268797879,0.18543913439894,0.25,0.267238582825178,0.329519130380692,
0.392905904843487,0.458231542232862,0.490447831179993,0.5,0.5658716799357,
0.633420574512136,0.703676255632175,0.732777413191121,0.75,0.821897558034854,
0.895738132611241,0.972481734941369,0.999925149981118),.UNSPECIFIED.);
#29847=B_SPLINE_CURVE_WITH_KNOTS('',3,(#143623,#143624,#143625,#143626,
#143627,#143628,#143629,#143630,#143631,#143632,#143633,#143634,#143635,
#143636,#143637,#143638,#143639,#143640,#143641),.UNSPECIFIED.,.F.,.F.,
(4,2,2,2,1,1,1,2,2,2,4),(0.,0.249999999999776,0.374999999999666,0.437499999999608,
0.468749999999578,0.484374999999568,0.49218749999957,0.496093749999578,
0.499999999999585,0.749999999999793,0.999999787290037),.UNSPECIFIED.);
#29848=B_SPLINE_CURVE_WITH_KNOTS('',3,(#143642,#143643,#143644,#143645,
#143646,#143647),.UNSPECIFIED.,.F.,.F.,(4,2,4),(0.,0.5,0.99999995988345),
 .UNSPECIFIED.);
#29849=B_SPLINE_CURVE_WITH_KNOTS('',3,(#143649,#143650,#143651,#143652,
#143653,#143654),.UNSPECIFIED.,.F.,.F.,(4,2,4),(0.,0.5,1.),
 .UNSPECIFIED.);
#29850=B_SPLINE_CURVE_WITH_KNOTS('',3,(#143690,#143691,#143692,#143693,
#143694,#143695,#143696,#143697,#143698,#143699,#143700,#143701,#143702,
#143703,#143704,#143705,#143706,#143707,#143708),.UNSPECIFIED.,.F.,.F.,
(4,2,2,2,1,1,1,2,2,2,4),(3.26475431587078E-8,0.249999999999144,0.374999999998711,
0.437499999998487,0.468749999998368,0.484374999998299,0.492187499998282,
0.496093749998283,0.499999999998285,0.749999999999143,0.999999893028112),
 .UNSPECIFIED.);
#29851=B_SPLINE_CURVE_WITH_KNOTS('',3,(#143792,#143793,#143794,#143795,
#143796,#143797,#143798,#143799,#143800,#143801,#143802,#143803,#143804,
#143805,#143806,#143807,#143808,#143809,#143810,#143811,#143812,#143813,
#143814,#143815,#143816,#143817,#143818,#143819,#143820,#143821,#143822,
#143823,#143824,#143825,#143826,#143827,#143828,#143829,#143830,#143831,
#143832,#143833,#143834,#143835,#143836,#143837,#143838,#143839,#143840,
#143841,#143842,#143843,#143844,#143845,#143846,#143847,#143848,#143849),
 .UNSPECIFIED.,.F.,.F.,(4,3,3,3,3,3,3,3,3,3,3,3,3,3,3,3,3,3,3,4),(7.4513935169651E-5,
0.0764390166688387,0.15077462552214,0.222227128795632,0.25,0.267224468266891,
0.337159446103622,0.405216324088469,0.47073909310234,0.5,0.509557862772661,
0.574682549819007,0.63847798460608,0.700563150132604,0.732763275912864,
0.75,0.812223755461616,0.876545948829822,0.940868142198028,1.),
 .UNSPECIFIED.);
#29852=B_SPLINE_CURVE_WITH_KNOTS('',3,(#143896,#143897,#143898,#143899,
#143900,#143901,#143902,#143903,#143904,#143905,#143906,#143907,#143908,
#143909,#143910,#143911,#143912,#143913,#143914,#143915,#143916,#143917,
#143918,#143919,#143920,#143921,#143922,#143923,#143924,#143925,#143926,
#143927,#143928,#143929,#143930,#143931,#143932,#143933,#143934,#143935,
#143936,#143937,#143938,#143939,#143940,#143941,#143942,#143943,#143944,
#143945,#143946,#143947,#143948,#143949,#143950,#143951,#143952,#143953,
#143954,#143955,#143956,#143957,#143958,#143959,#143960,#143961,#143962,
#143963,#143964,#143965,#143966,#143967,#143968),.UNSPECIFIED.,.F.,.F.,
(4,3,3,3,3,3,3,3,3,3,3,3,3,3,3,3,3,3,3,3,3,3,3,3,4),(0.,0.0533424467156048,
0.104743634528447,0.154982248749812,0.203334709437968,0.250000000000053,
0.296875000000063,0.341353352128222,0.384893437136361,0.427201223511014,
0.437500000000092,0.468750000000099,0.484375000000094,0.49218750000009,
0.496935227016766,0.500000000000086,0.556761117887998,0.615044467063844,
0.674247131807778,0.7348358278879,0.750000000000043,0.812906270780981,0.876937510189453,
0.942948224179702,1.),.UNSPECIFIED.);
#29853=B_SPLINE_CURVE_WITH_KNOTS('',3,(#143976,#143977,#143978,#143979,
#143980,#143981,#143982,#143983),.UNSPECIFIED.,.F.,.F.,(4,1,1,1,1,4),(1.14974297182232E-6,
0.199999999999993,0.399999999999986,0.599999999999979,0.799999999999972,
0.999999999999965),.UNSPECIFIED.);
#29854=B_SPLINE_CURVE_WITH_KNOTS('',3,(#143985,#143986,#143987,#143988,
#143989,#143990),.UNSPECIFIED.,.F.,.F.,(4,2,4),(0.,0.5,0.999787114378974),
 .UNSPECIFIED.);
#29855=B_SPLINE_CURVE_WITH_KNOTS('',3,(#143994,#143995,#143996,#143997),
 .UNSPECIFIED.,.F.,.F.,(4,4),(1.81327895980828E-5,1.),.UNSPECIFIED.);
#29856=B_SPLINE_CURVE_WITH_KNOTS('',3,(#143998,#143999,#144000,#144001),
 .UNSPECIFIED.,.F.,.F.,(4,4),(0.,1.),.UNSPECIFIED.);
#29857=B_SPLINE_CURVE_WITH_KNOTS('',3,(#144005,#144006,#144007,#144008,
#144009,#144010),.UNSPECIFIED.,.F.,.F.,(4,2,4),(5.64578029880314E-9,0.5,
0.999999996578219),.UNSPECIFIED.);
#29858=B_SPLINE_CURVE_WITH_KNOTS('',3,(#144012,#144013,#144014,#144015),
 .UNSPECIFIED.,.F.,.F.,(4,4),(0.,0.999999846333988),.UNSPECIFIED.);
#29859=B_SPLINE_CURVE_WITH_KNOTS('',3,(#144016,#144017,#144018,#144019),
 .UNSPECIFIED.,.F.,.F.,(4,4),(0.,1.),.UNSPECIFIED.);
#29860=B_SPLINE_CURVE_WITH_KNOTS('',3,(#144022,#144023,#144024,#144025,
#144026,#144027),.UNSPECIFIED.,.F.,.F.,(4,2,4),(0.,0.5,0.999999995317697),
 .UNSPECIFIED.);
#29861=B_SPLINE_CURVE_WITH_KNOTS('',3,(#144057,#144058,#144059,#144060,
#144061,#144062,#144063,#144064,#144065,#144066,#144067,#144068,#144069,
#144070,#144071,#144072,#144073,#144074,#144075,#144076,#144077,#144078),
 .UNSPECIFIED.,.F.,.F.,(4,3,3,3,3,3,3,4),(0.,0.234589466263676,0.25,0.467093428636511,
0.500000000000001,0.677237910839018,0.868423764703068,1.),.UNSPECIFIED.);
#29862=B_SPLINE_CURVE_WITH_KNOTS('',3,(#144097,#144098,#144099,#144100,
#144101,#144102,#144103,#144104,#144105,#144106,#144107,#144108,#144109,
#144110,#144111,#144112,#144113,#144114,#144115,#144116,#144117,#144118,
#144119,#144120,#144121),.UNSPECIFIED.,.F.,.F.,(4,3,3,3,3,3,3,3,4),(0.,
0.151395870213908,0.303640552398499,0.356919349785617,0.5,0.653533854511357,
0.807219568466739,0.960969667135148,1.),.UNSPECIFIED.);
#29863=B_SPLINE_CURVE_WITH_KNOTS('',3,(#144123,#144124,#144125,#144126,
#144127,#144128,#144129,#144130,#144131,#144132,#144133,#144134,#144135,
#144136,#144137,#144138,#144139,#144140,#144141),.UNSPECIFIED.,.F.,.F.,
(4,3,3,3,3,3,4),(7.3073587088353E-11,0.191104891355974,0.310139280686363,
0.5,0.678403737752968,0.853738983746465,0.999999999299965),
 .UNSPECIFIED.);
#29864=B_SPLINE_CURVE_WITH_KNOTS('',3,(#144160,#144161,#144162,#144163,
#144164,#144165,#144166,#144167,#144168,#144169,#144170,#144171,#144172),
 .UNSPECIFIED.,.F.,.F.,(4,2,2,1,2,2,4),(0.,0.249999999999996,0.374999999999994,
0.437499999999994,0.468749999999993,0.499999999999993,1.),.UNSPECIFIED.);
#29865=B_SPLINE_CURVE_WITH_KNOTS('',3,(#144174,#144175,#144176,#144177,
#144178,#144179,#144180,#144181,#144182,#144183,#144184,#144185,#144186,
#144187,#144188,#144189,#144190,#144191,#144192),.UNSPECIFIED.,.F.,.F.,
(4,3,3,3,3,3,4),(0.,0.175269520094249,0.326885779417009,0.5,0.695471343358672,
0.886047081605195,1.),.UNSPECIFIED.);
#29866=B_SPLINE_CURVE_WITH_KNOTS('',3,(#144211,#144212,#144213,#144214,
#144215,#144216,#144217,#144218,#144219,#144220,#144221,#144222,#144223,
#144224,#144225,#144226,#144227,#144228,#144229,#144230,#144231,#144232,
#144233,#144234,#144235,#144236,#144237,#144238,#144239,#144240,#144241,
#144242,#144243,#144244,#144245,#144246,#144247,#144248,#144249,#144250,
#144251,#144252,#144253,#144254,#144255,#144256,#144257,#144258,#144259,
#144260,#144261,#144262,#144263,#144264,#144265,#144266,#144267,#144268,
#144269,#144270,#144271,#144272,#144273,#144274,#144275,#144276,#144277,
#144278,#144279,#144280,#144281,#144282,#144283,#144284,#144285,#144286),
 .UNSPECIFIED.,.F.,.F.,(4,3,3,3,3,3,3,3,3,3,3,3,3,3,3,3,3,3,3,3,3,3,3,3,
3,4),(0.,0.0540181594619873,0.107259627625218,0.160152504466205,0.2125889741831,
0.250000000000005,0.297638439728598,0.344247373429098,0.375000000000007,
0.418390387038428,0.437500000000008,0.468750000000008,0.484375000000008,
0.492187500000008,0.498508254699402,0.500000000000007,0.549786412774844,
0.600525719911558,0.651666776290185,0.703442746339702,0.750000000000004,
0.802143792479376,0.856713325005992,0.912968224892903,0.972431465331863,
1.),.UNSPECIFIED.);
#29867=B_SPLINE_CURVE_WITH_KNOTS('',3,(#144287,#144288,#144289,#144290,
#144291,#144292,#144293,#144294,#144295,#144296,#144297,#144298,#144299,
#144300,#144301,#144302,#144303,#144304,#144305,#144306,#144307,#144308,
#144309,#144310,#144311,#144312,#144313,#144314,#144315,#144316,#144317,
#144318,#144319,#144320,#144321,#144322,#144323),.UNSPECIFIED.,.F.,.F.,
(4,3,3,3,3,3,3,3,3,3,3,3,4),(2.58573610941644E-9,0.0877143487115733,0.177079072050148,
0.268548046153447,0.360941000981022,0.45425873055312,0.5,0.5960451564699,
0.691319690101686,0.784873547168815,0.877122526712708,0.967109401539248,
0.999999999999998),.UNSPECIFIED.);
#29868=B_SPLINE_CURVE_WITH_KNOTS('',3,(#144327,#144328,#144329,#144330),
 .UNSPECIFIED.,.F.,.F.,(4,4),(4.0356730508919E-7,1.),.UNSPECIFIED.);
#29869=B_SPLINE_CURVE_WITH_KNOTS('',3,(#144332,#144333,#144334,#144335),
 .UNSPECIFIED.,.F.,.F.,(4,4),(0.,1.),.UNSPECIFIED.);
#29870=B_SPLINE_CURVE_WITH_KNOTS('',3,(#144336,#144337,#144338,#144339,
#144340,#144341),.UNSPECIFIED.,.F.,.F.,(4,2,4),(2.43156888848096E-9,0.5,
0.999999884413479),.UNSPECIFIED.);
#29871=B_SPLINE_CURVE_WITH_KNOTS('',3,(#144375,#144376,#144377,#144378),
 .UNSPECIFIED.,.F.,.F.,(4,4),(0.,1.),.UNSPECIFIED.);
#29872=B_SPLINE_CURVE_WITH_KNOTS('',3,(#144379,#144380,#144381,#144382,
#144383,#144384,#144385,#144386,#144387,#144388,#144389,#144390,#144391,
#144392,#144393,#144394,#144395,#144396,#144397,#144398,#144399,#144400,
#144401,#144402,#144403,#144404,#144405,#144406,#144407,#144408,#144409,
#144410,#144411,#144412,#144413,#144414,#144415,#144416,#144417,#144418,
#144419,#144420,#144421,#144422,#144423,#144424,#144425,#144426,#144427,
#144428,#144429,#144430),.UNSPECIFIED.,.F.,.F.,(4,3,3,3,3,3,3,3,3,3,3,3,
3,3,3,3,3,4),(0.,0.0957981934517183,0.15219996804128,0.252309664578997,
0.298257045469927,0.395284374327465,0.423903020998006,0.514444308082931,
0.534757075323245,0.617053500050071,0.634002062399949,0.726315695614125,
0.734247069000456,0.75,0.833172583328939,0.917077637468813,0.92726894121381,
0.999999840603065),.UNSPECIFIED.);
#29873=B_SPLINE_CURVE_WITH_KNOTS('',3,(#144547,#144548,#144549,#144550,
#144551,#144552,#144553,#144554,#144555,#144556,#144557,#144558,#144559,
#144560,#144561,#144562,#144563,#144564,#144565,#144566,#144567,#144568,
#144569,#144570,#144571,#144572,#144573,#144574,#144575,#144576,#144577,
#144578,#144579,#144580,#144581,#144582,#144583,#144584,#144585,#144586,
#144587,#144588,#144589,#144590,#144591,#144592,#144593,#144594,#144595,
#144596,#144597,#144598,#144599,#144600,#144601,#144602,#144603,#144604,
#144605,#144606,#144607),.UNSPECIFIED.,.F.,.F.,(4,3,3,3,3,3,3,3,3,3,3,3,
3,3,3,3,3,3,3,3,4),(0.,0.0425624458950865,0.116206183539185,0.192860166407389,
0.250000000000012,0.27276457930784,0.356076441493708,0.437500000000022,
0.442882711310174,0.468750000000024,0.484375000000025,0.492187500000025,
0.499023437500025,0.500000000000025,0.522730186331662,0.588945716513302,
0.660745283754589,0.73803325288249,0.821793505481187,0.913325820897002,
1.),.UNSPECIFIED.);
#29874=B_SPLINE_CURVE_WITH_KNOTS('',3,(#144662,#144663,#144664,#144665),
 .UNSPECIFIED.,.F.,.F.,(4,4),(2.76646221668592E-8,0.999999999601257),
 .UNSPECIFIED.);
#29875=B_SPLINE_CURVE_WITH_KNOTS('',3,(#144683,#144684,#144685,#144686),
 .UNSPECIFIED.,.F.,.F.,(4,4),(0.,1.),.UNSPECIFIED.);
#29876=B_SPLINE_CURVE_WITH_KNOTS('',3,(#144687,#144688,#144689,#144690,
#144691,#144692,#144693,#144694,#144695,#144696),.UNSPECIFIED.,.F.,.F.,
(4,3,3,4),(0.,0.320682330949903,0.721806394077566,0.999999187310508),
 .UNSPECIFIED.);
#29877=B_SPLINE_CURVE_WITH_KNOTS('',3,(#144774,#144775,#144776,#144777,
#144778,#144779,#144780,#144781,#144782,#144783,#144784,#144785,#144786,
#144787,#144788,#144789,#144790,#144791,#144792,#144793,#144794,#144795,
#144796,#144797,#144798,#144799,#144800,#144801,#144802,#144803,#144804,
#144805,#144806,#144807,#144808,#144809,#144810,#144811,#144812,#144813),
 .UNSPECIFIED.,.F.,.F.,(4,3,3,3,3,3,3,3,3,3,3,3,3,4),(0.,0.0869925140249388,
0.176057719812484,0.227923063318706,0.25,0.347107344576692,0.373508987913521,
0.457206582786402,0.525564563146908,0.621947310577417,0.687900209279146,
0.75,0.856805504898761,1.),.UNSPECIFIED.);
#29878=B_SPLINE_CURVE_WITH_KNOTS('',3,(#144874,#144875,#144876,#144877,
#144878,#144879,#144880,#144881,#144882,#144883,#144884,#144885,#144886,
#144887,#144888,#144889,#144890,#144891,#144892),.UNSPECIFIED.,.F.,.F.,
(4,3,3,3,3,3,4),(0.,0.249999996790803,0.443916949821269,0.622856224213297,
0.793090569014283,0.95621014018365,0.99999998716321),.UNSPECIFIED.);
#29879=B_SPLINE_CURVE_WITH_KNOTS('',3,(#144951,#144952,#144953,#144954,
#144955,#144956,#144957,#144958,#144959,#144960,#144961,#144962,#144963,
#144964,#144965,#144966,#144967,#144968,#144969,#144970,#144971,#144972,
#144973,#144974,#144975,#144976,#144977,#144978,#144979,#144980,#144981,
#144982,#144983,#144984,#144985,#144986,#144987,#144988,#144989,#144990,
#144991,#144992,#144993,#144994,#144995,#144996,#144997,#144998,#144999,
#145000,#145001,#145002,#145003,#145004,#145005,#145006,#145007,#145008,
#145009,#145010,#145011,#145012,#145013,#145014),.UNSPECIFIED.,.F.,.F.,
(4,3,3,3,3,3,3,3,3,3,3,3,3,3,3,3,3,3,3,3,3,4),(0.,0.0515115307653243,0.101465397062888,
0.150637075398089,0.200318537699045,0.25,0.29693317301872,0.343393495909613,
0.389491202373321,0.435297728742739,0.481002063614683,0.526697487832872,
0.572477227545014,0.618626393499786,0.665023537321272,0.712032314967765,
0.75,0.798017220119162,0.848512915089372,0.898501582141251,0.94994422338954,
1.),.UNSPECIFIED.);
#29880=B_SPLINE_CURVE_WITH_KNOTS('',3,(#145015,#145016,#145017,#145018,
#145019,#145020,#145021,#145022,#145023,#145024,#145025,#145026,#145027,
#145028,#145029,#145030,#145031,#145032,#145033,#145034,#145035,#145036,
#145037,#145038,#145039,#145040,#145041,#145042,#145043,#145044,#145045,
#145046,#145047,#145048,#145049,#145050,#145051,#145052,#145053,#145054,
#145055,#145056,#145057,#145058,#145059,#145060,#145061,#145062,#145063,
#145064,#145065,#145066),.UNSPECIFIED.,.F.,.F.,(4,3,3,3,3,3,3,3,3,3,3,3,
3,3,3,3,3,4),(0.,0.125000000000006,0.250000000000012,0.280520976309935,
0.375000000000025,0.437500000000022,0.468750000000023,0.491716905195655,
0.500000000000025,0.558110951675689,0.585560299651521,0.65132272256481,
0.7199614534636,0.750000000000013,0.810121111210684,0.882590846461046,0.941450522833902,
0.999999999705399),.UNSPECIFIED.);
#29881=B_SPLINE_CURVE_WITH_KNOTS('',3,(#145095,#145096,#145097,#145098),
 .UNSPECIFIED.,.F.,.F.,(4,4),(1.29351143961801E-10,1.),.UNSPECIFIED.);
#29882=B_SPLINE_CURVE_WITH_KNOTS('',3,(#145099,#145100,#145101,#145102,
#145103,#145104,#145105),.UNSPECIFIED.,.F.,.F.,(4,3,4),(0.,0.677804750977032,
1.),.UNSPECIFIED.);
#29883=B_SPLINE_CURVE_WITH_KNOTS('',3,(#145132,#145133,#145134,#145135,
#145136,#145137,#145138,#145139,#145140,#145141,#145142,#145143,#145144,
#145145,#145146,#145147,#145148,#145149,#145150,#145151,#145152,#145153,
#145154,#145155,#145156,#145157,#145158,#145159,#145160,#145161,#145162,
#145163,#145164,#145165,#145166,#145167,#145168,#145169,#145170,#145171,
#145172,#145173,#145174,#145175,#145176,#145177,#145178,#145179,#145180,
#145181,#145182,#145183,#145184,#145185,#145186,#145187,#145188,#145189),
 .UNSPECIFIED.,.F.,.F.,(4,3,3,3,3,3,3,3,3,3,3,3,3,3,3,3,3,3,3,4),(0.,0.0737543241068619,
0.145149085023866,0.213031250709547,0.25,0.31502001785785,0.376605523383129,
0.421989433543571,0.491109534182326,0.5,0.565784535589313,0.630017581033254,
0.692094840029708,0.74989259282035,0.75,0.807003071333124,0.861841800614466,
0.915723256400594,0.968482946301467,1.),.UNSPECIFIED.);
#29884=B_SPLINE_CURVE_WITH_KNOTS('',3,(#145257,#145258,#145259,#145260,
#145261,#145262,#145263,#145264,#145265,#145266,#145267,#145268,#145269,
#145270,#145271,#145272,#145273,#145274,#145275,#145276,#145277,#145278,
#145279,#145280,#145281,#145282,#145283,#145284,#145285,#145286,#145287,
#145288,#145289,#145290,#145291,#145292,#145293),.UNSPECIFIED.,.F.,.F.,
(4,3,3,3,3,3,3,3,3,3,3,3,4),(3.50891768936283E-5,0.0843180394326553,0.168576167404038,
0.252840967918579,0.337085284669226,0.421349077367453,0.5,0.584702371040028,
0.669398412098734,0.754116061274742,0.838817762323477,0.923533655731094,
1.),.UNSPECIFIED.);
#29885=B_SPLINE_CURVE_WITH_KNOTS('',3,(#145297,#145298,#145299,#145300,
#145301,#145302,#145303),.UNSPECIFIED.,.F.,.F.,(4,1,1,1,4),(0.,0.25,0.5,
0.75,1.),.UNSPECIFIED.);
#29886=B_SPLINE_CURVE_WITH_KNOTS('',3,(#145305,#145306,#145307,#145308,
#145309,#145310,#145311,#145312,#145313,#145314,#145315,#145316,#145317,
#145318,#145319,#145320,#145321,#145322,#145323,#145324,#145325,#145326,
#145327,#145328,#145329,#145330,#145331,#145332),.UNSPECIFIED.,.F.,.F.,
(4,3,3,3,3,3,3,3,3,4),(0.,0.160240490642099,0.320480981284198,0.3333333333333,
0.46964884726713,0.60577008378555,0.6666666666667,0.691528796069726,0.919246361875947,
1.),.UNSPECIFIED.);
#29887=B_SPLINE_CURVE_WITH_KNOTS('',3,(#145334,#145335,#145336,#145337,
#145338,#145339,#145340,#145341,#145342,#145343,#145344,#145345,#145346,
#145347,#145348,#145349,#145350,#145351,#145352,#145353,#145354,#145355,
#145356,#145357,#145358,#145359,#145360,#145361),.UNSPECIFIED.,.F.,.F.,
(4,3,3,3,3,3,3,3,3,4),(0.,0.223462991617817,0.313827993255978,0.3333333333333,
0.467162238544904,0.601309120325676,0.6666666666667,0.684616796514498,0.8431885857511,
1.),.UNSPECIFIED.);
#29888=B_SPLINE_CURVE_WITH_KNOTS('',3,(#145363,#145364,#145365,#145366,
#145367,#145368,#145369,#145370,#145371,#145372,#145373,#145374,#145375,
#145376,#145377,#145378,#145379,#145380,#145381,#145382,#145383,#145384,
#145385,#145386,#145387,#145388,#145389,#145390,#145391,#145392,#145393,
#145394,#145395),.UNSPECIFIED.,.F.,.F.,(4,1,2,2,2,2,2,2,2,2,2,2,2,2,2,2,
4),(0.,0.0312500000000643,0.0546875000001129,0.0625000000001292,0.109375000000229,
0.125000000000262,0.246093750000515,0.250000000000523,0.373046875000797,
0.375000000000802,0.499023437501035,0.500000000001037,0.624023437500881,
0.62500000000088,0.746093750000591,0.750000000000581,1.),.UNSPECIFIED.);
#29889=B_SPLINE_CURVE_WITH_KNOTS('',3,(#145417,#145418,#145419,#145420,
#145421,#145422,#145423,#145424,#145425,#145426,#145427,#145428,#145429,
#145430,#145431,#145432,#145433,#145434,#145435,#145436,#145437,#145438,
#145439,#145440,#145441,#145442,#145443,#145444,#145445,#145446,#145447,
#145448,#145449,#145450,#145451,#145452,#145453,#145454,#145455,#145456,
#145457,#145458,#145459,#145460,#145461,#145462,#145463,#145464,#145465,
#145466,#145467,#145468,#145469,#145470,#145471,#145472,#145473,#145474,
#145475,#145476,#145477,#145478,#145479,#145480,#145481,#145482,#145483,
#145484,#145485,#145486,#145487,#145488,#145489,#145490,#145491,#145492,
#145493,#145494,#145495,#145496,#145497,#145498),.UNSPECIFIED.,.F.,.F.,
(4,3,3,3,3,3,3,3,3,3,3,3,3,3,3,3,3,3,3,3,3,3,3,3,3,3,3,4),(0.,0.0588671038353967,
0.115769444603005,0.171765650658291,0.226748779862293,0.250000000000507,
0.312500000000632,0.320312500000644,0.326103898030806,0.328125000000656,
0.343750000000655,0.375000000000631,0.424118674845255,0.47154061341085,
0.500000000000517,0.545140118142051,0.562500000000471,0.578125000000458,
0.592606776586451,0.593750000000444,0.625000000000417,0.676269578279683,
0.729670216140662,0.750000000000281,0.812499188271712,0.874919170302411,
0.940466393599129,0.999996753086006),.UNSPECIFIED.);
#29890=B_SPLINE_CURVE_WITH_KNOTS('',3,(#145502,#145503,#145504,#145505,
#145506,#145507,#145508,#145509,#145510,#145511,#145512,#145513,#145514,
#145515,#145516,#145517,#145518,#145519,#145520,#145521,#145522,#145523,
#145524,#145525,#145526,#145527,#145528,#145529,#145530,#145531,#145532,
#145533,#145534,#145535,#145536,#145537,#145538,#145539,#145540,#145541,
#145542,#145543,#145544,#145545,#145546,#145547,#145548,#145549,#145550,
#145551,#145552,#145553,#145554,#145555,#145556,#145557,#145558,#145559,
#145560,#145561,#145562,#145563,#145564,#145565,#145566,#145567,#145568,
#145569,#145570,#145571,#145572,#145573,#145574),.UNSPECIFIED.,.F.,.F.,
(4,3,3,3,3,3,3,3,3,3,3,3,3,3,3,3,3,3,3,3,3,3,3,3,4),(1.9928678793837E-13,
0.0860107073934107,0.170441003692805,0.249999999999952,0.332517288333061,
0.413780234995208,0.437499999999927,0.468749999999926,0.484374999999937,
0.492187499999939,0.497856535392512,0.499999999999941,0.548330130830557,
0.595519789803843,0.641493515213737,0.686233649869448,0.729763227325348,
0.771593001760249,0.812496612229918,0.852092647954145,0.874999999999985,
0.912928094030672,0.950130538294064,0.986349268772354,1.),.UNSPECIFIED.);
#29891=B_SPLINE_CURVE_WITH_KNOTS('',3,(#145577,#145578,#145579,#145580,
#145581,#145582),.UNSPECIFIED.,.F.,.F.,(4,2,4),(-0.541273296520499,-0.270636648260383,
-0.132804212465021),.UNSPECIFIED.);
#29892=B_SPLINE_CURVE_WITH_KNOTS('',3,(#145583,#145584,#145585,#145586,
#145587,#145588),.UNSPECIFIED.,.F.,.F.,(4,2,4),(-1.54420814271699,-1.40637570692167,
-1.13573905866164),.UNSPECIFIED.);
#29893=B_SPLINE_CURVE_WITH_KNOTS('',3,(#145601,#145602,#145603,#145604,
#145605,#145606,#145607,#145608,#145609,#145610,#145611,#145612,#145613,
#145614,#145615,#145616),.UNSPECIFIED.,.F.,.F.,(4,3,3,3,3,4),(2.40891265344009E-9,
0.20000000192713,0.400000001445348,0.600000000963565,0.800000000481783,
1.),.UNSPECIFIED.);
#29894=B_SPLINE_CURVE_WITH_KNOTS('',3,(#145622,#145623,#145624,#145625,
#145626),.UNSPECIFIED.,.F.,.F.,(4,1,4),(0.,0.5,1.),.UNSPECIFIED.);
#29895=B_SPLINE_CURVE_WITH_KNOTS('',3,(#145704,#145705,#145706,#145707,
#145708,#145709,#145710,#145711,#145712,#145713,#145714,#145715,#145716,
#145717,#145718,#145719,#145720,#145721,#145722,#145723,#145724,#145725,
#145726,#145727,#145728,#145729,#145730,#145731,#145732,#145733,#145734,
#145735,#145736,#145737,#145738,#145739,#145740,#145741,#145742,#145743,
#145744,#145745,#145746,#145747,#145748,#145749,#145750,#145751,#145752,
#145753,#145754,#145755,#145756,#145757,#145758,#145759,#145760,#145761,
#145762,#145763,#145764,#145765,#145766,#145767,#145768,#145769,#145770,
#145771,#145772,#145773,#145774,#145775,#145776,#145777,#145778,#145779,
#145780,#145781,#145782,#145783,#145784,#145785,#145786,#145787,#145788,
#145789,#145790,#145791,#145792,#145793,#145794,#145795,#145796,#145797),
 .UNSPECIFIED.,.F.,.F.,(4,3,3,3,3,3,3,3,3,3,3,3,3,3,3,3,3,3,3,3,3,3,3,3,
3,3,3,3,3,3,3,4),(0.,0.0503273433392803,0.0705363966084534,0.09090909090909,
0.145845069792584,0.165424748295987,0.1818181818182,0.254342976911016,0.260135405827298,
0.2727272727273,0.354924390092219,0.3636363636364,0.43720034945726,0.449680449551842,
0.4545454545455,0.524937984162795,0.54443382589536,0.5454545454545,0.599437773241359,
0.6363636363636,0.639231171883239,0.701503428544661,0.7272727272727,0.733981119727695,
0.796476371383321,0.8181818181818,0.82875679278927,0.887282233501452,0.9090909090909,
0.92353921349181,0.975376204950871,0.999999996385405),.UNSPECIFIED.);
#29896=B_SPLINE_CURVE_WITH_KNOTS('',3,(#145800,#145801,#145802,#145803,
#145804,#145805,#145806,#145807,#145808,#145809,#145810,#145811,#145812,
#145813,#145814,#145815,#145816,#145817,#145818,#145819,#145820,#145821,
#145822,#145823,#145824,#145825,#145826,#145827,#145828,#145829,#145830),
 .UNSPECIFIED.,.F.,.F.,(4,3,3,3,3,3,3,3,3,3,4),(1.55097127508771E-10,0.185276535990514,
0.249999999999993,0.263984396772149,0.374999999999989,0.437499999999986,
0.499999999999984,0.691147771436497,0.825408769424091,0.970656694537131,
1.),.UNSPECIFIED.);
#29897=B_SPLINE_CURVE_WITH_KNOTS('',3,(#145836,#145837,#145838,#145839,
#145840,#145841,#145842,#145843,#145844,#145845,#145846,#145847,#145848,
#145849,#145850,#145851,#145852,#145853,#145854),.UNSPECIFIED.,.F.,.F.,
(4,3,3,3,3,3,4),(0.,0.249999999999992,0.374999999999993,0.463820810658223,
0.499999999999994,0.804024102868561,1.),.UNSPECIFIED.);
#29898=B_SPLINE_CURVE_WITH_KNOTS('',3,(#145871,#145872,#145873,#145874,
#145875,#145876,#145877,#145878,#145879,#145880),.UNSPECIFIED.,.F.,.F.,
(4,3,3,4),(0.,0.416125778815456,0.832277185977338,1.),.UNSPECIFIED.);
#29899=B_SPLINE_CURVE_WITH_KNOTS('',3,(#145887,#145888,#145889,#145890,
#145891,#145892,#145893,#145894,#145895,#145896,#145897,#145898,#145899,
#145900,#145901,#145902,#145903,#145904,#145905,#145906,#145907,#145908,
#145909,#145910,#145911,#145912,#145913,#145914,#145915,#145916,#145917,
#145918,#145919,#145920,#145921,#145922,#145923,#145924,#145925,#145926,
#145927,#145928,#145929,#145930,#145931,#145932,#145933,#145934,#145935,
#145936,#145937,#145938,#145939,#145940,#145941,#145942,#145943,#145944,
#145945,#145946,#145947),.UNSPECIFIED.,.F.,.F.,(4,3,3,3,3,3,3,3,3,3,3,3,
3,3,3,3,3,3,3,3,4),(0.,0.0302549049560431,0.107699539561875,0.187447489182287,
0.268742965198622,0.350914596186216,0.43361546396603,0.5,0.516809378194048,
0.583584210388533,0.597628782117945,0.660260938893525,0.676918155576055,
0.739525996857477,0.756610374301218,0.817971707078341,0.838101869863211,
0.902215138768424,0.922705812894093,0.990587366249333,1.),.UNSPECIFIED.);
#29900=B_SPLINE_CURVE_WITH_KNOTS('',3,(#146035,#146036,#146037,#146038,
#146039,#146040),.UNSPECIFIED.,.F.,.F.,(4,2,4),(3.71650158233969E-7,0.5,
0.999999989920246),.UNSPECIFIED.);
#29901=B_SPLINE_CURVE_WITH_KNOTS('',3,(#146041,#146042,#146043,#146044,
#146045,#146046,#146047,#146048,#146049,#146050,#146051,#146052,#146053,
#146054,#146055,#146056,#146057,#146058,#146059,#146060,#146061,#146062,
#146063,#146064,#146065,#146066,#146067,#146068,#146069,#146070,#146071,
#146072,#146073,#146074,#146075,#146076,#146077),.UNSPECIFIED.,.F.,.F.,
(4,3,3,3,3,3,3,3,3,3,3,3,4),(0.,0.0851665874734178,0.173246627155873,0.267902347683297,
0.368005119889117,0.478252701139369,0.5,0.601785236450079,0.701338926617578,
0.797284493127895,0.890006807195087,0.978859996903235,0.999999997120075),
 .UNSPECIFIED.);
#29902=B_SPLINE_CURVE_WITH_KNOTS('',3,(#146082,#146083,#146084,#146085,
#146086,#146087,#146088,#146089,#146090,#146091,#146092,#146093,#146094,
#146095,#146096,#146097,#146098,#146099,#146100,#146101,#146102,#146103,
#146104,#146105,#146106,#146107,#146108,#146109,#146110,#146111,#146112,
#146113,#146114,#146115,#146116,#146117,#146118,#146119,#146120,#146121,
#146122,#146123,#146124,#146125,#146126,#146127,#146128,#146129,#146130),
 .UNSPECIFIED.,.F.,.F.,(4,3,3,3,3,3,3,3,3,3,3,3,3,3,3,3,4),(9.31491747942225E-7,
0.0775965643526843,0.154644840464124,0.231115057634255,0.25,0.321927191564919,
0.393664323259736,0.465280451197901,0.5,0.571646826427887,0.643349061639341,
0.715296736344095,0.75,0.826607919696912,0.903602320363381,0.981339531684117,
1.),.UNSPECIFIED.);
#29903=B_SPLINE_CURVE_WITH_KNOTS('',3,(#146168,#146169,#146170,#146171,
#146172,#146173,#146174,#146175,#146176,#146177,#146178,#146179,#146180,
#146181,#146182,#146183,#146184,#146185,#146186,#146187,#146188,#146189),
 .UNSPECIFIED.,.F.,.F.,(4,3,3,3,3,3,3,4),(3.08423462885857E-7,0.152032233615953,
0.306191896926236,0.463527373595914,0.5,0.661792255427938,0.830896126248164,
0.99999999706839),.UNSPECIFIED.);
#29904=B_SPLINE_CURVE_WITH_KNOTS('',3,(#146227,#146228,#146229,#146230,
#146231,#146232,#146233,#146234,#146235,#146236,#146237,#146238,#146239,
#146240,#146241,#146242,#146243,#146244,#146245,#146246,#146247,#146248,
#146249,#146250,#146251,#146252,#146253,#146254,#146255,#146256,#146257,
#146258,#146259,#146260,#146261,#146262,#146263,#146264,#146265,#146266,
#146267,#146268,#146269,#146270,#146271,#146272,#146273,#146274,#146275,
#146276,#146277,#146278,#146279,#146280,#146281),.UNSPECIFIED.,.F.,.F.,
(4,3,3,3,3,3,3,3,3,3,3,3,3,3,3,3,3,3,4),(0.,0.113195272986155,0.216845394807799,
0.249999999999949,0.329316019412936,0.374999999999922,0.43749999999991,
0.468749999999903,0.484374999999899,0.4921874999999,0.4999999999999,0.591157716507977,
0.673823762126518,0.682315433016053,0.761940801371688,0.838990173165727,
0.914264268728704,0.988334189438011,1.),.UNSPECIFIED.);
#29905=B_SPLINE_CURVE_WITH_KNOTS('',3,(#146282,#146283,#146284,#146285,
#146286,#146287,#146288,#146289,#146290,#146291,#146292,#146293,#146294),
 .UNSPECIFIED.,.F.,.F.,(4,3,3,3,4),(0.,0.286212728725273,0.5,0.62499418580237,
1.),.UNSPECIFIED.);
#29906=B_SPLINE_CURVE_WITH_KNOTS('',3,(#146301,#146302,#146303,#146304,
#146305,#146306,#146307,#146308,#146309,#146310),.UNSPECIFIED.,.F.,.F.,
(4,3,3,4),(6.80373258488048E-7,0.3333333333333,0.6666666666667,1.),
 .UNSPECIFIED.);
#29907=B_SPLINE_CURVE_WITH_KNOTS('',3,(#146312,#146313,#146314,#146315,
#146316,#146317,#146318,#146319,#146320),.UNSPECIFIED.,.F.,.F.,(4,1,2,2,
4),(0.,0.249999999999992,0.43749999999999,0.499999999999991,1.),
 .UNSPECIFIED.);
#29908=B_SPLINE_CURVE_WITH_KNOTS('',3,(#146322,#146323,#146324,#146325,
#146326,#146327,#146328,#146329,#146330,#146331),.UNSPECIFIED.,.F.,.F.,
(4,3,3,4),(1.28220999446224E-10,0.395671114820227,0.5,0.999991077247271),
 .UNSPECIFIED.);
#29909=B_SPLINE_CURVE_WITH_KNOTS('',3,(#146335,#146336,#146337,#146338,
#146339,#146340,#146341),.UNSPECIFIED.,.F.,.F.,(4,3,4),(6.08353928510026E-5,
0.5,1.),.UNSPECIFIED.);
#29910=B_SPLINE_CURVE_WITH_KNOTS('',3,(#146343,#146344,#146345,#146346,
#146347,#146348,#146349,#146350,#146351),.UNSPECIFIED.,.F.,.F.,(4,1,2,2,
4),(0.,0.250000000000012,0.437500000000015,0.500000000000015,1.),
 .UNSPECIFIED.);
#29911=B_SPLINE_CURVE_WITH_KNOTS('',3,(#146353,#146354,#146355,#146356,
#146357,#146358,#146359,#146360,#146361,#146362),.UNSPECIFIED.,.F.,.F.,
(4,3,3,4),(0.,0.3333333333333,0.6666666666667,1.),.UNSPECIFIED.);
#29912=B_SPLINE_CURVE_WITH_KNOTS('',3,(#146370,#146371,#146372,#146373,
#146374,#146375,#146376,#146377,#146378,#146379,#146380,#146381,#146382,
#146383,#146384,#146385,#146386,#146387,#146388,#146389,#146390,#146391,
#146392,#146393,#146394,#146395,#146396,#146397),.UNSPECIFIED.,.F.,.F.,
(4,3,3,3,3,3,3,3,3,4),(7.74771400272031E-10,0.101808906684311,0.209007899927755,
0.319213880211576,0.433855115514003,0.5,0.633394711854997,0.769804406161013,
0.909129008998587,1.),.UNSPECIFIED.);
#29913=B_SPLINE_CURVE_WITH_KNOTS('',3,(#146398,#146399,#146400,#146401,
#146402,#146403,#146404,#146405,#146406,#146407,#146408,#146409,#146410,
#146411,#146412,#146413,#146414,#146415,#146416,#146417,#146418,#146419,
#146420,#146421,#146422,#146423,#146424,#146425,#146426,#146427,#146428),
 .UNSPECIFIED.,.F.,.F.,(4,3,3,3,3,3,3,3,3,3,4),(1.19933140293008E-6,0.131666198962597,
0.263331198593791,0.381665599296896,0.5,0.604251376078316,0.707930455352679,
0.809312850427695,0.85384492428718,0.947128621831252,0.999999999652553),
 .UNSPECIFIED.);
#29914=B_SPLINE_CURVE_WITH_KNOTS('',3,(#146462,#146463,#146464,#146465,
#146466,#146467,#146468,#146469,#146470,#146471,#146472,#146473,#146474,
#146475,#146476,#146477,#146478,#146479,#146480,#146481,#146482,#146483,
#146484,#146485,#146486,#146487,#146488,#146489,#146490,#146491,#146492,
#146493,#146494,#146495,#146496,#146497,#146498,#146499,#146500,#146501,
#146502,#146503,#146504,#146505,#146506,#146507),.UNSPECIFIED.,.F.,.F.,
(4,3,3,3,3,3,3,3,3,3,3,3,3,3,3,4),(0.,0.075211943614556,0.149374857838509,
0.222342548672234,0.24999999999999,0.321768616869141,0.393073017284843,
0.46409303977792,0.535569779833439,0.606705160188612,0.678432144318015,
0.749999999999997,0.823144987521618,0.897062157875133,0.972435540661161,
0.999997996759352),.UNSPECIFIED.);
#29915=B_SPLINE_CURVE_WITH_KNOTS('',3,(#146509,#146510,#146511,#146512,
#146513,#146514,#146515,#146516,#146517,#146518,#146519,#146520,#146521,
#146522,#146523,#146524,#146525,#146526,#146527,#146528,#146529,#146530,
#146531,#146532,#146533,#146534,#146535,#146536,#146537,#146538,#146539,
#146540,#146541,#146542,#146543,#146544,#146545,#146546,#146547,#146548,
#146549,#146550,#146551,#146552,#146553,#146554),.UNSPECIFIED.,.F.,.F.,
(4,3,3,3,3,3,3,3,3,3,3,3,3,3,3,4),(2.60632369190722E-5,0.0888951179664604,
0.174399962481206,0.250000000000064,0.331533505523139,0.375000000000089,
0.437500000000094,0.468750000000098,0.48601987249119,0.500000000000103,
0.59250523058956,0.685269749800581,0.77894690994834,0.873279069584689,0.968967243094595,
1.),.UNSPECIFIED.);
#29916=B_SPLINE_CURVE_WITH_KNOTS('',3,(#146555,#146556,#146557,#146558,
#146559,#146560,#146561,#146562,#146563,#146564,#146565,#146566,#146567,
#146568,#146569,#146570,#146571,#146572,#146573,#146574,#146575,#146576,
#146577,#146578,#146579,#146580,#146581,#146582,#146583,#146584,#146585,
#146586,#146587,#146588,#146589,#146590,#146591,#146592,#146593,#146594,
#146595,#146596,#146597,#146598,#146599,#146600,#146601,#146602,#146603,
#146604,#146605,#146606),.UNSPECIFIED.,.F.,.F.,(4,3,3,3,3,3,3,3,3,3,3,3,
3,3,3,3,3,4),(0.,0.0950940026076129,0.176000808070446,0.250000000000337,
0.341236634860541,0.375000000000488,0.437500000000555,0.468750000000575,
0.484375000000586,0.49218750000059,0.497660107483689,0.500000000000595,
0.593847149190447,0.684418942999604,0.770105050752368,0.853413617968863,
0.933763885470399,1.),.UNSPECIFIED.);
#29917=B_SPLINE_CURVE_WITH_KNOTS('',3,(#146618,#146619,#146620,#146621,
#146622,#146623,#146624,#146625,#146626,#146627,#146628,#146629,#146630,
#146631,#146632,#146633,#146634,#146635,#146636,#146637,#146638,#146639,
#146640,#146641,#146642,#146643,#146644,#146645,#146646,#146647,#146648,
#146649,#146650,#146651,#146652,#146653,#146654),.UNSPECIFIED.,.F.,.F.,
(4,3,3,3,3,3,3,3,3,3,3,3,4),(0.,0.0971273534595727,0.19784551509468,0.294981060322154,
0.392102579023238,0.489225386209634,0.5,0.597127342691812,0.697845507018859,
0.794981048125729,0.892102564806965,0.989225372332922,1.),.UNSPECIFIED.);
#29918=B_SPLINE_CURVE_WITH_KNOTS('',3,(#146659,#146660,#146661,#146662,
#146663,#146664,#146665,#146666,#146667,#146668,#146669,#146670,#146671,
#146672,#146673,#146674,#146675,#146676,#146677,#146678,#146679,#146680,
#146681,#146682,#146683,#146684,#146685,#146686,#146687,#146688,#146689,
#146690,#146691,#146692,#146693,#146694,#146695),.UNSPECIFIED.,.F.,.F.,
(4,3,3,3,3,3,3,3,3,3,3,3,4),(1.27559074915848E-5,0.0877775439371207,0.175537174689751,
0.263312957184923,0.351076072595288,0.438847608910549,0.5,0.587764801064224,
0.675524453920255,0.763300261792778,0.851063397830683,0.938834946164502,
1.),.UNSPECIFIED.);
#29919=B_SPLINE_CURVE_WITH_KNOTS('',3,(#146748,#146749,#146750,#146751,
#146752,#146753),.UNSPECIFIED.,.F.,.F.,(4,2,4),(0.,0.5,1.),
 .UNSPECIFIED.);
#29920=B_SPLINE_CURVE_WITH_KNOTS('',3,(#146754,#146755,#146756,#146757,
#146758,#146759,#146760,#146761,#146762,#146763,#146764,#146765,#146766,
#146767,#146768,#146769,#146770,#146771,#146772,#146773,#146774,#146775,
#146776,#146777,#146778,#146779,#146780,#146781,#146782,#146783,#146784,
#146785,#146786,#146787,#146788,#146789,#146790),.UNSPECIFIED.,.F.,.F.,
(4,3,3,3,3,3,3,3,3,3,3,3,4),(0.,0.0171128929119407,0.190218335415339,0.250000000000002,
0.342243520336091,0.478336826191752,0.600628348881761,0.711130774206828,
0.811077032826439,0.875000000000001,0.901524999490352,0.982438882590532,
0.999999999878368),.UNSPECIFIED.);
#29921=B_SPLINE_CURVE_WITH_KNOTS('',3,(#146791,#146792,#146793,#146794,
#146795,#146796,#146797,#146798,#146799,#146800,#146801,#146802,#146803,
#146804,#146805,#146806,#146807,#146808,#146809,#146810,#146811,#146812,
#146813,#146814,#146815,#146816,#146817,#146818,#146819,#146820,#146821,
#146822,#146823,#146824,#146825,#146826,#146827,#146828,#146829,#146830,
#146831,#146832,#146833,#146834,#146835,#146836),.UNSPECIFIED.,.F.,.F.,
(4,3,3,3,3,3,3,3,3,3,3,3,3,3,3,4),(0.,0.0645900761448876,0.191864486905108,
0.206466423904439,0.332843758757244,0.418999255127509,0.449056161984938,
0.5,0.55881796002962,0.665119182877143,0.770052640000822,0.860961845222702,
0.874974935448854,0.951626181348456,0.98078069154919,1.),.UNSPECIFIED.);
#29922=B_SPLINE_CURVE_WITH_KNOTS('',3,(#146925,#146926,#146927,#146928,
#146929,#146930,#146931,#146932,#146933,#146934),.UNSPECIFIED.,.F.,.F.,
(4,2,2,2,4),(2.04724411541053E-5,0.25,0.5,0.75,1.),.UNSPECIFIED.);
#29923=B_SPLINE_CURVE_WITH_KNOTS('',3,(#146960,#146961,#146962,#146963,
#146964,#146965,#146966,#146967,#146968,#146969,#146970,#146971,#146972,
#146973,#146974,#146975,#146976,#146977,#146978,#146979,#146980,#146981,
#146982,#146983,#146984,#146985,#146986,#146987,#146988,#146989,#146990,
#146991,#146992,#146993,#146994,#146995,#146996,#146997,#146998,#146999,
#147000,#147001,#147002,#147003,#147004,#147005,#147006,#147007,#147008),
 .UNSPECIFIED.,.F.,.F.,(4,3,3,3,3,3,3,3,3,3,3,3,3,3,3,3,4),(6.71413000258348E-9,
0.0675549200623969,0.134250059598761,0.199881392616613,0.25,0.314474527898111,
0.378587916313949,0.442420828705989,0.5,0.563842660090154,0.627812047922959,
0.692296526943969,0.75,0.815739886669369,0.882105973707192,0.949759631829514,
0.999999999917591),.UNSPECIFIED.);
#29924=B_SPLINE_CURVE_WITH_KNOTS('',3,(#147009,#147010,#147011,#147012,
#147013,#147014,#147015,#147016,#147017,#147018,#147019,#147020,#147021),
 .UNSPECIFIED.,.F.,.F.,(4,3,3,3,4),(8.57328517562898E-9,0.311955394560608,
0.68142062992333,0.716097880297857,0.999997541441199),.UNSPECIFIED.);
#29925=B_SPLINE_CURVE_WITH_KNOTS('',3,(#147098,#147099,#147100,#147101,
#147102,#147103,#147104,#147105,#147106,#147107,#147108,#147109,#147110,
#147111,#147112,#147113),.UNSPECIFIED.,.F.,.F.,(4,3,3,3,3,4),(0.,0.25,0.486439579144033,
0.5,0.723876910618796,0.999999995616857),.UNSPECIFIED.);
#29926=B_SPLINE_CURVE_WITH_KNOTS('',3,(#147116,#147117,#147118,#147119,
#147120,#147121,#147122,#147123,#147124,#147125,#147126,#147127,#147128,
#147129,#147130,#147131,#147132,#147133,#147134,#147135,#147136,#147137,
#147138,#147139,#147140,#147141,#147142,#147143,#147144,#147145,#147146,
#147147,#147148,#147149,#147150,#147151,#147152,#147153,#147154,#147155,
#147156,#147157,#147158,#147159,#147160,#147161,#147162,#147163,#147164,
#147165,#147166,#147167,#147168,#147169,#147170,#147171,#147172,#147173,
#147174,#147175,#147176,#147177,#147178,#147179,#147180,#147181,#147182,
#147183,#147184,#147185,#147186,#147187,#147188,#147189,#147190,#147191,
#147192,#147193,#147194,#147195,#147196,#147197,#147198,#147199,#147200,
#147201,#147202,#147203,#147204,#147205,#147206,#147207,#147208,#147209,
#147210,#147211,#147212,#147213,#147214,#147215,#147216,#147217,#147218),
 .UNSPECIFIED.,.F.,.F.,(4,3,3,3,3,3,3,3,3,3,3,3,3,3,3,3,3,3,3,3,3,3,3,3,
3,3,3,3,3,3,3,3,3,3,4),(0.,0.0271165187228091,0.0552398060865508,0.0805407362303379,
0.11740359361469,0.125000000000032,0.16370517204992,0.191078705246372,0.238272675229252,
0.287092952974552,0.326326031747244,0.381913015873678,0.437500000000112,
0.46875000000012,0.484375000000123,0.492187500000123,0.496093750000122,
0.498046875000122,0.498822511000944,0.500000000000122,0.550409406874595,
0.600158691511717,0.649053077344895,0.666386441247509,0.716491390494292,
0.764059731313792,0.805072474509961,0.843451464096043,0.87500000000003,
0.911087483580574,0.917362256906651,0.944900321435466,0.972450160717733,
0.998184909872044,1.),.UNSPECIFIED.);
#29927=B_SPLINE_CURVE_WITH_KNOTS('',3,(#147266,#147267,#147268,#147269,
#147270,#147271,#147272,#147273,#147274,#147275,#147276,#147277,#147278,
#147279,#147280,#147281,#147282,#147283,#147284,#147285,#147286,#147287,
#147288,#147289,#147290,#147291,#147292,#147293,#147294,#147295,#147296,
#147297,#147298,#147299,#147300,#147301,#147302,#147303,#147304,#147305,
#147306,#147307,#147308,#147309,#147310,#147311,#147312,#147313,#147314,
#147315,#147316,#147317,#147318,#147319,#147320,#147321,#147322,#147323,
#147324,#147325,#147326,#147327,#147328,#147329,#147330,#147331,#147332,
#147333,#147334,#147335,#147336,#147337,#147338,#147339,#147340,#147341,
#147342,#147343,#147344,#147345,#147346,#147347,#147348,#147349,#147350,
#147351,#147352,#147353,#147354,#147355,#147356,#147357,#147358,#147359,
#147360,#147361,#147362,#147363,#147364,#147365,#147366,#147367,#147368,
#147369,#147370,#147371,#147372,#147373,#147374),.UNSPECIFIED.,.F.,.F.,
(4,3,3,3,3,3,3,3,3,3,3,3,3,3,3,3,3,3,3,3,3,3,3,3,3,3,3,3,3,3,3,3,3,3,3,
3,4),(0.,0.0394411860672323,0.0768210319013784,0.111222926509573,0.125,
0.177992535930477,0.22748163487749,0.240547850416774,0.25,0.304443876426796,
0.357336889466944,0.369855255981034,0.375,0.408918181293526,0.442204793974763,
0.474505684652355,0.499217918791245,0.5,0.523587954797688,0.547077257231226,
0.570611985363674,0.594260904686012,0.618209786487464,0.625,0.628457442866467,
0.669404051401495,0.711444340562682,0.75,0.757882574283839,0.804582763960082,
0.852316761814482,0.875,0.887184989110887,0.920800954231189,0.955229031809878,
0.990899627273368,1.),.UNSPECIFIED.);
#29928=B_SPLINE_CURVE_WITH_KNOTS('',3,(#147401,#147402,#147403,#147404,
#147405,#147406),.UNSPECIFIED.,.F.,.F.,(4,1,1,4),(0.,0.3333333333333,0.6666666666667,
1.),.UNSPECIFIED.);
#29929=B_SPLINE_CURVE_WITH_KNOTS('',3,(#147408,#147409,#147410,#147411,
#147412,#147413),.UNSPECIFIED.,.F.,.F.,(4,2,4),(3.86991307802236E-7,0.5,
1.),.UNSPECIFIED.);
#29930=B_SPLINE_CURVE_WITH_KNOTS('',3,(#147414,#147415,#147416,#147417,
#147418,#147419,#147420,#147421,#147422,#147423,#147424,#147425,#147426),
 .UNSPECIFIED.,.F.,.F.,(4,3,3,3,4),(3.21889366672523E-15,0.236467493280666,
0.483668534912693,0.741834250234171,0.99999996555565),.UNSPECIFIED.);
#29931=B_SPLINE_CURVE_WITH_KNOTS('',3,(#147445,#147446,#147447,#147448),
 .UNSPECIFIED.,.F.,.F.,(4,4),(0.,1.),.UNSPECIFIED.);
#29932=B_SPLINE_CURVE_WITH_KNOTS('',3,(#147451,#147452,#147453,#147454,
#147455,#147456,#147457,#147458,#147459,#147460,#147461,#147462,#147463,
#147464,#147465,#147466,#147467,#147468,#147469,#147470,#147471,#147472,
#147473,#147474,#147475,#147476,#147477,#147478,#147479,#147480),
 .UNSPECIFIED.,.F.,.F.,(4,2,2,1,1,1,2,2,2,2,2,2,1,1,1,2,2,4),(0.,0.125000000000004,
0.187500000000005,0.218750000000006,0.234375000000007,0.242187500000007,
0.246093750000007,0.250000000000007,0.375000000000004,0.500000000000002,
0.624999999999999,0.687499999999998,0.718749999999998,0.734374999999997,
0.742187499999997,0.746093749999997,0.749999999999997,1.),.UNSPECIFIED.);
#29933=B_SPLINE_CURVE_WITH_KNOTS('',3,(#147481,#147482,#147483,#147484),
 .UNSPECIFIED.,.F.,.F.,(4,4),(0.,1.),.UNSPECIFIED.);
#29934=B_SPLINE_CURVE_WITH_KNOTS('',3,(#147578,#147579,#147580,#147581,
#147582,#147583,#147584,#147585,#147586,#147587,#147588,#147589,#147590,
#147591,#147592,#147593,#147594,#147595,#147596,#147597,#147598,#147599,
#147600,#147601,#147602,#147603,#147604,#147605,#147606,#147607,#147608,
#147609),.UNSPECIFIED.,.F.,.F.,(4,2,2,2,2,1,2,2,2,2,2,1,2,2,2,2,4),(0.,
0.0624999999999979,0.124999999999996,0.156249999999995,0.187499999999995,
0.218749999999994,0.234374999999994,0.249999999999994,0.374999999999995,
0.437499999999995,0.499999999999996,0.562499999999996,0.593749999999996,
0.624999999999997,0.687499999999997,0.749999999999998,1.),.UNSPECIFIED.);
#29935=B_SPLINE_CURVE_WITH_KNOTS('',3,(#147612,#147613,#147614,#147615,
#147616,#147617,#147618,#147619,#147620,#147621,#147622,#147623,#147624,
#147625,#147626,#147627,#147628,#147629,#147630,#147631,#147632,#147633,
#147634,#147635,#147636,#147637,#147638,#147639,#147640,#147641,#147642,
#147643,#147644,#147645,#147646,#147647,#147648,#147649,#147650,#147651,
#147652,#147653,#147654,#147655,#147656,#147657,#147658,#147659,#147660,
#147661,#147662,#147663,#147664,#147665,#147666,#147667,#147668,#147669,
#147670,#147671,#147672,#147673,#147674,#147675,#147676,#147677,#147678,
#147679,#147680,#147681,#147682,#147683,#147684,#147685,#147686,#147687,
#147688,#147689,#147690,#147691,#147692,#147693,#147694,#147695,#147696,
#147697,#147698,#147699,#147700,#147701,#147702),.UNSPECIFIED.,.F.,.F.,
(4,3,3,3,3,3,3,3,3,3,3,3,3,3,3,3,3,3,3,3,3,3,3,3,3,3,3,3,3,3,4),(1.67456784270334E-10,
0.0427557053620654,0.0840496960542369,0.125,0.16402161588874,0.202518234123198,
0.240354961866521,0.25,0.284884473303822,0.319542661327307,0.353941760428521,
0.375,0.407307079188093,0.439535083171299,0.471710072620308,0.5,0.532177878059925,
0.564377035663142,0.596685525002144,0.625,0.659425247468669,0.694006863967103,
0.728915833082306,0.75,0.787960510615582,0.826376766939918,0.865520707439689,
0.875,0.916019294839705,0.958474750871701,1.),.UNSPECIFIED.);
#29936=B_SPLINE_CURVE_WITH_KNOTS('',3,(#147703,#147704,#147705,#147706),
 .UNSPECIFIED.,.F.,.F.,(4,4),(2.04876468490802E-12,0.999998797216457),
 .UNSPECIFIED.);
#29937=B_SPLINE_CURVE_WITH_KNOTS('',3,(#147708,#147709,#147710,#147711),
 .UNSPECIFIED.,.F.,.F.,(4,4),(1.1801908511746E-6,1.),.UNSPECIFIED.);
#29938=B_SPLINE_CURVE_WITH_KNOTS('',3,(#147716,#147717,#147718,#147719,
#147720),.UNSPECIFIED.,.F.,.F.,(4,1,4),(0.000586994153978791,0.5,0.999443784375688),
 .UNSPECIFIED.);
#29939=B_SPLINE_CURVE_WITH_KNOTS('',3,(#147784,#147785,#147786,#147787,
#147788,#147789),.UNSPECIFIED.,.F.,.F.,(4,2,4),(1.44830354259436E-6,0.148225594517564,
0.296892255518428),.UNSPECIFIED.);
#29940=B_SPLINE_CURVE_WITH_KNOTS('',3,(#147790,#147791,#147792,#147793,
#147794,#147795,#147796,#147797,#147798,#147799,#147800,#147801,#147802,
#147803,#147804,#147805,#147806,#147807,#147808,#147809,#147810,#147811,
#147812,#147813,#147814,#147815,#147816,#147817),.UNSPECIFIED.,.F.,.F.,
(4,3,3,3,3,3,3,3,3,4),(0.,0.125349741004805,0.249758349526999,0.3748791747635,
0.5,0.625,0.74576818111402,0.866052850311141,0.985817153946618,1.),
 .UNSPECIFIED.);
#29941=B_SPLINE_CURVE_WITH_KNOTS('',3,(#147818,#147819,#147820,#147821,
#147822,#147823,#147824,#147825,#147826,#147827,#147828,#147829,#147830,
#147831,#147832,#147833,#147834),.UNSPECIFIED.,.F.,.F.,(4,2,2,1,1,1,2,2,
2,4),(0.,0.124999999999656,0.187499999999483,0.218749999999393,0.234374999999343,
0.242187499999318,0.24804687499931,0.24999999999931,0.49999999999954,1.),
 .UNSPECIFIED.);
#29942=B_SPLINE_CURVE_WITH_KNOTS('',3,(#147963,#147964,#147965,#147966,
#147967,#147968,#147969,#147970,#147971,#147972,#147973,#147974,#147975,
#147976),.UNSPECIFIED.,.F.,.F.,(4,2,2,2,2,2,4),(1.00000010829612E-6,0.0551684498922181,
0.111833996135768,0.16861384802555,0.226550710039574,0.281514160236136,
0.337551625530067),.UNSPECIFIED.);
#29943=B_SPLINE_CURVE_WITH_KNOTS('',3,(#147993,#147994,#147995,#147996,
#147997,#147998),.UNSPECIFIED.,.F.,.F.,(4,2,4),(4.92574313644089E-5,0.0292970799088927,
0.0585464725933476),.UNSPECIFIED.);
#29944=B_SPLINE_CURVE_WITH_KNOTS('',3,(#148081,#148082,#148083,#148084,
#148085,#148086,#148087,#148088,#148089,#148090,#148091,#148092,#148093,
#148094,#148095,#148096,#148097,#148098,#148099,#148100,#148101,#148102,
#148103,#148104,#148105,#148106,#148107,#148108,#148109,#148110,#148111,
#148112,#148113,#148114,#148115,#148116,#148117,#148118,#148119,#148120,
#148121,#148122,#148123,#148124,#148125,#148126,#148127,#148128,#148129,
#148130,#148131,#148132,#148133,#148134,#148135,#148136,#148137,#148138,
#148139,#148140,#148141,#148142,#148143,#148144,#148145,#148146,#148147,
#148148,#148149,#148150,#148151,#148152,#148153,#148154,#148155,#148156,
#148157,#148158,#148159,#148160,#148161,#148162,#148163,#148164,#148165,
#148166,#148167,#148168,#148169,#148170,#148171,#148172,#148173,#148174,
#148175,#148176,#148177,#148178,#148179,#148180,#148181,#148182,#148183,
#148184,#148185,#148186,#148187,#148188,#148189,#148190,#148191,#148192,
#148193,#148194,#148195,#148196,#148197,#148198,#148199,#148200,#148201,
#148202,#148203,#148204,#148205,#148206,#148207),.UNSPECIFIED.,.F.,.F.,
(4,3,3,3,3,3,3,3,3,3,3,3,3,3,3,3,3,3,3,3,3,3,3,3,3,3,3,3,3,3,3,3,3,3,3,
3,3,3,3,3,3,3,4),(0.,0.0395378850437958,0.0780200915431913,0.114432547161542,
0.125000000000007,0.159102920826881,0.191386870635889,0.201074434816447,
0.238265273042362,0.272243296330936,0.304871992254801,0.335705256204608,
0.365685268499672,0.400362784779306,0.434556392389667,0.466745053874986,
0.468750000000028,0.484375000000029,0.49218750000003,0.49609375000003,0.49804687500003,
0.499023437500029,0.500000000000029,0.507883393611758,0.532289603728898,
0.557189218947549,0.582919841466742,0.609182080991284,0.636315979770474,
0.6470686088343,0.678028335052706,0.710032700462084,0.718749999999933,0.734374999999928,
0.742187499999925,0.746093749999923,0.748046874999921,0.74999999999992,
0.803643684670449,0.849622242689776,0.910065827990631,0.968705713846152,
0.999999772449722),.UNSPECIFIED.);
#29945=B_SPLINE_CURVE_WITH_KNOTS('',3,(#148254,#148255,#148256,#148257,
#148258,#148259,#148260,#148261,#148262,#148263,#148264,#148265,#148266,
#148267,#148268,#148269,#148270,#148271,#148272,#148273,#148274,#148275,
#148276,#148277,#148278,#148279,#148280,#148281,#148282,#148283,#148284,
#148285,#148286,#148287,#148288,#148289,#148290,#148291,#148292,#148293,
#148294,#148295,#148296,#148297,#148298,#148299,#148300,#148301,#148302,
#148303,#148304,#148305,#148306,#148307,#148308,#148309,#148310,#148311,
#148312,#148313,#148314,#148315,#148316,#148317,#148318,#148319,#148320,
#148321,#148322,#148323,#148324,#148325,#148326,#148327,#148328,#148329,
#148330,#148331,#148332),.UNSPECIFIED.,.F.,.F.,(4,3,3,3,3,3,3,3,3,3,3,3,
3,3,3,3,3,3,3,3,3,3,3,3,3,3,4),(0.,0.0474320767126572,0.0946326886006528,
0.140923092999167,0.162439384980431,0.1666666666667,0.210993419848256,0.254956231845612,
0.298464378985549,0.3333333333333,0.337383184424287,0.387642864546409,0.436820715093529,
0.484559346746784,0.5,0.512349724231562,0.564394734908946,0.615530700787823,
0.6666666666667,0.687332440500564,0.74511395135353,0.800305157394242,0.8333333333333,
0.862289173200801,0.921296729034223,0.978711644555806,1.),.UNSPECIFIED.);
#29946=B_SPLINE_CURVE_WITH_KNOTS('',3,(#148333,#148334,#148335,#148336,
#148337,#148338,#148339,#148340,#148341,#148342,#148343,#148344,#148345,
#148346,#148347,#148348,#148349,#148350,#148351,#148352,#148353,#148354,
#148355,#148356,#148357,#148358,#148359,#148360,#148361,#148362,#148363,
#148364,#148365,#148366,#148367,#148368,#148369,#148370,#148371,#148372,
#148373,#148374,#148375,#148376,#148377,#148378,#148379,#148380,#148381,
#148382,#148383,#148384,#148385,#148386,#148387,#148388,#148389,#148390,
#148391,#148392,#148393,#148394,#148395,#148396,#148397,#148398,#148399,
#148400,#148401,#148402,#148403,#148404,#148405,#148406,#148407,#148408,
#148409,#148410,#148411,#148412,#148413,#148414,#148415,#148416,#148417),
 .UNSPECIFIED.,.F.,.F.,(4,3,3,3,3,3,3,3,3,3,3,3,3,3,3,3,3,3,3,3,3,3,3,3,
3,3,3,3,4),(0.,0.0455858941264268,0.0900676722499013,0.133106253218741,
0.175403108755941,0.216708992426193,0.250000000000003,0.290162447841863,
0.329903895741327,0.369192000698554,0.375000000000003,0.413876900465313,
0.452580956666026,0.491171017134247,0.500000000000004,0.538625685578037,
0.577322592156103,0.616249147781696,0.625000000000004,0.66442046172197,
0.704160089651944,0.744467769580063,0.750000000000004,0.791224950398625,
0.833139877316173,0.876352631852926,0.920342081968076,0.965764533040775,
1.),.UNSPECIFIED.);
#29947=B_SPLINE_CURVE_WITH_KNOTS('',3,(#148451,#148452,#148453,#148454,
#148455),.UNSPECIFIED.,.F.,.F.,(4,1,4),(0.,0.5,1.),.UNSPECIFIED.);
#29948=B_SPLINE_CURVE_WITH_KNOTS('',3,(#148489,#148490,#148491,#148492,
#148493,#148494,#148495,#148496,#148497,#148498),.UNSPECIFIED.,.F.,.F.,
(4,2,2,2,4),(-2.05526489217093,-1.54831938115258,-1.00799606378119,-0.491432960923045,
-0.000105186411817316),.UNSPECIFIED.);
#29949=B_SPLINE_CURVE_WITH_KNOTS('',3,(#148502,#148503,#148504,#148505),
 .UNSPECIFIED.,.F.,.F.,(4,4),(0.,0.999999598452425),.UNSPECIFIED.);
#29950=B_SPLINE_CURVE_WITH_KNOTS('',3,(#148507,#148508,#148509,#148510,
#148511,#148512,#148513,#148514,#148515,#148516,#148517,#148518,#148519,
#148520,#148521,#148522,#148523,#148524,#148525,#148526,#148527,#148528,
#148529,#148530,#148531,#148532,#148533,#148534,#148535,#148536,#148537),
 .UNSPECIFIED.,.F.,.F.,(4,3,3,3,3,3,3,3,3,3,4),(0.,0.124999894110832,0.24999992934917,
0.374999964587508,0.437499982206676,0.499999999825845,0.562500017445014,
0.625000035064183,0.750000070302521,0.875000105540858,1.),.UNSPECIFIED.);
#29951=B_SPLINE_CURVE_WITH_KNOTS('',3,(#148538,#148539,#148540,#148541),
 .UNSPECIFIED.,.F.,.F.,(4,4),(4.05016088455375E-7,1.),.UNSPECIFIED.);
#29952=B_SPLINE_CURVE_WITH_KNOTS('',3,(#148561,#148562,#148563,#148564),
 .UNSPECIFIED.,.F.,.F.,(4,4),(0.,1.),.UNSPECIFIED.);
#29953=B_SPLINE_CURVE_WITH_KNOTS('',3,(#148583,#148584,#148585,#148586,
#148587,#148588,#148589,#148590,#148591,#148592,#148593,#148594,#148595,
#148596,#148597,#148598,#148599,#148600,#148601,#148602,#148603,#148604,
#148605,#148606,#148607,#148608,#148609,#148610,#148611,#148612,#148613,
#148614,#148615,#148616,#148617,#148618,#148619,#148620,#148621,#148622,
#148623,#148624,#148625,#148626,#148627,#148628,#148629,#148630,#148631,
#148632,#148633,#148634,#148635,#148636,#148637,#148638,#148639,#148640,
#148641,#148642,#148643),.UNSPECIFIED.,.F.,.F.,(4,3,3,3,3,3,3,3,3,3,3,3,
3,3,3,3,3,3,3,3,4),(0.,0.190770165214888,0.250000000000013,0.375000000000016,
0.437500000000018,0.468750000000019,0.484375000000019,0.492187500000019,
0.500000000000019,0.569018803380385,0.636641230509603,0.702130813965924,
0.750000000000097,0.781250000000105,0.785156250000104,0.789062500000103,
0.7968750000001,0.812500000000088,0.875000000000057,0.976209630883769,1.),
 .UNSPECIFIED.);
#29954=B_SPLINE_CURVE_WITH_KNOTS('',3,(#148645,#148646,#148647,#148648,
#148649,#148650,#148651,#148652,#148653,#148654,#148655,#148656,#148657,
#148658,#148659,#148660,#148661,#148662,#148663,#148664,#148665,#148666),
 .UNSPECIFIED.,.F.,.F.,(4,3,3,3,3,3,3,4),(0.,0.187499999999997,0.374999999999994,
0.465346374523407,0.499999999999993,0.702063552429337,0.902036509644966,
1.),.UNSPECIFIED.);
#29955=B_SPLINE_CURVE_WITH_KNOTS('',3,(#148731,#148732,#148733,#148734,
#148735,#148736,#148737,#148738,#148739,#148740,#148741,#148742,#148743,
#148744,#148745,#148746,#148747,#148748,#148749,#148750,#148751,#148752,
#148753,#148754,#148755,#148756,#148757,#148758,#148759,#148760,#148761,
#148762,#148763,#148764),.UNSPECIFIED.,.F.,.F.,(4,2,2,1,1,1,2,2,2,2,2,2,
2,2,1,1,1,2,2,4),(0.,0.125000000000082,0.187500000000122,0.218750000000142,
0.234375000000152,0.242187500000155,0.246093750000156,0.250000000000157,
0.375000000000151,0.437500000000148,0.468750000000146,0.500000000000143,
0.625000000000127,0.687500000000118,0.718750000000113,0.734375000000109,
0.742187500000108,0.746093750000107,0.750000000000105,1.),.UNSPECIFIED.);
#29956=B_SPLINE_CURVE_WITH_KNOTS('',3,(#148767,#148768,#148769,#148770,
#148771,#148772,#148773,#148774,#148775,#148776,#148777,#148778,#148779,
#148780,#148781,#148782,#148783,#148784,#148785,#148786,#148787,#148788,
#148789,#148790,#148791,#148792,#148793,#148794,#148795,#148796,#148797,
#148798,#148799,#148800,#148801,#148802,#148803,#148804,#148805,#148806,
#148807,#148808,#148809,#148810,#148811,#148812,#148813,#148814,#148815,
#148816,#148817,#148818,#148819,#148820,#148821,#148822,#148823,#148824,
#148825,#148826,#148827,#148828,#148829,#148830,#148831,#148832,#148833,
#148834,#148835,#148836,#148837,#148838,#148839,#148840,#148841,#148842,
#148843,#148844,#148845,#148846,#148847,#148848,#148849,#148850,#148851,
#148852,#148853,#148854,#148855,#148856,#148857,#148858,#148859,#148860,
#148861,#148862,#148863,#148864,#148865,#148866,#148867,#148868,#148869,
#148870,#148871,#148872,#148873,#148874,#148875,#148876,#148877,#148878,
#148879,#148880,#148881,#148882,#148883,#148884,#148885,#148886,#148887,
#148888,#148889,#148890,#148891,#148892,#148893,#148894,#148895,#148896,
#148897,#148898,#148899,#148900,#148901,#148902,#148903,#148904,#148905,
#148906,#148907,#148908,#148909,#148910,#148911,#148912,#148913,#148914,
#148915,#148916,#148917,#148918,#148919,#148920,#148921,#148922,#148923,
#148924,#148925,#148926,#148927,#148928,#148929,#148930,#148931,#148932,
#148933,#148934,#148935,#148936,#148937,#148938,#148939,#148940,#148941,
#148942,#148943,#148944,#148945,#148946,#148947,#148948,#148949,#148950,
#148951,#148952,#148953,#148954,#148955,#148956),.UNSPECIFIED.,.F.,.F.,
(4,3,3,3,3,3,3,3,3,3,3,3,3,3,3,3,3,3,3,3,3,3,3,3,3,3,3,3,3,3,3,3,3,3,3,
3,3,3,3,3,3,3,3,3,3,3,3,3,3,3,3,3,3,3,3,3,3,3,3,3,3,3,3,4),(0.,0.0325663096439314,
0.0652395420398298,0.0979584965072984,0.125000000002429,0.140625000002734,
0.142578125002771,0.144377797393464,0.144531250002809,0.148437500002884,
0.156250000003032,0.187500000003627,0.229178571732012,0.250000000004818,
0.281250000005412,0.285156250005487,0.285644531255495,0.286132812505503,
0.287109375005499,0.289062500005488,0.296875000005429,0.312500000005324,
0.336074545739341,0.359628477884607,0.375000000004924,0.398483031248456,
0.421881190788266,0.437500000004523,0.460689275415805,0.468750000004323,
0.484375000004223,0.492187500004174,0.496093750004149,0.498046875004136,
0.500000000004123,0.553525721980606,0.60702301589617,0.625000000003431,
0.677521774987248,0.687500000003084,0.71875000000291,0.734375000002825,
0.742187500002782,0.749511718752743,0.75000000000274,0.765625000002564,
0.780744058039143,0.796622029020588,0.812500000002033,0.828125000001857,
0.843750000001681,0.858514060594805,0.859375000001504,0.867187500001415,
0.87109375000137,0.873046875001348,0.874023437501338,0.875000000001327,
0.897607080137333,0.920471072316808,0.937500000000664,0.960507524861031,
0.983627731936416,1.),.UNSPECIFIED.);
#29957=B_SPLINE_CURVE_WITH_KNOTS('',3,(#148958,#148959,#148960,#148961,
#148962,#148963,#148964,#148965,#148966,#148967,#148968,#148969,#148970,
#148971,#148972,#148973,#148974,#148975,#148976,#148977,#148978,#148979,
#148980,#148981,#148982,#148983,#148984,#148985,#148986,#148987,#148988,
#148989,#148990,#148991,#148992,#148993,#148994),.UNSPECIFIED.,.F.,.F.,
(4,3,3,3,3,3,3,3,3,3,3,3,4),(0.,0.0930590071063409,0.185651390275755,0.277313404654321,
0.368302886143633,0.45813055065145,0.5,0.588081733577098,0.674994332807131,
0.760020789035996,0.843967295660058,0.926160665559156,1.),.UNSPECIFIED.);
#29958=B_SPLINE_CURVE_WITH_KNOTS('',3,(#149136,#149137,#149138,#149139,
#149140,#149141,#149142,#149143,#149144,#149145,#149146,#149147,#149148,
#149149,#149150,#149151,#149152,#149153,#149154,#149155,#149156,#149157,
#149158,#149159,#149160,#149161,#149162,#149163,#149164,#149165,#149166,
#149167,#149168,#149169,#149170,#149171,#149172,#149173,#149174,#149175,
#149176,#149177,#149178,#149179,#149180,#149181,#149182,#149183,#149184,
#149185,#149186,#149187,#149188,#149189,#149190,#149191,#149192,#149193,
#149194,#149195,#149196,#149197,#149198,#149199,#149200,#149201,#149202,
#149203,#149204,#149205),.UNSPECIFIED.,.F.,.F.,(4,3,3,3,3,3,3,3,3,3,3,3,
3,3,3,3,3,3,3,3,3,3,3,4),(0.,0.0530696375713618,0.10597175525186,0.125000000000207,
0.184073079506744,0.242252390671621,0.250000000000417,0.300353856516711,
0.351927538736091,0.375000000000626,0.427736269402923,0.437500000000733,
0.468750000000782,0.484375000000809,0.492187500000819,0.496093750000821,
0.498046875000821,0.50000000000082,0.585242731062141,0.672617291309937,
0.763561346558681,0.856698761090278,0.953299858538298,1.),.UNSPECIFIED.);
#29959=B_SPLINE_CURVE_WITH_KNOTS('',3,(#149208,#149209,#149210,#149211,
#149212,#149213,#149214,#149215,#149216,#149217,#149218,#149219,#149220,
#149221,#149222,#149223,#149224,#149225,#149226,#149227,#149228,#149229,
#149230,#149231,#149232,#149233,#149234,#149235,#149236,#149237,#149238,
#149239,#149240,#149241,#149242,#149243,#149244,#149245,#149246,#149247,
#149248,#149249,#149250,#149251,#149252,#149253,#149254,#149255,#149256,
#149257,#149258,#149259,#149260,#149261,#149262,#149263,#149264,#149265,
#149266,#149267,#149268,#149269,#149270,#149271),.UNSPECIFIED.,.F.,.F.,
(4,3,3,3,3,3,3,3,3,3,3,3,3,3,3,3,3,3,3,3,3,4),(0.,0.101946695149731,0.202232035950964,
0.2500000000002,0.348102987925477,0.375000000000297,0.437500000000346,0.468750000000372,
0.484375000000385,0.49218750000039,0.498046875000392,0.500000000000393,
0.553018142384203,0.605910416481641,0.625000000000295,0.690733261304678,
0.750000000000197,0.802837365431866,0.856075997664884,0.909470261574667,
0.963029692389013,0.999997713195439),.UNSPECIFIED.);
#29960=B_SPLINE_CURVE_WITH_KNOTS('',3,(#149272,#149273,#149274,#149275,
#149276,#149277,#149278,#149279,#149280,#149281,#149282,#149283,#149284,
#149285,#149286,#149287,#149288,#149289,#149290,#149291,#149292,#149293,
#149294,#149295,#149296,#149297,#149298,#149299,#149300,#149301,#149302,
#149303,#149304,#149305,#149306,#149307,#149308,#149309,#149310,#149311,
#149312,#149313,#149314,#149315,#149316,#149317,#149318,#149319,#149320,
#149321,#149322,#149323,#149324,#149325,#149326,#149327,#149328,#149329,
#149330,#149331,#149332,#149333,#149334,#149335,#149336,#149337,#149338,
#149339,#149340,#149341,#149342,#149343,#149344,#149345,#149346,#149347,
#149348,#149349,#149350,#149351,#149352,#149353,#149354,#149355,#149356,
#149357,#149358,#149359,#149360,#149361,#149362,#149363,#149364,#149365,
#149366,#149367,#149368,#149369,#149370,#149371,#149372,#149373,#149374,
#149375,#149376,#149377,#149378,#149379,#149380,#149381,#149382,#149383,
#149384,#149385,#149386,#149387,#149388,#149389,#149390,#149391,#149392,
#149393,#149394,#149395,#149396,#149397,#149398,#149399,#149400,#149401,
#149402,#149403,#149404,#149405,#149406,#149407,#149408,#149409,#149410,
#149411,#149412,#149413,#149414,#149415,#149416,#149417,#149418,#149419,
#149420,#149421,#149422,#149423,#149424,#149425,#149426,#149427,#149428,
#149429,#149430,#149431,#149432,#149433,#149434,#149435,#149436,#149437,
#149438,#149439,#149440,#149441,#149442,#149443,#149444,#149445,#149446,
#149447,#149448,#149449,#149450,#149451,#149452,#149453,#149454,#149455,
#149456,#149457,#149458,#149459,#149460,#149461,#149462,#149463,#149464),
 .UNSPECIFIED.,.F.,.F.,(4,3,3,3,3,3,3,3,3,3,3,3,3,3,3,3,3,3,3,3,3,3,3,3,
3,3,3,3,3,3,3,3,3,3,3,3,3,3,3,3,3,3,3,3,3,3,3,3,3,3,3,3,3,3,3,3,3,3,3,3,
3,3,3,3,4),(0.,0.0824357364239239,0.119148634600739,0.125000000000686,0.18750000000103,
0.218750000001204,0.23437500000129,0.238310205703374,0.242187500001333,
0.246093750001353,0.248046875001364,0.249511718751369,0.250000000001371,
0.275393681203308,0.301516346052999,0.325694808248701,0.349380831708483,
0.372569384114915,0.395265609773867,0.417542957330609,0.439097282978513,
0.460279537636208,0.480970724120933,0.484375000000832,0.492187500000815,
0.496093750000807,0.498046875000803,0.498929468592768,0.499023437500802,
0.4995117187508,0.4997558593758,0.5000000000008,0.594238858917815,0.625000000000623,
0.687500000000534,0.695312500000524,0.699218750000517,0.701653256210494,
0.703125000000509,0.726683948334691,0.797244553002977,0.842069531868659,
0.843750000000286,0.848842741425888,0.851562500000274,0.865178344060018,
0.879352508045055,0.892721009198138,0.905807159823004,0.918394647074556,
0.921875000000165,0.923828125000163,0.92480468750016,0.925710282043078,
0.925781250000158,0.92968750000015,0.937500000000134,0.946187537931024,
0.95508063298552,0.964250861347624,0.968750000000067,0.97819414757121,0.987711388661645,
0.997278309415761,1.),.UNSPECIFIED.);
#29961=B_SPLINE_CURVE_WITH_KNOTS('',3,(#149529,#149530,#149531,#149532,
#149533,#149534,#149535,#149536,#149537,#149538,#149539,#149540,#149541,
#149542,#149543,#149544,#149545,#149546,#149547,#149548,#149549,#149550,
#149551,#149552,#149553,#149554,#149555,#149556,#149557,#149558,#149559,
#149560,#149561,#149562),.UNSPECIFIED.,.F.,.F.,(4,2,2,1,1,1,2,2,2,2,2,2,
2,2,1,1,1,2,2,4),(0.,0.125000000000023,0.187500000000035,0.218750000000042,
0.234375000000045,0.242187500000047,0.246093750000046,0.250000000000046,
0.375000000000051,0.437500000000054,0.468750000000056,0.500000000000057,
0.625000000000062,0.687500000000065,0.718750000000066,0.734375000000066,
0.742187500000066,0.746093750000067,0.750000000000067,1.),.UNSPECIFIED.);
#29962=B_SPLINE_CURVE_WITH_KNOTS('',3,(#149581,#149582,#149583,#149584,
#149585,#149586,#149587,#149588,#149589,#149590,#149591,#149592,#149593,
#149594,#149595,#149596,#149597,#149598,#149599,#149600,#149601,#149602,
#149603,#149604,#149605),.UNSPECIFIED.,.F.,.F.,(4,3,3,3,3,3,3,3,4),(0.,
0.195180283024368,0.250000000000003,0.375000000000002,0.4375,0.499999999999999,
0.682692802577324,0.866396269045124,1.),.UNSPECIFIED.);
#29963=B_SPLINE_CURVE_WITH_KNOTS('',3,(#149624,#149625,#149626,#149627,
#149628,#149629,#149630,#149631,#149632,#149633),.UNSPECIFIED.,.F.,.F.,
(4,3,3,4),(0.,0.464229907836084,0.91726039913087,1.),.UNSPECIFIED.);
#29964=B_SPLINE_CURVE_WITH_KNOTS('',3,(#149727,#149728,#149729,#149730,
#149731,#149732,#149733,#149734,#149735,#149736,#149737,#149738,#149739,
#149740,#149741,#149742,#149743,#149744,#149745,#149746,#149747,#149748,
#149749,#149750,#149751,#149752,#149753,#149754,#149755,#149756,#149757,
#149758,#149759,#149760,#149761,#149762,#149763,#149764,#149765,#149766,
#149767,#149768,#149769),.UNSPECIFIED.,.F.,.F.,(4,3,3,3,3,3,3,3,3,3,3,3,
3,3,4),(0.,0.105418333178882,0.210324340120241,0.313988331761175,0.375000000000047,
0.437500000000058,0.468750000000063,0.484375000000066,0.492187500000065,
0.500000000000064,0.625000000000048,0.742475783864713,0.856307677060081,
0.965238555229571,1.),.UNSPECIFIED.);
#29965=B_SPLINE_CURVE_WITH_KNOTS('',3,(#149770,#149771,#149772,#149773,
#149774,#149775,#149776,#149777,#149778,#149779,#149780,#149781,#149782,
#149783,#149784,#149785,#149786,#149787,#149788,#149789,#149790,#149791,
#149792,#149793,#149794,#149795,#149796,#149797,#149798,#149799,#149800,
#149801,#149802,#149803,#149804,#149805,#149806,#149807,#149808,#149809,
#149810,#149811,#149812,#149813,#149814,#149815),.UNSPECIFIED.,.F.,.F.,
(4,3,3,3,3,3,3,3,3,3,3,3,3,3,3,4),(0.,0.108316449197884,0.221360934376212,
0.250000000000046,0.368521273790907,0.375000000000071,0.437500000000084,
0.46875000000009,0.484375000000091,0.492187500000092,0.500000000000092,
0.601086242546387,0.704740924634103,0.809297948134376,0.914777359348703,
1.),.UNSPECIFIED.);
#29966=B_SPLINE_CURVE_WITH_KNOTS('',3,(#149830,#149831,#149832,#149833,
#149834,#149835,#149836,#149837,#149838,#149839,#149840,#149841,#149842,
#149843,#149844,#149845,#149846,#149847,#149848,#149849,#149850,#149851,
#149852,#149853,#149854,#149855,#149856,#149857,#149858,#149859,#149860,
#149861,#149862,#149863),.UNSPECIFIED.,.F.,.F.,(4,2,2,1,1,1,2,2,2,2,2,2,
2,2,1,1,1,2,2,4),(0.,0.124999999999981,0.187499999999971,0.218749999999967,
0.234374999999966,0.242187499999966,0.246093749999967,0.249999999999967,
0.374999999999974,0.437499999999977,0.468749999999979,0.499999999999981,
0.624999999999986,0.687499999999989,0.71874999999999,0.734374999999991,
0.742187499999992,0.746093749999993,0.749999999999994,1.),.UNSPECIFIED.);
#29967=B_SPLINE_CURVE_WITH_KNOTS('',3,(#149869,#149870,#149871,#149872,
#149873,#149874,#149875,#149876,#149877,#149878,#149879,#149880,#149881,
#149882,#149883,#149884,#149885,#149886,#149887,#149888,#149889,#149890,
#149891,#149892,#149893,#149894,#149895,#149896,#149897,#149898,#149899,
#149900,#149901,#149902,#149903,#149904,#149905,#149906,#149907,#149908,
#149909,#149910,#149911,#149912,#149913,#149914,#149915,#149916,#149917,
#149918,#149919,#149920,#149921,#149922,#149923,#149924,#149925,#149926,
#149927,#149928,#149929,#149930,#149931,#149932,#149933,#149934,#149935,
#149936,#149937,#149938,#149939,#149940,#149941,#149942,#149943,#149944,
#149945,#149946,#149947,#149948,#149949,#149950,#149951,#149952),
 .UNSPECIFIED.,.F.,.F.,(4,2,2,2,1,1,1,2,2,2,2,1,1,2,2,2,2,2,1,1,1,2,2,2,
2,2,2,2,1,1,1,1,2,2,2,2,2,1,2,2,2,2,2,1,1,1,2,2,2,4),(0.,0.0624999999999929,
0.0937499999999894,0.109374999999988,0.117187499999987,0.121093749999986,
0.123046874999986,0.124023437499986,0.124999999999986,0.187499999999978,
0.218749999999974,0.234374999999972,0.242187499999971,0.24609374999997,
0.24999999999997,0.312499999999963,0.34374999999996,0.359374999999958,0.367187499999957,
0.371093749999957,0.373046874999956,0.374511718749956,0.374999999999956,
0.43749999999996,0.499999999999964,0.562499999999968,0.59374999999997,0.609374999999971,
0.617187499999972,0.621093749999972,0.623046874999972,0.624023437499972,
0.624511718749972,0.624999999999972,0.687499999999977,0.718749999999979,
0.734374999999981,0.742187499999981,0.746093749999982,0.749999999999982,
0.812499999999987,0.84374999999999,0.859374999999991,0.867187499999992,
0.871093749999992,0.873046874999992,0.874023437499992,0.874999999999992,
0.937499999999996,1.),.UNSPECIFIED.);
#29968=B_SPLINE_CURVE_WITH_KNOTS('',3,(#149961,#149962,#149963,#149964,
#149965,#149966,#149967,#149968,#149969,#149970),.UNSPECIFIED.,.F.,.F.,
(4,3,3,4),(0.,0.373730880508955,0.752279314625459,1.),.UNSPECIFIED.);
#29969=B_SPLINE_CURVE_WITH_KNOTS('',3,(#149971,#149972,#149973,#149974,
#149975,#149976,#149977,#149978,#149979,#149980,#149981),.UNSPECIFIED.,
 .F.,.F.,(4,2,1,2,2,4),(0.,0.249999999999999,0.375000000000002,0.437500000000004,
0.500000000000006,1.),.UNSPECIFIED.);
#29970=B_SPLINE_CURVE_WITH_KNOTS('',3,(#149986,#149987,#149988,#149989,
#149990,#149991,#149992,#149993,#149994,#149995,#149996,#149997,#149998,
#149999,#150000,#150001,#150002,#150003,#150004,#150005,#150006,#150007,
#150008,#150009,#150010,#150011,#150012,#150013,#150014,#150015,#150016,
#150017,#150018,#150019,#150020,#150021,#150022,#150023,#150024,#150025,
#150026,#150027,#150028,#150029,#150030,#150031),.UNSPECIFIED.,.F.,.F.,
(4,3,3,3,3,3,3,3,3,3,3,3,3,3,3,4),(0.,0.108316449757411,0.221360935466982,
0.25000000000009,0.368521274253321,0.375000000000133,0.437500000000155,
0.468750000000163,0.484375000000169,0.49218750000017,0.500000000000171,
0.601086242782471,0.704740925103917,0.809297948826885,0.914777360240454,
1.),.UNSPECIFIED.);
#29971=B_SPLINE_CURVE_WITH_KNOTS('',3,(#150032,#150033,#150034,#150035,
#150036,#150037,#150038,#150039,#150040,#150041,#150042,#150043,#150044,
#150045,#150046,#150047,#150048,#150049,#150050,#150051,#150052,#150053,
#150054,#150055,#150056,#150057,#150058,#150059,#150060,#150061,#150062,
#150063,#150064,#150065,#150066,#150067,#150068,#150069,#150070,#150071,
#150072,#150073,#150074),.UNSPECIFIED.,.F.,.F.,(4,3,3,3,3,3,3,3,3,3,3,3,
3,3,4),(0.,0.105418332522525,0.210324338766372,0.313988329643646,0.374999999999986,
0.437499999999983,0.468749999999982,0.484374999999981,0.492187499999981,
0.499999999999981,0.624999999999986,0.742475782470587,0.856307674220441,
0.965238550848876,1.),.UNSPECIFIED.);
#29972=B_SPLINE_CURVE_WITH_KNOTS('',3,(#150085,#150086,#150087,#150088,
#150089,#150090,#150091,#150092,#150093,#150094,#150095,#150096,#150097,
#150098,#150099,#150100,#150101,#150102,#150103,#150104,#150105,#150106),
 .UNSPECIFIED.,.F.,.F.,(4,3,3,3,3,3,3,4),(0.,0.180289307661493,0.249999999999999,
0.431141781739715,0.499999999999998,0.702895542735386,0.903670705606259,
1.),.UNSPECIFIED.);
#29973=B_SPLINE_CURVE_WITH_KNOTS('',3,(#150107,#150108,#150109,#150110),
 .UNSPECIFIED.,.F.,.F.,(4,4),(0.,1.),.UNSPECIFIED.);
#29974=B_SPLINE_CURVE_WITH_KNOTS('',3,(#150113,#150114,#150115,#150116,
#150117,#150118,#150119,#150120,#150121,#150122,#150123,#150124,#150125,
#150126,#150127,#150128,#150129,#150130,#150131,#150132,#150133,#150134,
#150135,#150136,#150137,#150138,#150139,#150140,#150141,#150142,#150143,
#150144,#150145,#150146),.UNSPECIFIED.,.F.,.F.,(4,2,2,1,1,1,2,2,2,2,2,2,
2,2,1,1,1,2,2,4),(0.,0.125000000000041,0.18750000000006,0.218750000000069,
0.234375000000073,0.242187500000074,0.246093750000074,0.250000000000075,
0.375000000000062,0.437500000000056,0.468750000000052,0.500000000000048,
0.625000000000036,0.687500000000029,0.718750000000026,0.734375000000026,
0.742187500000025,0.746093750000024,0.750000000000024,1.),.UNSPECIFIED.);
#29975=B_SPLINE_CURVE_WITH_KNOTS('',3,(#150152,#150153,#150154,#150155,
#150156,#150157,#150158,#150159,#150160,#150161,#150162,#150163,#150164,
#150165,#150166,#150167,#150168,#150169,#150170,#150171,#150172,#150173,
#150174,#150175,#150176,#150177,#150178,#150179,#150180,#150181,#150182,
#150183,#150184,#150185,#150186,#150187,#150188,#150189,#150190,#150191,
#150192,#150193,#150194,#150195,#150196,#150197,#150198,#150199,#150200),
 .UNSPECIFIED.,.F.,.F.,(4,3,3,3,3,3,3,3,3,3,3,3,3,3,3,3,4),(0.,0.109992936268947,
0.221949217369093,0.334801520989419,0.449102907007153,0.5,0.603481968790449,
0.704814151412179,0.804699849390782,0.90242602165943,0.970121880641722,
0.97576964577923,0.981411740183398,0.987055876046289,0.992706300207867,
0.998373224606916,0.999999673423569),.UNSPECIFIED.);
#29976=B_SPLINE_CURVE_WITH_KNOTS('',3,(#150204,#150205,#150206,#150207,
#150208,#150209,#150210,#150211,#150212,#150213,#150214,#150215,#150216,
#150217,#150218,#150219,#150220,#150221,#150222,#150223,#150224,#150225,
#150226,#150227,#150228,#150229,#150230,#150231,#150232,#150233,#150234,
#150235,#150236,#150237,#150238,#150239,#150240,#150241,#150242,#150243,
#150244,#150245,#150246,#150247,#150248,#150249,#150250,#150251,#150252,
#150253,#150254,#150255),.UNSPECIFIED.,.F.,.F.,(4,3,3,3,3,3,3,3,3,3,3,3,
3,3,3,3,3,4),(3.07266740300672E-8,0.00572935959947857,0.0114446916406082,
0.0171497697196053,0.0228539059676719,0.0285640551379987,0.0303446246564232,
0.119140475170575,0.20920674037596,0.301032873773031,0.393773848547507,
0.487512351689386,0.5,0.613468602015531,0.725847537169989,0.837599874204618,
0.947948107414092,1.),.UNSPECIFIED.);
#29977=B_SPLINE_CURVE_WITH_KNOTS('',3,(#150279,#150280,#150281,#150282,
#150283,#150284,#150285,#150286,#150287,#150288,#150289,#150290,#150291,
#150292,#150293,#150294,#150295,#150296,#150297,#150298,#150299,#150300,
#150301,#150302,#150303,#150304,#150305,#150306,#150307,#150308,#150309,
#150310,#150311,#150312,#150313,#150314,#150315,#150316,#150317,#150318,
#150319,#150320,#150321,#150322,#150323,#150324,#150325,#150326,#150327,
#150328,#150329,#150330,#150331,#150332,#150333,#150334,#150335,#150336,
#150337,#150338,#150339,#150340,#150341,#150342),.UNSPECIFIED.,.F.,.F.,
(4,3,3,3,3,3,3,3,3,3,3,3,3,3,3,3,3,3,3,3,3,4),(0.,0.100687893601304,0.198167089124769,
0.250000000000073,0.3445731459175,0.375000000000112,0.43750000000013,0.46875000000014,
0.484375000000144,0.49218750000015,0.498046875000151,0.50000000000015,0.552999469608863,
0.605798665097521,0.625000000000113,0.687726037350389,0.750000000000075,
0.801899439950902,0.854740992711349,0.907950839930716,0.961508538596217,
1.),.UNSPECIFIED.);
#29978=B_SPLINE_CURVE_WITH_KNOTS('',3,(#150408,#150409,#150410,#150411,
#150412,#150413,#150414,#150415,#150416,#150417,#150418,#150419,#150420,
#150421,#150422,#150423,#150424,#150425,#150426,#150427,#150428,#150429,
#150430,#150431,#150432,#150433,#150434,#150435,#150436,#150437,#150438,
#150439,#150440,#150441,#150442,#150443,#150444,#150445,#150446,#150447,
#150448,#150449,#150450,#150451,#150452,#150453,#150454,#150455,#150456,
#150457,#150458,#150459,#150460,#150461,#150462,#150463,#150464,#150465,
#150466,#150467,#150468,#150469,#150470,#150471,#150472,#150473,#150474,
#150475,#150476,#150477,#150478,#150479,#150480,#150481,#150482,#150483,
#150484,#150485,#150486,#150487,#150488,#150489,#150490,#150491,#150492,
#150493,#150494,#150495,#150496,#150497,#150498,#150499,#150500,#150501,
#150502,#150503,#150504,#150505,#150506,#150507,#150508,#150509,#150510,
#150511,#150512,#150513,#150514,#150515,#150516,#150517,#150518,#150519,
#150520,#150521,#150522,#150523,#150524,#150525,#150526,#150527,#150528,
#150529,#150530,#150531,#150532,#150533,#150534,#150535,#150536,#150537,
#150538,#150539,#150540,#150541,#150542,#150543,#150544,#150545,#150546,
#150547,#150548,#150549,#150550,#150551,#150552,#150553,#150554,#150555,
#150556,#150557,#150558,#150559,#150560,#150561,#150562,#150563,#150564,
#150565,#150566,#150567,#150568,#150569,#150570,#150571,#150572,#150573,
#150574,#150575,#150576,#150577,#150578,#150579,#150580,#150581,#150582,
#150583,#150584,#150585,#150586,#150587,#150588,#150589,#150590,#150591,
#150592,#150593,#150594,#150595,#150596,#150597,#150598,#150599,#150600),
 .UNSPECIFIED.,.F.,.F.,(4,3,3,3,3,3,3,3,3,3,3,3,3,3,3,3,3,3,3,3,3,3,3,3,
3,3,3,3,3,3,3,3,3,3,3,3,3,3,3,3,3,3,3,3,3,3,3,3,3,3,3,3,3,3,3,3,3,3,3,3,
3,3,3,3,4),(0.,0.0824357367819663,0.119148634599032,0.124999999999361,0.187499999999041,
0.218749999998882,0.234374999998803,0.238310205699827,0.242187499998764,
0.246093749998744,0.248046874998735,0.249511718748729,0.249999999998727,
0.275393681554515,0.301516346360106,0.325694808867796,0.349380832626729,
0.372569385322311,0.39526561126473,0.417542958448358,0.439097284383825,
0.460279539328191,0.480970726129676,0.484374999999241,0.492187499999257,
0.496093749999266,0.49804687499927,0.498929468578901,0.499023437499272,
0.499511718749273,0.499755859374274,0.499999999999275,0.59423884968362,
0.624999999999407,0.687499999999472,0.695312499999481,0.699218749999488,
0.701653256213793,0.703124999999495,0.726683948276255,0.797244553124197,
0.842069531816328,0.843749999999701,0.848842741410648,0.851562499999713,
0.865178344045717,0.879352508034244,0.892721009175091,0.905807159789695,
0.918394647030647,0.921874999999826,0.923828124999829,0.924804687499831,
0.925710282042496,0.925781249999833,0.929687499999842,0.93749999999986,
0.946187537924857,0.955080632973159,0.964250861328642,0.96874999999993,
0.978194147563431,0.987711388645982,0.997278309392134,1.),.UNSPECIFIED.);
#29979=B_SPLINE_CURVE_WITH_KNOTS('',3,(#150619,#150620,#150621,#150622,
#150623,#150624,#150625,#150626,#150627,#150628,#150629,#150630,#150631,
#150632,#150633,#150634,#150635,#150636,#150637,#150638,#150639,#150640,
#150641,#150642,#150643,#150644,#150645,#150646,#150647,#150648,#150649,
#150650,#150651,#150652,#150653,#150654,#150655,#150656,#150657,#150658,
#150659,#150660,#150661,#150662,#150663,#150664,#150665,#150666,#150667,
#150668,#150669,#150670,#150671,#150672,#150673,#150674,#150675,#150676,
#150677,#150678,#150679,#150680,#150681,#150682,#150683,#150684,#150685,
#150686,#150687,#150688),.UNSPECIFIED.,.F.,.F.,(4,3,3,3,3,3,3,3,3,3,3,3,
3,3,3,3,3,3,3,3,3,3,3,4),(0.,0.0530717197273206,0.105975615459485,0.125000000000379,
0.184023522900716,0.242174112607182,0.250000000000761,0.300351902020698,
0.351923554506319,0.375000000001143,0.427734152108808,0.43750000000133,
0.468750000001425,0.484375000001472,0.492187500001492,0.496093750001495,
0.498046875001492,0.500000000001488,0.585242141687435,0.672616116979766,
0.763559607395129,0.856696459690941,0.95329701090269,1.),.UNSPECIFIED.);
#29980=B_SPLINE_CURVE_WITH_KNOTS('',3,(#150707,#150708,#150709,#150710),
 .UNSPECIFIED.,.F.,.F.,(4,4),(0.,1.),.UNSPECIFIED.);
#29981=B_SPLINE_CURVE_WITH_KNOTS('',3,(#150804,#150805,#150806,#150807,
#150808,#150809,#150810,#150811,#150812,#150813),.UNSPECIFIED.,.F.,.F.,
(4,2,2,2,4),(6.05089101874855E-5,0.409283590266413,0.822960520941385,1.23673775115811,
1.64591231877855),.UNSPECIFIED.);
#29982=B_SPLINE_CURVE_WITH_KNOTS('',3,(#150832,#150833,#150834,#150835),
 .UNSPECIFIED.,.F.,.F.,(4,4),(2.1150751113916E-14,1.),.UNSPECIFIED.);
#29983=B_SPLINE_CURVE_WITH_KNOTS('',3,(#150854,#150855,#150856,#150857,
#150858,#150859,#150860,#150861,#150862,#150863,#150864,#150865,#150866,
#150867,#150868,#150869,#150870,#150871,#150872,#150873,#150874,#150875,
#150876,#150877,#150878,#150879,#150880,#150881,#150882,#150883,#150884,
#150885,#150886,#150887,#150888,#150889,#150890),.UNSPECIFIED.,.F.,.F.,
(4,3,3,3,3,3,3,3,3,3,3,3,4),(3.61916304046134E-14,0.0930574396876964,0.185648309493891,
0.277308890382779,0.3682969898436,0.458123321944239,0.5,0.588079575907268,
0.674990027831864,0.760014342027675,0.843958727689798,0.92614995473359,
1.),.UNSPECIFIED.);
#29984=B_SPLINE_CURVE_WITH_KNOTS('',3,(#150956,#150957,#150958,#150959,
#150960,#150961,#150962,#150963,#150964,#150965,#150966,#150967,#150968,
#150969,#150970,#150971,#150972,#150973,#150974,#150975,#150976,#150977,
#150978,#150979,#150980,#150981,#150982,#150983,#150984,#150985,#150986,
#150987,#150988,#150989,#150990,#150991,#150992,#150993,#150994,#150995,
#150996,#150997,#150998,#150999,#151000,#151001,#151002,#151003,#151004,
#151005,#151006,#151007,#151008,#151009,#151010,#151011,#151012,#151013,
#151014,#151015,#151016,#151017,#151018,#151019,#151020,#151021,#151022,
#151023,#151024,#151025,#151026,#151027,#151028,#151029,#151030,#151031,
#151032,#151033,#151034,#151035,#151036,#151037,#151038,#151039,#151040,
#151041,#151042,#151043,#151044,#151045,#151046,#151047,#151048,#151049,
#151050,#151051,#151052,#151053,#151054,#151055,#151056,#151057,#151058,
#151059,#151060,#151061,#151062,#151063,#151064,#151065,#151066,#151067,
#151068,#151069,#151070,#151071,#151072,#151073,#151074,#151075,#151076,
#151077,#151078,#151079,#151080,#151081,#151082,#151083,#151084,#151085,
#151086,#151087,#151088,#151089,#151090,#151091,#151092,#151093,#151094,
#151095,#151096,#151097,#151098,#151099,#151100,#151101,#151102,#151103,
#151104,#151105,#151106,#151107,#151108,#151109,#151110,#151111,#151112,
#151113,#151114,#151115,#151116,#151117,#151118,#151119,#151120,#151121,
#151122,#151123,#151124,#151125,#151126,#151127,#151128,#151129,#151130,
#151131,#151132,#151133,#151134,#151135,#151136,#151137,#151138,#151139,
#151140,#151141,#151142,#151143,#151144,#151145),.UNSPECIFIED.,.F.,.F.,
(4,3,3,3,3,3,3,3,3,3,3,3,3,3,3,3,3,3,3,3,3,3,3,3,3,3,3,3,3,3,3,3,3,3,3,
3,3,3,3,3,3,3,3,3,3,3,3,3,3,3,3,3,3,3,3,3,3,3,3,3,3,3,3,4),(0.,0.0325663099035258,
0.0652395425604615,0.0979584972904591,0.12500000000312,0.14062500000351,
0.14257812500356,0.144377797408,0.144531250003609,0.148437500003707,0.156250000003902,
0.18750000000468,0.22917857178013,0.250000000006234,0.281250000007011,0.285156250007108,
0.285644531257119,0.28613281250713,0.287109375007128,0.289062500007128,
0.296875000007075,0.312500000006967,0.336074545596588,0.359628477597324,
0.375000000006548,0.398483031103689,0.421881190495673,0.437500000006129,
0.460689275266742,0.468750000005918,0.484375000005812,0.492187500005759,
0.496093750005733,0.49804687500572,0.500000000005706,0.553525722250135,
0.607023016338207,0.625000000004783,0.67752177447689,0.687500000004321,
0.718750000004092,0.734375000003977,0.74218750000392,0.749511718753869,
0.750000000003866,0.765625000003613,0.78074405805616,0.796622029029507,
0.812500000002854,0.828125000002601,0.843750000002347,0.858514060610061,
0.859375000002094,0.867187500001968,0.871093750001905,0.873046875001874,
0.874023437501859,0.875000000001845,0.897607080129362,0.920471072300298,
0.937500000000922,0.96050752485429,0.983627731922649,1.),.UNSPECIFIED.);
#29985=B_SPLINE_CURVE_WITH_KNOTS('',3,(#151164,#151165,#151166,#151167,
#151168,#151169,#151170,#151171,#151172,#151173,#151174,#151175,#151176,
#151177,#151178,#151179,#151180,#151181,#151182,#151183,#151184,#151185,
#151186,#151187,#151188,#151189,#151190,#151191,#151192,#151193,#151194,
#151195,#151196,#151197,#151198,#151199,#151200,#151201,#151202,#151203,
#151204,#151205,#151206,#151207,#151208,#151209,#151210,#151211,#151212,
#151213,#151214,#151215,#151216,#151217,#151218,#151219,#151220,#151221,
#151222,#151223,#151224),.UNSPECIFIED.,.F.,.F.,(4,3,3,3,3,3,3,3,3,3,3,3,
3,3,3,3,3,3,3,3,4),(0.,0.190753989572696,0.249999999999875,0.374999999999816,
0.437499999999784,0.468749999999765,0.484374999999756,0.492187499999754,
0.499999999999751,0.569019421689051,0.636642444566116,0.702132614905151,
0.749999999999842,0.78124999999985,0.785156249999851,0.789062499999853,
0.796874999999853,0.81249999999986,0.874999999999903,0.976210201063579,
1.),.UNSPECIFIED.);
#29986=B_SPLINE_CURVE_WITH_KNOTS('',3,(#151331,#151332,#151333,#151334,
#151335,#151336,#151337,#151338,#151339,#151340,#151341,#151342,#151343,
#151344,#151345),.UNSPECIFIED.,.F.,.F.,(4,1,1,1,1,1,1,1,1,1,1,1,4),(0.,
0.125000000000091,0.187500000000107,0.250000000000123,0.312500000000139,
0.375000000000156,0.437500000000172,0.500000000000188,0.562500000000204,
0.62500000000022,0.750000000000253,0.875000000000285,1.),.UNSPECIFIED.);
#29987=B_SPLINE_CURVE_WITH_KNOTS('',3,(#151368,#151369,#151370,#151371,
#151372,#151373,#151374,#151375,#151376,#151377,#151378,#151379,#151380,
#151381,#151382,#151383,#151384,#151385,#151386,#151387,#151388,#151389,
#151390,#151391,#151392,#151393,#151394,#151395,#151396,#151397,#151398,
#151399,#151400,#151401,#151402,#151403,#151404,#151405,#151406,#151407,
#151408,#151409,#151410,#151411,#151412,#151413,#151414,#151415,#151416,
#151417,#151418,#151419,#151420,#151421,#151422,#151423,#151424,#151425,
#151426,#151427,#151428,#151429,#151430,#151431,#151432,#151433,#151434,
#151435,#151436,#151437,#151438,#151439,#151440,#151441,#151442,#151443,
#151444,#151445,#151446,#151447,#151448,#151449,#151450,#151451,#151452,
#151453,#151454,#151455,#151456,#151457,#151458,#151459,#151460,#151461,
#151462,#151463,#151464,#151465,#151466,#151467),.UNSPECIFIED.,.F.,.F.,
(4,3,3,3,3,3,3,3,3,3,3,3,3,3,3,3,3,3,3,3,3,3,3,3,3,3,3,3,3,3,3,3,3,4),(0.,
0.0386486109998501,0.0777867154540601,0.117663230486258,0.157951378049023,
0.198841740487247,0.218749999999743,0.234374999999724,0.242187499999713,
0.246093749999708,0.249023437499706,0.249999999999706,0.298141994905816,
0.346774720025382,0.396229275286474,0.437499999999819,0.468749999999837,
0.484374999999846,0.492187499999852,0.496093749999854,0.498046874999855,
0.499999999999857,0.552515324753874,0.605587467781269,0.66122185083594,
0.715745966306094,0.771935483153023,0.828124999999952,0.835937499999954,
0.843749999999957,0.874999999999965,0.93110858870555,0.988008673189029,
1.),.UNSPECIFIED.);
#29988=B_SPLINE_CURVE_WITH_KNOTS('',3,(#151567,#151568,#151569,#151570,
#151571,#151572,#151573,#151574,#151575,#151576,#151577),.UNSPECIFIED.,
 .F.,.F.,(4,1,1,1,1,1,1,1,4),(0.,0.1245291089182,0.2495963790728,0.3746636492273,
0.4997309193818,0.6247981895364,0.7498654596909,0.8749327298455,1.),
 .UNSPECIFIED.);
#29989=B_SPLINE_CURVE_WITH_KNOTS('',3,(#151578,#151579,#151580,#151581,
#151582,#151583,#151584,#151585,#151586,#151587,#151588,#151589,#151590,
#151591,#151592,#151593,#151594,#151595,#151596,#151597,#151598,#151599,
#151600,#151601,#151602,#151603,#151604,#151605,#151606,#151607,#151608,
#151609,#151610,#151611,#151612,#151613,#151614,#151615,#151616,#151617,
#151618,#151619,#151620,#151621,#151622,#151623,#151624,#151625,#151626,
#151627,#151628,#151629,#151630,#151631,#151632,#151633,#151634,#151635),
 .UNSPECIFIED.,.F.,.F.,(4,3,3,3,3,3,3,3,3,3,3,3,3,3,3,3,3,3,3,4),(0.,0.115952588797155,
0.124516431282423,0.235365088827962,0.249596230510871,0.249941321206761,
0.338919844563841,0.37465645055649,0.462274221309376,0.49973067485326,0.500093646297469,
0.587781056470055,0.624805668103668,0.713861152125916,0.749865296158966,
0.750245971388176,0.861850585209343,0.874945606912365,0.991723863510178,
1.),.UNSPECIFIED.);
#29990=B_SPLINE_CURVE_WITH_KNOTS('',3,(#151703,#151704,#151705,#151706,
#151707,#151708,#151709,#151710,#151711,#151712,#151713,#151714,#151715,
#151716,#151717,#151718,#151719,#151720,#151721,#151722,#151723,#151724,
#151725,#151726,#151727,#151728,#151729,#151730,#151731,#151732,#151733,
#151734,#151735,#151736,#151737,#151738,#151739,#151740,#151741,#151742,
#151743,#151744,#151745,#151746,#151747,#151748,#151749,#151750,#151751,
#151752,#151753,#151754,#151755,#151756,#151757,#151758,#151759,#151760,
#151761,#151762,#151763,#151764,#151765,#151766,#151767,#151768,#151769,
#151770,#151771,#151772,#151773,#151774,#151775,#151776,#151777,#151778),
 .UNSPECIFIED.,.F.,.F.,(4,3,3,3,3,3,3,3,3,3,3,3,3,3,3,3,3,3,3,3,3,3,3,3,
3,4),(0.,0.0564989974727729,0.112185881107388,0.167214689987301,0.221006398970003,
0.249999999999978,0.302086836977158,0.35259446820029,0.374999999999967,
0.423333605828074,0.437499999999961,0.468749999999959,0.484374999999957,
0.492187499999956,0.49936885374005,0.499999999999955,0.551387355728607,
0.604385896613103,0.658323980269711,0.713760631639018,0.749999999999977,
0.805263132233714,0.862599288093799,0.921043602076914,0.980820544657335,
1.),.UNSPECIFIED.);
#29991=B_SPLINE_CURVE_WITH_KNOTS('',3,(#151779,#151780,#151781,#151782,
#151783,#151784,#151785,#151786,#151787,#151788,#151789,#151790,#151791,
#151792,#151793,#151794,#151795,#151796,#151797,#151798,#151799,#151800,
#151801,#151802,#151803),.UNSPECIFIED.,.F.,.F.,(4,3,3,3,3,3,3,3,4),(1.08860685774249E-9,
0.125010000617742,0.249999999999999,0.374999999999999,0.499999999999999,
0.624999999999999,0.749999999999999,0.875005695145605,1.),.UNSPECIFIED.);
#29992=B_SPLINE_CURVE_WITH_KNOTS('',3,(#151882,#151883,#151884,#151885,
#151886,#151887,#151888,#151889),.UNSPECIFIED.,.F.,.F.,(4,2,2,4),(0.,0.5,
0.75,1.),.UNSPECIFIED.);
#29993=B_SPLINE_CURVE_WITH_KNOTS('',3,(#151890,#151891,#151892,#151893,
#151894,#151895,#151896,#151897,#151898,#151899,#151900,#151901,#151902,
#151903,#151904,#151905,#151906,#151907),.UNSPECIFIED.,.F.,.F.,(4,2,1,1,
2,2,2,2,2,4),(0.,0.124999999999996,0.187499999999995,0.218749999999994,
0.234374999999993,0.249999999999993,0.374999999999995,0.437499999999996,
0.499999999999997,1.),.UNSPECIFIED.);
#29994=B_SPLINE_CURVE_WITH_KNOTS('',3,(#151908,#151909,#151910,#151911,
#151912,#151913,#151914,#151915,#151916,#151917,#151918,#151919,#151920,
#151921,#151922,#151923,#151924,#151925,#151926,#151927,#151928,#151929,
#151930,#151931,#151932),.UNSPECIFIED.,.F.,.F.,(4,3,3,3,3,3,3,3,4),(1.33819881907442E-9,
0.125001094910741,0.25,0.374998724065209,0.5,0.624998829992135,0.75,0.87499945771442,
1.),.UNSPECIFIED.);
#29995=B_SPLINE_CURVE_WITH_KNOTS('',3,(#151949,#151950,#151951,#151952),
 .UNSPECIFIED.,.F.,.F.,(4,4),(2.56540938759315E-6,0.999999991294677),
 .UNSPECIFIED.);
#29996=B_SPLINE_CURVE_WITH_KNOTS('',3,(#152184,#152185,#152186,#152187,
#152188,#152189,#152190,#152191,#152192,#152193,#152194,#152195,#152196,
#152197,#152198,#152199,#152200,#152201,#152202,#152203,#152204,#152205,
#152206,#152207,#152208,#152209,#152210,#152211,#152212,#152213,#152214,
#152215,#152216,#152217,#152218),.UNSPECIFIED.,.F.,.F.,(4,2,2,2,1,1,2,2,
2,2,2,2,2,1,1,1,2,2,2,4),(0.,0.124999999999998,0.187499999999997,0.218749999999997,
0.234374999999997,0.242187499999997,0.246093749999997,0.249999999999997,
0.374999999999998,0.437499999999998,0.499999999999999,0.625,0.6875,0.71875,
0.734375000000001,0.742187500000001,0.746093750000001,0.750000000000001,
0.875,1.),.UNSPECIFIED.);
#29997=B_SPLINE_CURVE_WITH_KNOTS('',3,(#152220,#152221,#152222,#152223,
#152224,#152225,#152226,#152227,#152228,#152229,#152230,#152231,#152232,
#152233,#152234,#152235,#152236,#152237,#152238,#152239,#152240,#152241,
#152242,#152243,#152244,#152245,#152246,#152247,#152248,#152249,#152250,
#152251,#152252,#152253,#152254,#152255,#152256,#152257,#152258,#152259,
#152260,#152261,#152262,#152263,#152264,#152265,#152266,#152267,#152268,
#152269,#152270,#152271,#152272,#152273,#152274,#152275,#152276,#152277,
#152278,#152279,#152280,#152281,#152282,#152283,#152284,#152285,#152286,
#152287,#152288,#152289,#152290,#152291,#152292,#152293,#152294,#152295,
#152296,#152297,#152298,#152299,#152300,#152301,#152302,#152303,#152304,
#152305,#152306,#152307,#152308,#152309,#152310,#152311,#152312,#152313,
#152314,#152315,#152316,#152317,#152318,#152319,#152320,#152321,#152322,
#152323,#152324),.UNSPECIFIED.,.F.,.F.,(4,2,2,2,2,2,2,1,2,2,2,2,2,2,2,2,
2,1,1,1,1,2,2,2,2,2,2,2,1,1,1,2,2,2,2,2,1,2,2,1,1,1,2,2,2,1,2,2,1,1,2,2,
2,2,2,1,2,2,1,1,1,4),(7.72626726236311E-7,0.031249999999956,0.062499999999912,
0.0937499999998679,0.109374999999846,0.117187499999835,0.121093749999829,
0.123046874999827,0.124023437499825,0.124999999999824,0.140624999999802,
0.15624999999978,0.171874999999758,0.187499999999736,0.218749999999693,
0.234374999999671,0.24218749999966,0.246093749999654,0.248046874999652,
0.24902343749965,0.24951171874965,0.249938964843399,0.249999999999649,0.281249999999659,
0.312499999999668,0.32031249999967,0.321289062499671,0.321533203124671,
0.321777343749671,0.322265624999671,0.324218749999673,0.328124999999677,
0.343749999999693,0.351562499999701,0.355468749999705,0.357421874999707,
0.359374999999709,0.367187499999717,0.371093749999721,0.373046874999723,
0.374023437499724,0.374511718749724,0.374938964843474,0.374999999999724,
0.390624999999737,0.392578124999738,0.392822265624738,0.393066406249738,
0.393554687499739,0.394531249999739,0.398437499999742,0.406249999999746,
0.421874999999755,0.437499999999764,0.453124999999773,0.453613281249774,
0.453979492187274,0.454101562499774,0.455078124999775,0.457031249999776,
0.460937499999778,0.465501376528164),.UNSPECIFIED.);
#29998=B_SPLINE_CURVE_WITH_KNOTS('',3,(#152325,#152326,#152327,#152328,
#152329,#152330,#152331,#152332,#152333,#152334,#152335,#152336,#152337,
#152338,#152339,#152340,#152341,#152342,#152343,#152344,#152345,#152346,
#152347,#152348,#152349,#152350,#152351,#152352,#152353,#152354,#152355,
#152356,#152357,#152358,#152359,#152360,#152361,#152362,#152363,#152364,
#152365,#152366,#152367,#152368,#152369,#152370,#152371,#152372,#152373,
#152374,#152375,#152376,#152377,#152378,#152379,#152380,#152381,#152382,
#152383,#152384,#152385,#152386,#152387,#152388,#152389,#152390,#152391,
#152392,#152393,#152394,#152395,#152396,#152397,#152398,#152399,#152400,
#152401,#152402,#152403,#152404,#152405,#152406,#152407,#152408,#152409,
#152410,#152411,#152412,#152413,#152414,#152415,#152416,#152417,#152418,
#152419,#152420,#152421,#152422,#152423,#152424,#152425,#152426,#152427,
#152428,#152429),.UNSPECIFIED.,.F.,.F.,(4,2,2,2,1,1,1,1,2,2,2,2,2,2,2,1,
1,1,2,2,2,2,2,1,2,2,1,2,2,2,2,2,2,2,2,2,2,2,1,1,2,2,2,2,1,1,1,1,2,2,2,2,
2,2,2,1,1,2,2,2,4),(0.465501376528164,0.468749999999783,0.484374999999792,
0.492187499999797,0.496093749999799,0.4980468749998,0.499023437499801,0.499511718749801,
0.499938964843552,0.499999999999802,0.515624999999806,0.531249999999811,
0.535156249999812,0.535644531249812,0.536132812499813,0.537109374999813,
0.539062499999813,0.546874999999816,0.562499999999821,0.570312499999824,
0.574218749999825,0.578124999999826,0.585937499999829,0.58789062499983,
0.58886718749983,0.58935546874983,0.58984374999983,0.593749999999831,0.601562499999834,
0.605468749999835,0.606445312499835,0.607421874999835,0.609374999999836,
0.62499999999984,0.640624999999843,0.642578124999844,0.642822265624844,
0.643066406249844,0.643554687499844,0.644531249999845,0.648437499999847,
0.65624999999985,0.687499999999867,0.718749999999883,0.734374999999891,
0.742187499999895,0.746093749999897,0.748046874999898,0.749511718749899,
0.749999999999899,0.781249999999915,0.812499999999931,0.843749999999946,
0.859374999999954,0.867187499999958,0.87109374999996,0.873046874999961,
0.874938964843712,0.874999999999962,0.937499999999981,0.999999692106287),
 .UNSPECIFIED.);
#29999=B_SPLINE_CURVE_WITH_KNOTS('',3,(#152431,#152432,#152433,#152434),
 .UNSPECIFIED.,.F.,.F.,(4,4),(6.46566861907642E-9,0.999998547516504),
 .UNSPECIFIED.);
#30000=B_SPLINE_CURVE_WITH_KNOTS('',3,(#152435,#152436,#152437,#152438,
#152439,#152440,#152441,#152442),.UNSPECIFIED.,.F.,.F.,(4,2,2,4),(0.,0.25,
0.5,1.),.UNSPECIFIED.);
#30001=B_SPLINE_CURVE_WITH_KNOTS('',3,(#152663,#152664,#152665,#152666,
#152667,#152668,#152669,#152670,#152671,#152672,#152673),.UNSPECIFIED.,
 .F.,.F.,(4,1,1,1,1,1,1,1,4),(0.,0.125,0.25,0.375,0.5,0.625,0.75,0.875,
1.),.UNSPECIFIED.);
#30002=B_SPLINE_CURVE_WITH_KNOTS('',3,(#152784,#152785,#152786,#152787,
#152788,#152789,#152790,#152791,#152792,#152793,#152794,#152795,#152796,
#152797,#152798,#152799,#152800,#152801,#152802,#152803,#152804,#152805,
#152806,#152807,#152808,#152809,#152810,#152811,#152812,#152813,#152814,
#152815,#152816,#152817,#152818,#152819,#152820,#152821,#152822,#152823,
#152824,#152825,#152826,#152827,#152828,#152829,#152830,#152831,#152832,
#152833,#152834,#152835,#152836,#152837,#152838,#152839,#152840,#152841),
 .UNSPECIFIED.,.F.,.F.,(4,3,3,3,3,3,3,3,3,3,3,3,3,3,3,3,3,3,3,4),(0.,0.067608122116081,
0.124556588133259,0.193621577458384,0.249619932699945,0.249837494557552,
0.324680401583297,0.37468327726673,0.471469027662659,0.499746621833416,
0.499948939665128,0.596293297167373,0.624809966400102,0.699690355925683,
0.749873310966788,0.750060380763928,0.818979536087593,0.874936655533574,
0.942644019861922,1.),.UNSPECIFIED.);
#30003=B_SPLINE_CURVE_WITH_KNOTS('',3,(#152842,#152843,#152844,#152845,
#152846,#152847,#152848,#152849,#152850,#152851,#152852,#152853,#152854,
#152855,#152856,#152857,#152858,#152859,#152860,#152861,#152862,#152863,
#152864,#152865,#152866,#152867,#152868,#152869,#152870,#152871,#152872,
#152873,#152874,#152875,#152876,#152877,#152878,#152879,#152880,#152881,
#152882),.UNSPECIFIED.,.F.,.F.,(4,2,2,1,1,1,2,2,2,2,1,1,1,1,2,2,2,2,1,1,
1,1,2,2,2,4),(0.,0.125000000000034,0.187500000000051,0.218750000000059,
0.234375000000063,0.242187500000065,0.246093750000066,0.250000000000068,
0.375000000000105,0.437500000000124,0.468750000000133,0.484375000000137,
0.492187500000139,0.49609375000014,0.498046875000141,0.500000000000143,
0.625000000000156,0.687500000000162,0.718750000000165,0.734375000000166,
0.742187500000166,0.746093750000167,0.749023437500166,0.750000000000166,
0.875000000000083,1.),.UNSPECIFIED.);
#30004=B_SPLINE_CURVE_WITH_KNOTS('',3,(#152888,#152889,#152890,#152891,
#152892,#152893,#152894,#152895,#152896,#152897,#152898,#152899,#152900,
#152901,#152902,#152903,#152904,#152905,#152906,#152907,#152908,#152909,
#152910,#152911,#152912,#152913,#152914,#152915,#152916,#152917,#152918,
#152919,#152920,#152921,#152922,#152923,#152924,#152925,#152926,#152927,
#152928,#152929,#152930,#152931,#152932,#152933,#152934,#152935,#152936,
#152937,#152938,#152939,#152940,#152941,#152942,#152943,#152944,#152945,
#152946,#152947,#152948,#152949,#152950,#152951,#152952,#152953,#152954,
#152955,#152956,#152957,#152958,#152959,#152960,#152961,#152962,#152963,
#152964,#152965,#152966),.UNSPECIFIED.,.F.,.F.,(4,3,3,3,3,3,3,3,3,3,3,3,
3,3,3,3,3,3,3,3,3,3,3,3,3,3,4),(1.59010835072902E-15,0.0624999999999996,
0.121020838093803,0.178392295984127,0.233986563636919,0.249999999999994,
0.305023024426928,0.358470295259852,0.37499999999999,0.427815351538303,
0.437499999999989,0.468749999999989,0.48437499999999,0.492187499999991,
0.499429264202313,0.499999999999991,0.546752076236196,0.594486765223972,
0.643796040196902,0.694112041083609,0.745881187044065,0.749999999999996,
0.803525367030386,0.858545471985278,0.914246979722377,0.970685664969118,
1.),.UNSPECIFIED.);
#30005=B_SPLINE_CURVE_WITH_KNOTS('',3,(#152967,#152968,#152969,#152970,
#152971,#152972,#152973,#152974,#152975,#152976,#152977,#152978,#152979,
#152980,#152981,#152982,#152983,#152984,#152985,#152986,#152987,#152988,
#152989,#152990,#152991,#152992,#152993,#152994,#152995,#152996,#152997,
#152998,#152999,#153000,#153001,#153002,#153003,#153004,#153005,#153006,
#153007,#153008,#153009,#153010,#153011,#153012,#153013,#153014,#153015,
#153016,#153017,#153018,#153019,#153020,#153021,#153022,#153023,#153024,
#153025,#153026,#153027,#153028,#153029,#153030,#153031,#153032,#153033,
#153034,#153035,#153036,#153037,#153038,#153039,#153040,#153041,#153042,
#153043,#153044,#153045,#153046,#153047,#153048,#153049,#153050,#153051,
#153052,#153053,#153054,#153055,#153056,#153057,#153058,#153059,#153060,
#153061,#153062,#153063),.UNSPECIFIED.,.F.,.F.,(4,3,3,3,3,3,3,3,3,3,3,3,
3,3,3,3,3,3,3,3,3,3,3,3,3,3,3,3,3,3,3,3,4),(0.,0.031249999999975,0.0607010736965204,
0.0897270673465461,0.118195311223028,0.1249999999999,0.15207935224579,0.178485600985883,
0.18749999999985,0.21311147226121,0.218749999999824,0.234374999999812,0.242187499999805,
0.246093749999802,0.248046874999801,0.2490234374998,0.249511718749799,0.249999999999799,
0.335458392498475,0.374999999999826,0.43749999999984,0.468749999999847,
0.48437499999985,0.492187499999852,0.499471027976032,0.499999999999853,
0.582099180943044,0.666049590471485,0.749999999999927,0.825751814325505,
0.90133264277272,0.976826393250221,1.),.UNSPECIFIED.);
#30006=B_SPLINE_CURVE_WITH_KNOTS('',3,(#153127,#153128,#153129,#153130,
#153131,#153132,#153133,#153134,#153135,#153136,#153137,#153138,#153139,
#153140,#153141,#153142,#153143,#153144,#153145,#153146,#153147,#153148,
#153149,#153150,#153151,#153152,#153153,#153154),.UNSPECIFIED.,.F.,.F.,
(4,3,3,3,3,3,3,3,3,4),(9.89807669334734E-10,0.232893555433494,0.25,0.250189537138593,
0.375284087663041,0.5,0.50037833656381,0.625472138461813,0.750565940359238,
1.),.UNSPECIFIED.);
#30007=B_SPLINE_CURVE_WITH_KNOTS('',3,(#153155,#153156,#153157,#153158,
#153159,#153160,#153161,#153162,#153163,#153164,#153165,#153166,#153167,
#153168),.UNSPECIFIED.,.F.,.F.,(4,2,2,2,2,2,4),(0.,0.250000000000001,0.375000000000001,
0.500000000000001,0.625000000000001,0.75,1.),.UNSPECIFIED.);
#30008=B_SPLINE_CURVE_WITH_KNOTS('',3,(#153282,#153283,#153284,#153285),
 .UNSPECIFIED.,.F.,.F.,(4,4),(0.,1.),.UNSPECIFIED.);
#30009=B_SPLINE_CURVE_WITH_KNOTS('',3,(#153286,#153287,#153288,#153289,
#153290,#153291,#153292,#153293,#153294,#153295,#153296,#153297,#153298,
#153299,#153300,#153301,#153302,#153303,#153304,#153305,#153306,#153307,
#153308,#153309,#153310,#153311,#153312,#153313,#153314,#153315,#153316,
#153317,#153318,#153319,#153320,#153321,#153322,#153323,#153324,#153325,
#153326,#153327,#153328,#153329,#153330,#153331,#153332,#153333,#153334,
#153335,#153336,#153337,#153338,#153339,#153340,#153341,#153342,#153343,
#153344,#153345,#153346,#153347,#153348,#153349,#153350,#153351,#153352,
#153353,#153354,#153355,#153356,#153357,#153358),.UNSPECIFIED.,.F.,.F.,
(4,3,3,3,3,3,3,3,3,3,3,3,3,3,3,3,3,3,3,3,3,3,3,3,4),(0.,0.0444154464726,
0.088382210368451,0.131763087129373,0.174838624328436,0.217515042786487,
0.249939927815387,0.291563369073533,0.332989920633538,0.37473289612189,
0.415853341206836,0.45790758189689,0.499961822586944,0.540995736379099,
0.582060349521465,0.624041191480699,0.665355026237124,0.707669371797763,
0.749983717358402,0.792598675882721,0.835493364945415,0.878917478176752,
0.92265717931407,0.966982523655085,1.),.UNSPECIFIED.);
#30010=B_SPLINE_CURVE_WITH_KNOTS('',3,(#153444,#153445,#153446,#153447,
#153448,#153449,#153450,#153451,#153452,#153453,#153454,#153455,#153456,
#153457,#153458,#153459,#153460,#153461,#153462,#153463,#153464,#153465,
#153466,#153467,#153468,#153469,#153470,#153471,#153472,#153473,#153474,
#153475,#153476,#153477,#153478,#153479,#153480,#153481,#153482,#153483,
#153484,#153485,#153486,#153487,#153488,#153489,#153490,#153491,#153492,
#153493,#153494,#153495,#153496,#153497,#153498,#153499,#153500,#153501,
#153502,#153503,#153504,#153505,#153506,#153507,#153508,#153509,#153510,
#153511,#153512,#153513,#153514,#153515,#153516,#153517,#153518,#153519,
#153520,#153521,#153522,#153523,#153524,#153525,#153526,#153527,#153528,
#153529,#153530,#153531,#153532,#153533,#153534,#153535,#153536,#153537,
#153538,#153539,#153540,#153541,#153542,#153543,#153544,#153545,#153546,
#153547,#153548,#153549,#153550,#153551,#153552,#153553,#153554,#153555,
#153556,#153557,#153558,#153559,#153560,#153561,#153562,#153563,#153564,
#153565,#153566,#153567,#153568,#153569,#153570,#153571,#153572,#153573,
#153574,#153575,#153576,#153577,#153578,#153579,#153580,#153581,#153582,
#153583,#153584,#153585,#153586,#153587,#153588,#153589,#153590,#153591,
#153592,#153593,#153594,#153595,#153596,#153597,#153598,#153599,#153600,
#153601,#153602,#153603,#153604,#153605,#153606,#153607,#153608,#153609,
#153610,#153611,#153612,#153613,#153614,#153615,#153616,#153617,#153618,
#153619,#153620,#153621,#153622,#153623,#153624,#153625,#153626,#153627,
#153628,#153629,#153630,#153631,#153632,#153633,#153634,#153635,#153636,
#153637,#153638,#153639,#153640,#153641,#153642,#153643,#153644,#153645,
#153646,#153647,#153648,#153649,#153650,#153651),.UNSPECIFIED.,.F.,.F.,
(4,3,3,3,3,3,3,3,3,3,3,3,3,3,3,3,3,3,3,3,3,3,3,3,3,3,3,3,3,3,3,3,3,3,3,
3,3,3,3,3,3,3,3,3,3,3,3,3,3,3,3,3,3,3,3,3,3,3,3,3,3,3,3,3,3,3,3,3,3,4),
(0.,0.0400589307361862,0.0797406453201286,0.118620801173798,0.125000000000011,
0.158233673552439,0.187500000000015,0.218750000000018,0.234375000000019,
0.24218750000002,0.24609375000002,0.249197866572958,0.25000000000002,0.274801018258469,
0.299154388956895,0.312500000000027,0.332141319272399,0.34375000000003,
0.359375000000031,0.367187500000032,0.371093750000032,0.373046875000033,
0.374023437500033,0.375000000000033,0.391246335883929,0.406278833684744,
0.413951005682541,0.430418756934123,0.437500000000032,0.453125000000031,
0.467852567759811,0.468750000000031,0.482935516148494,0.484375000000031,
0.493680329367665,0.499685418008973,0.50000000000003,0.512751122340329,
0.525998905586144,0.538496063904995,0.553131951474991,0.562500000000029,
0.578631755981225,0.585352841872323,0.593750000000029,0.609375000000029,
0.617187500000028,0.621093750000028,0.623046875000028,0.624023437500028,
0.625000000000028,0.643647435582588,0.662533544580982,0.68183911773363,
0.687500000000025,0.70072917260516,0.718750000000024,0.734375000000023,
0.742187500000022,0.746093750000022,0.749183103148108,0.750000000000021,
0.783169859588238,0.817376344468976,0.84161230871826,0.876448322903235,
0.911687871399364,0.94688403398269,0.981633629845859,1.),.UNSPECIFIED.);
#30011=B_SPLINE_CURVE_WITH_KNOTS('',3,(#153669,#153670,#153671,#153672),
 .UNSPECIFIED.,.F.,.F.,(4,4),(0.,1.),.UNSPECIFIED.);
#30012=B_SPLINE_CURVE_WITH_KNOTS('',3,(#153675,#153676,#153677,#153678,
#153679,#153680,#153681,#153682,#153683,#153684),.UNSPECIFIED.,.F.,.F.,
(4,3,3,4),(0.,0.355575480078952,0.708688526690115,1.),.UNSPECIFIED.);
#30013=B_SPLINE_CURVE_WITH_KNOTS('',3,(#153686,#153687,#153688,#153689,
#153690,#153691,#153692,#153693,#153694,#153695,#153696,#153697,#153698,
#153699,#153700,#153701,#153702,#153703,#153704,#153705,#153706,#153707,
#153708,#153709,#153710,#153711,#153712,#153713,#153714,#153715,#153716,
#153717,#153718,#153719,#153720,#153721,#153722,#153723,#153724,#153725,
#153726,#153727,#153728,#153729,#153730,#153731,#153732,#153733,#153734,
#153735,#153736,#153737,#153738,#153739,#153740,#153741,#153742,#153743,
#153744,#153745,#153746,#153747,#153748,#153749,#153750,#153751,#153752,
#153753,#153754,#153755,#153756,#153757,#153758,#153759,#153760,#153761,
#153762,#153763,#153764,#153765,#153766,#153767,#153768,#153769,#153770,
#153771,#153772,#153773,#153774,#153775,#153776,#153777,#153778,#153779,
#153780,#153781,#153782,#153783,#153784,#153785,#153786,#153787,#153788,
#153789,#153790,#153791,#153792,#153793,#153794,#153795,#153796,#153797,
#153798,#153799,#153800,#153801,#153802,#153803,#153804,#153805,#153806,
#153807,#153808,#153809,#153810,#153811,#153812,#153813,#153814,#153815,
#153816,#153817,#153818,#153819,#153820,#153821,#153822,#153823,#153824,
#153825,#153826,#153827,#153828,#153829,#153830,#153831,#153832,#153833,
#153834,#153835,#153836),.UNSPECIFIED.,.F.,.F.,(4,3,3,3,3,3,3,3,3,3,3,3,
3,3,3,3,3,3,3,3,3,3,3,3,3,3,3,3,3,3,3,3,3,3,3,3,3,3,3,3,3,3,3,3,3,3,3,3,
3,3,4),(0.,0.0266572530362359,0.0529474029428651,0.0625000000000029,0.0880857890087234,
0.0937500000000047,0.109375000000006,0.117187500000006,0.122072505131236,
0.124806686990945,0.125000000000006,0.150224861065753,0.175595927078806,
0.187142286124972,0.187500000000007,0.218750000000007,0.234375000000007,
0.242660532900981,0.250000000000007,0.282477540622239,0.313776512685994,
0.345310797249849,0.375000000000007,0.377013825968837,0.407760369476629,
0.438211040162093,0.469105520081049,0.500000000000006,0.532769453185549,
0.565934692720068,0.59970342888731,0.622796551583423,0.625000000000005,
0.656333797697557,0.687500000000005,0.718750000000005,0.734375000000005,
0.742187500000005,0.746093750000005,0.748046875000004,0.750000000000004,
0.776677040852684,0.804022779420661,0.83169633877836,0.859747497852255,
0.873068492291997,0.901180604984381,0.929428841358404,0.957620752845238,
0.98555271402396,1.),.UNSPECIFIED.);
#30014=B_SPLINE_CURVE_WITH_KNOTS('',3,(#153837,#153838,#153839,#153840,
#153841,#153842,#153843,#153844,#153845,#153846),.UNSPECIFIED.,.F.,.F.,
(4,3,3,4),(0.,0.371972328017731,0.745231674146774,1.),.UNSPECIFIED.);
#30015=B_SPLINE_CURVE_WITH_KNOTS('',3,(#153864,#153865,#153866,#153867,
#153868,#153869,#153870,#153871,#153872,#153873),.UNSPECIFIED.,.F.,.F.,
(4,2,2,2,4),(0.,0.25,0.5,0.75,1.),.UNSPECIFIED.);
#30016=B_SPLINE_CURVE_WITH_KNOTS('',3,(#153875,#153876,#153877,#153878,
#153879,#153880,#153881,#153882,#153883,#153884),.UNSPECIFIED.,.F.,.F.,
(4,3,3,4),(0.,0.341585033093189,0.68318654002556,1.),.UNSPECIFIED.);
#30017=B_SPLINE_CURVE_WITH_KNOTS('',3,(#153985,#153986,#153987,#153988,
#153989,#153990,#153991,#153992,#153993,#153994,#153995,#153996,#153997,
#153998,#153999,#154000,#154001,#154002,#154003,#154004,#154005,#154006,
#154007,#154008,#154009,#154010,#154011,#154012,#154013,#154014,#154015,
#154016,#154017,#154018,#154019,#154020,#154021,#154022,#154023,#154024,
#154025,#154026,#154027,#154028,#154029,#154030,#154031,#154032,#154033,
#154034,#154035,#154036,#154037,#154038,#154039,#154040,#154041,#154042,
#154043,#154044,#154045,#154046,#154047,#154048,#154049,#154050,#154051,
#154052,#154053,#154054,#154055,#154056,#154057,#154058,#154059,#154060,
#154061,#154062,#154063,#154064,#154065,#154066,#154067,#154068,#154069,
#154070,#154071,#154072,#154073,#154074,#154075,#154076,#154077,#154078,
#154079,#154080),.UNSPECIFIED.,.F.,.F.,(4,2,1,1,1,1,2,2,2,2,1,1,1,2,2,2,
1,1,1,1,2,2,2,2,1,1,1,2,2,2,2,2,1,1,1,2,2,2,2,1,1,1,1,2,2,2,2,1,1,1,1,2,
2,2,2,2,1,1,1,2,2,4),(0.,0.0624999999995465,0.0937499999993206,0.109374999999209,
0.117187499999153,0.121093749999124,0.123046874999109,0.124999999999095,
0.156249999998887,0.171874999998781,0.179687499998729,0.183593749998702,
0.185546874998689,0.186523437498682,0.187499999998676,0.218749999998446,
0.234374999998332,0.242187499998274,0.246093749998246,0.248046874998231,
0.249023437498222,0.249999999998212,0.312499999997693,0.343749999997435,
0.359374999997306,0.367187499997241,0.371093749997209,0.373046874997192,
0.374999999997174,0.499999999996056,0.562499999995497,0.593749999995218,
0.609374999995079,0.61718749999501,0.621093749994975,0.623046874994959,
0.624999999994943,0.687499999994446,0.718749999994198,0.734374999994075,
0.742187499994012,0.74609374999398,0.748046874993965,0.749023437493958,
0.749999999993951,0.812499999993504,0.843749999993281,0.859374999993169,
0.867187499993113,0.871093749993084,0.87304687499307,0.874755859368059,
0.874999999993057,0.906249999994804,0.921874999995676,0.929687499996112,
0.933593749996331,0.93554687499644,0.936523437496495,0.937011718746522,
0.93749999999655,1.),.UNSPECIFIED.);
#30018=B_SPLINE_CURVE_WITH_KNOTS('',3,(#154099,#154100,#154101,#154102,
#154103,#154104,#154105,#154106,#154107,#154108,#154109,#154110,#154111,
#154112,#154113,#154114,#154115),.UNSPECIFIED.,.F.,.F.,(4,2,2,2,1,1,1,2,
2,4),(0.,0.24999999999989,0.374999999999839,0.437499999999813,0.4687499999998,
0.484374999999796,0.492187499999792,0.496093749999792,0.499999999999793,
1.),.UNSPECIFIED.);
#30019=B_SPLINE_CURVE_WITH_KNOTS('',3,(#154118,#154119,#154120,#154121,
#154122,#154123,#154124,#154125,#154126,#154127),.UNSPECIFIED.,.F.,.F.,
(4,3,3,4),(6.77035784782114E-15,0.355575475820603,0.70868851966236,1.),
 .UNSPECIFIED.);
#30020=B_SPLINE_CURVE_WITH_KNOTS('',3,(#154129,#154130,#154131,#154132,
#154133,#154134,#154135,#154136,#154137,#154138,#154139,#154140,#154141,
#154142,#154143,#154144,#154145,#154146,#154147,#154148,#154149,#154150,
#154151,#154152,#154153,#154154,#154155,#154156,#154157,#154158,#154159,
#154160,#154161,#154162,#154163,#154164,#154165,#154166,#154167,#154168,
#154169,#154170,#154171,#154172,#154173,#154174,#154175,#154176,#154177),
 .UNSPECIFIED.,.F.,.F.,(4,3,3,3,3,3,3,3,3,3,3,3,3,3,3,3,4),(0.,0.0910455835011647,
0.182439138574727,0.250000000000011,0.339921904045264,0.375000000000017,
0.43750000000002,0.46875000000002,0.484375000000021,0.495831044563394,0.500000000000021,
0.5909385551545,0.681877417910837,0.772012506325215,0.861316606459104,0.948942207273129,
1.),.UNSPECIFIED.);
#30021=B_SPLINE_CURVE_WITH_KNOTS('',3,(#154195,#154196,#154197,#154198,
#154199,#154200),.UNSPECIFIED.,.F.,.F.,(4,2,4),(-0.606451718743048,-0.299493685602885,
-9.99999995198692E-7),.UNSPECIFIED.);
#30022=B_SPLINE_CURVE_WITH_KNOTS('',3,(#154223,#154224,#154225,#154226,
#154227,#154228),.UNSPECIFIED.,.F.,.F.,(4,2,4),(-0.372442319355049,-0.186223020487114,
-3.03100744253534E-6),.UNSPECIFIED.);
#30023=B_SPLINE_CURVE_WITH_KNOTS('',3,(#154229,#154230,#154231,#154232,
#154233),.UNSPECIFIED.,.F.,.F.,(4,1,4),(4.77483324436819E-6,0.503003588545041,
1.),.UNSPECIFIED.);
#30024=B_SPLINE_CURVE_WITH_KNOTS('',3,(#154251,#154252,#154253,#154254,
#154255,#154256),.UNSPECIFIED.,.F.,.F.,(4,2,4),(-0.3724515983366,-0.186230562103344,
-4.29627198925348E-6),.UNSPECIFIED.);
#30025=B_SPLINE_CURVE_WITH_KNOTS('',3,(#154257,#154258,#154259,#154260,
#154261,#154262,#154263,#154264,#154265,#154266,#154267,#154268,#154269,
#154270,#154271,#154272,#154273,#154274,#154275,#154276,#154277,#154278,
#154279,#154280,#154281,#154282,#154283,#154284,#154285,#154286,#154287,
#154288,#154289,#154290,#154291,#154292,#154293,#154294,#154295,#154296,
#154297,#154298,#154299,#154300,#154301,#154302,#154303,#154304,#154305,
#154306,#154307,#154308,#154309,#154310,#154311,#154312,#154313,#154314),
 .UNSPECIFIED.,.F.,.F.,(4,3,3,3,3,3,3,3,3,3,3,3,3,3,3,3,3,3,3,4),(2.72798627453737E-6,
0.0553540505734548,0.110169237189544,0.164514703027846,0.218455604332041,
0.272056050301599,0.325379106943922,0.378456718575932,0.431385880590234,
0.484247453423519,0.53709545654247,0.590321592406853,0.643381688533521,
0.696726047499516,0.75,0.803819714741727,0.858209994582057,0.912952977410288,
0.968345446498143,1.),.UNSPECIFIED.);
#30026=B_SPLINE_CURVE_WITH_KNOTS('',3,(#154332,#154333,#154334,#154335,
#154336,#154337),.UNSPECIFIED.,.F.,.F.,(4,2,4),(-0.608015977036257,-0.307733847198884,
-2.53573569086033E-6),.UNSPECIFIED.);
#30027=B_SPLINE_CURVE_WITH_KNOTS('',3,(#154340,#154341,#154342,#154343,
#154344,#154345,#154346,#154347,#154348,#154349,#154350,#154351,#154352,
#154353,#154354,#154355,#154356,#154357,#154358,#154359,#154360,#154361,
#154362,#154363,#154364,#154365,#154366,#154367,#154368,#154369,#154370,
#154371,#154372,#154373,#154374,#154375,#154376),.UNSPECIFIED.,.F.,.F.,
(4,3,3,3,3,3,3,3,3,3,3,3,4),(1.88907660345648E-10,0.0909364924096919,0.183637933662997,
0.278561470178532,0.37450130725563,0.471472916587379,0.5,0.597277769481169,
0.697958327110877,0.792495880377744,0.885613970721787,0.976356605035924,
1.),.UNSPECIFIED.);
#30028=B_SPLINE_CURVE_WITH_KNOTS('',3,(#154378,#154379,#154380,#154381,
#154382,#154383,#154384,#154385,#154386,#154387),.UNSPECIFIED.,.F.,.F.,
(4,3,3,4),(0.,0.371972324766811,0.745231666277941,0.999999999999995),
 .UNSPECIFIED.);
#30029=B_SPLINE_CURVE_WITH_KNOTS('',3,(#154405,#154406,#154407,#154408,
#154409,#154410,#154411,#154412,#154413,#154414),.UNSPECIFIED.,.F.,.F.,
(4,3,3,4),(0.,0.341585064612949,0.68318660305952,1.),.UNSPECIFIED.);
#30030=B_SPLINE_CURVE_WITH_KNOTS('',3,(#154515,#154516,#154517,#154518,
#154519,#154520,#154521,#154522,#154523,#154524,#154525,#154526,#154527,
#154528,#154529,#154530,#154531,#154532,#154533,#154534,#154535,#154536,
#154537,#154538,#154539,#154540,#154541,#154542,#154543,#154544,#154545,
#154546,#154547,#154548,#154549,#154550,#154551,#154552,#154553,#154554,
#154555,#154556,#154557,#154558,#154559,#154560,#154561,#154562,#154563,
#154564,#154565,#154566,#154567,#154568,#154569,#154570,#154571,#154572,
#154573,#154574,#154575,#154576,#154577,#154578,#154579,#154580,#154581,
#154582,#154583,#154584,#154585,#154586,#154587,#154588,#154589,#154590,
#154591,#154592,#154593,#154594,#154595,#154596,#154597,#154598,#154599,
#154600,#154601,#154602,#154603,#154604,#154605,#154606,#154607,#154608,
#154609,#154610),.UNSPECIFIED.,.F.,.F.,(4,2,1,1,1,1,2,2,2,2,1,1,1,2,2,2,
1,1,1,1,2,2,2,2,1,1,1,2,2,2,2,2,1,1,1,2,2,2,2,1,1,1,1,2,2,2,2,1,1,1,1,2,
2,2,2,2,1,1,1,2,2,4),(0.,0.0625000000001708,0.0937500000002552,0.109375000000297,
0.117187500000319,0.121093750000329,0.123046875000333,0.125000000000337,
0.156250000000383,0.171875000000407,0.179687500000418,0.183593750000423,
0.185546875000425,0.186523437500426,0.187500000000426,0.21875000000041,
0.234375000000404,0.2421875000004,0.2460937500004,0.248046875000401,0.249023437500402,
0.250000000000403,0.312500000000517,0.343750000000574,0.359375000000602,
0.367187500000616,0.371093750000624,0.373046875000628,0.375000000000633,
0.500000000001077,0.562500000001299,0.593750000001411,0.609375000001468,
0.617187500001496,0.621093750001509,0.623046875001517,0.625000000001525,
0.687500000001828,0.718750000001978,0.734375000002053,0.742187500002091,
0.746093750002109,0.748046875002119,0.749023437502122,0.750000000002126,
0.812500000002261,0.843750000002328,0.859375000002362,0.867187500002379,
0.871093750002388,0.873046875002393,0.874755859377398,0.875000000002398,
0.906250000001822,0.921875000001533,0.929687500001389,0.933593750001317,
0.935546875001281,0.936523437501262,0.937011718751253,0.937500000001243,
1.),.UNSPECIFIED.);
#30031=B_SPLINE_CURVE_WITH_KNOTS('',3,(#154629,#154630,#154631,#154632,
#154633,#154634,#154635,#154636,#154637,#154638,#154639,#154640,#154641,
#154642,#154643,#154644,#154645),.UNSPECIFIED.,.F.,.F.,(4,2,2,2,1,1,1,2,
2,4),(0.,0.249999999999954,0.374999999999937,0.437499999999928,0.468749999999923,
0.484374999999921,0.49218749999992,0.496093749999922,0.499999999999924,
1.),.UNSPECIFIED.);
#30032=B_SPLINE_CURVE_WITH_KNOTS('',3,(#154646,#154647,#154648,#154649,
#154650,#154651,#154652,#154653,#154654,#154655,#154656,#154657,#154658,
#154659,#154660,#154661,#154662,#154663,#154664,#154665,#154666,#154667,
#154668,#154669,#154670,#154671,#154672,#154673,#154674,#154675,#154676,
#154677,#154678,#154679,#154680,#154681,#154682,#154683,#154684,#154685,
#154686,#154687,#154688,#154689,#154690,#154691,#154692,#154693,#154694,
#154695,#154696,#154697,#154698,#154699,#154700,#154701,#154702,#154703,
#154704,#154705,#154706,#154707,#154708,#154709,#154710,#154711,#154712,
#154713,#154714,#154715),.UNSPECIFIED.,.F.,.F.,(4,3,3,3,3,3,3,3,3,3,3,3,
3,3,3,3,3,3,3,3,3,3,3,4),(0.,0.0497162850538284,0.0997854118434574,0.148349769878621,
0.19657310085876,0.244406250169066,0.249992792212344,0.296849141910662,
0.343480318803109,0.389891233648019,0.43620088824267,0.482450015571192,
0.499995230081589,0.5462432932865,0.592530815463781,0.638989031954228,0.685571564742959,
0.732423225621977,0.749997667950833,0.797873988738031,0.848405491553523,
0.897207740062206,0.948603870031103,1.),.UNSPECIFIED.);
#30033=B_SPLINE_CURVE_WITH_KNOTS('',3,(#154807,#154808,#154809,#154810,
#154811,#154812,#154813,#154814,#154815,#154816),.UNSPECIFIED.,.F.,.F.,
(4,2,2,2,4),(7.91321415605965E-5,0.461550908372518,0.883826720447071,1.3071784210996,
1.78873513688511),.UNSPECIFIED.);
#30034=B_SPLINE_CURVE_WITH_KNOTS('',3,(#154835,#154836,#154837,#154838,
#154839),.UNSPECIFIED.,.F.,.F.,(4,1,4),(1.32451275613523E-5,0.5,1.),
 .UNSPECIFIED.);
#30035=B_SPLINE_CURVE_WITH_KNOTS('',3,(#154841,#154842,#154843,#154844,
#154845,#154846,#154847,#154848,#154849,#154850,#154851,#154852,#154853,
#154854,#154855,#154856,#154857,#154858,#154859,#154860,#154861,#154862,
#154863,#154864,#154865,#154866,#154867,#154868,#154869,#154870,#154871,
#154872,#154873,#154874,#154875,#154876,#154877,#154878,#154879,#154880,
#154881,#154882,#154883,#154884,#154885,#154886,#154887,#154888,#154889,
#154890,#154891,#154892,#154893,#154894,#154895,#154896,#154897,#154898,
#154899,#154900,#154901,#154902,#154903,#154904,#154905,#154906,#154907,
#154908,#154909,#154910,#154911,#154912,#154913,#154914,#154915,#154916,
#154917,#154918,#154919,#154920,#154921,#154922,#154923,#154924,#154925,
#154926,#154927,#154928,#154929,#154930,#154931,#154932,#154933,#154934,
#154935,#154936,#154937,#154938,#154939,#154940,#154941,#154942,#154943,
#154944,#154945,#154946,#154947,#154948,#154949),.UNSPECIFIED.,.F.,.F.,
(4,3,3,3,3,3,3,3,3,3,3,3,3,3,3,3,3,3,3,3,3,3,3,3,3,3,3,3,3,3,3,3,3,3,3,
3,4),(2.73301476691168E-15,0.039441191303371,0.0768210354237637,0.11122288018331,
0.125,0.177992474343909,0.227481533149721,0.240547827143166,0.25,0.304443784156054,
0.357336706676159,0.369855256013052,0.375,0.40891821135081,0.442204853614617,
0.474505774150831,0.499217941560634,0.5,0.523587949419504,0.547077247101464,
0.57061197134477,0.594260887285262,0.618209766593177,0.625,0.628457488463763,
0.669404035577509,0.711444268396472,0.75,0.757882644294487,0.804582852109327,
0.852316895707969,0.875,0.887185081605594,0.920801047847144,0.955229129512886,
0.99089973413878,1.),.UNSPECIFIED.);
#30036=B_SPLINE_CURVE_WITH_KNOTS('',3,(#154951,#154952,#154953,#154954,
#154955,#154956),.UNSPECIFIED.,.F.,.F.,(4,1,1,4),(0.,0.3333333333333,0.6666666666667,
1.),.UNSPECIFIED.);
#30037=B_SPLINE_CURVE_WITH_KNOTS('',3,(#154958,#154959,#154960,#154961,
#154962,#154963,#154964),.UNSPECIFIED.,.F.,.F.,(4,3,4),(0.,0.5,1.),
 .UNSPECIFIED.);
#30038=B_SPLINE_CURVE_WITH_KNOTS('',3,(#154967,#154968,#154969,#154970,
#154971,#154972,#154973),.UNSPECIFIED.,.F.,.F.,(4,3,4),(0.,0.5,1.),
 .UNSPECIFIED.);
#30039=B_SPLINE_CURVE_WITH_KNOTS('',3,(#154974,#154975,#154976,#154977,
#154978),.UNSPECIFIED.,.F.,.F.,(4,1,4),(0.,0.5,0.999976693117295),
 .UNSPECIFIED.);
#30040=B_SPLINE_CURVE_WITH_KNOTS('',3,(#155022,#155023,#155024,#155025,
#155026,#155027,#155028),.UNSPECIFIED.,.F.,.F.,(4,3,4),(0.,0.737738535805643,
0.999999999999949),.UNSPECIFIED.);
#30041=B_SPLINE_CURVE_WITH_KNOTS('',3,(#155080,#155081,#155082,#155083),
 .UNSPECIFIED.,.F.,.F.,(4,4),(0.,0.999999733456458),.UNSPECIFIED.);
#30042=B_SPLINE_CURVE_WITH_KNOTS('',3,(#155149,#155150,#155151,#155152),
 .UNSPECIFIED.,.F.,.F.,(4,4),(0.,1.),.UNSPECIFIED.);
#30043=B_SPLINE_CURVE_WITH_KNOTS('',3,(#155154,#155155,#155156,#155157,
#155158,#155159,#155160,#155161,#155162,#155163,#155164,#155165,#155166,
#155167,#155168,#155169,#155170,#155171,#155172,#155173,#155174,#155175,
#155176,#155177,#155178,#155179,#155180,#155181,#155182,#155183,#155184,
#155185,#155186,#155187,#155188,#155189,#155190,#155191,#155192,#155193,
#155194,#155195,#155196,#155197,#155198,#155199,#155200,#155201,#155202,
#155203,#155204,#155205,#155206,#155207,#155208,#155209,#155210,#155211,
#155212,#155213,#155214,#155215,#155216,#155217,#155218,#155219,#155220,
#155221,#155222,#155223,#155224,#155225,#155226,#155227,#155228,#155229,
#155230,#155231,#155232,#155233,#155234,#155235,#155236,#155237,#155238,
#155239,#155240,#155241,#155242,#155243,#155244,#155245,#155246,#155247,
#155248,#155249,#155250,#155251,#155252,#155253,#155254,#155255,#155256,
#155257,#155258,#155259,#155260,#155261,#155262,#155263,#155264,#155265,
#155266,#155267,#155268,#155269,#155270,#155271,#155272,#155273,#155274,
#155275,#155276,#155277,#155278,#155279,#155280,#155281,#155282,#155283,
#155284,#155285,#155286,#155287,#155288,#155289,#155290,#155291,#155292,
#155293,#155294,#155295,#155296,#155297,#155298,#155299,#155300,#155301,
#155302,#155303,#155304,#155305,#155306,#155307,#155308,#155309,#155310,
#155311,#155312,#155313,#155314,#155315,#155316,#155317,#155318,#155319,
#155320,#155321,#155322,#155323,#155324,#155325,#155326,#155327,#155328,
#155329,#155330,#155331,#155332,#155333,#155334,#155335,#155336,#155337,
#155338,#155339,#155340,#155341,#155342,#155343,#155344,#155345,#155346,
#155347,#155348,#155349,#155350,#155351,#155352,#155353,#155354,#155355,
#155356,#155357,#155358,#155359,#155360,#155361,#155362,#155363,#155364,
#155365,#155366,#155367,#155368,#155369,#155370,#155371,#155372,#155373,
#155374,#155375,#155376,#155377,#155378,#155379,#155380,#155381,#155382,
#155383,#155384,#155385,#155386,#155387,#155388,#155389,#155390,#155391,
#155392,#155393,#155394,#155395,#155396,#155397,#155398,#155399,#155400,
#155401,#155402,#155403,#155404,#155405,#155406,#155407,#155408,#155409,
#155410,#155411,#155412,#155413,#155414,#155415,#155416,#155417,#155418,
#155419,#155420,#155421,#155422,#155423,#155424),.UNSPECIFIED.,.F.,.F.,
(4,3,3,3,3,3,3,3,3,3,3,3,3,3,3,3,3,3,3,3,3,3,3,3,3,3,3,3,3,3,3,3,3,3,3,
3,3,3,3,3,3,3,3,3,3,3,3,3,3,3,3,3,3,3,3,3,3,3,3,3,3,3,3,3,3,3,3,3,3,3,3,
3,3,3,3,3,3,3,3,3,3,3,3,3,3,3,3,3,3,3,4),(0.,0.0156249999999938,0.0312499999999876,
0.0468749999999821,0.05468749999998,0.0585937499999794,0.0605468749999791,
0.0615234374999789,0.0620117187499788,0.0624999999999787,0.0737022644319959,
0.084645872498037,0.0937499999999818,0.104685910244887,0.109374999999983,
0.118663537724106,0.124999999999984,0.139243619738437,0.146301019042459,
0.161162267135373,0.176716398763141,0.187499999999988,0.207644104682402,
0.21874999999999,0.234374999999992,0.242187499999992,0.246093749999993,
0.248046874999993,0.249023437499993,0.249511718749992,0.249999999999992,
0.272731652445828,0.302235313168796,0.312499999999973,0.326809661104179,
0.353843405339416,0.374999999999953,0.383302879496592,0.412729393604404,
0.437499999999933,0.442461712707441,0.468749999999924,0.484374999999919,
0.492215068290938,0.499999999999914,0.504389899607464,0.536742275540799,
0.569776777538791,0.602077537598559,0.622092744943588,0.624999999999875,
0.652975419385661,0.677138851153577,0.687499999999855,0.712581838697012,
0.718749999999845,0.730023511366994,0.73437499999984,0.742187499999838,
0.746093749999836,0.748046874999835,0.749023437499835,0.749511718749835,
0.749999999999835,0.772497759731973,0.794313424727545,0.812499999999868,
0.829511372540639,0.843749999999884,0.854252480274351,0.859374999999892,
0.867187499999896,0.872391286447649,0.8749999999999,0.885692729179628,0.896423825799802,
0.906249999999915,0.91699473121533,0.921874999999922,0.929687499999924,
0.933593749999927,0.935546874999927,0.936523437499928,0.937011718749928,
0.937255859374929,0.937499999999929,0.955209733027919,0.968749999999964,
0.98350921182179,0.998604231401742,1.),.UNSPECIFIED.);
#30044=B_SPLINE_CURVE_WITH_KNOTS('',3,(#155425,#155426,#155427,#155428),
 .UNSPECIFIED.,.F.,.F.,(4,4),(4.21851813676615E-6,1.),.UNSPECIFIED.);
#30045=B_SPLINE_CURVE_WITH_KNOTS('',3,(#155453,#155454,#155455,#155456,
#155457,#155458),.UNSPECIFIED.,.F.,.F.,(4,2,4),(6.01557958534666E-6,0.5,
1.),.UNSPECIFIED.);
#30046=B_SPLINE_CURVE_WITH_KNOTS('',3,(#155485,#155486,#155487,#155488,
#155489,#155490,#155491,#155492,#155493,#155494,#155495,#155496,#155497,
#155498,#155499,#155500),.UNSPECIFIED.,.F.,.F.,(4,3,3,3,3,4),(0.,0.25,0.499016891676494,
0.749508445838247,0.986332989034377,1.),.UNSPECIFIED.);
#30047=B_SPLINE_CURVE_WITH_KNOTS('',3,(#155517,#155518,#155519,#155520,
#155521,#155522,#155523,#155524,#155525,#155526,#155527,#155528,#155529,
#155530,#155531,#155532,#155533,#155534,#155535,#155536,#155537,#155538,
#155539,#155540,#155541),.UNSPECIFIED.,.F.,.F.,(4,3,3,3,3,3,3,3,4),(0.,
0.143229396317443,0.288391134800666,0.428837100197094,0.56846061529328,
0.707144473842968,0.723876350250335,0.861938175125168,1.),.UNSPECIFIED.);
#30048=B_SPLINE_CURVE_WITH_KNOTS('',3,(#155618,#155619,#155620,#155621,
#155622,#155623,#155624,#155625,#155626,#155627,#155628,#155629,#155630,
#155631,#155632,#155633,#155634,#155635,#155636,#155637,#155638,#155639,
#155640,#155641,#155642,#155643,#155644,#155645,#155646,#155647,#155648,
#155649,#155650,#155651,#155652,#155653,#155654,#155655,#155656,#155657,
#155658,#155659,#155660,#155661,#155662,#155663,#155664,#155665,#155666,
#155667,#155668,#155669,#155670,#155671,#155672,#155673,#155674,#155675,
#155676,#155677,#155678,#155679,#155680,#155681,#155682,#155683,#155684,
#155685,#155686,#155687,#155688,#155689,#155690,#155691,#155692,#155693,
#155694,#155695,#155696,#155697,#155698,#155699,#155700,#155701,#155702,
#155703,#155704,#155705,#155706,#155707,#155708,#155709,#155710,#155711,
#155712,#155713,#155714,#155715,#155716,#155717,#155718,#155719,#155720),
 .UNSPECIFIED.,.F.,.F.,(4,3,3,3,3,3,3,3,3,3,3,3,3,3,3,3,3,3,3,3,3,3,3,3,
3,3,3,3,3,3,3,3,3,3,4),(0.,0.0271165157246254,0.0552397979707361,0.0805406843846776,
0.117403543853953,0.124999999999937,0.163705158930506,0.191078655875936,
0.238272614623893,0.287092880371944,0.326326003103155,0.381913001551468,
0.437499999999781,0.468749999999766,0.484374999999758,0.492187499999756,
0.496093749999755,0.498046874999754,0.498822546661111,0.499999999999754,
0.550409420598624,0.600158718135214,0.649053115359039,0.666386519103641,
0.716491463985741,0.764059802343202,0.805072556691199,0.843451541598094,
0.874999999999939,0.911087468126675,0.917362338160448,0.944900395318624,
0.972450197659312,0.998184941463724,1.),.UNSPECIFIED.);
#30049=B_SPLINE_CURVE_WITH_KNOTS('',3,(#155723,#155724,#155725,#155726,
#155727,#155728,#155729,#155730,#155731,#155732,#155733,#155734,#155735,
#155736,#155737,#155738,#155739,#155740,#155741),.UNSPECIFIED.,.F.,.F.,
(4,3,3,3,3,3,4),(1.40360687088514E-7,0.188647371465953,0.385548650834157,
0.587125074313563,0.794262989574996,0.92226232086797,0.999999996838511),
 .UNSPECIFIED.);
#30050=B_SPLINE_CURVE_WITH_KNOTS('',3,(#155766,#155767,#155768,#155769,
#155770,#155771,#155772,#155773,#155774,#155775,#155776,#155777,#155778,
#155779,#155780,#155781,#155782,#155783,#155784,#155785,#155786,#155787,
#155788,#155789,#155790,#155791,#155792,#155793,#155794,#155795,#155796,
#155797,#155798,#155799,#155800,#155801,#155802,#155803,#155804,#155805,
#155806,#155807,#155808,#155809,#155810,#155811,#155812,#155813,#155814),
 .UNSPECIFIED.,.F.,.F.,(4,3,3,3,3,3,3,3,3,3,3,3,3,3,3,3,4),(2.72844949517765E-9,
0.0688980942246612,0.136773037531096,0.203343850945352,0.25,0.315004214893658,
0.379445255356854,0.443457188921027,0.507172269215425,0.570759851800854,
0.634335833368114,0.698186251307407,0.75,0.814712454999434,0.879894274521964,
0.946132007109019,1.),.UNSPECIFIED.);
#30051=B_SPLINE_CURVE_WITH_KNOTS('',3,(#155815,#155816,#155817,#155818,
#155819,#155820,#155821,#155822,#155823,#155824,#155825,#155826,#155827,
#155828,#155829,#155830,#155831,#155832,#155833,#155834,#155835,#155836,
#155837,#155838,#155839,#155840,#155841,#155842,#155843,#155844,#155845,
#155846,#155847,#155848,#155849,#155850,#155851,#155852,#155853,#155854,
#155855,#155856,#155857,#155858,#155859,#155860,#155861,#155862,#155863),
 .UNSPECIFIED.,.F.,.F.,(4,3,3,3,3,3,3,3,3,3,3,3,3,3,3,3,4),(0.,0.0692784102920228,
0.14120044859868,0.219196668058418,0.25,0.324115642155737,0.40008119894174,
0.478002093519741,0.5,0.577710157022752,0.654118301000089,0.727900984558949,
0.75,0.827504812018075,0.90052310253359,0.969341196485938,1.),
 .UNSPECIFIED.);
#30052=B_SPLINE_CURVE_WITH_KNOTS('',3,(#155870,#155871,#155872,#155873,
#155874,#155875,#155876,#155877,#155878,#155879,#155880,#155881,#155882,
#155883,#155884,#155885,#155886,#155887,#155888,#155889,#155890,#155891,
#155892,#155893,#155894,#155895,#155896,#155897,#155898,#155899,#155900,
#155901,#155902,#155903,#155904,#155905,#155906,#155907,#155908,#155909,
#155910,#155911,#155912,#155913,#155914,#155915,#155916,#155917,#155918,
#155919,#155920,#155921,#155922,#155923,#155924,#155925,#155926,#155927,
#155928,#155929,#155930,#155931,#155932,#155933,#155934,#155935,#155936,
#155937,#155938,#155939),.UNSPECIFIED.,.F.,.F.,(4,3,3,3,3,3,3,3,3,3,3,3,
3,3,3,3,3,3,3,3,3,3,3,4),(1.30324300997627E-11,0.0505870658958078,0.100440299421859,
0.149328502274208,0.19966425113711,0.247432688679266,0.250000000000012,
0.293728580204281,0.337185021169438,0.37500000000001,0.416703010961095,
0.458351505480552,0.500000000000008,0.541602652045577,0.583301326022791,
0.625000000000006,0.668398095794137,0.712079215319331,0.750000000000004,
0.79783378980656,0.84837534235492,0.89760075028844,0.94880037514422,1.),
 .UNSPECIFIED.);
#30053=B_SPLINE_CURVE_WITH_KNOTS('',3,(#155981,#155982,#155983,#155984,
#155985,#155986,#155987,#155988,#155989,#155990,#155991,#155992,#155993,
#155994,#155995,#155996,#155997,#155998,#155999,#156000,#156001,#156002,
#156003,#156004,#156005,#156006,#156007,#156008,#156009,#156010,#156011,
#156012,#156013,#156014),.UNSPECIFIED.,.F.,.F.,(4,2,2,1,1,1,2,2,2,2,2,1,
2,2,2,2,2,2,4),(0.,0.125000000000211,0.187500000000305,0.218750000000348,
0.234375000000365,0.242187500000373,0.246093750000373,0.250000000000373,
0.375000000000463,0.437500000000502,0.468750000000521,0.484375000000531,
0.492187500000526,0.50000000000052,0.62500000000035,0.687500000000268,0.718750000000221,
0.750000000000175,1.),.UNSPECIFIED.);
#30054=B_SPLINE_CURVE_WITH_KNOTS('',3,(#156015,#156016,#156017,#156018,
#156019,#156020,#156021,#156022,#156023,#156024),.UNSPECIFIED.,.F.,.F.,
(4,2,2,2,4),(2.13390469791841E-7,0.25,0.5,0.75,1.),.UNSPECIFIED.);
#30055=B_SPLINE_CURVE_WITH_KNOTS('',3,(#156049,#156050,#156051,#156052,
#156053,#156054,#156055,#156056,#156057,#156058,#156059,#156060,#156061),
 .UNSPECIFIED.,.F.,.F.,(4,3,3,3,4),(0.,0.266292368485203,0.529417506706766,
0.787742675205748,1.),.UNSPECIFIED.);
#30056=B_SPLINE_CURVE_WITH_KNOTS('',3,(#156063,#156064,#156065,#156066,
#156067,#156068,#156069,#156070,#156071,#156072,#156073,#156074,#156075,
#156076,#156077,#156078,#156079,#156080,#156081,#156082,#156083,#156084,
#156085,#156086,#156087,#156088,#156089,#156090,#156091,#156092,#156093,
#156094,#156095,#156096,#156097,#156098,#156099),.UNSPECIFIED.,.F.,.F.,
(4,3,3,3,3,3,3,3,3,3,3,3,4),(3.31179824555737E-10,0.017425231587708,0.0982830680925832,
0.125,0.188631792544538,0.288498005434872,0.398901768809661,0.521077852077812,
0.657045747770235,0.749999999999999,0.808620188251583,0.981759508105347,
1.),.UNSPECIFIED.);
#30057=B_SPLINE_CURVE_WITH_KNOTS('',3,(#156156,#156157,#156158,#156159),
 .UNSPECIFIED.,.F.,.F.,(4,4),(0.,1.),.UNSPECIFIED.);
#30058=B_SPLINE_CURVE_WITH_KNOTS('',3,(#156252,#156253,#156254,#156255,
#156256,#156257,#156258),.UNSPECIFIED.,.F.,.F.,(4,3,4),(2.76766290252202E-14,
0.394366854122773,1.),.UNSPECIFIED.);
#30059=B_SPLINE_CURVE_WITH_KNOTS('',3,(#156455,#156456,#156457,#156458,
#156459,#156460,#156461,#156462,#156463,#156464,#156465,#156466,#156467,
#156468,#156469,#156470,#156471,#156472,#156473,#156474,#156475,#156476,
#156477,#156478,#156479,#156480,#156481,#156482,#156483,#156484,#156485,
#156486,#156487,#156488,#156489,#156490,#156491,#156492,#156493,#156494,
#156495,#156496,#156497,#156498,#156499,#156500,#156501,#156502,#156503,
#156504,#156505,#156506,#156507,#156508,#156509,#156510,#156511,#156512,
#156513,#156514,#156515,#156516,#156517,#156518,#156519,#156520,#156521,
#156522,#156523,#156524,#156525,#156526,#156527,#156528,#156529,#156530,
#156531,#156532,#156533,#156534,#156535,#156536,#156537,#156538,#156539,
#156540,#156541,#156542,#156543,#156544,#156545,#156546,#156547,#156548,
#156549,#156550,#156551,#156552,#156553,#156554,#156555,#156556,#156557,
#156558,#156559,#156560,#156561,#156562,#156563,#156564,#156565,#156566,
#156567,#156568,#156569,#156570,#156571,#156572,#156573,#156574,#156575,
#156576,#156577,#156578,#156579,#156580,#156581,#156582,#156583,#156584,
#156585,#156586,#156587,#156588,#156589,#156590,#156591,#156592,#156593,
#156594,#156595,#156596,#156597,#156598,#156599,#156600,#156601,#156602,
#156603,#156604,#156605,#156606,#156607,#156608,#156609,#156610,#156611,
#156612,#156613,#156614,#156615,#156616,#156617,#156618,#156619,#156620,
#156621,#156622,#156623,#156624,#156625,#156626,#156627,#156628,#156629,
#156630,#156631,#156632,#156633,#156634,#156635,#156636,#156637,#156638,
#156639,#156640,#156641,#156642,#156643,#156644,#156645,#156646,#156647,
#156648,#156649,#156650,#156651,#156652,#156653,#156654,#156655,#156656,
#156657,#156658,#156659,#156660,#156661,#156662,#156663,#156664,#156665,
#156666,#156667,#156668,#156669,#156670,#156671,#156672,#156673,#156674,
#156675,#156676,#156677,#156678,#156679,#156680),.UNSPECIFIED.,.F.,.F.,
(4,3,3,3,3,3,3,3,3,3,3,3,3,3,3,3,3,3,3,3,3,3,3,3,3,3,3,3,3,3,3,3,3,3,3,
3,3,3,3,3,3,3,3,3,3,3,3,3,3,3,3,3,3,3,3,3,3,3,3,3,3,3,3,3,3,3,3,3,3,3,3,
3,3,3,3,4),(7.6013246015319E-11,0.0041559545228748,0.0210327898696483,0.0364291191706356,
0.0506222225081979,0.0518254484716229,0.062500000000003,0.0768035721053361,
0.0901372856082214,0.0937500000000051,0.0957761658748245,0.109375000000006,
0.117187500000006,0.121621389086509,0.125000000000006,0.138007198100994,
0.157743784493814,0.17744665752372,0.183453626090955,0.187500000000005,
0.211871023920911,0.218750000000005,0.229271298665007,0.234375000000004,
0.244589973646335,0.250000000000004,0.275239681532887,0.308690342494038,
0.322549049282618,0.357856894736005,0.368021252616143,0.375000000000001,
0.412158293166225,0.4375,0.456105693290628,0.468749999999999,0.484374999999998,
0.494801092711084,0.499999999999998,0.500025444460262,0.535118723365545,
0.543900825062066,0.585389277369181,0.588656357587658,0.624999999999995,
0.633432881746038,0.67375366506979,0.678858288706035,0.687499999999994,
0.718749999999993,0.725429350075826,0.734374999999993,0.742187499999993,
0.748453902845257,0.749999999999992,0.770125508965917,0.793523145696441,
0.812499999999992,0.814944956455603,0.834716949094254,0.843749999999992,
0.859374999999993,0.860947350563149,0.867187499999993,0.872125445495224,
0.874999999999993,0.891067994006378,0.90431467626986,0.918228777029266,
0.933515770458162,0.94866558411337,0.962510547721232,0.977069250318923,
0.992781062457308,0.996004191295995,0.999999999923944),.UNSPECIFIED.);
#30060=B_SPLINE_CURVE_WITH_KNOTS('',3,(#156772,#156773,#156774,#156775,
#156776,#156777,#156778,#156779,#156780,#156781,#156782,#156783,#156784,
#156785,#156786,#156787,#156788,#156789,#156790,#156791,#156792,#156793,
#156794,#156795,#156796,#156797,#156798,#156799,#156800,#156801),
 .UNSPECIFIED.,.F.,.F.,(4,1,2,2,2,2,2,2,2,2,2,2,1,2,2,4),(0.,0.0624999999999996,
0.0937499999999994,0.124999999999999,0.187499999999999,0.249999999999998,
0.374999999999997,0.499999999999997,0.562499999999996,0.624999999999996,
0.656249999999996,0.687499999999996,0.718749999999995,0.734374999999995,
0.749999999999995,1.),.UNSPECIFIED.);
#30061=B_SPLINE_CURVE_WITH_KNOTS('',3,(#156802,#156803,#156804,#156805),
 .UNSPECIFIED.,.F.,.F.,(4,4),(0.,1.),.UNSPECIFIED.);
#30062=B_SPLINE_CURVE_WITH_KNOTS('',3,(#156867,#156868,#156869,#156870,
#156871,#156872,#156873,#156874,#156875,#156876,#156877,#156878,#156879,
#156880,#156881,#156882,#156883,#156884,#156885,#156886,#156887,#156888,
#156889,#156890,#156891,#156892,#156893,#156894,#156895,#156896,#156897,
#156898,#156899,#156900,#156901,#156902,#156903,#156904,#156905,#156906,
#156907,#156908,#156909,#156910,#156911,#156912,#156913,#156914,#156915,
#156916,#156917,#156918,#156919,#156920,#156921,#156922,#156923,#156924,
#156925,#156926,#156927,#156928,#156929,#156930,#156931,#156932,#156933,
#156934,#156935,#156936,#156937,#156938,#156939,#156940,#156941,#156942,
#156943,#156944,#156945,#156946,#156947,#156948,#156949,#156950,#156951,
#156952,#156953,#156954,#156955,#156956,#156957,#156958,#156959,#156960,
#156961,#156962,#156963,#156964,#156965,#156966,#156967,#156968,#156969,
#156970,#156971,#156972,#156973,#156974,#156975,#156976,#156977,#156978,
#156979,#156980,#156981,#156982,#156983,#156984,#156985,#156986,#156987,
#156988,#156989,#156990,#156991,#156992,#156993,#156994,#156995,#156996),
 .UNSPECIFIED.,.F.,.F.,(4,3,3,3,3,3,3,3,3,3,3,3,3,3,3,3,3,3,3,3,3,3,3,3,
3,3,3,3,3,3,3,3,3,3,3,3,3,3,3,3,3,3,3,4),(0.,0.0222450806380213,0.0461572035151902,
0.073857491338037,0.107011041434932,0.125000000000011,0.136894536412116,
0.165629046527801,0.187500000000016,0.21875000000002,0.234375000000022,
0.248046875000024,0.249023437500024,0.250000000000024,0.276355845277275,
0.306209016223028,0.312500000000028,0.315840428150021,0.343618932232895,
0.371772527297605,0.375000000000032,0.406250000000034,0.429246372797829,
0.437500000000037,0.468750000000039,0.48437500000004,0.490901035393806,
0.492187500000041,0.500000000000042,0.532608092654646,0.567801163203751,
0.607335064867353,0.625000000000031,0.651439700206761,0.690432671400696,
0.727656080590827,0.750000000000021,0.799191181786869,0.817962618702426,
0.863110957751424,0.907571031864983,0.950396133988827,0.983659176247363,
0.999999999636422),.UNSPECIFIED.);
#30063=B_SPLINE_CURVE_WITH_KNOTS('',3,(#157001,#157002,#157003,#157004,
#157005,#157006,#157007,#157008,#157009,#157010,#157011,#157012,#157013,
#157014,#157015,#157016,#157017,#157018,#157019,#157020,#157021,#157022,
#157023,#157024,#157025,#157026,#157027),.UNSPECIFIED.,.F.,.F.,(4,1,1,2,
2,2,1,1,1,2,2,1,1,1,1,2,2,4),(3.14323848108535E-9,0.125000000000001,0.187500000000002,
0.218750000000002,0.250000000000002,0.375000000000001,0.4375,0.46875,0.484374999999999,
0.496093749999996,0.499999999999995,0.624999999999936,0.687499999999908,
0.718749999999894,0.734374999999886,0.748046874999877,0.749999999999876,
1.),.UNSPECIFIED.);
#30064=B_SPLINE_CURVE_WITH_KNOTS('',3,(#157051,#157052,#157053,#157054,
#157055,#157056,#157057,#157058,#157059,#157060,#157061,#157062,#157063,
#157064),.UNSPECIFIED.,.F.,.F.,(4,2,2,2,2,2,4),(0.,0.25,0.499999999999999,
0.624999999999999,0.75,0.875,1.),.UNSPECIFIED.);
#30065=B_SPLINE_CURVE_WITH_KNOTS('',3,(#157255,#157256,#157257,#157258,
#157259,#157260,#157261,#157262,#157263,#157264,#157265,#157266,#157267,
#157268,#157269,#157270,#157271,#157272,#157273,#157274,#157275,#157276,
#157277,#157278,#157279,#157280,#157281,#157282,#157283,#157284,#157285,
#157286,#157287,#157288,#157289,#157290,#157291),.UNSPECIFIED.,.F.,.F.,
(4,3,3,3,3,3,3,3,3,3,3,3,4),(0.,0.0396954288592127,0.184386182462915,0.194668024552279,
0.347219950006161,0.368101049680069,0.499999999999998,0.558416630619174,
0.724544290911746,0.76399353681739,0.924890186709707,0.981597205952527,
0.999999988137177),.UNSPECIFIED.);
#30066=B_SPLINE_CURVE_WITH_KNOTS('',3,(#157292,#157293,#157294,#157295,
#157296,#157297,#157298,#157299,#157300,#157301,#157302,#157303,#157304,
#157305),.UNSPECIFIED.,.F.,.F.,(4,2,2,2,2,2,4),(3.42050715226368E-6,0.0559041406044768,
0.110821873002056,0.16870681326424,0.225445105585076,0.2820690083687,0.337327565891503),
 .UNSPECIFIED.);
#30067=B_SPLINE_CURVE_WITH_KNOTS('',3,(#157363,#157364,#157365,#157366,
#157367,#157368),.UNSPECIFIED.,.F.,.F.,(4,2,4),(3.41822380810718E-6,0.143396991606946,
0.286369799377383),.UNSPECIFIED.);
#30068=B_SPLINE_CURVE_WITH_KNOTS('',3,(#157386,#157387,#157388,#157389,
#157390,#157391),.UNSPECIFIED.,.F.,.F.,(4,2,4),(4.9161935946595E-6,0.0292090733184409,
0.0584199189037688),.UNSPECIFIED.);
#30069=B_SPLINE_CURVE_WITH_KNOTS('',3,(#157449,#157450,#157451,#157452,
#157453),.UNSPECIFIED.,.F.,.F.,(4,1,4),(0.,0.5,0.999995825079256),
 .UNSPECIFIED.);
#30070=B_SPLINE_CURVE_WITH_KNOTS('',3,(#157496,#157497,#157498,#157499,
#157500,#157501,#157502,#157503,#157504,#157505,#157506,#157507,#157508,
#157509,#157510,#157511,#157512,#157513,#157514,#157515,#157516,#157517,
#157518,#157519,#157520,#157521,#157522,#157523,#157524,#157525,#157526,
#157527,#157528,#157529,#157530,#157531,#157532,#157533,#157534,#157535,
#157536,#157537,#157538,#157539,#157540,#157541,#157542,#157543,#157544,
#157545,#157546,#157547,#157548,#157549,#157550,#157551,#157552,#157553,
#157554,#157555,#157556,#157557,#157558,#157559),.UNSPECIFIED.,.F.,.F.,
(4,3,3,3,3,3,3,3,3,3,3,3,3,3,3,3,3,3,3,3,3,4),(0.0475883983781192,0.0504715149112503,
0.101359766783617,0.153027051352179,0.205253844737498,0.229513928442054,
0.249999999999997,0.3270059293996,0.374999999999996,0.412568101857693,0.456284050928844,
0.499999999999995,0.568529833373717,0.596947337798161,0.668057214031891,
0.735905642822662,0.749999999999998,0.78220040594856,0.848341524055653,
0.914724761179046,0.969216113718377,1.),.UNSPECIFIED.);
#30071=B_SPLINE_CURVE_WITH_KNOTS('',3,(#157560,#157561,#157562,#157563,
#157564,#157565,#157566,#157567,#157568,#157569,#157570,#157571,#157572,
#157573,#157574,#157575,#157576,#157577,#157578,#157579,#157580,#157581,
#157582,#157583,#157584,#157585,#157586,#157587,#157588,#157589,#157590,
#157591,#157592,#157593,#157594,#157595,#157596,#157597,#157598,#157599,
#157600,#157601,#157602,#157603,#157604,#157605,#157606,#157607,#157608,
#157609,#157610,#157611,#157612,#157613,#157614,#157615,#157616,#157617,
#157618,#157619,#157620),.UNSPECIFIED.,.F.,.F.,(4,3,3,3,3,3,3,3,3,3,3,3,
3,3,3,3,3,3,3,3,4),(3.7300084670044E-6,0.0744120387739684,0.125000000000108,
0.18750000000019,0.218750000000223,0.233569723016874,0.234375000000221,
0.246852766807326,0.250000000000218,0.500000000000137,0.625000000000087,
0.687500000000034,0.718750000000016,0.742152599453903,0.749999999999997,
0.804729863476949,0.859609535575322,0.874999999999999,0.928349847165128,
0.981841124851018,0.999998027188981),.UNSPECIFIED.);
#30072=B_SPLINE_CURVE_WITH_KNOTS('',3,(#157748,#157749,#157750,#157751,
#157752,#157753,#157754,#157755,#157756,#157757,#157758,#157759,#157760,
#157761,#157762,#157763,#157764),.UNSPECIFIED.,.F.,.F.,(4,2,2,1,1,1,2,2,
2,4),(1.43410335955E-5,0.249999999999933,0.374999999999896,0.437499999999873,
0.468749999999867,0.484374999999859,0.492187499999856,0.499999999999853,
0.749999999999926,1.),.UNSPECIFIED.);
#30073=B_SPLINE_CURVE_WITH_KNOTS('',3,(#157799,#157800,#157801,#157802,
#157803,#157804,#157805,#157806,#157807,#157808),.UNSPECIFIED.,.F.,.F.,
(4,2,2,2,4),(9.6294942429E-6,0.25,0.5,0.75,1.),.UNSPECIFIED.);
#30074=B_SPLINE_CURVE_WITH_KNOTS('',3,(#157841,#157842,#157843,#157844,
#157845,#157846,#157847,#157848,#157849,#157850,#157851,#157852,#157853,
#157854,#157855,#157856,#157857,#157858,#157859,#157860,#157861,#157862,
#157863,#157864,#157865,#157866,#157867,#157868,#157869,#157870,#157871,
#157872,#157873,#157874,#157875,#157876,#157877,#157878,#157879,#157880,
#157881,#157882,#157883,#157884,#157885,#157886,#157887,#157888,#157889,
#157890,#157891,#157892,#157893,#157894,#157895,#157896,#157897,#157898,
#157899,#157900,#157901,#157902,#157903,#157904,#157905,#157906,#157907),
 .UNSPECIFIED.,.F.,.F.,(4,3,3,3,3,3,3,3,3,3,3,3,3,3,3,3,3,3,3,3,3,3,4),
(1.24011628705212E-10,0.0531053496019451,0.10437770154546,0.154727528060671,
0.203864455437261,0.25,0.297836570659254,0.345161045291314,0.392002186152137,
0.438626827965545,0.485141010125923,0.5,0.546606499906862,0.593402564378951,
0.64074134746124,0.688461599503242,0.736927113385546,0.75,0.799583122725084,
0.85071410427355,0.90277575624421,0.95662774238403,1.),.UNSPECIFIED.);
#30075=B_SPLINE_CURVE_WITH_KNOTS('',3,(#157957,#157958,#157959,#157960,
#157961,#157962,#157963,#157964,#157965,#157966,#157967,#157968,#157969,
#157970,#157971,#157972,#157973,#157974,#157975,#157976,#157977,#157978,
#157979,#157980,#157981,#157982,#157983,#157984,#157985,#157986,#157987,
#157988,#157989,#157990,#157991,#157992,#157993,#157994,#157995,#157996,
#157997,#157998,#157999,#158000,#158001,#158002,#158003,#158004,#158005,
#158006,#158007,#158008,#158009,#158010,#158011,#158012,#158013,#158014,
#158015,#158016,#158017,#158018,#158019,#158020,#158021,#158022,#158023),
 .UNSPECIFIED.,.F.,.F.,(4,3,3,3,3,3,3,3,3,3,3,3,3,3,3,3,3,3,3,3,3,3,4),
(1.19754065422301E-14,0.0537123221293526,0.105496107116609,0.156304258830716,
0.20582389888184,0.25,0.298149632596059,0.34572619551662,0.392732615136169,
0.439472860332929,0.486031305273164,0.5,0.546563122917741,0.593256574146164,
0.640406002773063,0.687884574046229,0.736036975820931,0.75,0.799190988175816,
0.849837660146647,0.901356920133292,0.954590545665251,1.),.UNSPECIFIED.);
#30076=B_SPLINE_CURVE_WITH_KNOTS('',3,(#158053,#158054,#158055,#158056,
#158057,#158058),.UNSPECIFIED.,.F.,.F.,(4,2,4),(0.,0.5,1.),
 .UNSPECIFIED.);
#30077=B_SPLINE_CURVE_WITH_KNOTS('',3,(#158152,#158153,#158154,#158155,
#158156,#158157,#158158,#158159,#158160,#158161,#158162,#158163,#158164,
#158165,#158166,#158167,#158168,#158169,#158170,#158171,#158172,#158173,
#158174,#158175,#158176,#158177,#158178,#158179,#158180,#158181,#158182,
#158183,#158184,#158185,#158186,#158187,#158188,#158189,#158190,#158191,
#158192,#158193,#158194,#158195,#158196,#158197,#158198,#158199,#158200),
 .UNSPECIFIED.,.F.,.F.,(4,3,3,3,3,3,3,3,3,3,3,3,3,3,3,3,4),(0.,0.0693090958433355,
0.141292481527221,0.219438370094957,0.25,0.324257641112822,0.400369388793943,
0.47840899005484,0.5,0.577797592734866,0.654240606146742,0.728007698508539,
0.75,0.827331791071793,0.900155287073229,0.968761945896699,1.),
 .UNSPECIFIED.);
#30630=CIRCLE('',#79485,1.5);
#30631=CIRCLE('',#79486,1.5);
#30632=CIRCLE('',#79487,1.500000002703);
#30633=CIRCLE('',#79493,1.50000004292401);
#30634=CIRCLE('',#79494,1.5);
#30635=CIRCLE('',#79495,1.5);
#30636=CIRCLE('',#79501,20.5);
#30637=CIRCLE('',#79505,9.47898844935865);
#30638=CIRCLE('',#79508,20.5);
#30639=CIRCLE('',#79510,1.5);
#30640=CIRCLE('',#79513,9.52146805877686);
#30641=CIRCLE('',#79516,8.39999999999999);
#30642=CIRCLE('',#79520,8.4);
#30643=CIRCLE('',#79523,8.4);
#30644=CIRCLE('',#79529,17.);
#30645=CIRCLE('',#79531,16.375);
#30646=CIRCLE('',#79532,16.375);
#30647=CIRCLE('',#79535,16.375);
#30648=CIRCLE('',#79536,16.5);
#30649=CIRCLE('',#79537,29.9999999999995);
#30650=CIRCLE('',#79538,19.);
#30651=CIRCLE('',#79540,20.5);
#30652=CIRCLE('',#79541,20.5);
#30653=CIRCLE('',#79542,20.5);
#30654=CIRCLE('',#79544,1.499999982843);
#30655=CIRCLE('',#79545,1.5);
#30656=CIRCLE('',#79546,1.499999982843);
#30657=CIRCLE('',#79547,1.5);
#30658=CIRCLE('',#79548,1.5);
#30659=CIRCLE('',#79550,11.);
#30660=CIRCLE('',#79552,1.5);
#30661=CIRCLE('',#79553,1.469693767054);
#30662=CIRCLE('',#79554,1.50000000000001);
#30663=CIRCLE('',#79556,9.50000000000099);
#30664=CIRCLE('',#79557,10.0995446485457);
#30665=CIRCLE('',#79559,10.5);
#30666=CIRCLE('',#79560,10.5);
#30667=CIRCLE('',#79561,10.5);
#30668=CIRCLE('',#79563,10.99999310643);
#30669=CIRCLE('',#79564,0.5);
#30670=CIRCLE('',#79566,11.25);
#30671=CIRCLE('',#79567,11.25);
#30672=CIRCLE('',#79568,11.25);
#30673=CIRCLE('',#79570,11.7499940828);
#30674=CIRCLE('',#79571,0.5);
#30675=CIRCLE('',#79573,11.);
#30676=CIRCLE('',#79574,0.500000000000001);
#30677=CIRCLE('',#79575,10.5);
#30678=CIRCLE('',#79576,0.5);
#30679=CIRCLE('',#79580,21.);
#30680=CIRCLE('',#79583,10.5);
#30681=CIRCLE('',#79584,0.5);
#30682=CIRCLE('',#79585,0.500000000000001);
#30683=CIRCLE('',#79588,1.499999986109);
#30684=CIRCLE('',#79589,1.5);
#30685=CIRCLE('',#79590,1.499999986109);
#30686=CIRCLE('',#79591,1.5);
#30687=CIRCLE('',#79592,1.5);
#30688=CIRCLE('',#79594,9.50000000000099);
#30689=CIRCLE('',#79595,9.50000000000101);
#30690=CIRCLE('',#79597,8.249990255698);
#30691=CIRCLE('',#79598,0.5);
#30692=CIRCLE('',#79599,7.75);
#30693=CIRCLE('',#79600,7.75);
#30694=CIRCLE('',#79602,7.75);
#30695=CIRCLE('',#79604,6.5);
#30696=CIRCLE('',#79605,6.5);
#30697=CIRCLE('',#79606,6.5);
#30698=CIRCLE('',#79608,9.5);
#30699=CIRCLE('',#79609,9.5);
#30700=CIRCLE('',#79610,9.5);
#30701=CIRCLE('',#79611,9.5);
#30702=CIRCLE('',#79613,13.5);
#30703=CIRCLE('',#79614,13.5);
#30704=CIRCLE('',#79615,13.5);
#30705=CIRCLE('',#79617,14.0995393127475);
#30706=CIRCLE('',#79619,14.5);
#30707=CIRCLE('',#79620,14.5);
#30708=CIRCLE('',#79622,7.25);
#30709=CIRCLE('',#79628,6.5);
#30710=CIRCLE('',#79629,6.5);
#30711=CIRCLE('',#79630,0.5);
#30712=CIRCLE('',#79631,6.999991969209);
#30713=CIRCLE('',#79633,6.5);
#30714=CIRCLE('',#79635,5.5);
#30715=CIRCLE('',#79636,6.09968496709595);
#30716=CIRCLE('',#79637,5.5);
#30717=CIRCLE('',#79639,5.5);
#30718=CIRCLE('',#79640,5.5);
#30719=CIRCLE('',#79643,9.5);
#30720=CIRCLE('',#79645,37.5);
#30721=CIRCLE('',#79646,37.5);
#30722=CIRCLE('',#79649,16.);
#30723=CIRCLE('',#79650,16.);
#30724=CIRCLE('',#79651,16.);
#30725=CIRCLE('',#79654,17.);
#30726=CIRCLE('',#79655,17.175);
#30727=CIRCLE('',#79658,9.999992241343);
#30728=CIRCLE('',#79659,0.5);
#30729=CIRCLE('',#79660,9.49999999999999);
#30730=CIRCLE('',#79661,9.49999999999999);
#30731=CIRCLE('',#79663,9.49999999999999);
#30732=CIRCLE('',#79665,8.999610558584);
#30733=CIRCLE('',#79668,12.);
#30734=CIRCLE('',#79670,37.5);
#30735=CIRCLE('',#79671,37.5);
#30736=CIRCLE('',#79673,8.5);
#30737=CIRCLE('',#79675,10.25);
#30738=CIRCLE('',#79676,10.25);
#30739=CIRCLE('',#79678,11.75);
#30740=CIRCLE('',#79679,11.75);
#30741=CIRCLE('',#79680,11.75);
#30742=CIRCLE('',#79682,11.25);
#30743=CIRCLE('',#79684,7.75000000000001);
#30744=CIRCLE('',#79685,7.75000000000001);
#30745=CIRCLE('',#79686,7.75000000000001);
#30746=CIRCLE('',#79687,7.75000000000001);
#30747=CIRCLE('',#79690,7.95);
#30748=CIRCLE('',#79692,9.49999999999999);
#30749=CIRCLE('',#79693,9.49999999999999);
#30750=CIRCLE('',#79694,0.5);
#30751=CIRCLE('',#79695,10.);
#30752=CIRCLE('',#79697,9.49999999999999);
#30753=CIRCLE('',#79699,8.99961055858501);
#30754=CIRCLE('',#79701,8.4);
#30755=CIRCLE('',#79703,12.);
#30756=CIRCLE('',#79705,37.5);
#30757=CIRCLE('',#79706,37.5);
#30758=CIRCLE('',#79708,8.5);
#30759=CIRCLE('',#79710,10.25);
#30760=CIRCLE('',#79711,10.25);
#30761=CIRCLE('',#79713,11.75);
#30762=CIRCLE('',#79714,11.75);
#30763=CIRCLE('',#79715,11.75);
#30764=CIRCLE('',#79717,11.25);
#30765=CIRCLE('',#79719,7.75000000000001);
#30766=CIRCLE('',#79720,7.75000000000001);
#30767=CIRCLE('',#79721,7.75000000000001);
#30768=CIRCLE('',#79722,7.75000000000001);
#30769=CIRCLE('',#79725,7.95);
#30770=CIRCLE('',#79736,1.5);
#30771=CIRCLE('',#79737,1.5);
#30772=CIRCLE('',#79738,9.499999338856);
#30773=CIRCLE('',#79739,9.50002077009014);
#30774=CIRCLE('',#79741,18.5);
#30775=CIRCLE('',#79743,1.5);
#30776=CIRCLE('',#79744,1.499999950122);
#30777=CIRCLE('',#79747,1.);
#30778=CIRCLE('',#79749,1.);
#30779=CIRCLE('',#79751,20.5);
#30780=CIRCLE('',#79752,1.00001318723944);
#30781=CIRCLE('',#79754,1.5);
#30782=CIRCLE('',#79756,20.5);
#30783=CIRCLE('',#79758,0.999999999999988);
#30784=CIRCLE('',#79759,1.50000050755152);
#30785=CIRCLE('',#79760,1.5);
#30786=CIRCLE('',#79761,9.49592460421503);
#30787=CIRCLE('',#79763,1.5);
#30788=CIRCLE('',#79764,27.5);
#30789=CIRCLE('',#79765,1.5);
#30790=CIRCLE('',#79766,25.999999939);
#30791=CIRCLE('',#79768,1.5);
#30792=CIRCLE('',#79769,6.999999373843);
#30793=CIRCLE('',#79771,1.5);
#30794=CIRCLE('',#79772,27.5);
#30795=CIRCLE('',#79773,25.999999939);
#30796=CIRCLE('',#79774,9.499992460383);
#30797=CIRCLE('',#79777,67.5000000000001);
#30798=CIRCLE('',#79778,1.5);
#30799=CIRCLE('',#79779,66.);
#30800=CIRCLE('',#79781,3.999998543283);
#30801=CIRCLE('',#79782,35.99999881413);
#30802=CIRCLE('',#79784,1.5);
#30803=CIRCLE('',#79785,1.5);
#30804=CIRCLE('',#79787,0.999969185525436);
#30805=CIRCLE('',#79788,1.67878043484372);
#30806=CIRCLE('',#79790,36.);
#30807=CIRCLE('',#79791,3.99999530486);
#30808=CIRCLE('',#79793,1.5);
#30809=CIRCLE('',#79794,5.5);
#30810=CIRCLE('',#79797,5.5);
#30811=CIRCLE('',#79798,1.5);
#30812=CIRCLE('',#79799,3.99999479023);
#30813=CIRCLE('',#79801,35.99999988417);
#30814=CIRCLE('',#79802,3.999994788468);
#30815=CIRCLE('',#79804,1.5);
#30816=CIRCLE('',#79805,5.5);
#30817=CIRCLE('',#79809,1.5);
#30818=CIRCLE('',#79810,5.5);
#30819=CIRCLE('',#79816,37.5);
#30820=CIRCLE('',#79818,37.5);
#30821=CIRCLE('',#79821,7.49975097307099);
#30822=CIRCLE('',#79822,7.49996549760091);
#30823=CIRCLE('',#79823,7.499998842876);
#30824=CIRCLE('',#79824,7.4998364236414);
#30825=CIRCLE('',#79825,7.49981706173728);
#30826=CIRCLE('',#79826,7.50005935914293);
#30827=CIRCLE('',#79827,0.899997806293704);
#30828=CIRCLE('',#79828,0.8999999261735);
#30829=CIRCLE('',#79829,0.899996702628005);
#30830=CIRCLE('',#79830,0.899999963985599);
#30831=CIRCLE('',#79831,0.89999753573199);
#30832=CIRCLE('',#79832,0.900009083862835);
#30833=CIRCLE('',#79845,1.5);
#30834=CIRCLE('',#79846,1.5);
#30835=CIRCLE('',#79847,1.500044106112);
#30836=CIRCLE('',#79849,1.);
#30837=CIRCLE('',#79850,1.00000010883301);
#30838=CIRCLE('',#79852,1.);
#30839=CIRCLE('',#79854,1.5);
#30840=CIRCLE('',#79855,1.00000410138919);
#30841=CIRCLE('',#79859,1.5);
#30842=CIRCLE('',#79860,1.499999948802);
#30843=CIRCLE('',#79862,18.5);
#30844=CIRCLE('',#79864,20.5);
#30845=CIRCLE('',#79866,20.5);
#30846=CIRCLE('',#79867,9.5000384206471);
#30847=CIRCLE('',#79868,9.49986806483473);
#30848=CIRCLE('',#79869,9.50751370143532);
#30849=CIRCLE('',#79870,1.5);
#30850=CIRCLE('',#79871,0.9999958303961);
#30851=CIRCLE('',#79872,2.60851153982772);
#30852=CIRCLE('',#79873,1.68163933950004);
#30853=CIRCLE('',#79875,3.999995304826);
#30854=CIRCLE('',#79876,36.);
#30855=CIRCLE('',#79879,1.5);
#30856=CIRCLE('',#79880,1.5);
#30857=CIRCLE('',#79882,35.9999988124);
#30858=CIRCLE('',#79883,3.999998543287);
#30859=CIRCLE('',#79884,66.);
#30860=CIRCLE('',#79886,1.5);
#30861=CIRCLE('',#79887,67.5);
#30862=CIRCLE('',#79889,9.49998316126555);
#30863=CIRCLE('',#79891,1.5);
#30864=CIRCLE('',#79892,27.5);
#30865=CIRCLE('',#79893,1.5);
#30866=CIRCLE('',#79894,25.9999999388);
#30867=CIRCLE('',#79896,1.5);
#30868=CIRCLE('',#79897,6.999999378975);
#30869=CIRCLE('',#79899,1.5);
#30870=CIRCLE('',#79900,27.5);
#30871=CIRCLE('',#79901,25.9999999388);
#30872=CIRCLE('',#79904,1.5);
#30873=CIRCLE('',#79905,5.5);
#30874=CIRCLE('',#79909,1.5);
#30875=CIRCLE('',#79911,5.5);
#30876=CIRCLE('',#79915,5.5);
#30877=CIRCLE('',#79916,1.5);
#30878=CIRCLE('',#79917,3.999994788468);
#30879=CIRCLE('',#79919,35.99999988437);
#30880=CIRCLE('',#79920,3.99999479023);
#30881=CIRCLE('',#79922,1.5);
#30882=CIRCLE('',#79923,5.5);
#30883=CIRCLE('',#79927,37.5);
#30884=CIRCLE('',#79929,37.5);
#30885=CIRCLE('',#79931,7.49963123500319);
#30886=CIRCLE('',#79932,7.49983642367189);
#30887=CIRCLE('',#79933,7.4995737213981);
#30888=CIRCLE('',#79934,7.49996421205067);
#30889=CIRCLE('',#79935,7.49815090357793);
#30890=CIRCLE('',#79936,7.50024364842026);
#30891=CIRCLE('',#79937,0.899999997921601);
#30892=CIRCLE('',#79938,0.900001968871443);
#30893=CIRCLE('',#79939,0.899995896073665);
#30894=CIRCLE('',#79940,0.900004054655721);
#30895=CIRCLE('',#79941,0.899997812495222);
#30896=CIRCLE('',#79948,3.);
#30897=CIRCLE('',#79949,66.50000548541);
#30898=CIRCLE('',#79950,4.499997824719);
#30899=CIRCLE('',#79951,36.49999892491);
#30900=CIRCLE('',#79952,0.499990522764298);
#30901=CIRCLE('',#79954,0.4999905099229);
#30902=CIRCLE('',#79955,36.49999890351);
#30903=CIRCLE('',#79956,4.499997824561);
#30904=CIRCLE('',#79957,66.50000546274);
#30905=CIRCLE('',#79958,3.);
#30906=CIRCLE('',#79964,1.49999970075033);
#30907=CIRCLE('',#79965,1.49999998655821);
#30908=CIRCLE('',#79966,1.50016116215603);
#30909=CIRCLE('',#79969,15.5);
#30910=CIRCLE('',#79970,15.5);
#30911=CIRCLE('',#79972,15.5);
#30912=CIRCLE('',#79973,15.5);
#30913=CIRCLE('',#79975,5.498378496899);
#30914=CIRCLE('',#79977,5.498378496898);
#30915=CIRCLE('',#79978,10.50000198938);
#30916=CIRCLE('',#79980,1.);
#30917=CIRCLE('',#79982,1.);
#30918=CIRCLE('',#79983,10.5002831444245);
#30919=CIRCLE('',#79984,1.499999996972);
#30920=CIRCLE('',#79987,1.49997521686421);
#30921=CIRCLE('',#79988,1.50041791440912);
#30922=CIRCLE('',#79990,1.50000397930881);
#30923=CIRCLE('',#79991,1.50000460950488);
#30924=CIRCLE('',#79995,0.999998640941429);
#30925=CIRCLE('',#79998,0.999998603408247);
#30926=CIRCLE('',#80001,0.999995569663453);
#30927=CIRCLE('',#80003,1.);
#30928=CIRCLE('',#80004,1.);
#30929=CIRCLE('',#80006,67.5);
#30930=CIRCLE('',#80007,1.);
#30931=CIRCLE('',#80009,5.5);
#30932=CIRCLE('',#80011,5.5);
#30933=CIRCLE('',#80013,1.);
#30934=CIRCLE('',#80014,1.);
#30935=CIRCLE('',#80016,20.5);
#30936=CIRCLE('',#80019,1.5);
#30937=CIRCLE('',#80020,1.5);
#30938=CIRCLE('',#80021,10.5003945400646);
#30939=CIRCLE('',#80023,14.);
#30940=CIRCLE('',#80025,15.5);
#30941=CIRCLE('',#80026,15.5);
#30942=CIRCLE('',#80028,1.49990933380908);
#30943=CIRCLE('',#80029,13.99999933141);
#30944=CIRCLE('',#80030,1.4999999963081);
#30945=CIRCLE('',#80032,8.01643786925901);
#30946=CIRCLE('',#80033,1.49999999641083);
#30947=CIRCLE('',#80034,9.516437378118);
#30948=CIRCLE('',#80038,8.33645645579341);
#30949=CIRCLE('',#80043,7.999967894592);
#30950=CIRCLE('',#80046,0.300014002256891);
#30951=CIRCLE('',#80047,0.299999949983396);
#30952=CIRCLE('',#80051,12.0017324877834);
#30953=CIRCLE('',#80052,12.0017324881221);
#30954=CIRCLE('',#80059,0.299999960727201);
#30955=CIRCLE('',#80060,0.300014841061868);
#30956=CIRCLE('',#80065,7.99999976356479);
#30957=CIRCLE('',#80073,1.49999999999999);
#30958=CIRCLE('',#80074,1.50000000099398);
#30959=CIRCLE('',#80076,3.89386562528717);
#30960=CIRCLE('',#80077,1.50004717292849);
#30961=CIRCLE('',#80081,1.50005062266532);
#30962=CIRCLE('',#80083,15.5);
#30963=CIRCLE('',#80084,15.5);
#30964=CIRCLE('',#80085,1.49999999999785);
#30965=CIRCLE('',#80088,5.498378496899);
#30966=CIRCLE('',#80090,4.498380133177);
#30967=CIRCLE('',#80092,14.50000004627);
#30968=CIRCLE('',#80093,0.99996090845702);
#30969=CIRCLE('',#80095,0.999999999999999);
#30970=CIRCLE('',#80096,0.999998041963027);
#30971=CIRCLE('',#80098,14.50000488242);
#30972=CIRCLE('',#80099,1.);
#30973=CIRCLE('',#80102,0.999262032196716);
#30974=CIRCLE('',#80103,0.999999996008301);
#30975=CIRCLE('',#80105,14.50000488338);
#30976=CIRCLE('',#80106,1.00007468229929);
#30977=CIRCLE('',#80107,1.000000000272);
#30978=CIRCLE('',#80110,0.999975226270856);
#30979=CIRCLE('',#80112,14.50000004257);
#30980=CIRCLE('',#80113,0.999999999999993);
#30981=CIRCLE('',#80115,5.498378496898);
#30982=CIRCLE('',#80118,27.6468278765);
#30983=CIRCLE('',#80123,27.64683059909);
#30984=CIRCLE('',#80124,1.5);
#30985=CIRCLE('',#80125,1.5);
#30986=CIRCLE('',#80126,1.5);
#30987=CIRCLE('',#80127,1.50000003977618);
#30988=CIRCLE('',#80128,1.5);
#30989=CIRCLE('',#80129,3.88721692441433);
#30990=CIRCLE('',#80130,1.50002159187886);
#30991=CIRCLE('',#80132,26.64680776781);
#30992=CIRCLE('',#80134,26.64680492934);
#30993=CIRCLE('',#80141,9.50000000000099);
#30994=CIRCLE('',#80144,9.500000000001);
#30995=CIRCLE('',#80145,9.500000000001);
#30996=CIRCLE('',#80147,2.449482268868);
#30997=CIRCLE('',#80148,10.55050311408);
#30998=CIRCLE('',#80149,10.49985738567);
#30999=CIRCLE('',#80151,10.49988903328);
#31000=CIRCLE('',#80152,10.55050536419);
#31001=CIRCLE('',#80153,2.449485998643);
#31002=CIRCLE('',#80155,1.00004538195426);
#31003=CIRCLE('',#80156,11.5);
#31004=CIRCLE('',#80157,0.999999999999998);
#31005=CIRCLE('',#80158,1.00001406525855);
#31006=CIRCLE('',#80161,11.5);
#31007=CIRCLE('',#80164,13.99999938228);
#31008=CIRCLE('',#80166,0.999998820674145);
#31009=CIRCLE('',#80167,1.00000976363729);
#31010=CIRCLE('',#80168,0.999999855249661);
#31011=CIRCLE('',#80171,11.53030601499);
#31012=CIRCLE('',#80172,1.);
#31013=CIRCLE('',#80178,1.5);
#31014=CIRCLE('',#80179,1.5);
#31015=CIRCLE('',#80180,1.5);
#31016=CIRCLE('',#80181,1.469693696648);
#31017=CIRCLE('',#80183,0.999999999999999);
#31018=CIRCLE('',#80185,11.53030595098);
#31019=CIRCLE('',#80187,13.00000023588);
#31020=CIRCLE('',#80191,13.00000024132);
#31021=CIRCLE('',#80193,1.5);
#31022=CIRCLE('',#80195,1.5);
#31023=CIRCLE('',#80196,1.5);
#31024=CIRCLE('',#80200,1.5000306953952);
#31025=CIRCLE('',#80204,1.500000156322);
#31026=CIRCLE('',#80208,10.4988998342525);
#31027=CIRCLE('',#80209,1.5);
#31028=CIRCLE('',#80211,10.49999854524);
#31029=CIRCLE('',#80213,15.);
#31030=CIRCLE('',#80214,15.);
#31031=CIRCLE('',#80215,4.99999999388658);
#31032=CIRCLE('',#80216,4.99999999999388);
#31033=CIRCLE('',#80217,4.99999968198887);
#31034=CIRCLE('',#80218,5.00000000000995);
#31035=CIRCLE('',#80220,5.00000474327103);
#31036=CIRCLE('',#80221,4.99999999999405);
#31037=CIRCLE('',#80222,4.9999996844452);
#31038=CIRCLE('',#80224,4.99999968385975);
#31039=CIRCLE('',#80225,4.99999999999802);
#31040=CIRCLE('',#80226,5.00000000000122);
#31041=CIRCLE('',#80228,40.);
#31042=CIRCLE('',#80229,0.5);
#31043=CIRCLE('',#80230,39.5);
#31044=CIRCLE('',#80231,0.5);
#31045=CIRCLE('',#80232,40.);
#31046=CIRCLE('',#80235,8.);
#31047=CIRCLE('',#80236,8.);
#31048=CIRCLE('',#80238,40.);
#31049=CIRCLE('',#80240,0.5);
#31050=CIRCLE('',#80241,39.5);
#31051=CIRCLE('',#80242,0.500000000000001);
#31052=CIRCLE('',#80243,40.);
#31053=CIRCLE('',#80246,8.);
#31054=CIRCLE('',#80247,8.);
#31055=CIRCLE('',#80248,4.99999999991307);
#31056=CIRCLE('',#80249,5.00000000000412);
#31057=CIRCLE('',#80250,4.9999996846577);
#31058=CIRCLE('',#80251,4.999999999992);
#31059=CIRCLE('',#80252,4.99999999400135);
#31060=CIRCLE('',#80253,4.99999999999915);
#31061=CIRCLE('',#80254,5.00000000000267);
#31062=CIRCLE('',#80255,4.99999968222069);
#31063=CIRCLE('',#80256,4.99999968215304);
#31064=CIRCLE('',#80257,4.99999999999966);
#31065=CIRCLE('',#80259,15.);
#31066=CIRCLE('',#80260,15.);
#31067=CIRCLE('',#80265,7.5);
#31068=CIRCLE('',#80266,0.5);
#31069=CIRCLE('',#80268,29.5);
#31070=CIRCLE('',#80269,30.);
#31071=CIRCLE('',#80271,30.);
#31072=CIRCLE('',#80272,0.500000000000002);
#31073=CIRCLE('',#80273,29.5);
#31074=CIRCLE('',#80275,7.5);
#31075=CIRCLE('',#80278,6.999999985528);
#31076=CIRCLE('',#80280,30.);
#31077=CIRCLE('',#80282,30.);
#31078=CIRCLE('',#80283,6.9999999999976);
#31079=CIRCLE('',#80285,0.500000000000002);
#31080=CIRCLE('',#80286,29.5);
#31081=CIRCLE('',#80288,29.5);
#31082=CIRCLE('',#80289,0.5);
#31083=CIRCLE('',#80291,7.5);
#31084=CIRCLE('',#80293,7.5);
#31085=CIRCLE('',#80296,8.00000000037468);
#31086=CIRCLE('',#80298,6.0000000000044);
#31087=CIRCLE('',#80299,6.00000000004738);
#31088=CIRCLE('',#80300,6.00000000068573);
#31089=CIRCLE('',#80302,5.99998574891701);
#31090=CIRCLE('',#80303,6.00000003035761);
#31091=CIRCLE('',#80305,6.00000000004975);
#31092=CIRCLE('',#80306,6.00000000004976);
#31093=CIRCLE('',#80308,13.);
#31094=CIRCLE('',#80309,13.);
#31095=CIRCLE('',#80314,10.0997825859452);
#31096=CIRCLE('',#80317,1.5);
#31097=CIRCLE('',#80318,1.5);
#31098=CIRCLE('',#80320,1.5);
#31099=CIRCLE('',#80321,31.6373353297717);
#31100=CIRCLE('',#80322,1.500000028483);
#31101=CIRCLE('',#80327,1.5);
#31102=CIRCLE('',#80329,1.5);
#31103=CIRCLE('',#80330,1.5);
#31104=CIRCLE('',#80335,1.500000033965);
#31105=CIRCLE('',#80336,31.6434611407195);
#31106=CIRCLE('',#80337,1.49999999939402);
#31107=CIRCLE('',#80338,1.5);
#31108=CIRCLE('',#80344,1.5);
#31109=CIRCLE('',#80346,0.999995633686306);
#31110=CIRCLE('',#80348,67.5);
#31111=CIRCLE('',#80350,1.5);
#31112=CIRCLE('',#80351,1.5);
#31113=CIRCLE('',#80353,1.5);
#31114=CIRCLE('',#80354,1.5);
#31115=CIRCLE('',#80356,1.5);
#31116=CIRCLE('',#80358,1.);
#31117=CIRCLE('',#80362,1.5);
#31118=CIRCLE('',#80363,10.5004492687665);
#31119=CIRCLE('',#80366,14.);
#31120=CIRCLE('',#80372,1.00000780008503);
#31121=CIRCLE('',#80374,1.49987422447354);
#31122=CIRCLE('',#80377,20.5);
#33580=VERTEX_POINT('',#106598);
#33581=VERTEX_POINT('',#106599);
#33582=VERTEX_POINT('',#106601);
#33583=VERTEX_POINT('',#106603);
#33584=VERTEX_POINT('',#106612);
#33585=VERTEX_POINT('',#106614);
#33586=VERTEX_POINT('',#106653);
#33587=VERTEX_POINT('',#106752);
#33588=VERTEX_POINT('',#106878);
#33589=VERTEX_POINT('',#106879);
#33590=VERTEX_POINT('',#106881);
#33591=VERTEX_POINT('',#106883);
#33592=VERTEX_POINT('',#106927);
#33593=VERTEX_POINT('',#106947);
#33594=VERTEX_POINT('',#106949);
#33595=VERTEX_POINT('',#107028);
#33596=VERTEX_POINT('',#107154);
#33597=VERTEX_POINT('',#107155);
#33598=VERTEX_POINT('',#107168);
#33599=VERTEX_POINT('',#107191);
#33600=VERTEX_POINT('',#107193);
#33601=VERTEX_POINT('',#107206);
#33602=VERTEX_POINT('',#107208);
#33603=VERTEX_POINT('',#107299);
#33604=VERTEX_POINT('',#107300);
#33605=VERTEX_POINT('',#107332);
#33606=VERTEX_POINT('',#107442);
#33607=VERTEX_POINT('',#107577);
#33608=VERTEX_POINT('',#108207);
#33609=VERTEX_POINT('',#108208);
#33610=VERTEX_POINT('',#108210);
#33611=VERTEX_POINT('',#108233);
#33612=VERTEX_POINT('',#108246);
#33613=VERTEX_POINT('',#108253);
#33614=VERTEX_POINT('',#108266);
#33615=VERTEX_POINT('',#108281);
#33616=VERTEX_POINT('',#108282);
#33617=VERTEX_POINT('',#108284);
#33618=VERTEX_POINT('',#108617);
#33619=VERTEX_POINT('',#108635);
#33620=VERTEX_POINT('',#109123);
#33621=VERTEX_POINT('',#109124);
#33622=VERTEX_POINT('',#109126);
#33623=VERTEX_POINT('',#109171);
#33624=VERTEX_POINT('',#109198);
#33625=VERTEX_POINT('',#109253);
#33626=VERTEX_POINT('',#109255);
#33627=VERTEX_POINT('',#109264);
#33628=VERTEX_POINT('',#109324);
#33629=VERTEX_POINT('',#109325);
#33630=VERTEX_POINT('',#109379);
#33631=VERTEX_POINT('',#109439);
#33632=VERTEX_POINT('',#109440);
#33633=VERTEX_POINT('',#109442);
#33634=VERTEX_POINT('',#109455);
#33635=VERTEX_POINT('',#109457);
#33636=VERTEX_POINT('',#109489);
#33637=VERTEX_POINT('',#109490);
#33638=VERTEX_POINT('',#109544);
#33639=VERTEX_POINT('',#109602);
#33640=VERTEX_POINT('',#109603);
#33641=VERTEX_POINT('',#109605);
#33642=VERTEX_POINT('',#109630);
#33643=VERTEX_POINT('',#109679);
#33644=VERTEX_POINT('',#109680);
#33645=VERTEX_POINT('',#109682);
#33646=VERTEX_POINT('',#109723);
#33647=VERTEX_POINT('',#109766);
#33648=VERTEX_POINT('',#109767);
#33649=VERTEX_POINT('',#109994);
#33650=VERTEX_POINT('',#109995);
#33651=VERTEX_POINT('',#110220);
#33652=VERTEX_POINT('',#110221);
#33653=VERTEX_POINT('',#110452);
#33654=VERTEX_POINT('',#110453);
#33655=VERTEX_POINT('',#110455);
#33656=VERTEX_POINT('',#110484);
#33657=VERTEX_POINT('',#110485);
#33658=VERTEX_POINT('',#110487);
#33659=VERTEX_POINT('',#110566);
#33660=VERTEX_POINT('',#110568);
#33661=VERTEX_POINT('',#110647);
#33662=VERTEX_POINT('',#110649);
#33663=VERTEX_POINT('',#110785);
#33664=VERTEX_POINT('',#110786);
#33665=VERTEX_POINT('',#111045);
#33666=VERTEX_POINT('',#111046);
#33667=VERTEX_POINT('',#111048);
#33668=VERTEX_POINT('',#111151);
#33669=VERTEX_POINT('',#111298);
#33670=VERTEX_POINT('',#111300);
#33671=VERTEX_POINT('',#111304);
#33672=VERTEX_POINT('',#111305);
#33673=VERTEX_POINT('',#111307);
#33674=VERTEX_POINT('',#111314);
#33675=VERTEX_POINT('',#111321);
#33676=VERTEX_POINT('',#111330);
#33677=VERTEX_POINT('',#111337);
#33678=VERTEX_POINT('',#111342);
#33679=VERTEX_POINT('',#111349);
#33680=VERTEX_POINT('',#111360);
#33681=VERTEX_POINT('',#111365);
#33682=VERTEX_POINT('',#111367);
#33683=VERTEX_POINT('',#111387);
#33684=VERTEX_POINT('',#111389);
#33685=VERTEX_POINT('',#111394);
#33686=VERTEX_POINT('',#111405);
#33687=VERTEX_POINT('',#111412);
#33688=VERTEX_POINT('',#111417);
#33689=VERTEX_POINT('',#111425);
#33690=VERTEX_POINT('',#111434);
#33691=VERTEX_POINT('',#111448);
#33692=VERTEX_POINT('',#111449);
#33693=VERTEX_POINT('',#111451);
#33694=VERTEX_POINT('',#111453);
#33695=VERTEX_POINT('',#111455);
#33696=VERTEX_POINT('',#111459);
#33697=VERTEX_POINT('',#111460);
#33698=VERTEX_POINT('',#111462);
#33699=VERTEX_POINT('',#111464);
#33700=VERTEX_POINT('',#111481);
#33701=VERTEX_POINT('',#111494);
#33702=VERTEX_POINT('',#111495);
#33703=VERTEX_POINT('',#111497);
#33704=VERTEX_POINT('',#111529);
#33705=VERTEX_POINT('',#111570);
#33706=VERTEX_POINT('',#111574);
#33707=VERTEX_POINT('',#111575);
#33708=VERTEX_POINT('',#111577);
#33709=VERTEX_POINT('',#111579);
#33710=VERTEX_POINT('',#111583);
#33711=VERTEX_POINT('',#111584);
#33712=VERTEX_POINT('',#111586);
#33713=VERTEX_POINT('',#111591);
#33714=VERTEX_POINT('',#111595);
#33715=VERTEX_POINT('',#111596);
#33716=VERTEX_POINT('',#111598);
#33717=VERTEX_POINT('',#111603);
#33718=VERTEX_POINT('',#111607);
#33719=VERTEX_POINT('',#111608);
#33720=VERTEX_POINT('',#111610);
#33721=VERTEX_POINT('',#111612);
#33722=VERTEX_POINT('',#111616);
#33723=VERTEX_POINT('',#111617);
#33724=VERTEX_POINT('',#111624);
#33725=VERTEX_POINT('',#111653);
#33726=VERTEX_POINT('',#111654);
#33727=VERTEX_POINT('',#111716);
#33728=VERTEX_POINT('',#111898);
#33729=VERTEX_POINT('',#111978);
#33730=VERTEX_POINT('',#112004);
#33731=VERTEX_POINT('',#112047);
#33732=VERTEX_POINT('',#112055);
#33733=VERTEX_POINT('',#112234);
#33734=VERTEX_POINT('',#112253);
#33735=VERTEX_POINT('',#112255);
#33736=VERTEX_POINT('',#112258);
#33737=VERTEX_POINT('',#112260);
#33738=VERTEX_POINT('',#112370);
#33739=VERTEX_POINT('',#112451);
#33740=VERTEX_POINT('',#112459);
#33741=VERTEX_POINT('',#112674);
#33742=VERTEX_POINT('',#112703);
#33743=VERTEX_POINT('',#112726);
#33744=VERTEX_POINT('',#112934);
#33745=VERTEX_POINT('',#112935);
#33746=VERTEX_POINT('',#112940);
#33747=VERTEX_POINT('',#112941);
#33748=VERTEX_POINT('',#113000);
#33749=VERTEX_POINT('',#113101);
#33750=VERTEX_POINT('',#113127);
#33751=VERTEX_POINT('',#113129);
#33752=VERTEX_POINT('',#113152);
#33753=VERTEX_POINT('',#113211);
#33754=VERTEX_POINT('',#113312);
#33755=VERTEX_POINT('',#113324);
#33756=VERTEX_POINT('',#113349);
#33757=VERTEX_POINT('',#113350);
#33758=VERTEX_POINT('',#113352);
#33759=VERTEX_POINT('',#113354);
#33760=VERTEX_POINT('',#113356);
#33761=VERTEX_POINT('',#113361);
#33762=VERTEX_POINT('',#113363);
#33763=VERTEX_POINT('',#113370);
#33764=VERTEX_POINT('',#113379);
#33765=VERTEX_POINT('',#113381);
#33766=VERTEX_POINT('',#113383);
#33767=VERTEX_POINT('',#113387);
#33768=VERTEX_POINT('',#113391);
#33769=VERTEX_POINT('',#113393);
#33770=VERTEX_POINT('',#113395);
#33771=VERTEX_POINT('',#113397);
#33772=VERTEX_POINT('',#113410);
#33773=VERTEX_POINT('',#113411);
#33774=VERTEX_POINT('',#113413);
#33775=VERTEX_POINT('',#113428);
#33776=VERTEX_POINT('',#113430);
#33777=VERTEX_POINT('',#113433);
#33778=VERTEX_POINT('',#113450);
#33779=VERTEX_POINT('',#113452);
#33780=VERTEX_POINT('',#113454);
#33781=VERTEX_POINT('',#113458);
#33782=VERTEX_POINT('',#113462);
#33783=VERTEX_POINT('',#113464);
#33784=VERTEX_POINT('',#113468);
#33785=VERTEX_POINT('',#113470);
#33786=VERTEX_POINT('',#113472);
#33787=VERTEX_POINT('',#113474);
#33788=VERTEX_POINT('',#113491);
#33789=VERTEX_POINT('',#113493);
#33790=VERTEX_POINT('',#113495);
#33791=VERTEX_POINT('',#113514);
#33792=VERTEX_POINT('',#113515);
#33793=VERTEX_POINT('',#113518);
#33794=VERTEX_POINT('',#113522);
#33795=VERTEX_POINT('',#113526);
#33796=VERTEX_POINT('',#113527);
#33797=VERTEX_POINT('',#113529);
#33798=VERTEX_POINT('',#113534);
#33799=VERTEX_POINT('',#113535);
#33800=VERTEX_POINT('',#113540);
#33801=VERTEX_POINT('',#113541);
#33802=VERTEX_POINT('',#113543);
#33803=VERTEX_POINT('',#113599);
#33804=VERTEX_POINT('',#113660);
#33805=VERTEX_POINT('',#113661);
#33806=VERTEX_POINT('',#113663);
#33807=VERTEX_POINT('',#113665);
#33808=VERTEX_POINT('',#113926);
#33809=VERTEX_POINT('',#113927);
#33810=VERTEX_POINT('',#113929);
#33811=VERTEX_POINT('',#113936);
#33812=VERTEX_POINT('',#113938);
#33813=VERTEX_POINT('',#113959);
#33814=VERTEX_POINT('',#114226);
#33815=VERTEX_POINT('',#114228);
#33816=VERTEX_POINT('',#114230);
#33817=VERTEX_POINT('',#114234);
#33818=VERTEX_POINT('',#114238);
#33819=VERTEX_POINT('',#114239);
#33820=VERTEX_POINT('',#114274);
#33821=VERTEX_POINT('',#114281);
#33822=VERTEX_POINT('',#114290);
#33823=VERTEX_POINT('',#114319);
#33824=VERTEX_POINT('',#114413);
#33825=VERTEX_POINT('',#114414);
#33826=VERTEX_POINT('',#114461);
#33827=VERTEX_POINT('',#114505);
#33828=VERTEX_POINT('',#114672);
#33829=VERTEX_POINT('',#114812);
#33830=VERTEX_POINT('',#114856);
#33831=VERTEX_POINT('',#114913);
#33832=VERTEX_POINT('',#114916);
#33833=VERTEX_POINT('',#115068);
#33834=VERTEX_POINT('',#115276);
#33835=VERTEX_POINT('',#115277);
#33836=VERTEX_POINT('',#115279);
#33837=VERTEX_POINT('',#115281);
#33838=VERTEX_POINT('',#115283);
#33839=VERTEX_POINT('',#115285);
#33840=VERTEX_POINT('',#115416);
#33841=VERTEX_POINT('',#115457);
#33842=VERTEX_POINT('',#115458);
#33843=VERTEX_POINT('',#115460);
#33844=VERTEX_POINT('',#115462);
#33845=VERTEX_POINT('',#115530);
#33846=VERTEX_POINT('',#115606);
#33847=VERTEX_POINT('',#115608);
#33848=VERTEX_POINT('',#115612);
#33849=VERTEX_POINT('',#115613);
#33850=VERTEX_POINT('',#115615);
#33851=VERTEX_POINT('',#115620);
#33852=VERTEX_POINT('',#115624);
#33853=VERTEX_POINT('',#115625);
#33854=VERTEX_POINT('',#115627);
#33855=VERTEX_POINT('',#115629);
#33856=VERTEX_POINT('',#115634);
#33857=VERTEX_POINT('',#115635);
#33858=VERTEX_POINT('',#115639);
#33859=VERTEX_POINT('',#115643);
#33860=VERTEX_POINT('',#115647);
#33861=VERTEX_POINT('',#115652);
#33862=VERTEX_POINT('',#115656);
#33863=VERTEX_POINT('',#115664);
#33864=VERTEX_POINT('',#115668);
#33865=VERTEX_POINT('',#115669);
#33866=VERTEX_POINT('',#115672);
#33867=VERTEX_POINT('',#115676);
#33868=VERTEX_POINT('',#115680);
#33869=VERTEX_POINT('',#115697);
#33870=VERTEX_POINT('',#115716);
#33871=VERTEX_POINT('',#115718);
#33872=VERTEX_POINT('',#115732);
#33873=VERTEX_POINT('',#115757);
#33874=VERTEX_POINT('',#115764);
#33875=VERTEX_POINT('',#115779);
#33876=VERTEX_POINT('',#115780);
#33877=VERTEX_POINT('',#115827);
#33878=VERTEX_POINT('',#115934);
#33879=VERTEX_POINT('',#116035);
#33880=VERTEX_POINT('',#116092);
#33881=VERTEX_POINT('',#116095);
#33882=VERTEX_POINT('',#116247);
#33883=VERTEX_POINT('',#116273);
#33884=VERTEX_POINT('',#116557);
#33885=VERTEX_POINT('',#116639);
#33886=VERTEX_POINT('',#116640);
#33887=VERTEX_POINT('',#116669);
#33888=VERTEX_POINT('',#116706);
#33889=VERTEX_POINT('',#116708);
#33890=VERTEX_POINT('',#116710);
#33891=VERTEX_POINT('',#116712);
#33892=VERTEX_POINT('',#116716);
#33893=VERTEX_POINT('',#116717);
#33894=VERTEX_POINT('',#116727);
#33895=VERTEX_POINT('',#116747);
#33896=VERTEX_POINT('',#116749);
#33897=VERTEX_POINT('',#116753);
#33898=VERTEX_POINT('',#116755);
#33899=VERTEX_POINT('',#116759);
#33900=VERTEX_POINT('',#116760);
#33901=VERTEX_POINT('',#116762);
#33902=VERTEX_POINT('',#116767);
#33903=VERTEX_POINT('',#116771);
#33904=VERTEX_POINT('',#116772);
#33905=VERTEX_POINT('',#116774);
#33906=VERTEX_POINT('',#116776);
#33907=VERTEX_POINT('',#116781);
#33908=VERTEX_POINT('',#116782);
#33909=VERTEX_POINT('',#116786);
#33910=VERTEX_POINT('',#116790);
#33911=VERTEX_POINT('',#116794);
#33912=VERTEX_POINT('',#116799);
#33913=VERTEX_POINT('',#116803);
#33914=VERTEX_POINT('',#116811);
#33915=VERTEX_POINT('',#116815);
#33916=VERTEX_POINT('',#116816);
#33917=VERTEX_POINT('',#116818);
#33918=VERTEX_POINT('',#116820);
#33919=VERTEX_POINT('',#116822);
#33920=VERTEX_POINT('',#116824);
#33921=VERTEX_POINT('',#116842);
#33922=VERTEX_POINT('',#116843);
#33923=VERTEX_POINT('',#116845);
#33924=VERTEX_POINT('',#116847);
#33925=VERTEX_POINT('',#116882);
#33926=VERTEX_POINT('',#116883);
#33927=VERTEX_POINT('',#116945);
#33928=VERTEX_POINT('',#117049);
#33929=VERTEX_POINT('',#117051);
#33930=VERTEX_POINT('',#117060);
#33931=VERTEX_POINT('',#117062);
#33932=VERTEX_POINT('',#117108);
#33933=VERTEX_POINT('',#117112);
#33934=VERTEX_POINT('',#117114);
#33935=VERTEX_POINT('',#117116);
#33936=VERTEX_POINT('',#117171);
#33937=VERTEX_POINT('',#117230);
#33938=VERTEX_POINT('',#117299);
#33939=VERTEX_POINT('',#117356);
#33940=VERTEX_POINT('',#117360);
#33941=VERTEX_POINT('',#117361);
#33942=VERTEX_POINT('',#117406);
#33943=VERTEX_POINT('',#117407);
#33944=VERTEX_POINT('',#117489);
#33945=VERTEX_POINT('',#117490);
#33946=VERTEX_POINT('',#117503);
#33947=VERTEX_POINT('',#117505);
#33948=VERTEX_POINT('',#117510);
#33949=VERTEX_POINT('',#117512);
#33950=VERTEX_POINT('',#117615);
#33951=VERTEX_POINT('',#117616);
#33952=VERTEX_POINT('',#117680);
#33953=VERTEX_POINT('',#117775);
#33954=VERTEX_POINT('',#117913);
#33955=VERTEX_POINT('',#117922);
#33956=VERTEX_POINT('',#118017);
#33957=VERTEX_POINT('',#118198);
#33958=VERTEX_POINT('',#118200);
#33959=VERTEX_POINT('',#118202);
#33960=VERTEX_POINT('',#118206);
#33961=VERTEX_POINT('',#118210);
#33962=VERTEX_POINT('',#118211);
#33963=VERTEX_POINT('',#118239);
#33964=VERTEX_POINT('',#118363);
#33965=VERTEX_POINT('',#118539);
#33966=VERTEX_POINT('',#118720);
#33967=VERTEX_POINT('',#118957);
#33968=VERTEX_POINT('',#118959);
#33969=VERTEX_POINT('',#118963);
#33970=VERTEX_POINT('',#118970);
#33971=VERTEX_POINT('',#118996);
#33972=VERTEX_POINT('',#119000);
#33973=VERTEX_POINT('',#119359);
#33974=VERTEX_POINT('',#119361);
#33975=VERTEX_POINT('',#119365);
#33976=VERTEX_POINT('',#119369);
#33977=VERTEX_POINT('',#119498);
#33978=VERTEX_POINT('',#119625);
#33979=VERTEX_POINT('',#119650);
#33980=VERTEX_POINT('',#119771);
#33981=VERTEX_POINT('',#119805);
#33982=VERTEX_POINT('',#119870);
#33983=VERTEX_POINT('',#119872);
#33984=VERTEX_POINT('',#119913);
#33985=VERTEX_POINT('',#119973);
#33986=VERTEX_POINT('',#120090);
#33987=VERTEX_POINT('',#120386);
#33988=VERTEX_POINT('',#120452);
#33989=VERTEX_POINT('',#120536);
#33990=VERTEX_POINT('',#120635);
#33991=VERTEX_POINT('',#121905);
#33992=VERTEX_POINT('',#121906);
#33993=VERTEX_POINT('',#122084);
#33994=VERTEX_POINT('',#122356);
#33995=VERTEX_POINT('',#122649);
#33996=VERTEX_POINT('',#123070);
#33997=VERTEX_POINT('',#123593);
#33998=VERTEX_POINT('',#123594);
#33999=VERTEX_POINT('',#123596);
#34000=VERTEX_POINT('',#123598);
#34001=VERTEX_POINT('',#123600);
#34002=VERTEX_POINT('',#123602);
#34003=VERTEX_POINT('',#123651);
#34004=VERTEX_POINT('',#123652);
#34005=VERTEX_POINT('',#123702);
#34006=VERTEX_POINT('',#123741);
#34007=VERTEX_POINT('',#123742);
#34008=VERTEX_POINT('',#123744);
#34009=VERTEX_POINT('',#123746);
#34010=VERTEX_POINT('',#123809);
#34011=VERTEX_POINT('',#123910);
#34012=VERTEX_POINT('',#123912);
#34013=VERTEX_POINT('',#124096);
#34014=VERTEX_POINT('',#124097);
#34015=VERTEX_POINT('',#124099);
#34016=VERTEX_POINT('',#124261);
#34017=VERTEX_POINT('',#124262);
#34018=VERTEX_POINT('',#124360);
#34019=VERTEX_POINT('',#124361);
#34020=VERTEX_POINT('',#124363);
#34021=VERTEX_POINT('',#124365);
#34022=VERTEX_POINT('',#124420);
#34023=VERTEX_POINT('',#124421);
#34024=VERTEX_POINT('',#124432);
#34025=VERTEX_POINT('',#124434);
#34026=VERTEX_POINT('',#124461);
#34027=VERTEX_POINT('',#124468);
#34028=VERTEX_POINT('',#124534);
#34029=VERTEX_POINT('',#124655);
#34030=VERTEX_POINT('',#124659);
#34031=VERTEX_POINT('',#124660);
#34032=VERTEX_POINT('',#124707);
#34033=VERTEX_POINT('',#124714);
#34034=VERTEX_POINT('',#124718);
#34035=VERTEX_POINT('',#124725);
#34036=VERTEX_POINT('',#124842);
#34037=VERTEX_POINT('',#125047);
#34038=VERTEX_POINT('',#125048);
#34039=VERTEX_POINT('',#125109);
#34040=VERTEX_POINT('',#125110);
#34041=VERTEX_POINT('',#125115);
#34042=VERTEX_POINT('',#125410);
#34043=VERTEX_POINT('',#125412);
#34044=VERTEX_POINT('',#125416);
#34045=VERTEX_POINT('',#125509);
#34046=VERTEX_POINT('',#125685);
#34047=VERTEX_POINT('',#125893);
#34048=VERTEX_POINT('',#125898);
#34049=VERTEX_POINT('',#125963);
#34050=VERTEX_POINT('',#125965);
#34051=VERTEX_POINT('',#125967);
#34052=VERTEX_POINT('',#125971);
#34053=VERTEX_POINT('',#125975);
#34054=VERTEX_POINT('',#125976);
#34055=VERTEX_POINT('',#126216);
#34056=VERTEX_POINT('',#126218);
#34057=VERTEX_POINT('',#126222);
#34058=VERTEX_POINT('',#126226);
#34059=VERTEX_POINT('',#126230);
#34060=VERTEX_POINT('',#126357);
#34061=VERTEX_POINT('',#126372);
#34062=VERTEX_POINT('',#126389);
#34063=VERTEX_POINT('',#126411);
#34064=VERTEX_POINT('',#126533);
#34065=VERTEX_POINT('',#126611);
#34066=VERTEX_POINT('',#126613);
#34067=VERTEX_POINT('',#126618);
#34068=VERTEX_POINT('',#126730);
#34069=VERTEX_POINT('',#126973);
#34070=VERTEX_POINT('',#127057);
#34071=VERTEX_POINT('',#127144);
#34072=VERTEX_POINT('',#127205);
#34073=VERTEX_POINT('',#127390);
#34074=VERTEX_POINT('',#128608);
#34075=VERTEX_POINT('',#128623);
#34076=VERTEX_POINT('',#128692);
#34077=VERTEX_POINT('',#128798);
#34078=VERTEX_POINT('',#129092);
#34079=VERTEX_POINT('',#129503);
#34080=VERTEX_POINT('',#130321);
#34081=VERTEX_POINT('',#130322);
#34082=VERTEX_POINT('',#130324);
#34083=VERTEX_POINT('',#130326);
#34084=VERTEX_POINT('',#130328);
#34085=VERTEX_POINT('',#130330);
#34086=VERTEX_POINT('',#130332);
#34087=VERTEX_POINT('',#130334);
#34088=VERTEX_POINT('',#130336);
#34089=VERTEX_POINT('',#130340);
#34090=VERTEX_POINT('',#130341);
#34091=VERTEX_POINT('',#130343);
#34092=VERTEX_POINT('',#130345);
#34093=VERTEX_POINT('',#130347);
#34094=VERTEX_POINT('',#130349);
#34095=VERTEX_POINT('',#130351);
#34096=VERTEX_POINT('',#130353);
#34097=VERTEX_POINT('',#130355);
#34098=VERTEX_POINT('',#130359);
#34099=VERTEX_POINT('',#130361);
#34100=VERTEX_POINT('',#130365);
#34101=VERTEX_POINT('',#130367);
#34102=VERTEX_POINT('',#130371);
#34103=VERTEX_POINT('',#130373);
#34104=VERTEX_POINT('',#130375);
#34105=VERTEX_POINT('',#130403);
#34106=VERTEX_POINT('',#130404);
#34107=VERTEX_POINT('',#130406);
#34108=VERTEX_POINT('',#130460);
#34109=VERTEX_POINT('',#130543);
#34110=VERTEX_POINT('',#130577);
#34111=VERTEX_POINT('',#130582);
#34112=VERTEX_POINT('',#130596);
#34113=VERTEX_POINT('',#130598);
#34114=VERTEX_POINT('',#130600);
#34115=VERTEX_POINT('',#130613);
#34116=VERTEX_POINT('',#130615);
#34117=VERTEX_POINT('',#130827);
#34118=VERTEX_POINT('',#131000);
#34119=VERTEX_POINT('',#131010);
#34120=VERTEX_POINT('',#131015);
#34121=VERTEX_POINT('',#131017);
#34122=VERTEX_POINT('',#131030);
#34123=VERTEX_POINT('',#131032);
#34124=VERTEX_POINT('',#131034);
#34125=VERTEX_POINT('',#131053);
#34126=VERTEX_POINT('',#131157);
#34127=VERTEX_POINT('',#131159);
#34128=VERTEX_POINT('',#131161);
#34129=VERTEX_POINT('',#131189);
#34130=VERTEX_POINT('',#131191);
#34131=VERTEX_POINT('',#131258);
#34132=VERTEX_POINT('',#131314);
#34133=VERTEX_POINT('',#131322);
#34134=VERTEX_POINT('',#131324);
#34135=VERTEX_POINT('',#131348);
#34136=VERTEX_POINT('',#131350);
#34137=VERTEX_POINT('',#131524);
#34138=VERTEX_POINT('',#131535);
#34139=VERTEX_POINT('',#131582);
#34140=VERTEX_POINT('',#131584);
#34141=VERTEX_POINT('',#131865);
#34142=VERTEX_POINT('',#131876);
#34143=VERTEX_POINT('',#131880);
#34144=VERTEX_POINT('',#131891);
#34145=VERTEX_POINT('',#132049);
#34146=VERTEX_POINT('',#132056);
#34147=VERTEX_POINT('',#132383);
#34148=VERTEX_POINT('',#132385);
#34149=VERTEX_POINT('',#132487);
#34150=VERTEX_POINT('',#132489);
#34151=VERTEX_POINT('',#132585);
#34152=VERTEX_POINT('',#132586);
#34153=VERTEX_POINT('',#132588);
#34154=VERTEX_POINT('',#132727);
#34155=VERTEX_POINT('',#132847);
#34156=VERTEX_POINT('',#132848);
#34157=VERTEX_POINT('',#132850);
#34158=VERTEX_POINT('',#132915);
#34159=VERTEX_POINT('',#132916);
#34160=VERTEX_POINT('',#132918);
#34161=VERTEX_POINT('',#132965);
#34162=VERTEX_POINT('',#133060);
#34163=VERTEX_POINT('',#133061);
#34164=VERTEX_POINT('',#133090);
#34165=VERTEX_POINT('',#133153);
#34166=VERTEX_POINT('',#133154);
#34167=VERTEX_POINT('',#133156);
#34168=VERTEX_POINT('',#133206);
#34169=VERTEX_POINT('',#133211);
#34170=VERTEX_POINT('',#133213);
#34171=VERTEX_POINT('',#133248);
#34172=VERTEX_POINT('',#133322);
#34173=VERTEX_POINT('',#133333);
#34174=VERTEX_POINT('',#133377);
#34175=VERTEX_POINT('',#133414);
#34176=VERTEX_POINT('',#133452);
#34177=VERTEX_POINT('',#133458);
#34178=VERTEX_POINT('',#133468);
#34179=VERTEX_POINT('',#133469);
#34180=VERTEX_POINT('',#133471);
#34181=VERTEX_POINT('',#133474);
#34182=VERTEX_POINT('',#133608);
#34183=VERTEX_POINT('',#133771);
#34184=VERTEX_POINT('',#133848);
#34185=VERTEX_POINT('',#133979);
#34186=VERTEX_POINT('',#134347);
#34187=VERTEX_POINT('',#134348);
#34188=VERTEX_POINT('',#134410);
#34189=VERTEX_POINT('',#134412);
#34190=VERTEX_POINT('',#134435);
#34191=VERTEX_POINT('',#134437);
#34192=VERTEX_POINT('',#134562);
#34193=VERTEX_POINT('',#134564);
#34194=VERTEX_POINT('',#134569);
#34195=VERTEX_POINT('',#134582);
#34196=VERTEX_POINT('',#134584);
#34197=VERTEX_POINT('',#134696);
#34198=VERTEX_POINT('',#134698);
#34199=VERTEX_POINT('',#134702);
#34200=VERTEX_POINT('',#134707);
#34201=VERTEX_POINT('',#134709);
#34202=VERTEX_POINT('',#134711);
#34203=VERTEX_POINT('',#134715);
#34204=VERTEX_POINT('',#134904);
#34205=VERTEX_POINT('',#135034);
#34206=VERTEX_POINT('',#135062);
#34207=VERTEX_POINT('',#135215);
#34208=VERTEX_POINT('',#135220);
#34209=VERTEX_POINT('',#135395);
#34210=VERTEX_POINT('',#135397);
#34211=VERTEX_POINT('',#135399);
#34212=VERTEX_POINT('',#135576);
#34213=VERTEX_POINT('',#135605);
#34214=VERTEX_POINT('',#135607);
#34215=VERTEX_POINT('',#135611);
#34216=VERTEX_POINT('',#135613);
#34217=VERTEX_POINT('',#135615);
#34218=VERTEX_POINT('',#135617);
#34219=VERTEX_POINT('',#135621);
#34220=VERTEX_POINT('',#135622);
#34221=VERTEX_POINT('',#135624);
#34222=VERTEX_POINT('',#135626);
#34223=VERTEX_POINT('',#135628);
#34224=VERTEX_POINT('',#135632);
#34225=VERTEX_POINT('',#135643);
#34226=VERTEX_POINT('',#136405);
#34227=VERTEX_POINT('',#136521);
#34228=VERTEX_POINT('',#136819);
#34229=VERTEX_POINT('',#136834);
#34230=VERTEX_POINT('',#137188);
#34231=VERTEX_POINT('',#137834);
#34232=VERTEX_POINT('',#137847);
#34233=VERTEX_POINT('',#137849);
#34234=VERTEX_POINT('',#137881);
#34235=VERTEX_POINT('',#137894);
#34236=VERTEX_POINT('',#137896);
#34237=VERTEX_POINT('',#137933);
#34238=VERTEX_POINT('',#138649);
#34239=VERTEX_POINT('',#138665);
#34240=VERTEX_POINT('',#138667);
#34241=VERTEX_POINT('',#138704);
#34242=VERTEX_POINT('',#138940);
#34243=VERTEX_POINT('',#138986);
#34244=VERTEX_POINT('',#139024);
#34245=VERTEX_POINT('',#139065);
#34246=VERTEX_POINT('',#139067);
#34247=VERTEX_POINT('',#139142);
#34248=VERTEX_POINT('',#139466);
#34249=VERTEX_POINT('',#139468);
#34250=VERTEX_POINT('',#140049);
#34251=VERTEX_POINT('',#140176);
#34252=VERTEX_POINT('',#140244);
#34253=VERTEX_POINT('',#140440);
#34254=VERTEX_POINT('',#140441);
#34255=VERTEX_POINT('',#140536);
#34256=VERTEX_POINT('',#140547);
#34257=VERTEX_POINT('',#140593);
#34258=VERTEX_POINT('',#140648);
#34259=VERTEX_POINT('',#140698);
#34260=VERTEX_POINT('',#140705);
#34261=VERTEX_POINT('',#140806);
#34262=VERTEX_POINT('',#140904);
#34263=VERTEX_POINT('',#140911);
#34264=VERTEX_POINT('',#140964);
#34265=VERTEX_POINT('',#141028);
#34266=VERTEX_POINT('',#141094);
#34267=VERTEX_POINT('',#141096);
#34268=VERTEX_POINT('',#141402);
#34269=VERTEX_POINT('',#141461);
#34270=VERTEX_POINT('',#141478);
#34271=VERTEX_POINT('',#142789);
#34272=VERTEX_POINT('',#142794);
#34273=VERTEX_POINT('',#142796);
#34274=VERTEX_POINT('',#142939);
#34275=VERTEX_POINT('',#142941);
#34276=VERTEX_POINT('',#142964);
#34277=VERTEX_POINT('',#142966);
#34278=VERTEX_POINT('',#143053);
#34279=VERTEX_POINT('',#143055);
#34280=VERTEX_POINT('',#143110);
#34281=VERTEX_POINT('',#143240);
#34282=VERTEX_POINT('',#143251);
#34283=VERTEX_POINT('',#143256);
#34284=VERTEX_POINT('',#143263);
#34285=VERTEX_POINT('',#143301);
#34286=VERTEX_POINT('',#143310);
#34287=VERTEX_POINT('',#143353);
#34288=VERTEX_POINT('',#143480);
#34289=VERTEX_POINT('',#143523);
#34290=VERTEX_POINT('',#143584);
#34291=VERTEX_POINT('',#143688);
#34292=VERTEX_POINT('',#143748);
#34293=VERTEX_POINT('',#143791);
#34294=VERTEX_POINT('',#143852);
#34295=VERTEX_POINT('',#143895);
#34296=VERTEX_POINT('',#143971);
#34297=VERTEX_POINT('',#143975);
#34298=VERTEX_POINT('',#143984);
#34299=VERTEX_POINT('',#143993);
#34300=VERTEX_POINT('',#144003);
#34301=VERTEX_POINT('',#144004);
#34302=VERTEX_POINT('',#144011);
#34303=VERTEX_POINT('',#144020);
#34304=VERTEX_POINT('',#144056);
#34305=VERTEX_POINT('',#144096);
#34306=VERTEX_POINT('',#144122);
#34307=VERTEX_POINT('',#144159);
#34308=VERTEX_POINT('',#144173);
#34309=VERTEX_POINT('',#144210);
#34310=VERTEX_POINT('',#144326);
#34311=VERTEX_POINT('',#144331);
#34312=VERTEX_POINT('',#144372);
#34313=VERTEX_POINT('',#144374);
#34314=VERTEX_POINT('',#144545);
#34315=VERTEX_POINT('',#144682);
#34316=VERTEX_POINT('',#144873);
#34317=VERTEX_POINT('',#144950);
#34318=VERTEX_POINT('',#145130);
#34319=VERTEX_POINT('',#145256);
#34320=VERTEX_POINT('',#145296);
#34321=VERTEX_POINT('',#145304);
#34322=VERTEX_POINT('',#145333);
#34323=VERTEX_POINT('',#145362);
#34324=VERTEX_POINT('',#145408);
#34325=VERTEX_POINT('',#145409);
#34326=VERTEX_POINT('',#145413);
#34327=VERTEX_POINT('',#145414);
#34328=VERTEX_POINT('',#145416);
#34329=VERTEX_POINT('',#145499);
#34330=VERTEX_POINT('',#145501);
#34331=VERTEX_POINT('',#145575);
#34332=VERTEX_POINT('',#145590);
#34333=VERTEX_POINT('',#145594);
#34334=VERTEX_POINT('',#145596);
#34335=VERTEX_POINT('',#145598);
#34336=VERTEX_POINT('',#145600);
#34337=VERTEX_POINT('',#145619);
#34338=VERTEX_POINT('',#145621);
#34339=VERTEX_POINT('',#145627);
#34340=VERTEX_POINT('',#145629);
#34341=VERTEX_POINT('',#145633);
#34342=VERTEX_POINT('',#145635);
#34343=VERTEX_POINT('',#145702);
#34344=VERTEX_POINT('',#145799);
#34345=VERTEX_POINT('',#145833);
#34346=VERTEX_POINT('',#145835);
#34347=VERTEX_POINT('',#145855);
#34348=VERTEX_POINT('',#145886);
#34349=VERTEX_POINT('',#146034);
#34350=VERTEX_POINT('',#146167);
#34351=VERTEX_POINT('',#146226);
#34352=VERTEX_POINT('',#146298);
#34353=VERTEX_POINT('',#146300);
#34354=VERTEX_POINT('',#146311);
#34355=VERTEX_POINT('',#146321);
#34356=VERTEX_POINT('',#146332);
#34357=VERTEX_POINT('',#146334);
#34358=VERTEX_POINT('',#146342);
#34359=VERTEX_POINT('',#146352);
#34360=VERTEX_POINT('',#146363);
#34361=VERTEX_POINT('',#146365);
#34362=VERTEX_POINT('',#146369);
#34363=VERTEX_POINT('',#146461);
#34364=VERTEX_POINT('',#146508);
#34365=VERTEX_POINT('',#146609);
#34366=VERTEX_POINT('',#146611);
#34367=VERTEX_POINT('',#146617);
#34368=VERTEX_POINT('',#146657);
#34369=VERTEX_POINT('',#146908);
#34370=VERTEX_POINT('',#146912);
#34371=VERTEX_POINT('',#146913);
#34372=VERTEX_POINT('',#146915);
#34373=VERTEX_POINT('',#146959);
#34374=VERTEX_POINT('',#147097);
#34375=VERTEX_POINT('',#147114);
#34376=VERTEX_POINT('',#147263);
#34377=VERTEX_POINT('',#147265);
#34378=VERTEX_POINT('',#147400);
#34379=VERTEX_POINT('',#147407);
#34380=VERTEX_POINT('',#147443);
#34381=VERTEX_POINT('',#147450);
#34382=VERTEX_POINT('',#147573);
#34383=VERTEX_POINT('',#147576);
#34384=VERTEX_POINT('',#147611);
#34385=VERTEX_POINT('',#147713);
#34386=VERTEX_POINT('',#147715);
#34387=VERTEX_POINT('',#147782);
#34388=VERTEX_POINT('',#147783);
#34389=VERTEX_POINT('',#148079);
#34390=VERTEX_POINT('',#148248);
#34391=VERTEX_POINT('',#148253);
#34392=VERTEX_POINT('',#148450);
#34393=VERTEX_POINT('',#148456);
#34394=VERTEX_POINT('',#148485);
#34395=VERTEX_POINT('',#148486);
#34396=VERTEX_POINT('',#148488);
#34397=VERTEX_POINT('',#148499);
#34398=VERTEX_POINT('',#148501);
#34399=VERTEX_POINT('',#148506);
#34400=VERTEX_POINT('',#148558);
#34401=VERTEX_POINT('',#148560);
#34402=VERTEX_POINT('',#148582);
#34403=VERTEX_POINT('',#148644);
#34404=VERTEX_POINT('',#148765);
#34405=VERTEX_POINT('',#149134);
#34406=VERTEX_POINT('',#149207);
#34407=VERTEX_POINT('',#149528);
#34408=VERTEX_POINT('',#149580);
#34409=VERTEX_POINT('',#149623);
#34410=VERTEX_POINT('',#149726);
#34411=VERTEX_POINT('',#149817);
#34412=VERTEX_POINT('',#149819);
#34413=VERTEX_POINT('',#149821);
#34414=VERTEX_POINT('',#149823);
#34415=VERTEX_POINT('',#149829);
#34416=VERTEX_POINT('',#149864);
#34417=VERTEX_POINT('',#149866);
#34418=VERTEX_POINT('',#149868);
#34419=VERTEX_POINT('',#149953);
#34420=VERTEX_POINT('',#149955);
#34421=VERTEX_POINT('',#149959);
#34422=VERTEX_POINT('',#149960);
#34423=VERTEX_POINT('',#149984);
#34424=VERTEX_POINT('',#149985);
#34425=VERTEX_POINT('',#150075);
#34426=VERTEX_POINT('',#150077);
#34427=VERTEX_POINT('',#150079);
#34428=VERTEX_POINT('',#150083);
#34429=VERTEX_POINT('',#150084);
#34430=VERTEX_POINT('',#150147);
#34431=VERTEX_POINT('',#150149);
#34432=VERTEX_POINT('',#150151);
#34433=VERTEX_POINT('',#150201);
#34434=VERTEX_POINT('',#150203);
#34435=VERTEX_POINT('',#150256);
#34436=VERTEX_POINT('',#150276);
#34437=VERTEX_POINT('',#150278);
#34438=VERTEX_POINT('',#150407);
#34439=VERTEX_POINT('',#150618);
#34440=VERTEX_POINT('',#150706);
#34441=VERTEX_POINT('',#150803);
#34442=VERTEX_POINT('',#150831);
#34443=VERTEX_POINT('',#150853);
#34444=VERTEX_POINT('',#150955);
#34445=VERTEX_POINT('',#151163);
#34446=VERTEX_POINT('',#151353);
#34447=VERTEX_POINT('',#151361);
#34448=VERTEX_POINT('',#151702);
#34449=VERTEX_POINT('',#151881);
#34450=VERTEX_POINT('',#152219);
#34451=VERTEX_POINT('',#152430);
#34452=VERTEX_POINT('',#152887);
#34453=VERTEX_POINT('',#153252);
#34454=VERTEX_POINT('',#153256);
#34455=VERTEX_POINT('',#153281);
#34456=VERTEX_POINT('',#153443);
#34457=VERTEX_POINT('',#153674);
#34458=VERTEX_POINT('',#153685);
#34459=VERTEX_POINT('',#153863);
#34460=VERTEX_POINT('',#153874);
#34461=VERTEX_POINT('',#153984);
#34462=VERTEX_POINT('',#154098);
#34463=VERTEX_POINT('',#154116);
#34464=VERTEX_POINT('',#154194);
#34465=VERTEX_POINT('',#154222);
#34466=VERTEX_POINT('',#154250);
#34467=VERTEX_POINT('',#154331);
#34468=VERTEX_POINT('',#154338);
#34469=VERTEX_POINT('',#154404);
#34470=VERTEX_POINT('',#154514);
#34471=VERTEX_POINT('',#154628);
#34472=VERTEX_POINT('',#154827);
#34473=VERTEX_POINT('',#154830);
#34474=VERTEX_POINT('',#154834);
#34475=VERTEX_POINT('',#154840);
#34476=VERTEX_POINT('',#154950);
#34477=VERTEX_POINT('',#154957);
#34478=VERTEX_POINT('',#154965);
#34479=VERTEX_POINT('',#155003);
#34480=VERTEX_POINT('',#155075);
#34481=VERTEX_POINT('',#155148);
#34482=VERTEX_POINT('',#155153);
#34483=VERTEX_POINT('',#155483);
#34484=VERTEX_POINT('',#155617);
#34485=VERTEX_POINT('',#155721);
#34486=VERTEX_POINT('',#155980);
#34487=VERTEX_POINT('',#156250);
#34488=VERTEX_POINT('',#156807);
#34489=VERTEX_POINT('',#156865);
#34490=VERTEX_POINT('',#156998);
#34491=VERTEX_POINT('',#157254);
#34492=VERTEX_POINT('',#157362);
#41069=EDGE_CURVE('',#33580,#33581,#30630,.T.);
#41070=EDGE_CURVE('',#33582,#33581,#30631,.T.);
#41071=EDGE_CURVE('',#33583,#33582,#30632,.T.);
#41072=EDGE_CURVE('',#33580,#33583,#29387,.T.);
#41073=EDGE_CURVE('',#33581,#33584,#2701,.T.);
#41074=EDGE_CURVE('',#33584,#33585,#2702,.T.);
#41075=EDGE_CURVE('',#33585,#33581,#2634,.T.);
#41076=EDGE_CURVE('',#33583,#33586,#29388,.T.);
#41077=EDGE_CURVE('',#33586,#33582,#29389,.T.);
#41078=EDGE_CURVE('',#33587,#33582,#29390,.T.);
#41079=EDGE_CURVE('',#33587,#33586,#29391,.T.);
#41080=EDGE_CURVE('',#33587,#33585,#29392,.T.);
#41081=EDGE_CURVE('',#33584,#33580,#29393,.T.);
#41082=EDGE_CURVE('',#33588,#33589,#30633,.T.);
#41083=EDGE_CURVE('',#33590,#33589,#30634,.T.);
#41084=EDGE_CURVE('',#33591,#33590,#30635,.T.);
#41085=EDGE_CURVE('',#33588,#33591,#29394,.T.);
#41086=EDGE_CURVE('',#33592,#33588,#29395,.T.);
#41087=EDGE_CURVE('',#33589,#33592,#29396,.T.);
#41088=EDGE_CURVE('',#33590,#33593,#2635,.T.);
#41089=EDGE_CURVE('',#33593,#33594,#2703,.T.);
#41090=EDGE_CURVE('',#33594,#33590,#2704,.T.);
#41091=EDGE_CURVE('',#33593,#33595,#29397,.T.);
#41092=EDGE_CURVE('',#33589,#33595,#29398,.T.);
#41093=EDGE_CURVE('',#33592,#33595,#29399,.T.);
#41094=EDGE_CURVE('',#33591,#33594,#29400,.T.);
#41095=EDGE_CURVE('',#33596,#33597,#29401,.T.);
#41096=EDGE_CURVE('',#33596,#33598,#29402,.T.);
#41097=EDGE_CURVE('',#33599,#33598,#30636,.T.);
#41098=EDGE_CURVE('',#33599,#33600,#29403,.T.);
#41099=EDGE_CURVE('',#33601,#33600,#2705,.T.);
#41100=EDGE_CURVE('',#33601,#33602,#29404,.T.);
#41101=EDGE_CURVE('',#33597,#33602,#29405,.T.);
#41102=EDGE_CURVE('',#33603,#33604,#29406,.T.);
#41103=EDGE_CURVE('',#33605,#33604,#29407,.T.);
#41104=EDGE_CURVE('',#33606,#33605,#29408,.T.);
#41105=EDGE_CURVE('',#33606,#33603,#29409,.T.);
#41106=EDGE_CURVE('',#33607,#33605,#29410,.T.);
#41107=EDGE_CURVE('',#33607,#33606,#29411,.T.);
#41108=EDGE_CURVE('',#33599,#33607,#2706,.T.);
#41109=EDGE_CURVE('',#33600,#33605,#2707,.T.);
#41110=EDGE_CURVE('',#33604,#33601,#29412,.T.);
#41111=EDGE_CURVE('',#33603,#33602,#29413,.T.);
#41112=EDGE_CURVE('',#33597,#33603,#30637,.T.);
#41113=EDGE_CURVE('',#33596,#33606,#29414,.T.);
#41114=EDGE_CURVE('',#33598,#33607,#29415,.T.);
#41115=EDGE_CURVE('',#33608,#33609,#30638,.T.);
#41116=EDGE_CURVE('',#33608,#33610,#29416,.T.);
#41117=EDGE_CURVE('',#33611,#33610,#29417,.T.);
#41118=EDGE_CURVE('',#33612,#33611,#29418,.T.);
#41119=EDGE_CURVE('',#33612,#33613,#29419,.T.);
#41120=EDGE_CURVE('',#33614,#33613,#2708,.T.);
#41121=EDGE_CURVE('',#33614,#33609,#29420,.T.);
#41122=EDGE_CURVE('',#33615,#33616,#30639,.T.);
#41123=EDGE_CURVE('',#33617,#33616,#29421,.T.);
#41124=EDGE_CURVE('',#33617,#33615,#29422,.T.);
#41125=EDGE_CURVE('',#33618,#33616,#29423,.T.);
#41126=EDGE_CURVE('',#33619,#33618,#29424,.T.);
#41127=EDGE_CURVE('',#33619,#33617,#29425,.T.);
#41128=EDGE_CURVE('',#33612,#33619,#29426,.T.);
#41129=EDGE_CURVE('',#33613,#33618,#29427,.T.);
#41130=EDGE_CURVE('',#33616,#33614,#2709,.T.);
#41131=EDGE_CURVE('',#33615,#33609,#2710,.T.);
#41132=EDGE_CURVE('',#33611,#33619,#30640,.T.);
#41133=EDGE_CURVE('',#33617,#33610,#29428,.T.);
#41134=EDGE_CURVE('',#33615,#33608,#29429,.T.);
#41135=EDGE_CURVE('',#33620,#33621,#2711,.T.);
#41136=EDGE_CURVE('',#33620,#33622,#29430,.T.);
#41137=EDGE_CURVE('',#33622,#33623,#30641,.T.);
#41138=EDGE_CURVE('',#33623,#33621,#29431,.T.);
#41139=EDGE_CURVE('',#33621,#33624,#29432,.T.);
#41140=EDGE_CURVE('',#33625,#33624,#2712,.T.);
#41141=EDGE_CURVE('',#33625,#33626,#29433,.T.);
#41142=EDGE_CURVE('',#33626,#33627,#29434,.T.);
#41143=EDGE_CURVE('',#33627,#33620,#29435,.T.);
#41144=EDGE_CURVE('',#33628,#33629,#2713,.T.);
#41145=EDGE_CURVE('',#33628,#33625,#29436,.T.);
#41146=EDGE_CURVE('',#33624,#33630,#29437,.T.);
#41147=EDGE_CURVE('',#33630,#33629,#29438,.T.);
#41148=EDGE_CURVE('',#33631,#33632,#2714,.T.);
#41149=EDGE_CURVE('',#33632,#33633,#29439,.T.);
#41150=EDGE_CURVE('',#33634,#33633,#30642,.T.);
#41151=EDGE_CURVE('',#33635,#33634,#29440,.T.);
#41152=EDGE_CURVE('',#33631,#33635,#29441,.F.);
#41153=EDGE_CURVE('',#33636,#33637,#2715,.T.);
#41154=EDGE_CURVE('',#33637,#33632,#29442,.T.);
#41155=EDGE_CURVE('',#33638,#33631,#29443,.F.);
#41156=EDGE_CURVE('',#33638,#33636,#29444,.T.);
#41157=EDGE_CURVE('',#33639,#33640,#2716,.T.);
#41158=EDGE_CURVE('',#33639,#33641,#29445,.T.);
#41159=EDGE_CURVE('',#33641,#33642,#30643,.T.);
#41160=EDGE_CURVE('',#33640,#33642,#29446,.F.);
#41161=EDGE_CURVE('',#33643,#33644,#2717,.T.);
#41162=EDGE_CURVE('',#33644,#33645,#29447,.T.);
#41163=EDGE_CURVE('',#33646,#33645,#2718,.T.);
#41164=EDGE_CURVE('',#33646,#33643,#29448,.T.);
#41165=EDGE_CURVE('',#33647,#33648,#2719,.T.);
#41166=EDGE_CURVE('',#33648,#33644,#29449,.T.);
#41167=EDGE_CURVE('',#33643,#33647,#29450,.T.);
#41168=EDGE_CURVE('',#33649,#33650,#2720,.T.);
#41169=EDGE_CURVE('',#33650,#33648,#29451,.T.);
#41170=EDGE_CURVE('',#33647,#33649,#29452,.T.);
#41171=EDGE_CURVE('',#33651,#33652,#2721,.T.);
#41172=EDGE_CURVE('',#33652,#33650,#29453,.T.);
#41173=EDGE_CURVE('',#33649,#33651,#29454,.T.);
#41174=EDGE_CURVE('',#33653,#33654,#2722,.T.);
#41175=EDGE_CURVE('',#33653,#33655,#30644,.T.);
#41176=EDGE_CURVE('',#33655,#33654,#29455,.T.);
#41177=EDGE_CURVE('',#33656,#33657,#2723,.T.);
#41178=EDGE_CURVE('',#33657,#33658,#29456,.T.);
#41179=EDGE_CURVE('',#33659,#33658,#2724,.T.);
#41180=EDGE_CURVE('',#33659,#33660,#29457,.T.);
#41181=EDGE_CURVE('',#33660,#33661,#2725,.T.);
#41182=EDGE_CURVE('',#33661,#33662,#30645,.T.);
#41183=EDGE_CURVE('',#33662,#33661,#30646,.T.);
#41184=EDGE_CURVE('',#33660,#33656,#29458,.T.);
#41185=EDGE_CURVE('',#33663,#33664,#2726,.T.);
#41186=EDGE_CURVE('',#33664,#33657,#29459,.T.);
#41187=EDGE_CURVE('',#33656,#33663,#29460,.T.);
#41188=EDGE_CURVE('',#33665,#33666,#2727,.T.);
#41189=EDGE_CURVE('',#33665,#33667,#29461,.T.);
#41190=EDGE_CURVE('',#33667,#33668,#30647,.T.);
#41191=EDGE_CURVE('',#33668,#33666,#29462,.T.);
#41192=EDGE_CURVE('',#33669,#33669,#30648,.T.);
#41193=EDGE_CURVE('',#33669,#33670,#30649,.T.);
#41194=EDGE_CURVE('',#33670,#33670,#30650,.T.);
#41195=EDGE_CURVE('',#33671,#33672,#30651,.T.);
#41196=EDGE_CURVE('',#33673,#33671,#29463,.T.);
#41197=EDGE_CURVE('',#33674,#33673,#29464,.T.);
#41198=EDGE_CURVE('',#33675,#33674,#29465,.T.);
#41199=EDGE_CURVE('',#33675,#33676,#29466,.T.);
#41200=EDGE_CURVE('',#33676,#33677,#29467,.T.);
#41201=EDGE_CURVE('',#33678,#33677,#29468,.T.);
#41202=EDGE_CURVE('',#33678,#33679,#29469,.T.);
#41203=EDGE_CURVE('',#33679,#33680,#29470,.T.);
#41204=EDGE_CURVE('',#33681,#33680,#30652,.T.);
#41205=EDGE_CURVE('',#33682,#33681,#29471,.F.);
#41206=EDGE_CURVE('',#33683,#33682,#30653,.T.);
#41207=EDGE_CURVE('',#33683,#33684,#29472,.T.);
#41208=EDGE_CURVE('',#33684,#33685,#29473,.T.);
#41209=EDGE_CURVE('',#33686,#33685,#29474,.T.);
#41210=EDGE_CURVE('',#33686,#33687,#29475,.T.);
#41211=EDGE_CURVE('',#33687,#33688,#29476,.T.);
#41212=EDGE_CURVE('',#33689,#33688,#29477,.T.);
#41213=EDGE_CURVE('',#33690,#33689,#29478,.T.);
#41214=EDGE_CURVE('',#33672,#33690,#29479,.T.);
#41215=EDGE_CURVE('',#33691,#33692,#30654,.T.);
#41216=EDGE_CURVE('',#33692,#33693,#30655,.T.);
#41217=EDGE_CURVE('',#33692,#33694,#30656,.T.);
#41218=EDGE_CURVE('',#33694,#33695,#30657,.T.);
#41219=EDGE_CURVE('',#33691,#33695,#30658,.T.);
#41220=EDGE_CURVE('',#33696,#33697,#30659,.T.);
#41221=EDGE_CURVE('',#33698,#33696,#2728,.T.);
#41222=EDGE_CURVE('',#33699,#33698,#29480,.T.);
#41223=EDGE_CURVE('',#33700,#33699,#29481,.T.);
#41224=EDGE_CURVE('',#33700,#33697,#2729,.T.);
#41225=EDGE_CURVE('',#33701,#33702,#30660,.T.);
#41226=EDGE_CURVE('',#33702,#33703,#29482,.T.);
#41227=EDGE_CURVE('',#33704,#33703,#29483,.T.);
#41228=EDGE_CURVE('',#33705,#33704,#30661,.T.);
#41229=EDGE_CURVE('',#33701,#33705,#30662,.T.);
#41230=EDGE_CURVE('',#33706,#33707,#30663,.T.);
#41231=EDGE_CURVE('',#33707,#33708,#2730,.T.);
#41232=EDGE_CURVE('',#33709,#33708,#30664,.T.);
#41233=EDGE_CURVE('',#33706,#33709,#2731,.T.);
#41234=EDGE_CURVE('',#33710,#33711,#30665,.T.);
#41235=EDGE_CURVE('',#33710,#33712,#2732,.T.);
#41236=EDGE_CURVE('',#33712,#33712,#30666,.T.);
#41237=EDGE_CURVE('',#33711,#33710,#30667,.T.);
#41238=EDGE_CURVE('',#33713,#33713,#30668,.T.);
#41239=EDGE_CURVE('',#33713,#33711,#30669,.T.);
#41240=EDGE_CURVE('',#33714,#33715,#30670,.T.);
#41241=EDGE_CURVE('',#33714,#33716,#2733,.T.);
#41242=EDGE_CURVE('',#33716,#33716,#30671,.T.);
#41243=EDGE_CURVE('',#33715,#33714,#30672,.T.);
#41244=EDGE_CURVE('',#33717,#33717,#30673,.T.);
#41245=EDGE_CURVE('',#33717,#33715,#30674,.T.);
#41246=EDGE_CURVE('',#33718,#33719,#30675,.T.);
#41247=EDGE_CURVE('',#33719,#33720,#30676,.T.);
#41248=EDGE_CURVE('',#33721,#33720,#30677,.T.);
#41249=EDGE_CURVE('',#33721,#33718,#30678,.T.);
#41250=EDGE_CURVE('',#33722,#33723,#29484,.T.);
#41251=EDGE_CURVE('',#33724,#33722,#29485,.T.);
#41252=EDGE_CURVE('',#33719,#33724,#2734,.T.);
#41253=EDGE_CURVE('',#33718,#33723,#2735,.T.);
#41254=EDGE_CURVE('',#33725,#33726,#29486,.T.);
#41255=EDGE_CURVE('',#33727,#33726,#29487,.T.);
#41256=EDGE_CURVE('',#33727,#33728,#29488,.T.);
#41257=EDGE_CURVE('',#33728,#33729,#29489,.T.);
#41258=EDGE_CURVE('',#33729,#33730,#29490,.T.);
#41259=EDGE_CURVE('',#33730,#33731,#29491,.T.);
#41260=EDGE_CURVE('',#33732,#33731,#29492,.T.);
#41261=EDGE_CURVE('',#33733,#33732,#29493,.T.);
#41262=EDGE_CURVE('',#33733,#33734,#2636,.T.);
#41263=EDGE_CURVE('',#33734,#33735,#2736,.T.);
#41264=EDGE_CURVE('',#33735,#33735,#30679,.T.);
#41265=EDGE_CURVE('',#33734,#33736,#2637,.T.);
#41266=EDGE_CURVE('',#33737,#33736,#29494,.T.);
#41267=EDGE_CURVE('',#33738,#33737,#29495,.T.);
#41268=EDGE_CURVE('',#33738,#33739,#29496,.T.);
#41269=EDGE_CURVE('',#33740,#33739,#29497,.T.);
#41270=EDGE_CURVE('',#33740,#33741,#29498,.T.);
#41271=EDGE_CURVE('',#33741,#33742,#29499,.T.);
#41272=EDGE_CURVE('',#33743,#33742,#29500,.T.);
#41273=EDGE_CURVE('',#33743,#33725,#29501,.T.);
#41274=EDGE_CURVE('',#33744,#33745,#30680,.T.);
#41275=EDGE_CURVE('',#33744,#33696,#30681,.T.);
#41276=EDGE_CURVE('',#33697,#33745,#30682,.T.);
#41277=EDGE_CURVE('',#33746,#33747,#29502,.T.);
#41278=EDGE_CURVE('',#33747,#33748,#29503,.T.);
#41279=EDGE_CURVE('',#33748,#33749,#29504,.T.);
#41280=EDGE_CURVE('',#33750,#33749,#2737,.T.);
#41281=EDGE_CURVE('',#33750,#33751,#29505,.T.);
#41282=EDGE_CURVE('',#33751,#33752,#29506,.T.);
#41283=EDGE_CURVE('',#33752,#33753,#29507,.T.);
#41284=EDGE_CURVE('',#33753,#33754,#29508,.T.);
#41285=EDGE_CURVE('',#33755,#33754,#2738,.T.);
#41286=EDGE_CURVE('',#33755,#33746,#29509,.T.);
#41287=EDGE_CURVE('',#33756,#33757,#30683,.T.);
#41288=EDGE_CURVE('',#33757,#33758,#30684,.T.);
#41289=EDGE_CURVE('',#33757,#33759,#30685,.T.);
#41290=EDGE_CURVE('',#33759,#33760,#30686,.T.);
#41291=EDGE_CURVE('',#33756,#33760,#30687,.T.);
#41292=EDGE_CURVE('',#33707,#33706,#30688,.T.);
#41293=EDGE_CURVE('',#33707,#33761,#2739,.T.);
#41294=EDGE_CURVE('',#33762,#33761,#29510,.F.);
#41295=EDGE_CURVE('',#33762,#33763,#30689,.T.);
#41296=EDGE_CURVE('',#33761,#33763,#29511,.F.);
#41297=EDGE_CURVE('',#33764,#33764,#30690,.T.);
#41298=EDGE_CURVE('',#33764,#33765,#30691,.T.);
#41299=EDGE_CURVE('',#33765,#33766,#30692,.T.);
#41300=EDGE_CURVE('',#33766,#33765,#30693,.T.);
#41301=EDGE_CURVE('',#33766,#33767,#2740,.T.);
#41302=EDGE_CURVE('',#33767,#33767,#30694,.T.);
#41303=EDGE_CURVE('',#33768,#33768,#30695,.T.);
#41304=EDGE_CURVE('',#33768,#33769,#2741,.T.);
#41305=EDGE_CURVE('',#33769,#33770,#30696,.T.);
#41306=EDGE_CURVE('',#33771,#33770,#29512,.T.);
#41307=EDGE_CURVE('',#33771,#33769,#30697,.T.);
#41308=EDGE_CURVE('',#33772,#33773,#30698,.T.);
#41309=EDGE_CURVE('',#33774,#33773,#29513,.T.);
#41310=EDGE_CURVE('',#33775,#33774,#30699,.T.);
#41311=EDGE_CURVE('',#33775,#33776,#2742,.T.);
#41312=EDGE_CURVE('',#33776,#33776,#30700,.T.);
#41313=EDGE_CURVE('',#33777,#33775,#30701,.T.);
#41314=EDGE_CURVE('',#33772,#33777,#29514,.T.);
#41315=EDGE_CURVE('',#33778,#33778,#30702,.T.);
#41316=EDGE_CURVE('',#33778,#33779,#2743,.T.);
#41317=EDGE_CURVE('',#33779,#33780,#30703,.T.);
#41318=EDGE_CURVE('',#33780,#33779,#30704,.T.);
#41319=EDGE_CURVE('',#33780,#33781,#2744,.T.);
#41320=EDGE_CURVE('',#33781,#33781,#30705,.T.);
#41321=EDGE_CURVE('',#33782,#33782,#30706,.T.);
#41322=EDGE_CURVE('',#33782,#33783,#2745,.T.);
#41323=EDGE_CURVE('',#33783,#33783,#30707,.T.);
#41324=EDGE_CURVE('',#33784,#33784,#30708,.T.);
#41325=EDGE_CURVE('',#33784,#33785,#2746,.T.);
#41326=EDGE_CURVE('',#33786,#33785,#2638,.T.);
#41327=EDGE_CURVE('',#33787,#33786,#1729,.T.);
#41328=EDGE_CURVE('',#33788,#33787,#2639,.T.);
#41329=EDGE_CURVE('',#33789,#33788,#2640,.T.);
#41330=EDGE_CURVE('',#33790,#33789,#1730,.T.);
#41331=EDGE_CURVE('',#33785,#33790,#2641,.T.);
#41332=EDGE_CURVE('',#33791,#33792,#30709,.T.);
#41333=EDGE_CURVE('',#33792,#33791,#30710,.T.);
#41334=EDGE_CURVE('',#33792,#33793,#30711,.T.);
#41335=EDGE_CURVE('',#33793,#33793,#30712,.T.);
#41336=EDGE_CURVE('',#33794,#33794,#30713,.T.);
#41337=EDGE_CURVE('',#33794,#33791,#2747,.T.);
#41338=EDGE_CURVE('',#33795,#33796,#30714,.T.);
#41339=EDGE_CURVE('',#33795,#33797,#2748,.T.);
#41340=EDGE_CURVE('',#33797,#33797,#30715,.T.);
#41341=EDGE_CURVE('',#33796,#33795,#30716,.T.);
#41342=EDGE_CURVE('',#33798,#33799,#30717,.T.);
#41343=EDGE_CURVE('',#33799,#33798,#30718,.T.);
#41344=EDGE_CURVE('',#33799,#33796,#2749,.T.);
#41345=EDGE_CURVE('',#33800,#33801,#2642,.T.);
#41346=EDGE_CURVE('',#33801,#33802,#29515,.T.);
#41347=EDGE_CURVE('',#33803,#33802,#30719,.T.);
#41348=EDGE_CURVE('',#33803,#33800,#29516,.T.);
#41349=EDGE_CURVE('',#33804,#33805,#30720,.T.);
#41350=EDGE_CURVE('',#33805,#33806,#2750,.T.);
#41351=EDGE_CURVE('',#33806,#33807,#30721,.T.);
#41352=EDGE_CURVE('',#33807,#33804,#2751,.T.);
#41353=EDGE_CURVE('',#33666,#33664,#29517,.T.);
#41354=EDGE_CURVE('',#33663,#33665,#29518,.T.);
#41355=EDGE_CURVE('',#33808,#33809,#30722,.T.);
#41356=EDGE_CURVE('',#33809,#33810,#2752,.T.);
#41357=EDGE_CURVE('',#33810,#33810,#30723,.T.);
#41358=EDGE_CURVE('',#33809,#33808,#30724,.T.);
#41359=EDGE_CURVE('',#33808,#33662,#2753,.T.);
#41360=EDGE_CURVE('',#33811,#33653,#30725,.T.);
#41361=EDGE_CURVE('',#33812,#33811,#29519,.F.);
#41362=EDGE_CURVE('',#33812,#33813,#2754,.T.);
#41363=EDGE_CURVE('',#33813,#33813,#30726,.T.);
#41364=EDGE_CURVE('',#33668,#33812,#29520,.F.);
#41365=EDGE_CURVE('',#33655,#33667,#29521,.T.);
#41366=EDGE_CURVE('',#33654,#33652,#29522,.T.);
#41367=EDGE_CURVE('',#33651,#33811,#29523,.T.);
#41368=EDGE_CURVE('',#33814,#33814,#30727,.T.);
#41369=EDGE_CURVE('',#33814,#33815,#30728,.T.);
#41370=EDGE_CURVE('',#33815,#33816,#30729,.T.);
#41371=EDGE_CURVE('',#33816,#33815,#30730,.T.);
#41372=EDGE_CURVE('',#33816,#33817,#2755,.T.);
#41373=EDGE_CURVE('',#33817,#33817,#30731,.T.);
#41374=EDGE_CURVE('',#33818,#33819,#29524,.T.);
#41375=EDGE_CURVE('',#33642,#33818,#29525,.T.);
#41376=EDGE_CURVE('',#33820,#33641,#29526,.T.);
#41377=EDGE_CURVE('',#33821,#33820,#29527,.T.);
#41378=EDGE_CURVE('',#33819,#33821,#30732,.T.);
#41379=EDGE_CURVE('',#33822,#33640,#29528,.F.);
#41380=EDGE_CURVE('',#33822,#33823,#29529,.T.);
#41381=EDGE_CURVE('',#33823,#33637,#29530,.T.);
#41382=EDGE_CURVE('',#33636,#33639,#29531,.T.);
#41383=EDGE_CURVE('',#33824,#33825,#29532,.T.);
#41384=EDGE_CURVE('',#33825,#33826,#29533,.T.);
#41385=EDGE_CURVE('',#33826,#33827,#29534,.T.);
#41386=EDGE_CURVE('',#33827,#33828,#29535,.T.);
#41387=EDGE_CURVE('',#33828,#33829,#29536,.T.);
#41388=EDGE_CURVE('',#33829,#33830,#29537,.T.);
#41389=EDGE_CURVE('',#33830,#33831,#2756,.T.);
#41390=EDGE_CURVE('',#33831,#33831,#30733,.T.);
#41391=EDGE_CURVE('',#33830,#33832,#29538,.T.);
#41392=EDGE_CURVE('',#33832,#33833,#29539,.T.);
#41393=EDGE_CURVE('',#33833,#33824,#29540,.T.);
#41394=EDGE_CURVE('',#33834,#33835,#30734,.T.);
#41395=EDGE_CURVE('',#33834,#33836,#2757,.T.);
#41396=EDGE_CURVE('',#33837,#33836,#30735,.T.);
#41397=EDGE_CURVE('',#33837,#33838,#2758,.T.);
#41398=EDGE_CURVE('',#33838,#33839,#29541,.T.);
#41399=EDGE_CURVE('',#33839,#33840,#29542,.T.);
#41400=EDGE_CURVE('',#33840,#33835,#2759,.T.);
#41401=EDGE_CURVE('',#33841,#33842,#30736,.T.);
#41402=EDGE_CURVE('',#33843,#33842,#2760,.T.);
#41403=EDGE_CURVE('',#33844,#33843,#29543,.T.);
#41404=EDGE_CURVE('',#33845,#33844,#29544,.T.);
#41405=EDGE_CURVE('',#33845,#33841,#2761,.T.);
#41406=EDGE_CURVE('',#33846,#33846,#30737,.T.);
#41407=EDGE_CURVE('',#33846,#33847,#2762,.T.);
#41408=EDGE_CURVE('',#33847,#33847,#30738,.T.);
#41409=EDGE_CURVE('',#33848,#33849,#30739,.T.);
#41410=EDGE_CURVE('',#33849,#33850,#2763,.T.);
#41411=EDGE_CURVE('',#33850,#33850,#30740,.T.);
#41412=EDGE_CURVE('',#33849,#33848,#30741,.T.);
#41413=EDGE_CURVE('',#33848,#33851,#2764,.T.);
#41414=EDGE_CURVE('',#33851,#33851,#30742,.T.);
#41415=EDGE_CURVE('',#33852,#33853,#30743,.T.);
#41416=EDGE_CURVE('',#33853,#33854,#2765,.T.);
#41417=EDGE_CURVE('',#33855,#33854,#30744,.T.);
#41418=EDGE_CURVE('',#33854,#33855,#30745,.T.);
#41419=EDGE_CURVE('',#33853,#33852,#30746,.T.);
#41420=EDGE_CURVE('',#33856,#33857,#1731,.T.);
#41421=EDGE_CURVE('',#33858,#33856,#1732,.T.);
#41422=EDGE_CURVE('',#33859,#33858,#1733,.T.);
#41423=EDGE_CURVE('',#33860,#33859,#1734,.F.);
#41424=EDGE_CURVE('',#33860,#33855,#2766,.T.);
#41425=EDGE_CURVE('',#33861,#33860,#1735,.F.);
#41426=EDGE_CURVE('',#33862,#33861,#1736,.T.);
#41427=EDGE_CURVE('',#33857,#33862,#1737,.T.);
#41428=EDGE_CURVE('',#33852,#33863,#2767,.T.);
#41429=EDGE_CURVE('',#33863,#33863,#30747,.T.);
#41430=EDGE_CURVE('',#33864,#33865,#30748,.T.);
#41431=EDGE_CURVE('',#33865,#33864,#30749,.T.);
#41432=EDGE_CURVE('',#33864,#33866,#30750,.T.);
#41433=EDGE_CURVE('',#33866,#33866,#30751,.T.);
#41434=EDGE_CURVE('',#33867,#33867,#30752,.T.);
#41435=EDGE_CURVE('',#33867,#33865,#2768,.T.);
#41436=EDGE_CURVE('',#33868,#33622,#29545,.T.);
#41437=EDGE_CURVE('',#33869,#33868,#29546,.T.);
#41438=EDGE_CURVE('',#33870,#33869,#30753,.T.);
#41439=EDGE_CURVE('',#33871,#33870,#29547,.T.);
#41440=EDGE_CURVE('',#33623,#33871,#29548,.T.);
#41441=EDGE_CURVE('',#33629,#33872,#29549,.T.);
#41442=EDGE_CURVE('',#33873,#33872,#29550,.T.);
#41443=EDGE_CURVE('',#33874,#33873,#30754,.T.);
#41444=EDGE_CURVE('',#33874,#33628,#29551,.T.);
#41445=EDGE_CURVE('',#33875,#33876,#29552,.T.);
#41446=EDGE_CURVE('',#33876,#33877,#29553,.T.);
#41447=EDGE_CURVE('',#33877,#33878,#29554,.T.);
#41448=EDGE_CURVE('',#33878,#33879,#29555,.T.);
#41449=EDGE_CURVE('',#33879,#33880,#2769,.T.);
#41450=EDGE_CURVE('',#33880,#33880,#30755,.T.);
#41451=EDGE_CURVE('',#33879,#33881,#29556,.T.);
#41452=EDGE_CURVE('',#33881,#33882,#29557,.T.);
#41453=EDGE_CURVE('',#33882,#33883,#29558,.T.);
#41454=EDGE_CURVE('',#33883,#33884,#29559,.T.);
#41455=EDGE_CURVE('',#33884,#33875,#29560,.T.);
#41456=EDGE_CURVE('',#33885,#33886,#29561,.T.);
#41457=EDGE_CURVE('',#33886,#33887,#29562,.T.);
#41458=EDGE_CURVE('',#33887,#33888,#2770,.T.);
#41459=EDGE_CURVE('',#33889,#33888,#30756,.T.);
#41460=EDGE_CURVE('',#33889,#33890,#2771,.T.);
#41461=EDGE_CURVE('',#33891,#33890,#30757,.T.);
#41462=EDGE_CURVE('',#33891,#33885,#2772,.T.);
#41463=EDGE_CURVE('',#33892,#33893,#1738,.T.);
#41464=EDGE_CURVE('',#33894,#33892,#29563,.T.);
#41465=EDGE_CURVE('',#33895,#33894,#2773,.T.);
#41466=EDGE_CURVE('',#33895,#33896,#30758,.T.);
#41467=EDGE_CURVE('',#33896,#33893,#2774,.T.);
#41468=EDGE_CURVE('',#33897,#33897,#30759,.T.);
#41469=EDGE_CURVE('',#33897,#33898,#2775,.T.);
#41470=EDGE_CURVE('',#33898,#33898,#30760,.T.);
#41471=EDGE_CURVE('',#33899,#33900,#30761,.T.);
#41472=EDGE_CURVE('',#33900,#33901,#2776,.T.);
#41473=EDGE_CURVE('',#33901,#33901,#30762,.T.);
#41474=EDGE_CURVE('',#33900,#33899,#30763,.T.);
#41475=EDGE_CURVE('',#33899,#33902,#2777,.T.);
#41476=EDGE_CURVE('',#33902,#33902,#30764,.T.);
#41477=EDGE_CURVE('',#33903,#33904,#30765,.T.);
#41478=EDGE_CURVE('',#33904,#33905,#2778,.T.);
#41479=EDGE_CURVE('',#33906,#33905,#30766,.T.);
#41480=EDGE_CURVE('',#33905,#33906,#30767,.T.);
#41481=EDGE_CURVE('',#33904,#33903,#30768,.T.);
#41482=EDGE_CURVE('',#33907,#33908,#1739,.T.);
#41483=EDGE_CURVE('',#33909,#33907,#1740,.T.);
#41484=EDGE_CURVE('',#33910,#33909,#1741,.T.);
#41485=EDGE_CURVE('',#33911,#33910,#1742,.F.);
#41486=EDGE_CURVE('',#33911,#33906,#2779,.T.);
#41487=EDGE_CURVE('',#33912,#33911,#1743,.F.);
#41488=EDGE_CURVE('',#33913,#33912,#1744,.T.);
#41489=EDGE_CURVE('',#33908,#33913,#1745,.T.);
#41490=EDGE_CURVE('',#33903,#33914,#2780,.T.);
#41491=EDGE_CURVE('',#33914,#33914,#30769,.T.);
#41492=EDGE_CURVE('',#33915,#33916,#2781,.T.);
#41493=EDGE_CURVE('',#33916,#33917,#2782,.T.);
#41494=EDGE_CURVE('',#33917,#33918,#2783,.T.);
#41495=EDGE_CURVE('',#33918,#33919,#2784,.T.);
#41496=EDGE_CURVE('',#33919,#33920,#2785,.T.);
#41497=EDGE_CURVE('',#33920,#33915,#2786,.T.);
#41498=EDGE_CURVE('',#33915,#33909,#2787,.T.);
#41499=EDGE_CURVE('',#33916,#33907,#2788,.T.);
#41500=EDGE_CURVE('',#33917,#33908,#2789,.T.);
#41501=EDGE_CURVE('',#33918,#33913,#2790,.T.);
#41502=EDGE_CURVE('',#33919,#33912,#2791,.T.);
#41503=EDGE_CURVE('',#33920,#33910,#2792,.T.);
#41504=EDGE_CURVE('',#33921,#33922,#2793,.T.);
#41505=EDGE_CURVE('',#33921,#33923,#30770,.T.);
#41506=EDGE_CURVE('',#33923,#33924,#2794,.T.);
#41507=EDGE_CURVE('',#33924,#33922,#30771,.T.);
#41508=EDGE_CURVE('',#33925,#33926,#29564,.T.);
#41509=EDGE_CURVE('',#33925,#33927,#29565,.T.);
#41510=EDGE_CURVE('',#33927,#33926,#29566,.T.);
#41511=EDGE_CURVE('',#33928,#33893,#30772,.T.);
#41512=EDGE_CURVE('',#33928,#33929,#29567,.T.);
#41513=EDGE_CURVE('',#33929,#33894,#30773,.T.);
#41514=EDGE_CURVE('',#33923,#33930,#30774,.T.);
#41515=EDGE_CURVE('',#33930,#33931,#29568,.T.);
#41516=EDGE_CURVE('',#33924,#33931,#29569,.T.);
#41517=EDGE_CURVE('',#33932,#33922,#30775,.T.);
#41518=EDGE_CURVE('',#33924,#33932,#30776,.T.);
#41519=EDGE_CURVE('',#33921,#33933,#2795,.T.);
#41520=EDGE_CURVE('',#33922,#33934,#2796,.T.);
#41521=EDGE_CURVE('',#33934,#33935,#2643,.T.);
#41522=EDGE_CURVE('',#33935,#33933,#2797,.T.);
#41523=EDGE_CURVE('',#33936,#33934,#29570,.T.);
#41524=EDGE_CURVE('',#33937,#33936,#29571,.T.);
#41525=EDGE_CURVE('',#33937,#33934,#30777,.T.);
#41526=EDGE_CURVE('',#33938,#33937,#29572,.T.);
#41527=EDGE_CURVE('',#33938,#33935,#29573,.T.);
#41528=EDGE_CURVE('',#33938,#33939,#2798,.T.);
#41529=EDGE_CURVE('',#33939,#33933,#30778,.T.);
#41530=EDGE_CURVE('',#33940,#33941,#30779,.T.);
#41531=EDGE_CURVE('',#33941,#33930,#29574,.T.);
#41532=EDGE_CURVE('',#33939,#33940,#2799,.T.);
#41533=EDGE_CURVE('',#33942,#33943,#30780,.T.);
#41534=EDGE_CURVE('',#33943,#33927,#1746,.T.);
#41535=EDGE_CURVE('',#33942,#33925,#29575,.T.);
#41536=EDGE_CURVE('',#33944,#33945,#29576,.T.);
#41537=EDGE_CURVE('',#33946,#33944,#2800,.T.);
#41538=EDGE_CURVE('',#33947,#33946,#30781,.T.);
#41539=EDGE_CURVE('',#33947,#33945,#2801,.T.);
#41540=EDGE_CURVE('',#33944,#33940,#2802,.T.);
#41541=EDGE_CURVE('',#33948,#33945,#30782,.T.);
#41542=EDGE_CURVE('',#33948,#33949,#29577,.T.);
#41543=EDGE_CURVE('',#33929,#33949,#29578,.T.);
#41544=EDGE_CURVE('',#33941,#33928,#29579,.T.);
#41545=EDGE_CURVE('',#33925,#33948,#29580,.T.);
#41546=EDGE_CURVE('',#33926,#33949,#1747,.T.);
#41547=EDGE_CURVE('',#33950,#33951,#30783,.T.);
#41548=EDGE_CURVE('',#33951,#33943,#2803,.T.);
#41549=EDGE_CURVE('',#33950,#33942,#2804,.T.);
#41550=EDGE_CURVE('',#33952,#33943,#29581,.T.);
#41551=EDGE_CURVE('',#33953,#33952,#30784,.T.);
#41552=EDGE_CURVE('',#33926,#33953,#29582,.T.);
#41553=EDGE_CURVE('',#33954,#33952,#29583,.T.);
#41554=EDGE_CURVE('',#33955,#33954,#30785,.T.);
#41555=EDGE_CURVE('',#33955,#33953,#29584,.T.);
#41556=EDGE_CURVE('',#33953,#33956,#30786,.T.);
#41557=EDGE_CURVE('',#33956,#33894,#29585,.T.);
#41558=EDGE_CURVE('',#33957,#33895,#30787,.T.);
#41559=EDGE_CURVE('',#33958,#33895,#30788,.T.);
#41560=EDGE_CURVE('',#33959,#33958,#30789,.T.);
#41561=EDGE_CURVE('',#33959,#33957,#30790,.T.);
#41562=EDGE_CURVE('',#33960,#33896,#30791,.T.);
#41563=EDGE_CURVE('',#33957,#33960,#30792,.T.);
#41564=EDGE_CURVE('',#33961,#33962,#30793,.T.);
#41565=EDGE_CURVE('',#33896,#33962,#30794,.T.);
#41566=EDGE_CURVE('',#33960,#33961,#30795,.T.);
#41567=EDGE_CURVE('',#33893,#33963,#29586,.T.);
#41568=EDGE_CURVE('',#33931,#33963,#30796,.T.);
#41569=EDGE_CURVE('',#33963,#33964,#29587,.T.);
#41570=EDGE_CURVE('',#33965,#33964,#1748,.T.);
#41571=EDGE_CURVE('',#33931,#33965,#29588,.T.);
#41572=EDGE_CURVE('',#33965,#33966,#29589,.T.);
#41573=EDGE_CURVE('',#33932,#33966,#29590,.T.);
#41574=EDGE_CURVE('',#33932,#33936,#2805,.T.);
#41575=EDGE_CURVE('',#33936,#33967,#30797,.T.);
#41576=EDGE_CURVE('',#33967,#33968,#30798,.T.);
#41577=EDGE_CURVE('',#33938,#33968,#30799,.T.);
#41578=EDGE_CURVE('',#33968,#33969,#30800,.T.);
#41579=EDGE_CURVE('',#33969,#33946,#30801,.T.);
#41580=EDGE_CURVE('',#33890,#33946,#30802,.T.);
#41581=EDGE_CURVE('',#33890,#33947,#30803,.T.);
#41582=EDGE_CURVE('',#33970,#33947,#2806,.T.);
#41583=EDGE_CURVE('',#33970,#33950,#29591,.T.);
#41584=EDGE_CURVE('',#33970,#33971,#30804,.T.);
#41585=EDGE_CURVE('',#33971,#33951,#30805,.T.);
#41586=EDGE_CURVE('',#33951,#33972,#30806,.T.);
#41587=EDGE_CURVE('',#33972,#33954,#30807,.T.);
#41588=EDGE_CURVE('',#33889,#33971,#29592,.T.);
#41589=EDGE_CURVE('',#33889,#33970,#29593,.T.);
#41590=EDGE_CURVE('',#33888,#33972,#30808,.T.);
#41591=EDGE_CURVE('',#33888,#33955,#30809,.T.);
#41592=EDGE_CURVE('',#33955,#33956,#29594,.T.);
#41593=EDGE_CURVE('',#33958,#33956,#2807,.T.);
#41594=EDGE_CURVE('',#33973,#33958,#30810,.T.);
#41595=EDGE_CURVE('',#33974,#33973,#30811,.T.);
#41596=EDGE_CURVE('',#33974,#33959,#30812,.T.);
#41597=EDGE_CURVE('',#33975,#33974,#30813,.T.);
#41598=EDGE_CURVE('',#33961,#33975,#30814,.T.);
#41599=EDGE_CURVE('',#33975,#33976,#30815,.T.);
#41600=EDGE_CURVE('',#33962,#33976,#30816,.T.);
#41601=EDGE_CURVE('',#33964,#33962,#2808,.T.);
#41602=EDGE_CURVE('',#33964,#33966,#29595,.T.);
#41603=EDGE_CURVE('',#33967,#33966,#2809,.T.);
#41604=EDGE_CURVE('',#33891,#33969,#30817,.T.);
#41605=EDGE_CURVE('',#33967,#33891,#30818,.T.);
#41606=EDGE_CURVE('',#33887,#33977,#29596,.T.);
#41607=EDGE_CURVE('',#33973,#33977,#2810,.T.);
#41608=EDGE_CURVE('',#33977,#33978,#29597,.T.);
#41609=EDGE_CURVE('',#33978,#33973,#30819,.T.);
#41610=EDGE_CURVE('',#33978,#33979,#29598,.T.);
#41611=EDGE_CURVE('',#33976,#33979,#30820,.T.);
#41612=EDGE_CURVE('',#33979,#33980,#29599,.T.);
#41613=EDGE_CURVE('',#33980,#33976,#2811,.T.);
#41614=EDGE_CURVE('',#33980,#33981,#29600,.T.);
#41615=EDGE_CURVE('',#33981,#33885,#29601,.T.);
#41616=EDGE_CURVE('',#33977,#33982,#30821,.T.);
#41617=EDGE_CURVE('',#33887,#33983,#29602,.T.);
#41618=EDGE_CURVE('',#33984,#33983,#29603,.T.);
#41619=EDGE_CURVE('',#33982,#33984,#29604,.T.);
#41620=EDGE_CURVE('',#33978,#33985,#30822,.T.);
#41621=EDGE_CURVE('',#33985,#33982,#29605,.T.);
#41622=EDGE_CURVE('',#33979,#33986,#30823,.T.);
#41623=EDGE_CURVE('',#33986,#33985,#29606,.T.);
#41624=EDGE_CURVE('',#33980,#33987,#1749,.T.);
#41625=EDGE_CURVE('',#33987,#33986,#29607,.T.);
#41626=EDGE_CURVE('',#33981,#33988,#30824,.T.);
#41627=EDGE_CURVE('',#33988,#33987,#29608,.T.);
#41628=EDGE_CURVE('',#33885,#33989,#30825,.T.);
#41629=EDGE_CURVE('',#33989,#33988,#29609,.T.);
#41630=EDGE_CURVE('',#33886,#33990,#30826,.T.);
#41631=EDGE_CURVE('',#33990,#33989,#29610,.T.);
#41632=EDGE_CURVE('',#33983,#33990,#29611,.T.);
#41633=EDGE_CURVE('',#33983,#33876,#30827,.T.);
#41634=EDGE_CURVE('',#33984,#33875,#29612,.T.);
#41635=EDGE_CURVE('',#33982,#33884,#30828,.T.);
#41636=EDGE_CURVE('',#33985,#33883,#30829,.T.);
#41637=EDGE_CURVE('',#33986,#33882,#30830,.T.);
#41638=EDGE_CURVE('',#33987,#33881,#30831,.T.);
#41639=EDGE_CURVE('',#33988,#33879,#29613,.T.);
#41640=EDGE_CURVE('',#33989,#33878,#30832,.T.);
#41641=EDGE_CURVE('',#33990,#33877,#29614,.T.);
#41642=EDGE_CURVE('',#33991,#33992,#29615,.T.);
#41643=EDGE_CURVE('',#33992,#33874,#29616,.T.);
#41644=EDGE_CURVE('',#33873,#33991,#29617,.T.);
#41645=EDGE_CURVE('',#33993,#33991,#29618,.T.);
#41646=EDGE_CURVE('',#33630,#33993,#2812,.T.);
#41647=EDGE_CURVE('',#33993,#33994,#2813,.T.);
#41648=EDGE_CURVE('',#33994,#33992,#29619,.T.);
#41649=EDGE_CURVE('',#33994,#33626,#2814,.T.);
#41650=EDGE_CURVE('',#33995,#33870,#29620,.T.);
#41651=EDGE_CURVE('',#33995,#33993,#29621,.T.);
#41652=EDGE_CURVE('',#33996,#33995,#29622,.T.);
#41653=EDGE_CURVE('',#33996,#33994,#29623,.T.);
#41654=EDGE_CURVE('',#33869,#33996,#29624,.T.);
#41655=EDGE_CURVE('',#33997,#33998,#2815,.T.);
#41656=EDGE_CURVE('',#33998,#33999,#2816,.T.);
#41657=EDGE_CURVE('',#33999,#34000,#2817,.T.);
#41658=EDGE_CURVE('',#34000,#34001,#2818,.T.);
#41659=EDGE_CURVE('',#34001,#34002,#2819,.T.);
#41660=EDGE_CURVE('',#34002,#33997,#2820,.T.);
#41661=EDGE_CURVE('',#33997,#33858,#2821,.T.);
#41662=EDGE_CURVE('',#33998,#33856,#2822,.T.);
#41663=EDGE_CURVE('',#33999,#33857,#2823,.T.);
#41664=EDGE_CURVE('',#34000,#33862,#2824,.T.);
#41665=EDGE_CURVE('',#34001,#33861,#2825,.T.);
#41666=EDGE_CURVE('',#34002,#33859,#2826,.T.);
#41667=EDGE_CURVE('',#34003,#34004,#29625,.T.);
#41668=EDGE_CURVE('',#34003,#34005,#29626,.T.);
#41669=EDGE_CURVE('',#34005,#34004,#29627,.T.);
#41670=EDGE_CURVE('',#34006,#34007,#2827,.T.);
#41671=EDGE_CURVE('',#34007,#34008,#30833,.T.);
#41672=EDGE_CURVE('',#34009,#34008,#2828,.T.);
#41673=EDGE_CURVE('',#34006,#34009,#30834,.T.);
#41674=EDGE_CURVE('',#34010,#34004,#29628,.T.);
#41675=EDGE_CURVE('',#34010,#34011,#30835,.T.);
#41676=EDGE_CURVE('',#34012,#34011,#29629,.T.);
#41677=EDGE_CURVE('',#34012,#34003,#29630,.T.);
#41678=EDGE_CURVE('',#34013,#34014,#30836,.T.);
#41679=EDGE_CURVE('',#34014,#34015,#2829,.T.);
#41680=EDGE_CURVE('',#34012,#34015,#30837,.T.);
#41681=EDGE_CURVE('',#34013,#34012,#2830,.T.);
#41682=EDGE_CURVE('',#34015,#34005,#29631,.T.);
#41683=EDGE_CURVE('',#34016,#34017,#29632,.T.);
#41684=EDGE_CURVE('',#34004,#34016,#29633,.T.);
#41685=EDGE_CURVE('',#34005,#34017,#29634,.T.);
#41686=EDGE_CURVE('',#34018,#34019,#2831,.T.);
#41687=EDGE_CURVE('',#34018,#34020,#30838,.T.);
#41688=EDGE_CURVE('',#34020,#34021,#29635,.T.);
#41689=EDGE_CURVE('',#34019,#34021,#29636,.T.);
#41690=EDGE_CURVE('',#34022,#34023,#29637,.T.);
#41691=EDGE_CURVE('',#34022,#34024,#2832,.T.);
#41692=EDGE_CURVE('',#34024,#34025,#30839,.T.);
#41693=EDGE_CURVE('',#34023,#34025,#2833,.T.);
#41694=EDGE_CURVE('',#34026,#34021,#29638,.T.);
#41695=EDGE_CURVE('',#34027,#34026,#30840,.T.);
#41696=EDGE_CURVE('',#34027,#34019,#2644,.T.);
#41697=EDGE_CURVE('',#34018,#34008,#2834,.T.);
#41698=EDGE_CURVE('',#34027,#34009,#2835,.T.);
#41699=EDGE_CURVE('',#34028,#34026,#29639,.T.);
#41700=EDGE_CURVE('',#34027,#34028,#29640,.T.);
#41701=EDGE_CURVE('',#34029,#34009,#30841,.T.);
#41702=EDGE_CURVE('',#34029,#34006,#30842,.T.);
#41703=EDGE_CURVE('',#34030,#34031,#29641,.T.);
#41704=EDGE_CURVE('',#34031,#34007,#30843,.T.);
#41705=EDGE_CURVE('',#34030,#34006,#29642,.T.);
#41706=EDGE_CURVE('',#34031,#34032,#29643,.T.);
#41707=EDGE_CURVE('',#34032,#34033,#30844,.T.);
#41708=EDGE_CURVE('',#34033,#34020,#2836,.T.);
#41709=EDGE_CURVE('',#34034,#34032,#29644,.T.);
#41710=EDGE_CURVE('',#34035,#34034,#29645,.T.);
#41711=EDGE_CURVE('',#34016,#34035,#29646,.T.);
#41712=EDGE_CURVE('',#34022,#34017,#30845,.T.);
#41713=EDGE_CURVE('',#34033,#34023,#2837,.T.);
#41714=EDGE_CURVE('',#34035,#33843,#30846,.T.);
#41715=EDGE_CURVE('',#34034,#33845,#30847,.T.);
#41716=EDGE_CURVE('',#33843,#34036,#29647,.T.);
#41717=EDGE_CURVE('',#34010,#34036,#30848,.T.);
#41718=EDGE_CURVE('',#34037,#34038,#30849,.T.);
#41719=EDGE_CURVE('',#34011,#34038,#29648,.T.);
#41720=EDGE_CURVE('',#34010,#34037,#29649,.T.);
#41721=EDGE_CURVE('',#34039,#34040,#30850,.T.);
#41722=EDGE_CURVE('',#34040,#34014,#30851,.T.);
#41723=EDGE_CURVE('',#34039,#34013,#30852,.T.);
#41724=EDGE_CURVE('',#34038,#34041,#30853,.T.);
#41725=EDGE_CURVE('',#34041,#34013,#30854,.T.);
#41726=EDGE_CURVE('',#33836,#34040,#29650,.T.);
#41727=EDGE_CURVE('',#33836,#34039,#29651,.T.);
#41728=EDGE_CURVE('',#34024,#34040,#2838,.T.);
#41729=EDGE_CURVE('',#33834,#34025,#30855,.T.);
#41730=EDGE_CURVE('',#34024,#33834,#30856,.T.);
#41731=EDGE_CURVE('',#34025,#34042,#30857,.T.);
#41732=EDGE_CURVE('',#34042,#34043,#30858,.T.);
#41733=EDGE_CURVE('',#34043,#34021,#30859,.T.);
#41734=EDGE_CURVE('',#34044,#34043,#30860,.T.);
#41735=EDGE_CURVE('',#34044,#34028,#30861,.T.);
#41736=EDGE_CURVE('',#34028,#34029,#2839,.T.);
#41737=EDGE_CURVE('',#34045,#34029,#29652,.T.);
#41738=EDGE_CURVE('',#34045,#34046,#29653,.T.);
#41739=EDGE_CURVE('',#34046,#34030,#29654,.T.);
#41740=EDGE_CURVE('',#34046,#34047,#1750,.T.);
#41741=EDGE_CURVE('',#34047,#34048,#29655,.T.);
#41742=EDGE_CURVE('',#34030,#34048,#30862,.T.);
#41743=EDGE_CURVE('',#34048,#33845,#1751,.T.);
#41744=EDGE_CURVE('',#34049,#33841,#30863,.T.);
#41745=EDGE_CURVE('',#34050,#33841,#30864,.T.);
#41746=EDGE_CURVE('',#34051,#34050,#30865,.T.);
#41747=EDGE_CURVE('',#34051,#34049,#30866,.T.);
#41748=EDGE_CURVE('',#34052,#33842,#30867,.T.);
#41749=EDGE_CURVE('',#34049,#34052,#30868,.T.);
#41750=EDGE_CURVE('',#34053,#34054,#30869,.T.);
#41751=EDGE_CURVE('',#33842,#34054,#30870,.T.);
#41752=EDGE_CURVE('',#34052,#34053,#30871,.T.);
#41753=EDGE_CURVE('',#34036,#34054,#2840,.T.);
#41754=EDGE_CURVE('',#34036,#34037,#29656,.T.);
#41755=EDGE_CURVE('',#33837,#34041,#30872,.T.);
#41756=EDGE_CURVE('',#34037,#33837,#30873,.T.);
#41757=EDGE_CURVE('',#33835,#34042,#30874,.T.);
#41758=EDGE_CURVE('',#33835,#34044,#30875,.T.);
#41759=EDGE_CURVE('',#34045,#34044,#2841,.T.);
#41760=EDGE_CURVE('',#34045,#34047,#29657,.T.);
#41761=EDGE_CURVE('',#34047,#34050,#2842,.T.);
#41762=EDGE_CURVE('',#34055,#34050,#30876,.T.);
#41763=EDGE_CURVE('',#34056,#34055,#30877,.T.);
#41764=EDGE_CURVE('',#34056,#34051,#30878,.T.);
#41765=EDGE_CURVE('',#34057,#34056,#30879,.T.);
#41766=EDGE_CURVE('',#34053,#34057,#30880,.T.);
#41767=EDGE_CURVE('',#34057,#34058,#30881,.T.);
#41768=EDGE_CURVE('',#34054,#34058,#30882,.T.);
#41769=EDGE_CURVE('',#34059,#34058,#2843,.T.);
#41770=EDGE_CURVE('',#34059,#33838,#29658,.T.);
#41771=EDGE_CURVE('',#33840,#34060,#29659,.T.);
#41772=EDGE_CURVE('',#34060,#34061,#29660,.T.);
#41773=EDGE_CURVE('',#34055,#34061,#2844,.T.);
#41774=EDGE_CURVE('',#34061,#34062,#29661,.T.);
#41775=EDGE_CURVE('',#34062,#34055,#30883,.T.);
#41776=EDGE_CURVE('',#34062,#34063,#29662,.T.);
#41777=EDGE_CURVE('',#34063,#34064,#29663,.T.);
#41778=EDGE_CURVE('',#34058,#34064,#30884,.T.);
#41779=EDGE_CURVE('',#34064,#34059,#29664,.T.);
#41780=EDGE_CURVE('',#33838,#34065,#30885,.T.);
#41781=EDGE_CURVE('',#34059,#34066,#1752,.T.);
#41782=EDGE_CURVE('',#34067,#34066,#29665,.T.);
#41783=EDGE_CURVE('',#34065,#34067,#29666,.T.);
#41784=EDGE_CURVE('',#33840,#34068,#1753,.T.);
#41785=EDGE_CURVE('',#34068,#34065,#29667,.T.);
#41786=EDGE_CURVE('',#34060,#34069,#30886,.T.);
#41787=EDGE_CURVE('',#34069,#34068,#29668,.T.);
#41788=EDGE_CURVE('',#34061,#34070,#30887,.T.);
#41789=EDGE_CURVE('',#34070,#34069,#29669,.T.);
#41790=EDGE_CURVE('',#34062,#34071,#30888,.T.);
#41791=EDGE_CURVE('',#34071,#34070,#29670,.T.);
#41792=EDGE_CURVE('',#34063,#34072,#30889,.T.);
#41793=EDGE_CURVE('',#34072,#34071,#29671,.T.);
#41794=EDGE_CURVE('',#34064,#34073,#30890,.T.);
#41795=EDGE_CURVE('',#34073,#34072,#29672,.T.);
#41796=EDGE_CURVE('',#34066,#34073,#29673,.T.);
#41797=EDGE_CURVE('',#34066,#33825,#30891,.T.);
#41798=EDGE_CURVE('',#34067,#33824,#29674,.T.);
#41799=EDGE_CURVE('',#34065,#33833,#30892,.T.);
#41800=EDGE_CURVE('',#34068,#33832,#30893,.T.);
#41801=EDGE_CURVE('',#34069,#33830,#29675,.T.);
#41802=EDGE_CURVE('',#34070,#33829,#30894,.T.);
#41803=EDGE_CURVE('',#34071,#33828,#30895,.T.);
#41804=EDGE_CURVE('',#34072,#33827,#29676,.T.);
#41805=EDGE_CURVE('',#34073,#33826,#29677,.T.);
#41806=EDGE_CURVE('',#33633,#34074,#29678,.T.);
#41807=EDGE_CURVE('',#34074,#34075,#29679,.T.);
#41808=EDGE_CURVE('',#34075,#33634,#29680,.T.);
#41809=EDGE_CURVE('',#34076,#34075,#29681,.T.);
#41810=EDGE_CURVE('',#33638,#34076,#2845,.T.);
#41811=EDGE_CURVE('',#34077,#33823,#2846,.T.);
#41812=EDGE_CURVE('',#34077,#34074,#29682,.T.);
#41813=EDGE_CURVE('',#34076,#34077,#2847,.T.);
#41814=EDGE_CURVE('',#34078,#34076,#29683,.T.);
#41815=EDGE_CURVE('',#33821,#34078,#29684,.T.);
#41816=EDGE_CURVE('',#34079,#34077,#29685,.T.);
#41817=EDGE_CURVE('',#34079,#33819,#29686,.T.);
#41818=EDGE_CURVE('',#34078,#34079,#29687,.T.);
#41819=EDGE_CURVE('',#33658,#33646,#2848,.T.);
#41820=EDGE_CURVE('',#33645,#33659,#2849,.T.);
#41821=EDGE_CURVE('',#34080,#34081,#2850,.T.);
#41822=EDGE_CURVE('',#34080,#34082,#2851,.T.);
#41823=EDGE_CURVE('',#34083,#34082,#2852,.T.);
#41824=EDGE_CURVE('',#34083,#34084,#2853,.T.);
#41825=EDGE_CURVE('',#34084,#34085,#30896,.T.);
#41826=EDGE_CURVE('',#34086,#34085,#30897,.T.);
#41827=EDGE_CURVE('',#34087,#34086,#30898,.T.);
#41828=EDGE_CURVE('',#34088,#34087,#30899,.T.);
#41829=EDGE_CURVE('',#34081,#34088,#30900,.T.);
#41830=EDGE_CURVE('',#34089,#34090,#2854,.T.);
#41831=EDGE_CURVE('',#34089,#34091,#2855,.T.);
#41832=EDGE_CURVE('',#34092,#34091,#2856,.T.);
#41833=EDGE_CURVE('',#34093,#34092,#30901,.T.);
#41834=EDGE_CURVE('',#34094,#34093,#30902,.T.);
#41835=EDGE_CURVE('',#34095,#34094,#30903,.T.);
#41836=EDGE_CURVE('',#34096,#34095,#30904,.T.);
#41837=EDGE_CURVE('',#34096,#34097,#30905,.T.);
#41838=EDGE_CURVE('',#34097,#34090,#2857,.T.);
#41839=EDGE_CURVE('',#33683,#34098,#2858,.T.);
#41840=EDGE_CURVE('',#34099,#33682,#2859,.T.);
#41841=EDGE_CURVE('',#34098,#34099,#2645,.T.);
#41842=EDGE_CURVE('',#33681,#34100,#2860,.T.);
#41843=EDGE_CURVE('',#34101,#33680,#2861,.T.);
#41844=EDGE_CURVE('',#34100,#34101,#2646,.T.);
#41845=EDGE_CURVE('',#34098,#34102,#30906,.T.);
#41846=EDGE_CURVE('',#34102,#34103,#30907,.T.);
#41847=EDGE_CURVE('',#34104,#34103,#2862,.T.);
#41848=EDGE_CURVE('',#33684,#34104,#30908,.T.);
#41849=EDGE_CURVE('',#33685,#34104,#29688,.T.);
#41850=EDGE_CURVE('',#34105,#34106,#2863,.T.);
#41851=EDGE_CURVE('',#34105,#34107,#29689,.T.);
#41852=EDGE_CURVE('',#34107,#33760,#2864,.T.);
#41853=EDGE_CURVE('',#33760,#34108,#2865,.T.);
#41854=EDGE_CURVE('',#34106,#34108,#2866,.T.);
#41855=EDGE_CURVE('',#34109,#33678,#29690,.T.);
#41856=EDGE_CURVE('',#33677,#34109,#29691,.T.);
#41857=EDGE_CURVE('',#34110,#33676,#29692,.T.);
#41858=EDGE_CURVE('',#34111,#34110,#29693,.T.);
#41859=EDGE_CURVE('',#34112,#34111,#30909,.T.);
#41860=EDGE_CURVE('',#34113,#34112,#2867,.T.);
#41861=EDGE_CURVE('',#34114,#34113,#29694,.T.);
#41862=EDGE_CURVE('',#34115,#34114,#30910,.T.);
#41863=EDGE_CURVE('',#34115,#34116,#29695,.T.);
#41864=EDGE_CURVE('',#34116,#34109,#2868,.T.);
#41865=EDGE_CURVE('',#34104,#33686,#29696,.T.);
#41866=EDGE_CURVE('',#34103,#34117,#29697,.T.);
#41867=EDGE_CURVE('',#34117,#34118,#29698,.T.);
#41868=EDGE_CURVE('',#34118,#34119,#29699,.T.);
#41869=EDGE_CURVE('',#34120,#34119,#30911,.T.);
#41870=EDGE_CURVE('',#34121,#34120,#29700,.T.);
#41871=EDGE_CURVE('',#34121,#34122,#2869,.T.);
#41872=EDGE_CURVE('',#34123,#34122,#30912,.T.);
#41873=EDGE_CURVE('',#34124,#34123,#29701,.T.);
#41874=EDGE_CURVE('',#33687,#34124,#29702,.T.);
#41875=EDGE_CURVE('',#34125,#34124,#29703,.T.);
#41876=EDGE_CURVE('',#34126,#34125,#2870,.T.);
#41877=EDGE_CURVE('',#34127,#34126,#30913,.T.);
#41878=EDGE_CURVE('',#34127,#34128,#29704,.T.);
#41879=EDGE_CURVE('',#34129,#34128,#2871,.T.);
#41880=EDGE_CURVE('',#34130,#34129,#29705,.T.);
#41881=EDGE_CURVE('',#33688,#34130,#29706,.T.);
#41882=EDGE_CURVE('',#34131,#33675,#29707,.T.);
#41883=EDGE_CURVE('',#34132,#34131,#29708,.T.);
#41884=EDGE_CURVE('',#34132,#34133,#2872,.T.);
#41885=EDGE_CURVE('',#34133,#34134,#29709,.T.);
#41886=EDGE_CURVE('',#34135,#34134,#30914,.T.);
#41887=EDGE_CURVE('',#34136,#34135,#2873,.T.);
#41888=EDGE_CURVE('',#34110,#34136,#29710,.T.);
#41889=EDGE_CURVE('',#33672,#34137,#29711,.T.);
#41890=EDGE_CURVE('',#33690,#34129,#1754,.T.);
#41891=EDGE_CURVE('',#34129,#34138,#29712,.T.);
#41892=EDGE_CURVE('',#34139,#34138,#30915,.T.);
#41893=EDGE_CURVE('',#34140,#34139,#29713,.T.);
#41894=EDGE_CURVE('',#34140,#34137,#1755,.T.);
#41895=EDGE_CURVE('',#33689,#34130,#29714,.T.);
#41896=EDGE_CURVE('',#34080,#34141,#29715,.T.);
#41897=EDGE_CURVE('',#34081,#34142,#30916,.T.);
#41898=EDGE_CURVE('',#34141,#34142,#2874,.T.);
#41899=EDGE_CURVE('',#34143,#34091,#29716,.T.);
#41900=EDGE_CURVE('',#34144,#34143,#2875,.T.);
#41901=EDGE_CURVE('',#34092,#34144,#30917,.T.);
#41902=EDGE_CURVE('',#33674,#34131,#30918,.T.);
#41903=EDGE_CURVE('',#33673,#34132,#29717,.T.);
#41904=EDGE_CURVE('',#34145,#33671,#29718,.T.);
#41905=EDGE_CURVE('',#34146,#34145,#29719,.T.);
#41906=EDGE_CURVE('',#34139,#34146,#29720,.T.);
#41907=EDGE_CURVE('',#34138,#34132,#29721,.T.);
#41908=EDGE_CURVE('',#33679,#34109,#30919,.T.);
#41909=EDGE_CURVE('',#34101,#34116,#29722,.T.);
#41910=EDGE_CURVE('',#34147,#34100,#30920,.T.);
#41911=EDGE_CURVE('',#34148,#34147,#2876,.T.);
#41912=EDGE_CURVE('',#34148,#34099,#29723,.T.);
#41913=EDGE_CURVE('',#34149,#34118,#30921,.T.);
#41914=EDGE_CURVE('',#34149,#34150,#29724,.T.);
#41915=EDGE_CURVE('',#34119,#34150,#29725,.T.);
#41916=EDGE_CURVE('',#34151,#34152,#2647,.T.);
#41917=EDGE_CURVE('',#34153,#34151,#30922,.T.);
#41918=EDGE_CURVE('',#34153,#34152,#29726,.T.);
#41919=EDGE_CURVE('',#34152,#34149,#29727,.T.);
#41920=EDGE_CURVE('',#34151,#34117,#30923,.T.);
#41921=EDGE_CURVE('',#34102,#34154,#29728,.T.);
#41922=EDGE_CURVE('',#34098,#34154,#29729,.T.);
#41923=EDGE_CURVE('',#34155,#34156,#2648,.T.);
#41924=EDGE_CURVE('',#34157,#34155,#29730,.T.);
#41925=EDGE_CURVE('',#34157,#34156,#29731,.T.);
#41926=EDGE_CURVE('',#34158,#34159,#2649,.T.);
#41927=EDGE_CURVE('',#34158,#34160,#29732,.T.);
#41928=EDGE_CURVE('',#34159,#34160,#2650,.T.);
#41929=EDGE_CURVE('',#34155,#34161,#29733,.T.);
#41930=EDGE_CURVE('',#34156,#34158,#29734,.T.);
#41931=EDGE_CURVE('',#34161,#34159,#30924,.T.);
#41932=EDGE_CURVE('',#34162,#34163,#29735,.T.);
#41933=EDGE_CURVE('',#34162,#34164,#29736,.T.);
#41934=EDGE_CURVE('',#34163,#34164,#29737,.T.);
#41935=EDGE_CURVE('',#34165,#34166,#2651,.T.);
#41936=EDGE_CURVE('',#34167,#34165,#29738,.T.);
#41937=EDGE_CURVE('',#34167,#34166,#29739,.T.);
#41938=EDGE_CURVE('',#34165,#34168,#29740,.T.);
#41939=EDGE_CURVE('',#34166,#34169,#2652,.T.);
#41940=EDGE_CURVE('',#34170,#34169,#30925,.T.);
#41941=EDGE_CURVE('',#34168,#34170,#2653,.T.);
#41942=EDGE_CURVE('',#34168,#34171,#29741,.T.);
#41943=EDGE_CURVE('',#34171,#34170,#2654,.T.);
#41944=EDGE_CURVE('',#34171,#34172,#29742,.T.);
#41945=EDGE_CURVE('',#34169,#34173,#29743,.T.);
#41946=EDGE_CURVE('',#34174,#34173,#30926,.T.);
#41947=EDGE_CURVE('',#34172,#34174,#29744,.T.);
#41948=EDGE_CURVE('',#34087,#33807,#30927,.T.);
#41949=EDGE_CURVE('',#34088,#33806,#30928,.T.);
#41950=EDGE_CURVE('',#34085,#34175,#29745,.T.);
#41951=EDGE_CURVE('',#34176,#34175,#30929,.T.);
#41952=EDGE_CURVE('',#34086,#34176,#30930,.T.);
#41953=EDGE_CURVE('',#33807,#34176,#30931,.T.);
#41954=EDGE_CURVE('',#34176,#34177,#2877,.T.);
#41955=EDGE_CURVE('',#34177,#33804,#30932,.T.);
#41956=EDGE_CURVE('',#34094,#33804,#30933,.T.);
#41957=EDGE_CURVE('',#34095,#34177,#30934,.T.);
#41958=EDGE_CURVE('',#34143,#34141,#30935,.T.);
#41959=EDGE_CURVE('',#34144,#34142,#2878,.T.);
#41960=EDGE_CURVE('',#34178,#34179,#2879,.T.);
#41961=EDGE_CURVE('',#34180,#34178,#2880,.T.);
#41962=EDGE_CURVE('',#34180,#33695,#2881,.T.);
#41963=EDGE_CURVE('',#33695,#34181,#2882,.T.);
#41964=EDGE_CURVE('',#34181,#34179,#29746,.T.);
#41965=EDGE_CURVE('',#34090,#34178,#30936,.T.);
#41966=EDGE_CURVE('',#34097,#34180,#30937,.T.);
#41967=EDGE_CURVE('',#34182,#34113,#30938,.T.);
#41968=EDGE_CURVE('',#34114,#34182,#29747,.T.);
#41969=EDGE_CURVE('',#34182,#34183,#29748,.T.);
#41970=EDGE_CURVE('',#34184,#34183,#29749,.T.);
#41971=EDGE_CURVE('',#34114,#34184,#29750,.T.);
#41972=EDGE_CURVE('',#34147,#34184,#30939,.T.);
#41973=EDGE_CURVE('',#34147,#34185,#29751,.T.);
#41974=EDGE_CURVE('',#34115,#34185,#29752,.T.);
#41975=EDGE_CURVE('',#34185,#34101,#29753,.T.);
#41976=EDGE_CURVE('',#34186,#34187,#29754,.T.);
#41977=EDGE_CURVE('',#34188,#34186,#30940,.T.);
#41978=EDGE_CURVE('',#34189,#34188,#29755,.T.);
#41979=EDGE_CURVE('',#34190,#34189,#2883,.T.);
#41980=EDGE_CURVE('',#34191,#34190,#29756,.T.);
#41981=EDGE_CURVE('',#34192,#34191,#30941,.T.);
#41982=EDGE_CURVE('',#34193,#34192,#29757,.T.);
#41983=EDGE_CURVE('',#34194,#34193,#29758,.T.);
#41984=EDGE_CURVE('',#34195,#34194,#2884,.T.);
#41985=EDGE_CURVE('',#34195,#34196,#29759,.T.);
#41986=EDGE_CURVE('',#34187,#34196,#2885,.T.);
#41987=EDGE_CURVE('',#34111,#34197,#30942,.T.);
#41988=EDGE_CURVE('',#34198,#34197,#30943,.T.);
#41989=EDGE_CURVE('',#34112,#34198,#30944,.T.);
#41990=EDGE_CURVE('',#34199,#34198,#30945,.T.);
#41991=EDGE_CURVE('',#34122,#34199,#30946,.T.);
#41992=EDGE_CURVE('',#34122,#34112,#30947,.T.);
#41993=EDGE_CURVE('',#34200,#34194,#2655,.T.);
#41994=EDGE_CURVE('',#34201,#34200,#2656,.T.);
#41995=EDGE_CURVE('',#34202,#34201,#2886,.T.);
#41996=EDGE_CURVE('',#34195,#34202,#30948,.T.);
#41997=EDGE_CURVE('',#34203,#34121,#2657,.T.);
#41998=EDGE_CURVE('',#34113,#34203,#2658,.T.);
#41999=EDGE_CURVE('',#34202,#33801,#29760,.T.);
#42000=EDGE_CURVE('',#34195,#33800,#29761,.T.);
#42001=EDGE_CURVE('',#34204,#33803,#29762,.T.);
#42002=EDGE_CURVE('',#34196,#34204,#29763,.T.);
#42003=EDGE_CURVE('',#34205,#34202,#29764,.T.);
#42004=EDGE_CURVE('',#34206,#34205,#29765,.T.);
#42005=EDGE_CURVE('',#33802,#34206,#29766,.T.);
#42006=EDGE_CURVE('',#34207,#33802,#1756,.T.);
#42007=EDGE_CURVE('',#34208,#34206,#29767,.T.);
#42008=EDGE_CURVE('',#34207,#34208,#29768,.T.);
#42009=EDGE_CURVE('',#34209,#33798,#2887,.T.);
#42010=EDGE_CURVE('',#34209,#34210,#2888,.T.);
#42011=EDGE_CURVE('',#34210,#34211,#29769,.T.);
#42012=EDGE_CURVE('',#34211,#34207,#30949,.T.);
#42013=EDGE_CURVE('',#34208,#34212,#2889,.T.);
#42014=EDGE_CURVE('',#33798,#34212,#2890,.T.);
#42015=EDGE_CURVE('',#34213,#33786,#30950,.T.);
#42016=EDGE_CURVE('',#34214,#33785,#30951,.T.);
#42017=EDGE_CURVE('',#34213,#34214,#2659,.T.);
#42018=EDGE_CURVE('',#34214,#34215,#2660,.T.);
#42019=EDGE_CURVE('',#34215,#34216,#2891,.T.);
#42020=EDGE_CURVE('',#34216,#34217,#30952,.T.);
#42021=EDGE_CURVE('',#34217,#34218,#30953,.T.);
#42022=EDGE_CURVE('',#34213,#34218,#2892,.T.);
#42023=EDGE_CURVE('',#34219,#34220,#2661,.T.);
#42024=EDGE_CURVE('',#34221,#34220,#2893,.T.);
#42025=EDGE_CURVE('',#34221,#34222,#2662,.T.);
#42026=EDGE_CURVE('',#34222,#34223,#2894,.T.);
#42027=EDGE_CURVE('',#34223,#34219,#2663,.T.);
#42028=EDGE_CURVE('',#34218,#34224,#29770,.T.);
#42029=EDGE_CURVE('',#34224,#34225,#2895,.T.);
#42030=EDGE_CURVE('',#34221,#34225,#29771,.T.);
#42031=EDGE_CURVE('',#34220,#34213,#29772,.T.);
#42032=EDGE_CURVE('',#34220,#33787,#2664,.T.);
#42033=EDGE_CURVE('',#34219,#33788,#30954,.T.);
#42034=EDGE_CURVE('',#34223,#33789,#30955,.T.);
#42035=EDGE_CURVE('',#34215,#33790,#2665,.T.);
#42036=EDGE_CURVE('',#34215,#34223,#29773,.T.);
#42037=EDGE_CURVE('',#34226,#34222,#29774,.T.);
#42038=EDGE_CURVE('',#34226,#34227,#2896,.T.);
#42039=EDGE_CURVE('',#34227,#34216,#29775,.T.);
#42040=EDGE_CURVE('',#34228,#34227,#29776,.T.);
#42041=EDGE_CURVE('',#34229,#34228,#29777,.T.);
#42042=EDGE_CURVE('',#34217,#34229,#29778,.T.);
#42043=EDGE_CURVE('',#34230,#34229,#29779,.T.);
#42044=EDGE_CURVE('',#34230,#34224,#29780,.T.);
#42045=EDGE_CURVE('',#34231,#34230,#29781,.T.);
#42046=EDGE_CURVE('',#34232,#34231,#2897,.T.);
#42047=EDGE_CURVE('',#34232,#34233,#29782,.T.);
#42048=EDGE_CURVE('',#34234,#34233,#2666,.T.);
#42049=EDGE_CURVE('',#34224,#34234,#29783,.T.);
#42050=EDGE_CURVE('',#34235,#34234,#2898,.T.);
#42051=EDGE_CURVE('',#34235,#34236,#29784,.T.);
#42052=EDGE_CURVE('',#34237,#34236,#2899,.T.);
#42053=EDGE_CURVE('',#34225,#34237,#29785,.T.);
#42054=EDGE_CURVE('',#34237,#33738,#29786,.T.);
#42055=EDGE_CURVE('',#33737,#34225,#29787,.T.);
#42056=EDGE_CURVE('',#33736,#34221,#29788,.T.);
#42057=EDGE_CURVE('',#33733,#34222,#29789,.T.);
#42058=EDGE_CURVE('',#33732,#34226,#29790,.T.);
#42059=EDGE_CURVE('',#34238,#33731,#30956,.T.);
#42060=EDGE_CURVE('',#34238,#34226,#29791,.T.);
#42061=EDGE_CURVE('',#34238,#34239,#2900,.T.);
#42062=EDGE_CURVE('',#34239,#34240,#29792,.T.);
#42063=EDGE_CURVE('',#34240,#34241,#2901,.T.);
#42064=EDGE_CURVE('',#34241,#34227,#29793,.T.);
#42065=EDGE_CURVE('',#34242,#34241,#2667,.T.);
#42066=EDGE_CURVE('',#34232,#34242,#29794,.T.);
#42067=EDGE_CURVE('',#34228,#34231,#29795,.T.);
#42068=EDGE_CURVE('',#33774,#34243,#29796,.T.);
#42069=EDGE_CURVE('',#34243,#34244,#29797,.T.);
#42070=EDGE_CURVE('',#34245,#34244,#2902,.T.);
#42071=EDGE_CURVE('',#34245,#34246,#29798,.T.);
#42072=EDGE_CURVE('',#34246,#33777,#29799,.T.);
#42073=EDGE_CURVE('',#34247,#33772,#29800,.T.);
#42074=EDGE_CURVE('',#33773,#34247,#29801,.T.);
#42075=EDGE_CURVE('',#34248,#34247,#30957,.T.);
#42076=EDGE_CURVE('',#34248,#34249,#29802,.T.);
#42077=EDGE_CURVE('',#34249,#34243,#1757,.T.);
#42078=EDGE_CURVE('',#34249,#34250,#29803,.T.);
#42079=EDGE_CURVE('',#34250,#34244,#30958,.T.);
#42080=EDGE_CURVE('',#34244,#34251,#29804,.T.);
#42081=EDGE_CURVE('',#34250,#34252,#29805,.T.);
#42082=EDGE_CURVE('',#34252,#34251,#29806,.T.);
#42083=EDGE_CURVE('',#34253,#34254,#29807,.T.);
#42084=EDGE_CURVE('',#34251,#34254,#2668,.T.);
#42085=EDGE_CURVE('',#34252,#34253,#30959,.T.);
#42086=EDGE_CURVE('',#34252,#34193,#29808,.T.);
#42087=EDGE_CURVE('',#34193,#34255,#29809,.T.);
#42088=EDGE_CURVE('',#34256,#34255,#29810,.T.);
#42089=EDGE_CURVE('',#34253,#34256,#29811,.T.);
#42090=EDGE_CURVE('',#34256,#34257,#30960,.T.);
#42091=EDGE_CURVE('',#34254,#34257,#29812,.T.);
#42092=EDGE_CURVE('',#34257,#34258,#29813,.T.);
#42093=EDGE_CURVE('',#34258,#34259,#29814,.T.);
#42094=EDGE_CURVE('',#34259,#34260,#29815,.T.);
#42095=EDGE_CURVE('',#34260,#34261,#29816,.T.);
#42096=EDGE_CURVE('',#34261,#34262,#29817,.T.);
#42097=EDGE_CURVE('',#34262,#34263,#29818,.T.);
#42098=EDGE_CURVE('',#34263,#34264,#29819,.T.);
#42099=EDGE_CURVE('',#34264,#34254,#2903,.T.);
#42100=EDGE_CURVE('',#34264,#34265,#2669,.T.);
#42101=EDGE_CURVE('',#34265,#34245,#29820,.T.);
#42102=EDGE_CURVE('',#34266,#34245,#30961,.T.);
#42103=EDGE_CURVE('',#34267,#34265,#29821,.T.);
#42104=EDGE_CURVE('',#34267,#34266,#29822,.T.);
#42105=EDGE_CURVE('',#34267,#34268,#29823,.T.);
#42106=EDGE_CURVE('',#34268,#34201,#29824,.T.);
#42107=EDGE_CURVE('',#34200,#34269,#29825,.T.);
#42108=EDGE_CURVE('',#34270,#34269,#29826,.T.);
#42109=EDGE_CURVE('',#34266,#34270,#29827,.T.);
#42110=EDGE_CURVE('',#34270,#34246,#29828,.T.);
#42111=EDGE_CURVE('',#34270,#34248,#29829,.T.);
#42112=EDGE_CURVE('',#34269,#34248,#29830,.T.);
#42113=EDGE_CURVE('',#34269,#34249,#29831,.T.);
#42114=EDGE_CURVE('',#34271,#34268,#29832,.T.);
#42115=EDGE_CURVE('',#34272,#34271,#30962,.T.);
#42116=EDGE_CURVE('',#34273,#34272,#29833,.T.);
#42117=EDGE_CURVE('',#34274,#34273,#2904,.T.);
#42118=EDGE_CURVE('',#34275,#34274,#29834,.T.);
#42119=EDGE_CURVE('',#34276,#34275,#30963,.T.);
#42120=EDGE_CURVE('',#34277,#34276,#29835,.T.);
#42121=EDGE_CURVE('',#34205,#34277,#2905,.T.);
#42122=EDGE_CURVE('',#34123,#34278,#30964,.T.);
#42123=EDGE_CURVE('',#34279,#34278,#29836,.T.);
#42124=EDGE_CURVE('',#34124,#34279,#2670,.T.);
#42125=EDGE_CURVE('',#34280,#34279,#29837,.T.);
#42126=EDGE_CURVE('',#34125,#34280,#29838,.T.);
#42127=EDGE_CURVE('',#34281,#34268,#29839,.T.);
#42128=EDGE_CURVE('',#34282,#34281,#29840,.T.);
#42129=EDGE_CURVE('',#34283,#34282,#29841,.T.);
#42130=EDGE_CURVE('',#34271,#34283,#30965,.T.);
#42131=EDGE_CURVE('',#34283,#34284,#29842,.T.);
#42132=EDGE_CURVE('',#34285,#34284,#30966,.T.);
#42133=EDGE_CURVE('',#34271,#34285,#29843,.T.);
#42134=EDGE_CURVE('',#34286,#34285,#30967,.T.);
#42135=EDGE_CURVE('',#34272,#34286,#30968,.T.);
#42136=EDGE_CURVE('',#34287,#34286,#29844,.T.);
#42137=EDGE_CURVE('',#34273,#34287,#29845,.T.);
#42138=EDGE_CURVE('',#34288,#34287,#2906,.T.);
#42139=EDGE_CURVE('',#34274,#34288,#30969,.T.);
#42140=EDGE_CURVE('',#34289,#34288,#29846,.T.);
#42141=EDGE_CURVE('',#34275,#34289,#30970,.T.);
#42142=EDGE_CURVE('',#34290,#34289,#30971,.T.);
#42143=EDGE_CURVE('',#34276,#34290,#30972,.T.);
#42144=EDGE_CURVE('',#34212,#34290,#29847,.T.);
#42145=EDGE_CURVE('',#34277,#34212,#29848,.T.);
#42146=EDGE_CURVE('',#34208,#34205,#29849,.T.);
#42147=EDGE_CURVE('',#34291,#34290,#2907,.T.);
#42148=EDGE_CURVE('',#34291,#34209,#29850,.T.);
#42149=EDGE_CURVE('',#34187,#34209,#30973,.T.);
#42150=EDGE_CURVE('',#34186,#34291,#30974,.T.);
#42151=EDGE_CURVE('',#34292,#34291,#30975,.T.);
#42152=EDGE_CURVE('',#34188,#34292,#30976,.T.);
#42153=EDGE_CURVE('',#34293,#34292,#29851,.T.);
#42154=EDGE_CURVE('',#34189,#34293,#30977,.T.);
#42155=EDGE_CURVE('',#34294,#34293,#2908,.T.);
#42156=EDGE_CURVE('',#34190,#34294,#2671,.T.);
#42157=EDGE_CURVE('',#34295,#34294,#29852,.T.);
#42158=EDGE_CURVE('',#34191,#34295,#30978,.T.);
#42159=EDGE_CURVE('',#34296,#34295,#30979,.T.);
#42160=EDGE_CURVE('',#34192,#34296,#30980,.T.);
#42161=EDGE_CURVE('',#34297,#34296,#29853,.T.);
#42162=EDGE_CURVE('',#34298,#34297,#29854,.T.);
#42163=EDGE_CURVE('',#34298,#34192,#30981,.T.);
#42164=EDGE_CURVE('',#34255,#34299,#29855,.T.);
#42165=EDGE_CURVE('',#34298,#34299,#29856,.T.);
#42166=EDGE_CURVE('',#34300,#34301,#29857,.T.);
#42167=EDGE_CURVE('',#34302,#34300,#29858,.T.);
#42168=EDGE_CURVE('',#34299,#34302,#29859,.T.);
#42169=EDGE_CURVE('',#34303,#34298,#30982,.T.);
#42170=EDGE_CURVE('',#34303,#34301,#29860,.T.);
#42171=EDGE_CURVE('',#34304,#34303,#29861,.T.);
#42172=EDGE_CURVE('',#34304,#34301,#2672,.T.);
#42173=EDGE_CURVE('',#34301,#34305,#29862,.T.);
#42174=EDGE_CURVE('',#34306,#34304,#29863,.T.);
#42175=EDGE_CURVE('',#34306,#34305,#2673,.T.);
#42176=EDGE_CURVE('',#34305,#34307,#29864,.T.);
#42177=EDGE_CURVE('',#34308,#34306,#29865,.T.);
#42178=EDGE_CURVE('',#34308,#34307,#2674,.T.);
#42179=EDGE_CURVE('',#34309,#34308,#29866,.T.);
#42180=EDGE_CURVE('',#34307,#34309,#29867,.T.);
#42181=EDGE_CURVE('',#34283,#34309,#30983,.T.);
#42182=EDGE_CURVE('',#34310,#34282,#29868,.T.);
#42183=EDGE_CURVE('',#34311,#34310,#29869,.T.);
#42184=EDGE_CURVE('',#34307,#34311,#29870,.T.);
#42185=EDGE_CURVE('',#34305,#34312,#2909,.T.);
#42186=EDGE_CURVE('',#34311,#34313,#29871,.T.);
#42187=EDGE_CURVE('',#34312,#34313,#29872,.T.);
#42188=EDGE_CURVE('',#34313,#34261,#30984,.T.);
#42189=EDGE_CURVE('',#34312,#34260,#30985,.T.);
#42190=EDGE_CURVE('',#34314,#34259,#30986,.T.);
#42191=EDGE_CURVE('',#34314,#34312,#29873,.T.);
#42192=EDGE_CURVE('',#34314,#34300,#29874,.T.);
#42193=EDGE_CURVE('',#34315,#34302,#29875,.T.);
#42194=EDGE_CURVE('',#34315,#34314,#29876,.T.);
#42195=EDGE_CURVE('',#34315,#34258,#30987,.T.);
#42196=EDGE_CURVE('',#34256,#34315,#29877,.T.);
#42197=EDGE_CURVE('',#34313,#34316,#29878,.T.);
#42198=EDGE_CURVE('',#34316,#34262,#30988,.T.);
#42199=EDGE_CURVE('',#34317,#34263,#29879,.T.);
#42200=EDGE_CURVE('',#34316,#34317,#29880,.T.);
#42201=EDGE_CURVE('',#34310,#34316,#29881,.T.);
#42202=EDGE_CURVE('',#34281,#34317,#29882,.T.);
#42203=EDGE_CURVE('',#34318,#34267,#30989,.T.);
#42204=EDGE_CURVE('',#34317,#34318,#29883,.T.);
#42205=EDGE_CURVE('',#34318,#34264,#30990,.T.);
#42206=EDGE_CURVE('',#34309,#34319,#29884,.T.);
#42207=EDGE_CURVE('',#34284,#34319,#30991,.T.);
#42208=EDGE_CURVE('',#34319,#34320,#29885,.T.);
#42209=EDGE_CURVE('',#34320,#34321,#29886,.T.);
#42210=EDGE_CURVE('',#34321,#34322,#29887,.T.);
#42211=EDGE_CURVE('',#34322,#34323,#29888,.T.);
#42212=EDGE_CURVE('',#34323,#34297,#30992,.T.);
#42213=EDGE_CURVE('',#34286,#34295,#2910,.T.);
#42214=EDGE_CURVE('',#34287,#34294,#2911,.T.);
#42215=EDGE_CURVE('',#33771,#34288,#2912,.T.);
#42216=EDGE_CURVE('',#34293,#33770,#2913,.T.);
#42217=EDGE_CURVE('',#34292,#34289,#2914,.T.);
#42218=EDGE_CURVE('',#34324,#34325,#30993,.T.);
#42219=EDGE_CURVE('',#34325,#34324,#2915,.T.);
#42220=EDGE_CURVE('',#34326,#34327,#2916,.T.);
#42221=EDGE_CURVE('',#34328,#34326,#29889,.T.);
#42222=EDGE_CURVE('',#34328,#34329,#2917,.T.);
#42223=EDGE_CURVE('',#34329,#34330,#29890,.T.);
#42224=EDGE_CURVE('',#34331,#34330,#2918,.T.);
#42225=EDGE_CURVE('',#34331,#34324,#29891,.T.);
#42226=EDGE_CURVE('',#34325,#34327,#29892,.T.);
#42227=EDGE_CURVE('',#34332,#34331,#30994,.T.);
#42228=EDGE_CURVE('',#34327,#34332,#30995,.T.);
#42229=EDGE_CURVE('',#34333,#34332,#2919,.T.);
#42230=EDGE_CURVE('',#34334,#34333,#30996,.T.);
#42231=EDGE_CURVE('',#34335,#34334,#30997,.T.);
#42232=EDGE_CURVE('',#34336,#34335,#29893,.T.);
#42233=EDGE_CURVE('',#34326,#34336,#30998,.T.);
#42234=EDGE_CURVE('',#34330,#34337,#30999,.T.);
#42235=EDGE_CURVE('',#34337,#34338,#29894,.T.);
#42236=EDGE_CURVE('',#34338,#34339,#31000,.T.);
#42237=EDGE_CURVE('',#34339,#34340,#31001,.T.);
#42238=EDGE_CURVE('',#34332,#34340,#2920,.T.);
#42239=EDGE_CURVE('',#34341,#34336,#31002,.T.);
#42240=EDGE_CURVE('',#34342,#34341,#31003,.T.);
#42241=EDGE_CURVE('',#34342,#34326,#31004,.T.);
#42242=EDGE_CURVE('',#34343,#34328,#31005,.T.);
#42243=EDGE_CURVE('',#34343,#34342,#29895,.T.);
#42244=EDGE_CURVE('',#34341,#34344,#29896,.T.);
#42245=EDGE_CURVE('',#34344,#34343,#2921,.T.);
#42246=EDGE_CURVE('',#34164,#34345,#2922,.T.);
#42247=EDGE_CURVE('',#34164,#34346,#29897,.T.);
#42248=EDGE_CURVE('',#34347,#34346,#31006,.T.);
#42249=EDGE_CURVE('',#34345,#34347,#1758,.T.);
#42250=EDGE_CURVE('',#34344,#34174,#29898,.T.);
#42251=EDGE_CURVE('',#34173,#34328,#2923,.T.);
#42252=EDGE_CURVE('',#34278,#34167,#2924,.T.);
#42253=EDGE_CURVE('',#34278,#34199,#31007,.T.);
#42254=EDGE_CURVE('',#34157,#34197,#2925,.T.);
#42255=EDGE_CURVE('',#34161,#34348,#29899,.T.);
#42256=EDGE_CURVE('',#34348,#34329,#2926,.T.);
#42257=EDGE_CURVE('',#34348,#34163,#31008,.T.);
#42258=EDGE_CURVE('',#34329,#34345,#31009,.T.);
#42259=EDGE_CURVE('',#34330,#34347,#31010,.T.);
#42260=EDGE_CURVE('',#34337,#34346,#1759,.T.);
#42261=EDGE_CURVE('',#34346,#34349,#29900,.T.);
#42262=EDGE_CURVE('',#34338,#34349,#29901,.T.);
#42263=EDGE_CURVE('',#34349,#33705,#31011,.T.);
#42264=EDGE_CURVE('',#34339,#33705,#31012,.T.);
#42265=EDGE_CURVE('',#34340,#33704,#29902,.T.);
#42266=EDGE_CURVE('',#34340,#34350,#29903,.T.);
#42267=EDGE_CURVE('',#34350,#33703,#1760,.T.);
#42268=EDGE_CURVE('',#34350,#34351,#29904,.T.);
#42269=EDGE_CURVE('',#33703,#34351,#29905,.T.);
#42270=EDGE_CURVE('',#34351,#33702,#2927,.T.);
#42271=EDGE_CURVE('',#34352,#33702,#2928,.T.);
#42272=EDGE_CURVE('',#34352,#34353,#29906,.T.);
#42273=EDGE_CURVE('',#34353,#34354,#29907,.T.);
#42274=EDGE_CURVE('',#34354,#34355,#29908,.T.);
#42275=EDGE_CURVE('',#34355,#34356,#2929,.T.);
#42276=EDGE_CURVE('',#34356,#34357,#29909,.T.);
#42277=EDGE_CURVE('',#34357,#34358,#29910,.T.);
#42278=EDGE_CURVE('',#34358,#34359,#29911,.T.);
#42279=EDGE_CURVE('',#34360,#34359,#2930,.T.);
#42280=EDGE_CURVE('',#34360,#34361,#2931,.T.);
#42281=EDGE_CURVE('',#34361,#34351,#2932,.T.);
#42282=EDGE_CURVE('',#34362,#34361,#29912,.T.);
#42283=EDGE_CURVE('',#34333,#34362,#29913,.T.);
#42284=EDGE_CURVE('',#34363,#34333,#29914,.T.);
#42285=EDGE_CURVE('',#34364,#34362,#29915,.T.);
#42286=EDGE_CURVE('',#34363,#34364,#29916,.T.);
#42287=EDGE_CURVE('',#34360,#34364,#31013,.T.);
#42288=EDGE_CURVE('',#34360,#34365,#31014,.T.);
#42289=EDGE_CURVE('',#34365,#34366,#31015,.T.);
#42290=EDGE_CURVE('',#34366,#34363,#31016,.T.);
#42291=EDGE_CURVE('',#34366,#34334,#31017,.T.);
#42292=EDGE_CURVE('',#34367,#34335,#29917,.T.);
#42293=EDGE_CURVE('',#34367,#34366,#31018,.T.);
#42294=EDGE_CURVE('',#34365,#34368,#31019,.T.);
#42295=EDGE_CURVE('',#34368,#34367,#29918,.T.);
#42296=EDGE_CURVE('',#34341,#34367,#29919,.T.);
#42297=EDGE_CURVE('',#34368,#34167,#29920,.T.);
#42298=EDGE_CURVE('',#34172,#34344,#29921,.T.);
#42299=EDGE_CURVE('',#34280,#34368,#2933,.T.);
#42300=EDGE_CURVE('',#34365,#34369,#2934,.T.);
#42301=EDGE_CURVE('',#34369,#34280,#2935,.T.);
#42302=EDGE_CURVE('',#34370,#34371,#2936,.T.);
#42303=EDGE_CURVE('',#34371,#34372,#2937,.T.);
#42304=EDGE_CURVE('',#34372,#33701,#2938,.T.);
#42305=EDGE_CURVE('',#34370,#33701,#31020,.T.);
#42306=EDGE_CURVE('',#34126,#34369,#31021,.T.);
#42307=EDGE_CURVE('',#34359,#34369,#31022,.T.);
#42308=EDGE_CURVE('',#34126,#34359,#31023,.T.);
#42309=EDGE_CURVE('',#34127,#34358,#29922,.T.);
#42310=EDGE_CURVE('',#34373,#34357,#29923,.T.);
#42311=EDGE_CURVE('',#34373,#34127,#29924,.T.);
#42312=EDGE_CURVE('',#34128,#34374,#29925,.T.);
#42313=EDGE_CURVE('',#34373,#34375,#2675,.T.);
#42314=EDGE_CURVE('',#34374,#34375,#29926,.T.);
#42315=EDGE_CURVE('',#34375,#34376,#2676,.T.);
#42316=EDGE_CURVE('',#34377,#34376,#29927,.T.);
#42317=EDGE_CURVE('',#34374,#34377,#31024,.T.);
#42318=EDGE_CURVE('',#34378,#34377,#29928,.T.);
#42319=EDGE_CURVE('',#34379,#34378,#29929,.T.);
#42320=EDGE_CURVE('',#34379,#34374,#29930,.T.);
#42321=EDGE_CURVE('',#34380,#34379,#2677,.T.);
#42322=EDGE_CURVE('',#34128,#34380,#29931,.T.);
#42323=EDGE_CURVE('',#34380,#34381,#29932,.T.);
#42324=EDGE_CURVE('',#34381,#34133,#29933,.T.);
#42325=EDGE_CURVE('',#33756,#34382,#2939,.T.);
#42326=EDGE_CURVE('',#34382,#34140,#2678,.T.);
#42327=EDGE_CURVE('',#34139,#34383,#31025,.T.);
#42328=EDGE_CURVE('',#33759,#34383,#29934,.T.);
#42329=EDGE_CURVE('',#34384,#34107,#29935,.T.);
#42330=EDGE_CURVE('',#34384,#33756,#29936,.T.);
#42331=EDGE_CURVE('',#34384,#34382,#29937,.T.);
#42332=EDGE_CURVE('',#34385,#33694,#2940,.T.);
#42333=EDGE_CURVE('',#34385,#34386,#29938,.T.);
#42334=EDGE_CURVE('',#33694,#34386,#2941,.T.);
#42335=EDGE_CURVE('',#34387,#34388,#29939,.T.);
#42336=EDGE_CURVE('',#34382,#34387,#29940,.T.);
#42337=EDGE_CURVE('',#34388,#34384,#29941,.T.);
#42338=EDGE_CURVE('',#34105,#34388,#29942,.T.);
#42339=EDGE_CURVE('',#34137,#34387,#29943,.T.);
#42340=EDGE_CURVE('',#34389,#34121,#31026,.T.);
#42341=EDGE_CURVE('',#34389,#34120,#29944,.T.);
#42342=EDGE_CURVE('',#34120,#34390,#1761,.T.);
#42343=EDGE_CURVE('',#34391,#34390,#29945,.T.);
#42344=EDGE_CURVE('',#34389,#34391,#29946,.T.);
#42345=EDGE_CURVE('',#34392,#34391,#29947,.T.);
#42346=EDGE_CURVE('',#34393,#34392,#31027,.T.);
#42347=EDGE_CURVE('',#34393,#34389,#2679,.T.);
#42348=EDGE_CURVE('',#34393,#34203,#31028,.T.);
#42349=EDGE_CURVE('',#34394,#34395,#31029,.T.);
#42350=EDGE_CURVE('',#34395,#34396,#29948,.T.);
#42351=EDGE_CURVE('',#34396,#34397,#31030,.T.);
#42352=EDGE_CURVE('',#34397,#34398,#29949,.T.);
#42353=EDGE_CURVE('',#34398,#34399,#29950,.T.);
#42354=EDGE_CURVE('',#34399,#34394,#29951,.T.);
#42355=EDGE_CURVE('',#34399,#34400,#31031,.T.);
#42356=EDGE_CURVE('',#34401,#34400,#29952,.T.);
#42357=EDGE_CURVE('',#34394,#34401,#31032,.T.);
#42358=EDGE_CURVE('',#34394,#34402,#29953,.T.);
#42359=EDGE_CURVE('',#34403,#34401,#29954,.T.);
#42360=EDGE_CURVE('',#34403,#34402,#31033,.T.);
#42361=EDGE_CURVE('',#33754,#34403,#29955,.T.);
#42362=EDGE_CURVE('',#33754,#34404,#31034,.T.);
#42363=EDGE_CURVE('',#34404,#34402,#29956,.T.);
#42364=EDGE_CURVE('',#34404,#34395,#29957,.T.);
#42365=EDGE_CURVE('',#33753,#34395,#31035,.T.);
#42366=EDGE_CURVE('',#33751,#34396,#31036,.T.);
#42367=EDGE_CURVE('',#33750,#34405,#31037,.T.);
#42368=EDGE_CURVE('',#34396,#34405,#29958,.T.);
#42369=EDGE_CURVE('',#34406,#34397,#29959,.T.);
#42370=EDGE_CURVE('',#34406,#34405,#29960,.T.);
#42371=EDGE_CURVE('',#34407,#33750,#29961,.T.);
#42372=EDGE_CURVE('',#34406,#34407,#31038,.T.);
#42373=EDGE_CURVE('',#34408,#34407,#29962,.T.);
#42374=EDGE_CURVE('',#34397,#34408,#31039,.T.);
#42375=EDGE_CURVE('',#34409,#34408,#29963,.T.);
#42376=EDGE_CURVE('',#34398,#34409,#31040,.T.);
#42377=EDGE_CURVE('',#34410,#34409,#29964,.T.);
#42378=EDGE_CURVE('',#34400,#34410,#29965,.T.);
#42379=EDGE_CURVE('',#34409,#34411,#31041,.T.);
#42380=EDGE_CURVE('',#34412,#34411,#31042,.T.);
#42381=EDGE_CURVE('',#34413,#34412,#31043,.T.);
#42382=EDGE_CURVE('',#34414,#34413,#31044,.T.);
#42383=EDGE_CURVE('',#34414,#34400,#31045,.T.);
#42384=EDGE_CURVE('',#34403,#34414,#2942,.T.);
#42385=EDGE_CURVE('',#34415,#33755,#29966,.T.);
#42386=EDGE_CURVE('',#34416,#34414,#31046,.T.);
#42387=EDGE_CURVE('',#34417,#34416,#2943,.T.);
#42388=EDGE_CURVE('',#34417,#34418,#29967,.T.);
#42389=EDGE_CURVE('',#34419,#34418,#2944,.T.);
#42390=EDGE_CURVE('',#34420,#34419,#31047,.T.);
#42391=EDGE_CURVE('',#34420,#34415,#2945,.T.);
#42392=EDGE_CURVE('',#34421,#34422,#29968,.T.);
#42393=EDGE_CURVE('',#34422,#34415,#29969,.T.);
#42394=EDGE_CURVE('',#34421,#34420,#31048,.T.);
#42395=EDGE_CURVE('',#34423,#34424,#29970,.T.);
#42396=EDGE_CURVE('',#34424,#34421,#29971,.T.);
#42397=EDGE_CURVE('',#34425,#34420,#31049,.T.);
#42398=EDGE_CURVE('',#34426,#34425,#31050,.T.);
#42399=EDGE_CURVE('',#34427,#34426,#31051,.T.);
#42400=EDGE_CURVE('',#34427,#34423,#31052,.T.);
#42401=EDGE_CURVE('',#34428,#34429,#29972,.T.);
#42402=EDGE_CURVE('',#34429,#34423,#29973,.T.);
#42403=EDGE_CURVE('',#34428,#34427,#2946,.T.);
#42404=EDGE_CURVE('',#33749,#34428,#29974,.T.);
#42405=EDGE_CURVE('',#34430,#34427,#31053,.T.);
#42406=EDGE_CURVE('',#34430,#34431,#2947,.T.);
#42407=EDGE_CURVE('',#34431,#34432,#29975,.T.);
#42408=EDGE_CURVE('',#34433,#34432,#2948,.T.);
#42409=EDGE_CURVE('',#34433,#34434,#29976,.T.);
#42410=EDGE_CURVE('',#34434,#34435,#2949,.T.);
#42411=EDGE_CURVE('',#34411,#34435,#31054,.T.);
#42412=EDGE_CURVE('',#34411,#34407,#2950,.T.);
#42413=EDGE_CURVE('',#33748,#34436,#31055,.T.);
#42414=EDGE_CURVE('',#34437,#34436,#29977,.T.);
#42415=EDGE_CURVE('',#33749,#34437,#31056,.T.);
#42416=EDGE_CURVE('',#34437,#34438,#29978,.T.);
#42417=EDGE_CURVE('',#34428,#34438,#31057,.T.);
#42418=EDGE_CURVE('',#34439,#34438,#29979,.T.);
#42419=EDGE_CURVE('',#34439,#34429,#31058,.T.);
#42420=EDGE_CURVE('',#34440,#34439,#29980,.T.);
#42421=EDGE_CURVE('',#34440,#34423,#31059,.T.);
#42422=EDGE_CURVE('',#34441,#34440,#29981,.F.);
#42423=EDGE_CURVE('',#34441,#34421,#31060,.T.);
#42424=EDGE_CURVE('',#34442,#34441,#29982,.T.);
#42425=EDGE_CURVE('',#34442,#34422,#31061,.T.);
#42426=EDGE_CURVE('',#34443,#34442,#29983,.T.);
#42427=EDGE_CURVE('',#34443,#34415,#31062,.T.);
#42428=EDGE_CURVE('',#34443,#34444,#29984,.T.);
#42429=EDGE_CURVE('',#33755,#34444,#31063,.T.);
#42430=EDGE_CURVE('',#34445,#34444,#29985,.T.);
#42431=EDGE_CURVE('',#33746,#34445,#31064,.T.);
#42432=EDGE_CURVE('',#34436,#34445,#29986,.T.);
#42433=EDGE_CURVE('',#34439,#34436,#31065,.T.);
#42434=EDGE_CURVE('',#34445,#34442,#31066,.T.);
#42435=EDGE_CURVE('',#34412,#34446,#31067,.T.);
#42436=EDGE_CURVE('',#34446,#34435,#31068,.T.);
#42437=EDGE_CURVE('',#34446,#33744,#31069,.T.);
#42438=EDGE_CURVE('',#34435,#33696,#31070,.T.);
#42439=EDGE_CURVE('',#33697,#34416,#31071,.T.);
#42440=EDGE_CURVE('',#34416,#34447,#31072,.T.);
#42441=EDGE_CURVE('',#33745,#34447,#31073,.T.);
#42442=EDGE_CURVE('',#34447,#34413,#31074,.T.);
#42443=EDGE_CURVE('',#33700,#34417,#29987,.T.);
#42444=EDGE_CURVE('',#33726,#34417,#29988,.T.);
#42445=EDGE_CURVE('',#33727,#33700,#29989,.T.);
#42446=EDGE_CURVE('',#33728,#33698,#31075,.T.);
#42447=EDGE_CURVE('',#34448,#33698,#29990,.T.);
#42448=EDGE_CURVE('',#33729,#34448,#29991,.T.);
#42449=EDGE_CURVE('',#33729,#34449,#29992,.T.);
#42450=EDGE_CURVE('',#34434,#34448,#29993,.T.);
#42451=EDGE_CURVE('',#34449,#34434,#29994,.T.);
#42452=EDGE_CURVE('',#34433,#34449,#29995,.T.);
#42453=EDGE_CURVE('',#33739,#33730,#29996,.T.);
#42454=EDGE_CURVE('',#34433,#34450,#29997,.T.);
#42455=EDGE_CURVE('',#34450,#34432,#29998,.T.);
#42456=EDGE_CURVE('',#34451,#34432,#29999,.T.);
#42457=EDGE_CURVE('',#34451,#33740,#30000,.T.);
#42458=EDGE_CURVE('',#33743,#34418,#30001,.T.);
#42459=EDGE_CURVE('',#33742,#33723,#30002,.T.);
#42460=EDGE_CURVE('',#34418,#33723,#30003,.T.);
#42461=EDGE_CURVE('',#34419,#33718,#31076,.T.);
#42462=EDGE_CURVE('',#33719,#34430,#31077,.T.);
#42463=EDGE_CURVE('',#33724,#34452,#30004,.T.);
#42464=EDGE_CURVE('',#34431,#34452,#30005,.T.);
#42465=EDGE_CURVE('',#34451,#34431,#30006,.T.);
#42466=EDGE_CURVE('',#33740,#34452,#30007,.T.);
#42467=EDGE_CURVE('',#33741,#33724,#31078,.T.);
#42468=EDGE_CURVE('',#34430,#34453,#31079,.T.);
#42469=EDGE_CURVE('',#33720,#34453,#31080,.T.);
#42470=EDGE_CURVE('',#34454,#33721,#31081,.T.);
#42471=EDGE_CURVE('',#34454,#34419,#31082,.T.);
#42472=EDGE_CURVE('',#34425,#34454,#31083,.T.);
#42473=EDGE_CURVE('',#34453,#34426,#31084,.T.);
#42474=EDGE_CURVE('',#34238,#34455,#30008,.T.);
#42475=EDGE_CURVE('',#34455,#33730,#30009,.T.);
#42476=EDGE_CURVE('',#34455,#34456,#30010,.T.);
#42477=EDGE_CURVE('',#34456,#33739,#31085,.T.);
#42478=EDGE_CURVE('',#34456,#34237,#30011,.T.);
#42479=EDGE_CURVE('',#34236,#34457,#30012,.T.);
#42480=EDGE_CURVE('',#34457,#34458,#30013,.T.);
#42481=EDGE_CURVE('',#34458,#34239,#30014,.T.);
#42482=EDGE_CURVE('',#34458,#34459,#30015,.T.);
#42483=EDGE_CURVE('',#34460,#34459,#30016,.T.);
#42484=EDGE_CURVE('',#34239,#34460,#31086,.T.);
#42485=EDGE_CURVE('',#34461,#34460,#30017,.T.);
#42486=EDGE_CURVE('',#34240,#34461,#31087,.T.);
#42487=EDGE_CURVE('',#34462,#34461,#30018,.T.);
#42488=EDGE_CURVE('',#34462,#34463,#31088,.T.);
#42489=EDGE_CURVE('',#34240,#34463,#30019,.T.);
#42490=EDGE_CURVE('',#34463,#34242,#30020,.T.);
#42491=EDGE_CURVE('',#34464,#34462,#30021,.T.);
#42492=EDGE_CURVE('',#34464,#34242,#31089,.T.);
#42493=EDGE_CURVE('',#34465,#34464,#30022,.T.);
#42494=EDGE_CURVE('',#34465,#34232,#30023,.T.);
#42495=EDGE_CURVE('',#34466,#34465,#30024,.T.);
#42496=EDGE_CURVE('',#34466,#34233,#30025,.T.);
#42497=EDGE_CURVE('',#34467,#34466,#30026,.T.);
#42498=EDGE_CURVE('',#34467,#34468,#31090,.T.);
#42499=EDGE_CURVE('',#34233,#34468,#30027,.T.);
#42500=EDGE_CURVE('',#34468,#34235,#30028,.T.);
#42501=EDGE_CURVE('',#34469,#34467,#30029,.T.);
#42502=EDGE_CURVE('',#34469,#34235,#31091,.T.);
#42503=EDGE_CURVE('',#34470,#34469,#30030,.T.);
#42504=EDGE_CURVE('',#34236,#34470,#31092,.T.);
#42505=EDGE_CURVE('',#34471,#34470,#30031,.T.);
#42506=EDGE_CURVE('',#34457,#34471,#30032,.T.);
#42507=EDGE_CURVE('',#34459,#34471,#30033,.F.);
#42508=EDGE_CURVE('',#34462,#34459,#31093,.T.);
#42509=EDGE_CURVE('',#34471,#34467,#31094,.T.);
#42510=EDGE_CURVE('',#33708,#33709,#31095,.T.);
#42511=EDGE_CURVE('',#33763,#34472,#2951,.T.);
#42512=EDGE_CURVE('',#34472,#34356,#31096,.T.);
#42513=EDGE_CURVE('',#34355,#34473,#31097,.T.);
#42514=EDGE_CURVE('',#34473,#33762,#2952,.T.);
#42515=EDGE_CURVE('',#34473,#34474,#30034,.T.);
#42516=EDGE_CURVE('',#34474,#34475,#30035,.T.);
#42517=EDGE_CURVE('',#34475,#34476,#30036,.T.);
#42518=EDGE_CURVE('',#34476,#34477,#30037,.T.);
#42519=EDGE_CURVE('',#34478,#34477,#2953,.T.);
#42520=EDGE_CURVE('',#34478,#34378,#30038,.T.);
#42521=EDGE_CURVE('',#34376,#34472,#30039,.T.);
#42522=EDGE_CURVE('',#34479,#34472,#31098,.T.);
#42523=EDGE_CURVE('',#34375,#34479,#31099,.T.);
#42524=EDGE_CURVE('',#34479,#34373,#30040,.T.);
#42525=EDGE_CURVE('',#34479,#34356,#31100,.T.);
#42526=EDGE_CURVE('',#34480,#34478,#1762,.T.);
#42527=EDGE_CURVE('',#34480,#34379,#30041,.T.);
#42528=EDGE_CURVE('',#34381,#34481,#30042,.T.);
#42529=EDGE_CURVE('',#34482,#34480,#30043,.T.);
#42530=EDGE_CURVE('',#34481,#34482,#30044,.T.);
#42531=EDGE_CURVE('',#34482,#34477,#1763,.T.);
#42532=EDGE_CURVE('',#34481,#34476,#30045,.T.);
#42533=EDGE_CURVE('',#34483,#34475,#2680,.T.);
#42534=EDGE_CURVE('',#34483,#34481,#30046,.T.);
#42535=EDGE_CURVE('',#34133,#34483,#30047,.T.);
#42536=EDGE_CURVE('',#34484,#34483,#30048,.T.);
#42537=EDGE_CURVE('',#34484,#34485,#2681,.T.);
#42538=EDGE_CURVE('',#34134,#34485,#30049,.T.);
#42539=EDGE_CURVE('',#34485,#34354,#30050,.T.);
#42540=EDGE_CURVE('',#34134,#34353,#30051,.T.);
#42541=EDGE_CURVE('',#34135,#34352,#31101,.T.);
#42542=EDGE_CURVE('',#34372,#34352,#31102,.T.);
#42543=EDGE_CURVE('',#34135,#34372,#31103,.T.);
#42544=EDGE_CURVE('',#34136,#34371,#30052,.T.);
#42545=EDGE_CURVE('',#34486,#34371,#30053,.T.);
#42546=EDGE_CURVE('',#34110,#34486,#30054,.T.);
#42547=EDGE_CURVE('',#34197,#34486,#30055,.T.);
#42548=EDGE_CURVE('',#34157,#34370,#30056,.T.);
#42549=EDGE_CURVE('',#34370,#34349,#1764,.T.);
#42550=EDGE_CURVE('',#34160,#34162,#30057,.T.);
#42551=EDGE_CURVE('',#34487,#34355,#31104,.T.);
#42552=EDGE_CURVE('',#34485,#34487,#30058,.T.);
#42553=EDGE_CURVE('',#34487,#34484,#31105,.T.);
#42554=EDGE_CURVE('',#34484,#34474,#31106,.T.);
#42555=EDGE_CURVE('',#34487,#34473,#31107,.T.);
#42556=EDGE_CURVE('',#34477,#34478,#30059,.T.);
#42557=EDGE_CURVE('',#34383,#33691,#30060,.T.);
#42558=EDGE_CURVE('',#34146,#34385,#30061,.T.);
#42559=EDGE_CURVE('',#34488,#33691,#2954,.T.);
#42560=EDGE_CURVE('',#34488,#34180,#31108,.T.);
#42561=EDGE_CURVE('',#34488,#34096,#1765,.T.);
#42562=EDGE_CURVE('',#34096,#34489,#31109,.T.);
#42563=EDGE_CURVE('',#34488,#34489,#30062,.T.);
#42564=EDGE_CURVE('',#33759,#34490,#2955,.T.);
#42565=EDGE_CURVE('',#34489,#34177,#31110,.T.);
#42566=EDGE_CURVE('',#34175,#34490,#30063,.T.);
#42567=EDGE_CURVE('',#33805,#34144,#31111,.T.);
#42568=EDGE_CURVE('',#34142,#33806,#31112,.T.);
#42569=EDGE_CURVE('',#34106,#34083,#31113,.T.);
#42570=EDGE_CURVE('',#34084,#34108,#31114,.T.);
#42571=EDGE_CURVE('',#34108,#34490,#31115,.T.);
#42572=EDGE_CURVE('',#34085,#34490,#30064,.T.);
#42573=EDGE_CURVE('',#34093,#33805,#31116,.T.);
#42574=EDGE_CURVE('',#34386,#34181,#31117,.T.);
#42575=EDGE_CURVE('',#34386,#34491,#30065,.T.);
#42576=EDGE_CURVE('',#34491,#34179,#30066,.T.);
#42577=EDGE_CURVE('',#34491,#34492,#30067,.T.);
#42578=EDGE_CURVE('',#34385,#34492,#31118,.T.);
#42579=EDGE_CURVE('',#34492,#34145,#30068,.T.);
#42580=EDGE_CURVE('',#34182,#34393,#2682,.T.);
#42581=EDGE_CURVE('',#34183,#34392,#30069,.T.);
#42582=EDGE_CURVE('',#34390,#34148,#31119,.T.);
#42583=EDGE_CURVE('',#34150,#34148,#30070,.T.);
#42584=EDGE_CURVE('',#34154,#34153,#30071,.T.);
#42585=EDGE_CURVE('',#34364,#34361,#30072,.T.);
#42586=EDGE_CURVE('',#34303,#34323,#30073,.T.);
#42587=EDGE_CURVE('',#34304,#34322,#30074,.T.);
#42588=EDGE_CURVE('',#34306,#34321,#31120,.T.);
#42589=EDGE_CURVE('',#34308,#34320,#30075,.T.);
#42590=EDGE_CURVE('',#34196,#34210,#30076,.T.);
#42591=EDGE_CURVE('',#34210,#34204,#31121,.T.);
#42592=EDGE_CURVE('',#34211,#33803,#30077,.T.);
#42593=EDGE_CURVE('',#34082,#34089,#31122,.T.);
#52473=ORIENTED_EDGE('',*,*,#41069,.T.);
#52474=ORIENTED_EDGE('',*,*,#41070,.F.);
#52475=ORIENTED_EDGE('',*,*,#41071,.F.);
#52476=ORIENTED_EDGE('',*,*,#41072,.F.);
#52477=ORIENTED_EDGE('',*,*,#41073,.T.);
#52478=ORIENTED_EDGE('',*,*,#41074,.T.);
#52479=ORIENTED_EDGE('',*,*,#41075,.T.);
#52480=ORIENTED_EDGE('',*,*,#41076,.F.);
#52481=ORIENTED_EDGE('',*,*,#41071,.T.);
#52482=ORIENTED_EDGE('',*,*,#41077,.F.);
#52483=ORIENTED_EDGE('',*,*,#41078,.F.);
#52484=ORIENTED_EDGE('',*,*,#41079,.T.);
#52485=ORIENTED_EDGE('',*,*,#41077,.T.);
#52486=ORIENTED_EDGE('',*,*,#41080,.F.);
#52487=ORIENTED_EDGE('',*,*,#41078,.T.);
#52488=ORIENTED_EDGE('',*,*,#41070,.T.);
#52489=ORIENTED_EDGE('',*,*,#41075,.F.);
#52490=ORIENTED_EDGE('',*,*,#41081,.F.);
#52491=ORIENTED_EDGE('',*,*,#41073,.F.);
#52492=ORIENTED_EDGE('',*,*,#41069,.F.);
#52493=ORIENTED_EDGE('',*,*,#41072,.T.);
#52494=ORIENTED_EDGE('',*,*,#41076,.T.);
#52495=ORIENTED_EDGE('',*,*,#41079,.F.);
#52496=ORIENTED_EDGE('',*,*,#41080,.T.);
#52497=ORIENTED_EDGE('',*,*,#41074,.F.);
#52498=ORIENTED_EDGE('',*,*,#41081,.T.);
#52499=ORIENTED_EDGE('',*,*,#41082,.T.);
#52500=ORIENTED_EDGE('',*,*,#41083,.F.);
#52501=ORIENTED_EDGE('',*,*,#41084,.F.);
#52502=ORIENTED_EDGE('',*,*,#41085,.F.);
#52503=ORIENTED_EDGE('',*,*,#41086,.F.);
#52504=ORIENTED_EDGE('',*,*,#41087,.F.);
#52505=ORIENTED_EDGE('',*,*,#41082,.F.);
#52506=ORIENTED_EDGE('',*,*,#41088,.T.);
#52507=ORIENTED_EDGE('',*,*,#41089,.T.);
#52508=ORIENTED_EDGE('',*,*,#41090,.T.);
#52509=ORIENTED_EDGE('',*,*,#41091,.F.);
#52510=ORIENTED_EDGE('',*,*,#41088,.F.);
#52511=ORIENTED_EDGE('',*,*,#41083,.T.);
#52512=ORIENTED_EDGE('',*,*,#41092,.T.);
#52513=ORIENTED_EDGE('',*,*,#41087,.T.);
#52514=ORIENTED_EDGE('',*,*,#41093,.T.);
#52515=ORIENTED_EDGE('',*,*,#41092,.F.);
#52516=ORIENTED_EDGE('',*,*,#41094,.F.);
#52517=ORIENTED_EDGE('',*,*,#41084,.T.);
#52518=ORIENTED_EDGE('',*,*,#41090,.F.);
#52519=ORIENTED_EDGE('',*,*,#41086,.T.);
#52520=ORIENTED_EDGE('',*,*,#41085,.T.);
#52521=ORIENTED_EDGE('',*,*,#41094,.T.);
#52522=ORIENTED_EDGE('',*,*,#41089,.F.);
#52523=ORIENTED_EDGE('',*,*,#41091,.T.);
#52524=ORIENTED_EDGE('',*,*,#41093,.F.);
#52525=ORIENTED_EDGE('',*,*,#41095,.F.);
#52526=ORIENTED_EDGE('',*,*,#41096,.T.);
#52527=ORIENTED_EDGE('',*,*,#41097,.F.);
#52528=ORIENTED_EDGE('',*,*,#41098,.T.);
#52529=ORIENTED_EDGE('',*,*,#41099,.F.);
#52530=ORIENTED_EDGE('',*,*,#41100,.T.);
#52531=ORIENTED_EDGE('',*,*,#41101,.F.);
#52532=ORIENTED_EDGE('',*,*,#41102,.T.);
#52533=ORIENTED_EDGE('',*,*,#41103,.F.);
#52534=ORIENTED_EDGE('',*,*,#41104,.F.);
#52535=ORIENTED_EDGE('',*,*,#41105,.T.);
#52536=ORIENTED_EDGE('',*,*,#41104,.T.);
#52537=ORIENTED_EDGE('',*,*,#41106,.F.);
#52538=ORIENTED_EDGE('',*,*,#41107,.T.);
#52539=ORIENTED_EDGE('',*,*,#41098,.F.);
#52540=ORIENTED_EDGE('',*,*,#41108,.T.);
#52541=ORIENTED_EDGE('',*,*,#41106,.T.);
#52542=ORIENTED_EDGE('',*,*,#41109,.F.);
#52543=ORIENTED_EDGE('',*,*,#41110,.T.);
#52544=ORIENTED_EDGE('',*,*,#41099,.T.);
#52545=ORIENTED_EDGE('',*,*,#41109,.T.);
#52546=ORIENTED_EDGE('',*,*,#41103,.T.);
#52547=ORIENTED_EDGE('',*,*,#41100,.F.);
#52548=ORIENTED_EDGE('',*,*,#41110,.F.);
#52549=ORIENTED_EDGE('',*,*,#41102,.F.);
#52550=ORIENTED_EDGE('',*,*,#41111,.T.);
#52551=ORIENTED_EDGE('',*,*,#41112,.F.);
#52552=ORIENTED_EDGE('',*,*,#41101,.T.);
#52553=ORIENTED_EDGE('',*,*,#41111,.F.);
#52554=ORIENTED_EDGE('',*,*,#41096,.F.);
#52555=ORIENTED_EDGE('',*,*,#41113,.T.);
#52556=ORIENTED_EDGE('',*,*,#41107,.F.);
#52557=ORIENTED_EDGE('',*,*,#41114,.F.);
#52558=ORIENTED_EDGE('',*,*,#41113,.F.);
#52559=ORIENTED_EDGE('',*,*,#41095,.T.);
#52560=ORIENTED_EDGE('',*,*,#41112,.T.);
#52561=ORIENTED_EDGE('',*,*,#41105,.F.);
#52562=ORIENTED_EDGE('',*,*,#41108,.F.);
#52563=ORIENTED_EDGE('',*,*,#41097,.T.);
#52564=ORIENTED_EDGE('',*,*,#41114,.T.);
#52565=ORIENTED_EDGE('',*,*,#41115,.F.);
#52566=ORIENTED_EDGE('',*,*,#41116,.T.);
#52567=ORIENTED_EDGE('',*,*,#41117,.F.);
#52568=ORIENTED_EDGE('',*,*,#41118,.F.);
#52569=ORIENTED_EDGE('',*,*,#41119,.T.);
#52570=ORIENTED_EDGE('',*,*,#41120,.F.);
#52571=ORIENTED_EDGE('',*,*,#41121,.T.);
#52572=ORIENTED_EDGE('',*,*,#41122,.T.);
#52573=ORIENTED_EDGE('',*,*,#41123,.F.);
#52574=ORIENTED_EDGE('',*,*,#41124,.T.);
#52575=ORIENTED_EDGE('',*,*,#41123,.T.);
#52576=ORIENTED_EDGE('',*,*,#41125,.F.);
#52577=ORIENTED_EDGE('',*,*,#41126,.F.);
#52578=ORIENTED_EDGE('',*,*,#41127,.T.);
#52579=ORIENTED_EDGE('',*,*,#41119,.F.);
#52580=ORIENTED_EDGE('',*,*,#41128,.T.);
#52581=ORIENTED_EDGE('',*,*,#41126,.T.);
#52582=ORIENTED_EDGE('',*,*,#41129,.F.);
#52583=ORIENTED_EDGE('',*,*,#41130,.T.);
#52584=ORIENTED_EDGE('',*,*,#41120,.T.);
#52585=ORIENTED_EDGE('',*,*,#41129,.T.);
#52586=ORIENTED_EDGE('',*,*,#41125,.T.);
#52587=ORIENTED_EDGE('',*,*,#41121,.F.);
#52588=ORIENTED_EDGE('',*,*,#41130,.F.);
#52589=ORIENTED_EDGE('',*,*,#41122,.F.);
#52590=ORIENTED_EDGE('',*,*,#41131,.T.);
#52591=ORIENTED_EDGE('',*,*,#41128,.F.);
#52592=ORIENTED_EDGE('',*,*,#41118,.T.);
#52593=ORIENTED_EDGE('',*,*,#41132,.T.);
#52594=ORIENTED_EDGE('',*,*,#41132,.F.);
#52595=ORIENTED_EDGE('',*,*,#41117,.T.);
#52596=ORIENTED_EDGE('',*,*,#41133,.F.);
#52597=ORIENTED_EDGE('',*,*,#41127,.F.);
#52598=ORIENTED_EDGE('',*,*,#41116,.F.);
#52599=ORIENTED_EDGE('',*,*,#41134,.F.);
#52600=ORIENTED_EDGE('',*,*,#41124,.F.);
#52601=ORIENTED_EDGE('',*,*,#41133,.T.);
#52602=ORIENTED_EDGE('',*,*,#41134,.T.);
#52603=ORIENTED_EDGE('',*,*,#41115,.T.);
#52604=ORIENTED_EDGE('',*,*,#41131,.F.);
#52605=ORIENTED_EDGE('',*,*,#41135,.F.);
#52606=ORIENTED_EDGE('',*,*,#41136,.T.);
#52607=ORIENTED_EDGE('',*,*,#41137,.T.);
#52608=ORIENTED_EDGE('',*,*,#41138,.T.);
#52609=ORIENTED_EDGE('',*,*,#41139,.T.);
#52610=ORIENTED_EDGE('',*,*,#41140,.F.);
#52611=ORIENTED_EDGE('',*,*,#41141,.T.);
#52612=ORIENTED_EDGE('',*,*,#41142,.T.);
#52613=ORIENTED_EDGE('',*,*,#41143,.T.);
#52614=ORIENTED_EDGE('',*,*,#41135,.T.);
#52615=ORIENTED_EDGE('',*,*,#41144,.F.);
#52616=ORIENTED_EDGE('',*,*,#41145,.T.);
#52617=ORIENTED_EDGE('',*,*,#41140,.T.);
#52618=ORIENTED_EDGE('',*,*,#41146,.T.);
#52619=ORIENTED_EDGE('',*,*,#41147,.T.);
#52620=ORIENTED_EDGE('',*,*,#41148,.T.);
#52621=ORIENTED_EDGE('',*,*,#41149,.T.);
#52622=ORIENTED_EDGE('',*,*,#41150,.F.);
#52623=ORIENTED_EDGE('',*,*,#41151,.F.);
#52624=ORIENTED_EDGE('',*,*,#41152,.F.);
#52625=ORIENTED_EDGE('',*,*,#41153,.T.);
#52626=ORIENTED_EDGE('',*,*,#41154,.T.);
#52627=ORIENTED_EDGE('',*,*,#41148,.F.);
#52628=ORIENTED_EDGE('',*,*,#41155,.F.);
#52629=ORIENTED_EDGE('',*,*,#41156,.T.);
#52630=ORIENTED_EDGE('',*,*,#41157,.F.);
#52631=ORIENTED_EDGE('',*,*,#41158,.T.);
#52632=ORIENTED_EDGE('',*,*,#41159,.T.);
#52633=ORIENTED_EDGE('',*,*,#41160,.F.);
#52634=ORIENTED_EDGE('',*,*,#41161,.T.);
#52635=ORIENTED_EDGE('',*,*,#41162,.T.);
#52636=ORIENTED_EDGE('',*,*,#41163,.F.);
#52637=ORIENTED_EDGE('',*,*,#41164,.T.);
#52638=ORIENTED_EDGE('',*,*,#41165,.T.);
#52639=ORIENTED_EDGE('',*,*,#41166,.T.);
#52640=ORIENTED_EDGE('',*,*,#41161,.F.);
#52641=ORIENTED_EDGE('',*,*,#41167,.T.);
#52642=ORIENTED_EDGE('',*,*,#41168,.T.);
#52643=ORIENTED_EDGE('',*,*,#41169,.T.);
#52644=ORIENTED_EDGE('',*,*,#41165,.F.);
#52645=ORIENTED_EDGE('',*,*,#41170,.T.);
#52646=ORIENTED_EDGE('',*,*,#41171,.T.);
#52647=ORIENTED_EDGE('',*,*,#41172,.T.);
#52648=ORIENTED_EDGE('',*,*,#41168,.F.);
#52649=ORIENTED_EDGE('',*,*,#41173,.T.);
#52650=ORIENTED_EDGE('',*,*,#41174,.F.);
#52651=ORIENTED_EDGE('',*,*,#41175,.T.);
#52652=ORIENTED_EDGE('',*,*,#41176,.T.);
#52653=ORIENTED_EDGE('',*,*,#41177,.T.);
#52654=ORIENTED_EDGE('',*,*,#41178,.T.);
#52655=ORIENTED_EDGE('',*,*,#41179,.F.);
#52656=ORIENTED_EDGE('',*,*,#41180,.T.);
#52657=ORIENTED_EDGE('',*,*,#41181,.T.);
#52658=ORIENTED_EDGE('',*,*,#41182,.T.);
#52659=ORIENTED_EDGE('',*,*,#41183,.T.);
#52660=ORIENTED_EDGE('',*,*,#41181,.F.);
#52661=ORIENTED_EDGE('',*,*,#41184,.T.);
#52662=ORIENTED_EDGE('',*,*,#41185,.T.);
#52663=ORIENTED_EDGE('',*,*,#41186,.T.);
#52664=ORIENTED_EDGE('',*,*,#41177,.F.);
#52665=ORIENTED_EDGE('',*,*,#41187,.T.);
#52666=ORIENTED_EDGE('',*,*,#41188,.F.);
#52667=ORIENTED_EDGE('',*,*,#41189,.T.);
#52668=ORIENTED_EDGE('',*,*,#41190,.T.);
#52669=ORIENTED_EDGE('',*,*,#41191,.T.);
#52670=ORIENTED_EDGE('',*,*,#41192,.F.);
#52671=ORIENTED_EDGE('',*,*,#41193,.T.);
#52672=ORIENTED_EDGE('',*,*,#41194,.T.);
#52673=ORIENTED_EDGE('',*,*,#41193,.F.);
#52674=ORIENTED_EDGE('',*,*,#41195,.F.);
#52675=ORIENTED_EDGE('',*,*,#41196,.F.);
#52676=ORIENTED_EDGE('',*,*,#41197,.F.);
#52677=ORIENTED_EDGE('',*,*,#41198,.F.);
#52678=ORIENTED_EDGE('',*,*,#41199,.T.);
#52679=ORIENTED_EDGE('',*,*,#41200,.T.);
#52680=ORIENTED_EDGE('',*,*,#41201,.F.);
#52681=ORIENTED_EDGE('',*,*,#41202,.T.);
#52682=ORIENTED_EDGE('',*,*,#41203,.T.);
#52683=ORIENTED_EDGE('',*,*,#41204,.F.);
#52684=ORIENTED_EDGE('',*,*,#41205,.F.);
#52685=ORIENTED_EDGE('',*,*,#41206,.F.);
#52686=ORIENTED_EDGE('',*,*,#41207,.T.);
#52687=ORIENTED_EDGE('',*,*,#41208,.T.);
#52688=ORIENTED_EDGE('',*,*,#41209,.F.);
#52689=ORIENTED_EDGE('',*,*,#41210,.T.);
#52690=ORIENTED_EDGE('',*,*,#41211,.T.);
#52691=ORIENTED_EDGE('',*,*,#41212,.F.);
#52692=ORIENTED_EDGE('',*,*,#41213,.F.);
#52693=ORIENTED_EDGE('',*,*,#41214,.F.);
#52694=ORIENTED_EDGE('',*,*,#41215,.T.);
#52695=ORIENTED_EDGE('',*,*,#41216,.T.);
#52696=ORIENTED_EDGE('',*,*,#41216,.F.);
#52697=ORIENTED_EDGE('',*,*,#41217,.T.);
#52698=ORIENTED_EDGE('',*,*,#41218,.T.);
#52699=ORIENTED_EDGE('',*,*,#41219,.F.);
#52700=ORIENTED_EDGE('',*,*,#41220,.F.);
#52701=ORIENTED_EDGE('',*,*,#41221,.F.);
#52702=ORIENTED_EDGE('',*,*,#41222,.F.);
#52703=ORIENTED_EDGE('',*,*,#41223,.F.);
#52704=ORIENTED_EDGE('',*,*,#41224,.T.);
#52705=ORIENTED_EDGE('',*,*,#41225,.T.);
#52706=ORIENTED_EDGE('',*,*,#41226,.T.);
#52707=ORIENTED_EDGE('',*,*,#41227,.F.);
#52708=ORIENTED_EDGE('',*,*,#41228,.F.);
#52709=ORIENTED_EDGE('',*,*,#41229,.F.);
#52710=ORIENTED_EDGE('',*,*,#41230,.T.);
#52711=ORIENTED_EDGE('',*,*,#41231,.T.);
#52712=ORIENTED_EDGE('',*,*,#41232,.F.);
#52713=ORIENTED_EDGE('',*,*,#41233,.F.);
#52714=ORIENTED_EDGE('',*,*,#41234,.F.);
#52715=ORIENTED_EDGE('',*,*,#41235,.T.);
#52716=ORIENTED_EDGE('',*,*,#41236,.T.);
#52717=ORIENTED_EDGE('',*,*,#41235,.F.);
#52718=ORIENTED_EDGE('',*,*,#41237,.F.);
#52719=ORIENTED_EDGE('',*,*,#41238,.F.);
#52720=ORIENTED_EDGE('',*,*,#41239,.T.);
#52721=ORIENTED_EDGE('',*,*,#41237,.T.);
#52722=ORIENTED_EDGE('',*,*,#41234,.T.);
#52723=ORIENTED_EDGE('',*,*,#41239,.F.);
#52724=ORIENTED_EDGE('',*,*,#41240,.F.);
#52725=ORIENTED_EDGE('',*,*,#41241,.T.);
#52726=ORIENTED_EDGE('',*,*,#41242,.T.);
#52727=ORIENTED_EDGE('',*,*,#41241,.F.);
#52728=ORIENTED_EDGE('',*,*,#41243,.F.);
#52729=ORIENTED_EDGE('',*,*,#41244,.F.);
#52730=ORIENTED_EDGE('',*,*,#41245,.T.);
#52731=ORIENTED_EDGE('',*,*,#41243,.T.);
#52732=ORIENTED_EDGE('',*,*,#41240,.T.);
#52733=ORIENTED_EDGE('',*,*,#41245,.F.);
#52734=ORIENTED_EDGE('',*,*,#41246,.T.);
#52735=ORIENTED_EDGE('',*,*,#41247,.T.);
#52736=ORIENTED_EDGE('',*,*,#41248,.F.);
#52737=ORIENTED_EDGE('',*,*,#41249,.T.);
#52738=ORIENTED_EDGE('',*,*,#41250,.F.);
#52739=ORIENTED_EDGE('',*,*,#41251,.F.);
#52740=ORIENTED_EDGE('',*,*,#41252,.F.);
#52741=ORIENTED_EDGE('',*,*,#41246,.F.);
#52742=ORIENTED_EDGE('',*,*,#41253,.T.);
#52743=ORIENTED_EDGE('',*,*,#41254,.T.);
#52744=ORIENTED_EDGE('',*,*,#41255,.F.);
#52745=ORIENTED_EDGE('',*,*,#41256,.T.);
#52746=ORIENTED_EDGE('',*,*,#41257,.T.);
#52747=ORIENTED_EDGE('',*,*,#41258,.T.);
#52748=ORIENTED_EDGE('',*,*,#41259,.T.);
#52749=ORIENTED_EDGE('',*,*,#41260,.F.);
#52750=ORIENTED_EDGE('',*,*,#41261,.F.);
#52751=ORIENTED_EDGE('',*,*,#41262,.T.);
#52752=ORIENTED_EDGE('',*,*,#41263,.T.);
#52753=ORIENTED_EDGE('',*,*,#41264,.F.);
#52754=ORIENTED_EDGE('',*,*,#41263,.F.);
#52755=ORIENTED_EDGE('',*,*,#41265,.T.);
#52756=ORIENTED_EDGE('',*,*,#41266,.F.);
#52757=ORIENTED_EDGE('',*,*,#41267,.F.);
#52758=ORIENTED_EDGE('',*,*,#41268,.T.);
#52759=ORIENTED_EDGE('',*,*,#41269,.F.);
#52760=ORIENTED_EDGE('',*,*,#41270,.T.);
#52761=ORIENTED_EDGE('',*,*,#41271,.T.);
#52762=ORIENTED_EDGE('',*,*,#41272,.F.);
#52763=ORIENTED_EDGE('',*,*,#41273,.T.);
#52764=ORIENTED_EDGE('',*,*,#41274,.F.);
#52765=ORIENTED_EDGE('',*,*,#41275,.T.);
#52766=ORIENTED_EDGE('',*,*,#41220,.T.);
#52767=ORIENTED_EDGE('',*,*,#41276,.T.);
#52768=ORIENTED_EDGE('',*,*,#41277,.T.);
#52769=ORIENTED_EDGE('',*,*,#41278,.T.);
#52770=ORIENTED_EDGE('',*,*,#41279,.T.);
#52771=ORIENTED_EDGE('',*,*,#41280,.F.);
#52772=ORIENTED_EDGE('',*,*,#41281,.T.);
#52773=ORIENTED_EDGE('',*,*,#41282,.T.);
#52774=ORIENTED_EDGE('',*,*,#41283,.T.);
#52775=ORIENTED_EDGE('',*,*,#41284,.T.);
#52776=ORIENTED_EDGE('',*,*,#41285,.F.);
#52777=ORIENTED_EDGE('',*,*,#41286,.T.);
#52778=ORIENTED_EDGE('',*,*,#41287,.T.);
#52779=ORIENTED_EDGE('',*,*,#41288,.T.);
#52780=ORIENTED_EDGE('',*,*,#41288,.F.);
#52781=ORIENTED_EDGE('',*,*,#41289,.T.);
#52782=ORIENTED_EDGE('',*,*,#41290,.T.);
#52783=ORIENTED_EDGE('',*,*,#41291,.F.);
#52784=ORIENTED_EDGE('',*,*,#41292,.F.);
#52785=ORIENTED_EDGE('',*,*,#41293,.T.);
#52786=ORIENTED_EDGE('',*,*,#41294,.F.);
#52787=ORIENTED_EDGE('',*,*,#41295,.T.);
#52788=ORIENTED_EDGE('',*,*,#41296,.F.);
#52789=ORIENTED_EDGE('',*,*,#41293,.F.);
#52790=ORIENTED_EDGE('',*,*,#41230,.F.);
#52791=ORIENTED_EDGE('',*,*,#41297,.F.);
#52792=ORIENTED_EDGE('',*,*,#41298,.T.);
#52793=ORIENTED_EDGE('',*,*,#41299,.T.);
#52794=ORIENTED_EDGE('',*,*,#41300,.T.);
#52795=ORIENTED_EDGE('',*,*,#41298,.F.);
#52796=ORIENTED_EDGE('',*,*,#41300,.F.);
#52797=ORIENTED_EDGE('',*,*,#41301,.T.);
#52798=ORIENTED_EDGE('',*,*,#41302,.T.);
#52799=ORIENTED_EDGE('',*,*,#41301,.F.);
#52800=ORIENTED_EDGE('',*,*,#41299,.F.);
#52801=ORIENTED_EDGE('',*,*,#41303,.F.);
#52802=ORIENTED_EDGE('',*,*,#41304,.T.);
#52803=ORIENTED_EDGE('',*,*,#41305,.T.);
#52804=ORIENTED_EDGE('',*,*,#41306,.F.);
#52805=ORIENTED_EDGE('',*,*,#41307,.T.);
#52806=ORIENTED_EDGE('',*,*,#41304,.F.);
#52807=ORIENTED_EDGE('',*,*,#41308,.T.);
#52808=ORIENTED_EDGE('',*,*,#41309,.F.);
#52809=ORIENTED_EDGE('',*,*,#41310,.F.);
#52810=ORIENTED_EDGE('',*,*,#41311,.T.);
#52811=ORIENTED_EDGE('',*,*,#41312,.T.);
#52812=ORIENTED_EDGE('',*,*,#41311,.F.);
#52813=ORIENTED_EDGE('',*,*,#41313,.F.);
#52814=ORIENTED_EDGE('',*,*,#41314,.F.);
#52815=ORIENTED_EDGE('',*,*,#41315,.F.);
#52816=ORIENTED_EDGE('',*,*,#41316,.T.);
#52817=ORIENTED_EDGE('',*,*,#41317,.T.);
#52818=ORIENTED_EDGE('',*,*,#41318,.T.);
#52819=ORIENTED_EDGE('',*,*,#41316,.F.);
#52820=ORIENTED_EDGE('',*,*,#41318,.F.);
#52821=ORIENTED_EDGE('',*,*,#41319,.T.);
#52822=ORIENTED_EDGE('',*,*,#41320,.T.);
#52823=ORIENTED_EDGE('',*,*,#41319,.F.);
#52824=ORIENTED_EDGE('',*,*,#41317,.F.);
#52825=ORIENTED_EDGE('',*,*,#41321,.F.);
#52826=ORIENTED_EDGE('',*,*,#41322,.T.);
#52827=ORIENTED_EDGE('',*,*,#41323,.T.);
#52828=ORIENTED_EDGE('',*,*,#41322,.F.);
#52829=ORIENTED_EDGE('',*,*,#41324,.F.);
#52830=ORIENTED_EDGE('',*,*,#41325,.T.);
#52831=ORIENTED_EDGE('',*,*,#41326,.F.);
#52832=ORIENTED_EDGE('',*,*,#41327,.F.);
#52833=ORIENTED_EDGE('',*,*,#41328,.F.);
#52834=ORIENTED_EDGE('',*,*,#41329,.F.);
#52835=ORIENTED_EDGE('',*,*,#41330,.F.);
#52836=ORIENTED_EDGE('',*,*,#41331,.F.);
#52837=ORIENTED_EDGE('',*,*,#41325,.F.);
#52838=ORIENTED_EDGE('',*,*,#41332,.F.);
#52839=ORIENTED_EDGE('',*,*,#41333,.F.);
#52840=ORIENTED_EDGE('',*,*,#41334,.T.);
#52841=ORIENTED_EDGE('',*,*,#41335,.T.);
#52842=ORIENTED_EDGE('',*,*,#41334,.F.);
#52843=ORIENTED_EDGE('',*,*,#41336,.F.);
#52844=ORIENTED_EDGE('',*,*,#41337,.T.);
#52845=ORIENTED_EDGE('',*,*,#41332,.T.);
#52846=ORIENTED_EDGE('',*,*,#41333,.T.);
#52847=ORIENTED_EDGE('',*,*,#41337,.F.);
#52848=ORIENTED_EDGE('',*,*,#41338,.F.);
#52849=ORIENTED_EDGE('',*,*,#41339,.T.);
#52850=ORIENTED_EDGE('',*,*,#41340,.T.);
#52851=ORIENTED_EDGE('',*,*,#41339,.F.);
#52852=ORIENTED_EDGE('',*,*,#41341,.F.);
#52853=ORIENTED_EDGE('',*,*,#41342,.F.);
#52854=ORIENTED_EDGE('',*,*,#41343,.F.);
#52855=ORIENTED_EDGE('',*,*,#41344,.T.);
#52856=ORIENTED_EDGE('',*,*,#41341,.T.);
#52857=ORIENTED_EDGE('',*,*,#41338,.T.);
#52858=ORIENTED_EDGE('',*,*,#41344,.F.);
#52859=ORIENTED_EDGE('',*,*,#41345,.T.);
#52860=ORIENTED_EDGE('',*,*,#41346,.T.);
#52861=ORIENTED_EDGE('',*,*,#41347,.F.);
#52862=ORIENTED_EDGE('',*,*,#41348,.T.);
#52863=ORIENTED_EDGE('',*,*,#41349,.T.);
#52864=ORIENTED_EDGE('',*,*,#41350,.T.);
#52865=ORIENTED_EDGE('',*,*,#41351,.T.);
#52866=ORIENTED_EDGE('',*,*,#41352,.T.);
#52867=ORIENTED_EDGE('',*,*,#41188,.T.);
#52868=ORIENTED_EDGE('',*,*,#41353,.T.);
#52869=ORIENTED_EDGE('',*,*,#41185,.F.);
#52870=ORIENTED_EDGE('',*,*,#41354,.T.);
#52871=ORIENTED_EDGE('',*,*,#41355,.T.);
#52872=ORIENTED_EDGE('',*,*,#41356,.T.);
#52873=ORIENTED_EDGE('',*,*,#41357,.T.);
#52874=ORIENTED_EDGE('',*,*,#41356,.F.);
#52875=ORIENTED_EDGE('',*,*,#41358,.T.);
#52876=ORIENTED_EDGE('',*,*,#41355,.F.);
#52877=ORIENTED_EDGE('',*,*,#41359,.T.);
#52878=ORIENTED_EDGE('',*,*,#41182,.F.);
#52879=ORIENTED_EDGE('',*,*,#41183,.F.);
#52880=ORIENTED_EDGE('',*,*,#41359,.F.);
#52881=ORIENTED_EDGE('',*,*,#41358,.F.);
#52882=ORIENTED_EDGE('',*,*,#41360,.F.);
#52883=ORIENTED_EDGE('',*,*,#41361,.F.);
#52884=ORIENTED_EDGE('',*,*,#41362,.T.);
#52885=ORIENTED_EDGE('',*,*,#41363,.F.);
#52886=ORIENTED_EDGE('',*,*,#41362,.F.);
#52887=ORIENTED_EDGE('',*,*,#41364,.F.);
#52888=ORIENTED_EDGE('',*,*,#41190,.F.);
#52889=ORIENTED_EDGE('',*,*,#41365,.F.);
#52890=ORIENTED_EDGE('',*,*,#41175,.F.);
#52891=ORIENTED_EDGE('',*,*,#41174,.T.);
#52892=ORIENTED_EDGE('',*,*,#41366,.T.);
#52893=ORIENTED_EDGE('',*,*,#41171,.F.);
#52894=ORIENTED_EDGE('',*,*,#41367,.T.);
#52895=ORIENTED_EDGE('',*,*,#41360,.T.);
#52896=ORIENTED_EDGE('',*,*,#41368,.F.);
#52897=ORIENTED_EDGE('',*,*,#41369,.T.);
#52898=ORIENTED_EDGE('',*,*,#41370,.T.);
#52899=ORIENTED_EDGE('',*,*,#41371,.T.);
#52900=ORIENTED_EDGE('',*,*,#41369,.F.);
#52901=ORIENTED_EDGE('',*,*,#41370,.F.);
#52902=ORIENTED_EDGE('',*,*,#41371,.F.);
#52903=ORIENTED_EDGE('',*,*,#41372,.T.);
#52904=ORIENTED_EDGE('',*,*,#41373,.F.);
#52905=ORIENTED_EDGE('',*,*,#41372,.F.);
#52906=ORIENTED_EDGE('',*,*,#41374,.F.);
#52907=ORIENTED_EDGE('',*,*,#41375,.F.);
#52908=ORIENTED_EDGE('',*,*,#41159,.F.);
#52909=ORIENTED_EDGE('',*,*,#41376,.F.);
#52910=ORIENTED_EDGE('',*,*,#41377,.F.);
#52911=ORIENTED_EDGE('',*,*,#41378,.F.);
#52912=ORIENTED_EDGE('',*,*,#41157,.T.);
#52913=ORIENTED_EDGE('',*,*,#41379,.F.);
#52914=ORIENTED_EDGE('',*,*,#41380,.T.);
#52915=ORIENTED_EDGE('',*,*,#41381,.T.);
#52916=ORIENTED_EDGE('',*,*,#41153,.F.);
#52917=ORIENTED_EDGE('',*,*,#41382,.T.);
#52918=ORIENTED_EDGE('',*,*,#41383,.T.);
#52919=ORIENTED_EDGE('',*,*,#41384,.T.);
#52920=ORIENTED_EDGE('',*,*,#41385,.T.);
#52921=ORIENTED_EDGE('',*,*,#41386,.T.);
#52922=ORIENTED_EDGE('',*,*,#41387,.T.);
#52923=ORIENTED_EDGE('',*,*,#41388,.T.);
#52924=ORIENTED_EDGE('',*,*,#41389,.T.);
#52925=ORIENTED_EDGE('',*,*,#41390,.T.);
#52926=ORIENTED_EDGE('',*,*,#41389,.F.);
#52927=ORIENTED_EDGE('',*,*,#41391,.T.);
#52928=ORIENTED_EDGE('',*,*,#41392,.T.);
#52929=ORIENTED_EDGE('',*,*,#41393,.T.);
#52930=ORIENTED_EDGE('',*,*,#41394,.F.);
#52931=ORIENTED_EDGE('',*,*,#41395,.T.);
#52932=ORIENTED_EDGE('',*,*,#41396,.F.);
#52933=ORIENTED_EDGE('',*,*,#41397,.T.);
#52934=ORIENTED_EDGE('',*,*,#41398,.T.);
#52935=ORIENTED_EDGE('',*,*,#41399,.T.);
#52936=ORIENTED_EDGE('',*,*,#41400,.T.);
#52937=ORIENTED_EDGE('',*,*,#41401,.T.);
#52938=ORIENTED_EDGE('',*,*,#41402,.F.);
#52939=ORIENTED_EDGE('',*,*,#41403,.F.);
#52940=ORIENTED_EDGE('',*,*,#41404,.F.);
#52941=ORIENTED_EDGE('',*,*,#41405,.T.);
#52942=ORIENTED_EDGE('',*,*,#41406,.F.);
#52943=ORIENTED_EDGE('',*,*,#41407,.T.);
#52944=ORIENTED_EDGE('',*,*,#41408,.F.);
#52945=ORIENTED_EDGE('',*,*,#41407,.F.);
#52946=ORIENTED_EDGE('',*,*,#41409,.T.);
#52947=ORIENTED_EDGE('',*,*,#41410,.T.);
#52948=ORIENTED_EDGE('',*,*,#41411,.T.);
#52949=ORIENTED_EDGE('',*,*,#41410,.F.);
#52950=ORIENTED_EDGE('',*,*,#41412,.T.);
#52951=ORIENTED_EDGE('',*,*,#41409,.F.);
#52952=ORIENTED_EDGE('',*,*,#41413,.T.);
#52953=ORIENTED_EDGE('',*,*,#41414,.F.);
#52954=ORIENTED_EDGE('',*,*,#41413,.F.);
#52955=ORIENTED_EDGE('',*,*,#41412,.F.);
#52956=ORIENTED_EDGE('',*,*,#41415,.T.);
#52957=ORIENTED_EDGE('',*,*,#41416,.T.);
#52958=ORIENTED_EDGE('',*,*,#41417,.F.);
#52959=ORIENTED_EDGE('',*,*,#41418,.F.);
#52960=ORIENTED_EDGE('',*,*,#41416,.F.);
#52961=ORIENTED_EDGE('',*,*,#41419,.T.);
#52962=ORIENTED_EDGE('',*,*,#41420,.F.);
#52963=ORIENTED_EDGE('',*,*,#41421,.F.);
#52964=ORIENTED_EDGE('',*,*,#41422,.F.);
#52965=ORIENTED_EDGE('',*,*,#41423,.F.);
#52966=ORIENTED_EDGE('',*,*,#41424,.T.);
#52967=ORIENTED_EDGE('',*,*,#41417,.T.);
#52968=ORIENTED_EDGE('',*,*,#41418,.T.);
#52969=ORIENTED_EDGE('',*,*,#41424,.F.);
#52970=ORIENTED_EDGE('',*,*,#41425,.F.);
#52971=ORIENTED_EDGE('',*,*,#41426,.F.);
#52972=ORIENTED_EDGE('',*,*,#41427,.F.);
#52973=ORIENTED_EDGE('',*,*,#41415,.F.);
#52974=ORIENTED_EDGE('',*,*,#41428,.T.);
#52975=ORIENTED_EDGE('',*,*,#41429,.F.);
#52976=ORIENTED_EDGE('',*,*,#41428,.F.);
#52977=ORIENTED_EDGE('',*,*,#41419,.F.);
#52978=ORIENTED_EDGE('',*,*,#41430,.T.);
#52979=ORIENTED_EDGE('',*,*,#41431,.T.);
#52980=ORIENTED_EDGE('',*,*,#41432,.T.);
#52981=ORIENTED_EDGE('',*,*,#41433,.T.);
#52982=ORIENTED_EDGE('',*,*,#41432,.F.);
#52983=ORIENTED_EDGE('',*,*,#41434,.F.);
#52984=ORIENTED_EDGE('',*,*,#41435,.T.);
#52985=ORIENTED_EDGE('',*,*,#41430,.F.);
#52986=ORIENTED_EDGE('',*,*,#41431,.F.);
#52987=ORIENTED_EDGE('',*,*,#41435,.F.);
#52988=ORIENTED_EDGE('',*,*,#41137,.F.);
#52989=ORIENTED_EDGE('',*,*,#41436,.F.);
#52990=ORIENTED_EDGE('',*,*,#41437,.F.);
#52991=ORIENTED_EDGE('',*,*,#41438,.F.);
#52992=ORIENTED_EDGE('',*,*,#41439,.F.);
#52993=ORIENTED_EDGE('',*,*,#41440,.F.);
#52994=ORIENTED_EDGE('',*,*,#41144,.T.);
#52995=ORIENTED_EDGE('',*,*,#41441,.T.);
#52996=ORIENTED_EDGE('',*,*,#41442,.F.);
#52997=ORIENTED_EDGE('',*,*,#41443,.F.);
#52998=ORIENTED_EDGE('',*,*,#41444,.T.);
#52999=ORIENTED_EDGE('',*,*,#41445,.T.);
#53000=ORIENTED_EDGE('',*,*,#41446,.T.);
#53001=ORIENTED_EDGE('',*,*,#41447,.T.);
#53002=ORIENTED_EDGE('',*,*,#41448,.T.);
#53003=ORIENTED_EDGE('',*,*,#41449,.T.);
#53004=ORIENTED_EDGE('',*,*,#41450,.T.);
#53005=ORIENTED_EDGE('',*,*,#41449,.F.);
#53006=ORIENTED_EDGE('',*,*,#41451,.T.);
#53007=ORIENTED_EDGE('',*,*,#41452,.T.);
#53008=ORIENTED_EDGE('',*,*,#41453,.T.);
#53009=ORIENTED_EDGE('',*,*,#41454,.T.);
#53010=ORIENTED_EDGE('',*,*,#41455,.T.);
#53011=ORIENTED_EDGE('',*,*,#41456,.T.);
#53012=ORIENTED_EDGE('',*,*,#41457,.T.);
#53013=ORIENTED_EDGE('',*,*,#41458,.T.);
#53014=ORIENTED_EDGE('',*,*,#41459,.F.);
#53015=ORIENTED_EDGE('',*,*,#41460,.T.);
#53016=ORIENTED_EDGE('',*,*,#41461,.F.);
#53017=ORIENTED_EDGE('',*,*,#41462,.T.);
#53018=ORIENTED_EDGE('',*,*,#41463,.F.);
#53019=ORIENTED_EDGE('',*,*,#41464,.F.);
#53020=ORIENTED_EDGE('',*,*,#41465,.F.);
#53021=ORIENTED_EDGE('',*,*,#41466,.T.);
#53022=ORIENTED_EDGE('',*,*,#41467,.T.);
#53023=ORIENTED_EDGE('',*,*,#41468,.F.);
#53024=ORIENTED_EDGE('',*,*,#41469,.T.);
#53025=ORIENTED_EDGE('',*,*,#41470,.F.);
#53026=ORIENTED_EDGE('',*,*,#41469,.F.);
#53027=ORIENTED_EDGE('',*,*,#41471,.T.);
#53028=ORIENTED_EDGE('',*,*,#41472,.T.);
#53029=ORIENTED_EDGE('',*,*,#41473,.T.);
#53030=ORIENTED_EDGE('',*,*,#41472,.F.);
#53031=ORIENTED_EDGE('',*,*,#41474,.T.);
#53032=ORIENTED_EDGE('',*,*,#41471,.F.);
#53033=ORIENTED_EDGE('',*,*,#41475,.T.);
#53034=ORIENTED_EDGE('',*,*,#41476,.F.);
#53035=ORIENTED_EDGE('',*,*,#41475,.F.);
#53036=ORIENTED_EDGE('',*,*,#41474,.F.);
#53037=ORIENTED_EDGE('',*,*,#41477,.T.);
#53038=ORIENTED_EDGE('',*,*,#41478,.T.);
#53039=ORIENTED_EDGE('',*,*,#41479,.F.);
#53040=ORIENTED_EDGE('',*,*,#41480,.F.);
#53041=ORIENTED_EDGE('',*,*,#41478,.F.);
#53042=ORIENTED_EDGE('',*,*,#41481,.T.);
#53043=ORIENTED_EDGE('',*,*,#41482,.F.);
#53044=ORIENTED_EDGE('',*,*,#41483,.F.);
#53045=ORIENTED_EDGE('',*,*,#41484,.F.);
#53046=ORIENTED_EDGE('',*,*,#41485,.F.);
#53047=ORIENTED_EDGE('',*,*,#41486,.T.);
#53048=ORIENTED_EDGE('',*,*,#41479,.T.);
#53049=ORIENTED_EDGE('',*,*,#41480,.T.);
#53050=ORIENTED_EDGE('',*,*,#41486,.F.);
#53051=ORIENTED_EDGE('',*,*,#41487,.F.);
#53052=ORIENTED_EDGE('',*,*,#41488,.F.);
#53053=ORIENTED_EDGE('',*,*,#41489,.F.);
#53054=ORIENTED_EDGE('',*,*,#41477,.F.);
#53055=ORIENTED_EDGE('',*,*,#41490,.T.);
#53056=ORIENTED_EDGE('',*,*,#41491,.F.);
#53057=ORIENTED_EDGE('',*,*,#41490,.F.);
#53058=ORIENTED_EDGE('',*,*,#41481,.F.);
#53059=ORIENTED_EDGE('',*,*,#41433,.F.);
#53060=ORIENTED_EDGE('',*,*,#41492,.T.);
#53061=ORIENTED_EDGE('',*,*,#41493,.T.);
#53062=ORIENTED_EDGE('',*,*,#41494,.T.);
#53063=ORIENTED_EDGE('',*,*,#41495,.T.);
#53064=ORIENTED_EDGE('',*,*,#41496,.T.);
#53065=ORIENTED_EDGE('',*,*,#41497,.T.);
#53066=ORIENTED_EDGE('',*,*,#41492,.F.);
#53067=ORIENTED_EDGE('',*,*,#41498,.T.);
#53068=ORIENTED_EDGE('',*,*,#41483,.T.);
#53069=ORIENTED_EDGE('',*,*,#41499,.F.);
#53070=ORIENTED_EDGE('',*,*,#41493,.F.);
#53071=ORIENTED_EDGE('',*,*,#41499,.T.);
#53072=ORIENTED_EDGE('',*,*,#41482,.T.);
#53073=ORIENTED_EDGE('',*,*,#41500,.F.);
#53074=ORIENTED_EDGE('',*,*,#41494,.F.);
#53075=ORIENTED_EDGE('',*,*,#41500,.T.);
#53076=ORIENTED_EDGE('',*,*,#41489,.T.);
#53077=ORIENTED_EDGE('',*,*,#41501,.F.);
#53078=ORIENTED_EDGE('',*,*,#41495,.F.);
#53079=ORIENTED_EDGE('',*,*,#41501,.T.);
#53080=ORIENTED_EDGE('',*,*,#41488,.T.);
#53081=ORIENTED_EDGE('',*,*,#41502,.F.);
#53082=ORIENTED_EDGE('',*,*,#41496,.F.);
#53083=ORIENTED_EDGE('',*,*,#41502,.T.);
#53084=ORIENTED_EDGE('',*,*,#41487,.T.);
#53085=ORIENTED_EDGE('',*,*,#41485,.T.);
#53086=ORIENTED_EDGE('',*,*,#41503,.F.);
#53087=ORIENTED_EDGE('',*,*,#41497,.F.);
#53088=ORIENTED_EDGE('',*,*,#41503,.T.);
#53089=ORIENTED_EDGE('',*,*,#41484,.T.);
#53090=ORIENTED_EDGE('',*,*,#41498,.F.);
#53091=ORIENTED_EDGE('',*,*,#41473,.F.);
#53092=ORIENTED_EDGE('',*,*,#41468,.T.);
#53093=ORIENTED_EDGE('',*,*,#41476,.T.);
#53094=ORIENTED_EDGE('',*,*,#41491,.T.);
#53095=ORIENTED_EDGE('',*,*,#41504,.F.);
#53096=ORIENTED_EDGE('',*,*,#41505,.T.);
#53097=ORIENTED_EDGE('',*,*,#41506,.T.);
#53098=ORIENTED_EDGE('',*,*,#41507,.T.);
#53099=ORIENTED_EDGE('',*,*,#41508,.F.);
#53100=ORIENTED_EDGE('',*,*,#41509,.T.);
#53101=ORIENTED_EDGE('',*,*,#41510,.T.);
#53102=ORIENTED_EDGE('',*,*,#41511,.F.);
#53103=ORIENTED_EDGE('',*,*,#41512,.T.);
#53104=ORIENTED_EDGE('',*,*,#41513,.T.);
#53105=ORIENTED_EDGE('',*,*,#41464,.T.);
#53106=ORIENTED_EDGE('',*,*,#41463,.T.);
#53107=ORIENTED_EDGE('',*,*,#41506,.F.);
#53108=ORIENTED_EDGE('',*,*,#41514,.T.);
#53109=ORIENTED_EDGE('',*,*,#41515,.T.);
#53110=ORIENTED_EDGE('',*,*,#41516,.F.);
#53111=ORIENTED_EDGE('',*,*,#41517,.T.);
#53112=ORIENTED_EDGE('',*,*,#41507,.F.);
#53113=ORIENTED_EDGE('',*,*,#41518,.T.);
#53114=ORIENTED_EDGE('',*,*,#41519,.F.);
#53115=ORIENTED_EDGE('',*,*,#41504,.T.);
#53116=ORIENTED_EDGE('',*,*,#41520,.T.);
#53117=ORIENTED_EDGE('',*,*,#41521,.T.);
#53118=ORIENTED_EDGE('',*,*,#41522,.T.);
#53119=ORIENTED_EDGE('',*,*,#41523,.F.);
#53120=ORIENTED_EDGE('',*,*,#41524,.F.);
#53121=ORIENTED_EDGE('',*,*,#41525,.T.);
#53122=ORIENTED_EDGE('',*,*,#41525,.F.);
#53123=ORIENTED_EDGE('',*,*,#41526,.F.);
#53124=ORIENTED_EDGE('',*,*,#41527,.T.);
#53125=ORIENTED_EDGE('',*,*,#41521,.F.);
#53126=ORIENTED_EDGE('',*,*,#41528,.T.);
#53127=ORIENTED_EDGE('',*,*,#41529,.T.);
#53128=ORIENTED_EDGE('',*,*,#41522,.F.);
#53129=ORIENTED_EDGE('',*,*,#41527,.F.);
#53130=ORIENTED_EDGE('',*,*,#41530,.T.);
#53131=ORIENTED_EDGE('',*,*,#41531,.T.);
#53132=ORIENTED_EDGE('',*,*,#41514,.F.);
#53133=ORIENTED_EDGE('',*,*,#41505,.F.);
#53134=ORIENTED_EDGE('',*,*,#41519,.T.);
#53135=ORIENTED_EDGE('',*,*,#41529,.F.);
#53136=ORIENTED_EDGE('',*,*,#41532,.T.);
#53137=ORIENTED_EDGE('',*,*,#41533,.T.);
#53138=ORIENTED_EDGE('',*,*,#41534,.T.);
#53139=ORIENTED_EDGE('',*,*,#41509,.F.);
#53140=ORIENTED_EDGE('',*,*,#41535,.F.);
#53141=ORIENTED_EDGE('',*,*,#41536,.F.);
#53142=ORIENTED_EDGE('',*,*,#41537,.F.);
#53143=ORIENTED_EDGE('',*,*,#41538,.F.);
#53144=ORIENTED_EDGE('',*,*,#41539,.T.);
#53145=ORIENTED_EDGE('',*,*,#41540,.F.);
#53146=ORIENTED_EDGE('',*,*,#41536,.T.);
#53147=ORIENTED_EDGE('',*,*,#41541,.F.);
#53148=ORIENTED_EDGE('',*,*,#41542,.T.);
#53149=ORIENTED_EDGE('',*,*,#41543,.F.);
#53150=ORIENTED_EDGE('',*,*,#41512,.F.);
#53151=ORIENTED_EDGE('',*,*,#41544,.F.);
#53152=ORIENTED_EDGE('',*,*,#41530,.F.);
#53153=ORIENTED_EDGE('',*,*,#41542,.F.);
#53154=ORIENTED_EDGE('',*,*,#41545,.F.);
#53155=ORIENTED_EDGE('',*,*,#41508,.T.);
#53156=ORIENTED_EDGE('',*,*,#41546,.T.);
#53157=ORIENTED_EDGE('',*,*,#41547,.T.);
#53158=ORIENTED_EDGE('',*,*,#41548,.T.);
#53159=ORIENTED_EDGE('',*,*,#41533,.F.);
#53160=ORIENTED_EDGE('',*,*,#41549,.F.);
#53161=ORIENTED_EDGE('',*,*,#41534,.F.);
#53162=ORIENTED_EDGE('',*,*,#41550,.F.);
#53163=ORIENTED_EDGE('',*,*,#41551,.F.);
#53164=ORIENTED_EDGE('',*,*,#41552,.F.);
#53165=ORIENTED_EDGE('',*,*,#41510,.F.);
#53166=ORIENTED_EDGE('',*,*,#41551,.T.);
#53167=ORIENTED_EDGE('',*,*,#41553,.F.);
#53168=ORIENTED_EDGE('',*,*,#41554,.F.);
#53169=ORIENTED_EDGE('',*,*,#41555,.T.);
#53170=ORIENTED_EDGE('',*,*,#41513,.F.);
#53171=ORIENTED_EDGE('',*,*,#41543,.T.);
#53172=ORIENTED_EDGE('',*,*,#41546,.F.);
#53173=ORIENTED_EDGE('',*,*,#41552,.T.);
#53174=ORIENTED_EDGE('',*,*,#41556,.T.);
#53175=ORIENTED_EDGE('',*,*,#41557,.T.);
#53176=ORIENTED_EDGE('',*,*,#41558,.T.);
#53177=ORIENTED_EDGE('',*,*,#41559,.F.);
#53178=ORIENTED_EDGE('',*,*,#41560,.F.);
#53179=ORIENTED_EDGE('',*,*,#41561,.T.);
#53180=ORIENTED_EDGE('',*,*,#41562,.T.);
#53181=ORIENTED_EDGE('',*,*,#41466,.F.);
#53182=ORIENTED_EDGE('',*,*,#41558,.F.);
#53183=ORIENTED_EDGE('',*,*,#41563,.T.);
#53184=ORIENTED_EDGE('',*,*,#41564,.T.);
#53185=ORIENTED_EDGE('',*,*,#41565,.F.);
#53186=ORIENTED_EDGE('',*,*,#41562,.F.);
#53187=ORIENTED_EDGE('',*,*,#41566,.T.);
#53188=ORIENTED_EDGE('',*,*,#41531,.F.);
#53189=ORIENTED_EDGE('',*,*,#41544,.T.);
#53190=ORIENTED_EDGE('',*,*,#41511,.T.);
#53191=ORIENTED_EDGE('',*,*,#41567,.T.);
#53192=ORIENTED_EDGE('',*,*,#41568,.F.);
#53193=ORIENTED_EDGE('',*,*,#41515,.F.);
#53194=ORIENTED_EDGE('',*,*,#41568,.T.);
#53195=ORIENTED_EDGE('',*,*,#41569,.T.);
#53196=ORIENTED_EDGE('',*,*,#41570,.F.);
#53197=ORIENTED_EDGE('',*,*,#41571,.F.);
#53198=ORIENTED_EDGE('',*,*,#41516,.T.);
#53199=ORIENTED_EDGE('',*,*,#41571,.T.);
#53200=ORIENTED_EDGE('',*,*,#41572,.T.);
#53201=ORIENTED_EDGE('',*,*,#41573,.F.);
#53202=ORIENTED_EDGE('',*,*,#41518,.F.);
#53203=ORIENTED_EDGE('',*,*,#41523,.T.);
#53204=ORIENTED_EDGE('',*,*,#41520,.F.);
#53205=ORIENTED_EDGE('',*,*,#41517,.F.);
#53206=ORIENTED_EDGE('',*,*,#41574,.T.);
#53207=ORIENTED_EDGE('',*,*,#41526,.T.);
#53208=ORIENTED_EDGE('',*,*,#41524,.T.);
#53209=ORIENTED_EDGE('',*,*,#41575,.T.);
#53210=ORIENTED_EDGE('',*,*,#41576,.T.);
#53211=ORIENTED_EDGE('',*,*,#41577,.F.);
#53212=ORIENTED_EDGE('',*,*,#41537,.T.);
#53213=ORIENTED_EDGE('',*,*,#41540,.T.);
#53214=ORIENTED_EDGE('',*,*,#41532,.F.);
#53215=ORIENTED_EDGE('',*,*,#41528,.F.);
#53216=ORIENTED_EDGE('',*,*,#41577,.T.);
#53217=ORIENTED_EDGE('',*,*,#41578,.T.);
#53218=ORIENTED_EDGE('',*,*,#41579,.T.);
#53219=ORIENTED_EDGE('',*,*,#41538,.T.);
#53220=ORIENTED_EDGE('',*,*,#41580,.F.);
#53221=ORIENTED_EDGE('',*,*,#41581,.T.);
#53222=ORIENTED_EDGE('',*,*,#41545,.T.);
#53223=ORIENTED_EDGE('',*,*,#41541,.T.);
#53224=ORIENTED_EDGE('',*,*,#41539,.F.);
#53225=ORIENTED_EDGE('',*,*,#41582,.F.);
#53226=ORIENTED_EDGE('',*,*,#41583,.T.);
#53227=ORIENTED_EDGE('',*,*,#41549,.T.);
#53228=ORIENTED_EDGE('',*,*,#41535,.T.);
#53229=ORIENTED_EDGE('',*,*,#41584,.T.);
#53230=ORIENTED_EDGE('',*,*,#41585,.T.);
#53231=ORIENTED_EDGE('',*,*,#41547,.F.);
#53232=ORIENTED_EDGE('',*,*,#41583,.F.);
#53233=ORIENTED_EDGE('',*,*,#41586,.T.);
#53234=ORIENTED_EDGE('',*,*,#41587,.T.);
#53235=ORIENTED_EDGE('',*,*,#41553,.T.);
#53236=ORIENTED_EDGE('',*,*,#41550,.T.);
#53237=ORIENTED_EDGE('',*,*,#41548,.F.);
#53238=ORIENTED_EDGE('',*,*,#41588,.T.);
#53239=ORIENTED_EDGE('',*,*,#41584,.F.);
#53240=ORIENTED_EDGE('',*,*,#41589,.F.);
#53241=ORIENTED_EDGE('',*,*,#41554,.T.);
#53242=ORIENTED_EDGE('',*,*,#41587,.F.);
#53243=ORIENTED_EDGE('',*,*,#41590,.F.);
#53244=ORIENTED_EDGE('',*,*,#41591,.T.);
#53245=ORIENTED_EDGE('',*,*,#41592,.T.);
#53246=ORIENTED_EDGE('',*,*,#41556,.F.);
#53247=ORIENTED_EDGE('',*,*,#41555,.F.);
#53248=ORIENTED_EDGE('',*,*,#41465,.T.);
#53249=ORIENTED_EDGE('',*,*,#41557,.F.);
#53250=ORIENTED_EDGE('',*,*,#41593,.F.);
#53251=ORIENTED_EDGE('',*,*,#41559,.T.);
#53252=ORIENTED_EDGE('',*,*,#41560,.T.);
#53253=ORIENTED_EDGE('',*,*,#41594,.F.);
#53254=ORIENTED_EDGE('',*,*,#41595,.F.);
#53255=ORIENTED_EDGE('',*,*,#41596,.T.);
#53256=ORIENTED_EDGE('',*,*,#41596,.F.);
#53257=ORIENTED_EDGE('',*,*,#41597,.F.);
#53258=ORIENTED_EDGE('',*,*,#41598,.F.);
#53259=ORIENTED_EDGE('',*,*,#41566,.F.);
#53260=ORIENTED_EDGE('',*,*,#41563,.F.);
#53261=ORIENTED_EDGE('',*,*,#41561,.F.);
#53262=ORIENTED_EDGE('',*,*,#41599,.T.);
#53263=ORIENTED_EDGE('',*,*,#41600,.F.);
#53264=ORIENTED_EDGE('',*,*,#41564,.F.);
#53265=ORIENTED_EDGE('',*,*,#41598,.T.);
#53266=ORIENTED_EDGE('',*,*,#41601,.F.);
#53267=ORIENTED_EDGE('',*,*,#41569,.F.);
#53268=ORIENTED_EDGE('',*,*,#41567,.F.);
#53269=ORIENTED_EDGE('',*,*,#41467,.F.);
#53270=ORIENTED_EDGE('',*,*,#41565,.T.);
#53271=ORIENTED_EDGE('',*,*,#41572,.F.);
#53272=ORIENTED_EDGE('',*,*,#41570,.T.);
#53273=ORIENTED_EDGE('',*,*,#41602,.T.);
#53274=ORIENTED_EDGE('',*,*,#41574,.F.);
#53275=ORIENTED_EDGE('',*,*,#41573,.T.);
#53276=ORIENTED_EDGE('',*,*,#41603,.F.);
#53277=ORIENTED_EDGE('',*,*,#41575,.F.);
#53278=ORIENTED_EDGE('',*,*,#41604,.T.);
#53279=ORIENTED_EDGE('',*,*,#41578,.F.);
#53280=ORIENTED_EDGE('',*,*,#41576,.F.);
#53281=ORIENTED_EDGE('',*,*,#41605,.T.);
#53282=ORIENTED_EDGE('',*,*,#41580,.T.);
#53283=ORIENTED_EDGE('',*,*,#41579,.F.);
#53284=ORIENTED_EDGE('',*,*,#41604,.F.);
#53285=ORIENTED_EDGE('',*,*,#41461,.T.);
#53286=ORIENTED_EDGE('',*,*,#41582,.T.);
#53287=ORIENTED_EDGE('',*,*,#41581,.F.);
#53288=ORIENTED_EDGE('',*,*,#41460,.F.);
#53289=ORIENTED_EDGE('',*,*,#41589,.T.);
#53290=ORIENTED_EDGE('',*,*,#41588,.F.);
#53291=ORIENTED_EDGE('',*,*,#41459,.T.);
#53292=ORIENTED_EDGE('',*,*,#41590,.T.);
#53293=ORIENTED_EDGE('',*,*,#41586,.F.);
#53294=ORIENTED_EDGE('',*,*,#41585,.F.);
#53295=ORIENTED_EDGE('',*,*,#41594,.T.);
#53296=ORIENTED_EDGE('',*,*,#41593,.T.);
#53297=ORIENTED_EDGE('',*,*,#41592,.F.);
#53298=ORIENTED_EDGE('',*,*,#41591,.F.);
#53299=ORIENTED_EDGE('',*,*,#41458,.F.);
#53300=ORIENTED_EDGE('',*,*,#41606,.T.);
#53301=ORIENTED_EDGE('',*,*,#41607,.F.);
#53302=ORIENTED_EDGE('',*,*,#41607,.T.);
#53303=ORIENTED_EDGE('',*,*,#41608,.T.);
#53304=ORIENTED_EDGE('',*,*,#41609,.T.);
#53305=ORIENTED_EDGE('',*,*,#41599,.F.);
#53306=ORIENTED_EDGE('',*,*,#41597,.T.);
#53307=ORIENTED_EDGE('',*,*,#41595,.T.);
#53308=ORIENTED_EDGE('',*,*,#41609,.F.);
#53309=ORIENTED_EDGE('',*,*,#41610,.T.);
#53310=ORIENTED_EDGE('',*,*,#41611,.F.);
#53311=ORIENTED_EDGE('',*,*,#41612,.T.);
#53312=ORIENTED_EDGE('',*,*,#41613,.T.);
#53313=ORIENTED_EDGE('',*,*,#41611,.T.);
#53314=ORIENTED_EDGE('',*,*,#41605,.F.);
#53315=ORIENTED_EDGE('',*,*,#41603,.T.);
#53316=ORIENTED_EDGE('',*,*,#41602,.F.);
#53317=ORIENTED_EDGE('',*,*,#41601,.T.);
#53318=ORIENTED_EDGE('',*,*,#41600,.T.);
#53319=ORIENTED_EDGE('',*,*,#41613,.F.);
#53320=ORIENTED_EDGE('',*,*,#41614,.T.);
#53321=ORIENTED_EDGE('',*,*,#41615,.T.);
#53322=ORIENTED_EDGE('',*,*,#41462,.F.);
#53323=ORIENTED_EDGE('',*,*,#41616,.F.);
#53324=ORIENTED_EDGE('',*,*,#41606,.F.);
#53325=ORIENTED_EDGE('',*,*,#41617,.T.);
#53326=ORIENTED_EDGE('',*,*,#41618,.F.);
#53327=ORIENTED_EDGE('',*,*,#41619,.F.);
#53328=ORIENTED_EDGE('',*,*,#41620,.F.);
#53329=ORIENTED_EDGE('',*,*,#41608,.F.);
#53330=ORIENTED_EDGE('',*,*,#41616,.T.);
#53331=ORIENTED_EDGE('',*,*,#41621,.F.);
#53332=ORIENTED_EDGE('',*,*,#41622,.F.);
#53333=ORIENTED_EDGE('',*,*,#41610,.F.);
#53334=ORIENTED_EDGE('',*,*,#41620,.T.);
#53335=ORIENTED_EDGE('',*,*,#41623,.F.);
#53336=ORIENTED_EDGE('',*,*,#41624,.F.);
#53337=ORIENTED_EDGE('',*,*,#41612,.F.);
#53338=ORIENTED_EDGE('',*,*,#41622,.T.);
#53339=ORIENTED_EDGE('',*,*,#41625,.F.);
#53340=ORIENTED_EDGE('',*,*,#41626,.F.);
#53341=ORIENTED_EDGE('',*,*,#41614,.F.);
#53342=ORIENTED_EDGE('',*,*,#41624,.T.);
#53343=ORIENTED_EDGE('',*,*,#41627,.F.);
#53344=ORIENTED_EDGE('',*,*,#41628,.F.);
#53345=ORIENTED_EDGE('',*,*,#41615,.F.);
#53346=ORIENTED_EDGE('',*,*,#41626,.T.);
#53347=ORIENTED_EDGE('',*,*,#41629,.F.);
#53348=ORIENTED_EDGE('',*,*,#41630,.F.);
#53349=ORIENTED_EDGE('',*,*,#41456,.F.);
#53350=ORIENTED_EDGE('',*,*,#41628,.T.);
#53351=ORIENTED_EDGE('',*,*,#41631,.F.);
#53352=ORIENTED_EDGE('',*,*,#41617,.F.);
#53353=ORIENTED_EDGE('',*,*,#41457,.F.);
#53354=ORIENTED_EDGE('',*,*,#41630,.T.);
#53355=ORIENTED_EDGE('',*,*,#41632,.F.);
#53356=ORIENTED_EDGE('',*,*,#41633,.T.);
#53357=ORIENTED_EDGE('',*,*,#41445,.F.);
#53358=ORIENTED_EDGE('',*,*,#41634,.F.);
#53359=ORIENTED_EDGE('',*,*,#41618,.T.);
#53360=ORIENTED_EDGE('',*,*,#41634,.T.);
#53361=ORIENTED_EDGE('',*,*,#41455,.F.);
#53362=ORIENTED_EDGE('',*,*,#41635,.F.);
#53363=ORIENTED_EDGE('',*,*,#41619,.T.);
#53364=ORIENTED_EDGE('',*,*,#41635,.T.);
#53365=ORIENTED_EDGE('',*,*,#41454,.F.);
#53366=ORIENTED_EDGE('',*,*,#41636,.F.);
#53367=ORIENTED_EDGE('',*,*,#41621,.T.);
#53368=ORIENTED_EDGE('',*,*,#41636,.T.);
#53369=ORIENTED_EDGE('',*,*,#41453,.F.);
#53370=ORIENTED_EDGE('',*,*,#41637,.F.);
#53371=ORIENTED_EDGE('',*,*,#41623,.T.);
#53372=ORIENTED_EDGE('',*,*,#41637,.T.);
#53373=ORIENTED_EDGE('',*,*,#41452,.F.);
#53374=ORIENTED_EDGE('',*,*,#41638,.F.);
#53375=ORIENTED_EDGE('',*,*,#41625,.T.);
#53376=ORIENTED_EDGE('',*,*,#41638,.T.);
#53377=ORIENTED_EDGE('',*,*,#41451,.F.);
#53378=ORIENTED_EDGE('',*,*,#41639,.F.);
#53379=ORIENTED_EDGE('',*,*,#41627,.T.);
#53380=ORIENTED_EDGE('',*,*,#41639,.T.);
#53381=ORIENTED_EDGE('',*,*,#41448,.F.);
#53382=ORIENTED_EDGE('',*,*,#41640,.F.);
#53383=ORIENTED_EDGE('',*,*,#41629,.T.);
#53384=ORIENTED_EDGE('',*,*,#41640,.T.);
#53385=ORIENTED_EDGE('',*,*,#41447,.F.);
#53386=ORIENTED_EDGE('',*,*,#41641,.F.);
#53387=ORIENTED_EDGE('',*,*,#41631,.T.);
#53388=ORIENTED_EDGE('',*,*,#41641,.T.);
#53389=ORIENTED_EDGE('',*,*,#41446,.F.);
#53390=ORIENTED_EDGE('',*,*,#41633,.F.);
#53391=ORIENTED_EDGE('',*,*,#41632,.T.);
#53392=ORIENTED_EDGE('',*,*,#41450,.F.);
#53393=ORIENTED_EDGE('',*,*,#41642,.T.);
#53394=ORIENTED_EDGE('',*,*,#41643,.T.);
#53395=ORIENTED_EDGE('',*,*,#41443,.T.);
#53396=ORIENTED_EDGE('',*,*,#41644,.T.);
#53397=ORIENTED_EDGE('',*,*,#41645,.T.);
#53398=ORIENTED_EDGE('',*,*,#41644,.F.);
#53399=ORIENTED_EDGE('',*,*,#41442,.T.);
#53400=ORIENTED_EDGE('',*,*,#41441,.F.);
#53401=ORIENTED_EDGE('',*,*,#41147,.F.);
#53402=ORIENTED_EDGE('',*,*,#41646,.T.);
#53403=ORIENTED_EDGE('',*,*,#41647,.T.);
#53404=ORIENTED_EDGE('',*,*,#41648,.T.);
#53405=ORIENTED_EDGE('',*,*,#41642,.F.);
#53406=ORIENTED_EDGE('',*,*,#41645,.F.);
#53407=ORIENTED_EDGE('',*,*,#41145,.F.);
#53408=ORIENTED_EDGE('',*,*,#41444,.F.);
#53409=ORIENTED_EDGE('',*,*,#41643,.F.);
#53410=ORIENTED_EDGE('',*,*,#41648,.F.);
#53411=ORIENTED_EDGE('',*,*,#41649,.T.);
#53412=ORIENTED_EDGE('',*,*,#41141,.F.);
#53413=ORIENTED_EDGE('',*,*,#41138,.F.);
#53414=ORIENTED_EDGE('',*,*,#41440,.T.);
#53415=ORIENTED_EDGE('',*,*,#41439,.T.);
#53416=ORIENTED_EDGE('',*,*,#41650,.F.);
#53417=ORIENTED_EDGE('',*,*,#41651,.T.);
#53418=ORIENTED_EDGE('',*,*,#41646,.F.);
#53419=ORIENTED_EDGE('',*,*,#41146,.F.);
#53420=ORIENTED_EDGE('',*,*,#41139,.F.);
#53421=ORIENTED_EDGE('',*,*,#41652,.F.);
#53422=ORIENTED_EDGE('',*,*,#41653,.T.);
#53423=ORIENTED_EDGE('',*,*,#41647,.F.);
#53424=ORIENTED_EDGE('',*,*,#41651,.F.);
#53425=ORIENTED_EDGE('',*,*,#41653,.F.);
#53426=ORIENTED_EDGE('',*,*,#41654,.F.);
#53427=ORIENTED_EDGE('',*,*,#41437,.T.);
#53428=ORIENTED_EDGE('',*,*,#41436,.T.);
#53429=ORIENTED_EDGE('',*,*,#41136,.F.);
#53430=ORIENTED_EDGE('',*,*,#41143,.F.);
#53431=ORIENTED_EDGE('',*,*,#41142,.F.);
#53432=ORIENTED_EDGE('',*,*,#41649,.F.);
#53433=ORIENTED_EDGE('',*,*,#41434,.T.);
#53434=ORIENTED_EDGE('',*,*,#41438,.T.);
#53435=ORIENTED_EDGE('',*,*,#41654,.T.);
#53436=ORIENTED_EDGE('',*,*,#41652,.T.);
#53437=ORIENTED_EDGE('',*,*,#41650,.T.);
#53438=ORIENTED_EDGE('',*,*,#41368,.T.);
#53439=ORIENTED_EDGE('',*,*,#41655,.T.);
#53440=ORIENTED_EDGE('',*,*,#41656,.T.);
#53441=ORIENTED_EDGE('',*,*,#41657,.T.);
#53442=ORIENTED_EDGE('',*,*,#41658,.T.);
#53443=ORIENTED_EDGE('',*,*,#41659,.T.);
#53444=ORIENTED_EDGE('',*,*,#41660,.T.);
#53445=ORIENTED_EDGE('',*,*,#41655,.F.);
#53446=ORIENTED_EDGE('',*,*,#41661,.T.);
#53447=ORIENTED_EDGE('',*,*,#41421,.T.);
#53448=ORIENTED_EDGE('',*,*,#41662,.F.);
#53449=ORIENTED_EDGE('',*,*,#41656,.F.);
#53450=ORIENTED_EDGE('',*,*,#41662,.T.);
#53451=ORIENTED_EDGE('',*,*,#41420,.T.);
#53452=ORIENTED_EDGE('',*,*,#41663,.F.);
#53453=ORIENTED_EDGE('',*,*,#41657,.F.);
#53454=ORIENTED_EDGE('',*,*,#41663,.T.);
#53455=ORIENTED_EDGE('',*,*,#41427,.T.);
#53456=ORIENTED_EDGE('',*,*,#41664,.F.);
#53457=ORIENTED_EDGE('',*,*,#41658,.F.);
#53458=ORIENTED_EDGE('',*,*,#41664,.T.);
#53459=ORIENTED_EDGE('',*,*,#41426,.T.);
#53460=ORIENTED_EDGE('',*,*,#41665,.F.);
#53461=ORIENTED_EDGE('',*,*,#41659,.F.);
#53462=ORIENTED_EDGE('',*,*,#41665,.T.);
#53463=ORIENTED_EDGE('',*,*,#41425,.T.);
#53464=ORIENTED_EDGE('',*,*,#41423,.T.);
#53465=ORIENTED_EDGE('',*,*,#41666,.F.);
#53466=ORIENTED_EDGE('',*,*,#41660,.F.);
#53467=ORIENTED_EDGE('',*,*,#41666,.T.);
#53468=ORIENTED_EDGE('',*,*,#41422,.T.);
#53469=ORIENTED_EDGE('',*,*,#41661,.F.);
#53470=ORIENTED_EDGE('',*,*,#41411,.F.);
#53471=ORIENTED_EDGE('',*,*,#41406,.T.);
#53472=ORIENTED_EDGE('',*,*,#41414,.T.);
#53473=ORIENTED_EDGE('',*,*,#41429,.T.);
#53474=ORIENTED_EDGE('',*,*,#41667,.F.);
#53475=ORIENTED_EDGE('',*,*,#41668,.T.);
#53476=ORIENTED_EDGE('',*,*,#41669,.T.);
#53477=ORIENTED_EDGE('',*,*,#41670,.T.);
#53478=ORIENTED_EDGE('',*,*,#41671,.T.);
#53479=ORIENTED_EDGE('',*,*,#41672,.F.);
#53480=ORIENTED_EDGE('',*,*,#41673,.F.);
#53481=ORIENTED_EDGE('',*,*,#41674,.F.);
#53482=ORIENTED_EDGE('',*,*,#41675,.T.);
#53483=ORIENTED_EDGE('',*,*,#41676,.F.);
#53484=ORIENTED_EDGE('',*,*,#41677,.T.);
#53485=ORIENTED_EDGE('',*,*,#41667,.T.);
#53486=ORIENTED_EDGE('',*,*,#41678,.T.);
#53487=ORIENTED_EDGE('',*,*,#41679,.T.);
#53488=ORIENTED_EDGE('',*,*,#41680,.F.);
#53489=ORIENTED_EDGE('',*,*,#41681,.F.);
#53490=ORIENTED_EDGE('',*,*,#41680,.T.);
#53491=ORIENTED_EDGE('',*,*,#41682,.T.);
#53492=ORIENTED_EDGE('',*,*,#41668,.F.);
#53493=ORIENTED_EDGE('',*,*,#41677,.F.);
#53494=ORIENTED_EDGE('',*,*,#41683,.F.);
#53495=ORIENTED_EDGE('',*,*,#41684,.F.);
#53496=ORIENTED_EDGE('',*,*,#41669,.F.);
#53497=ORIENTED_EDGE('',*,*,#41685,.T.);
#53498=ORIENTED_EDGE('',*,*,#41686,.F.);
#53499=ORIENTED_EDGE('',*,*,#41687,.T.);
#53500=ORIENTED_EDGE('',*,*,#41688,.T.);
#53501=ORIENTED_EDGE('',*,*,#41689,.F.);
#53502=ORIENTED_EDGE('',*,*,#41690,.F.);
#53503=ORIENTED_EDGE('',*,*,#41691,.T.);
#53504=ORIENTED_EDGE('',*,*,#41692,.T.);
#53505=ORIENTED_EDGE('',*,*,#41693,.F.);
#53506=ORIENTED_EDGE('',*,*,#41689,.T.);
#53507=ORIENTED_EDGE('',*,*,#41694,.F.);
#53508=ORIENTED_EDGE('',*,*,#41695,.F.);
#53509=ORIENTED_EDGE('',*,*,#41696,.T.);
#53510=ORIENTED_EDGE('',*,*,#41697,.F.);
#53511=ORIENTED_EDGE('',*,*,#41686,.T.);
#53512=ORIENTED_EDGE('',*,*,#41696,.F.);
#53513=ORIENTED_EDGE('',*,*,#41698,.T.);
#53514=ORIENTED_EDGE('',*,*,#41672,.T.);
#53515=ORIENTED_EDGE('',*,*,#41699,.F.);
#53516=ORIENTED_EDGE('',*,*,#41700,.F.);
#53517=ORIENTED_EDGE('',*,*,#41695,.T.);
#53518=ORIENTED_EDGE('',*,*,#41673,.T.);
#53519=ORIENTED_EDGE('',*,*,#41701,.F.);
#53520=ORIENTED_EDGE('',*,*,#41702,.T.);
#53521=ORIENTED_EDGE('',*,*,#41703,.T.);
#53522=ORIENTED_EDGE('',*,*,#41704,.T.);
#53523=ORIENTED_EDGE('',*,*,#41670,.F.);
#53524=ORIENTED_EDGE('',*,*,#41705,.F.);
#53525=ORIENTED_EDGE('',*,*,#41704,.F.);
#53526=ORIENTED_EDGE('',*,*,#41706,.T.);
#53527=ORIENTED_EDGE('',*,*,#41707,.T.);
#53528=ORIENTED_EDGE('',*,*,#41708,.T.);
#53529=ORIENTED_EDGE('',*,*,#41687,.F.);
#53530=ORIENTED_EDGE('',*,*,#41697,.T.);
#53531=ORIENTED_EDGE('',*,*,#41671,.F.);
#53532=ORIENTED_EDGE('',*,*,#41709,.F.);
#53533=ORIENTED_EDGE('',*,*,#41710,.F.);
#53534=ORIENTED_EDGE('',*,*,#41711,.F.);
#53535=ORIENTED_EDGE('',*,*,#41683,.T.);
#53536=ORIENTED_EDGE('',*,*,#41712,.F.);
#53537=ORIENTED_EDGE('',*,*,#41690,.T.);
#53538=ORIENTED_EDGE('',*,*,#41713,.F.);
#53539=ORIENTED_EDGE('',*,*,#41707,.F.);
#53540=ORIENTED_EDGE('',*,*,#41714,.F.);
#53541=ORIENTED_EDGE('',*,*,#41710,.T.);
#53542=ORIENTED_EDGE('',*,*,#41715,.T.);
#53543=ORIENTED_EDGE('',*,*,#41404,.T.);
#53544=ORIENTED_EDGE('',*,*,#41403,.T.);
#53545=ORIENTED_EDGE('',*,*,#41684,.T.);
#53546=ORIENTED_EDGE('',*,*,#41711,.T.);
#53547=ORIENTED_EDGE('',*,*,#41714,.T.);
#53548=ORIENTED_EDGE('',*,*,#41716,.T.);
#53549=ORIENTED_EDGE('',*,*,#41717,.F.);
#53550=ORIENTED_EDGE('',*,*,#41674,.T.);
#53551=ORIENTED_EDGE('',*,*,#41718,.T.);
#53552=ORIENTED_EDGE('',*,*,#41719,.F.);
#53553=ORIENTED_EDGE('',*,*,#41675,.F.);
#53554=ORIENTED_EDGE('',*,*,#41720,.T.);
#53555=ORIENTED_EDGE('',*,*,#41721,.T.);
#53556=ORIENTED_EDGE('',*,*,#41722,.T.);
#53557=ORIENTED_EDGE('',*,*,#41678,.F.);
#53558=ORIENTED_EDGE('',*,*,#41723,.F.);
#53559=ORIENTED_EDGE('',*,*,#41676,.T.);
#53560=ORIENTED_EDGE('',*,*,#41719,.T.);
#53561=ORIENTED_EDGE('',*,*,#41724,.T.);
#53562=ORIENTED_EDGE('',*,*,#41725,.T.);
#53563=ORIENTED_EDGE('',*,*,#41681,.T.);
#53564=ORIENTED_EDGE('',*,*,#41726,.T.);
#53565=ORIENTED_EDGE('',*,*,#41721,.F.);
#53566=ORIENTED_EDGE('',*,*,#41727,.F.);
#53567=ORIENTED_EDGE('',*,*,#41691,.F.);
#53568=ORIENTED_EDGE('',*,*,#41712,.T.);
#53569=ORIENTED_EDGE('',*,*,#41685,.F.);
#53570=ORIENTED_EDGE('',*,*,#41682,.F.);
#53571=ORIENTED_EDGE('',*,*,#41679,.F.);
#53572=ORIENTED_EDGE('',*,*,#41722,.F.);
#53573=ORIENTED_EDGE('',*,*,#41728,.F.);
#53574=ORIENTED_EDGE('',*,*,#41729,.T.);
#53575=ORIENTED_EDGE('',*,*,#41692,.F.);
#53576=ORIENTED_EDGE('',*,*,#41730,.T.);
#53577=ORIENTED_EDGE('',*,*,#41708,.F.);
#53578=ORIENTED_EDGE('',*,*,#41713,.T.);
#53579=ORIENTED_EDGE('',*,*,#41693,.T.);
#53580=ORIENTED_EDGE('',*,*,#41731,.T.);
#53581=ORIENTED_EDGE('',*,*,#41732,.T.);
#53582=ORIENTED_EDGE('',*,*,#41733,.T.);
#53583=ORIENTED_EDGE('',*,*,#41688,.F.);
#53584=ORIENTED_EDGE('',*,*,#41699,.T.);
#53585=ORIENTED_EDGE('',*,*,#41694,.T.);
#53586=ORIENTED_EDGE('',*,*,#41733,.F.);
#53587=ORIENTED_EDGE('',*,*,#41734,.F.);
#53588=ORIENTED_EDGE('',*,*,#41735,.T.);
#53589=ORIENTED_EDGE('',*,*,#41700,.T.);
#53590=ORIENTED_EDGE('',*,*,#41736,.T.);
#53591=ORIENTED_EDGE('',*,*,#41701,.T.);
#53592=ORIENTED_EDGE('',*,*,#41698,.F.);
#53593=ORIENTED_EDGE('',*,*,#41737,.F.);
#53594=ORIENTED_EDGE('',*,*,#41738,.T.);
#53595=ORIENTED_EDGE('',*,*,#41739,.T.);
#53596=ORIENTED_EDGE('',*,*,#41705,.T.);
#53597=ORIENTED_EDGE('',*,*,#41702,.F.);
#53598=ORIENTED_EDGE('',*,*,#41740,.T.);
#53599=ORIENTED_EDGE('',*,*,#41741,.T.);
#53600=ORIENTED_EDGE('',*,*,#41742,.F.);
#53601=ORIENTED_EDGE('',*,*,#41739,.F.);
#53602=ORIENTED_EDGE('',*,*,#41715,.F.);
#53603=ORIENTED_EDGE('',*,*,#41709,.T.);
#53604=ORIENTED_EDGE('',*,*,#41706,.F.);
#53605=ORIENTED_EDGE('',*,*,#41703,.F.);
#53606=ORIENTED_EDGE('',*,*,#41742,.T.);
#53607=ORIENTED_EDGE('',*,*,#41743,.T.);
#53608=ORIENTED_EDGE('',*,*,#41744,.T.);
#53609=ORIENTED_EDGE('',*,*,#41745,.F.);
#53610=ORIENTED_EDGE('',*,*,#41746,.F.);
#53611=ORIENTED_EDGE('',*,*,#41747,.T.);
#53612=ORIENTED_EDGE('',*,*,#41748,.T.);
#53613=ORIENTED_EDGE('',*,*,#41401,.F.);
#53614=ORIENTED_EDGE('',*,*,#41744,.F.);
#53615=ORIENTED_EDGE('',*,*,#41749,.T.);
#53616=ORIENTED_EDGE('',*,*,#41750,.T.);
#53617=ORIENTED_EDGE('',*,*,#41751,.F.);
#53618=ORIENTED_EDGE('',*,*,#41748,.F.);
#53619=ORIENTED_EDGE('',*,*,#41752,.T.);
#53620=ORIENTED_EDGE('',*,*,#41753,.F.);
#53621=ORIENTED_EDGE('',*,*,#41716,.F.);
#53622=ORIENTED_EDGE('',*,*,#41402,.T.);
#53623=ORIENTED_EDGE('',*,*,#41751,.T.);
#53624=ORIENTED_EDGE('',*,*,#41717,.T.);
#53625=ORIENTED_EDGE('',*,*,#41754,.T.);
#53626=ORIENTED_EDGE('',*,*,#41720,.F.);
#53627=ORIENTED_EDGE('',*,*,#41755,.T.);
#53628=ORIENTED_EDGE('',*,*,#41724,.F.);
#53629=ORIENTED_EDGE('',*,*,#41718,.F.);
#53630=ORIENTED_EDGE('',*,*,#41756,.T.);
#53631=ORIENTED_EDGE('',*,*,#41725,.F.);
#53632=ORIENTED_EDGE('',*,*,#41755,.F.);
#53633=ORIENTED_EDGE('',*,*,#41396,.T.);
#53634=ORIENTED_EDGE('',*,*,#41727,.T.);
#53635=ORIENTED_EDGE('',*,*,#41723,.T.);
#53636=ORIENTED_EDGE('',*,*,#41395,.F.);
#53637=ORIENTED_EDGE('',*,*,#41730,.F.);
#53638=ORIENTED_EDGE('',*,*,#41728,.T.);
#53639=ORIENTED_EDGE('',*,*,#41726,.F.);
#53640=ORIENTED_EDGE('',*,*,#41757,.T.);
#53641=ORIENTED_EDGE('',*,*,#41731,.F.);
#53642=ORIENTED_EDGE('',*,*,#41729,.F.);
#53643=ORIENTED_EDGE('',*,*,#41394,.T.);
#53644=ORIENTED_EDGE('',*,*,#41734,.T.);
#53645=ORIENTED_EDGE('',*,*,#41732,.F.);
#53646=ORIENTED_EDGE('',*,*,#41757,.F.);
#53647=ORIENTED_EDGE('',*,*,#41758,.T.);
#53648=ORIENTED_EDGE('',*,*,#41759,.F.);
#53649=ORIENTED_EDGE('',*,*,#41737,.T.);
#53650=ORIENTED_EDGE('',*,*,#41736,.F.);
#53651=ORIENTED_EDGE('',*,*,#41735,.F.);
#53652=ORIENTED_EDGE('',*,*,#41760,.T.);
#53653=ORIENTED_EDGE('',*,*,#41740,.F.);
#53654=ORIENTED_EDGE('',*,*,#41738,.F.);
#53655=ORIENTED_EDGE('',*,*,#41405,.F.);
#53656=ORIENTED_EDGE('',*,*,#41743,.F.);
#53657=ORIENTED_EDGE('',*,*,#41741,.F.);
#53658=ORIENTED_EDGE('',*,*,#41761,.T.);
#53659=ORIENTED_EDGE('',*,*,#41745,.T.);
#53660=ORIENTED_EDGE('',*,*,#41746,.T.);
#53661=ORIENTED_EDGE('',*,*,#41762,.F.);
#53662=ORIENTED_EDGE('',*,*,#41763,.F.);
#53663=ORIENTED_EDGE('',*,*,#41764,.T.);
#53664=ORIENTED_EDGE('',*,*,#41752,.F.);
#53665=ORIENTED_EDGE('',*,*,#41749,.F.);
#53666=ORIENTED_EDGE('',*,*,#41747,.F.);
#53667=ORIENTED_EDGE('',*,*,#41764,.F.);
#53668=ORIENTED_EDGE('',*,*,#41765,.F.);
#53669=ORIENTED_EDGE('',*,*,#41766,.F.);
#53670=ORIENTED_EDGE('',*,*,#41767,.T.);
#53671=ORIENTED_EDGE('',*,*,#41768,.F.);
#53672=ORIENTED_EDGE('',*,*,#41750,.F.);
#53673=ORIENTED_EDGE('',*,*,#41766,.T.);
#53674=ORIENTED_EDGE('',*,*,#41756,.F.);
#53675=ORIENTED_EDGE('',*,*,#41754,.F.);
#53676=ORIENTED_EDGE('',*,*,#41753,.T.);
#53677=ORIENTED_EDGE('',*,*,#41768,.T.);
#53678=ORIENTED_EDGE('',*,*,#41769,.F.);
#53679=ORIENTED_EDGE('',*,*,#41770,.T.);
#53680=ORIENTED_EDGE('',*,*,#41397,.F.);
#53681=ORIENTED_EDGE('',*,*,#41762,.T.);
#53682=ORIENTED_EDGE('',*,*,#41761,.F.);
#53683=ORIENTED_EDGE('',*,*,#41760,.F.);
#53684=ORIENTED_EDGE('',*,*,#41759,.T.);
#53685=ORIENTED_EDGE('',*,*,#41758,.F.);
#53686=ORIENTED_EDGE('',*,*,#41400,.F.);
#53687=ORIENTED_EDGE('',*,*,#41771,.T.);
#53688=ORIENTED_EDGE('',*,*,#41772,.T.);
#53689=ORIENTED_EDGE('',*,*,#41773,.F.);
#53690=ORIENTED_EDGE('',*,*,#41773,.T.);
#53691=ORIENTED_EDGE('',*,*,#41774,.T.);
#53692=ORIENTED_EDGE('',*,*,#41775,.T.);
#53693=ORIENTED_EDGE('',*,*,#41767,.F.);
#53694=ORIENTED_EDGE('',*,*,#41765,.T.);
#53695=ORIENTED_EDGE('',*,*,#41763,.T.);
#53696=ORIENTED_EDGE('',*,*,#41775,.F.);
#53697=ORIENTED_EDGE('',*,*,#41776,.T.);
#53698=ORIENTED_EDGE('',*,*,#41777,.T.);
#53699=ORIENTED_EDGE('',*,*,#41778,.F.);
#53700=ORIENTED_EDGE('',*,*,#41779,.T.);
#53701=ORIENTED_EDGE('',*,*,#41769,.T.);
#53702=ORIENTED_EDGE('',*,*,#41778,.T.);
#53703=ORIENTED_EDGE('',*,*,#41780,.F.);
#53704=ORIENTED_EDGE('',*,*,#41770,.F.);
#53705=ORIENTED_EDGE('',*,*,#41781,.T.);
#53706=ORIENTED_EDGE('',*,*,#41782,.F.);
#53707=ORIENTED_EDGE('',*,*,#41783,.F.);
#53708=ORIENTED_EDGE('',*,*,#41784,.F.);
#53709=ORIENTED_EDGE('',*,*,#41399,.F.);
#53710=ORIENTED_EDGE('',*,*,#41398,.F.);
#53711=ORIENTED_EDGE('',*,*,#41780,.T.);
#53712=ORIENTED_EDGE('',*,*,#41785,.F.);
#53713=ORIENTED_EDGE('',*,*,#41786,.F.);
#53714=ORIENTED_EDGE('',*,*,#41771,.F.);
#53715=ORIENTED_EDGE('',*,*,#41784,.T.);
#53716=ORIENTED_EDGE('',*,*,#41787,.F.);
#53717=ORIENTED_EDGE('',*,*,#41788,.F.);
#53718=ORIENTED_EDGE('',*,*,#41772,.F.);
#53719=ORIENTED_EDGE('',*,*,#41786,.T.);
#53720=ORIENTED_EDGE('',*,*,#41789,.F.);
#53721=ORIENTED_EDGE('',*,*,#41790,.F.);
#53722=ORIENTED_EDGE('',*,*,#41774,.F.);
#53723=ORIENTED_EDGE('',*,*,#41788,.T.);
#53724=ORIENTED_EDGE('',*,*,#41791,.F.);
#53725=ORIENTED_EDGE('',*,*,#41792,.F.);
#53726=ORIENTED_EDGE('',*,*,#41776,.F.);
#53727=ORIENTED_EDGE('',*,*,#41790,.T.);
#53728=ORIENTED_EDGE('',*,*,#41793,.F.);
#53729=ORIENTED_EDGE('',*,*,#41794,.F.);
#53730=ORIENTED_EDGE('',*,*,#41777,.F.);
#53731=ORIENTED_EDGE('',*,*,#41792,.T.);
#53732=ORIENTED_EDGE('',*,*,#41795,.F.);
#53733=ORIENTED_EDGE('',*,*,#41781,.F.);
#53734=ORIENTED_EDGE('',*,*,#41779,.F.);
#53735=ORIENTED_EDGE('',*,*,#41794,.T.);
#53736=ORIENTED_EDGE('',*,*,#41796,.F.);
#53737=ORIENTED_EDGE('',*,*,#41797,.T.);
#53738=ORIENTED_EDGE('',*,*,#41383,.F.);
#53739=ORIENTED_EDGE('',*,*,#41798,.F.);
#53740=ORIENTED_EDGE('',*,*,#41782,.T.);
#53741=ORIENTED_EDGE('',*,*,#41798,.T.);
#53742=ORIENTED_EDGE('',*,*,#41393,.F.);
#53743=ORIENTED_EDGE('',*,*,#41799,.F.);
#53744=ORIENTED_EDGE('',*,*,#41783,.T.);
#53745=ORIENTED_EDGE('',*,*,#41799,.T.);
#53746=ORIENTED_EDGE('',*,*,#41392,.F.);
#53747=ORIENTED_EDGE('',*,*,#41800,.F.);
#53748=ORIENTED_EDGE('',*,*,#41785,.T.);
#53749=ORIENTED_EDGE('',*,*,#41800,.T.);
#53750=ORIENTED_EDGE('',*,*,#41391,.F.);
#53751=ORIENTED_EDGE('',*,*,#41801,.F.);
#53752=ORIENTED_EDGE('',*,*,#41787,.T.);
#53753=ORIENTED_EDGE('',*,*,#41801,.T.);
#53754=ORIENTED_EDGE('',*,*,#41388,.F.);
#53755=ORIENTED_EDGE('',*,*,#41802,.F.);
#53756=ORIENTED_EDGE('',*,*,#41789,.T.);
#53757=ORIENTED_EDGE('',*,*,#41802,.T.);
#53758=ORIENTED_EDGE('',*,*,#41387,.F.);
#53759=ORIENTED_EDGE('',*,*,#41803,.F.);
#53760=ORIENTED_EDGE('',*,*,#41791,.T.);
#53761=ORIENTED_EDGE('',*,*,#41803,.T.);
#53762=ORIENTED_EDGE('',*,*,#41386,.F.);
#53763=ORIENTED_EDGE('',*,*,#41804,.F.);
#53764=ORIENTED_EDGE('',*,*,#41793,.T.);
#53765=ORIENTED_EDGE('',*,*,#41804,.T.);
#53766=ORIENTED_EDGE('',*,*,#41385,.F.);
#53767=ORIENTED_EDGE('',*,*,#41805,.F.);
#53768=ORIENTED_EDGE('',*,*,#41795,.T.);
#53769=ORIENTED_EDGE('',*,*,#41805,.T.);
#53770=ORIENTED_EDGE('',*,*,#41384,.F.);
#53771=ORIENTED_EDGE('',*,*,#41797,.F.);
#53772=ORIENTED_EDGE('',*,*,#41796,.T.);
#53773=ORIENTED_EDGE('',*,*,#41390,.F.);
#53774=ORIENTED_EDGE('',*,*,#41150,.T.);
#53775=ORIENTED_EDGE('',*,*,#41806,.T.);
#53776=ORIENTED_EDGE('',*,*,#41807,.T.);
#53777=ORIENTED_EDGE('',*,*,#41808,.T.);
#53778=ORIENTED_EDGE('',*,*,#41809,.F.);
#53779=ORIENTED_EDGE('',*,*,#41810,.F.);
#53780=ORIENTED_EDGE('',*,*,#41155,.T.);
#53781=ORIENTED_EDGE('',*,*,#41152,.T.);
#53782=ORIENTED_EDGE('',*,*,#41151,.T.);
#53783=ORIENTED_EDGE('',*,*,#41808,.F.);
#53784=ORIENTED_EDGE('',*,*,#41381,.F.);
#53785=ORIENTED_EDGE('',*,*,#41811,.F.);
#53786=ORIENTED_EDGE('',*,*,#41812,.T.);
#53787=ORIENTED_EDGE('',*,*,#41806,.F.);
#53788=ORIENTED_EDGE('',*,*,#41149,.F.);
#53789=ORIENTED_EDGE('',*,*,#41154,.F.);
#53790=ORIENTED_EDGE('',*,*,#41812,.F.);
#53791=ORIENTED_EDGE('',*,*,#41813,.F.);
#53792=ORIENTED_EDGE('',*,*,#41809,.T.);
#53793=ORIENTED_EDGE('',*,*,#41807,.F.);
#53794=ORIENTED_EDGE('',*,*,#41382,.F.);
#53795=ORIENTED_EDGE('',*,*,#41156,.F.);
#53796=ORIENTED_EDGE('',*,*,#41810,.T.);
#53797=ORIENTED_EDGE('',*,*,#41814,.F.);
#53798=ORIENTED_EDGE('',*,*,#41815,.F.);
#53799=ORIENTED_EDGE('',*,*,#41377,.T.);
#53800=ORIENTED_EDGE('',*,*,#41376,.T.);
#53801=ORIENTED_EDGE('',*,*,#41158,.F.);
#53802=ORIENTED_EDGE('',*,*,#41816,.T.);
#53803=ORIENTED_EDGE('',*,*,#41811,.T.);
#53804=ORIENTED_EDGE('',*,*,#41380,.F.);
#53805=ORIENTED_EDGE('',*,*,#41379,.T.);
#53806=ORIENTED_EDGE('',*,*,#41160,.T.);
#53807=ORIENTED_EDGE('',*,*,#41375,.T.);
#53808=ORIENTED_EDGE('',*,*,#41374,.T.);
#53809=ORIENTED_EDGE('',*,*,#41817,.F.);
#53810=ORIENTED_EDGE('',*,*,#41814,.T.);
#53811=ORIENTED_EDGE('',*,*,#41813,.T.);
#53812=ORIENTED_EDGE('',*,*,#41816,.F.);
#53813=ORIENTED_EDGE('',*,*,#41818,.F.);
#53814=ORIENTED_EDGE('',*,*,#41373,.T.);
#53815=ORIENTED_EDGE('',*,*,#41818,.T.);
#53816=ORIENTED_EDGE('',*,*,#41817,.T.);
#53817=ORIENTED_EDGE('',*,*,#41378,.T.);
#53818=ORIENTED_EDGE('',*,*,#41815,.T.);
#53819=ORIENTED_EDGE('',*,*,#41364,.T.);
#53820=ORIENTED_EDGE('',*,*,#41361,.T.);
#53821=ORIENTED_EDGE('',*,*,#41367,.F.);
#53822=ORIENTED_EDGE('',*,*,#41173,.F.);
#53823=ORIENTED_EDGE('',*,*,#41170,.F.);
#53824=ORIENTED_EDGE('',*,*,#41167,.F.);
#53825=ORIENTED_EDGE('',*,*,#41164,.F.);
#53826=ORIENTED_EDGE('',*,*,#41819,.F.);
#53827=ORIENTED_EDGE('',*,*,#41178,.F.);
#53828=ORIENTED_EDGE('',*,*,#41186,.F.);
#53829=ORIENTED_EDGE('',*,*,#41353,.F.);
#53830=ORIENTED_EDGE('',*,*,#41191,.F.);
#53831=ORIENTED_EDGE('',*,*,#41820,.F.);
#53832=ORIENTED_EDGE('',*,*,#41162,.F.);
#53833=ORIENTED_EDGE('',*,*,#41166,.F.);
#53834=ORIENTED_EDGE('',*,*,#41169,.F.);
#53835=ORIENTED_EDGE('',*,*,#41172,.F.);
#53836=ORIENTED_EDGE('',*,*,#41366,.F.);
#53837=ORIENTED_EDGE('',*,*,#41176,.F.);
#53838=ORIENTED_EDGE('',*,*,#41365,.T.);
#53839=ORIENTED_EDGE('',*,*,#41189,.F.);
#53840=ORIENTED_EDGE('',*,*,#41354,.F.);
#53841=ORIENTED_EDGE('',*,*,#41187,.F.);
#53842=ORIENTED_EDGE('',*,*,#41184,.F.);
#53843=ORIENTED_EDGE('',*,*,#41180,.F.);
#53844=ORIENTED_EDGE('',*,*,#41179,.T.);
#53845=ORIENTED_EDGE('',*,*,#41819,.T.);
#53846=ORIENTED_EDGE('',*,*,#41163,.T.);
#53847=ORIENTED_EDGE('',*,*,#41820,.T.);
#53848=ORIENTED_EDGE('',*,*,#41192,.T.);
#53849=ORIENTED_EDGE('',*,*,#41357,.F.);
#53850=ORIENTED_EDGE('',*,*,#41363,.T.);
#53851=ORIENTED_EDGE('',*,*,#41821,.F.);
#53852=ORIENTED_EDGE('',*,*,#41822,.T.);
#53853=ORIENTED_EDGE('',*,*,#41823,.F.);
#53854=ORIENTED_EDGE('',*,*,#41824,.T.);
#53855=ORIENTED_EDGE('',*,*,#41825,.T.);
#53856=ORIENTED_EDGE('',*,*,#41826,.F.);
#53857=ORIENTED_EDGE('',*,*,#41827,.F.);
#53858=ORIENTED_EDGE('',*,*,#41828,.F.);
#53859=ORIENTED_EDGE('',*,*,#41829,.F.);
#53860=ORIENTED_EDGE('',*,*,#41830,.F.);
#53861=ORIENTED_EDGE('',*,*,#41831,.T.);
#53862=ORIENTED_EDGE('',*,*,#41832,.F.);
#53863=ORIENTED_EDGE('',*,*,#41833,.F.);
#53864=ORIENTED_EDGE('',*,*,#41834,.F.);
#53865=ORIENTED_EDGE('',*,*,#41835,.F.);
#53866=ORIENTED_EDGE('',*,*,#41836,.F.);
#53867=ORIENTED_EDGE('',*,*,#41837,.T.);
#53868=ORIENTED_EDGE('',*,*,#41838,.T.);
#53869=ORIENTED_EDGE('',*,*,#41839,.F.);
#53870=ORIENTED_EDGE('',*,*,#41206,.T.);
#53871=ORIENTED_EDGE('',*,*,#41840,.F.);
#53872=ORIENTED_EDGE('',*,*,#41841,.F.);
#53873=ORIENTED_EDGE('',*,*,#41842,.F.);
#53874=ORIENTED_EDGE('',*,*,#41204,.T.);
#53875=ORIENTED_EDGE('',*,*,#41843,.F.);
#53876=ORIENTED_EDGE('',*,*,#41844,.F.);
#53877=ORIENTED_EDGE('',*,*,#41207,.F.);
#53878=ORIENTED_EDGE('',*,*,#41839,.T.);
#53879=ORIENTED_EDGE('',*,*,#41845,.T.);
#53880=ORIENTED_EDGE('',*,*,#41846,.T.);
#53881=ORIENTED_EDGE('',*,*,#41847,.F.);
#53882=ORIENTED_EDGE('',*,*,#41848,.F.);
#53883=ORIENTED_EDGE('',*,*,#41208,.F.);
#53884=ORIENTED_EDGE('',*,*,#41848,.T.);
#53885=ORIENTED_EDGE('',*,*,#41849,.F.);
#53886=ORIENTED_EDGE('',*,*,#41850,.F.);
#53887=ORIENTED_EDGE('',*,*,#41851,.T.);
#53888=ORIENTED_EDGE('',*,*,#41852,.T.);
#53889=ORIENTED_EDGE('',*,*,#41853,.T.);
#53890=ORIENTED_EDGE('',*,*,#41854,.F.);
#53891=ORIENTED_EDGE('',*,*,#41855,.T.);
#53892=ORIENTED_EDGE('',*,*,#41201,.T.);
#53893=ORIENTED_EDGE('',*,*,#41856,.T.);
#53894=ORIENTED_EDGE('',*,*,#41200,.F.);
#53895=ORIENTED_EDGE('',*,*,#41857,.F.);
#53896=ORIENTED_EDGE('',*,*,#41858,.F.);
#53897=ORIENTED_EDGE('',*,*,#41859,.F.);
#53898=ORIENTED_EDGE('',*,*,#41860,.F.);
#53899=ORIENTED_EDGE('',*,*,#41861,.F.);
#53900=ORIENTED_EDGE('',*,*,#41862,.F.);
#53901=ORIENTED_EDGE('',*,*,#41863,.T.);
#53902=ORIENTED_EDGE('',*,*,#41864,.T.);
#53903=ORIENTED_EDGE('',*,*,#41856,.F.);
#53904=ORIENTED_EDGE('',*,*,#41210,.F.);
#53905=ORIENTED_EDGE('',*,*,#41865,.F.);
#53906=ORIENTED_EDGE('',*,*,#41847,.T.);
#53907=ORIENTED_EDGE('',*,*,#41866,.T.);
#53908=ORIENTED_EDGE('',*,*,#41867,.T.);
#53909=ORIENTED_EDGE('',*,*,#41868,.T.);
#53910=ORIENTED_EDGE('',*,*,#41869,.F.);
#53911=ORIENTED_EDGE('',*,*,#41870,.F.);
#53912=ORIENTED_EDGE('',*,*,#41871,.T.);
#53913=ORIENTED_EDGE('',*,*,#41872,.F.);
#53914=ORIENTED_EDGE('',*,*,#41873,.F.);
#53915=ORIENTED_EDGE('',*,*,#41874,.F.);
#53916=ORIENTED_EDGE('',*,*,#41211,.F.);
#53917=ORIENTED_EDGE('',*,*,#41874,.T.);
#53918=ORIENTED_EDGE('',*,*,#41875,.F.);
#53919=ORIENTED_EDGE('',*,*,#41876,.F.);
#53920=ORIENTED_EDGE('',*,*,#41877,.F.);
#53921=ORIENTED_EDGE('',*,*,#41878,.T.);
#53922=ORIENTED_EDGE('',*,*,#41879,.F.);
#53923=ORIENTED_EDGE('',*,*,#41880,.F.);
#53924=ORIENTED_EDGE('',*,*,#41881,.F.);
#53925=ORIENTED_EDGE('',*,*,#41199,.F.);
#53926=ORIENTED_EDGE('',*,*,#41882,.F.);
#53927=ORIENTED_EDGE('',*,*,#41883,.F.);
#53928=ORIENTED_EDGE('',*,*,#41884,.T.);
#53929=ORIENTED_EDGE('',*,*,#41885,.T.);
#53930=ORIENTED_EDGE('',*,*,#41886,.F.);
#53931=ORIENTED_EDGE('',*,*,#41887,.F.);
#53932=ORIENTED_EDGE('',*,*,#41888,.F.);
#53933=ORIENTED_EDGE('',*,*,#41857,.T.);
#53934=ORIENTED_EDGE('',*,*,#41889,.F.);
#53935=ORIENTED_EDGE('',*,*,#41214,.T.);
#53936=ORIENTED_EDGE('',*,*,#41890,.T.);
#53937=ORIENTED_EDGE('',*,*,#41891,.T.);
#53938=ORIENTED_EDGE('',*,*,#41892,.F.);
#53939=ORIENTED_EDGE('',*,*,#41893,.F.);
#53940=ORIENTED_EDGE('',*,*,#41894,.T.);
#53941=ORIENTED_EDGE('',*,*,#41895,.F.);
#53942=ORIENTED_EDGE('',*,*,#41212,.T.);
#53943=ORIENTED_EDGE('',*,*,#41881,.T.);
#53944=ORIENTED_EDGE('',*,*,#41890,.F.);
#53945=ORIENTED_EDGE('',*,*,#41213,.T.);
#53946=ORIENTED_EDGE('',*,*,#41895,.T.);
#53947=ORIENTED_EDGE('',*,*,#41880,.T.);
#53948=ORIENTED_EDGE('',*,*,#41865,.T.);
#53949=ORIENTED_EDGE('',*,*,#41209,.T.);
#53950=ORIENTED_EDGE('',*,*,#41849,.T.);
#53951=ORIENTED_EDGE('',*,*,#41896,.F.);
#53952=ORIENTED_EDGE('',*,*,#41821,.T.);
#53953=ORIENTED_EDGE('',*,*,#41897,.T.);
#53954=ORIENTED_EDGE('',*,*,#41898,.F.);
#53955=ORIENTED_EDGE('',*,*,#41899,.F.);
#53956=ORIENTED_EDGE('',*,*,#41900,.F.);
#53957=ORIENTED_EDGE('',*,*,#41901,.F.);
#53958=ORIENTED_EDGE('',*,*,#41832,.T.);
#53959=ORIENTED_EDGE('',*,*,#41882,.T.);
#53960=ORIENTED_EDGE('',*,*,#41198,.T.);
#53961=ORIENTED_EDGE('',*,*,#41902,.T.);
#53962=ORIENTED_EDGE('',*,*,#41902,.F.);
#53963=ORIENTED_EDGE('',*,*,#41197,.T.);
#53964=ORIENTED_EDGE('',*,*,#41903,.T.);
#53965=ORIENTED_EDGE('',*,*,#41883,.T.);
#53966=ORIENTED_EDGE('',*,*,#41903,.F.);
#53967=ORIENTED_EDGE('',*,*,#41196,.T.);
#53968=ORIENTED_EDGE('',*,*,#41904,.F.);
#53969=ORIENTED_EDGE('',*,*,#41905,.F.);
#53970=ORIENTED_EDGE('',*,*,#41906,.F.);
#53971=ORIENTED_EDGE('',*,*,#41892,.T.);
#53972=ORIENTED_EDGE('',*,*,#41907,.T.);
#53973=ORIENTED_EDGE('',*,*,#41202,.F.);
#53974=ORIENTED_EDGE('',*,*,#41855,.F.);
#53975=ORIENTED_EDGE('',*,*,#41908,.F.);
#53976=ORIENTED_EDGE('',*,*,#41203,.F.);
#53977=ORIENTED_EDGE('',*,*,#41908,.T.);
#53978=ORIENTED_EDGE('',*,*,#41864,.F.);
#53979=ORIENTED_EDGE('',*,*,#41909,.F.);
#53980=ORIENTED_EDGE('',*,*,#41843,.T.);
#53981=ORIENTED_EDGE('',*,*,#41840,.T.);
#53982=ORIENTED_EDGE('',*,*,#41205,.T.);
#53983=ORIENTED_EDGE('',*,*,#41842,.T.);
#53984=ORIENTED_EDGE('',*,*,#41910,.F.);
#53985=ORIENTED_EDGE('',*,*,#41911,.F.);
#53986=ORIENTED_EDGE('',*,*,#41912,.T.);
#53987=ORIENTED_EDGE('',*,*,#41913,.F.);
#53988=ORIENTED_EDGE('',*,*,#41914,.T.);
#53989=ORIENTED_EDGE('',*,*,#41915,.F.);
#53990=ORIENTED_EDGE('',*,*,#41868,.F.);
#53991=ORIENTED_EDGE('',*,*,#41916,.F.);
#53992=ORIENTED_EDGE('',*,*,#41917,.F.);
#53993=ORIENTED_EDGE('',*,*,#41918,.T.);
#53994=ORIENTED_EDGE('',*,*,#41919,.T.);
#53995=ORIENTED_EDGE('',*,*,#41913,.T.);
#53996=ORIENTED_EDGE('',*,*,#41867,.F.);
#53997=ORIENTED_EDGE('',*,*,#41920,.F.);
#53998=ORIENTED_EDGE('',*,*,#41916,.T.);
#53999=ORIENTED_EDGE('',*,*,#41921,.F.);
#54000=ORIENTED_EDGE('',*,*,#41845,.F.);
#54001=ORIENTED_EDGE('',*,*,#41922,.T.);
#54002=ORIENTED_EDGE('',*,*,#41923,.F.);
#54003=ORIENTED_EDGE('',*,*,#41924,.F.);
#54004=ORIENTED_EDGE('',*,*,#41925,.T.);
#54005=ORIENTED_EDGE('',*,*,#41926,.F.);
#54006=ORIENTED_EDGE('',*,*,#41927,.T.);
#54007=ORIENTED_EDGE('',*,*,#41928,.F.);
#54008=ORIENTED_EDGE('',*,*,#41929,.F.);
#54009=ORIENTED_EDGE('',*,*,#41923,.T.);
#54010=ORIENTED_EDGE('',*,*,#41930,.T.);
#54011=ORIENTED_EDGE('',*,*,#41926,.T.);
#54012=ORIENTED_EDGE('',*,*,#41931,.F.);
#54013=ORIENTED_EDGE('',*,*,#41932,.F.);
#54014=ORIENTED_EDGE('',*,*,#41933,.T.);
#54015=ORIENTED_EDGE('',*,*,#41934,.F.);
#54016=ORIENTED_EDGE('',*,*,#41935,.F.);
#54017=ORIENTED_EDGE('',*,*,#41936,.F.);
#54018=ORIENTED_EDGE('',*,*,#41937,.T.);
#54019=ORIENTED_EDGE('',*,*,#41938,.F.);
#54020=ORIENTED_EDGE('',*,*,#41935,.T.);
#54021=ORIENTED_EDGE('',*,*,#41939,.T.);
#54022=ORIENTED_EDGE('',*,*,#41940,.F.);
#54023=ORIENTED_EDGE('',*,*,#41941,.F.);
#54024=ORIENTED_EDGE('',*,*,#41942,.F.);
#54025=ORIENTED_EDGE('',*,*,#41941,.T.);
#54026=ORIENTED_EDGE('',*,*,#41943,.F.);
#54027=ORIENTED_EDGE('',*,*,#41944,.F.);
#54028=ORIENTED_EDGE('',*,*,#41943,.T.);
#54029=ORIENTED_EDGE('',*,*,#41940,.T.);
#54030=ORIENTED_EDGE('',*,*,#41945,.T.);
#54031=ORIENTED_EDGE('',*,*,#41946,.F.);
#54032=ORIENTED_EDGE('',*,*,#41947,.F.);
#54033=ORIENTED_EDGE('',*,*,#41948,.T.);
#54034=ORIENTED_EDGE('',*,*,#41351,.F.);
#54035=ORIENTED_EDGE('',*,*,#41949,.F.);
#54036=ORIENTED_EDGE('',*,*,#41828,.T.);
#54037=ORIENTED_EDGE('',*,*,#41950,.T.);
#54038=ORIENTED_EDGE('',*,*,#41951,.F.);
#54039=ORIENTED_EDGE('',*,*,#41952,.F.);
#54040=ORIENTED_EDGE('',*,*,#41826,.T.);
#54041=ORIENTED_EDGE('',*,*,#41952,.T.);
#54042=ORIENTED_EDGE('',*,*,#41953,.F.);
#54043=ORIENTED_EDGE('',*,*,#41948,.F.);
#54044=ORIENTED_EDGE('',*,*,#41827,.T.);
#54045=ORIENTED_EDGE('',*,*,#41954,.T.);
#54046=ORIENTED_EDGE('',*,*,#41955,.T.);
#54047=ORIENTED_EDGE('',*,*,#41352,.F.);
#54048=ORIENTED_EDGE('',*,*,#41953,.T.);
#54049=ORIENTED_EDGE('',*,*,#41956,.T.);
#54050=ORIENTED_EDGE('',*,*,#41955,.F.);
#54051=ORIENTED_EDGE('',*,*,#41957,.F.);
#54052=ORIENTED_EDGE('',*,*,#41835,.T.);
#54053=ORIENTED_EDGE('',*,*,#41900,.T.);
#54054=ORIENTED_EDGE('',*,*,#41958,.T.);
#54055=ORIENTED_EDGE('',*,*,#41898,.T.);
#54056=ORIENTED_EDGE('',*,*,#41959,.F.);
#54057=ORIENTED_EDGE('',*,*,#41960,.F.);
#54058=ORIENTED_EDGE('',*,*,#41961,.F.);
#54059=ORIENTED_EDGE('',*,*,#41962,.T.);
#54060=ORIENTED_EDGE('',*,*,#41963,.T.);
#54061=ORIENTED_EDGE('',*,*,#41964,.T.);
#54062=ORIENTED_EDGE('',*,*,#41965,.F.);
#54063=ORIENTED_EDGE('',*,*,#41838,.F.);
#54064=ORIENTED_EDGE('',*,*,#41966,.T.);
#54065=ORIENTED_EDGE('',*,*,#41961,.T.);
#54066=ORIENTED_EDGE('',*,*,#41861,.T.);
#54067=ORIENTED_EDGE('',*,*,#41967,.F.);
#54068=ORIENTED_EDGE('',*,*,#41968,.F.);
#54069=ORIENTED_EDGE('',*,*,#41969,.T.);
#54070=ORIENTED_EDGE('',*,*,#41970,.F.);
#54071=ORIENTED_EDGE('',*,*,#41971,.F.);
#54072=ORIENTED_EDGE('',*,*,#41968,.T.);
#54073=ORIENTED_EDGE('',*,*,#41862,.T.);
#54074=ORIENTED_EDGE('',*,*,#41971,.T.);
#54075=ORIENTED_EDGE('',*,*,#41972,.F.);
#54076=ORIENTED_EDGE('',*,*,#41973,.T.);
#54077=ORIENTED_EDGE('',*,*,#41974,.F.);
#54078=ORIENTED_EDGE('',*,*,#41975,.F.);
#54079=ORIENTED_EDGE('',*,*,#41973,.F.);
#54080=ORIENTED_EDGE('',*,*,#41910,.T.);
#54081=ORIENTED_EDGE('',*,*,#41844,.T.);
#54082=ORIENTED_EDGE('',*,*,#41975,.T.);
#54083=ORIENTED_EDGE('',*,*,#41909,.T.);
#54084=ORIENTED_EDGE('',*,*,#41863,.F.);
#54085=ORIENTED_EDGE('',*,*,#41974,.T.);
#54086=ORIENTED_EDGE('',*,*,#41976,.F.);
#54087=ORIENTED_EDGE('',*,*,#41977,.F.);
#54088=ORIENTED_EDGE('',*,*,#41978,.F.);
#54089=ORIENTED_EDGE('',*,*,#41979,.F.);
#54090=ORIENTED_EDGE('',*,*,#41980,.F.);
#54091=ORIENTED_EDGE('',*,*,#41981,.F.);
#54092=ORIENTED_EDGE('',*,*,#41982,.F.);
#54093=ORIENTED_EDGE('',*,*,#41983,.F.);
#54094=ORIENTED_EDGE('',*,*,#41984,.F.);
#54095=ORIENTED_EDGE('',*,*,#41985,.T.);
#54096=ORIENTED_EDGE('',*,*,#41986,.F.);
#54097=ORIENTED_EDGE('',*,*,#41987,.T.);
#54098=ORIENTED_EDGE('',*,*,#41988,.F.);
#54099=ORIENTED_EDGE('',*,*,#41989,.F.);
#54100=ORIENTED_EDGE('',*,*,#41859,.T.);
#54101=ORIENTED_EDGE('',*,*,#41989,.T.);
#54102=ORIENTED_EDGE('',*,*,#41990,.F.);
#54103=ORIENTED_EDGE('',*,*,#41991,.F.);
#54104=ORIENTED_EDGE('',*,*,#41992,.T.);
#54105=ORIENTED_EDGE('',*,*,#41984,.T.);
#54106=ORIENTED_EDGE('',*,*,#41993,.F.);
#54107=ORIENTED_EDGE('',*,*,#41994,.F.);
#54108=ORIENTED_EDGE('',*,*,#41995,.F.);
#54109=ORIENTED_EDGE('',*,*,#41996,.F.);
#54110=ORIENTED_EDGE('',*,*,#41871,.F.);
#54111=ORIENTED_EDGE('',*,*,#41997,.F.);
#54112=ORIENTED_EDGE('',*,*,#41998,.F.);
#54113=ORIENTED_EDGE('',*,*,#41860,.T.);
#54114=ORIENTED_EDGE('',*,*,#41992,.F.);
#54115=ORIENTED_EDGE('',*,*,#41999,.T.);
#54116=ORIENTED_EDGE('',*,*,#41345,.F.);
#54117=ORIENTED_EDGE('',*,*,#42000,.F.);
#54118=ORIENTED_EDGE('',*,*,#41996,.T.);
#54119=ORIENTED_EDGE('',*,*,#42001,.F.);
#54120=ORIENTED_EDGE('',*,*,#42002,.F.);
#54121=ORIENTED_EDGE('',*,*,#41985,.F.);
#54122=ORIENTED_EDGE('',*,*,#42000,.T.);
#54123=ORIENTED_EDGE('',*,*,#41348,.F.);
#54124=ORIENTED_EDGE('',*,*,#41999,.F.);
#54125=ORIENTED_EDGE('',*,*,#42003,.F.);
#54126=ORIENTED_EDGE('',*,*,#42004,.F.);
#54127=ORIENTED_EDGE('',*,*,#42005,.F.);
#54128=ORIENTED_EDGE('',*,*,#41346,.F.);
#54129=ORIENTED_EDGE('',*,*,#42006,.T.);
#54130=ORIENTED_EDGE('',*,*,#42005,.T.);
#54131=ORIENTED_EDGE('',*,*,#42007,.F.);
#54132=ORIENTED_EDGE('',*,*,#42008,.F.);
#54133=ORIENTED_EDGE('',*,*,#41342,.T.);
#54134=ORIENTED_EDGE('',*,*,#41343,.T.);
#54135=ORIENTED_EDGE('',*,*,#42009,.F.);
#54136=ORIENTED_EDGE('',*,*,#42010,.T.);
#54137=ORIENTED_EDGE('',*,*,#42011,.T.);
#54138=ORIENTED_EDGE('',*,*,#42012,.T.);
#54139=ORIENTED_EDGE('',*,*,#42008,.T.);
#54140=ORIENTED_EDGE('',*,*,#42013,.T.);
#54141=ORIENTED_EDGE('',*,*,#42014,.F.);
#54142=ORIENTED_EDGE('',*,*,#41336,.T.);
#54143=ORIENTED_EDGE('',*,*,#41340,.F.);
#54144=ORIENTED_EDGE('',*,*,#41324,.T.);
#54145=ORIENTED_EDGE('',*,*,#41335,.F.);
#54146=ORIENTED_EDGE('',*,*,#42015,.T.);
#54147=ORIENTED_EDGE('',*,*,#41326,.T.);
#54148=ORIENTED_EDGE('',*,*,#42016,.F.);
#54149=ORIENTED_EDGE('',*,*,#42017,.F.);
#54150=ORIENTED_EDGE('',*,*,#42018,.T.);
#54151=ORIENTED_EDGE('',*,*,#42019,.T.);
#54152=ORIENTED_EDGE('',*,*,#42020,.T.);
#54153=ORIENTED_EDGE('',*,*,#42021,.T.);
#54154=ORIENTED_EDGE('',*,*,#42022,.F.);
#54155=ORIENTED_EDGE('',*,*,#42017,.T.);
#54156=ORIENTED_EDGE('',*,*,#42023,.T.);
#54157=ORIENTED_EDGE('',*,*,#42024,.F.);
#54158=ORIENTED_EDGE('',*,*,#42025,.T.);
#54159=ORIENTED_EDGE('',*,*,#42026,.T.);
#54160=ORIENTED_EDGE('',*,*,#42027,.T.);
#54161=ORIENTED_EDGE('',*,*,#42022,.T.);
#54162=ORIENTED_EDGE('',*,*,#42028,.T.);
#54163=ORIENTED_EDGE('',*,*,#42029,.T.);
#54164=ORIENTED_EDGE('',*,*,#42030,.F.);
#54165=ORIENTED_EDGE('',*,*,#42024,.T.);
#54166=ORIENTED_EDGE('',*,*,#42031,.T.);
#54167=ORIENTED_EDGE('',*,*,#42032,.T.);
#54168=ORIENTED_EDGE('',*,*,#41327,.T.);
#54169=ORIENTED_EDGE('',*,*,#42015,.F.);
#54170=ORIENTED_EDGE('',*,*,#42031,.F.);
#54171=ORIENTED_EDGE('',*,*,#42033,.T.);
#54172=ORIENTED_EDGE('',*,*,#41328,.T.);
#54173=ORIENTED_EDGE('',*,*,#42032,.F.);
#54174=ORIENTED_EDGE('',*,*,#42023,.F.);
#54175=ORIENTED_EDGE('',*,*,#42034,.T.);
#54176=ORIENTED_EDGE('',*,*,#41329,.T.);
#54177=ORIENTED_EDGE('',*,*,#42033,.F.);
#54178=ORIENTED_EDGE('',*,*,#42027,.F.);
#54179=ORIENTED_EDGE('',*,*,#42016,.T.);
#54180=ORIENTED_EDGE('',*,*,#41331,.T.);
#54181=ORIENTED_EDGE('',*,*,#42035,.F.);
#54182=ORIENTED_EDGE('',*,*,#42018,.F.);
#54183=ORIENTED_EDGE('',*,*,#42035,.T.);
#54184=ORIENTED_EDGE('',*,*,#41330,.T.);
#54185=ORIENTED_EDGE('',*,*,#42034,.F.);
#54186=ORIENTED_EDGE('',*,*,#42036,.F.);
#54187=ORIENTED_EDGE('',*,*,#42026,.F.);
#54188=ORIENTED_EDGE('',*,*,#42037,.F.);
#54189=ORIENTED_EDGE('',*,*,#42038,.T.);
#54190=ORIENTED_EDGE('',*,*,#42039,.T.);
#54191=ORIENTED_EDGE('',*,*,#42019,.F.);
#54192=ORIENTED_EDGE('',*,*,#42036,.T.);
#54193=ORIENTED_EDGE('',*,*,#42040,.F.);
#54194=ORIENTED_EDGE('',*,*,#42041,.F.);
#54195=ORIENTED_EDGE('',*,*,#42042,.F.);
#54196=ORIENTED_EDGE('',*,*,#42020,.F.);
#54197=ORIENTED_EDGE('',*,*,#42039,.F.);
#54198=ORIENTED_EDGE('',*,*,#42042,.T.);
#54199=ORIENTED_EDGE('',*,*,#42043,.F.);
#54200=ORIENTED_EDGE('',*,*,#42044,.T.);
#54201=ORIENTED_EDGE('',*,*,#42028,.F.);
#54202=ORIENTED_EDGE('',*,*,#42021,.F.);
#54203=ORIENTED_EDGE('',*,*,#42044,.F.);
#54204=ORIENTED_EDGE('',*,*,#42045,.F.);
#54205=ORIENTED_EDGE('',*,*,#42046,.F.);
#54206=ORIENTED_EDGE('',*,*,#42047,.T.);
#54207=ORIENTED_EDGE('',*,*,#42048,.F.);
#54208=ORIENTED_EDGE('',*,*,#42049,.F.);
#54209=ORIENTED_EDGE('',*,*,#42049,.T.);
#54210=ORIENTED_EDGE('',*,*,#42050,.F.);
#54211=ORIENTED_EDGE('',*,*,#42051,.T.);
#54212=ORIENTED_EDGE('',*,*,#42052,.F.);
#54213=ORIENTED_EDGE('',*,*,#42053,.F.);
#54214=ORIENTED_EDGE('',*,*,#42029,.F.);
#54215=ORIENTED_EDGE('',*,*,#42054,.T.);
#54216=ORIENTED_EDGE('',*,*,#41267,.T.);
#54217=ORIENTED_EDGE('',*,*,#42055,.T.);
#54218=ORIENTED_EDGE('',*,*,#42053,.T.);
#54219=ORIENTED_EDGE('',*,*,#42055,.F.);
#54220=ORIENTED_EDGE('',*,*,#41266,.T.);
#54221=ORIENTED_EDGE('',*,*,#42056,.T.);
#54222=ORIENTED_EDGE('',*,*,#42030,.T.);
#54223=ORIENTED_EDGE('',*,*,#42056,.F.);
#54224=ORIENTED_EDGE('',*,*,#41265,.F.);
#54225=ORIENTED_EDGE('',*,*,#41262,.F.);
#54226=ORIENTED_EDGE('',*,*,#42057,.T.);
#54227=ORIENTED_EDGE('',*,*,#42025,.F.);
#54228=ORIENTED_EDGE('',*,*,#42057,.F.);
#54229=ORIENTED_EDGE('',*,*,#41261,.T.);
#54230=ORIENTED_EDGE('',*,*,#42058,.T.);
#54231=ORIENTED_EDGE('',*,*,#42037,.T.);
#54232=ORIENTED_EDGE('',*,*,#42058,.F.);
#54233=ORIENTED_EDGE('',*,*,#41260,.T.);
#54234=ORIENTED_EDGE('',*,*,#42059,.F.);
#54235=ORIENTED_EDGE('',*,*,#42060,.T.);
#54236=ORIENTED_EDGE('',*,*,#42060,.F.);
#54237=ORIENTED_EDGE('',*,*,#42061,.T.);
#54238=ORIENTED_EDGE('',*,*,#42062,.T.);
#54239=ORIENTED_EDGE('',*,*,#42063,.T.);
#54240=ORIENTED_EDGE('',*,*,#42064,.T.);
#54241=ORIENTED_EDGE('',*,*,#42038,.F.);
#54242=ORIENTED_EDGE('',*,*,#42065,.F.);
#54243=ORIENTED_EDGE('',*,*,#42066,.F.);
#54244=ORIENTED_EDGE('',*,*,#42046,.T.);
#54245=ORIENTED_EDGE('',*,*,#42067,.F.);
#54246=ORIENTED_EDGE('',*,*,#42040,.T.);
#54247=ORIENTED_EDGE('',*,*,#42064,.F.);
#54248=ORIENTED_EDGE('',*,*,#42043,.T.);
#54249=ORIENTED_EDGE('',*,*,#42041,.T.);
#54250=ORIENTED_EDGE('',*,*,#42067,.T.);
#54251=ORIENTED_EDGE('',*,*,#42045,.T.);
#54252=ORIENTED_EDGE('',*,*,#41323,.F.);
#54253=ORIENTED_EDGE('',*,*,#41321,.T.);
#54254=ORIENTED_EDGE('',*,*,#41320,.F.);
#54255=ORIENTED_EDGE('',*,*,#41315,.T.);
#54256=ORIENTED_EDGE('',*,*,#41312,.F.);
#54257=ORIENTED_EDGE('',*,*,#41313,.T.);
#54258=ORIENTED_EDGE('',*,*,#41310,.T.);
#54259=ORIENTED_EDGE('',*,*,#42068,.T.);
#54260=ORIENTED_EDGE('',*,*,#42069,.T.);
#54261=ORIENTED_EDGE('',*,*,#42070,.F.);
#54262=ORIENTED_EDGE('',*,*,#42071,.T.);
#54263=ORIENTED_EDGE('',*,*,#42072,.T.);
#54264=ORIENTED_EDGE('',*,*,#42073,.F.);
#54265=ORIENTED_EDGE('',*,*,#42074,.F.);
#54266=ORIENTED_EDGE('',*,*,#41308,.F.);
#54267=ORIENTED_EDGE('',*,*,#42074,.T.);
#54268=ORIENTED_EDGE('',*,*,#42075,.F.);
#54269=ORIENTED_EDGE('',*,*,#42076,.T.);
#54270=ORIENTED_EDGE('',*,*,#42077,.T.);
#54271=ORIENTED_EDGE('',*,*,#42068,.F.);
#54272=ORIENTED_EDGE('',*,*,#41309,.T.);
#54273=ORIENTED_EDGE('',*,*,#42078,.T.);
#54274=ORIENTED_EDGE('',*,*,#42079,.T.);
#54275=ORIENTED_EDGE('',*,*,#42069,.F.);
#54276=ORIENTED_EDGE('',*,*,#42077,.F.);
#54277=ORIENTED_EDGE('',*,*,#42080,.F.);
#54278=ORIENTED_EDGE('',*,*,#42079,.F.);
#54279=ORIENTED_EDGE('',*,*,#42081,.T.);
#54280=ORIENTED_EDGE('',*,*,#42082,.T.);
#54281=ORIENTED_EDGE('',*,*,#42083,.T.);
#54282=ORIENTED_EDGE('',*,*,#42084,.F.);
#54283=ORIENTED_EDGE('',*,*,#42082,.F.);
#54284=ORIENTED_EDGE('',*,*,#42085,.T.);
#54285=ORIENTED_EDGE('',*,*,#42086,.T.);
#54286=ORIENTED_EDGE('',*,*,#42087,.T.);
#54287=ORIENTED_EDGE('',*,*,#42088,.F.);
#54288=ORIENTED_EDGE('',*,*,#42089,.F.);
#54289=ORIENTED_EDGE('',*,*,#42085,.F.);
#54290=ORIENTED_EDGE('',*,*,#42090,.T.);
#54291=ORIENTED_EDGE('',*,*,#42091,.F.);
#54292=ORIENTED_EDGE('',*,*,#42083,.F.);
#54293=ORIENTED_EDGE('',*,*,#42089,.T.);
#54294=ORIENTED_EDGE('',*,*,#42092,.T.);
#54295=ORIENTED_EDGE('',*,*,#42093,.T.);
#54296=ORIENTED_EDGE('',*,*,#42094,.T.);
#54297=ORIENTED_EDGE('',*,*,#42095,.T.);
#54298=ORIENTED_EDGE('',*,*,#42096,.T.);
#54299=ORIENTED_EDGE('',*,*,#42097,.T.);
#54300=ORIENTED_EDGE('',*,*,#42098,.T.);
#54301=ORIENTED_EDGE('',*,*,#42099,.T.);
#54302=ORIENTED_EDGE('',*,*,#42091,.T.);
#54303=ORIENTED_EDGE('',*,*,#42099,.F.);
#54304=ORIENTED_EDGE('',*,*,#42100,.T.);
#54305=ORIENTED_EDGE('',*,*,#42101,.T.);
#54306=ORIENTED_EDGE('',*,*,#42070,.T.);
#54307=ORIENTED_EDGE('',*,*,#42080,.T.);
#54308=ORIENTED_EDGE('',*,*,#42084,.T.);
#54309=ORIENTED_EDGE('',*,*,#42102,.T.);
#54310=ORIENTED_EDGE('',*,*,#42101,.F.);
#54311=ORIENTED_EDGE('',*,*,#42103,.F.);
#54312=ORIENTED_EDGE('',*,*,#42104,.T.);
#54313=ORIENTED_EDGE('',*,*,#42105,.T.);
#54314=ORIENTED_EDGE('',*,*,#42106,.T.);
#54315=ORIENTED_EDGE('',*,*,#41994,.T.);
#54316=ORIENTED_EDGE('',*,*,#42107,.T.);
#54317=ORIENTED_EDGE('',*,*,#42108,.F.);
#54318=ORIENTED_EDGE('',*,*,#42109,.F.);
#54319=ORIENTED_EDGE('',*,*,#42104,.F.);
#54320=ORIENTED_EDGE('',*,*,#42071,.F.);
#54321=ORIENTED_EDGE('',*,*,#42102,.F.);
#54322=ORIENTED_EDGE('',*,*,#42109,.T.);
#54323=ORIENTED_EDGE('',*,*,#42110,.T.);
#54324=ORIENTED_EDGE('',*,*,#42072,.F.);
#54325=ORIENTED_EDGE('',*,*,#42110,.F.);
#54326=ORIENTED_EDGE('',*,*,#42111,.T.);
#54327=ORIENTED_EDGE('',*,*,#42075,.T.);
#54328=ORIENTED_EDGE('',*,*,#42073,.T.);
#54329=ORIENTED_EDGE('',*,*,#41314,.T.);
#54330=ORIENTED_EDGE('',*,*,#42108,.T.);
#54331=ORIENTED_EDGE('',*,*,#42112,.T.);
#54332=ORIENTED_EDGE('',*,*,#42111,.F.);
#54333=ORIENTED_EDGE('',*,*,#42112,.F.);
#54334=ORIENTED_EDGE('',*,*,#42113,.T.);
#54335=ORIENTED_EDGE('',*,*,#42076,.F.);
#54336=ORIENTED_EDGE('',*,*,#42113,.F.);
#54337=ORIENTED_EDGE('',*,*,#42107,.F.);
#54338=ORIENTED_EDGE('',*,*,#41993,.T.);
#54339=ORIENTED_EDGE('',*,*,#41983,.T.);
#54340=ORIENTED_EDGE('',*,*,#42086,.F.);
#54341=ORIENTED_EDGE('',*,*,#42081,.F.);
#54342=ORIENTED_EDGE('',*,*,#42078,.F.);
#54343=ORIENTED_EDGE('',*,*,#42003,.T.);
#54344=ORIENTED_EDGE('',*,*,#41995,.T.);
#54345=ORIENTED_EDGE('',*,*,#42106,.F.);
#54346=ORIENTED_EDGE('',*,*,#42114,.F.);
#54347=ORIENTED_EDGE('',*,*,#42115,.F.);
#54348=ORIENTED_EDGE('',*,*,#42116,.F.);
#54349=ORIENTED_EDGE('',*,*,#42117,.F.);
#54350=ORIENTED_EDGE('',*,*,#42118,.F.);
#54351=ORIENTED_EDGE('',*,*,#42119,.F.);
#54352=ORIENTED_EDGE('',*,*,#42120,.F.);
#54353=ORIENTED_EDGE('',*,*,#42121,.F.);
#54354=ORIENTED_EDGE('',*,*,#42122,.T.);
#54355=ORIENTED_EDGE('',*,*,#42123,.F.);
#54356=ORIENTED_EDGE('',*,*,#42124,.F.);
#54357=ORIENTED_EDGE('',*,*,#41873,.T.);
#54358=ORIENTED_EDGE('',*,*,#42124,.T.);
#54359=ORIENTED_EDGE('',*,*,#42125,.F.);
#54360=ORIENTED_EDGE('',*,*,#42126,.F.);
#54361=ORIENTED_EDGE('',*,*,#41875,.T.);
#54362=ORIENTED_EDGE('',*,*,#42127,.F.);
#54363=ORIENTED_EDGE('',*,*,#42128,.F.);
#54364=ORIENTED_EDGE('',*,*,#42129,.F.);
#54365=ORIENTED_EDGE('',*,*,#42130,.F.);
#54366=ORIENTED_EDGE('',*,*,#42114,.T.);
#54367=ORIENTED_EDGE('',*,*,#42131,.T.);
#54368=ORIENTED_EDGE('',*,*,#42132,.F.);
#54369=ORIENTED_EDGE('',*,*,#42133,.F.);
#54370=ORIENTED_EDGE('',*,*,#42130,.T.);
#54371=ORIENTED_EDGE('',*,*,#42133,.T.);
#54372=ORIENTED_EDGE('',*,*,#42134,.F.);
#54373=ORIENTED_EDGE('',*,*,#42135,.F.);
#54374=ORIENTED_EDGE('',*,*,#42115,.T.);
#54375=ORIENTED_EDGE('',*,*,#42135,.T.);
#54376=ORIENTED_EDGE('',*,*,#42136,.F.);
#54377=ORIENTED_EDGE('',*,*,#42137,.F.);
#54378=ORIENTED_EDGE('',*,*,#42116,.T.);
#54379=ORIENTED_EDGE('',*,*,#42137,.T.);
#54380=ORIENTED_EDGE('',*,*,#42138,.F.);
#54381=ORIENTED_EDGE('',*,*,#42139,.F.);
#54382=ORIENTED_EDGE('',*,*,#42117,.T.);
#54383=ORIENTED_EDGE('',*,*,#42139,.T.);
#54384=ORIENTED_EDGE('',*,*,#42140,.F.);
#54385=ORIENTED_EDGE('',*,*,#42141,.F.);
#54386=ORIENTED_EDGE('',*,*,#42118,.T.);
#54387=ORIENTED_EDGE('',*,*,#42141,.T.);
#54388=ORIENTED_EDGE('',*,*,#42142,.F.);
#54389=ORIENTED_EDGE('',*,*,#42143,.F.);
#54390=ORIENTED_EDGE('',*,*,#42119,.T.);
#54391=ORIENTED_EDGE('',*,*,#42143,.T.);
#54392=ORIENTED_EDGE('',*,*,#42144,.F.);
#54393=ORIENTED_EDGE('',*,*,#42145,.F.);
#54394=ORIENTED_EDGE('',*,*,#42120,.T.);
#54395=ORIENTED_EDGE('',*,*,#42121,.T.);
#54396=ORIENTED_EDGE('',*,*,#42145,.T.);
#54397=ORIENTED_EDGE('',*,*,#42013,.F.);
#54398=ORIENTED_EDGE('',*,*,#42146,.T.);
#54399=ORIENTED_EDGE('',*,*,#42146,.F.);
#54400=ORIENTED_EDGE('',*,*,#42007,.T.);
#54401=ORIENTED_EDGE('',*,*,#42004,.T.);
#54402=ORIENTED_EDGE('',*,*,#42014,.T.);
#54403=ORIENTED_EDGE('',*,*,#42144,.T.);
#54404=ORIENTED_EDGE('',*,*,#42147,.F.);
#54405=ORIENTED_EDGE('',*,*,#42148,.T.);
#54406=ORIENTED_EDGE('',*,*,#42009,.T.);
#54407=ORIENTED_EDGE('',*,*,#42149,.T.);
#54408=ORIENTED_EDGE('',*,*,#42148,.F.);
#54409=ORIENTED_EDGE('',*,*,#42150,.F.);
#54410=ORIENTED_EDGE('',*,*,#41976,.T.);
#54411=ORIENTED_EDGE('',*,*,#42150,.T.);
#54412=ORIENTED_EDGE('',*,*,#42151,.F.);
#54413=ORIENTED_EDGE('',*,*,#42152,.F.);
#54414=ORIENTED_EDGE('',*,*,#41977,.T.);
#54415=ORIENTED_EDGE('',*,*,#42152,.T.);
#54416=ORIENTED_EDGE('',*,*,#42153,.F.);
#54417=ORIENTED_EDGE('',*,*,#42154,.F.);
#54418=ORIENTED_EDGE('',*,*,#41978,.T.);
#54419=ORIENTED_EDGE('',*,*,#42154,.T.);
#54420=ORIENTED_EDGE('',*,*,#42155,.F.);
#54421=ORIENTED_EDGE('',*,*,#42156,.F.);
#54422=ORIENTED_EDGE('',*,*,#41979,.T.);
#54423=ORIENTED_EDGE('',*,*,#42156,.T.);
#54424=ORIENTED_EDGE('',*,*,#42157,.F.);
#54425=ORIENTED_EDGE('',*,*,#42158,.F.);
#54426=ORIENTED_EDGE('',*,*,#41980,.T.);
#54427=ORIENTED_EDGE('',*,*,#42158,.T.);
#54428=ORIENTED_EDGE('',*,*,#42159,.F.);
#54429=ORIENTED_EDGE('',*,*,#42160,.F.);
#54430=ORIENTED_EDGE('',*,*,#41981,.T.);
#54431=ORIENTED_EDGE('',*,*,#42160,.T.);
#54432=ORIENTED_EDGE('',*,*,#42161,.F.);
#54433=ORIENTED_EDGE('',*,*,#42162,.F.);
#54434=ORIENTED_EDGE('',*,*,#42163,.T.);
#54435=ORIENTED_EDGE('',*,*,#42164,.F.);
#54436=ORIENTED_EDGE('',*,*,#42087,.F.);
#54437=ORIENTED_EDGE('',*,*,#41982,.T.);
#54438=ORIENTED_EDGE('',*,*,#42163,.F.);
#54439=ORIENTED_EDGE('',*,*,#42165,.T.);
#54440=ORIENTED_EDGE('',*,*,#42166,.F.);
#54441=ORIENTED_EDGE('',*,*,#42167,.F.);
#54442=ORIENTED_EDGE('',*,*,#42168,.F.);
#54443=ORIENTED_EDGE('',*,*,#42165,.F.);
#54444=ORIENTED_EDGE('',*,*,#42169,.F.);
#54445=ORIENTED_EDGE('',*,*,#42170,.T.);
#54446=ORIENTED_EDGE('',*,*,#42171,.F.);
#54447=ORIENTED_EDGE('',*,*,#42172,.T.);
#54448=ORIENTED_EDGE('',*,*,#42170,.F.);
#54449=ORIENTED_EDGE('',*,*,#42173,.F.);
#54450=ORIENTED_EDGE('',*,*,#42172,.F.);
#54451=ORIENTED_EDGE('',*,*,#42174,.F.);
#54452=ORIENTED_EDGE('',*,*,#42175,.T.);
#54453=ORIENTED_EDGE('',*,*,#42176,.F.);
#54454=ORIENTED_EDGE('',*,*,#42175,.F.);
#54455=ORIENTED_EDGE('',*,*,#42177,.F.);
#54456=ORIENTED_EDGE('',*,*,#42178,.T.);
#54457=ORIENTED_EDGE('',*,*,#42178,.F.);
#54458=ORIENTED_EDGE('',*,*,#42179,.F.);
#54459=ORIENTED_EDGE('',*,*,#42180,.F.);
#54460=ORIENTED_EDGE('',*,*,#42181,.F.);
#54461=ORIENTED_EDGE('',*,*,#42129,.T.);
#54462=ORIENTED_EDGE('',*,*,#42182,.F.);
#54463=ORIENTED_EDGE('',*,*,#42183,.F.);
#54464=ORIENTED_EDGE('',*,*,#42184,.F.);
#54465=ORIENTED_EDGE('',*,*,#42180,.T.);
#54466=ORIENTED_EDGE('',*,*,#42185,.F.);
#54467=ORIENTED_EDGE('',*,*,#42176,.T.);
#54468=ORIENTED_EDGE('',*,*,#42184,.T.);
#54469=ORIENTED_EDGE('',*,*,#42186,.T.);
#54470=ORIENTED_EDGE('',*,*,#42187,.F.);
#54471=ORIENTED_EDGE('',*,*,#42188,.T.);
#54472=ORIENTED_EDGE('',*,*,#42095,.F.);
#54473=ORIENTED_EDGE('',*,*,#42189,.F.);
#54474=ORIENTED_EDGE('',*,*,#42187,.T.);
#54475=ORIENTED_EDGE('',*,*,#42189,.T.);
#54476=ORIENTED_EDGE('',*,*,#42094,.F.);
#54477=ORIENTED_EDGE('',*,*,#42190,.F.);
#54478=ORIENTED_EDGE('',*,*,#42191,.T.);
#54479=ORIENTED_EDGE('',*,*,#42192,.T.);
#54480=ORIENTED_EDGE('',*,*,#42166,.T.);
#54481=ORIENTED_EDGE('',*,*,#42173,.T.);
#54482=ORIENTED_EDGE('',*,*,#42185,.T.);
#54483=ORIENTED_EDGE('',*,*,#42191,.F.);
#54484=ORIENTED_EDGE('',*,*,#42193,.T.);
#54485=ORIENTED_EDGE('',*,*,#42167,.T.);
#54486=ORIENTED_EDGE('',*,*,#42192,.F.);
#54487=ORIENTED_EDGE('',*,*,#42194,.F.);
#54488=ORIENTED_EDGE('',*,*,#42190,.T.);
#54489=ORIENTED_EDGE('',*,*,#42093,.F.);
#54490=ORIENTED_EDGE('',*,*,#42195,.F.);
#54491=ORIENTED_EDGE('',*,*,#42194,.T.);
#54492=ORIENTED_EDGE('',*,*,#42195,.T.);
#54493=ORIENTED_EDGE('',*,*,#42092,.F.);
#54494=ORIENTED_EDGE('',*,*,#42090,.F.);
#54495=ORIENTED_EDGE('',*,*,#42196,.T.);
#54496=ORIENTED_EDGE('',*,*,#42088,.T.);
#54497=ORIENTED_EDGE('',*,*,#42164,.T.);
#54498=ORIENTED_EDGE('',*,*,#42168,.T.);
#54499=ORIENTED_EDGE('',*,*,#42193,.F.);
#54500=ORIENTED_EDGE('',*,*,#42196,.F.);
#54501=ORIENTED_EDGE('',*,*,#42096,.F.);
#54502=ORIENTED_EDGE('',*,*,#42188,.F.);
#54503=ORIENTED_EDGE('',*,*,#42197,.T.);
#54504=ORIENTED_EDGE('',*,*,#42198,.T.);
#54505=ORIENTED_EDGE('',*,*,#42199,.T.);
#54506=ORIENTED_EDGE('',*,*,#42097,.F.);
#54507=ORIENTED_EDGE('',*,*,#42198,.F.);
#54508=ORIENTED_EDGE('',*,*,#42200,.T.);
#54509=ORIENTED_EDGE('',*,*,#42201,.F.);
#54510=ORIENTED_EDGE('',*,*,#42182,.T.);
#54511=ORIENTED_EDGE('',*,*,#42128,.T.);
#54512=ORIENTED_EDGE('',*,*,#42202,.T.);
#54513=ORIENTED_EDGE('',*,*,#42200,.F.);
#54514=ORIENTED_EDGE('',*,*,#42202,.F.);
#54515=ORIENTED_EDGE('',*,*,#42127,.T.);
#54516=ORIENTED_EDGE('',*,*,#42105,.F.);
#54517=ORIENTED_EDGE('',*,*,#42203,.F.);
#54518=ORIENTED_EDGE('',*,*,#42204,.F.);
#54519=ORIENTED_EDGE('',*,*,#42205,.T.);
#54520=ORIENTED_EDGE('',*,*,#42098,.F.);
#54521=ORIENTED_EDGE('',*,*,#42199,.F.);
#54522=ORIENTED_EDGE('',*,*,#42204,.T.);
#54523=ORIENTED_EDGE('',*,*,#42103,.T.);
#54524=ORIENTED_EDGE('',*,*,#42100,.F.);
#54525=ORIENTED_EDGE('',*,*,#42205,.F.);
#54526=ORIENTED_EDGE('',*,*,#42203,.T.);
#54527=ORIENTED_EDGE('',*,*,#42186,.F.);
#54528=ORIENTED_EDGE('',*,*,#42183,.T.);
#54529=ORIENTED_EDGE('',*,*,#42201,.T.);
#54530=ORIENTED_EDGE('',*,*,#42197,.F.);
#54531=ORIENTED_EDGE('',*,*,#42206,.T.);
#54532=ORIENTED_EDGE('',*,*,#42207,.F.);
#54533=ORIENTED_EDGE('',*,*,#42131,.F.);
#54534=ORIENTED_EDGE('',*,*,#42181,.T.);
#54535=ORIENTED_EDGE('',*,*,#42134,.T.);
#54536=ORIENTED_EDGE('',*,*,#42132,.T.);
#54537=ORIENTED_EDGE('',*,*,#42207,.T.);
#54538=ORIENTED_EDGE('',*,*,#42208,.T.);
#54539=ORIENTED_EDGE('',*,*,#42209,.T.);
#54540=ORIENTED_EDGE('',*,*,#42210,.T.);
#54541=ORIENTED_EDGE('',*,*,#42211,.T.);
#54542=ORIENTED_EDGE('',*,*,#42212,.T.);
#54543=ORIENTED_EDGE('',*,*,#42161,.T.);
#54544=ORIENTED_EDGE('',*,*,#42159,.T.);
#54545=ORIENTED_EDGE('',*,*,#42213,.F.);
#54546=ORIENTED_EDGE('',*,*,#42157,.T.);
#54547=ORIENTED_EDGE('',*,*,#42214,.F.);
#54548=ORIENTED_EDGE('',*,*,#42136,.T.);
#54549=ORIENTED_EDGE('',*,*,#42213,.T.);
#54550=ORIENTED_EDGE('',*,*,#42215,.T.);
#54551=ORIENTED_EDGE('',*,*,#42138,.T.);
#54552=ORIENTED_EDGE('',*,*,#42214,.T.);
#54553=ORIENTED_EDGE('',*,*,#42155,.T.);
#54554=ORIENTED_EDGE('',*,*,#42216,.T.);
#54555=ORIENTED_EDGE('',*,*,#41305,.F.);
#54556=ORIENTED_EDGE('',*,*,#41307,.F.);
#54557=ORIENTED_EDGE('',*,*,#41306,.T.);
#54558=ORIENTED_EDGE('',*,*,#42216,.F.);
#54559=ORIENTED_EDGE('',*,*,#42153,.T.);
#54560=ORIENTED_EDGE('',*,*,#42217,.T.);
#54561=ORIENTED_EDGE('',*,*,#42140,.T.);
#54562=ORIENTED_EDGE('',*,*,#42215,.F.);
#54563=ORIENTED_EDGE('',*,*,#42142,.T.);
#54564=ORIENTED_EDGE('',*,*,#42217,.F.);
#54565=ORIENTED_EDGE('',*,*,#42151,.T.);
#54566=ORIENTED_EDGE('',*,*,#42147,.T.);
#54567=ORIENTED_EDGE('',*,*,#41302,.F.);
#54568=ORIENTED_EDGE('',*,*,#41303,.T.);
#54569=ORIENTED_EDGE('',*,*,#42218,.T.);
#54570=ORIENTED_EDGE('',*,*,#42219,.T.);
#54571=ORIENTED_EDGE('',*,*,#41297,.T.);
#54572=ORIENTED_EDGE('',*,*,#42220,.F.);
#54573=ORIENTED_EDGE('',*,*,#42221,.F.);
#54574=ORIENTED_EDGE('',*,*,#42222,.T.);
#54575=ORIENTED_EDGE('',*,*,#42223,.T.);
#54576=ORIENTED_EDGE('',*,*,#42224,.F.);
#54577=ORIENTED_EDGE('',*,*,#42225,.T.);
#54578=ORIENTED_EDGE('',*,*,#42219,.F.);
#54579=ORIENTED_EDGE('',*,*,#42226,.T.);
#54580=ORIENTED_EDGE('',*,*,#42226,.F.);
#54581=ORIENTED_EDGE('',*,*,#42218,.F.);
#54582=ORIENTED_EDGE('',*,*,#42225,.F.);
#54583=ORIENTED_EDGE('',*,*,#42227,.F.);
#54584=ORIENTED_EDGE('',*,*,#42228,.F.);
#54585=ORIENTED_EDGE('',*,*,#42229,.F.);
#54586=ORIENTED_EDGE('',*,*,#42230,.F.);
#54587=ORIENTED_EDGE('',*,*,#42231,.F.);
#54588=ORIENTED_EDGE('',*,*,#42232,.F.);
#54589=ORIENTED_EDGE('',*,*,#42233,.F.);
#54590=ORIENTED_EDGE('',*,*,#42220,.T.);
#54591=ORIENTED_EDGE('',*,*,#42228,.T.);
#54592=ORIENTED_EDGE('',*,*,#42224,.T.);
#54593=ORIENTED_EDGE('',*,*,#42234,.T.);
#54594=ORIENTED_EDGE('',*,*,#42235,.T.);
#54595=ORIENTED_EDGE('',*,*,#42236,.T.);
#54596=ORIENTED_EDGE('',*,*,#42237,.T.);
#54597=ORIENTED_EDGE('',*,*,#42238,.F.);
#54598=ORIENTED_EDGE('',*,*,#42227,.T.);
#54599=ORIENTED_EDGE('',*,*,#42239,.F.);
#54600=ORIENTED_EDGE('',*,*,#42240,.F.);
#54601=ORIENTED_EDGE('',*,*,#42241,.T.);
#54602=ORIENTED_EDGE('',*,*,#42233,.T.);
#54603=ORIENTED_EDGE('',*,*,#42242,.T.);
#54604=ORIENTED_EDGE('',*,*,#42221,.T.);
#54605=ORIENTED_EDGE('',*,*,#42241,.F.);
#54606=ORIENTED_EDGE('',*,*,#42243,.F.);
#54607=ORIENTED_EDGE('',*,*,#42244,.T.);
#54608=ORIENTED_EDGE('',*,*,#42245,.T.);
#54609=ORIENTED_EDGE('',*,*,#42243,.T.);
#54610=ORIENTED_EDGE('',*,*,#42240,.T.);
#54611=ORIENTED_EDGE('',*,*,#42246,.F.);
#54612=ORIENTED_EDGE('',*,*,#42247,.T.);
#54613=ORIENTED_EDGE('',*,*,#42248,.F.);
#54614=ORIENTED_EDGE('',*,*,#42249,.F.);
#54615=ORIENTED_EDGE('',*,*,#42250,.T.);
#54616=ORIENTED_EDGE('',*,*,#41946,.T.);
#54617=ORIENTED_EDGE('',*,*,#42251,.T.);
#54618=ORIENTED_EDGE('',*,*,#42242,.F.);
#54619=ORIENTED_EDGE('',*,*,#42245,.F.);
#54620=ORIENTED_EDGE('',*,*,#41937,.F.);
#54621=ORIENTED_EDGE('',*,*,#42252,.F.);
#54622=ORIENTED_EDGE('',*,*,#42253,.T.);
#54623=ORIENTED_EDGE('',*,*,#41990,.T.);
#54624=ORIENTED_EDGE('',*,*,#41988,.T.);
#54625=ORIENTED_EDGE('',*,*,#42254,.F.);
#54626=ORIENTED_EDGE('',*,*,#41924,.T.);
#54627=ORIENTED_EDGE('',*,*,#41929,.T.);
#54628=ORIENTED_EDGE('',*,*,#42255,.T.);
#54629=ORIENTED_EDGE('',*,*,#42256,.T.);
#54630=ORIENTED_EDGE('',*,*,#42222,.F.);
#54631=ORIENTED_EDGE('',*,*,#42251,.F.);
#54632=ORIENTED_EDGE('',*,*,#41945,.F.);
#54633=ORIENTED_EDGE('',*,*,#41939,.F.);
#54634=ORIENTED_EDGE('',*,*,#42257,.T.);
#54635=ORIENTED_EDGE('',*,*,#41934,.T.);
#54636=ORIENTED_EDGE('',*,*,#42246,.T.);
#54637=ORIENTED_EDGE('',*,*,#42258,.F.);
#54638=ORIENTED_EDGE('',*,*,#42256,.F.);
#54639=ORIENTED_EDGE('',*,*,#42258,.T.);
#54640=ORIENTED_EDGE('',*,*,#42249,.T.);
#54641=ORIENTED_EDGE('',*,*,#42259,.F.);
#54642=ORIENTED_EDGE('',*,*,#42223,.F.);
#54643=ORIENTED_EDGE('',*,*,#42259,.T.);
#54644=ORIENTED_EDGE('',*,*,#42248,.T.);
#54645=ORIENTED_EDGE('',*,*,#42260,.F.);
#54646=ORIENTED_EDGE('',*,*,#42234,.F.);
#54647=ORIENTED_EDGE('',*,*,#42260,.T.);
#54648=ORIENTED_EDGE('',*,*,#42261,.T.);
#54649=ORIENTED_EDGE('',*,*,#42262,.F.);
#54650=ORIENTED_EDGE('',*,*,#42235,.F.);
#54651=ORIENTED_EDGE('',*,*,#42262,.T.);
#54652=ORIENTED_EDGE('',*,*,#42263,.T.);
#54653=ORIENTED_EDGE('',*,*,#42264,.F.);
#54654=ORIENTED_EDGE('',*,*,#42236,.F.);
#54655=ORIENTED_EDGE('',*,*,#42264,.T.);
#54656=ORIENTED_EDGE('',*,*,#41228,.T.);
#54657=ORIENTED_EDGE('',*,*,#42265,.F.);
#54658=ORIENTED_EDGE('',*,*,#42237,.F.);
#54659=ORIENTED_EDGE('',*,*,#42266,.F.);
#54660=ORIENTED_EDGE('',*,*,#42265,.T.);
#54661=ORIENTED_EDGE('',*,*,#41227,.T.);
#54662=ORIENTED_EDGE('',*,*,#42267,.F.);
#54663=ORIENTED_EDGE('',*,*,#42268,.F.);
#54664=ORIENTED_EDGE('',*,*,#42267,.T.);
#54665=ORIENTED_EDGE('',*,*,#42269,.T.);
#54666=ORIENTED_EDGE('',*,*,#41226,.F.);
#54667=ORIENTED_EDGE('',*,*,#42270,.F.);
#54668=ORIENTED_EDGE('',*,*,#42269,.F.);
#54669=ORIENTED_EDGE('',*,*,#42270,.T.);
#54670=ORIENTED_EDGE('',*,*,#42271,.F.);
#54671=ORIENTED_EDGE('',*,*,#42272,.T.);
#54672=ORIENTED_EDGE('',*,*,#42273,.T.);
#54673=ORIENTED_EDGE('',*,*,#42274,.T.);
#54674=ORIENTED_EDGE('',*,*,#42275,.T.);
#54675=ORIENTED_EDGE('',*,*,#42276,.T.);
#54676=ORIENTED_EDGE('',*,*,#42277,.T.);
#54677=ORIENTED_EDGE('',*,*,#42278,.T.);
#54678=ORIENTED_EDGE('',*,*,#42279,.F.);
#54679=ORIENTED_EDGE('',*,*,#42280,.T.);
#54680=ORIENTED_EDGE('',*,*,#42281,.T.);
#54681=ORIENTED_EDGE('',*,*,#42238,.T.);
#54682=ORIENTED_EDGE('',*,*,#42266,.T.);
#54683=ORIENTED_EDGE('',*,*,#42268,.T.);
#54684=ORIENTED_EDGE('',*,*,#42281,.F.);
#54685=ORIENTED_EDGE('',*,*,#42282,.F.);
#54686=ORIENTED_EDGE('',*,*,#42283,.F.);
#54687=ORIENTED_EDGE('',*,*,#42229,.T.);
#54688=ORIENTED_EDGE('',*,*,#42284,.T.);
#54689=ORIENTED_EDGE('',*,*,#42283,.T.);
#54690=ORIENTED_EDGE('',*,*,#42285,.F.);
#54691=ORIENTED_EDGE('',*,*,#42286,.F.);
#54692=ORIENTED_EDGE('',*,*,#42287,.F.);
#54693=ORIENTED_EDGE('',*,*,#42288,.T.);
#54694=ORIENTED_EDGE('',*,*,#42289,.T.);
#54695=ORIENTED_EDGE('',*,*,#42290,.T.);
#54696=ORIENTED_EDGE('',*,*,#42286,.T.);
#54697=ORIENTED_EDGE('',*,*,#42291,.T.);
#54698=ORIENTED_EDGE('',*,*,#42230,.T.);
#54699=ORIENTED_EDGE('',*,*,#42284,.F.);
#54700=ORIENTED_EDGE('',*,*,#42290,.F.);
#54701=ORIENTED_EDGE('',*,*,#42292,.T.);
#54702=ORIENTED_EDGE('',*,*,#42231,.T.);
#54703=ORIENTED_EDGE('',*,*,#42291,.F.);
#54704=ORIENTED_EDGE('',*,*,#42293,.F.);
#54705=ORIENTED_EDGE('',*,*,#42289,.F.);
#54706=ORIENTED_EDGE('',*,*,#42294,.T.);
#54707=ORIENTED_EDGE('',*,*,#42295,.T.);
#54708=ORIENTED_EDGE('',*,*,#42293,.T.);
#54709=ORIENTED_EDGE('',*,*,#42244,.F.);
#54710=ORIENTED_EDGE('',*,*,#42296,.T.);
#54711=ORIENTED_EDGE('',*,*,#42295,.F.);
#54712=ORIENTED_EDGE('',*,*,#42297,.T.);
#54713=ORIENTED_EDGE('',*,*,#41936,.T.);
#54714=ORIENTED_EDGE('',*,*,#41938,.T.);
#54715=ORIENTED_EDGE('',*,*,#41942,.T.);
#54716=ORIENTED_EDGE('',*,*,#41944,.T.);
#54717=ORIENTED_EDGE('',*,*,#42298,.T.);
#54718=ORIENTED_EDGE('',*,*,#42298,.F.);
#54719=ORIENTED_EDGE('',*,*,#41947,.T.);
#54720=ORIENTED_EDGE('',*,*,#42250,.F.);
#54721=ORIENTED_EDGE('',*,*,#42299,.F.);
#54722=ORIENTED_EDGE('',*,*,#42125,.T.);
#54723=ORIENTED_EDGE('',*,*,#42123,.T.);
#54724=ORIENTED_EDGE('',*,*,#42252,.T.);
#54725=ORIENTED_EDGE('',*,*,#42297,.F.);
#54726=ORIENTED_EDGE('',*,*,#42300,.T.);
#54727=ORIENTED_EDGE('',*,*,#42301,.T.);
#54728=ORIENTED_EDGE('',*,*,#42299,.T.);
#54729=ORIENTED_EDGE('',*,*,#42294,.F.);
#54730=ORIENTED_EDGE('',*,*,#42302,.T.);
#54731=ORIENTED_EDGE('',*,*,#42303,.T.);
#54732=ORIENTED_EDGE('',*,*,#42304,.T.);
#54733=ORIENTED_EDGE('',*,*,#42305,.F.);
#54734=ORIENTED_EDGE('',*,*,#42126,.T.);
#54735=ORIENTED_EDGE('',*,*,#42301,.F.);
#54736=ORIENTED_EDGE('',*,*,#42306,.F.);
#54737=ORIENTED_EDGE('',*,*,#41876,.T.);
#54738=ORIENTED_EDGE('',*,*,#42307,.F.);
#54739=ORIENTED_EDGE('',*,*,#42308,.F.);
#54740=ORIENTED_EDGE('',*,*,#42306,.T.);
#54741=ORIENTED_EDGE('',*,*,#42308,.T.);
#54742=ORIENTED_EDGE('',*,*,#42278,.F.);
#54743=ORIENTED_EDGE('',*,*,#42309,.F.);
#54744=ORIENTED_EDGE('',*,*,#41877,.T.);
#54745=ORIENTED_EDGE('',*,*,#42309,.T.);
#54746=ORIENTED_EDGE('',*,*,#42277,.F.);
#54747=ORIENTED_EDGE('',*,*,#42310,.F.);
#54748=ORIENTED_EDGE('',*,*,#42311,.T.);
#54749=ORIENTED_EDGE('',*,*,#42312,.F.);
#54750=ORIENTED_EDGE('',*,*,#41878,.F.);
#54751=ORIENTED_EDGE('',*,*,#42311,.F.);
#54752=ORIENTED_EDGE('',*,*,#42313,.T.);
#54753=ORIENTED_EDGE('',*,*,#42314,.F.);
#54754=ORIENTED_EDGE('',*,*,#42315,.T.);
#54755=ORIENTED_EDGE('',*,*,#42316,.F.);
#54756=ORIENTED_EDGE('',*,*,#42317,.F.);
#54757=ORIENTED_EDGE('',*,*,#42314,.T.);
#54758=ORIENTED_EDGE('',*,*,#42317,.T.);
#54759=ORIENTED_EDGE('',*,*,#42318,.F.);
#54760=ORIENTED_EDGE('',*,*,#42319,.F.);
#54761=ORIENTED_EDGE('',*,*,#42320,.T.);
#54762=ORIENTED_EDGE('',*,*,#42321,.F.);
#54763=ORIENTED_EDGE('',*,*,#42322,.F.);
#54764=ORIENTED_EDGE('',*,*,#42312,.T.);
#54765=ORIENTED_EDGE('',*,*,#42320,.F.);
#54766=ORIENTED_EDGE('',*,*,#42322,.T.);
#54767=ORIENTED_EDGE('',*,*,#42323,.T.);
#54768=ORIENTED_EDGE('',*,*,#42324,.T.);
#54769=ORIENTED_EDGE('',*,*,#41884,.F.);
#54770=ORIENTED_EDGE('',*,*,#41907,.F.);
#54771=ORIENTED_EDGE('',*,*,#41891,.F.);
#54772=ORIENTED_EDGE('',*,*,#41879,.T.);
#54773=ORIENTED_EDGE('',*,*,#42325,.T.);
#54774=ORIENTED_EDGE('',*,*,#42326,.T.);
#54775=ORIENTED_EDGE('',*,*,#41893,.T.);
#54776=ORIENTED_EDGE('',*,*,#42327,.T.);
#54777=ORIENTED_EDGE('',*,*,#42328,.F.);
#54778=ORIENTED_EDGE('',*,*,#41289,.F.);
#54779=ORIENTED_EDGE('',*,*,#41287,.F.);
#54780=ORIENTED_EDGE('',*,*,#41291,.T.);
#54781=ORIENTED_EDGE('',*,*,#41852,.F.);
#54782=ORIENTED_EDGE('',*,*,#42329,.F.);
#54783=ORIENTED_EDGE('',*,*,#42330,.T.);
#54784=ORIENTED_EDGE('',*,*,#42331,.T.);
#54785=ORIENTED_EDGE('',*,*,#42325,.F.);
#54786=ORIENTED_EDGE('',*,*,#42330,.F.);
#54787=ORIENTED_EDGE('',*,*,#42332,.F.);
#54788=ORIENTED_EDGE('',*,*,#42333,.T.);
#54789=ORIENTED_EDGE('',*,*,#42334,.F.);
#54790=ORIENTED_EDGE('',*,*,#42335,.F.);
#54791=ORIENTED_EDGE('',*,*,#42336,.F.);
#54792=ORIENTED_EDGE('',*,*,#42331,.F.);
#54793=ORIENTED_EDGE('',*,*,#42337,.F.);
#54794=ORIENTED_EDGE('',*,*,#41851,.F.);
#54795=ORIENTED_EDGE('',*,*,#42338,.T.);
#54796=ORIENTED_EDGE('',*,*,#42337,.T.);
#54797=ORIENTED_EDGE('',*,*,#42329,.T.);
#54798=ORIENTED_EDGE('',*,*,#42339,.F.);
#54799=ORIENTED_EDGE('',*,*,#41894,.F.);
#54800=ORIENTED_EDGE('',*,*,#42326,.F.);
#54801=ORIENTED_EDGE('',*,*,#42336,.T.);
#54802=ORIENTED_EDGE('',*,*,#42340,.T.);
#54803=ORIENTED_EDGE('',*,*,#41870,.T.);
#54804=ORIENTED_EDGE('',*,*,#42341,.F.);
#54805=ORIENTED_EDGE('',*,*,#42342,.T.);
#54806=ORIENTED_EDGE('',*,*,#42343,.F.);
#54807=ORIENTED_EDGE('',*,*,#42344,.F.);
#54808=ORIENTED_EDGE('',*,*,#42341,.T.);
#54809=ORIENTED_EDGE('',*,*,#42344,.T.);
#54810=ORIENTED_EDGE('',*,*,#42345,.F.);
#54811=ORIENTED_EDGE('',*,*,#42346,.F.);
#54812=ORIENTED_EDGE('',*,*,#42347,.T.);
#54813=ORIENTED_EDGE('',*,*,#42348,.T.);
#54814=ORIENTED_EDGE('',*,*,#41997,.T.);
#54815=ORIENTED_EDGE('',*,*,#42340,.F.);
#54816=ORIENTED_EDGE('',*,*,#42347,.F.);
#54817=ORIENTED_EDGE('',*,*,#42349,.T.);
#54818=ORIENTED_EDGE('',*,*,#42350,.T.);
#54819=ORIENTED_EDGE('',*,*,#42351,.T.);
#54820=ORIENTED_EDGE('',*,*,#42352,.T.);
#54821=ORIENTED_EDGE('',*,*,#42353,.T.);
#54822=ORIENTED_EDGE('',*,*,#42354,.T.);
#54823=ORIENTED_EDGE('',*,*,#41408,.T.);
#54824=ORIENTED_EDGE('',*,*,#42354,.F.);
#54825=ORIENTED_EDGE('',*,*,#42355,.T.);
#54826=ORIENTED_EDGE('',*,*,#42356,.F.);
#54827=ORIENTED_EDGE('',*,*,#42357,.F.);
#54828=ORIENTED_EDGE('',*,*,#42358,.F.);
#54829=ORIENTED_EDGE('',*,*,#42357,.T.);
#54830=ORIENTED_EDGE('',*,*,#42359,.F.);
#54831=ORIENTED_EDGE('',*,*,#42360,.T.);
#54832=ORIENTED_EDGE('',*,*,#42361,.F.);
#54833=ORIENTED_EDGE('',*,*,#42362,.T.);
#54834=ORIENTED_EDGE('',*,*,#42363,.T.);
#54835=ORIENTED_EDGE('',*,*,#42360,.F.);
#54836=ORIENTED_EDGE('',*,*,#42358,.T.);
#54837=ORIENTED_EDGE('',*,*,#42363,.F.);
#54838=ORIENTED_EDGE('',*,*,#42364,.T.);
#54839=ORIENTED_EDGE('',*,*,#42349,.F.);
#54840=ORIENTED_EDGE('',*,*,#41284,.F.);
#54841=ORIENTED_EDGE('',*,*,#42365,.T.);
#54842=ORIENTED_EDGE('',*,*,#42364,.F.);
#54843=ORIENTED_EDGE('',*,*,#42362,.F.);
#54844=ORIENTED_EDGE('',*,*,#41283,.F.);
#54845=ORIENTED_EDGE('',*,*,#41282,.F.);
#54846=ORIENTED_EDGE('',*,*,#42366,.T.);
#54847=ORIENTED_EDGE('',*,*,#42350,.F.);
#54848=ORIENTED_EDGE('',*,*,#42365,.F.);
#54849=ORIENTED_EDGE('',*,*,#41281,.F.);
#54850=ORIENTED_EDGE('',*,*,#42367,.T.);
#54851=ORIENTED_EDGE('',*,*,#42368,.F.);
#54852=ORIENTED_EDGE('',*,*,#42366,.F.);
#54853=ORIENTED_EDGE('',*,*,#42369,.T.);
#54854=ORIENTED_EDGE('',*,*,#42351,.F.);
#54855=ORIENTED_EDGE('',*,*,#42368,.T.);
#54856=ORIENTED_EDGE('',*,*,#42370,.F.);
#54857=ORIENTED_EDGE('',*,*,#42370,.T.);
#54858=ORIENTED_EDGE('',*,*,#42367,.F.);
#54859=ORIENTED_EDGE('',*,*,#42371,.F.);
#54860=ORIENTED_EDGE('',*,*,#42372,.F.);
#54861=ORIENTED_EDGE('',*,*,#42369,.F.);
#54862=ORIENTED_EDGE('',*,*,#42372,.T.);
#54863=ORIENTED_EDGE('',*,*,#42373,.F.);
#54864=ORIENTED_EDGE('',*,*,#42374,.F.);
#54865=ORIENTED_EDGE('',*,*,#42352,.F.);
#54866=ORIENTED_EDGE('',*,*,#42374,.T.);
#54867=ORIENTED_EDGE('',*,*,#42375,.F.);
#54868=ORIENTED_EDGE('',*,*,#42376,.F.);
#54869=ORIENTED_EDGE('',*,*,#42353,.F.);
#54870=ORIENTED_EDGE('',*,*,#42376,.T.);
#54871=ORIENTED_EDGE('',*,*,#42377,.F.);
#54872=ORIENTED_EDGE('',*,*,#42378,.F.);
#54873=ORIENTED_EDGE('',*,*,#42355,.F.);
#54874=ORIENTED_EDGE('',*,*,#42378,.T.);
#54875=ORIENTED_EDGE('',*,*,#42377,.T.);
#54876=ORIENTED_EDGE('',*,*,#42379,.T.);
#54877=ORIENTED_EDGE('',*,*,#42380,.F.);
#54878=ORIENTED_EDGE('',*,*,#42381,.F.);
#54879=ORIENTED_EDGE('',*,*,#42382,.F.);
#54880=ORIENTED_EDGE('',*,*,#42383,.T.);
#54881=ORIENTED_EDGE('',*,*,#42359,.T.);
#54882=ORIENTED_EDGE('',*,*,#42356,.T.);
#54883=ORIENTED_EDGE('',*,*,#42383,.F.);
#54884=ORIENTED_EDGE('',*,*,#42384,.F.);
#54885=ORIENTED_EDGE('',*,*,#42385,.T.);
#54886=ORIENTED_EDGE('',*,*,#41285,.T.);
#54887=ORIENTED_EDGE('',*,*,#42361,.T.);
#54888=ORIENTED_EDGE('',*,*,#42384,.T.);
#54889=ORIENTED_EDGE('',*,*,#42386,.F.);
#54890=ORIENTED_EDGE('',*,*,#42387,.F.);
#54891=ORIENTED_EDGE('',*,*,#42388,.T.);
#54892=ORIENTED_EDGE('',*,*,#42389,.F.);
#54893=ORIENTED_EDGE('',*,*,#42390,.F.);
#54894=ORIENTED_EDGE('',*,*,#42391,.T.);
#54895=ORIENTED_EDGE('',*,*,#42392,.T.);
#54896=ORIENTED_EDGE('',*,*,#42393,.T.);
#54897=ORIENTED_EDGE('',*,*,#42391,.F.);
#54898=ORIENTED_EDGE('',*,*,#42394,.F.);
#54899=ORIENTED_EDGE('',*,*,#42395,.T.);
#54900=ORIENTED_EDGE('',*,*,#42396,.T.);
#54901=ORIENTED_EDGE('',*,*,#42394,.T.);
#54902=ORIENTED_EDGE('',*,*,#42397,.F.);
#54903=ORIENTED_EDGE('',*,*,#42398,.F.);
#54904=ORIENTED_EDGE('',*,*,#42399,.F.);
#54905=ORIENTED_EDGE('',*,*,#42400,.T.);
#54906=ORIENTED_EDGE('',*,*,#42401,.T.);
#54907=ORIENTED_EDGE('',*,*,#42402,.T.);
#54908=ORIENTED_EDGE('',*,*,#42400,.F.);
#54909=ORIENTED_EDGE('',*,*,#42403,.F.);
#54910=ORIENTED_EDGE('',*,*,#42404,.T.);
#54911=ORIENTED_EDGE('',*,*,#42403,.T.);
#54912=ORIENTED_EDGE('',*,*,#42405,.F.);
#54913=ORIENTED_EDGE('',*,*,#42406,.T.);
#54914=ORIENTED_EDGE('',*,*,#42407,.T.);
#54915=ORIENTED_EDGE('',*,*,#42408,.F.);
#54916=ORIENTED_EDGE('',*,*,#42409,.T.);
#54917=ORIENTED_EDGE('',*,*,#42410,.T.);
#54918=ORIENTED_EDGE('',*,*,#42411,.F.);
#54919=ORIENTED_EDGE('',*,*,#42412,.T.);
#54920=ORIENTED_EDGE('',*,*,#42371,.T.);
#54921=ORIENTED_EDGE('',*,*,#41280,.T.);
#54922=ORIENTED_EDGE('',*,*,#41279,.F.);
#54923=ORIENTED_EDGE('',*,*,#42413,.T.);
#54924=ORIENTED_EDGE('',*,*,#42414,.F.);
#54925=ORIENTED_EDGE('',*,*,#42415,.F.);
#54926=ORIENTED_EDGE('',*,*,#42404,.F.);
#54927=ORIENTED_EDGE('',*,*,#42415,.T.);
#54928=ORIENTED_EDGE('',*,*,#42416,.T.);
#54929=ORIENTED_EDGE('',*,*,#42417,.F.);
#54930=ORIENTED_EDGE('',*,*,#42418,.F.);
#54931=ORIENTED_EDGE('',*,*,#42419,.T.);
#54932=ORIENTED_EDGE('',*,*,#42401,.F.);
#54933=ORIENTED_EDGE('',*,*,#42417,.T.);
#54934=ORIENTED_EDGE('',*,*,#42420,.F.);
#54935=ORIENTED_EDGE('',*,*,#42421,.T.);
#54936=ORIENTED_EDGE('',*,*,#42402,.F.);
#54937=ORIENTED_EDGE('',*,*,#42419,.F.);
#54938=ORIENTED_EDGE('',*,*,#42422,.F.);
#54939=ORIENTED_EDGE('',*,*,#42423,.T.);
#54940=ORIENTED_EDGE('',*,*,#42396,.F.);
#54941=ORIENTED_EDGE('',*,*,#42395,.F.);
#54942=ORIENTED_EDGE('',*,*,#42421,.F.);
#54943=ORIENTED_EDGE('',*,*,#42424,.F.);
#54944=ORIENTED_EDGE('',*,*,#42425,.T.);
#54945=ORIENTED_EDGE('',*,*,#42392,.F.);
#54946=ORIENTED_EDGE('',*,*,#42423,.F.);
#54947=ORIENTED_EDGE('',*,*,#42426,.F.);
#54948=ORIENTED_EDGE('',*,*,#42427,.T.);
#54949=ORIENTED_EDGE('',*,*,#42393,.F.);
#54950=ORIENTED_EDGE('',*,*,#42425,.F.);
#54951=ORIENTED_EDGE('',*,*,#42428,.T.);
#54952=ORIENTED_EDGE('',*,*,#42429,.F.);
#54953=ORIENTED_EDGE('',*,*,#42385,.F.);
#54954=ORIENTED_EDGE('',*,*,#42427,.F.);
#54955=ORIENTED_EDGE('',*,*,#41286,.F.);
#54956=ORIENTED_EDGE('',*,*,#42429,.T.);
#54957=ORIENTED_EDGE('',*,*,#42430,.F.);
#54958=ORIENTED_EDGE('',*,*,#42431,.F.);
#54959=ORIENTED_EDGE('',*,*,#41278,.F.);
#54960=ORIENTED_EDGE('',*,*,#41277,.F.);
#54961=ORIENTED_EDGE('',*,*,#42431,.T.);
#54962=ORIENTED_EDGE('',*,*,#42432,.F.);
#54963=ORIENTED_EDGE('',*,*,#42413,.F.);
#54964=ORIENTED_EDGE('',*,*,#42424,.T.);
#54965=ORIENTED_EDGE('',*,*,#42422,.T.);
#54966=ORIENTED_EDGE('',*,*,#42420,.T.);
#54967=ORIENTED_EDGE('',*,*,#42433,.T.);
#54968=ORIENTED_EDGE('',*,*,#42432,.T.);
#54969=ORIENTED_EDGE('',*,*,#42434,.T.);
#54970=ORIENTED_EDGE('',*,*,#41470,.T.);
#54971=ORIENTED_EDGE('',*,*,#42426,.T.);
#54972=ORIENTED_EDGE('',*,*,#42434,.F.);
#54973=ORIENTED_EDGE('',*,*,#42430,.T.);
#54974=ORIENTED_EDGE('',*,*,#42428,.F.);
#54975=ORIENTED_EDGE('',*,*,#42418,.T.);
#54976=ORIENTED_EDGE('',*,*,#42416,.F.);
#54977=ORIENTED_EDGE('',*,*,#42414,.T.);
#54978=ORIENTED_EDGE('',*,*,#42433,.F.);
#54979=ORIENTED_EDGE('',*,*,#42375,.T.);
#54980=ORIENTED_EDGE('',*,*,#42373,.T.);
#54981=ORIENTED_EDGE('',*,*,#42412,.F.);
#54982=ORIENTED_EDGE('',*,*,#42379,.F.);
#54983=ORIENTED_EDGE('',*,*,#42435,.F.);
#54984=ORIENTED_EDGE('',*,*,#42380,.T.);
#54985=ORIENTED_EDGE('',*,*,#42411,.T.);
#54986=ORIENTED_EDGE('',*,*,#42436,.F.);
#54987=ORIENTED_EDGE('',*,*,#42437,.F.);
#54988=ORIENTED_EDGE('',*,*,#42436,.T.);
#54989=ORIENTED_EDGE('',*,*,#42438,.T.);
#54990=ORIENTED_EDGE('',*,*,#41275,.F.);
#54991=ORIENTED_EDGE('',*,*,#42439,.T.);
#54992=ORIENTED_EDGE('',*,*,#42440,.T.);
#54993=ORIENTED_EDGE('',*,*,#42441,.F.);
#54994=ORIENTED_EDGE('',*,*,#41276,.F.);
#54995=ORIENTED_EDGE('',*,*,#42381,.T.);
#54996=ORIENTED_EDGE('',*,*,#42435,.T.);
#54997=ORIENTED_EDGE('',*,*,#42437,.T.);
#54998=ORIENTED_EDGE('',*,*,#41274,.T.);
#54999=ORIENTED_EDGE('',*,*,#42441,.T.);
#55000=ORIENTED_EDGE('',*,*,#42442,.T.);
#55001=ORIENTED_EDGE('',*,*,#42386,.T.);
#55002=ORIENTED_EDGE('',*,*,#42382,.T.);
#55003=ORIENTED_EDGE('',*,*,#42442,.F.);
#55004=ORIENTED_EDGE('',*,*,#42440,.F.);
#55005=ORIENTED_EDGE('',*,*,#42439,.F.);
#55006=ORIENTED_EDGE('',*,*,#41224,.F.);
#55007=ORIENTED_EDGE('',*,*,#42443,.T.);
#55008=ORIENTED_EDGE('',*,*,#42387,.T.);
#55009=ORIENTED_EDGE('',*,*,#41255,.T.);
#55010=ORIENTED_EDGE('',*,*,#42444,.T.);
#55011=ORIENTED_EDGE('',*,*,#42443,.F.);
#55012=ORIENTED_EDGE('',*,*,#42445,.F.);
#55013=ORIENTED_EDGE('',*,*,#41256,.F.);
#55014=ORIENTED_EDGE('',*,*,#42445,.T.);
#55015=ORIENTED_EDGE('',*,*,#41223,.T.);
#55016=ORIENTED_EDGE('',*,*,#41222,.T.);
#55017=ORIENTED_EDGE('',*,*,#42446,.F.);
#55018=ORIENTED_EDGE('',*,*,#41257,.F.);
#55019=ORIENTED_EDGE('',*,*,#42446,.T.);
#55020=ORIENTED_EDGE('',*,*,#42447,.F.);
#55021=ORIENTED_EDGE('',*,*,#42448,.F.);
#55022=ORIENTED_EDGE('',*,*,#42449,.F.);
#55023=ORIENTED_EDGE('',*,*,#42448,.T.);
#55024=ORIENTED_EDGE('',*,*,#42450,.F.);
#55025=ORIENTED_EDGE('',*,*,#42451,.F.);
#55026=ORIENTED_EDGE('',*,*,#42452,.T.);
#55027=ORIENTED_EDGE('',*,*,#42451,.T.);
#55028=ORIENTED_EDGE('',*,*,#42409,.F.);
#55029=ORIENTED_EDGE('',*,*,#42453,.T.);
#55030=ORIENTED_EDGE('',*,*,#41258,.F.);
#55031=ORIENTED_EDGE('',*,*,#42449,.T.);
#55032=ORIENTED_EDGE('',*,*,#42452,.F.);
#55033=ORIENTED_EDGE('',*,*,#42454,.T.);
#55034=ORIENTED_EDGE('',*,*,#42455,.T.);
#55035=ORIENTED_EDGE('',*,*,#42456,.F.);
#55036=ORIENTED_EDGE('',*,*,#42457,.T.);
#55037=ORIENTED_EDGE('',*,*,#41269,.T.);
#55038=ORIENTED_EDGE('',*,*,#41254,.F.);
#55039=ORIENTED_EDGE('',*,*,#41273,.F.);
#55040=ORIENTED_EDGE('',*,*,#42458,.T.);
#55041=ORIENTED_EDGE('',*,*,#42388,.F.);
#55042=ORIENTED_EDGE('',*,*,#42444,.F.);
#55043=ORIENTED_EDGE('',*,*,#41272,.T.);
#55044=ORIENTED_EDGE('',*,*,#42459,.T.);
#55045=ORIENTED_EDGE('',*,*,#42460,.F.);
#55046=ORIENTED_EDGE('',*,*,#42458,.F.);
#55047=ORIENTED_EDGE('',*,*,#42461,.F.);
#55048=ORIENTED_EDGE('',*,*,#42389,.T.);
#55049=ORIENTED_EDGE('',*,*,#42460,.T.);
#55050=ORIENTED_EDGE('',*,*,#41253,.F.);
#55051=ORIENTED_EDGE('',*,*,#42462,.F.);
#55052=ORIENTED_EDGE('',*,*,#41252,.T.);
#55053=ORIENTED_EDGE('',*,*,#42463,.T.);
#55054=ORIENTED_EDGE('',*,*,#42464,.F.);
#55055=ORIENTED_EDGE('',*,*,#42406,.F.);
#55056=ORIENTED_EDGE('',*,*,#42457,.F.);
#55057=ORIENTED_EDGE('',*,*,#42465,.T.);
#55058=ORIENTED_EDGE('',*,*,#42464,.T.);
#55059=ORIENTED_EDGE('',*,*,#42466,.F.);
#55060=ORIENTED_EDGE('',*,*,#41270,.F.);
#55061=ORIENTED_EDGE('',*,*,#42466,.T.);
#55062=ORIENTED_EDGE('',*,*,#42463,.F.);
#55063=ORIENTED_EDGE('',*,*,#42467,.F.);
#55064=ORIENTED_EDGE('',*,*,#41271,.F.);
#55065=ORIENTED_EDGE('',*,*,#42467,.T.);
#55066=ORIENTED_EDGE('',*,*,#41251,.T.);
#55067=ORIENTED_EDGE('',*,*,#41250,.T.);
#55068=ORIENTED_EDGE('',*,*,#42459,.F.);
#55069=ORIENTED_EDGE('',*,*,#42456,.T.);
#55070=ORIENTED_EDGE('',*,*,#42407,.F.);
#55071=ORIENTED_EDGE('',*,*,#42465,.F.);
#55072=ORIENTED_EDGE('',*,*,#42462,.T.);
#55073=ORIENTED_EDGE('',*,*,#42468,.T.);
#55074=ORIENTED_EDGE('',*,*,#42469,.F.);
#55075=ORIENTED_EDGE('',*,*,#41247,.F.);
#55076=ORIENTED_EDGE('',*,*,#42470,.F.);
#55077=ORIENTED_EDGE('',*,*,#42471,.T.);
#55078=ORIENTED_EDGE('',*,*,#42461,.T.);
#55079=ORIENTED_EDGE('',*,*,#41249,.F.);
#55080=ORIENTED_EDGE('',*,*,#42472,.F.);
#55081=ORIENTED_EDGE('',*,*,#42397,.T.);
#55082=ORIENTED_EDGE('',*,*,#42390,.T.);
#55083=ORIENTED_EDGE('',*,*,#42471,.F.);
#55084=ORIENTED_EDGE('',*,*,#42398,.T.);
#55085=ORIENTED_EDGE('',*,*,#42472,.T.);
#55086=ORIENTED_EDGE('',*,*,#42470,.T.);
#55087=ORIENTED_EDGE('',*,*,#41248,.T.);
#55088=ORIENTED_EDGE('',*,*,#42469,.T.);
#55089=ORIENTED_EDGE('',*,*,#42473,.T.);
#55090=ORIENTED_EDGE('',*,*,#42405,.T.);
#55091=ORIENTED_EDGE('',*,*,#42399,.T.);
#55092=ORIENTED_EDGE('',*,*,#42473,.F.);
#55093=ORIENTED_EDGE('',*,*,#42468,.F.);
#55094=ORIENTED_EDGE('',*,*,#41264,.T.);
#55095=ORIENTED_EDGE('',*,*,#41194,.F.);
#55096=ORIENTED_EDGE('',*,*,#42474,.F.);
#55097=ORIENTED_EDGE('',*,*,#42059,.T.);
#55098=ORIENTED_EDGE('',*,*,#41259,.F.);
#55099=ORIENTED_EDGE('',*,*,#42475,.F.);
#55100=ORIENTED_EDGE('',*,*,#42476,.F.);
#55101=ORIENTED_EDGE('',*,*,#42475,.T.);
#55102=ORIENTED_EDGE('',*,*,#42453,.F.);
#55103=ORIENTED_EDGE('',*,*,#42477,.F.);
#55104=ORIENTED_EDGE('',*,*,#42478,.F.);
#55105=ORIENTED_EDGE('',*,*,#42477,.T.);
#55106=ORIENTED_EDGE('',*,*,#41268,.F.);
#55107=ORIENTED_EDGE('',*,*,#42054,.F.);
#55108=ORIENTED_EDGE('',*,*,#42474,.T.);
#55109=ORIENTED_EDGE('',*,*,#42476,.T.);
#55110=ORIENTED_EDGE('',*,*,#42478,.T.);
#55111=ORIENTED_EDGE('',*,*,#42052,.T.);
#55112=ORIENTED_EDGE('',*,*,#42479,.T.);
#55113=ORIENTED_EDGE('',*,*,#42480,.T.);
#55114=ORIENTED_EDGE('',*,*,#42481,.T.);
#55115=ORIENTED_EDGE('',*,*,#42061,.F.);
#55116=ORIENTED_EDGE('',*,*,#42481,.F.);
#55117=ORIENTED_EDGE('',*,*,#42482,.T.);
#55118=ORIENTED_EDGE('',*,*,#42483,.F.);
#55119=ORIENTED_EDGE('',*,*,#42484,.F.);
#55120=ORIENTED_EDGE('',*,*,#42062,.F.);
#55121=ORIENTED_EDGE('',*,*,#42484,.T.);
#55122=ORIENTED_EDGE('',*,*,#42485,.F.);
#55123=ORIENTED_EDGE('',*,*,#42486,.F.);
#55124=ORIENTED_EDGE('',*,*,#42487,.F.);
#55125=ORIENTED_EDGE('',*,*,#42488,.T.);
#55126=ORIENTED_EDGE('',*,*,#42489,.F.);
#55127=ORIENTED_EDGE('',*,*,#42486,.T.);
#55128=ORIENTED_EDGE('',*,*,#42489,.T.);
#55129=ORIENTED_EDGE('',*,*,#42490,.T.);
#55130=ORIENTED_EDGE('',*,*,#42065,.T.);
#55131=ORIENTED_EDGE('',*,*,#42063,.F.);
#55132=ORIENTED_EDGE('',*,*,#42491,.F.);
#55133=ORIENTED_EDGE('',*,*,#42492,.T.);
#55134=ORIENTED_EDGE('',*,*,#42490,.F.);
#55135=ORIENTED_EDGE('',*,*,#42488,.F.);
#55136=ORIENTED_EDGE('',*,*,#42493,.F.);
#55137=ORIENTED_EDGE('',*,*,#42494,.T.);
#55138=ORIENTED_EDGE('',*,*,#42066,.T.);
#55139=ORIENTED_EDGE('',*,*,#42492,.F.);
#55140=ORIENTED_EDGE('',*,*,#42495,.F.);
#55141=ORIENTED_EDGE('',*,*,#42496,.T.);
#55142=ORIENTED_EDGE('',*,*,#42047,.F.);
#55143=ORIENTED_EDGE('',*,*,#42494,.F.);
#55144=ORIENTED_EDGE('',*,*,#42497,.F.);
#55145=ORIENTED_EDGE('',*,*,#42498,.T.);
#55146=ORIENTED_EDGE('',*,*,#42499,.F.);
#55147=ORIENTED_EDGE('',*,*,#42496,.F.);
#55148=ORIENTED_EDGE('',*,*,#42499,.T.);
#55149=ORIENTED_EDGE('',*,*,#42500,.T.);
#55150=ORIENTED_EDGE('',*,*,#42050,.T.);
#55151=ORIENTED_EDGE('',*,*,#42048,.T.);
#55152=ORIENTED_EDGE('',*,*,#42501,.F.);
#55153=ORIENTED_EDGE('',*,*,#42502,.T.);
#55154=ORIENTED_EDGE('',*,*,#42500,.F.);
#55155=ORIENTED_EDGE('',*,*,#42498,.F.);
#55156=ORIENTED_EDGE('',*,*,#42051,.F.);
#55157=ORIENTED_EDGE('',*,*,#42502,.F.);
#55158=ORIENTED_EDGE('',*,*,#42503,.F.);
#55159=ORIENTED_EDGE('',*,*,#42504,.F.);
#55160=ORIENTED_EDGE('',*,*,#42479,.F.);
#55161=ORIENTED_EDGE('',*,*,#42504,.T.);
#55162=ORIENTED_EDGE('',*,*,#42505,.F.);
#55163=ORIENTED_EDGE('',*,*,#42506,.F.);
#55164=ORIENTED_EDGE('',*,*,#42480,.F.);
#55165=ORIENTED_EDGE('',*,*,#42506,.T.);
#55166=ORIENTED_EDGE('',*,*,#42507,.F.);
#55167=ORIENTED_EDGE('',*,*,#42482,.F.);
#55168=ORIENTED_EDGE('',*,*,#42491,.T.);
#55169=ORIENTED_EDGE('',*,*,#42508,.T.);
#55170=ORIENTED_EDGE('',*,*,#42507,.T.);
#55171=ORIENTED_EDGE('',*,*,#42509,.T.);
#55172=ORIENTED_EDGE('',*,*,#42497,.T.);
#55173=ORIENTED_EDGE('',*,*,#42495,.T.);
#55174=ORIENTED_EDGE('',*,*,#42493,.T.);
#55175=ORIENTED_EDGE('',*,*,#41244,.T.);
#55176=ORIENTED_EDGE('',*,*,#42505,.T.);
#55177=ORIENTED_EDGE('',*,*,#42503,.T.);
#55178=ORIENTED_EDGE('',*,*,#42501,.T.);
#55179=ORIENTED_EDGE('',*,*,#42509,.F.);
#55180=ORIENTED_EDGE('',*,*,#42483,.T.);
#55181=ORIENTED_EDGE('',*,*,#42508,.F.);
#55182=ORIENTED_EDGE('',*,*,#42487,.T.);
#55183=ORIENTED_EDGE('',*,*,#42485,.T.);
#55184=ORIENTED_EDGE('',*,*,#41242,.F.);
#55185=ORIENTED_EDGE('',*,*,#41238,.T.);
#55186=ORIENTED_EDGE('',*,*,#41236,.F.);
#55187=ORIENTED_EDGE('',*,*,#41232,.T.);
#55188=ORIENTED_EDGE('',*,*,#42510,.T.);
#55189=ORIENTED_EDGE('',*,*,#41231,.F.);
#55190=ORIENTED_EDGE('',*,*,#41292,.T.);
#55191=ORIENTED_EDGE('',*,*,#41233,.T.);
#55192=ORIENTED_EDGE('',*,*,#42510,.F.);
#55193=ORIENTED_EDGE('',*,*,#42511,.T.);
#55194=ORIENTED_EDGE('',*,*,#42512,.T.);
#55195=ORIENTED_EDGE('',*,*,#42275,.F.);
#55196=ORIENTED_EDGE('',*,*,#42513,.T.);
#55197=ORIENTED_EDGE('',*,*,#42514,.T.);
#55198=ORIENTED_EDGE('',*,*,#41294,.T.);
#55199=ORIENTED_EDGE('',*,*,#41296,.T.);
#55200=ORIENTED_EDGE('',*,*,#41295,.F.);
#55201=ORIENTED_EDGE('',*,*,#42514,.F.);
#55202=ORIENTED_EDGE('',*,*,#42515,.T.);
#55203=ORIENTED_EDGE('',*,*,#42516,.T.);
#55204=ORIENTED_EDGE('',*,*,#42517,.T.);
#55205=ORIENTED_EDGE('',*,*,#42518,.T.);
#55206=ORIENTED_EDGE('',*,*,#42519,.F.);
#55207=ORIENTED_EDGE('',*,*,#42520,.T.);
#55208=ORIENTED_EDGE('',*,*,#42318,.T.);
#55209=ORIENTED_EDGE('',*,*,#42316,.T.);
#55210=ORIENTED_EDGE('',*,*,#42521,.T.);
#55211=ORIENTED_EDGE('',*,*,#42511,.F.);
#55212=ORIENTED_EDGE('',*,*,#42522,.T.);
#55213=ORIENTED_EDGE('',*,*,#42521,.F.);
#55214=ORIENTED_EDGE('',*,*,#42315,.F.);
#55215=ORIENTED_EDGE('',*,*,#42523,.T.);
#55216=ORIENTED_EDGE('',*,*,#42313,.F.);
#55217=ORIENTED_EDGE('',*,*,#42524,.F.);
#55218=ORIENTED_EDGE('',*,*,#42523,.F.);
#55219=ORIENTED_EDGE('',*,*,#42310,.T.);
#55220=ORIENTED_EDGE('',*,*,#42276,.F.);
#55221=ORIENTED_EDGE('',*,*,#42525,.F.);
#55222=ORIENTED_EDGE('',*,*,#42524,.T.);
#55223=ORIENTED_EDGE('',*,*,#42522,.F.);
#55224=ORIENTED_EDGE('',*,*,#42525,.T.);
#55225=ORIENTED_EDGE('',*,*,#42512,.F.);
#55226=ORIENTED_EDGE('',*,*,#42319,.T.);
#55227=ORIENTED_EDGE('',*,*,#42520,.F.);
#55228=ORIENTED_EDGE('',*,*,#42526,.F.);
#55229=ORIENTED_EDGE('',*,*,#42527,.T.);
#55230=ORIENTED_EDGE('',*,*,#42528,.F.);
#55231=ORIENTED_EDGE('',*,*,#42323,.F.);
#55232=ORIENTED_EDGE('',*,*,#42321,.T.);
#55233=ORIENTED_EDGE('',*,*,#42527,.F.);
#55234=ORIENTED_EDGE('',*,*,#42529,.F.);
#55235=ORIENTED_EDGE('',*,*,#42530,.F.);
#55236=ORIENTED_EDGE('',*,*,#42531,.T.);
#55237=ORIENTED_EDGE('',*,*,#42518,.F.);
#55238=ORIENTED_EDGE('',*,*,#42532,.F.);
#55239=ORIENTED_EDGE('',*,*,#42530,.T.);
#55240=ORIENTED_EDGE('',*,*,#42532,.T.);
#55241=ORIENTED_EDGE('',*,*,#42517,.F.);
#55242=ORIENTED_EDGE('',*,*,#42533,.F.);
#55243=ORIENTED_EDGE('',*,*,#42534,.T.);
#55244=ORIENTED_EDGE('',*,*,#42535,.F.);
#55245=ORIENTED_EDGE('',*,*,#42324,.F.);
#55246=ORIENTED_EDGE('',*,*,#42528,.T.);
#55247=ORIENTED_EDGE('',*,*,#42534,.F.);
#55248=ORIENTED_EDGE('',*,*,#41885,.F.);
#55249=ORIENTED_EDGE('',*,*,#42535,.T.);
#55250=ORIENTED_EDGE('',*,*,#42536,.F.);
#55251=ORIENTED_EDGE('',*,*,#42537,.T.);
#55252=ORIENTED_EDGE('',*,*,#42538,.F.);
#55253=ORIENTED_EDGE('',*,*,#42539,.T.);
#55254=ORIENTED_EDGE('',*,*,#42273,.F.);
#55255=ORIENTED_EDGE('',*,*,#42540,.F.);
#55256=ORIENTED_EDGE('',*,*,#42538,.T.);
#55257=ORIENTED_EDGE('',*,*,#42540,.T.);
#55258=ORIENTED_EDGE('',*,*,#42272,.F.);
#55259=ORIENTED_EDGE('',*,*,#42541,.F.);
#55260=ORIENTED_EDGE('',*,*,#41886,.T.);
#55261=ORIENTED_EDGE('',*,*,#42542,.F.);
#55262=ORIENTED_EDGE('',*,*,#42543,.F.);
#55263=ORIENTED_EDGE('',*,*,#42541,.T.);
#55264=ORIENTED_EDGE('',*,*,#42543,.T.);
#55265=ORIENTED_EDGE('',*,*,#42303,.F.);
#55266=ORIENTED_EDGE('',*,*,#42544,.F.);
#55267=ORIENTED_EDGE('',*,*,#41887,.T.);
#55268=ORIENTED_EDGE('',*,*,#42544,.T.);
#55269=ORIENTED_EDGE('',*,*,#42545,.F.);
#55270=ORIENTED_EDGE('',*,*,#42546,.F.);
#55271=ORIENTED_EDGE('',*,*,#41888,.T.);
#55272=ORIENTED_EDGE('',*,*,#42546,.T.);
#55273=ORIENTED_EDGE('',*,*,#42547,.F.);
#55274=ORIENTED_EDGE('',*,*,#41987,.F.);
#55275=ORIENTED_EDGE('',*,*,#41858,.T.);
#55276=ORIENTED_EDGE('',*,*,#42254,.T.);
#55277=ORIENTED_EDGE('',*,*,#42547,.T.);
#55278=ORIENTED_EDGE('',*,*,#42545,.T.);
#55279=ORIENTED_EDGE('',*,*,#42302,.F.);
#55280=ORIENTED_EDGE('',*,*,#42548,.F.);
#55281=ORIENTED_EDGE('',*,*,#42548,.T.);
#55282=ORIENTED_EDGE('',*,*,#42549,.T.);
#55283=ORIENTED_EDGE('',*,*,#42261,.F.);
#55284=ORIENTED_EDGE('',*,*,#42247,.F.);
#55285=ORIENTED_EDGE('',*,*,#41933,.F.);
#55286=ORIENTED_EDGE('',*,*,#42550,.F.);
#55287=ORIENTED_EDGE('',*,*,#41927,.F.);
#55288=ORIENTED_EDGE('',*,*,#41930,.F.);
#55289=ORIENTED_EDGE('',*,*,#41925,.F.);
#55290=ORIENTED_EDGE('',*,*,#42255,.F.);
#55291=ORIENTED_EDGE('',*,*,#41931,.T.);
#55292=ORIENTED_EDGE('',*,*,#41928,.T.);
#55293=ORIENTED_EDGE('',*,*,#42550,.T.);
#55294=ORIENTED_EDGE('',*,*,#41932,.T.);
#55295=ORIENTED_EDGE('',*,*,#42257,.F.);
#55296=ORIENTED_EDGE('',*,*,#42263,.F.);
#55297=ORIENTED_EDGE('',*,*,#42549,.F.);
#55298=ORIENTED_EDGE('',*,*,#42305,.T.);
#55299=ORIENTED_EDGE('',*,*,#41229,.T.);
#55300=ORIENTED_EDGE('',*,*,#42304,.F.);
#55301=ORIENTED_EDGE('',*,*,#42542,.T.);
#55302=ORIENTED_EDGE('',*,*,#42271,.T.);
#55303=ORIENTED_EDGE('',*,*,#41225,.F.);
#55304=ORIENTED_EDGE('',*,*,#42551,.T.);
#55305=ORIENTED_EDGE('',*,*,#42274,.F.);
#55306=ORIENTED_EDGE('',*,*,#42539,.F.);
#55307=ORIENTED_EDGE('',*,*,#42552,.T.);
#55308=ORIENTED_EDGE('',*,*,#42537,.F.);
#55309=ORIENTED_EDGE('',*,*,#42553,.F.);
#55310=ORIENTED_EDGE('',*,*,#42552,.F.);
#55311=ORIENTED_EDGE('',*,*,#42554,.T.);
#55312=ORIENTED_EDGE('',*,*,#42515,.F.);
#55313=ORIENTED_EDGE('',*,*,#42555,.F.);
#55314=ORIENTED_EDGE('',*,*,#42553,.T.);
#55315=ORIENTED_EDGE('',*,*,#42551,.F.);
#55316=ORIENTED_EDGE('',*,*,#42555,.T.);
#55317=ORIENTED_EDGE('',*,*,#42513,.F.);
#55318=ORIENTED_EDGE('',*,*,#42533,.T.);
#55319=ORIENTED_EDGE('',*,*,#42516,.F.);
#55320=ORIENTED_EDGE('',*,*,#42554,.F.);
#55321=ORIENTED_EDGE('',*,*,#42536,.T.);
#55322=ORIENTED_EDGE('',*,*,#42526,.T.);
#55323=ORIENTED_EDGE('',*,*,#42556,.F.);
#55324=ORIENTED_EDGE('',*,*,#42531,.F.);
#55325=ORIENTED_EDGE('',*,*,#42529,.T.);
#55326=ORIENTED_EDGE('',*,*,#42519,.T.);
#55327=ORIENTED_EDGE('',*,*,#42556,.T.);
#55328=ORIENTED_EDGE('',*,*,#42454,.F.);
#55329=ORIENTED_EDGE('',*,*,#42408,.T.);
#55330=ORIENTED_EDGE('',*,*,#42455,.F.);
#55331=ORIENTED_EDGE('',*,*,#42438,.F.);
#55332=ORIENTED_EDGE('',*,*,#42410,.F.);
#55333=ORIENTED_EDGE('',*,*,#42450,.T.);
#55334=ORIENTED_EDGE('',*,*,#42447,.T.);
#55335=ORIENTED_EDGE('',*,*,#41221,.T.);
#55336=ORIENTED_EDGE('',*,*,#42557,.F.);
#55337=ORIENTED_EDGE('',*,*,#42327,.F.);
#55338=ORIENTED_EDGE('',*,*,#41906,.T.);
#55339=ORIENTED_EDGE('',*,*,#42558,.T.);
#55340=ORIENTED_EDGE('',*,*,#42332,.T.);
#55341=ORIENTED_EDGE('',*,*,#41217,.F.);
#55342=ORIENTED_EDGE('',*,*,#41215,.F.);
#55343=ORIENTED_EDGE('',*,*,#42559,.T.);
#55344=ORIENTED_EDGE('',*,*,#41219,.T.);
#55345=ORIENTED_EDGE('',*,*,#41962,.F.);
#55346=ORIENTED_EDGE('',*,*,#42560,.F.);
#55347=ORIENTED_EDGE('',*,*,#42560,.T.);
#55348=ORIENTED_EDGE('',*,*,#41966,.F.);
#55349=ORIENTED_EDGE('',*,*,#41837,.F.);
#55350=ORIENTED_EDGE('',*,*,#42561,.F.);
#55351=ORIENTED_EDGE('',*,*,#42561,.T.);
#55352=ORIENTED_EDGE('',*,*,#42562,.T.);
#55353=ORIENTED_EDGE('',*,*,#42563,.F.);
#55354=ORIENTED_EDGE('',*,*,#42564,.F.);
#55355=ORIENTED_EDGE('',*,*,#42328,.T.);
#55356=ORIENTED_EDGE('',*,*,#42557,.T.);
#55357=ORIENTED_EDGE('',*,*,#42559,.F.);
#55358=ORIENTED_EDGE('',*,*,#42563,.T.);
#55359=ORIENTED_EDGE('',*,*,#42565,.T.);
#55360=ORIENTED_EDGE('',*,*,#41954,.F.);
#55361=ORIENTED_EDGE('',*,*,#41951,.T.);
#55362=ORIENTED_EDGE('',*,*,#42566,.T.);
#55363=ORIENTED_EDGE('',*,*,#41350,.F.);
#55364=ORIENTED_EDGE('',*,*,#42567,.T.);
#55365=ORIENTED_EDGE('',*,*,#41959,.T.);
#55366=ORIENTED_EDGE('',*,*,#42568,.T.);
#55367=ORIENTED_EDGE('',*,*,#41949,.T.);
#55368=ORIENTED_EDGE('',*,*,#42568,.F.);
#55369=ORIENTED_EDGE('',*,*,#41897,.F.);
#55370=ORIENTED_EDGE('',*,*,#41829,.T.);
#55371=ORIENTED_EDGE('',*,*,#42569,.F.);
#55372=ORIENTED_EDGE('',*,*,#41854,.T.);
#55373=ORIENTED_EDGE('',*,*,#42570,.F.);
#55374=ORIENTED_EDGE('',*,*,#41824,.F.);
#55375=ORIENTED_EDGE('',*,*,#41825,.F.);
#55376=ORIENTED_EDGE('',*,*,#42570,.T.);
#55377=ORIENTED_EDGE('',*,*,#42571,.T.);
#55378=ORIENTED_EDGE('',*,*,#42572,.F.);
#55379=ORIENTED_EDGE('',*,*,#42566,.F.);
#55380=ORIENTED_EDGE('',*,*,#41950,.F.);
#55381=ORIENTED_EDGE('',*,*,#42572,.T.);
#55382=ORIENTED_EDGE('',*,*,#41853,.F.);
#55383=ORIENTED_EDGE('',*,*,#41290,.F.);
#55384=ORIENTED_EDGE('',*,*,#42564,.T.);
#55385=ORIENTED_EDGE('',*,*,#42571,.F.);
#55386=ORIENTED_EDGE('',*,*,#41901,.T.);
#55387=ORIENTED_EDGE('',*,*,#42567,.F.);
#55388=ORIENTED_EDGE('',*,*,#42573,.F.);
#55389=ORIENTED_EDGE('',*,*,#41833,.T.);
#55390=ORIENTED_EDGE('',*,*,#42573,.T.);
#55391=ORIENTED_EDGE('',*,*,#41349,.F.);
#55392=ORIENTED_EDGE('',*,*,#41956,.F.);
#55393=ORIENTED_EDGE('',*,*,#41834,.T.);
#55394=ORIENTED_EDGE('',*,*,#41957,.T.);
#55395=ORIENTED_EDGE('',*,*,#42565,.F.);
#55396=ORIENTED_EDGE('',*,*,#42562,.F.);
#55397=ORIENTED_EDGE('',*,*,#41836,.T.);
#55398=ORIENTED_EDGE('',*,*,#42574,.T.);
#55399=ORIENTED_EDGE('',*,*,#41963,.F.);
#55400=ORIENTED_EDGE('',*,*,#41218,.F.);
#55401=ORIENTED_EDGE('',*,*,#42334,.T.);
#55402=ORIENTED_EDGE('',*,*,#42575,.T.);
#55403=ORIENTED_EDGE('',*,*,#42576,.T.);
#55404=ORIENTED_EDGE('',*,*,#41964,.F.);
#55405=ORIENTED_EDGE('',*,*,#42574,.F.);
#55406=ORIENTED_EDGE('',*,*,#42577,.F.);
#55407=ORIENTED_EDGE('',*,*,#42575,.F.);
#55408=ORIENTED_EDGE('',*,*,#42333,.F.);
#55409=ORIENTED_EDGE('',*,*,#42578,.T.);
#55410=ORIENTED_EDGE('',*,*,#42579,.F.);
#55411=ORIENTED_EDGE('',*,*,#42578,.F.);
#55412=ORIENTED_EDGE('',*,*,#42558,.F.);
#55413=ORIENTED_EDGE('',*,*,#41905,.T.);
#55414=ORIENTED_EDGE('',*,*,#41967,.T.);
#55415=ORIENTED_EDGE('',*,*,#41998,.T.);
#55416=ORIENTED_EDGE('',*,*,#42348,.F.);
#55417=ORIENTED_EDGE('',*,*,#42580,.F.);
#55418=ORIENTED_EDGE('',*,*,#42346,.T.);
#55419=ORIENTED_EDGE('',*,*,#42581,.F.);
#55420=ORIENTED_EDGE('',*,*,#41969,.F.);
#55421=ORIENTED_EDGE('',*,*,#42580,.T.);
#55422=ORIENTED_EDGE('',*,*,#41972,.T.);
#55423=ORIENTED_EDGE('',*,*,#41970,.T.);
#55424=ORIENTED_EDGE('',*,*,#42581,.T.);
#55425=ORIENTED_EDGE('',*,*,#42345,.T.);
#55426=ORIENTED_EDGE('',*,*,#42343,.T.);
#55427=ORIENTED_EDGE('',*,*,#42582,.T.);
#55428=ORIENTED_EDGE('',*,*,#41911,.T.);
#55429=ORIENTED_EDGE('',*,*,#42583,.F.);
#55430=ORIENTED_EDGE('',*,*,#41914,.F.);
#55431=ORIENTED_EDGE('',*,*,#41919,.F.);
#55432=ORIENTED_EDGE('',*,*,#41918,.F.);
#55433=ORIENTED_EDGE('',*,*,#42584,.F.);
#55434=ORIENTED_EDGE('',*,*,#41922,.F.);
#55435=ORIENTED_EDGE('',*,*,#41841,.T.);
#55436=ORIENTED_EDGE('',*,*,#41912,.F.);
#55437=ORIENTED_EDGE('',*,*,#42584,.T.);
#55438=ORIENTED_EDGE('',*,*,#41917,.T.);
#55439=ORIENTED_EDGE('',*,*,#41920,.T.);
#55440=ORIENTED_EDGE('',*,*,#41866,.F.);
#55441=ORIENTED_EDGE('',*,*,#41846,.F.);
#55442=ORIENTED_EDGE('',*,*,#41921,.T.);
#55443=ORIENTED_EDGE('',*,*,#42582,.F.);
#55444=ORIENTED_EDGE('',*,*,#42342,.F.);
#55445=ORIENTED_EDGE('',*,*,#41869,.T.);
#55446=ORIENTED_EDGE('',*,*,#41915,.T.);
#55447=ORIENTED_EDGE('',*,*,#42583,.T.);
#55448=ORIENTED_EDGE('',*,*,#42279,.T.);
#55449=ORIENTED_EDGE('',*,*,#42307,.T.);
#55450=ORIENTED_EDGE('',*,*,#42300,.F.);
#55451=ORIENTED_EDGE('',*,*,#42288,.F.);
#55452=ORIENTED_EDGE('',*,*,#42239,.T.);
#55453=ORIENTED_EDGE('',*,*,#42232,.T.);
#55454=ORIENTED_EDGE('',*,*,#42292,.F.);
#55455=ORIENTED_EDGE('',*,*,#42296,.F.);
#55456=ORIENTED_EDGE('',*,*,#42280,.F.);
#55457=ORIENTED_EDGE('',*,*,#42287,.T.);
#55458=ORIENTED_EDGE('',*,*,#42585,.T.);
#55459=ORIENTED_EDGE('',*,*,#42585,.F.);
#55460=ORIENTED_EDGE('',*,*,#42285,.T.);
#55461=ORIENTED_EDGE('',*,*,#42282,.T.);
#55462=ORIENTED_EDGE('',*,*,#41991,.T.);
#55463=ORIENTED_EDGE('',*,*,#42253,.F.);
#55464=ORIENTED_EDGE('',*,*,#42122,.F.);
#55465=ORIENTED_EDGE('',*,*,#41872,.T.);
#55466=ORIENTED_EDGE('',*,*,#42162,.T.);
#55467=ORIENTED_EDGE('',*,*,#42212,.F.);
#55468=ORIENTED_EDGE('',*,*,#42586,.F.);
#55469=ORIENTED_EDGE('',*,*,#42169,.T.);
#55470=ORIENTED_EDGE('',*,*,#42586,.T.);
#55471=ORIENTED_EDGE('',*,*,#42211,.F.);
#55472=ORIENTED_EDGE('',*,*,#42587,.F.);
#55473=ORIENTED_EDGE('',*,*,#42171,.T.);
#55474=ORIENTED_EDGE('',*,*,#42587,.T.);
#55475=ORIENTED_EDGE('',*,*,#42210,.F.);
#55476=ORIENTED_EDGE('',*,*,#42588,.F.);
#55477=ORIENTED_EDGE('',*,*,#42174,.T.);
#55478=ORIENTED_EDGE('',*,*,#42588,.T.);
#55479=ORIENTED_EDGE('',*,*,#42209,.F.);
#55480=ORIENTED_EDGE('',*,*,#42589,.F.);
#55481=ORIENTED_EDGE('',*,*,#42177,.T.);
#55482=ORIENTED_EDGE('',*,*,#42589,.T.);
#55483=ORIENTED_EDGE('',*,*,#42208,.F.);
#55484=ORIENTED_EDGE('',*,*,#42206,.F.);
#55485=ORIENTED_EDGE('',*,*,#42179,.T.);
#55486=ORIENTED_EDGE('',*,*,#42010,.F.);
#55487=ORIENTED_EDGE('',*,*,#42149,.F.);
#55488=ORIENTED_EDGE('',*,*,#41986,.T.);
#55489=ORIENTED_EDGE('',*,*,#42590,.T.);
#55490=ORIENTED_EDGE('',*,*,#42002,.T.);
#55491=ORIENTED_EDGE('',*,*,#42591,.F.);
#55492=ORIENTED_EDGE('',*,*,#42590,.F.);
#55493=ORIENTED_EDGE('',*,*,#42591,.T.);
#55494=ORIENTED_EDGE('',*,*,#42001,.T.);
#55495=ORIENTED_EDGE('',*,*,#42592,.F.);
#55496=ORIENTED_EDGE('',*,*,#42011,.F.);
#55497=ORIENTED_EDGE('',*,*,#42592,.T.);
#55498=ORIENTED_EDGE('',*,*,#41347,.T.);
#55499=ORIENTED_EDGE('',*,*,#42006,.F.);
#55500=ORIENTED_EDGE('',*,*,#42012,.F.);
#55501=ORIENTED_EDGE('',*,*,#41195,.T.);
#55502=ORIENTED_EDGE('',*,*,#41889,.T.);
#55503=ORIENTED_EDGE('',*,*,#42339,.T.);
#55504=ORIENTED_EDGE('',*,*,#42335,.T.);
#55505=ORIENTED_EDGE('',*,*,#42338,.F.);
#55506=ORIENTED_EDGE('',*,*,#41850,.T.);
#55507=ORIENTED_EDGE('',*,*,#42569,.T.);
#55508=ORIENTED_EDGE('',*,*,#41823,.T.);
#55509=ORIENTED_EDGE('',*,*,#42593,.T.);
#55510=ORIENTED_EDGE('',*,*,#41830,.T.);
#55511=ORIENTED_EDGE('',*,*,#41965,.T.);
#55512=ORIENTED_EDGE('',*,*,#41960,.T.);
#55513=ORIENTED_EDGE('',*,*,#42576,.F.);
#55514=ORIENTED_EDGE('',*,*,#42577,.T.);
#55515=ORIENTED_EDGE('',*,*,#42579,.T.);
#55516=ORIENTED_EDGE('',*,*,#41904,.T.);
#55517=ORIENTED_EDGE('',*,*,#41822,.F.);
#55518=ORIENTED_EDGE('',*,*,#41896,.T.);
#55519=ORIENTED_EDGE('',*,*,#41958,.F.);
#55520=ORIENTED_EDGE('',*,*,#41899,.T.);
#55521=ORIENTED_EDGE('',*,*,#41831,.F.);
#55522=ORIENTED_EDGE('',*,*,#42593,.F.);
#75281=SPHERICAL_SURFACE('',#79484,1.5);
#75282=SPHERICAL_SURFACE('',#79492,1.5);
#75283=SPHERICAL_SURFACE('',#79502,1.5);
#75284=SPHERICAL_SURFACE('',#79509,1.5);
#75285=SPHERICAL_SURFACE('',#79543,1.5);
#75286=SPHERICAL_SURFACE('',#79551,1.5);
#75287=SPHERICAL_SURFACE('',#79587,1.5);
#75288=SPHERICAL_SURFACE('',#79742,1.5);
#75289=SPHERICAL_SURFACE('',#79783,1.5);
#75290=SPHERICAL_SURFACE('',#79858,1.5);
#75291=SPHERICAL_SURFACE('',#79878,1.5);
#75292=SPHERICAL_SURFACE('',#80177,1.5);
#75293=SPHERICAL_SURFACE('',#80194,1.5);
#75294=SPHERICAL_SURFACE('',#80323,1.5);
#75295=SPHERICAL_SURFACE('',#80328,1.5);
#75296=SPHERICAL_SURFACE('',#80339,1.5);
#75303=ADVANCED_FACE('',(#19873),#75281,.F.);
#75304=ADVANCED_FACE('',(#19874),#16835,.T.);
#75305=ADVANCED_FACE('',(#19875),#2389,.F.);
#75306=ADVANCED_FACE('',(#19876),#2390,.T.);
#75307=ADVANCED_FACE('',(#19877),#2391,.F.);
#75308=ADVANCED_FACE('',(#19878),#1980,.F.);
#75309=ADVANCED_FACE('',(#19879),#1981,.T.);
#75310=ADVANCED_FACE('',(#19880),#75282,.F.);
#75311=ADVANCED_FACE('',(#19881),#2392,.F.);
#75312=ADVANCED_FACE('',(#19882),#16836,.T.);
#75313=ADVANCED_FACE('',(#19883),#2393,.F.);
#75314=ADVANCED_FACE('',(#19884),#2394,.T.);
#75315=ADVANCED_FACE('',(#19885),#1982,.F.);
#75316=ADVANCED_FACE('',(#19886),#1983,.T.);
#75317=ADVANCED_FACE('',(#19887),#1984,.T.);
#75318=ADVANCED_FACE('',(#19888),#2395,.F.);
#75319=ADVANCED_FACE('',(#19889),#75283,.F.);
#75320=ADVANCED_FACE('',(#19890),#1985,.F.);
#75321=ADVANCED_FACE('',(#19891),#16837,.T.);
#75322=ADVANCED_FACE('',(#19892),#2396,.F.);
#75323=ADVANCED_FACE('',(#19893),#2397,.T.);
#75324=ADVANCED_FACE('',(#19894),#2398,.F.);
#75325=ADVANCED_FACE('',(#19895),#2399,.T.);
#75326=ADVANCED_FACE('',(#19896),#16838,.T.);
#75327=ADVANCED_FACE('',(#19897),#1986,.T.);
#75328=ADVANCED_FACE('',(#19898),#75284,.F.);
#75329=ADVANCED_FACE('',(#19899),#2400,.F.);
#75330=ADVANCED_FACE('',(#19900),#2401,.F.);
#75331=ADVANCED_FACE('',(#19901),#16839,.T.);
#75332=ADVANCED_FACE('',(#19902),#1987,.F.);
#75333=ADVANCED_FACE('',(#19903),#2402,.T.);
#75334=ADVANCED_FACE('',(#19904),#2403,.T.);
#75335=ADVANCED_FACE('',(#19905),#2404,.F.);
#75336=ADVANCED_FACE('',(#19906),#16840,.T.);
#75337=ADVANCED_FACE('',(#19907),#1988,.F.);
#75338=ADVANCED_FACE('',(#19908),#1989,.F.);
#75339=ADVANCED_FACE('',(#19909),#1990,.F.);
#75340=ADVANCED_FACE('',(#19910),#1991,.F.);
#75341=ADVANCED_FACE('',(#19911),#1992,.F.);
#75342=ADVANCED_FACE('',(#19912),#1993,.F.);
#75343=ADVANCED_FACE('',(#19913),#1994,.F.);
#75344=ADVANCED_FACE('',(#19914),#1995,.F.);
#75345=ADVANCED_FACE('',(#19915),#1996,.F.);
#75346=ADVANCED_FACE('',(#19916),#1997,.F.);
#75347=ADVANCED_FACE('',(#19917),#1998,.F.);
#75348=ADVANCED_FACE('',(#19918),#1999,.F.);
#75349=ADVANCED_FACE('',(#19919),#2000,.F.);
#75350=ADVANCED_FACE('',(#19920),#2001,.F.);
#75351=ADVANCED_FACE('',(#19921),#2405,.F.);
#75352=ADVANCED_FACE('',(#19922),#2002,.T.);
#75353=ADVANCED_FACE('',(#19923),#75285,.F.);
#75354=ADVANCED_FACE('',(#19924),#2003,.T.);
#75355=ADVANCED_FACE('',(#19925),#75286,.F.);
#75356=ADVANCED_FACE('',(#19926),#1910,.F.);
#75357=ADVANCED_FACE('',(#19927),#2004,.F.);
#75358=ADVANCED_FACE('',(#19928),#1806,.T.);
#75359=ADVANCED_FACE('',(#19929),#2005,.F.);
#75360=ADVANCED_FACE('',(#19930),#1807,.T.);
#75361=ADVANCED_FACE('',(#19931),#1808,.T.);
#75362=ADVANCED_FACE('',(#19932),#2006,.T.);
#75363=ADVANCED_FACE('',(#19933),#2007,.T.);
#75364=ADVANCED_FACE('',(#19934),#1809,.T.);
#75365=ADVANCED_FACE('',(#19935),#2008,.T.);
#75366=ADVANCED_FACE('',(#19936),#75287,.F.);
#75367=ADVANCED_FACE('',(#19937),#2009,.F.);
#75368=ADVANCED_FACE('',(#19938),#1810,.T.);
#75369=ADVANCED_FACE('',(#19939),#2010,.F.);
#75370=ADVANCED_FACE('',(#19940),#2011,.F.);
#75371=ADVANCED_FACE('',(#19941),#2012,.F.);
#75372=ADVANCED_FACE('',(#19942),#2013,.F.);
#75373=ADVANCED_FACE('',(#19943),#1911,.F.);
#75374=ADVANCED_FACE('',(#19944),#2014,.F.);
#75375=ADVANCED_FACE('',(#19945),#2015,.F.);
#75376=ADVANCED_FACE('',(#19946),#1811,.T.);
#75377=ADVANCED_FACE('',(#19947),#2016,.F.);
#75378=ADVANCED_FACE('',(#19948),#1912,.F.);
#75379=ADVANCED_FACE('',(#19949),#2017,.F.);
#75380=ADVANCED_FACE('',(#19950),#2018,.T.);
#75381=ADVANCED_FACE('',(#19951),#2019,.F.);
#75382=ADVANCED_FACE('',(#19952),#2020,.F.);
#75383=ADVANCED_FACE('',(#19953),#2021,.F.);
#75384=ADVANCED_FACE('',(#19954),#1913,.F.);
#75385=ADVANCED_FACE('',(#19955),#1914,.F.);
#75386=ADVANCED_FACE('',(#19956),#2022,.F.);
#75387=ADVANCED_FACE('',(#19957),#1812,.T.);
#75388=ADVANCED_FACE('',(#19958),#2023,.F.);
#75389=ADVANCED_FACE('',(#19959),#1915,.F.);
#75390=ADVANCED_FACE('',(#19960),#2024,.F.);
#75391=ADVANCED_FACE('',(#19961),#2025,.T.);
#75392=ADVANCED_FACE('',(#19962),#2026,.F.);
#75393=ADVANCED_FACE('',(#19963),#2027,.F.);
#75394=ADVANCED_FACE('',(#19964),#2028,.T.);
#75395=ADVANCED_FACE('',(#19965),#2029,.T.);
#75396=ADVANCED_FACE('',(#19966),#1916,.T.);
#75397=ADVANCED_FACE('',(#19967),#2030,.F.);
#75398=ADVANCED_FACE('',(#19968),#1917,.F.);
#75399=ADVANCED_FACE('',(#19969),#1918,.F.);
#75400=ADVANCED_FACE('',(#19970),#1813,.T.);
#75401=ADVANCED_FACE('',(#19971),#2031,.F.);
#75402=ADVANCED_FACE('',(#19972),#1919,.F.);
#75403=ADVANCED_FACE('',(#19973),#2032,.F.);
#75404=ADVANCED_FACE('',(#19974),#2033,.T.);
#75405=ADVANCED_FACE('',(#19975),#2034,.F.);
#75406=ADVANCED_FACE('',(#19976),#2035,.F.);
#75407=ADVANCED_FACE('',(#19977),#2036,.T.);
#75408=ADVANCED_FACE('',(#19978),#2037,.T.);
#75409=ADVANCED_FACE('',(#19979),#1920,.T.);
#75410=ADVANCED_FACE('',(#19980),#2038,.F.);
#75411=ADVANCED_FACE('',(#19981),#1921,.F.);
#75412=ADVANCED_FACE('',(#19982),#1922,.F.);
#75413=ADVANCED_FACE('',(#19983,#245),#16841,.T.);
#75414=ADVANCED_FACE('',(#19984),#16842,.F.);
#75415=ADVANCED_FACE('',(#19985),#16843,.F.);
#75416=ADVANCED_FACE('',(#19986),#16844,.F.);
#75417=ADVANCED_FACE('',(#19987),#16845,.F.);
#75418=ADVANCED_FACE('',(#19988),#16846,.F.);
#75419=ADVANCED_FACE('',(#19989),#16847,.F.);
#75420=ADVANCED_FACE('',(#19990,#246),#16848,.T.);
#75421=ADVANCED_FACE('',(#19991,#247),#16849,.T.);
#75422=ADVANCED_FACE('',(#19992),#2039,.F.);
#75423=ADVANCED_FACE('',(#19993),#2406,.T.);
#75424=ADVANCED_FACE('',(#19994),#2407,.T.);
#75425=ADVANCED_FACE('',(#19995),#2040,.F.);
#75426=ADVANCED_FACE('',(#19996),#75288,.F.);
#75427=ADVANCED_FACE('',(#19997),#16850,.T.);
#75428=ADVANCED_FACE('',(#19998),#2408,.F.);
#75429=ADVANCED_FACE('',(#19999),#2409,.F.);
#75430=ADVANCED_FACE('',(#20000),#2041,.F.);
#75431=ADVANCED_FACE('',(#20001),#16851,.T.);
#75432=ADVANCED_FACE('',(#20002),#2410,.T.);
#75433=ADVANCED_FACE('',(#20003),#2042,.F.);
#75434=ADVANCED_FACE('',(#20004),#2043,.T.);
#75435=ADVANCED_FACE('',(#20005),#2411,.F.);
#75436=ADVANCED_FACE('',(#20006),#2044,.T.);
#75437=ADVANCED_FACE('',(#20007),#2412,.F.);
#75438=ADVANCED_FACE('',(#20008),#2413,.F.);
#75439=ADVANCED_FACE('',(#20009),#2414,.T.);
#75440=ADVANCED_FACE('',(#20010),#1814,.F.);
#75441=ADVANCED_FACE('',(#20011),#1815,.F.);
#75442=ADVANCED_FACE('',(#20012),#1816,.F.);
#75443=ADVANCED_FACE('',(#20013),#2415,.T.);
#75444=ADVANCED_FACE('',(#20014),#2416,.T.);
#75445=ADVANCED_FACE('',(#20015),#2417,.F.);
#75446=ADVANCED_FACE('',(#20016),#2045,.F.);
#75447=ADVANCED_FACE('',(#20017),#1817,.F.);
#75448=ADVANCED_FACE('',(#20018),#16852,.T.);
#75449=ADVANCED_FACE('',(#20019),#75289,.F.);
#75450=ADVANCED_FACE('',(#20020),#16853,.T.);
#75451=ADVANCED_FACE('',(#20021),#2418,.T.);
#75452=ADVANCED_FACE('',(#20022),#16854,.T.);
#75453=ADVANCED_FACE('',(#20023),#2419,.T.);
#75454=ADVANCED_FACE('',(#20024),#1818,.F.);
#75455=ADVANCED_FACE('',(#20025),#2420,.T.);
#75456=ADVANCED_FACE('',(#20026),#2046,.F.);
#75457=ADVANCED_FACE('',(#20027),#1819,.F.);
#75458=ADVANCED_FACE('',(#20028),#16855,.F.);
#75459=ADVANCED_FACE('',(#20029),#1820,.F.);
#75460=ADVANCED_FACE('',(#20030),#2047,.F.);
#75461=ADVANCED_FACE('',(#20031),#2421,.T.);
#75462=ADVANCED_FACE('',(#20032),#2048,.F.);
#75463=ADVANCED_FACE('',(#20033),#1821,.F.);
#75464=ADVANCED_FACE('',(#20034),#1822,.F.);
#75465=ADVANCED_FACE('',(#20035),#2049,.F.);
#75466=ADVANCED_FACE('',(#20036),#1823,.F.);
#75467=ADVANCED_FACE('',(#20037),#2050,.F.);
#75468=ADVANCED_FACE('',(#20038),#2051,.F.);
#75469=ADVANCED_FACE('',(#20039),#1824,.F.);
#75470=ADVANCED_FACE('',(#20040),#2052,.F.);
#75471=ADVANCED_FACE('',(#20041),#2053,.F.);
#75472=ADVANCED_FACE('',(#20042),#2422,.T.);
#75473=ADVANCED_FACE('',(#20043),#2423,.T.);
#75474=ADVANCED_FACE('',(#20044),#2424,.T.);
#75475=ADVANCED_FACE('',(#20045),#2425,.T.);
#75476=ADVANCED_FACE('',(#20046),#2426,.T.);
#75477=ADVANCED_FACE('',(#20047),#2427,.T.);
#75478=ADVANCED_FACE('',(#20048),#2428,.T.);
#75479=ADVANCED_FACE('',(#20049),#2429,.T.);
#75480=ADVANCED_FACE('',(#20050),#2430,.F.);
#75481=ADVANCED_FACE('',(#20051),#2431,.F.);
#75482=ADVANCED_FACE('',(#20052),#2432,.F.);
#75483=ADVANCED_FACE('',(#20053),#2433,.F.);
#75484=ADVANCED_FACE('',(#20054),#2434,.F.);
#75485=ADVANCED_FACE('',(#20055),#2435,.F.);
#75486=ADVANCED_FACE('',(#20056),#2436,.F.);
#75487=ADVANCED_FACE('',(#20057),#2437,.F.);
#75488=ADVANCED_FACE('',(#20058),#2438,.F.);
#75489=ADVANCED_FACE('',(#20059,#248),#16856,.F.);
#75490=ADVANCED_FACE('',(#20060),#113,.T.);
#75491=ADVANCED_FACE('',(#20061),#114,.T.);
#75492=ADVANCED_FACE('',(#20062),#115,.T.);
#75493=ADVANCED_FACE('',(#20063),#116,.T.);
#75494=ADVANCED_FACE('',(#20064),#117,.T.);
#75495=ADVANCED_FACE('',(#20065),#118,.T.);
#75496=ADVANCED_FACE('',(#20066,#249),#16857,.T.);
#75497=ADVANCED_FACE('',(#20067,#250),#16858,.T.);
#75498=ADVANCED_FACE('',(#20068),#16859,.F.);
#75499=ADVANCED_FACE('',(#20069),#16860,.F.);
#75500=ADVANCED_FACE('',(#20070),#16861,.F.);
#75501=ADVANCED_FACE('',(#20071),#16862,.F.);
#75502=ADVANCED_FACE('',(#20072),#16863,.F.);
#75503=ADVANCED_FACE('',(#20073),#16864,.F.);
#75504=ADVANCED_FACE('',(#20074,#251),#16865,.T.);
#75505=ADVANCED_FACE('',(#20075,#252),#16866,.T.);
#75506=ADVANCED_FACE('',(#20076),#2439,.T.);
#75507=ADVANCED_FACE('',(#20077),#2054,.F.);
#75508=ADVANCED_FACE('',(#20078),#2440,.F.);
#75509=ADVANCED_FACE('',(#20079),#2055,.T.);
#75510=ADVANCED_FACE('',(#20080),#2441,.T.);
#75511=ADVANCED_FACE('',(#20081),#2442,.F.);
#75512=ADVANCED_FACE('',(#20082),#2056,.F.);
#75513=ADVANCED_FACE('',(#20083),#2057,.F.);
#75514=ADVANCED_FACE('',(#20084),#2443,.F.);
#75515=ADVANCED_FACE('',(#20085),#16867,.T.);
#75516=ADVANCED_FACE('',(#20086),#2444,.F.);
#75517=ADVANCED_FACE('',(#20087),#75290,.F.);
#75518=ADVANCED_FACE('',(#20088),#2058,.F.);
#75519=ADVANCED_FACE('',(#20089),#16868,.T.);
#75520=ADVANCED_FACE('',(#20090),#2059,.T.);
#75521=ADVANCED_FACE('',(#20091),#2445,.T.);
#75522=ADVANCED_FACE('',(#20092),#2446,.T.);
#75523=ADVANCED_FACE('',(#20093),#2447,.F.);
#75524=ADVANCED_FACE('',(#20094),#2448,.T.);
#75525=ADVANCED_FACE('',(#20095),#16869,.T.);
#75526=ADVANCED_FACE('',(#20096),#2449,.T.);
#75527=ADVANCED_FACE('',(#20097),#16870,.T.);
#75528=ADVANCED_FACE('',(#20098),#75291,.F.);
#75529=ADVANCED_FACE('',(#20099),#16871,.T.);
#75530=ADVANCED_FACE('',(#20100),#1825,.F.);
#75531=ADVANCED_FACE('',(#20101),#2060,.F.);
#75532=ADVANCED_FACE('',(#20102),#2450,.F.);
#75533=ADVANCED_FACE('',(#20103),#2451,.T.);
#75534=ADVANCED_FACE('',(#20104),#2452,.T.);
#75535=ADVANCED_FACE('',(#20105),#1826,.F.);
#75536=ADVANCED_FACE('',(#20106),#1827,.F.);
#75537=ADVANCED_FACE('',(#20107),#1828,.F.);
#75538=ADVANCED_FACE('',(#20108),#2061,.F.);
#75539=ADVANCED_FACE('',(#20109),#2453,.T.);
#75540=ADVANCED_FACE('',(#20110),#1829,.F.);
#75541=ADVANCED_FACE('',(#20111),#1830,.F.);
#75542=ADVANCED_FACE('',(#20112),#2062,.F.);
#75543=ADVANCED_FACE('',(#20113),#1831,.F.);
#75544=ADVANCED_FACE('',(#20114),#1832,.F.);
#75545=ADVANCED_FACE('',(#20115),#2063,.F.);
#75546=ADVANCED_FACE('',(#20116),#2454,.T.);
#75547=ADVANCED_FACE('',(#20117),#2064,.F.);
#75548=ADVANCED_FACE('',(#20118),#1833,.F.);
#75549=ADVANCED_FACE('',(#20119),#16872,.T.);
#75550=ADVANCED_FACE('',(#20120),#1834,.F.);
#75551=ADVANCED_FACE('',(#20121),#2065,.F.);
#75552=ADVANCED_FACE('',(#20122),#2066,.F.);
#75553=ADVANCED_FACE('',(#20123),#2067,.F.);
#75554=ADVANCED_FACE('',(#20124),#1835,.F.);
#75555=ADVANCED_FACE('',(#20125),#2068,.F.);
#75556=ADVANCED_FACE('',(#20126),#2455,.T.);
#75557=ADVANCED_FACE('',(#20127),#2456,.T.);
#75558=ADVANCED_FACE('',(#20128),#2457,.T.);
#75559=ADVANCED_FACE('',(#20129),#2458,.T.);
#75560=ADVANCED_FACE('',(#20130),#2459,.T.);
#75561=ADVANCED_FACE('',(#20131),#2460,.T.);
#75562=ADVANCED_FACE('',(#20132),#2461,.T.);
#75563=ADVANCED_FACE('',(#20133),#2462,.T.);
#75564=ADVANCED_FACE('',(#20134),#2463,.F.);
#75565=ADVANCED_FACE('',(#20135),#2464,.F.);
#75566=ADVANCED_FACE('',(#20136),#2465,.F.);
#75567=ADVANCED_FACE('',(#20137),#2466,.F.);
#75568=ADVANCED_FACE('',(#20138),#2467,.F.);
#75569=ADVANCED_FACE('',(#20139),#2468,.F.);
#75570=ADVANCED_FACE('',(#20140),#2469,.F.);
#75571=ADVANCED_FACE('',(#20141),#2470,.F.);
#75572=ADVANCED_FACE('',(#20142),#2471,.F.);
#75573=ADVANCED_FACE('',(#20143,#253),#16873,.F.);
#75574=ADVANCED_FACE('',(#20144),#119,.F.);
#75575=ADVANCED_FACE('',(#20145),#120,.F.);
#75576=ADVANCED_FACE('',(#20146),#121,.F.);
#75577=ADVANCED_FACE('',(#20147),#122,.F.);
#75578=ADVANCED_FACE('',(#20148),#123,.F.);
#75579=ADVANCED_FACE('',(#20149),#124,.F.);
#75580=ADVANCED_FACE('',(#20150,#254),#16874,.F.);
#75581=ADVANCED_FACE('',(#20151),#125,.F.);
#75582=ADVANCED_FACE('',(#20152),#126,.F.);
#75583=ADVANCED_FACE('',(#20153),#16875,.T.);
#75584=ADVANCED_FACE('',(#20154,#255),#16876,.T.);
#75585=ADVANCED_FACE('',(#20155),#16877,.F.);
#75586=ADVANCED_FACE('',(#20156),#16878,.T.);
#75587=ADVANCED_FACE('',(#20157),#16879,.T.);
#75588=ADVANCED_FACE('',(#20158),#16880,.T.);
#75589=ADVANCED_FACE('',(#20159),#16881,.T.);
#75590=ADVANCED_FACE('',(#20160),#2069,.F.);
#75591=ADVANCED_FACE('',(#20161),#2472,.F.);
#75592=ADVANCED_FACE('',(#20162),#16882,.T.);
#75593=ADVANCED_FACE('',(#20163),#2473,.T.);
#75594=ADVANCED_FACE('',(#20164),#2070,.F.);
#75595=ADVANCED_FACE('',(#20165),#2071,.F.);
#75596=ADVANCED_FACE('',(#20166),#2072,.F.);
#75597=ADVANCED_FACE('',(#20167),#2073,.F.);
#75598=ADVANCED_FACE('',(#20168),#2474,.T.);
#75599=ADVANCED_FACE('',(#20169),#2475,.T.);
#75600=ADVANCED_FACE('',(#20170),#2476,.T.);
#75601=ADVANCED_FACE('',(#20171),#2477,.T.);
#75602=ADVANCED_FACE('',(#20172),#2074,.F.);
#75603=ADVANCED_FACE('',(#20173),#2075,.F.);
#75604=ADVANCED_FACE('',(#20174),#2478,.T.);
#75605=ADVANCED_FACE('',(#20175),#2479,.T.);
#75606=ADVANCED_FACE('',(#20176),#2480,.T.);
#75607=ADVANCED_FACE('',(#20177),#2481,.F.);
#75608=ADVANCED_FACE('',(#20178),#2076,.F.);
#75609=ADVANCED_FACE('',(#20179),#2077,.T.);
#75610=ADVANCED_FACE('',(#20180),#127,.F.);
#75611=ADVANCED_FACE('',(#20181),#2482,.F.);
#75612=ADVANCED_FACE('',(#20182),#2483,.F.);
#75613=ADVANCED_FACE('',(#20183),#2484,.F.);
#75614=ADVANCED_FACE('',(#20184),#2485,.T.);
#75615=ADVANCED_FACE('',(#20185),#2486,.T.);
#75616=ADVANCED_FACE('',(#20186),#2487,.T.);
#75617=ADVANCED_FACE('',(#20187),#2488,.T.);
#75618=ADVANCED_FACE('',(#20188),#2489,.T.);
#75619=ADVANCED_FACE('',(#20189),#2490,.T.);
#75620=ADVANCED_FACE('',(#20190),#2491,.T.);
#75621=ADVANCED_FACE('',(#20191),#2492,.T.);
#75622=ADVANCED_FACE('',(#20192),#1836,.F.);
#75623=ADVANCED_FACE('',(#20193),#1837,.F.);
#75624=ADVANCED_FACE('',(#20194),#1838,.F.);
#75625=ADVANCED_FACE('',(#20195),#2078,.F.);
#75626=ADVANCED_FACE('',(#20196),#1839,.F.);
#75627=ADVANCED_FACE('',(#20197),#16883,.T.);
#75628=ADVANCED_FACE('',(#20198),#16884,.T.);
#75629=ADVANCED_FACE('',(#20199),#2079,.T.);
#75630=ADVANCED_FACE('',(#20200),#2493,.T.);
#75631=ADVANCED_FACE('',(#20201),#2494,.F.);
#75632=ADVANCED_FACE('',(#20202),#1840,.F.);
#75633=ADVANCED_FACE('',(#20203),#2495,.T.);
#75634=ADVANCED_FACE('',(#20204),#2496,.F.);
#75635=ADVANCED_FACE('',(#20205),#2080,.F.);
#75636=ADVANCED_FACE('',(#20206),#1841,.F.);
#75637=ADVANCED_FACE('',(#20207),#1842,.F.);
#75638=ADVANCED_FACE('',(#20208),#2081,.F.);
#75639=ADVANCED_FACE('',(#20209),#2082,.F.);
#75640=ADVANCED_FACE('',(#20210),#2497,.F.);
#75641=ADVANCED_FACE('',(#20211),#2498,.F.);
#75642=ADVANCED_FACE('',(#20212),#2499,.F.);
#75643=ADVANCED_FACE('',(#20213),#2500,.T.);
#75644=ADVANCED_FACE('',(#20214),#16885,.T.);
#75645=ADVANCED_FACE('',(#20215,#256),#16886,.T.);
#75646=ADVANCED_FACE('',(#20216,#257),#16887,.T.);
#75647=ADVANCED_FACE('',(#20217),#2501,.T.);
#75648=ADVANCED_FACE('',(#20218),#2083,.T.);
#75649=ADVANCED_FACE('',(#20219),#2084,.T.);
#75650=ADVANCED_FACE('',(#20220),#2085,.T.);
#75651=ADVANCED_FACE('',(#20221),#2502,.T.);
#75652=ADVANCED_FACE('',(#20222),#2503,.T.);
#75653=ADVANCED_FACE('',(#20223),#2504,.T.);
#75654=ADVANCED_FACE('',(#20224),#2505,.T.);
#75655=ADVANCED_FACE('',(#20225),#2506,.T.);
#75656=ADVANCED_FACE('',(#20226),#2086,.T.);
#75657=ADVANCED_FACE('',(#20227),#128,.T.);
#75658=ADVANCED_FACE('',(#20228),#129,.F.);
#75659=ADVANCED_FACE('',(#20229),#130,.T.);
#75660=ADVANCED_FACE('',(#20230),#2087,.T.);
#75661=ADVANCED_FACE('',(#20231),#131,.T.);
#75662=ADVANCED_FACE('',(#20232),#132,.T.);
#75663=ADVANCED_FACE('',(#20233),#2507,.T.);
#75664=ADVANCED_FACE('',(#20234),#133,.T.);
#75665=ADVANCED_FACE('',(#20235),#134,.T.);
#75666=ADVANCED_FACE('',(#20236),#2088,.T.);
#75667=ADVANCED_FACE('',(#20237),#135,.F.);
#75668=ADVANCED_FACE('',(#20238,#258),#16888,.F.);
#75669=ADVANCED_FACE('',(#20239,#259),#16889,.T.);
#75670=ADVANCED_FACE('',(#20240,#260),#16890,.T.);
#75671=ADVANCED_FACE('',(#20241),#16891,.T.);
#75672=ADVANCED_FACE('',(#20242),#16892,.T.);
#75673=ADVANCED_FACE('',(#20243),#2508,.F.);
#75674=ADVANCED_FACE('',(#20244),#2509,.F.);
#75675=ADVANCED_FACE('',(#20245),#2510,.F.);
#75676=ADVANCED_FACE('',(#20246),#2511,.F.);
#75677=ADVANCED_FACE('',(#20247),#136,.T.);
#75678=ADVANCED_FACE('',(#20248),#2512,.F.);
#75679=ADVANCED_FACE('',(#20249),#16893,.T.);
#75680=ADVANCED_FACE('',(#20250),#2089,.T.);
#75681=ADVANCED_FACE('',(#20251),#2513,.F.);
#75682=ADVANCED_FACE('',(#20252),#137,.T.);
#75683=ADVANCED_FACE('',(#20253),#2514,.F.);
#75684=ADVANCED_FACE('',(#20254),#2515,.F.);
#75685=ADVANCED_FACE('',(#20255),#138,.T.);
#75686=ADVANCED_FACE('',(#20256),#139,.T.);
#75687=ADVANCED_FACE('',(#20257),#140,.T.);
#75688=ADVANCED_FACE('',(#20258),#2090,.F.);
#75689=ADVANCED_FACE('',(#20259),#2516,.F.);
#75690=ADVANCED_FACE('',(#20260),#2517,.F.);
#75691=ADVANCED_FACE('',(#20261),#2091,.F.);
#75692=ADVANCED_FACE('',(#20262),#1843,.F.);
#75693=ADVANCED_FACE('',(#20263),#1844,.F.);
#75694=ADVANCED_FACE('',(#20264),#2518,.F.);
#75695=ADVANCED_FACE('',(#20265),#2092,.F.);
#75696=ADVANCED_FACE('',(#20266),#2519,.F.);
#75697=ADVANCED_FACE('',(#20267),#1845,.F.);
#75698=ADVANCED_FACE('',(#20268),#2520,.F.);
#75699=ADVANCED_FACE('',(#20269),#2093,.F.);
#75700=ADVANCED_FACE('',(#20270),#2521,.T.);
#75701=ADVANCED_FACE('',(#20271),#2094,.F.);
#75702=ADVANCED_FACE('',(#20272),#2522,.F.);
#75703=ADVANCED_FACE('',(#20273),#1846,.F.);
#75704=ADVANCED_FACE('',(#20274),#2523,.F.);
#75705=ADVANCED_FACE('',(#20275),#2095,.F.);
#75706=ADVANCED_FACE('',(#20276),#2524,.F.);
#75707=ADVANCED_FACE('',(#20277),#1847,.F.);
#75708=ADVANCED_FACE('',(#20278),#1848,.F.);
#75709=ADVANCED_FACE('',(#20279),#2096,.F.);
#75710=ADVANCED_FACE('',(#20280),#2097,.F.);
#75711=ADVANCED_FACE('',(#20281),#141,.T.);
#75712=ADVANCED_FACE('',(#20282),#142,.T.);
#75713=ADVANCED_FACE('',(#20283),#143,.T.);
#75714=ADVANCED_FACE('',(#20284),#144,.T.);
#75715=ADVANCED_FACE('',(#20285),#2098,.F.);
#75716=ADVANCED_FACE('',(#20286),#145,.T.);
#75717=ADVANCED_FACE('',(#20287),#2525,.F.);
#75718=ADVANCED_FACE('',(#20288),#2526,.F.);
#75719=ADVANCED_FACE('',(#20289),#146,.T.);
#75720=ADVANCED_FACE('',(#20290),#147,.T.);
#75721=ADVANCED_FACE('',(#20291),#2527,.F.);
#75722=ADVANCED_FACE('',(#20292),#2528,.F.);
#75723=ADVANCED_FACE('',(#20293),#148,.T.);
#75724=ADVANCED_FACE('',(#20294),#2529,.F.);
#75725=ADVANCED_FACE('',(#20295),#2530,.F.);
#75726=ADVANCED_FACE('',(#20296),#149,.T.);
#75727=ADVANCED_FACE('',(#20297),#150,.T.);
#75728=ADVANCED_FACE('',(#20298),#2531,.F.);
#75729=ADVANCED_FACE('',(#20299),#2532,.F.);
#75730=ADVANCED_FACE('',(#20300),#151,.T.);
#75731=ADVANCED_FACE('',(#20301),#1849,.F.);
#75732=ADVANCED_FACE('',(#20302),#16894,.T.);
#75733=ADVANCED_FACE('',(#20303),#2099,.T.);
#75734=ADVANCED_FACE('',(#20304),#16895,.T.);
#75735=ADVANCED_FACE('',(#20305),#2100,.F.);
#75736=ADVANCED_FACE('',(#20306),#16896,.T.);
#75737=ADVANCED_FACE('',(#20307,#261),#16897,.F.);
#75738=ADVANCED_FACE('',(#20308,#262),#16898,.F.);
#75739=ADVANCED_FACE('',(#20309),#2101,.T.);
#75740=ADVANCED_FACE('',(#20310),#2102,.F.);
#75741=ADVANCED_FACE('',(#20311),#16899,.T.);
#75742=ADVANCED_FACE('',(#20312),#16900,.T.);
#75743=ADVANCED_FACE('',(#20313),#1850,.T.);
#75744=ADVANCED_FACE('',(#20314),#2533,.T.);
#75745=ADVANCED_FACE('',(#20315),#2103,.T.);
#75746=ADVANCED_FACE('',(#20316),#2104,.T.);
#75747=ADVANCED_FACE('',(#20317),#2105,.T.);
#75748=ADVANCED_FACE('',(#20318),#16901,.T.);
#75749=ADVANCED_FACE('',(#20319),#2106,.T.);
#75750=ADVANCED_FACE('',(#20320),#2534,.T.);
#75751=ADVANCED_FACE('',(#20321),#1851,.T.);
#75752=ADVANCED_FACE('',(#20322),#2535,.T.);
#75753=ADVANCED_FACE('',(#20323),#1852,.T.);
#75754=ADVANCED_FACE('',(#20324),#1853,.T.);
#75755=ADVANCED_FACE('',(#20325),#2536,.T.);
#75756=ADVANCED_FACE('',(#20326),#2537,.T.);
#75757=ADVANCED_FACE('',(#20327),#2107,.F.);
#75758=ADVANCED_FACE('',(#20328),#16902,.T.);
#75759=ADVANCED_FACE('',(#20329),#2108,.F.);
#75760=ADVANCED_FACE('',(#20330),#2538,.T.);
#75761=ADVANCED_FACE('',(#20331),#75292,.F.);
#75762=ADVANCED_FACE('',(#20332),#1854,.T.);
#75763=ADVANCED_FACE('',(#20333),#1855,.T.);
#75764=ADVANCED_FACE('',(#20334),#1856,.F.);
#75765=ADVANCED_FACE('',(#20335),#2539,.F.);
#75766=ADVANCED_FACE('',(#20336),#2540,.T.);
#75767=ADVANCED_FACE('',(#20337),#2109,.T.);
#75768=ADVANCED_FACE('',(#20338),#16903,.T.);
#75769=ADVANCED_FACE('',(#20339),#16904,.T.);
#75770=ADVANCED_FACE('',(#20340),#2110,.F.);
#75771=ADVANCED_FACE('',(#20341),#75293,.F.);
#75772=ADVANCED_FACE('',(#20342),#1857,.F.);
#75773=ADVANCED_FACE('',(#20343),#2541,.F.);
#75774=ADVANCED_FACE('',(#20344),#152,.T.);
#75775=ADVANCED_FACE('',(#20345),#2542,.F.);
#75776=ADVANCED_FACE('',(#20346),#2543,.F.);
#75777=ADVANCED_FACE('',(#20347),#2544,.T.);
#75778=ADVANCED_FACE('',(#20348),#2111,.F.);
#75779=ADVANCED_FACE('',(#20349),#2545,.F.);
#75780=ADVANCED_FACE('',(#20350),#2112,.F.);
#75781=ADVANCED_FACE('',(#20351),#2113,.F.);
#75782=ADVANCED_FACE('',(#20352),#2114,.F.);
#75783=ADVANCED_FACE('',(#20353),#2546,.T.);
#75784=ADVANCED_FACE('',(#20354),#2547,.F.);
#75785=ADVANCED_FACE('',(#20355),#2548,.T.);
#75786=ADVANCED_FACE('',(#20356),#2549,.T.);
#75787=ADVANCED_FACE('',(#20357),#2550,.F.);
#75788=ADVANCED_FACE('',(#20358),#2551,.F.);
#75789=ADVANCED_FACE('',(#20359),#2552,.T.);
#75790=ADVANCED_FACE('',(#20360,#263),#16905,.T.);
#75791=ADVANCED_FACE('',(#20361),#2553,.T.);
#75792=ADVANCED_FACE('',(#20362),#2554,.T.);
#75793=ADVANCED_FACE('',(#20363),#153,.T.);
#75794=ADVANCED_FACE('',(#20364),#2115,.T.);
#75795=ADVANCED_FACE('',(#20365),#2555,.T.);
#75796=ADVANCED_FACE('',(#20366),#154,.T.);
#75797=ADVANCED_FACE('',(#20367),#2556,.T.);
#75798=ADVANCED_FACE('',(#20368),#2116,.T.);
#75799=ADVANCED_FACE('',(#20369),#155,.T.);
#75800=ADVANCED_FACE('',(#20370),#2557,.T.);
#75801=ADVANCED_FACE('',(#20371),#2558,.T.);
#75802=ADVANCED_FACE('',(#20372),#156,.T.);
#75803=ADVANCED_FACE('',(#20373),#1858,.T.);
#75804=ADVANCED_FACE('',(#20374),#2117,.T.);
#75805=ADVANCED_FACE('',(#20375),#2118,.T.);
#75806=ADVANCED_FACE('',(#20376),#2119,.T.);
#75807=ADVANCED_FACE('',(#20377),#1859,.T.);
#75808=ADVANCED_FACE('',(#20378),#2120,.T.);
#75809=ADVANCED_FACE('',(#20379),#2121,.T.);
#75810=ADVANCED_FACE('',(#20380),#2559,.T.);
#75811=ADVANCED_FACE('',(#20381),#157,.T.);
#75812=ADVANCED_FACE('',(#20382),#2560,.T.);
#75813=ADVANCED_FACE('',(#20383),#2561,.T.);
#75814=ADVANCED_FACE('',(#20384),#158,.T.);
#75815=ADVANCED_FACE('',(#20385),#2562,.T.);
#75816=ADVANCED_FACE('',(#20386),#2563,.T.);
#75817=ADVANCED_FACE('',(#20387),#159,.T.);
#75818=ADVANCED_FACE('',(#20388),#2564,.T.);
#75819=ADVANCED_FACE('',(#20389),#160,.T.);
#75820=ADVANCED_FACE('',(#20390,#264),#16906,.T.);
#75821=ADVANCED_FACE('',(#20391),#2122,.T.);
#75822=ADVANCED_FACE('',(#20392),#2123,.T.);
#75823=ADVANCED_FACE('',(#20393),#2124,.T.);
#75824=ADVANCED_FACE('',(#20394),#1860,.T.);
#75825=ADVANCED_FACE('',(#20395),#1861,.T.);
#75826=ADVANCED_FACE('',(#20396),#1862,.T.);
#75827=ADVANCED_FACE('',(#20397),#16907,.F.);
#75828=ADVANCED_FACE('',(#20398),#1863,.T.);
#75829=ADVANCED_FACE('',(#20399),#2125,.T.);
#75830=ADVANCED_FACE('',(#20400),#161,.T.);
#75831=ADVANCED_FACE('',(#20401),#162,.T.);
#75832=ADVANCED_FACE('',(#20402),#2565,.T.);
#75833=ADVANCED_FACE('',(#20403),#163,.T.);
#75834=ADVANCED_FACE('',(#20404),#2566,.T.);
#75835=ADVANCED_FACE('',(#20405),#164,.T.);
#75836=ADVANCED_FACE('',(#20406),#165,.T.);
#75837=ADVANCED_FACE('',(#20407),#166,.T.);
#75838=ADVANCED_FACE('',(#20408),#2126,.T.);
#75839=ADVANCED_FACE('',(#20409),#2127,.T.);
#75840=ADVANCED_FACE('',(#20410),#167,.T.);
#75841=ADVANCED_FACE('',(#20411),#2567,.T.);
#75842=ADVANCED_FACE('',(#20412),#168,.T.);
#75843=ADVANCED_FACE('',(#20413),#2568,.T.);
#75844=ADVANCED_FACE('',(#20414),#1864,.T.);
#75845=ADVANCED_FACE('',(#20415),#1865,.T.);
#75846=ADVANCED_FACE('',(#20416),#1866,.T.);
#75847=ADVANCED_FACE('',(#20417),#16908,.T.);
#75848=ADVANCED_FACE('',(#20418),#1867,.T.);
#75849=ADVANCED_FACE('',(#20419,#265),#16909,.F.);
#75850=ADVANCED_FACE('',(#20420),#2569,.T.);
#75851=ADVANCED_FACE('',(#20421),#169,.T.);
#75852=ADVANCED_FACE('',(#20422),#2570,.T.);
#75853=ADVANCED_FACE('',(#20423),#2128,.T.);
#75854=ADVANCED_FACE('',(#20424),#2571,.T.);
#75855=ADVANCED_FACE('',(#20425),#170,.T.);
#75856=ADVANCED_FACE('',(#20426),#2572,.T.);
#75857=ADVANCED_FACE('',(#20427),#2129,.T.);
#75858=ADVANCED_FACE('',(#20428),#2573,.T.);
#75859=ADVANCED_FACE('',(#20429),#171,.T.);
#75860=ADVANCED_FACE('',(#20430),#2574,.T.);
#75861=ADVANCED_FACE('',(#20431),#2575,.T.);
#75862=ADVANCED_FACE('',(#20432),#2130,.T.);
#75863=ADVANCED_FACE('',(#20433),#2576,.T.);
#75864=ADVANCED_FACE('',(#20434),#172,.T.);
#75865=ADVANCED_FACE('',(#20435),#2577,.T.);
#75866=ADVANCED_FACE('',(#20436),#173,.T.);
#75867=ADVANCED_FACE('',(#20437,#266),#16910,.T.);
#75868=ADVANCED_FACE('',(#20438),#2131,.T.);
#75869=ADVANCED_FACE('',(#20439),#2132,.T.);
#75870=ADVANCED_FACE('',(#20440,#267),#16911,.F.);
#75871=ADVANCED_FACE('',(#20441,#268),#16912,.F.);
#75872=ADVANCED_FACE('',(#20442),#1923,.F.);
#75873=ADVANCED_FACE('',(#20443),#2133,.F.);
#75874=ADVANCED_FACE('',(#20444),#16913,.T.);
#75875=ADVANCED_FACE('',(#20445),#2578,.F.);
#75876=ADVANCED_FACE('',(#20446),#2579,.T.);
#75877=ADVANCED_FACE('',(#20447),#2580,.F.);
#75878=ADVANCED_FACE('',(#20448),#75294,.F.);
#75879=ADVANCED_FACE('',(#20449),#2581,.F.);
#75880=ADVANCED_FACE('',(#20450),#174,.T.);
#75881=ADVANCED_FACE('',(#20451),#2582,.F.);
#75882=ADVANCED_FACE('',(#20452),#2583,.F.);
#75883=ADVANCED_FACE('',(#20453),#2584,.T.);
#75884=ADVANCED_FACE('',(#20454),#175,.T.);
#75885=ADVANCED_FACE('',(#20455),#2585,.F.);
#75886=ADVANCED_FACE('',(#20456),#1868,.F.);
#75887=ADVANCED_FACE('',(#20457),#75295,.F.);
#75888=ADVANCED_FACE('',(#20458),#2134,.F.);
#75889=ADVANCED_FACE('',(#20459),#2586,.F.);
#75890=ADVANCED_FACE('',(#20460),#2587,.F.);
#75891=ADVANCED_FACE('',(#20461),#2135,.T.);
#75892=ADVANCED_FACE('',(#20462),#2588,.F.);
#75893=ADVANCED_FACE('',(#20463),#2589,.T.);
#75894=ADVANCED_FACE('',(#20464),#1869,.F.);
#75895=ADVANCED_FACE('',(#20465),#2136,.F.);
#75896=ADVANCED_FACE('',(#20466),#2590,.F.);
#75897=ADVANCED_FACE('',(#20467),#2591,.T.);
#75898=ADVANCED_FACE('',(#20468),#2592,.F.);
#75899=ADVANCED_FACE('',(#20469),#75296,.F.);
#75900=ADVANCED_FACE('',(#20470),#2593,.F.);
#75901=ADVANCED_FACE('',(#20471),#2594,.F.);
#75902=ADVANCED_FACE('',(#20472),#2137,.T.);
#75903=ADVANCED_FACE('',(#20473),#2138,.T.);
#75904=ADVANCED_FACE('',(#20474),#2139,.T.);
#75905=ADVANCED_FACE('',(#20475),#2595,.F.);
#75906=ADVANCED_FACE('',(#20476),#2140,.F.);
#75907=ADVANCED_FACE('',(#20477),#1870,.T.);
#75908=ADVANCED_FACE('',(#20478),#2596,.F.);
#75909=ADVANCED_FACE('',(#20479),#2141,.F.);
#75910=ADVANCED_FACE('',(#20480),#2142,.F.);
#75911=ADVANCED_FACE('',(#20481),#2597,.T.);
#75912=ADVANCED_FACE('',(#20482),#2143,.T.);
#75913=ADVANCED_FACE('',(#20483),#1871,.T.);
#75914=ADVANCED_FACE('',(#20484),#2598,.F.);
#75915=ADVANCED_FACE('',(#20485),#2144,.F.);
#75916=ADVANCED_FACE('',(#20486),#2599,.T.);
#75917=ADVANCED_FACE('',(#20487),#1872,.F.);
#75918=ADVANCED_FACE('',(#20488),#1873,.F.);
#75919=ADVANCED_FACE('',(#20489),#2145,.F.);
#75920=ADVANCED_FACE('',(#20490),#2600,.F.);
#75921=ADVANCED_FACE('',(#20491),#2601,.T.);
#75922=ADVANCED_FACE('',(#20492),#2602,.T.);
#75923=ADVANCED_FACE('',(#20493),#2603,.T.);
#75924=ADVANCED_FACE('',(#20494),#2604,.F.);
#75925=ADVANCED_FACE('',(#20495),#16914,.T.);
#75926=ADVANCED_FACE('',(#20496),#2605,.T.);
#75927=ADVANCED_FACE('',(#20497),#2606,.F.);
#75928=ADVANCED_FACE('',(#20498),#1874,.F.);
#75929=ADVANCED_FACE('',(#20499),#2146,.F.);
#75930=ADVANCED_FACE('',(#20500),#2607,.T.);
#75931=ADVANCED_FACE('',(#20501),#2147,.F.);
#75932=ADVANCED_FACE('',(#20502),#2608,.T.);
#75933=ADVANCED_FACE('',(#20503),#1875,.F.);
#75934=ADVANCED_FACE('',(#20504),#1876,.F.);
#75935=ADVANCED_FACE('',(#20505),#2609,.F.);
#75936=ADVANCED_FACE('',(#20506),#2610,.F.);
#75937=ADVANCED_FACE('',(#20507),#2611,.F.);
#75938=ADVANCED_FACE('',(#20508),#2612,.F.);
#75939=ADVANCED_FACE('',(#20509),#2148,.F.);
#75940=ADVANCED_FACE('',(#20510),#2613,.T.);
#75941=ADVANCED_FACE('',(#20511),#2614,.T.);
#75942=ADVANCED_FACE('',(#20512),#1877,.T.);
#75943=ADVANCED_FACE('',(#20513),#16915,.T.);
#75944=ADVANCED_FACE('',(#20514),#2149,.T.);
#79318=CLOSED_SHELL('',(#75303,#75304,#75305,#75306,#75307,#75308,#75309));
#79319=CLOSED_SHELL('',(#75310,#75311,#75312,#75313,#75314,#75315,#75316));
#79320=CLOSED_SHELL('',(#75317,#75318,#75319,#75320,#75321,#75322,#75323,
#75324,#75325,#75326));
#79321=CLOSED_SHELL('',(#75327,#75328,#75329,#75330,#75331,#75332,#75333,
#75334,#75335,#75336));
#79322=CLOSED_SHELL('',(#75337,#75338,#75339,#75340,#75341,#75342,#75343,
#75344,#75345,#75346,#75347,#75348,#75349,#75350,#75351,#75352,#75353,#75354,
#75355,#75356,#75357,#75358,#75359,#75360,#75361,#75362,#75363,#75364,#75365,
#75366,#75367,#75368,#75369,#75370,#75371,#75372,#75373,#75374,#75375,#75376,
#75377,#75378,#75379,#75380,#75381,#75382,#75383,#75384,#75385,#75386,#75387,
#75388,#75389,#75390,#75391,#75392,#75393,#75394,#75395,#75396,#75397,#75398,
#75399,#75400,#75401,#75402,#75403,#75404,#75405,#75406,#75407,#75408,#75409,
#75410,#75411,#75412,#75413,#75414,#75415,#75416,#75417,#75418,#75419,#75420,
#75421,#75422,#75423,#75424,#75425,#75426,#75427,#75428,#75429,#75430,#75431,
#75432,#75433,#75434,#75435,#75436,#75437,#75438,#75439,#75440,#75441,#75442,
#75443,#75444,#75445,#75446,#75447,#75448,#75449,#75450,#75451,#75452,#75453,
#75454,#75455,#75456,#75457,#75458,#75459,#75460,#75461,#75462,#75463,#75464,
#75465,#75466,#75467,#75468,#75469,#75470,#75471,#75472,#75473,#75474,#75475,
#75476,#75477,#75478,#75479,#75480,#75481,#75482,#75483,#75484,#75485,#75486,
#75487,#75488,#75489,#75490,#75491,#75492,#75493,#75494,#75495,#75496,#75497,
#75498,#75499,#75500,#75501,#75502,#75503,#75504,#75505,#75506,#75507,#75508,
#75509,#75510,#75511,#75512,#75513,#75514,#75515,#75516,#75517,#75518,#75519,
#75520,#75521,#75522,#75523,#75524,#75525,#75526,#75527,#75528,#75529,#75530,
#75531,#75532,#75533,#75534,#75535,#75536,#75537,#75538,#75539,#75540,#75541,
#75542,#75543,#75544,#75545,#75546,#75547,#75548,#75549,#75550,#75551,#75552,
#75553,#75554,#75555,#75556,#75557,#75558,#75559,#75560,#75561,#75562,#75563,
#75564,#75565,#75566,#75567,#75568,#75569,#75570,#75571,#75572,#75573,#75574,
#75575,#75576,#75577,#75578,#75579,#75580,#75581,#75582,#75583,#75584,#75585,
#75586,#75587,#75588,#75589,#75590,#75591,#75592,#75593,#75594,#75595,#75596,
#75597,#75598,#75599,#75600,#75601,#75602,#75603,#75604,#75605,#75606,#75607,
#75608,#75609,#75610,#75611,#75612,#75613,#75614,#75615,#75616,#75617,#75618,
#75619,#75620,#75621,#75622,#75623,#75624,#75625,#75626,#75627,#75628,#75629,
#75630,#75631,#75632,#75633,#75634,#75635,#75636,#75637,#75638,#75639,#75640,
#75641,#75642,#75643,#75644,#75645,#75646,#75647,#75648,#75649,#75650,#75651,
#75652,#75653,#75654,#75655,#75656,#75657,#75658,#75659,#75660,#75661,#75662,
#75663,#75664,#75665,#75666,#75667,#75668,#75669,#75670,#75671,#75672,#75673,
#75674,#75675,#75676,#75677,#75678,#75679,#75680,#75681,#75682,#75683,#75684,
#75685,#75686,#75687,#75688,#75689,#75690,#75691,#75692,#75693,#75694,#75695,
#75696,#75697,#75698,#75699,#75700,#75701,#75702,#75703,#75704,#75705,#75706,
#75707,#75708,#75709,#75710,#75711,#75712,#75713,#75714,#75715,#75716,#75717,
#75718,#75719,#75720,#75721,#75722,#75723,#75724,#75725,#75726,#75727,#75728,
#75729,#75730,#75731,#75732,#75733,#75734,#75735,#75736,#75737,#75738,#75739,
#75740,#75741,#75742,#75743,#75744,#75745,#75746,#75747,#75748,#75749,#75750,
#75751,#75752,#75753,#75754,#75755,#75756,#75757,#75758,#75759,#75760,#75761,
#75762,#75763,#75764,#75765,#75766,#75767,#75768,#75769,#75770,#75771,#75772,
#75773,#75774,#75775,#75776,#75777,#75778,#75779,#75780,#75781,#75782,#75783,
#75784,#75785,#75786,#75787,#75788,#75789,#75790,#75791,#75792,#75793,#75794,
#75795,#75796,#75797,#75798,#75799,#75800,#75801,#75802,#75803,#75804,#75805,
#75806,#75807,#75808,#75809,#75810,#75811,#75812,#75813,#75814,#75815,#75816,
#75817,#75818,#75819,#75820,#75821,#75822,#75823,#75824,#75825,#75826,#75827,
#75828,#75829,#75830,#75831,#75832,#75833,#75834,#75835,#75836,#75837,#75838,
#75839,#75840,#75841,#75842,#75843,#75844,#75845,#75846,#75847,#75848,#75849,
#75850,#75851,#75852,#75853,#75854,#75855,#75856,#75857,#75858,#75859,#75860,
#75861,#75862,#75863,#75864,#75865,#75866,#75867,#75868,#75869,#75870,#75871,
#75872,#75873,#75874,#75875,#75876,#75877,#75878,#75879,#75880,#75881,#75882,
#75883,#75884,#75885,#75886,#75887,#75888,#75889,#75890,#75891,#75892,#75893,
#75894,#75895,#75896,#75897,#75898,#75899,#75900,#75901,#75902,#75903,#75904,
#75905,#75906,#75907,#75908,#75909,#75910,#75911,#75912,#75913,#75914,#75915,
#75916,#75917,#75918,#75919,#75920,#75921,#75922,#75923,#75924,#75925,#75926,
#75927,#75928,#75929,#75930,#75931,#75932,#75933,#75934,#75935,#75936,#75937,
#75938,#75939,#75940,#75941,#75942,#75943,#75944));
#79336=BREP_WITH_VOIDS('Body1',#79322,(#1975,#1976,#1977,#1978));
#79483=AXIS2_PLACEMENT_3D('',#106596,#86166,#86167);
#79484=AXIS2_PLACEMENT_3D('',#106597,#86168,#86169);
#79485=AXIS2_PLACEMENT_3D('',#106600,#86170,#86171);
#79486=AXIS2_PLACEMENT_3D('',#106602,#86172,#86173);
#79487=AXIS2_PLACEMENT_3D('',#106604,#86174,#86175);
#79488=AXIS2_PLACEMENT_3D('',#106611,#86176,#86177);
#79489=AXIS2_PLACEMENT_3D('',#106616,#86180,#86181);
#79490=AXIS2_PLACEMENT_3D('',#106865,#86182,#86183);
#79491=AXIS2_PLACEMENT_3D('',#106876,#86184,#86185);
#79492=AXIS2_PLACEMENT_3D('',#106877,#86186,#86187);
#79493=AXIS2_PLACEMENT_3D('',#106880,#86188,#86189);
#79494=AXIS2_PLACEMENT_3D('',#106882,#86190,#86191);
#79495=AXIS2_PLACEMENT_3D('',#106884,#86192,#86193);
#79496=AXIS2_PLACEMENT_3D('',#106946,#86194,#86195);
#79497=AXIS2_PLACEMENT_3D('',#106948,#86196,#86197);
#79498=AXIS2_PLACEMENT_3D('',#107141,#86200,#86201);
#79499=AXIS2_PLACEMENT_3D('',#107152,#86202,#86203);
#79500=AXIS2_PLACEMENT_3D('',#107153,#86204,#86205);
#79501=AXIS2_PLACEMENT_3D('',#107192,#86206,#86207);
#79502=AXIS2_PLACEMENT_3D('',#107576,#86209,#86210);
#79503=AXIS2_PLACEMENT_3D('',#107757,#86211,#86212);
#79504=AXIS2_PLACEMENT_3D('',#107760,#86215,#86216);
#79505=AXIS2_PLACEMENT_3D('',#107983,#86217,#86218);
#79506=AXIS2_PLACEMENT_3D('',#108205,#86219,#86220);
#79507=AXIS2_PLACEMENT_3D('',#108206,#86221,#86222);
#79508=AXIS2_PLACEMENT_3D('',#108209,#86223,#86224);
#79509=AXIS2_PLACEMENT_3D('',#108280,#86226,#86227);
#79510=AXIS2_PLACEMENT_3D('',#108283,#86228,#86229);
#79511=AXIS2_PLACEMENT_3D('',#108824,#86230,#86231);
#79512=AXIS2_PLACEMENT_3D('',#108826,#86233,#86234);
#79513=AXIS2_PLACEMENT_3D('',#108896,#86236,#86237);
#79514=AXIS2_PLACEMENT_3D('',#109121,#86238,#86239);
#79515=AXIS2_PLACEMENT_3D('',#109122,#86240,#86241);
#79516=AXIS2_PLACEMENT_3D('',#109172,#86243,#86244);
#79517=AXIS2_PLACEMENT_3D('',#109197,#86245,#86246);
#79518=AXIS2_PLACEMENT_3D('',#109323,#86248,#86249);
#79519=AXIS2_PLACEMENT_3D('',#109438,#86251,#86252);
#79520=AXIS2_PLACEMENT_3D('',#109456,#86254,#86255);
#79521=AXIS2_PLACEMENT_3D('',#109488,#86256,#86257);
#79522=AXIS2_PLACEMENT_3D('',#109601,#86259,#86260);
#79523=AXIS2_PLACEMENT_3D('',#109631,#86262,#86263);
#79524=AXIS2_PLACEMENT_3D('',#109678,#86264,#86265);
#79525=AXIS2_PLACEMENT_3D('',#109765,#86268,#86269);
#79526=AXIS2_PLACEMENT_3D('',#109993,#86271,#86272);
#79527=AXIS2_PLACEMENT_3D('',#110219,#86274,#86275);
#79528=AXIS2_PLACEMENT_3D('',#110451,#86277,#86278);
#79529=AXIS2_PLACEMENT_3D('',#110456,#86280,#86281);
#79530=AXIS2_PLACEMENT_3D('',#110483,#86282,#86283);
#79531=AXIS2_PLACEMENT_3D('',#110650,#86287,#86288);
#79532=AXIS2_PLACEMENT_3D('',#110651,#86289,#86290);
#79533=AXIS2_PLACEMENT_3D('',#110784,#86291,#86292);
#79534=AXIS2_PLACEMENT_3D('',#111044,#86294,#86295);
#79535=AXIS2_PLACEMENT_3D('',#111152,#86297,#86298);
#79536=AXIS2_PLACEMENT_3D('',#111299,#86299,#86300);
#79537=AXIS2_PLACEMENT_3D('',#111301,#86301,#86302);
#79538=AXIS2_PLACEMENT_3D('',#111302,#86303,#86304);
#79539=AXIS2_PLACEMENT_3D('',#111303,#86305,#86306);
#79540=AXIS2_PLACEMENT_3D('',#111306,#86307,#86308);
#79541=AXIS2_PLACEMENT_3D('',#111366,#86309,#86310);
#79542=AXIS2_PLACEMENT_3D('',#111388,#86311,#86312);
#79543=AXIS2_PLACEMENT_3D('',#111447,#86313,#86314);
#79544=AXIS2_PLACEMENT_3D('',#111450,#86315,#86316);
#79545=AXIS2_PLACEMENT_3D('',#111452,#86317,#86318);
#79546=AXIS2_PLACEMENT_3D('',#111454,#86319,#86320);
#79547=AXIS2_PLACEMENT_3D('',#111456,#86321,#86322);
#79548=AXIS2_PLACEMENT_3D('',#111457,#86323,#86324);
#79549=AXIS2_PLACEMENT_3D('',#111458,#86325,#86326);
#79550=AXIS2_PLACEMENT_3D('',#111461,#86327,#86328);
#79551=AXIS2_PLACEMENT_3D('',#111493,#86331,#86332);
#79552=AXIS2_PLACEMENT_3D('',#111496,#86333,#86334);
#79553=AXIS2_PLACEMENT_3D('',#111571,#86335,#86336);
#79554=AXIS2_PLACEMENT_3D('',#111572,#86337,#86338);
#79555=AXIS2_PLACEMENT_3D('',#111573,#86339,#86340);
#79556=AXIS2_PLACEMENT_3D('',#111576,#86341,#86342);
#79557=AXIS2_PLACEMENT_3D('',#111580,#86344,#86345);
#79558=AXIS2_PLACEMENT_3D('',#111582,#86347,#86348);
#79559=AXIS2_PLACEMENT_3D('',#111585,#86349,#86350);
#79560=AXIS2_PLACEMENT_3D('',#111588,#86352,#86353);
#79561=AXIS2_PLACEMENT_3D('',#111589,#86354,#86355);
#79562=AXIS2_PLACEMENT_3D('',#111590,#86356,#86357);
#79563=AXIS2_PLACEMENT_3D('',#111592,#86358,#86359);
#79564=AXIS2_PLACEMENT_3D('',#111593,#86360,#86361);
#79565=AXIS2_PLACEMENT_3D('',#111594,#86362,#86363);
#79566=AXIS2_PLACEMENT_3D('',#111597,#86364,#86365);
#79567=AXIS2_PLACEMENT_3D('',#111600,#86367,#86368);
#79568=AXIS2_PLACEMENT_3D('',#111601,#86369,#86370);
#79569=AXIS2_PLACEMENT_3D('',#111602,#86371,#86372);
#79570=AXIS2_PLACEMENT_3D('',#111604,#86373,#86374);
#79571=AXIS2_PLACEMENT_3D('',#111605,#86375,#86376);
#79572=AXIS2_PLACEMENT_3D('',#111606,#86377,#86378);
#79573=AXIS2_PLACEMENT_3D('',#111609,#86379,#86380);
#79574=AXIS2_PLACEMENT_3D('',#111611,#86381,#86382);
#79575=AXIS2_PLACEMENT_3D('',#111613,#86383,#86384);
#79576=AXIS2_PLACEMENT_3D('',#111614,#86385,#86386);
#79577=AXIS2_PLACEMENT_3D('',#111615,#86387,#86388);
#79578=AXIS2_PLACEMENT_3D('',#111652,#86391,#86392);
#79579=AXIS2_PLACEMENT_3D('',#112254,#86393,#86394);
#79580=AXIS2_PLACEMENT_3D('',#112257,#86396,#86397);
#79581=AXIS2_PLACEMENT_3D('',#112259,#86398,#86399);
#79582=AXIS2_PLACEMENT_3D('',#112933,#86400,#86401);
#79583=AXIS2_PLACEMENT_3D('',#112936,#86402,#86403);
#79584=AXIS2_PLACEMENT_3D('',#112937,#86404,#86405);
#79585=AXIS2_PLACEMENT_3D('',#112938,#86406,#86407);
#79586=AXIS2_PLACEMENT_3D('',#112939,#86408,#86409);
#79587=AXIS2_PLACEMENT_3D('',#113348,#86412,#86413);
#79588=AXIS2_PLACEMENT_3D('',#113351,#86414,#86415);
#79589=AXIS2_PLACEMENT_3D('',#113353,#86416,#86417);
#79590=AXIS2_PLACEMENT_3D('',#113355,#86418,#86419);
#79591=AXIS2_PLACEMENT_3D('',#113357,#86420,#86421);
#79592=AXIS2_PLACEMENT_3D('',#113358,#86422,#86423);
#79593=AXIS2_PLACEMENT_3D('',#113359,#86424,#86425);
#79594=AXIS2_PLACEMENT_3D('',#113360,#86426,#86427);
#79595=AXIS2_PLACEMENT_3D('',#113371,#86429,#86430);
#79596=AXIS2_PLACEMENT_3D('',#113378,#86431,#86432);
#79597=AXIS2_PLACEMENT_3D('',#113380,#86433,#86434);
#79598=AXIS2_PLACEMENT_3D('',#113382,#86435,#86436);
#79599=AXIS2_PLACEMENT_3D('',#113384,#86437,#86438);
#79600=AXIS2_PLACEMENT_3D('',#113385,#86439,#86440);
#79601=AXIS2_PLACEMENT_3D('',#113386,#86441,#86442);
#79602=AXIS2_PLACEMENT_3D('',#113389,#86444,#86445);
#79603=AXIS2_PLACEMENT_3D('',#113390,#86446,#86447);
#79604=AXIS2_PLACEMENT_3D('',#113392,#86448,#86449);
#79605=AXIS2_PLACEMENT_3D('',#113396,#86451,#86452);
#79606=AXIS2_PLACEMENT_3D('',#113408,#86453,#86454);
#79607=AXIS2_PLACEMENT_3D('',#113409,#86455,#86456);
#79608=AXIS2_PLACEMENT_3D('',#113412,#86457,#86458);
#79609=AXIS2_PLACEMENT_3D('',#113429,#86459,#86460);
#79610=AXIS2_PLACEMENT_3D('',#113432,#86462,#86463);
#79611=AXIS2_PLACEMENT_3D('',#113434,#86464,#86465);
#79612=AXIS2_PLACEMENT_3D('',#113449,#86466,#86467);
#79613=AXIS2_PLACEMENT_3D('',#113451,#86468,#86469);
#79614=AXIS2_PLACEMENT_3D('',#113455,#86471,#86472);
#79615=AXIS2_PLACEMENT_3D('',#113456,#86473,#86474);
#79616=AXIS2_PLACEMENT_3D('',#113457,#86475,#86476);
#79617=AXIS2_PLACEMENT_3D('',#113460,#86478,#86479);
#79618=AXIS2_PLACEMENT_3D('',#113461,#86480,#86481);
#79619=AXIS2_PLACEMENT_3D('',#113463,#86482,#86483);
#79620=AXIS2_PLACEMENT_3D('',#113466,#86485,#86486);
#79621=AXIS2_PLACEMENT_3D('',#113467,#86487,#86488);
#79622=AXIS2_PLACEMENT_3D('',#113469,#86489,#86490);
#79623=AXIS2_PLACEMENT_3D('',#113473,#86492,#86493);
#79624=AXIS2_PLACEMENT_3D('',#113492,#86494,#86495);
#79625=AXIS2_PLACEMENT_3D('',#113494,#86496,#86497);
#79626=AXIS2_PLACEMENT_3D('',#113512,#86498,#86499);
#79627=AXIS2_PLACEMENT_3D('',#113513,#86500,#86501);
#79628=AXIS2_PLACEMENT_3D('',#113516,#86502,#86503);
#79629=AXIS2_PLACEMENT_3D('',#113517,#86504,#86505);
#79630=AXIS2_PLACEMENT_3D('',#113519,#86506,#86507);
#79631=AXIS2_PLACEMENT_3D('',#113520,#86508,#86509);
#79632=AXIS2_PLACEMENT_3D('',#113521,#86510,#86511);
#79633=AXIS2_PLACEMENT_3D('',#113523,#86512,#86513);
#79634=AXIS2_PLACEMENT_3D('',#113525,#86515,#86516);
#79635=AXIS2_PLACEMENT_3D('',#113528,#86517,#86518);
#79636=AXIS2_PLACEMENT_3D('',#113531,#86520,#86521);
#79637=AXIS2_PLACEMENT_3D('',#113532,#86522,#86523);
#79638=AXIS2_PLACEMENT_3D('',#113533,#86524,#86525);
#79639=AXIS2_PLACEMENT_3D('',#113536,#86526,#86527);
#79640=AXIS2_PLACEMENT_3D('',#113537,#86528,#86529);
#79641=AXIS2_PLACEMENT_3D('',#113539,#86531,#86532);
#79642=AXIS2_PLACEMENT_3D('',#113542,#86533,#86534);
#79643=AXIS2_PLACEMENT_3D('',#113600,#86535,#86536);
#79644=AXIS2_PLACEMENT_3D('',#113659,#86537,#86538);
#79645=AXIS2_PLACEMENT_3D('',#113662,#86539,#86540);
#79646=AXIS2_PLACEMENT_3D('',#113666,#86542,#86543);
#79647=AXIS2_PLACEMENT_3D('',#113668,#86545,#86546);
#79648=AXIS2_PLACEMENT_3D('',#113925,#86547,#86548);
#79649=AXIS2_PLACEMENT_3D('',#113928,#86549,#86550);
#79650=AXIS2_PLACEMENT_3D('',#113931,#86552,#86553);
#79651=AXIS2_PLACEMENT_3D('',#113932,#86554,#86555);
#79652=AXIS2_PLACEMENT_3D('',#113933,#86556,#86557);
#79653=AXIS2_PLACEMENT_3D('',#113935,#86559,#86560);
#79654=AXIS2_PLACEMENT_3D('',#113937,#86561,#86562);
#79655=AXIS2_PLACEMENT_3D('',#113961,#86564,#86565);
#79656=AXIS2_PLACEMENT_3D('',#113998,#86566,#86567);
#79657=AXIS2_PLACEMENT_3D('',#114225,#86568,#86569);
#79658=AXIS2_PLACEMENT_3D('',#114227,#86570,#86571);
#79659=AXIS2_PLACEMENT_3D('',#114229,#86572,#86573);
#79660=AXIS2_PLACEMENT_3D('',#114231,#86574,#86575);
#79661=AXIS2_PLACEMENT_3D('',#114232,#86576,#86577);
#79662=AXIS2_PLACEMENT_3D('',#114233,#86578,#86579);
#79663=AXIS2_PLACEMENT_3D('',#114236,#86581,#86582);
#79664=AXIS2_PLACEMENT_3D('',#114237,#86583,#86584);
#79665=AXIS2_PLACEMENT_3D('',#114288,#86585,#86586);
#79666=AXIS2_PLACEMENT_3D('',#114289,#86587,#86588);
#79667=AXIS2_PLACEMENT_3D('',#114412,#86589,#86590);
#79668=AXIS2_PLACEMENT_3D('',#114915,#86592,#86593);
#79669=AXIS2_PLACEMENT_3D('',#115275,#86594,#86595);
#79670=AXIS2_PLACEMENT_3D('',#115278,#86596,#86597);
#79671=AXIS2_PLACEMENT_3D('',#115282,#86599,#86600);
#79672=AXIS2_PLACEMENT_3D('',#115456,#86603,#86604);
#79673=AXIS2_PLACEMENT_3D('',#115459,#86605,#86606);
#79674=AXIS2_PLACEMENT_3D('',#115605,#86609,#86610);
#79675=AXIS2_PLACEMENT_3D('',#115607,#86611,#86612);
#79676=AXIS2_PLACEMENT_3D('',#115610,#86614,#86615);
#79677=AXIS2_PLACEMENT_3D('',#115611,#86616,#86617);
#79678=AXIS2_PLACEMENT_3D('',#115614,#86618,#86619);
#79679=AXIS2_PLACEMENT_3D('',#115617,#86621,#86622);
#79680=AXIS2_PLACEMENT_3D('',#115618,#86623,#86624);
#79681=AXIS2_PLACEMENT_3D('',#115619,#86625,#86626);
#79682=AXIS2_PLACEMENT_3D('',#115622,#86628,#86629);
#79683=AXIS2_PLACEMENT_3D('',#115623,#86630,#86631);
#79684=AXIS2_PLACEMENT_3D('',#115626,#86632,#86633);
#79685=AXIS2_PLACEMENT_3D('',#115630,#86635,#86636);
#79686=AXIS2_PLACEMENT_3D('',#115631,#86637,#86638);
#79687=AXIS2_PLACEMENT_3D('',#115632,#86639,#86640);
#79688=AXIS2_PLACEMENT_3D('',#115633,#86641,#86642);
#79689=AXIS2_PLACEMENT_3D('',#115663,#86644,#86645);
#79690=AXIS2_PLACEMENT_3D('',#115666,#86647,#86648);
#79691=AXIS2_PLACEMENT_3D('',#115667,#86649,#86650);
#79692=AXIS2_PLACEMENT_3D('',#115670,#86651,#86652);
#79693=AXIS2_PLACEMENT_3D('',#115671,#86653,#86654);
#79694=AXIS2_PLACEMENT_3D('',#115673,#86655,#86656);
#79695=AXIS2_PLACEMENT_3D('',#115674,#86657,#86658);
#79696=AXIS2_PLACEMENT_3D('',#115675,#86659,#86660);
#79697=AXIS2_PLACEMENT_3D('',#115677,#86661,#86662);
#79698=AXIS2_PLACEMENT_3D('',#115679,#86664,#86665);
#79699=AXIS2_PLACEMENT_3D('',#115717,#86666,#86667);
#79700=AXIS2_PLACEMENT_3D('',#115731,#86668,#86669);
#79701=AXIS2_PLACEMENT_3D('',#115765,#86670,#86671);
#79702=AXIS2_PLACEMENT_3D('',#115778,#86672,#86673);
#79703=AXIS2_PLACEMENT_3D('',#116094,#86675,#86676);
#79704=AXIS2_PLACEMENT_3D('',#116638,#86677,#86678);
#79705=AXIS2_PLACEMENT_3D('',#116709,#86680,#86681);
#79706=AXIS2_PLACEMENT_3D('',#116713,#86683,#86684);
#79707=AXIS2_PLACEMENT_3D('',#116715,#86686,#86687);
#79708=AXIS2_PLACEMENT_3D('',#116750,#86689,#86690);
#79709=AXIS2_PLACEMENT_3D('',#116752,#86692,#86693);
#79710=AXIS2_PLACEMENT_3D('',#116754,#86694,#86695);
#79711=AXIS2_PLACEMENT_3D('',#116757,#86697,#86698);
#79712=AXIS2_PLACEMENT_3D('',#116758,#86699,#86700);
#79713=AXIS2_PLACEMENT_3D('',#116761,#86701,#86702);
#79714=AXIS2_PLACEMENT_3D('',#116764,#86704,#86705);
#79715=AXIS2_PLACEMENT_3D('',#116765,#86706,#86707);
#79716=AXIS2_PLACEMENT_3D('',#116766,#86708,#86709);
#79717=AXIS2_PLACEMENT_3D('',#116769,#86711,#86712);
#79718=AXIS2_PLACEMENT_3D('',#116770,#86713,#86714);
#79719=AXIS2_PLACEMENT_3D('',#116773,#86715,#86716);
#79720=AXIS2_PLACEMENT_3D('',#116777,#86718,#86719);
#79721=AXIS2_PLACEMENT_3D('',#116778,#86720,#86721);
#79722=AXIS2_PLACEMENT_3D('',#116779,#86722,#86723);
#79723=AXIS2_PLACEMENT_3D('',#116780,#86724,#86725);
#79724=AXIS2_PLACEMENT_3D('',#116810,#86727,#86728);
#79725=AXIS2_PLACEMENT_3D('',#116813,#86730,#86731);
#79726=AXIS2_PLACEMENT_3D('',#116814,#86732,#86733);
#79727=AXIS2_PLACEMENT_3D('',#116827,#86740,#86741);
#79728=AXIS2_PLACEMENT_3D('',#116830,#86744,#86745);
#79729=AXIS2_PLACEMENT_3D('',#116832,#86747,#86748);
#79730=AXIS2_PLACEMENT_3D('',#116834,#86750,#86751);
#79731=AXIS2_PLACEMENT_3D('',#116836,#86753,#86754);
#79732=AXIS2_PLACEMENT_3D('',#116838,#86756,#86757);
#79733=AXIS2_PLACEMENT_3D('',#116839,#86758,#86759);
#79734=AXIS2_PLACEMENT_3D('',#116840,#86760,#86761);
#79735=AXIS2_PLACEMENT_3D('',#116841,#86762,#86763);
#79736=AXIS2_PLACEMENT_3D('',#116846,#86765,#86766);
#79737=AXIS2_PLACEMENT_3D('',#116849,#86768,#86769);
#79738=AXIS2_PLACEMENT_3D('',#117050,#86770,#86771);
#79739=AXIS2_PLACEMENT_3D('',#117058,#86772,#86773);
#79740=AXIS2_PLACEMENT_3D('',#117059,#86774,#86775);
#79741=AXIS2_PLACEMENT_3D('',#117061,#86776,#86777);
#79742=AXIS2_PLACEMENT_3D('',#117107,#86778,#86779);
#79743=AXIS2_PLACEMENT_3D('',#117109,#86780,#86781);
#79744=AXIS2_PLACEMENT_3D('',#117110,#86782,#86783);
#79745=AXIS2_PLACEMENT_3D('',#117111,#86784,#86785);
#79746=AXIS2_PLACEMENT_3D('',#117117,#86788,#86789);
#79747=AXIS2_PLACEMENT_3D('',#117274,#86791,#86792);
#79748=AXIS2_PLACEMENT_3D('',#117355,#86793,#86794);
#79749=AXIS2_PLACEMENT_3D('',#117358,#86796,#86797);
#79750=AXIS2_PLACEMENT_3D('',#117359,#86798,#86799);
#79751=AXIS2_PLACEMENT_3D('',#117362,#86800,#86801);
#79752=AXIS2_PLACEMENT_3D('',#117408,#86803,#86804);
#79753=AXIS2_PLACEMENT_3D('',#117488,#86805,#86806);
#79754=AXIS2_PLACEMENT_3D('',#117506,#86808,#86809);
#79755=AXIS2_PLACEMENT_3D('',#117508,#86811,#86812);
#79756=AXIS2_PLACEMENT_3D('',#117511,#86814,#86815);
#79757=AXIS2_PLACEMENT_3D('',#117614,#86816,#86817);
#79758=AXIS2_PLACEMENT_3D('',#117617,#86818,#86819);
#79759=AXIS2_PLACEMENT_3D('',#117776,#86822,#86823);
#79760=AXIS2_PLACEMENT_3D('',#117923,#86824,#86825);
#79761=AXIS2_PLACEMENT_3D('',#118018,#86826,#86827);
#79762=AXIS2_PLACEMENT_3D('',#118197,#86828,#86829);
#79763=AXIS2_PLACEMENT_3D('',#118199,#86830,#86831);
#79764=AXIS2_PLACEMENT_3D('',#118201,#86832,#86833);
#79765=AXIS2_PLACEMENT_3D('',#118203,#86834,#86835);
#79766=AXIS2_PLACEMENT_3D('',#118204,#86836,#86837);
#79767=AXIS2_PLACEMENT_3D('',#118205,#86838,#86839);
#79768=AXIS2_PLACEMENT_3D('',#118207,#86840,#86841);
#79769=AXIS2_PLACEMENT_3D('',#118208,#86842,#86843);
#79770=AXIS2_PLACEMENT_3D('',#118209,#86844,#86845);
#79771=AXIS2_PLACEMENT_3D('',#118212,#86846,#86847);
#79772=AXIS2_PLACEMENT_3D('',#118213,#86848,#86849);
#79773=AXIS2_PLACEMENT_3D('',#118214,#86850,#86851);
#79774=AXIS2_PLACEMENT_3D('',#118310,#86852,#86853);
#79775=AXIS2_PLACEMENT_3D('',#118954,#86854,#86855);
#79776=AXIS2_PLACEMENT_3D('',#118956,#86857,#86858);
#79777=AXIS2_PLACEMENT_3D('',#118958,#86859,#86860);
#79778=AXIS2_PLACEMENT_3D('',#118960,#86861,#86862);
#79779=AXIS2_PLACEMENT_3D('',#118961,#86863,#86864);
#79780=AXIS2_PLACEMENT_3D('',#118962,#86865,#86866);
#79781=AXIS2_PLACEMENT_3D('',#118964,#86867,#86868);
#79782=AXIS2_PLACEMENT_3D('',#118965,#86869,#86870);
#79783=AXIS2_PLACEMENT_3D('',#118966,#86871,#86872);
#79784=AXIS2_PLACEMENT_3D('',#118967,#86873,#86874);
#79785=AXIS2_PLACEMENT_3D('',#118968,#86875,#86876);
#79786=AXIS2_PLACEMENT_3D('',#118969,#86877,#86878);
#79787=AXIS2_PLACEMENT_3D('',#118997,#86880,#86881);
#79788=AXIS2_PLACEMENT_3D('',#118998,#86882,#86883);
#79789=AXIS2_PLACEMENT_3D('',#118999,#86884,#86885);
#79790=AXIS2_PLACEMENT_3D('',#119001,#86886,#86887);
#79791=AXIS2_PLACEMENT_3D('',#119002,#86888,#86889);
#79792=AXIS2_PLACEMENT_3D('',#119269,#86890,#86891);
#79793=AXIS2_PLACEMENT_3D('',#119270,#86892,#86893);
#79794=AXIS2_PLACEMENT_3D('',#119271,#86894,#86895);
#79795=AXIS2_PLACEMENT_3D('',#119356,#86896,#86897);
#79796=AXIS2_PLACEMENT_3D('',#119358,#86899,#86900);
#79797=AXIS2_PLACEMENT_3D('',#119360,#86901,#86902);
#79798=AXIS2_PLACEMENT_3D('',#119362,#86903,#86904);
#79799=AXIS2_PLACEMENT_3D('',#119363,#86905,#86906);
#79800=AXIS2_PLACEMENT_3D('',#119364,#86907,#86908);
#79801=AXIS2_PLACEMENT_3D('',#119366,#86909,#86910);
#79802=AXIS2_PLACEMENT_3D('',#119367,#86911,#86912);
#79803=AXIS2_PLACEMENT_3D('',#119368,#86913,#86914);
#79804=AXIS2_PLACEMENT_3D('',#119370,#86915,#86916);
#79805=AXIS2_PLACEMENT_3D('',#119371,#86917,#86918);
#79806=AXIS2_PLACEMENT_3D('',#119372,#86919,#86920);
#79807=AXIS2_PLACEMENT_3D('',#119489,#86922,#86923);
#79808=AXIS2_PLACEMENT_3D('',#119491,#86925,#86926);
#79809=AXIS2_PLACEMENT_3D('',#119492,#86927,#86928);
#79810=AXIS2_PLACEMENT_3D('',#119493,#86929,#86930);
#79811=AXIS2_PLACEMENT_3D('',#119494,#86931,#86932);
#79812=AXIS2_PLACEMENT_3D('',#119495,#86933,#86934);
#79813=AXIS2_PLACEMENT_3D('',#119496,#86935,#86936);
#79814=AXIS2_PLACEMENT_3D('',#119497,#86937,#86938);
#79815=AXIS2_PLACEMENT_3D('',#119624,#86940,#86941);
#79816=AXIS2_PLACEMENT_3D('',#119648,#86942,#86943);
#79817=AXIS2_PLACEMENT_3D('',#119649,#86944,#86945);
#79818=AXIS2_PLACEMENT_3D('',#119769,#86946,#86947);
#79819=AXIS2_PLACEMENT_3D('',#119770,#86948,#86949);
#79820=AXIS2_PLACEMENT_3D('',#119804,#86951,#86952);
#79821=AXIS2_PLACEMENT_3D('',#119871,#86953,#86954);
#79822=AXIS2_PLACEMENT_3D('',#119974,#86955,#86956);
#79823=AXIS2_PLACEMENT_3D('',#120091,#86957,#86958);
#79824=AXIS2_PLACEMENT_3D('',#120453,#86959,#86960);
#79825=AXIS2_PLACEMENT_3D('',#120537,#86961,#86962);
#79826=AXIS2_PLACEMENT_3D('',#120636,#86963,#86964);
#79827=AXIS2_PLACEMENT_3D('',#120949,#86965,#86966);
#79828=AXIS2_PLACEMENT_3D('',#121105,#86967,#86968);
#79829=AXIS2_PLACEMENT_3D('',#121190,#86969,#86970);
#79830=AXIS2_PLACEMENT_3D('',#121429,#86971,#86972);
#79831=AXIS2_PLACEMENT_3D('',#121514,#86973,#86974);
#79832=AXIS2_PLACEMENT_3D('',#121680,#86975,#86976);
#79833=AXIS2_PLACEMENT_3D('',#121904,#86977,#86978);
#79834=AXIS2_PLACEMENT_3D('',#123591,#86982,#86983);
#79835=AXIS2_PLACEMENT_3D('',#123592,#86984,#86985);
#79836=AXIS2_PLACEMENT_3D('',#123605,#86992,#86993);
#79837=AXIS2_PLACEMENT_3D('',#123608,#86996,#86997);
#79838=AXIS2_PLACEMENT_3D('',#123610,#86999,#87000);
#79839=AXIS2_PLACEMENT_3D('',#123612,#87002,#87003);
#79840=AXIS2_PLACEMENT_3D('',#123614,#87005,#87006);
#79841=AXIS2_PLACEMENT_3D('',#123616,#87008,#87009);
#79842=AXIS2_PLACEMENT_3D('',#123617,#87010,#87011);
#79843=AXIS2_PLACEMENT_3D('',#123618,#87012,#87013);
#79844=AXIS2_PLACEMENT_3D('',#123740,#87014,#87015);
#79845=AXIS2_PLACEMENT_3D('',#123745,#87017,#87018);
#79846=AXIS2_PLACEMENT_3D('',#123748,#87020,#87021);
#79847=AXIS2_PLACEMENT_3D('',#123911,#87022,#87023);
#79848=AXIS2_PLACEMENT_3D('',#124095,#87024,#87025);
#79849=AXIS2_PLACEMENT_3D('',#124098,#87026,#87027);
#79850=AXIS2_PLACEMENT_3D('',#124101,#87029,#87030);
#79851=AXIS2_PLACEMENT_3D('',#124359,#87032,#87033);
#79852=AXIS2_PLACEMENT_3D('',#124364,#87035,#87036);
#79853=AXIS2_PLACEMENT_3D('',#124419,#87037,#87038);
#79854=AXIS2_PLACEMENT_3D('',#124435,#87040,#87041);
#79855=AXIS2_PLACEMENT_3D('',#124469,#87043,#87044);
#79856=AXIS2_PLACEMENT_3D('',#124470,#87045,#87046);
#79857=AXIS2_PLACEMENT_3D('',#124471,#87047,#87048);
#79858=AXIS2_PLACEMENT_3D('',#124654,#87051,#87052);
#79859=AXIS2_PLACEMENT_3D('',#124656,#87053,#87054);
#79860=AXIS2_PLACEMENT_3D('',#124657,#87055,#87056);
#79861=AXIS2_PLACEMENT_3D('',#124658,#87057,#87058);
#79862=AXIS2_PLACEMENT_3D('',#124686,#87059,#87060);
#79863=AXIS2_PLACEMENT_3D('',#124706,#87061,#87062);
#79864=AXIS2_PLACEMENT_3D('',#124715,#87063,#87064);
#79865=AXIS2_PLACEMENT_3D('',#124717,#87066,#87067);
#79866=AXIS2_PLACEMENT_3D('',#124738,#87068,#87069);
#79867=AXIS2_PLACEMENT_3D('',#124772,#87071,#87072);
#79868=AXIS2_PLACEMENT_3D('',#124773,#87073,#87074);
#79869=AXIS2_PLACEMENT_3D('',#125006,#87075,#87076);
#79870=AXIS2_PLACEMENT_3D('',#125049,#87077,#87078);
#79871=AXIS2_PLACEMENT_3D('',#125111,#87079,#87080);
#79872=AXIS2_PLACEMENT_3D('',#125112,#87081,#87082);
#79873=AXIS2_PLACEMENT_3D('',#125113,#87083,#87084);
#79874=AXIS2_PLACEMENT_3D('',#125114,#87085,#87086);
#79875=AXIS2_PLACEMENT_3D('',#125116,#87087,#87088);
#79876=AXIS2_PLACEMENT_3D('',#125117,#87089,#87090);
#79877=AXIS2_PLACEMENT_3D('',#125404,#87091,#87092);
#79878=AXIS2_PLACEMENT_3D('',#125406,#87094,#87095);
#79879=AXIS2_PLACEMENT_3D('',#125407,#87096,#87097);
#79880=AXIS2_PLACEMENT_3D('',#125408,#87098,#87099);
#79881=AXIS2_PLACEMENT_3D('',#125409,#87100,#87101);
#79882=AXIS2_PLACEMENT_3D('',#125411,#87102,#87103);
#79883=AXIS2_PLACEMENT_3D('',#125413,#87104,#87105);
#79884=AXIS2_PLACEMENT_3D('',#125414,#87106,#87107);
#79885=AXIS2_PLACEMENT_3D('',#125415,#87108,#87109);
#79886=AXIS2_PLACEMENT_3D('',#125417,#87110,#87111);
#79887=AXIS2_PLACEMENT_3D('',#125418,#87112,#87113);
#79888=AXIS2_PLACEMENT_3D('',#125419,#87114,#87115);
#79889=AXIS2_PLACEMENT_3D('',#125931,#87117,#87118);
#79890=AXIS2_PLACEMENT_3D('',#125962,#87119,#87120);
#79891=AXIS2_PLACEMENT_3D('',#125964,#87121,#87122);
#79892=AXIS2_PLACEMENT_3D('',#125966,#87123,#87124);
#79893=AXIS2_PLACEMENT_3D('',#125968,#87125,#87126);
#79894=AXIS2_PLACEMENT_3D('',#125969,#87127,#87128);
#79895=AXIS2_PLACEMENT_3D('',#125970,#87129,#87130);
#79896=AXIS2_PLACEMENT_3D('',#125972,#87131,#87132);
#79897=AXIS2_PLACEMENT_3D('',#125973,#87133,#87134);
#79898=AXIS2_PLACEMENT_3D('',#125974,#87135,#87136);
#79899=AXIS2_PLACEMENT_3D('',#125977,#87137,#87138);
#79900=AXIS2_PLACEMENT_3D('',#125978,#87139,#87140);
#79901=AXIS2_PLACEMENT_3D('',#125979,#87141,#87142);
#79902=AXIS2_PLACEMENT_3D('',#125980,#87143,#87144);
#79903=AXIS2_PLACEMENT_3D('',#126066,#87146,#87147);
#79904=AXIS2_PLACEMENT_3D('',#126067,#87148,#87149);
#79905=AXIS2_PLACEMENT_3D('',#126068,#87150,#87151);
#79906=AXIS2_PLACEMENT_3D('',#126069,#87152,#87153);
#79907=AXIS2_PLACEMENT_3D('',#126070,#87154,#87155);
#79908=AXIS2_PLACEMENT_3D('',#126071,#87156,#87157);
#79909=AXIS2_PLACEMENT_3D('',#126072,#87158,#87159);
#79910=AXIS2_PLACEMENT_3D('',#126073,#87160,#87161);
#79911=AXIS2_PLACEMENT_3D('',#126074,#87162,#87163);
#79912=AXIS2_PLACEMENT_3D('',#126075,#87164,#87165);
#79913=AXIS2_PLACEMENT_3D('',#126213,#87167,#87168);
#79914=AXIS2_PLACEMENT_3D('',#126215,#87170,#87171);
#79915=AXIS2_PLACEMENT_3D('',#126217,#87172,#87173);
#79916=AXIS2_PLACEMENT_3D('',#126219,#87174,#87175);
#79917=AXIS2_PLACEMENT_3D('',#126220,#87176,#87177);
#79918=AXIS2_PLACEMENT_3D('',#126221,#87178,#87179);
#79919=AXIS2_PLACEMENT_3D('',#126223,#87180,#87181);
#79920=AXIS2_PLACEMENT_3D('',#126224,#87182,#87183);
#79921=AXIS2_PLACEMENT_3D('',#126225,#87184,#87185);
#79922=AXIS2_PLACEMENT_3D('',#126227,#87186,#87187);
#79923=AXIS2_PLACEMENT_3D('',#126228,#87188,#87189);
#79924=AXIS2_PLACEMENT_3D('',#126229,#87190,#87191);
#79925=AXIS2_PLACEMENT_3D('',#126356,#87193,#87194);
#79926=AXIS2_PLACEMENT_3D('',#126388,#87196,#87197);
#79927=AXIS2_PLACEMENT_3D('',#126409,#87198,#87199);
#79928=AXIS2_PLACEMENT_3D('',#126410,#87200,#87201);
#79929=AXIS2_PLACEMENT_3D('',#126554,#87202,#87203);
#79930=AXIS2_PLACEMENT_3D('',#126555,#87204,#87205);
#79931=AXIS2_PLACEMENT_3D('',#126612,#87206,#87207);
#79932=AXIS2_PLACEMENT_3D('',#126974,#87208,#87209);
#79933=AXIS2_PLACEMENT_3D('',#127058,#87210,#87211);
#79934=AXIS2_PLACEMENT_3D('',#127145,#87212,#87213);
#79935=AXIS2_PLACEMENT_3D('',#127206,#87214,#87215);
#79936=AXIS2_PLACEMENT_3D('',#127391,#87216,#87217);
#79937=AXIS2_PLACEMENT_3D('',#127559,#87218,#87219);
#79938=AXIS2_PLACEMENT_3D('',#127715,#87220,#87221);
#79939=AXIS2_PLACEMENT_3D('',#127898,#87222,#87223);
#79940=AXIS2_PLACEMENT_3D('',#128064,#87224,#87225);
#79941=AXIS2_PLACEMENT_3D('',#128149,#87226,#87227);
#79942=AXIS2_PLACEMENT_3D('',#128607,#87228,#87229);
#79943=AXIS2_PLACEMENT_3D('',#129974,#87233,#87234);
#79944=AXIS2_PLACEMENT_3D('',#130317,#87237,#87238);
#79945=AXIS2_PLACEMENT_3D('',#130318,#87239,#87240);
#79946=AXIS2_PLACEMENT_3D('',#130319,#87241,#87242);
#79947=AXIS2_PLACEMENT_3D('',#130320,#87243,#87244);
#79948=AXIS2_PLACEMENT_3D('',#130331,#87249,#87250);
#79949=AXIS2_PLACEMENT_3D('',#130333,#87251,#87252);
#79950=AXIS2_PLACEMENT_3D('',#130335,#87253,#87254);
#79951=AXIS2_PLACEMENT_3D('',#130337,#87255,#87256);
#79952=AXIS2_PLACEMENT_3D('',#130338,#87257,#87258);
#79953=AXIS2_PLACEMENT_3D('',#130339,#87259,#87260);
#79954=AXIS2_PLACEMENT_3D('',#130348,#87264,#87265);
#79955=AXIS2_PLACEMENT_3D('',#130350,#87266,#87267);
#79956=AXIS2_PLACEMENT_3D('',#130352,#87268,#87269);
#79957=AXIS2_PLACEMENT_3D('',#130354,#87270,#87271);
#79958=AXIS2_PLACEMENT_3D('',#130356,#87272,#87273);
#79959=AXIS2_PLACEMENT_3D('',#130358,#87275,#87276);
#79960=AXIS2_PLACEMENT_3D('',#130363,#87279,#87280);
#79961=AXIS2_PLACEMENT_3D('',#130364,#87281,#87282);
#79962=AXIS2_PLACEMENT_3D('',#130369,#87285,#87286);
#79963=AXIS2_PLACEMENT_3D('',#130370,#87287,#87288);
#79964=AXIS2_PLACEMENT_3D('',#130372,#87289,#87290);
#79965=AXIS2_PLACEMENT_3D('',#130374,#87291,#87292);
#79966=AXIS2_PLACEMENT_3D('',#130377,#87294,#87295);
#79967=AXIS2_PLACEMENT_3D('',#130402,#87296,#87297);
#79968=AXIS2_PLACEMENT_3D('',#130576,#87302,#87303);
#79969=AXIS2_PLACEMENT_3D('',#130597,#87304,#87305);
#79970=AXIS2_PLACEMENT_3D('',#130614,#87307,#87308);
#79971=AXIS2_PLACEMENT_3D('',#130810,#87310,#87311);
#79972=AXIS2_PLACEMENT_3D('',#131016,#87312,#87313);
#79973=AXIS2_PLACEMENT_3D('',#131033,#87315,#87316);
#79974=AXIS2_PLACEMENT_3D('',#131052,#87317,#87318);
#79975=AXIS2_PLACEMENT_3D('',#131160,#87320,#87321);
#79976=AXIS2_PLACEMENT_3D('',#131257,#87323,#87324);
#79977=AXIS2_PLACEMENT_3D('',#131349,#87326,#87327);
#79978=AXIS2_PLACEMENT_3D('',#131583,#87329,#87330);
#79979=AXIS2_PLACEMENT_3D('',#131864,#87331,#87332);
#79980=AXIS2_PLACEMENT_3D('',#131877,#87333,#87334);
#79981=AXIS2_PLACEMENT_3D('',#131879,#87336,#87337);
#79982=AXIS2_PLACEMENT_3D('',#131893,#87339,#87340);
#79983=AXIS2_PLACEMENT_3D('',#131950,#87341,#87342);
#79984=AXIS2_PLACEMENT_3D('',#132331,#87343,#87344);
#79985=AXIS2_PLACEMENT_3D('',#132332,#87345,#87346);
#79986=AXIS2_PLACEMENT_3D('',#132382,#87347,#87348);
#79987=AXIS2_PLACEMENT_3D('',#132384,#87349,#87350);
#79988=AXIS2_PLACEMENT_3D('',#132488,#87352,#87353);
#79989=AXIS2_PLACEMENT_3D('',#132587,#87354,#87355);
#79990=AXIS2_PLACEMENT_3D('',#132589,#87356,#87357);
#79991=AXIS2_PLACEMENT_3D('',#132642,#87358,#87359);
#79992=AXIS2_PLACEMENT_3D('',#132849,#87360,#87361);
#79993=AXIS2_PLACEMENT_3D('',#132917,#87362,#87363);
#79994=AXIS2_PLACEMENT_3D('',#132932,#87364,#87365);
#79995=AXIS2_PLACEMENT_3D('',#132995,#87366,#87367);
#79996=AXIS2_PLACEMENT_3D('',#133155,#87368,#87369);
#79997=AXIS2_PLACEMENT_3D('',#133212,#87370,#87371);
#79998=AXIS2_PLACEMENT_3D('',#133214,#87372,#87373);
#79999=AXIS2_PLACEMENT_3D('',#133215,#87374,#87375);
#80000=AXIS2_PLACEMENT_3D('',#133253,#87376,#87377);
#80001=AXIS2_PLACEMENT_3D('',#133378,#87378,#87379);
#80002=AXIS2_PLACEMENT_3D('',#133410,#87380,#87381);
#80003=AXIS2_PLACEMENT_3D('',#133411,#87382,#87383);
#80004=AXIS2_PLACEMENT_3D('',#133412,#87384,#87385);
#80005=AXIS2_PLACEMENT_3D('',#133413,#87386,#87387);
#80006=AXIS2_PLACEMENT_3D('',#133453,#87388,#87389);
#80007=AXIS2_PLACEMENT_3D('',#133454,#87390,#87391);
#80008=AXIS2_PLACEMENT_3D('',#133455,#87392,#87393);
#80009=AXIS2_PLACEMENT_3D('',#133456,#87394,#87395);
#80010=AXIS2_PLACEMENT_3D('',#133457,#87396,#87397);
#80011=AXIS2_PLACEMENT_3D('',#133460,#87399,#87400);
#80012=AXIS2_PLACEMENT_3D('',#133461,#87401,#87402);
#80013=AXIS2_PLACEMENT_3D('',#133462,#87403,#87404);
#80014=AXIS2_PLACEMENT_3D('',#133463,#87405,#87406);
#80015=AXIS2_PLACEMENT_3D('',#133464,#87407,#87408);
#80016=AXIS2_PLACEMENT_3D('',#133465,#87409,#87410);
#80017=AXIS2_PLACEMENT_3D('',#133467,#87412,#87413);
#80018=AXIS2_PLACEMENT_3D('',#133525,#87418,#87419);
#80019=AXIS2_PLACEMENT_3D('',#133526,#87420,#87421);
#80020=AXIS2_PLACEMENT_3D('',#133527,#87422,#87423);
#80021=AXIS2_PLACEMENT_3D('',#133609,#87424,#87425);
#80022=AXIS2_PLACEMENT_3D('',#133977,#87426,#87427);
#80023=AXIS2_PLACEMENT_3D('',#133978,#87428,#87429);
#80024=AXIS2_PLACEMENT_3D('',#134346,#87430,#87431);
#80025=AXIS2_PLACEMENT_3D('',#134411,#87432,#87433);
#80026=AXIS2_PLACEMENT_3D('',#134563,#87435,#87436);
#80027=AXIS2_PLACEMENT_3D('',#134695,#87439,#87440);
#80028=AXIS2_PLACEMENT_3D('',#134697,#87441,#87442);
#80029=AXIS2_PLACEMENT_3D('',#134699,#87443,#87444);
#80030=AXIS2_PLACEMENT_3D('',#134700,#87445,#87446);
#80031=AXIS2_PLACEMENT_3D('',#134701,#87447,#87448);
#80032=AXIS2_PLACEMENT_3D('',#134703,#87449,#87450);
#80033=AXIS2_PLACEMENT_3D('',#134704,#87451,#87452);
#80034=AXIS2_PLACEMENT_3D('',#134705,#87453,#87454);
#80035=AXIS2_PLACEMENT_3D('',#134706,#87455,#87456);
#80036=AXIS2_PLACEMENT_3D('',#134708,#87457,#87458);
#80037=AXIS2_PLACEMENT_3D('',#134710,#87459,#87460);
#80038=AXIS2_PLACEMENT_3D('',#134713,#87462,#87463);
#80039=AXIS2_PLACEMENT_3D('',#134714,#87464,#87465);
#80040=AXIS2_PLACEMENT_3D('',#134716,#87466,#87467);
#80041=AXIS2_PLACEMENT_3D('',#134717,#87468,#87469);
#80042=AXIS2_PLACEMENT_3D('',#135394,#87470,#87471);
#80043=AXIS2_PLACEMENT_3D('',#135575,#87474,#87475);
#80044=AXIS2_PLACEMENT_3D('',#135579,#87478,#87479);
#80045=AXIS2_PLACEMENT_3D('',#135580,#87480,#87481);
#80046=AXIS2_PLACEMENT_3D('',#135606,#87482,#87483);
#80047=AXIS2_PLACEMENT_3D('',#135608,#87484,#87485);
#80048=AXIS2_PLACEMENT_3D('',#135609,#87486,#87487);
#80049=AXIS2_PLACEMENT_3D('',#135610,#87488,#87489);
#80050=AXIS2_PLACEMENT_3D('',#135612,#87490,#87491);
#80051=AXIS2_PLACEMENT_3D('',#135616,#87493,#87494);
#80052=AXIS2_PLACEMENT_3D('',#135618,#87495,#87496);
#80053=AXIS2_PLACEMENT_3D('',#135620,#87498,#87499);
#80054=AXIS2_PLACEMENT_3D('',#135623,#87500,#87501);
#80055=AXIS2_PLACEMENT_3D('',#135627,#87503,#87504);
#80056=AXIS2_PLACEMENT_3D('',#135630,#87506,#87507);
#80057=AXIS2_PLACEMENT_3D('',#135631,#87508,#87509);
#80058=AXIS2_PLACEMENT_3D('',#135951,#87511,#87512);
#80059=AXIS2_PLACEMENT_3D('',#135976,#87513,#87514);
#80060=AXIS2_PLACEMENT_3D('',#136019,#87515,#87516);
#80061=AXIS2_PLACEMENT_3D('',#136044,#87517,#87518);
#80062=AXIS2_PLACEMENT_3D('',#136404,#87519,#87520);
#80063=AXIS2_PLACEMENT_3D('',#137882,#87523,#87524);
#80064=AXIS2_PLACEMENT_3D('',#137893,#87525,#87526);
#80065=AXIS2_PLACEMENT_3D('',#138650,#87529,#87530);
#80066=AXIS2_PLACEMENT_3D('',#138664,#87531,#87532);
#80067=AXIS2_PLACEMENT_3D('',#138941,#87535,#87536);
#80068=AXIS2_PLACEMENT_3D('',#138982,#87537,#87538);
#80069=AXIS2_PLACEMENT_3D('',#138983,#87539,#87540);
#80070=AXIS2_PLACEMENT_3D('',#138984,#87541,#87542);
#80071=AXIS2_PLACEMENT_3D('',#138985,#87543,#87544);
#80072=AXIS2_PLACEMENT_3D('',#139141,#87546,#87547);
#80073=AXIS2_PLACEMENT_3D('',#139467,#87548,#87549);
#80074=AXIS2_PLACEMENT_3D('',#140135,#87550,#87551);
#80075=AXIS2_PLACEMENT_3D('',#140500,#87552,#87553);
#80076=AXIS2_PLACEMENT_3D('',#140501,#87554,#87555);
#80077=AXIS2_PLACEMENT_3D('',#140594,#87556,#87557);
#80078=AXIS2_PLACEMENT_3D('',#140647,#87558,#87559);
#80079=AXIS2_PLACEMENT_3D('',#141027,#87561,#87562);
#80080=AXIS2_PLACEMENT_3D('',#141029,#87563,#87564);
#80081=AXIS2_PLACEMENT_3D('',#141095,#87565,#87566);
#80082=AXIS2_PLACEMENT_3D('',#142788,#87567,#87568);
#80083=AXIS2_PLACEMENT_3D('',#142795,#87569,#87570);
#80084=AXIS2_PLACEMENT_3D('',#142965,#87572,#87573);
#80085=AXIS2_PLACEMENT_3D('',#143054,#87575,#87576);
#80086=AXIS2_PLACEMENT_3D('',#143069,#87577,#87578);
#80087=AXIS2_PLACEMENT_3D('',#143239,#87579,#87580);
#80088=AXIS2_PLACEMENT_3D('',#143261,#87581,#87582);
#80089=AXIS2_PLACEMENT_3D('',#143262,#87583,#87584);
#80090=AXIS2_PLACEMENT_3D('',#143302,#87585,#87586);
#80091=AXIS2_PLACEMENT_3D('',#143309,#87587,#87588);
#80092=AXIS2_PLACEMENT_3D('',#143311,#87589,#87590);
#80093=AXIS2_PLACEMENT_3D('',#143312,#87591,#87592);
#80094=AXIS2_PLACEMENT_3D('',#143479,#87593,#87594);
#80095=AXIS2_PLACEMENT_3D('',#143482,#87596,#87597);
#80096=AXIS2_PLACEMENT_3D('',#143582,#87598,#87599);
#80097=AXIS2_PLACEMENT_3D('',#143583,#87600,#87601);
#80098=AXIS2_PLACEMENT_3D('',#143585,#87602,#87603);
#80099=AXIS2_PLACEMENT_3D('',#143586,#87604,#87605);
#80100=AXIS2_PLACEMENT_3D('',#143648,#87606,#87607);
#80101=AXIS2_PLACEMENT_3D('',#143687,#87608,#87609);
#80102=AXIS2_PLACEMENT_3D('',#143745,#87611,#87612);
#80103=AXIS2_PLACEMENT_3D('',#143746,#87613,#87614);
#80104=AXIS2_PLACEMENT_3D('',#143747,#87615,#87616);
#80105=AXIS2_PLACEMENT_3D('',#143749,#87617,#87618);
#80106=AXIS2_PLACEMENT_3D('',#143750,#87619,#87620);
#80107=AXIS2_PLACEMENT_3D('',#143850,#87621,#87622);
#80108=AXIS2_PLACEMENT_3D('',#143851,#87623,#87624);
#80109=AXIS2_PLACEMENT_3D('',#143854,#87626,#87627);
#80110=AXIS2_PLACEMENT_3D('',#143969,#87628,#87629);
#80111=AXIS2_PLACEMENT_3D('',#143970,#87630,#87631);
#80112=AXIS2_PLACEMENT_3D('',#143972,#87632,#87633);
#80113=AXIS2_PLACEMENT_3D('',#143973,#87634,#87635);
#80114=AXIS2_PLACEMENT_3D('',#143974,#87636,#87637);
#80115=AXIS2_PLACEMENT_3D('',#143991,#87638,#87639);
#80116=AXIS2_PLACEMENT_3D('',#143992,#87640,#87641);
#80117=AXIS2_PLACEMENT_3D('',#144002,#87642,#87643);
#80118=AXIS2_PLACEMENT_3D('',#144021,#87644,#87645);
#80119=AXIS2_PLACEMENT_3D('',#144079,#87646,#87647);
#80120=AXIS2_PLACEMENT_3D('',#144142,#87648,#87649);
#80121=AXIS2_PLACEMENT_3D('',#144193,#87650,#87651);
#80122=AXIS2_PLACEMENT_3D('',#144324,#87652,#87653);
#80123=AXIS2_PLACEMENT_3D('',#144325,#87654,#87655);
#80124=AXIS2_PLACEMENT_3D('',#144479,#87657,#87658);
#80125=AXIS2_PLACEMENT_3D('',#144480,#87659,#87660);
#80126=AXIS2_PLACEMENT_3D('',#144546,#87661,#87662);
#80127=AXIS2_PLACEMENT_3D('',#144725,#87663,#87664);
#80128=AXIS2_PLACEMENT_3D('',#144893,#87665,#87666);
#80129=AXIS2_PLACEMENT_3D('',#145131,#87667,#87668);
#80130=AXIS2_PLACEMENT_3D('',#145222,#87669,#87670);
#80131=AXIS2_PLACEMENT_3D('',#145255,#87671,#87672);
#80132=AXIS2_PLACEMENT_3D('',#145294,#87673,#87674);
#80133=AXIS2_PLACEMENT_3D('',#145295,#87675,#87676);
#80134=AXIS2_PLACEMENT_3D('',#145396,#87677,#87678);
#80135=AXIS2_PLACEMENT_3D('',#145398,#87680,#87681);
#80136=AXIS2_PLACEMENT_3D('',#145400,#87683,#87684);
#80137=AXIS2_PLACEMENT_3D('',#145403,#87687,#87688);
#80138=AXIS2_PLACEMENT_3D('',#145405,#87690,#87691);
#80139=AXIS2_PLACEMENT_3D('',#145406,#87692,#87693);
#80140=AXIS2_PLACEMENT_3D('',#145407,#87694,#87695);
#80141=AXIS2_PLACEMENT_3D('',#145410,#87696,#87697);
#80142=AXIS2_PLACEMENT_3D('',#145412,#87699,#87700);
#80143=AXIS2_PLACEMENT_3D('',#145589,#87704,#87705);
#80144=AXIS2_PLACEMENT_3D('',#145591,#87706,#87707);
#80145=AXIS2_PLACEMENT_3D('',#145592,#87708,#87709);
#80146=AXIS2_PLACEMENT_3D('',#145593,#87710,#87711);
#80147=AXIS2_PLACEMENT_3D('',#145597,#87713,#87714);
#80148=AXIS2_PLACEMENT_3D('',#145599,#87715,#87716);
#80149=AXIS2_PLACEMENT_3D('',#145617,#87717,#87718);
#80150=AXIS2_PLACEMENT_3D('',#145618,#87719,#87720);
#80151=AXIS2_PLACEMENT_3D('',#145620,#87721,#87722);
#80152=AXIS2_PLACEMENT_3D('',#145628,#87723,#87724);
#80153=AXIS2_PLACEMENT_3D('',#145630,#87725,#87726);
#80154=AXIS2_PLACEMENT_3D('',#145632,#87728,#87729);
#80155=AXIS2_PLACEMENT_3D('',#145634,#87730,#87731);
#80156=AXIS2_PLACEMENT_3D('',#145636,#87732,#87733);
#80157=AXIS2_PLACEMENT_3D('',#145637,#87734,#87735);
#80158=AXIS2_PLACEMENT_3D('',#145703,#87736,#87737);
#80159=AXIS2_PLACEMENT_3D('',#145798,#87738,#87739);
#80160=AXIS2_PLACEMENT_3D('',#145832,#87741,#87742);
#80161=AXIS2_PLACEMENT_3D('',#145856,#87744,#87745);
#80162=AXIS2_PLACEMENT_3D('',#145870,#87746,#87747);
#80163=AXIS2_PLACEMENT_3D('',#145882,#87749,#87750);
#80164=AXIS2_PLACEMENT_3D('',#145884,#87752,#87753);
#80165=AXIS2_PLACEMENT_3D('',#145949,#87756,#87757);
#80166=AXIS2_PLACEMENT_3D('',#145950,#87758,#87759);
#80167=AXIS2_PLACEMENT_3D('',#145951,#87760,#87761);
#80168=AXIS2_PLACEMENT_3D('',#146004,#87762,#87763);
#80169=AXIS2_PLACEMENT_3D('',#146005,#87764,#87765);
#80170=AXIS2_PLACEMENT_3D('',#146078,#87766,#87767);
#80171=AXIS2_PLACEMENT_3D('',#146079,#87768,#87769);
#80172=AXIS2_PLACEMENT_3D('',#146080,#87770,#87771);
#80173=AXIS2_PLACEMENT_3D('',#146081,#87772,#87773);
#80174=AXIS2_PLACEMENT_3D('',#146295,#87774,#87775);
#80175=AXIS2_PLACEMENT_3D('',#146297,#87777,#87778);
#80176=AXIS2_PLACEMENT_3D('',#146368,#87784,#87785);
#80177=AXIS2_PLACEMENT_3D('',#146607,#87786,#87787);
#80178=AXIS2_PLACEMENT_3D('',#146608,#87788,#87789);
#80179=AXIS2_PLACEMENT_3D('',#146610,#87790,#87791);
#80180=AXIS2_PLACEMENT_3D('',#146612,#87792,#87793);
#80181=AXIS2_PLACEMENT_3D('',#146613,#87794,#87795);
#80182=AXIS2_PLACEMENT_3D('',#146614,#87796,#87797);
#80183=AXIS2_PLACEMENT_3D('',#146615,#87798,#87799);
#80184=AXIS2_PLACEMENT_3D('',#146616,#87800,#87801);
#80185=AXIS2_PLACEMENT_3D('',#146655,#87802,#87803);
#80186=AXIS2_PLACEMENT_3D('',#146656,#87804,#87805);
#80187=AXIS2_PLACEMENT_3D('',#146658,#87806,#87807);
#80188=AXIS2_PLACEMENT_3D('',#146905,#87808,#87809);
#80189=AXIS2_PLACEMENT_3D('',#146907,#87811,#87812);
#80190=AXIS2_PLACEMENT_3D('',#146911,#87815,#87816);
#80191=AXIS2_PLACEMENT_3D('',#146918,#87820,#87821);
#80192=AXIS2_PLACEMENT_3D('',#146919,#87822,#87823);
#80193=AXIS2_PLACEMENT_3D('',#146920,#87824,#87825);
#80194=AXIS2_PLACEMENT_3D('',#146921,#87826,#87827);
#80195=AXIS2_PLACEMENT_3D('',#146922,#87828,#87829);
#80196=AXIS2_PLACEMENT_3D('',#146923,#87830,#87831);
#80197=AXIS2_PLACEMENT_3D('',#146924,#87832,#87833);
#80198=AXIS2_PLACEMENT_3D('',#147115,#87834,#87835);
#80199=AXIS2_PLACEMENT_3D('',#147264,#87836,#87837);
#80200=AXIS2_PLACEMENT_3D('',#147375,#87838,#87839);
#80201=AXIS2_PLACEMENT_3D('',#147444,#87840,#87841);
#80202=AXIS2_PLACEMENT_3D('',#147449,#87842,#87843);
#80203=AXIS2_PLACEMENT_3D('',#147575,#87845,#87846);
#80204=AXIS2_PLACEMENT_3D('',#147577,#87847,#87848);
#80205=AXIS2_PLACEMENT_3D('',#147610,#87849,#87850);
#80206=AXIS2_PLACEMENT_3D('',#147707,#87851,#87852);
#80207=AXIS2_PLACEMENT_3D('',#147712,#87853,#87854);
#80208=AXIS2_PLACEMENT_3D('',#148080,#87857,#87858);
#80209=AXIS2_PLACEMENT_3D('',#148457,#87859,#87860);
#80210=AXIS2_PLACEMENT_3D('',#148458,#87861,#87862);
#80211=AXIS2_PLACEMENT_3D('',#148483,#87863,#87864);
#80212=AXIS2_PLACEMENT_3D('',#148484,#87865,#87866);
#80213=AXIS2_PLACEMENT_3D('',#148487,#87867,#87868);
#80214=AXIS2_PLACEMENT_3D('',#148500,#87869,#87870);
#80215=AXIS2_PLACEMENT_3D('',#148559,#87871,#87872);
#80216=AXIS2_PLACEMENT_3D('',#148565,#87873,#87874);
#80217=AXIS2_PLACEMENT_3D('',#148667,#87875,#87876);
#80218=AXIS2_PLACEMENT_3D('',#148766,#87877,#87878);
#80219=AXIS2_PLACEMENT_3D('',#148957,#87879,#87880);
#80220=AXIS2_PLACEMENT_3D('',#149011,#87881,#87882);
#80221=AXIS2_PLACEMENT_3D('',#149117,#87883,#87884);
#80222=AXIS2_PLACEMENT_3D('',#149135,#87885,#87886);
#80223=AXIS2_PLACEMENT_3D('',#149206,#87887,#87888);
#80224=AXIS2_PLACEMENT_3D('',#149563,#87889,#87890);
#80225=AXIS2_PLACEMENT_3D('',#149606,#87891,#87892);
#80226=AXIS2_PLACEMENT_3D('',#149634,#87893,#87894);
#80227=AXIS2_PLACEMENT_3D('',#149816,#87895,#87896);
#80228=AXIS2_PLACEMENT_3D('',#149818,#87897,#87898);
#80229=AXIS2_PLACEMENT_3D('',#149820,#87899,#87900);
#80230=AXIS2_PLACEMENT_3D('',#149822,#87901,#87902);
#80231=AXIS2_PLACEMENT_3D('',#149824,#87903,#87904);
#80232=AXIS2_PLACEMENT_3D('',#149825,#87905,#87906);
#80233=AXIS2_PLACEMENT_3D('',#149826,#87907,#87908);
#80234=AXIS2_PLACEMENT_3D('',#149828,#87910,#87911);
#80235=AXIS2_PLACEMENT_3D('',#149865,#87912,#87913);
#80236=AXIS2_PLACEMENT_3D('',#149956,#87916,#87917);
#80237=AXIS2_PLACEMENT_3D('',#149958,#87919,#87920);
#80238=AXIS2_PLACEMENT_3D('',#149982,#87921,#87922);
#80239=AXIS2_PLACEMENT_3D('',#149983,#87923,#87924);
#80240=AXIS2_PLACEMENT_3D('',#150076,#87925,#87926);
#80241=AXIS2_PLACEMENT_3D('',#150078,#87927,#87928);
#80242=AXIS2_PLACEMENT_3D('',#150080,#87929,#87930);
#80243=AXIS2_PLACEMENT_3D('',#150081,#87931,#87932);
#80244=AXIS2_PLACEMENT_3D('',#150082,#87933,#87934);
#80245=AXIS2_PLACEMENT_3D('',#150112,#87936,#87937);
#80246=AXIS2_PLACEMENT_3D('',#150148,#87938,#87939);
#80247=AXIS2_PLACEMENT_3D('',#150258,#87943,#87944);
#80248=AXIS2_PLACEMENT_3D('',#150277,#87946,#87947);
#80249=AXIS2_PLACEMENT_3D('',#150343,#87948,#87949);
#80250=AXIS2_PLACEMENT_3D('',#150601,#87950,#87951);
#80251=AXIS2_PLACEMENT_3D('',#150689,#87952,#87953);
#80252=AXIS2_PLACEMENT_3D('',#150711,#87954,#87955);
#80253=AXIS2_PLACEMENT_3D('',#150814,#87956,#87957);
#80254=AXIS2_PLACEMENT_3D('',#150836,#87958,#87959);
#80255=AXIS2_PLACEMENT_3D('',#150891,#87960,#87961);
#80256=AXIS2_PLACEMENT_3D('',#151146,#87962,#87963);
#80257=AXIS2_PLACEMENT_3D('',#151225,#87964,#87965);
#80258=AXIS2_PLACEMENT_3D('',#151346,#87966,#87967);
#80259=AXIS2_PLACEMENT_3D('',#151347,#87968,#87969);
#80260=AXIS2_PLACEMENT_3D('',#151348,#87970,#87971);
#80261=AXIS2_PLACEMENT_3D('',#151349,#87972,#87973);
#80262=AXIS2_PLACEMENT_3D('',#151350,#87974,#87975);
#80263=AXIS2_PLACEMENT_3D('',#151351,#87976,#87977);
#80264=AXIS2_PLACEMENT_3D('',#151352,#87978,#87979);
#80265=AXIS2_PLACEMENT_3D('',#151354,#87980,#87981);
#80266=AXIS2_PLACEMENT_3D('',#151355,#87982,#87983);
#80267=AXIS2_PLACEMENT_3D('',#151356,#87984,#87985);
#80268=AXIS2_PLACEMENT_3D('',#151357,#87986,#87987);
#80269=AXIS2_PLACEMENT_3D('',#151358,#87988,#87989);
#80270=AXIS2_PLACEMENT_3D('',#151359,#87990,#87991);
#80271=AXIS2_PLACEMENT_3D('',#151360,#87992,#87993);
#80272=AXIS2_PLACEMENT_3D('',#151362,#87994,#87995);
#80273=AXIS2_PLACEMENT_3D('',#151363,#87996,#87997);
#80274=AXIS2_PLACEMENT_3D('',#151364,#87998,#87999);
#80275=AXIS2_PLACEMENT_3D('',#151365,#88000,#88001);
#80276=AXIS2_PLACEMENT_3D('',#151366,#88002,#88003);
#80277=AXIS2_PLACEMENT_3D('',#151367,#88004,#88005);
#80278=AXIS2_PLACEMENT_3D('',#151685,#88006,#88007);
#80279=AXIS2_PLACEMENT_3D('',#152883,#88008,#88009);
#80280=AXIS2_PLACEMENT_3D('',#152884,#88010,#88011);
#80281=AXIS2_PLACEMENT_3D('',#152885,#88012,#88013);
#80282=AXIS2_PLACEMENT_3D('',#152886,#88014,#88015);
#80283=AXIS2_PLACEMENT_3D('',#153185,#88016,#88017);
#80284=AXIS2_PLACEMENT_3D('',#153251,#88018,#88019);
#80285=AXIS2_PLACEMENT_3D('',#153253,#88020,#88021);
#80286=AXIS2_PLACEMENT_3D('',#153254,#88022,#88023);
#80287=AXIS2_PLACEMENT_3D('',#153255,#88024,#88025);
#80288=AXIS2_PLACEMENT_3D('',#153257,#88026,#88027);
#80289=AXIS2_PLACEMENT_3D('',#153258,#88028,#88029);
#80290=AXIS2_PLACEMENT_3D('',#153259,#88030,#88031);
#80291=AXIS2_PLACEMENT_3D('',#153260,#88032,#88033);
#80292=AXIS2_PLACEMENT_3D('',#153261,#88034,#88035);
#80293=AXIS2_PLACEMENT_3D('',#153262,#88036,#88037);
#80294=AXIS2_PLACEMENT_3D('',#153263,#88038,#88039);
#80295=AXIS2_PLACEMENT_3D('',#153264,#88040,#88041);
#80296=AXIS2_PLACEMENT_3D('',#153652,#88042,#88043);
#80297=AXIS2_PLACEMENT_3D('',#153673,#88044,#88045);
#80298=AXIS2_PLACEMENT_3D('',#153885,#88046,#88047);
#80299=AXIS2_PLACEMENT_3D('',#154081,#88048,#88049);
#80300=AXIS2_PLACEMENT_3D('',#154117,#88050,#88051);
#80301=AXIS2_PLACEMENT_3D('',#154128,#88052,#88053);
#80302=AXIS2_PLACEMENT_3D('',#154201,#88054,#88055);
#80303=AXIS2_PLACEMENT_3D('',#154339,#88056,#88057);
#80304=AXIS2_PLACEMENT_3D('',#154377,#88058,#88059);
#80305=AXIS2_PLACEMENT_3D('',#154415,#88060,#88061);
#80306=AXIS2_PLACEMENT_3D('',#154611,#88062,#88063);
#80307=AXIS2_PLACEMENT_3D('',#154817,#88064,#88065);
#80308=AXIS2_PLACEMENT_3D('',#154818,#88066,#88067);
#80309=AXIS2_PLACEMENT_3D('',#154819,#88068,#88069);
#80310=AXIS2_PLACEMENT_3D('',#154820,#88070,#88071);
#80311=AXIS2_PLACEMENT_3D('',#154821,#88072,#88073);
#80312=AXIS2_PLACEMENT_3D('',#154822,#88074,#88075);
#80313=AXIS2_PLACEMENT_3D('',#154823,#88076,#88077);
#80314=AXIS2_PLACEMENT_3D('',#154824,#88078,#88079);
#80315=AXIS2_PLACEMENT_3D('',#154825,#88080,#88081);
#80316=AXIS2_PLACEMENT_3D('',#154826,#88082,#88083);
#80317=AXIS2_PLACEMENT_3D('',#154829,#88085,#88086);
#80318=AXIS2_PLACEMENT_3D('',#154831,#88087,#88088);
#80319=AXIS2_PLACEMENT_3D('',#154833,#88090,#88091);
#80320=AXIS2_PLACEMENT_3D('',#155004,#88093,#88094);
#80321=AXIS2_PLACEMENT_3D('',#155005,#88095,#88096);
#80322=AXIS2_PLACEMENT_3D('',#155053,#88097,#88098);
#80323=AXIS2_PLACEMENT_3D('',#155054,#88099,#88100);
#80324=AXIS2_PLACEMENT_3D('',#155484,#88101,#88102);
#80325=AXIS2_PLACEMENT_3D('',#155722,#88103,#88104);
#80326=AXIS2_PLACEMENT_3D('',#155864,#88105,#88106);
#80327=AXIS2_PLACEMENT_3D('',#155865,#88107,#88108);
#80328=AXIS2_PLACEMENT_3D('',#155866,#88109,#88110);
#80329=AXIS2_PLACEMENT_3D('',#155867,#88111,#88112);
#80330=AXIS2_PLACEMENT_3D('',#155868,#88113,#88114);
#80331=AXIS2_PLACEMENT_3D('',#155869,#88115,#88116);
#80332=AXIS2_PLACEMENT_3D('',#156062,#88117,#88118);
#80333=AXIS2_PLACEMENT_3D('',#156224,#88119,#88120);
#80334=AXIS2_PLACEMENT_3D('',#156225,#88121,#88122);
#80335=AXIS2_PLACEMENT_3D('',#156251,#88123,#88124);
#80336=AXIS2_PLACEMENT_3D('',#156275,#88125,#88126);
#80337=AXIS2_PLACEMENT_3D('',#156300,#88127,#88128);
#80338=AXIS2_PLACEMENT_3D('',#156301,#88129,#88130);
#80339=AXIS2_PLACEMENT_3D('',#156302,#88131,#88132);
#80340=AXIS2_PLACEMENT_3D('',#156681,#88133,#88134);
#80341=AXIS2_PLACEMENT_3D('',#156682,#88135,#88136);
#80342=AXIS2_PLACEMENT_3D('',#156683,#88137,#88138);
#80343=AXIS2_PLACEMENT_3D('',#156806,#88139,#88140);
#80344=AXIS2_PLACEMENT_3D('',#156809,#88142,#88143);
#80345=AXIS2_PLACEMENT_3D('',#156810,#88144,#88145);
#80346=AXIS2_PLACEMENT_3D('',#156866,#88146,#88147);
#80347=AXIS2_PLACEMENT_3D('',#156997,#88148,#88149);
#80348=AXIS2_PLACEMENT_3D('',#157000,#88151,#88152);
#80349=AXIS2_PLACEMENT_3D('',#157028,#88153,#88154);
#80350=AXIS2_PLACEMENT_3D('',#157029,#88155,#88156);
#80351=AXIS2_PLACEMENT_3D('',#157030,#88157,#88158);
#80352=AXIS2_PLACEMENT_3D('',#157046,#88159,#88160);
#80353=AXIS2_PLACEMENT_3D('',#157047,#88161,#88162);
#80354=AXIS2_PLACEMENT_3D('',#157048,#88163,#88164);
#80355=AXIS2_PLACEMENT_3D('',#157049,#88165,#88166);
#80356=AXIS2_PLACEMENT_3D('',#157050,#88167,#88168);
#80357=AXIS2_PLACEMENT_3D('',#157105,#88169,#88170);
#80358=AXIS2_PLACEMENT_3D('',#157121,#88171,#88172);
#80359=AXIS2_PLACEMENT_3D('',#157122,#88173,#88174);
#80360=AXIS2_PLACEMENT_3D('',#157123,#88175,#88176);
#80361=AXIS2_PLACEMENT_3D('',#157124,#88177,#88178);
#80362=AXIS2_PLACEMENT_3D('',#157125,#88179,#88180);
#80363=AXIS2_PLACEMENT_3D('',#157369,#88181,#88182);
#80364=AXIS2_PLACEMENT_3D('',#157416,#88183,#88184);
#80365=AXIS2_PLACEMENT_3D('',#157454,#88185,#88186);
#80366=AXIS2_PLACEMENT_3D('',#157455,#88187,#88188);
#80367=AXIS2_PLACEMENT_3D('',#157705,#88189,#88190);
#80368=AXIS2_PLACEMENT_3D('',#157706,#88191,#88192);
#80369=AXIS2_PLACEMENT_3D('',#157747,#88193,#88194);
#80370=AXIS2_PLACEMENT_3D('',#157797,#88195,#88196);
#80371=AXIS2_PLACEMENT_3D('',#157798,#88197,#88198);
#80372=AXIS2_PLACEMENT_3D('',#157932,#88199,#88200);
#80373=AXIS2_PLACEMENT_3D('',#158052,#88201,#88202);
#80374=AXIS2_PLACEMENT_3D('',#158091,#88203,#88204);
#80375=AXIS2_PLACEMENT_3D('',#158201,#88205,#88206);
#80376=AXIS2_PLACEMENT_3D('',#158202,#88207,#88208);
#80377=AXIS2_PLACEMENT_3D('',#158203,#88209,#88210);
#80378=AXIS2_PLACEMENT_3D('',#158204,#88211,#88212);
#86166=DIRECTION('axis',(0.,0.,1.));
#86167=DIRECTION('refdir',(1.,0.,0.));
#86168=DIRECTION('center_axis',(0.156610083413696,-0.431983230632625,0.888180032552723));
#86169=DIRECTION('ref_axis',(0.961785334650907,0.271198694721067,-0.037686045587615));
#86170=DIRECTION('center_axis',(0.,-1.,0.));
#86171=DIRECTION('ref_axis',(-0.173648177666903,0.,-0.984807753012213));
#86172=DIRECTION('center_axis',(-0.156610100625892,0.431983257504582,-0.888180016448061));
#86173=DIRECTION('ref_axis',(0.338848737580694,0.868195889116037,0.362515421964341));
#86174=DIRECTION('center_axis',(0.940152247861526,-0.297712383088708,-0.165774207271705));
#86175=DIRECTION('ref_axis',(-0.173647839019125,1.10267237741349E-6,-0.984807812724276));
#86176=DIRECTION('center_axis',(-0.984807753012213,0.,0.173648177666902));
#86177=DIRECTION('ref_axis',(0.,1.,0.));
#86178=DIRECTION('',(-2.025323837648E-10,-1.,-2.189203733894E-10));
#86179=DIRECTION('',(0.173648177666902,0.,0.984807753012213));
#86180=DIRECTION('center_axis',(-0.984807753040743,-3.31556822456762E-10,
0.173648177505103));
#86181=DIRECTION('ref_axis',(0.155995631336126,-0.439294647618469,0.884695187947696));
#86182=DIRECTION('center_axis',(0.,-1.,0.));
#86183=DIRECTION('ref_axis',(0.173648177666903,0.,0.984807753012213));
#86184=DIRECTION('center_axis',(0.173648177666902,0.,0.984807753012213));
#86185=DIRECTION('ref_axis',(0.984807753012213,0.,-0.173648177666902));
#86186=DIRECTION('center_axis',(0.156610200040416,0.431982195134571,0.888180515621694));
#86187=DIRECTION('ref_axis',(0.961785732595754,-0.271197107788908,-0.0376873095641012));
#86188=DIRECTION('center_axis',(-0.940152146377266,-0.297712713531889,0.165774189377293));
#86189=DIRECTION('ref_axis',(-0.173647969304453,-6.78449113130987E-7,-0.984807789751878));
#86190=DIRECTION('center_axis',(-0.156610083777503,-0.4319834600727,-0.888179920895998));
#86191=DIRECTION('ref_axis',(0.98480775277219,2.88567290812795E-9,-0.173648179028143));
#86192=DIRECTION('center_axis',(0.,-1.,0.));
#86193=DIRECTION('ref_axis',(-0.173648177666903,0.,-0.984807753012213));
#86194=DIRECTION('center_axis',(-0.984807753012213,0.,0.173648177666902));
#86195=DIRECTION('ref_axis',(0.,1.,0.));
#86196=DIRECTION('center_axis',(-0.984807752957808,-6.43089184032011E-10,
0.173648177975449));
#86197=DIRECTION('ref_axis',(0.156008598329541,0.439141908993185,0.884768727415856));
#86198=DIRECTION('',(-0.173648177666902,0.,-0.984807753012213));
#86199=DIRECTION('',(-2.025323837648E-10,-1.,-2.189203733894E-10));
#86200=DIRECTION('center_axis',(0.,-1.,0.));
#86201=DIRECTION('ref_axis',(0.173648177666903,0.,0.984807753012213));
#86202=DIRECTION('center_axis',(0.173648177666902,0.,0.984807753012213));
#86203=DIRECTION('ref_axis',(0.984807753012213,0.,-0.173648177666902));
#86204=DIRECTION('center_axis',(0.173648177666902,0.,0.984807753012213));
#86205=DIRECTION('ref_axis',(0.984807753012213,0.,-0.173648177666902));
#86206=DIRECTION('center_axis',(-0.173648177666902,0.,-0.984807753012213));
#86207=DIRECTION('ref_axis',(0.984807753012213,0.,-0.173648177666902));
#86208=DIRECTION('',(-0.173648177666902,0.,-0.984807753012213));
#86209=DIRECTION('center_axis',(0.0391216869526731,-0.999210589338024,-0.00690592243911207));
#86210=DIRECTION('ref_axis',(-0.99913461352629,-0.0390191476249176,-0.0144059075484885));
#86211=DIRECTION('center_axis',(-0.984807753012213,0.,0.173648177666903));
#86212=DIRECTION('ref_axis',(0.173648177666903,0.,0.984807753012213));
#86213=DIRECTION('',(-0.984807631231399,0.,0.1736488683188));
#86214=DIRECTION('',(-0.984809724314531,4.00369164637112E-9,0.173636997484805));
#86215=DIRECTION('center_axis',(0.,1.,0.));
#86216=DIRECTION('ref_axis',(1.,0.,0.));
#86217=DIRECTION('center_axis',(-0.810842955514487,0.459818666371144,0.362078024117999));
#86218=DIRECTION('ref_axis',(0.0796317671110352,0.699582071269321,-0.710101195059761));
#86219=DIRECTION('center_axis',(0.173648177666902,0.,0.984807753012213));
#86220=DIRECTION('ref_axis',(0.,-1.,0.));
#86221=DIRECTION('center_axis',(0.173648177666902,0.,0.984807753012213));
#86222=DIRECTION('ref_axis',(0.984807753012213,0.,-0.173648177666902));
#86223=DIRECTION('center_axis',(-0.173648177666902,0.,-0.984807753012213));
#86224=DIRECTION('ref_axis',(0.984807753012213,0.,-0.173648177666902));
#86225=DIRECTION('',(0.173648177666902,0.,0.984807753012213));
#86226=DIRECTION('center_axis',(0.0387475933097257,0.999225688321113,-0.00682992034369552));
#86227=DIRECTION('ref_axis',(-0.999147598170087,0.0386453691656854,-0.0145124950643757));
#86228=DIRECTION('center_axis',(0.984807753012213,0.,-0.173648177666902));
#86229=DIRECTION('ref_axis',(-0.173648177666902,0.,-0.984807753012213));
#86230=DIRECTION('center_axis',(0.,-1.,0.));
#86231=DIRECTION('ref_axis',(0.,0.,-1.));
#86232=DIRECTION('',(0.984811647878971,1.54338751793195E-8,-0.173626087331095));
#86233=DIRECTION('center_axis',(0.984807753012213,0.,-0.173648177666902));
#86234=DIRECTION('ref_axis',(0.173648177666902,0.,0.984807753012213));
#86235=DIRECTION('',(0.984807759252478,-3.52789443014592E-8,-0.173648142276596));
#86236=DIRECTION('center_axis',(0.810782065545516,0.460194129063917,-0.361737205392049));
#86237=DIRECTION('ref_axis',(0.0802095373079066,-0.699502947700354,-0.710114114972634));
#86238=DIRECTION('center_axis',(0.173648177666902,0.,0.984807753012213));
#86239=DIRECTION('ref_axis',(0.,-1.,0.));
#86240=DIRECTION('center_axis',(-1.,0.,0.));
#86241=DIRECTION('ref_axis',(0.,1.,0.));
#86242=DIRECTION('',(-1.,0.,0.));
#86243=DIRECTION('center_axis',(-1.,0.,0.));
#86244=DIRECTION('ref_axis',(0.,0.139931005087302,0.990161256470509));
#86245=DIRECTION('center_axis',(-1.,0.,0.));
#86246=DIRECTION('ref_axis',(0.,1.,0.));
#86247=DIRECTION('',(-1.,0.,0.));
#86248=DIRECTION('center_axis',(-1.,0.,0.));
#86249=DIRECTION('ref_axis',(0.,1.,0.));
#86250=DIRECTION('',(-1.,0.,0.));
#86251=DIRECTION('center_axis',(1.,0.,0.));
#86252=DIRECTION('ref_axis',(0.,-1.,0.));
#86253=DIRECTION('',(1.,0.,0.));
#86254=DIRECTION('center_axis',(-1.,0.,0.));
#86255=DIRECTION('ref_axis',(0.,-0.992397367379901,-0.1230750389699));
#86256=DIRECTION('center_axis',(1.,0.,0.));
#86257=DIRECTION('ref_axis',(0.,-1.,0.));
#86258=DIRECTION('',(1.,0.,0.));
#86259=DIRECTION('center_axis',(1.,0.,0.));
#86260=DIRECTION('ref_axis',(0.,-1.,0.));
#86261=DIRECTION('',(1.,0.,0.));
#86262=DIRECTION('center_axis',(-1.,0.,0.));
#86263=DIRECTION('ref_axis',(0.,-0.857325768567308,-0.514774248142304));
#86264=DIRECTION('center_axis',(0.173648177666903,0.,0.984807753012213));
#86265=DIRECTION('ref_axis',(0.984807753012213,0.,-0.173648177666903));
#86266=DIRECTION('',(0.173648177666903,0.,0.984807753012213));
#86267=DIRECTION('',(0.173648177666903,0.,0.984807753012213));
#86268=DIRECTION('center_axis',(0.173648177666903,0.,0.984807753012213));
#86269=DIRECTION('ref_axis',(0.984807753012213,0.,-0.173648177666903));
#86270=DIRECTION('',(0.173648177666903,0.,0.984807753012213));
#86271=DIRECTION('center_axis',(0.173648177666903,0.,0.984807753012213));
#86272=DIRECTION('ref_axis',(0.984807753012213,0.,-0.173648177666903));
#86273=DIRECTION('',(0.173648177666903,0.,0.984807753012213));
#86274=DIRECTION('center_axis',(0.173648177666903,0.,0.984807753012213));
#86275=DIRECTION('ref_axis',(0.984807753012213,0.,-0.173648177666903));
#86276=DIRECTION('',(0.173648177666903,0.,0.984807753012213));
#86277=DIRECTION('center_axis',(0.173648177666903,0.,0.984807753012213));
#86278=DIRECTION('ref_axis',(0.984807753012213,0.,-0.173648177666903));
#86279=DIRECTION('',(0.173648177666903,0.,0.984807753012213));
#86280=DIRECTION('center_axis',(-0.173648177666903,0.,-0.984807753012213));
#86281=DIRECTION('ref_axis',(-0.984807753012213,0.,0.173648177666903));
#86282=DIRECTION('center_axis',(0.173648177666903,0.,0.984807753012213));
#86283=DIRECTION('ref_axis',(0.,-1.,0.));
#86284=DIRECTION('',(0.173648177666903,0.,0.984807753012213));
#86285=DIRECTION('',(-0.173648177666903,0.,-0.984807753012213));
#86286=DIRECTION('',(0.173648177666903,0.,0.984807753012213));
#86287=DIRECTION('center_axis',(0.173648177666903,0.,0.984807753012213));
#86288=DIRECTION('ref_axis',(0.,-1.,0.));
#86289=DIRECTION('center_axis',(0.173648177666903,0.,0.984807753012213));
#86290=DIRECTION('ref_axis',(0.,-1.,0.));
#86291=DIRECTION('center_axis',(0.173648177666903,0.,0.984807753012213));
#86292=DIRECTION('ref_axis',(0.,-1.,0.));
#86293=DIRECTION('',(0.173648177666903,0.,0.984807753012213));
#86294=DIRECTION('center_axis',(0.173648177666903,0.,0.984807753012213));
#86295=DIRECTION('ref_axis',(0.,-1.,0.));
#86296=DIRECTION('',(0.173648177666903,0.,0.984807753012213));
#86297=DIRECTION('center_axis',(-0.173648177666903,0.,-0.984807753012213));
#86298=DIRECTION('ref_axis',(0.984807753012213,0.,-0.173648177666903));
#86299=DIRECTION('center_axis',(0.173648177666902,0.,0.984807753012213));
#86300=DIRECTION('ref_axis',(0.984807753012213,0.,-0.173648177666902));
#86301=DIRECTION('center_axis',(-3.77535033790721E-16,-1.,-2.84635355732631E-15));
#86302=DIRECTION('ref_axis',(-0.984807753012204,-1.22464679914735E-16,0.173648177666953));
#86303=DIRECTION('center_axis',(0.173648177666902,0.,0.984807753012213));
#86304=DIRECTION('ref_axis',(0.984807753012213,0.,-0.173648177666902));
#86305=DIRECTION('center_axis',(0.173648177666902,0.,0.984807753012213));
#86306=DIRECTION('ref_axis',(0.984807753012213,0.,-0.173648177666902));
#86307=DIRECTION('center_axis',(-0.173648177666902,0.,-0.984807753012213));
#86308=DIRECTION('ref_axis',(-0.984807753012213,0.,0.173648177666902));
#86309=DIRECTION('center_axis',(0.173648177666902,0.,0.984807753012213));
#86310=DIRECTION('ref_axis',(-0.984807753012213,0.,0.173648177666902));
#86311=DIRECTION('center_axis',(0.173648177666902,0.,0.984807753012213));
#86312=DIRECTION('ref_axis',(-0.984807753012213,0.,0.173648177666902));
#86313=DIRECTION('center_axis',(-0.62194003125718,0.74694017202758,-0.235097802905997));
#86314=DIRECTION('ref_axis',(-0.677339878007115,-0.362498100233908,0.640160774327914));
#86315=DIRECTION('center_axis',(0.621933305629086,-0.746947822272283,0.235091288975095));
#86316=DIRECTION('ref_axis',(0.353583401256323,2.62174188094628E-7,-0.935403003178813));
#86317=DIRECTION('center_axis',(0.39293929197921,0.557382729135213,0.73138444478992));
#86318=DIRECTION('ref_axis',(0.677339878007116,0.362498100233908,-0.640160774327913));
#86319=DIRECTION('center_axis',(0.621933305629086,-0.746947822272283,0.235091288975095));
#86320=DIRECTION('ref_axis',(0.353583401256323,2.62174188094628E-7,-0.935403003178813));
#86321=DIRECTION('center_axis',(0.173648177666902,0.,0.984807753012213));
#86322=DIRECTION('ref_axis',(0.782050857825719,0.607767196495907,-0.137896666520851));
#86323=DIRECTION('center_axis',(0.,1.,0.));
#86324=DIRECTION('ref_axis',(0.353585017730993,0.,-0.935402392147985));
#86325=DIRECTION('center_axis',(0.,1.,0.));
#86326=DIRECTION('ref_axis',(1.,0.,0.));
#86327=DIRECTION('center_axis',(0.,-1.,0.));
#86328=DIRECTION('ref_axis',(0.916673510305537,0.,-0.399636929605017));
#86329=DIRECTION('',(1.794251608235E-8,-0.999999999999999,4.127905851638E-8));
#86330=DIRECTION('',(-5.50004478946E-11,-1.,-3.753192811798E-11));
#86331=DIRECTION('center_axis',(3.02975422528107E-10,-1.,-4.69337161727405E-11));
#86332=DIRECTION('ref_axis',(0.312852999424802,5.02069497088088E-11,0.949801558616801));
#86333=DIRECTION('center_axis',(0.,1.,0.));
#86334=DIRECTION('ref_axis',(0.173648177666898,0.,0.984807753012214));
#86335=DIRECTION('center_axis',(0.173648177666904,2.09451819877512E-15,
0.984807753012213));
#86336=DIRECTION('ref_axis',(-0.681789982854609,-0.721602424588219,0.120217969154012));
#86337=DIRECTION('center_axis',(0.710639662326888,-0.692307692307688,-0.125304946029797));
#86338=DIRECTION('ref_axis',(0.173648177666926,-2.4450854095363E-14,0.984807753012209));
#86339=DIRECTION('center_axis',(-0.173648177666902,-1.35349239628917E-17,
-0.984807753012213));
#86340=DIRECTION('ref_axis',(2.35031488101622E-18,-1.,1.33292980550865E-17));
#86341=DIRECTION('center_axis',(0.173648177666902,0.,0.984807753012213));
#86342=DIRECTION('ref_axis',(0.984807753012213,0.,-0.173648177666902));
#86343=DIRECTION('',(0.573567618895493,-3.99540154301384E-14,-0.819158218267115));
#86344=DIRECTION('center_axis',(0.173648177666902,0.,0.984807753012213));
#86345=DIRECTION('ref_axis',(-0.984807753012213,0.,0.173648177666902));
#86346=DIRECTION('',(-0.819139113627864,-3.7946361193661E-14,-0.573594902805942));
#86347=DIRECTION('center_axis',(0.173648177666902,0.,0.984807753012213));
#86348=DIRECTION('ref_axis',(-0.984807753012213,0.,0.173648177666902));
#86349=DIRECTION('center_axis',(0.173648177666902,0.,0.984807753012213));
#86350=DIRECTION('ref_axis',(0.984807753012213,0.,-0.173648177666902));
#86351=DIRECTION('',(0.173648177666902,0.,0.984807753012213));
#86352=DIRECTION('center_axis',(0.173648177666902,0.,0.984807753012213));
#86353=DIRECTION('ref_axis',(-0.984807753012213,0.,0.173648177666902));
#86354=DIRECTION('center_axis',(0.173648177666902,0.,0.984807753012213));
#86355=DIRECTION('ref_axis',(0.984807753012213,0.,-0.173648177666902));
#86356=DIRECTION('center_axis',(0.173648177666903,-1.10104762772743E-17,
0.984807753012213));
#86357=DIRECTION('ref_axis',(-0.984138869602196,0.0368502742755397,0.173530235474769));
#86358=DIRECTION('center_axis',(0.173648177666902,0.,0.984807753012213));
#86359=DIRECTION('ref_axis',(-0.984807753012213,0.,0.173648177666902));
#86360=DIRECTION('center_axis',(0.0362904358071779,0.99932079798522,-0.00639898297447297));
#86361=DIRECTION('ref_axis',(0.984138869602196,-0.0368502742755396,-0.173530235474768));
#86362=DIRECTION('center_axis',(0.173648177666902,0.,0.984807753012213));
#86363=DIRECTION('ref_axis',(-0.984807753012213,0.,0.173648177666902));
#86364=DIRECTION('center_axis',(0.173648177666902,0.,0.984807753012213));
#86365=DIRECTION('ref_axis',(0.984807753012213,0.,-0.173648177666902));
#86366=DIRECTION('',(0.173648177666902,0.,0.984807753012213));
#86367=DIRECTION('center_axis',(0.173648177666902,0.,0.984807753012213));
#86368=DIRECTION('ref_axis',(-0.984807753012213,0.,0.173648177666902));
#86369=DIRECTION('center_axis',(0.173648177666902,0.,0.984807753012213));
#86370=DIRECTION('ref_axis',(0.984807753012213,0.,-0.173648177666902));
#86371=DIRECTION('center_axis',(0.173648177666902,-8.04145241919534E-18,
0.984807753012213));
#86372=DIRECTION('ref_axis',(-0.984225072739169,0.0343945931603786,0.173545435413638));
#86373=DIRECTION('center_axis',(0.173648177666902,0.,0.984807753012213));
#86374=DIRECTION('ref_axis',(-0.984807753012213,0.,0.173648177666902));
#86375=DIRECTION('center_axis',(0.0338720620060416,0.99940833094453,-0.00597255842389421));
#86376=DIRECTION('ref_axis',(0.984225072739169,-0.0343945931603785,-0.173545435413638));
#86377=DIRECTION('center_axis',(0.,1.,0.));
#86378=DIRECTION('ref_axis',(1.,0.,0.));
#86379=DIRECTION('center_axis',(0.,1.,0.));
#86380=DIRECTION('ref_axis',(1.,0.,0.));
#86381=DIRECTION('center_axis',(0.399636929605014,0.,0.916673510305538));
#86382=DIRECTION('ref_axis',(0.916673510305538,0.,-0.399636929605014));
#86383=DIRECTION('center_axis',(0.,1.,0.));
#86384=DIRECTION('ref_axis',(1.,0.,0.));
#86385=DIRECTION('center_axis',(0.399636929605016,0.,-0.916673510305537));
#86386=DIRECTION('ref_axis',(0.,1.,0.));
#86387=DIRECTION('center_axis',(0.,1.,0.));
#86388=DIRECTION('ref_axis',(1.,0.,0.));
#86389=DIRECTION('',(3.93130974098696E-8,-0.999999999999995,9.01091822956491E-8));
#86390=DIRECTION('',(1.026064694511E-11,-1.,6.99782860462E-12));
#86391=DIRECTION('center_axis',(-0.173648177666902,0.,-0.984807753012213));
#86392=DIRECTION('ref_axis',(-0.984807753012213,0.,0.173648177666902));
#86393=DIRECTION('center_axis',(-0.803670499663718,1.75978326149641E-7,
0.595074556648357));
#86394=DIRECTION('ref_axis',(0.595074539966384,-0.000236546883935123,0.80367047720404));
#86395=DIRECTION('',(0.173648177666902,0.,0.984807753012213));
#86396=DIRECTION('center_axis',(0.173648177666902,0.,0.984807753012213));
#86397=DIRECTION('ref_axis',(0.984807753012213,0.,-0.173648177666902));
#86398=DIRECTION('center_axis',(-0.803670499663718,1.75978326149641E-7,
0.595074556648357));
#86399=DIRECTION('ref_axis',(0.595074539966384,-0.000236546883935123,0.80367047720404));
#86400=DIRECTION('center_axis',(0.,1.,0.));
#86401=DIRECTION('ref_axis',(1.,0.,0.));
#86402=DIRECTION('center_axis',(0.,-1.,0.));
#86403=DIRECTION('ref_axis',(1.,0.,0.));
#86404=DIRECTION('center_axis',(0.399636929605016,0.,0.916673510305537));
#86405=DIRECTION('ref_axis',(0.,-1.,0.));
#86406=DIRECTION('center_axis',(0.399636929605014,0.,-0.916673510305538));
#86407=DIRECTION('ref_axis',(0.916673510305538,0.,0.399636929605014));
#86408=DIRECTION('center_axis',(0.,-1.,0.));
#86409=DIRECTION('ref_axis',(-1.,0.,0.));
#86410=DIRECTION('',(1.548136098957E-14,1.,-3.664781422684E-14));
#86411=DIRECTION('',(0.,-1.,0.));
#86412=DIRECTION('center_axis',(-0.62193825517579,-0.746941405650846,-0.235098582031521));
#86413=DIRECTION('ref_axis',(-0.677340854507514,0.362495984395913,0.640160939226901));
#86414=DIRECTION('center_axis',(0.621933330370316,0.746947780441719,0.235091356429106));
#86415=DIRECTION('ref_axis',(0.782054095085269,-0.607763215737225,-0.137895851848809));
#86416=DIRECTION('center_axis',(-0.392940419865306,0.55738245202121,-0.731384050014013));
#86417=DIRECTION('ref_axis',(0.677340854507515,-0.362495984395913,-0.640160939226901));
#86418=DIRECTION('center_axis',(0.621933330370316,0.746947780441719,0.235091356429106));
#86419=DIRECTION('ref_axis',(0.782054095085269,-0.607763215737225,-0.137895851848809));
#86420=DIRECTION('center_axis',(0.,1.,0.));
#86421=DIRECTION('ref_axis',(0.353584869536014,0.,-0.935402448166135));
#86422=DIRECTION('center_axis',(-0.173648177666903,7.27812871698714E-16,
-0.984807753012213));
#86423=DIRECTION('ref_axis',(0.782051073965749,-0.607766909728233,-0.137896704632171));
#86424=DIRECTION('center_axis',(0.173648177666902,0.,0.984807753012213));
#86425=DIRECTION('ref_axis',(-0.984807753012213,0.,0.173648177666902));
#86426=DIRECTION('center_axis',(0.173648177666902,0.,0.984807753012213));
#86427=DIRECTION('ref_axis',(0.984807753012213,0.,-0.173648177666902));
#86428=DIRECTION('',(0.173648177666902,0.,0.984807753012213));
#86429=DIRECTION('center_axis',(0.173648177666903,1.2793705768531E-16,0.984807753012213));
#86430=DIRECTION('ref_axis',(0.9329757660115,0.320145396331696,-0.164508799894948));
#86431=DIRECTION('center_axis',(0.173648177666902,4.8935450121219E-18,0.984807753012213));
#86432=DIRECTION('ref_axis',(-0.983580074845734,0.0499167317439819,0.173431704882525));
#86433=DIRECTION('center_axis',(0.173648177666903,0.,0.984807753012213));
#86434=DIRECTION('ref_axis',(0.984807753012213,0.,-0.173648177666903));
#86435=DIRECTION('center_axis',(0.0491583844265041,0.998753382918926,-0.00866794950243004));
#86436=DIRECTION('ref_axis',(0.983580074845734,-0.0499167317439817,-0.173431704882525));
#86437=DIRECTION('center_axis',(0.173648177666902,0.,0.984807753012213));
#86438=DIRECTION('ref_axis',(0.984807753012213,0.,-0.173648177666902));
#86439=DIRECTION('center_axis',(0.173648177666902,0.,0.984807753012213));
#86440=DIRECTION('ref_axis',(0.984807753012213,0.,-0.173648177666902));
#86441=DIRECTION('center_axis',(0.173648177666902,0.,0.984807753012213));
#86442=DIRECTION('ref_axis',(-0.984807753012213,0.,0.173648177666902));
#86443=DIRECTION('',(0.173648177666902,0.,0.984807753012213));
#86444=DIRECTION('center_axis',(0.173648177666902,0.,0.984807753012213));
#86445=DIRECTION('ref_axis',(-0.984807753012213,0.,0.173648177666902));
#86446=DIRECTION('center_axis',(0.173648177666902,0.,0.984807753012213));
#86447=DIRECTION('ref_axis',(-0.984807753012213,0.,0.173648177666902));
#86448=DIRECTION('center_axis',(0.173648177666903,0.,0.984807753012213));
#86449=DIRECTION('ref_axis',(-0.984807753012213,0.,0.173648177666903));
#86450=DIRECTION('',(0.173648177666902,0.,0.984807753012213));
#86451=DIRECTION('center_axis',(0.173648177666903,0.,0.984807753012213));
#86452=DIRECTION('ref_axis',(0.984807753012213,0.,-0.173648177666903));
#86453=DIRECTION('center_axis',(0.173648177666903,0.,0.984807753012213));
#86454=DIRECTION('ref_axis',(0.984807753012213,0.,-0.173648177666903));
#86455=DIRECTION('center_axis',(0.190809912898503,0.,-0.981627005099017));
#86456=DIRECTION('ref_axis',(0.981627005099017,0.,0.190809912898503));
#86457=DIRECTION('center_axis',(-0.190809912898503,0.,0.981627005099017));
#86458=DIRECTION('ref_axis',(0.981627005099017,0.,0.190809912898503));
#86459=DIRECTION('center_axis',(0.190809912898503,0.,-0.981627005099017));
#86460=DIRECTION('ref_axis',(-0.981627005099017,0.,-0.190809912898503));
#86461=DIRECTION('',(0.190809912898503,0.,-0.981627005099017));
#86462=DIRECTION('center_axis',(0.190809912898503,0.,-0.981627005099017));
#86463=DIRECTION('ref_axis',(0.981627005099017,0.,0.190809912898503));
#86464=DIRECTION('center_axis',(0.190809912898503,0.,-0.981627005099017));
#86465=DIRECTION('ref_axis',(-0.981627005099017,0.,-0.190809912898503));
#86466=DIRECTION('center_axis',(0.190809912898503,0.,-0.981627005099017));
#86467=DIRECTION('ref_axis',(0.981627005099017,0.,0.190809912898503));
#86468=DIRECTION('center_axis',(0.190809912898503,0.,-0.981627005099017));
#86469=DIRECTION('ref_axis',(0.981627005099017,0.,0.190809912898503));
#86470=DIRECTION('',(0.190809912898503,0.,-0.981627005099017));
#86471=DIRECTION('center_axis',(0.190809912898503,0.,-0.981627005099017));
#86472=DIRECTION('ref_axis',(0.981627005099017,0.,0.190809912898503));
#86473=DIRECTION('center_axis',(0.190809912898503,0.,-0.981627005099017));
#86474=DIRECTION('ref_axis',(0.981627005099017,0.,0.190809912898503));
#86475=DIRECTION('center_axis',(0.190809912898503,2.42635641189931E-17,
-0.981627005099017));
#86476=DIRECTION('ref_axis',(4.62972855615232E-18,-1.,-2.38177697791552E-17));
#86477=DIRECTION('',(0.134925187626816,0.707095228669965,-0.69412645197834));
#86478=DIRECTION('center_axis',(0.190809912898503,0.,-0.981627005099017));
#86479=DIRECTION('ref_axis',(0.981627005099017,0.,0.190809912898503));
#86480=DIRECTION('center_axis',(0.190809912898504,0.,-0.981627005099017));
#86481=DIRECTION('ref_axis',(0.981627005099017,0.,0.190809912898504));
#86482=DIRECTION('center_axis',(0.190809912898503,0.,-0.981627005099017));
#86483=DIRECTION('ref_axis',(0.981627005099017,0.,0.190809912898503));
#86484=DIRECTION('',(0.190809912898504,0.,-0.981627005099017));
#86485=DIRECTION('center_axis',(0.190809912898504,0.,-0.981627005099017));
#86486=DIRECTION('ref_axis',(-0.981627005099017,0.,-0.190809912898504));
#86487=DIRECTION('center_axis',(0.173648177666903,0.,0.984807753012213));
#86488=DIRECTION('ref_axis',(-0.984807753012213,0.,0.173648177666903));
#86489=DIRECTION('center_axis',(0.173648177666902,0.,0.984807753012213));
#86490=DIRECTION('ref_axis',(-0.984807753012213,0.,0.173648177666902));
#86491=DIRECTION('',(0.173648177666903,0.,0.984807753012213));
#86492=DIRECTION('center_axis',(0.403404352147799,-6.13683761632244E-5,
-0.915021816626324));
#86493=DIRECTION('ref_axis',(0.914262104708908,-0.0407141998164361,0.403072149653813));
#86494=DIRECTION('center_axis',(-0.691975445312705,-6.74709518344435E-5,
-0.721921033446148));
#86495=DIRECTION('ref_axis',(0.721885115931311,0.00991088319453953,-0.691941943945547));
#86496=DIRECTION('center_axis',(-0.692027149057367,6.1891542016879E-5,-0.721871471341657));
#86497=DIRECTION('ref_axis',(0.721167827159643,-0.0440831886297046,-0.691356375214749));
#86498=DIRECTION('center_axis',(0.403333139961256,6.74332542398484E-5,-0.915053208104179));
#86499=DIRECTION('ref_axis',(0.914881149946327,0.0193618170927673,0.403258727756452));
#86500=DIRECTION('center_axis',(0.173648177666903,-3.1720657846433E-17,
0.984807753012213));
#86501=DIRECTION('ref_axis',(-0.982890310181394,0.0623719011882791,0.173310080761864));
#86502=DIRECTION('center_axis',(0.173648177666903,0.,0.984807753012213));
#86503=DIRECTION('ref_axis',(0.984807753012213,0.,-0.173648177666903));
#86504=DIRECTION('center_axis',(0.173648177666903,0.,0.984807753012213));
#86505=DIRECTION('ref_axis',(0.984807753012213,0.,-0.173648177666903));
#86506=DIRECTION('center_axis',(0.0614243318603288,0.998052977522816,-0.0108307669789647));
#86507=DIRECTION('ref_axis',(0.982890310181394,-0.062371901188279,-0.173310080761863));
#86508=DIRECTION('center_axis',(0.173648177666903,0.,0.984807753012213));
#86509=DIRECTION('ref_axis',(0.984807753012213,0.,-0.173648177666903));
#86510=DIRECTION('center_axis',(0.173648177666902,0.,0.984807753012213));
#86511=DIRECTION('ref_axis',(-0.984807753012213,0.,0.173648177666902));
#86512=DIRECTION('center_axis',(0.173648177666903,0.,0.984807753012213));
#86513=DIRECTION('ref_axis',(-0.984807753012213,0.,0.173648177666903));
#86514=DIRECTION('',(0.173648177666902,0.,0.984807753012213));
#86515=DIRECTION('center_axis',(0.173648177666902,-5.19592868310163E-17,
0.984807753012213));
#86516=DIRECTION('ref_axis',(-9.02263547107784E-18,-1.,-5.11699085121702E-17));
#86517=DIRECTION('center_axis',(0.173648177666902,0.,0.984807753012213));
#86518=DIRECTION('ref_axis',(-0.984807753012213,0.,0.173648177666902));
#86519=DIRECTION('',(0.12279097479207,0.707088520672423,0.696382222951518));
#86520=DIRECTION('center_axis',(0.173648177666902,0.,0.984807753012213));
#86521=DIRECTION('ref_axis',(-0.984807753012213,0.,0.173648177666902));
#86522=DIRECTION('center_axis',(0.173648177666902,0.,0.984807753012213));
#86523=DIRECTION('ref_axis',(-0.984807753012213,0.,0.173648177666902));
#86524=DIRECTION('center_axis',(0.173648177666902,0.,0.984807753012213));
#86525=DIRECTION('ref_axis',(-0.984807753012213,0.,0.173648177666902));
#86526=DIRECTION('center_axis',(0.173648177666902,0.,0.984807753012213));
#86527=DIRECTION('ref_axis',(0.984807753012213,0.,-0.173648177666902));
#86528=DIRECTION('center_axis',(0.173648177666902,0.,0.984807753012213));
#86529=DIRECTION('ref_axis',(0.984807753012213,0.,-0.173648177666902));
#86530=DIRECTION('',(0.173648177666902,0.,0.984807753012213));
#86531=DIRECTION('center_axis',(-0.173648177666902,0.,-0.984807753012213));
#86532=DIRECTION('ref_axis',(0.984807753012213,0.,-0.173648177666902));
#86533=DIRECTION('center_axis',(0.768062672188182,-3.57030663143955E-6,
-0.640374680619403));
#86534=DIRECTION('ref_axis',(0.640373969760258,-0.00148573958139851,0.768061827870247));
#86535=DIRECTION('center_axis',(-0.173648177666902,-1.37778369814978E-16,
-0.984807753012213));
#86536=DIRECTION('ref_axis',(0.791088680366871,0.59558472277628,-0.139490278481711));
#86537=DIRECTION('center_axis',(0.,-1.,0.));
#86538=DIRECTION('ref_axis',(-1.,0.,0.));
#86539=DIRECTION('center_axis',(0.,1.,0.));
#86540=DIRECTION('ref_axis',(-0.92054989510347,0.,-0.390624999999987));
#86541=DIRECTION('',(2.085442929456E-13,-1.,6.417977260753E-13));
#86542=DIRECTION('center_axis',(0.,-1.,0.));
#86543=DIRECTION('ref_axis',(-0.951104406813915,0.,0.308869563633505));
#86544=DIRECTION('',(2.04281036531E-14,1.,-4.831690603169E-14));
#86545=DIRECTION('center_axis',(0.173648177666903,0.,0.984807753012213));
#86546=DIRECTION('ref_axis',(0.,-1.,0.));
#86547=DIRECTION('center_axis',(0.173648177666903,0.,0.984807753012213));
#86548=DIRECTION('ref_axis',(0.,-1.,0.));
#86549=DIRECTION('center_axis',(-0.173648177666902,0.,-0.984807753012213));
#86550=DIRECTION('ref_axis',(0.984807753012213,0.,-0.173648177666902));
#86551=DIRECTION('',(0.173648177666903,0.,0.984807753012213));
#86552=DIRECTION('center_axis',(0.173648177666902,0.,0.984807753012213));
#86553=DIRECTION('ref_axis',(0.984807753012213,0.,-0.173648177666902));
#86554=DIRECTION('center_axis',(-0.173648177666902,0.,-0.984807753012213));
#86555=DIRECTION('ref_axis',(0.984807753012213,0.,-0.173648177666902));
#86556=DIRECTION('center_axis',(-0.173648177666903,0.,-0.984807753012213));
#86557=DIRECTION('ref_axis',(-0.984807753012213,0.,0.173648177666903));
#86558=DIRECTION('',(0.0425655252567249,-2.63800745320352E-17,-0.999093677319409));
#86559=DIRECTION('center_axis',(-0.173648177666903,0.,-0.984807753012213));
#86560=DIRECTION('ref_axis',(-0.984807753012213,0.,0.173648177666903));
#86561=DIRECTION('center_axis',(-0.173648177666903,0.,-0.984807753012213));
#86562=DIRECTION('ref_axis',(-0.984807753012213,0.,0.173648177666903));
#86563=DIRECTION('',(0.573576435615923,-8.65956055458343E-17,-0.819152044803731));
#86564=DIRECTION('center_axis',(0.173648177666903,0.,0.984807753012213));
#86565=DIRECTION('ref_axis',(0.984807753012213,0.,-0.173648177666903));
#86566=DIRECTION('center_axis',(0.173648177666903,0.,0.984807753012213));
#86567=DIRECTION('ref_axis',(0.984807753012213,0.,-0.173648177666903));
#86568=DIRECTION('center_axis',(1.,0.,0.));
#86569=DIRECTION('ref_axis',(0.,0.999170306594043,-0.040727121439721));
#86570=DIRECTION('center_axis',(1.,0.,0.));
#86571=DIRECTION('ref_axis',(0.,-1.,0.));
#86572=DIRECTION('center_axis',(0.,-0.0407271214397213,-0.999170306594043));
#86573=DIRECTION('ref_axis',(0.,-0.999170306594043,0.0407271214397213));
#86574=DIRECTION('center_axis',(1.,0.,0.));
#86575=DIRECTION('ref_axis',(0.,-1.,0.));
#86576=DIRECTION('center_axis',(1.,0.,0.));
#86577=DIRECTION('ref_axis',(0.,-1.,0.));
#86578=DIRECTION('center_axis',(1.,0.,0.));
#86579=DIRECTION('ref_axis',(0.,-1.,0.));
#86580=DIRECTION('',(1.,0.,0.));
#86581=DIRECTION('center_axis',(-1.,0.,0.));
#86582=DIRECTION('ref_axis',(0.,-1.,0.));
#86583=DIRECTION('center_axis',(-1.,-1.04909975265626E-16,0.));
#86584=DIRECTION('ref_axis',(-7.91782854057881E-17,0.754725994409142,0.656040146151995));
#86585=DIRECTION('center_axis',(1.,0.,0.));
#86586=DIRECTION('ref_axis',(0.,-0.628687890661713,-0.777657724281915));
#86587=DIRECTION('center_axis',(1.,0.,0.));
#86588=DIRECTION('ref_axis',(0.,-1.,0.));
#86589=DIRECTION('center_axis',(-1.,0.,0.));
#86590=DIRECTION('ref_axis',(0.,0.,1.));
#86591=DIRECTION('',(1.,0.,0.));
#86592=DIRECTION('center_axis',(-1.,0.,0.));
#86593=DIRECTION('ref_axis',(0.,0.,1.));
#86594=DIRECTION('center_axis',(0.,-1.,0.));
#86595=DIRECTION('ref_axis',(-1.,0.,0.));
#86596=DIRECTION('center_axis',(0.,-1.,0.));
#86597=DIRECTION('ref_axis',(-0.951104406813915,0.,0.308869563633505));
#86598=DIRECTION('',(-1.424093909463E-10,-1.,-4.385222496239E-10));
#86599=DIRECTION('center_axis',(0.,-1.,0.));
#86600=DIRECTION('ref_axis',(-0.92054989510347,0.,0.390624999999987));
#86601=DIRECTION('',(0.,-1.,0.));
#86602=DIRECTION('',(0.,1.,0.));
#86603=DIRECTION('center_axis',(0.,1.,0.));
#86604=DIRECTION('ref_axis',(1.,0.,0.));
#86605=DIRECTION('center_axis',(0.,-1.,0.));
#86606=DIRECTION('ref_axis',(0.916673510305537,0.,-0.399636929605016));
#86607=DIRECTION('',(1.15953143331196E-6,-0.999999999996469,-2.39123208817793E-6));
#86608=DIRECTION('',(9.96499151473735E-7,-0.999999999997636,1.93274404172707E-6));
#86609=DIRECTION('center_axis',(-1.,0.,0.));
#86610=DIRECTION('ref_axis',(0.,0.,1.));
#86611=DIRECTION('center_axis',(-1.,0.,0.));
#86612=DIRECTION('ref_axis',(0.,0.,1.));
#86613=DIRECTION('',(1.,0.,0.));
#86614=DIRECTION('center_axis',(1.,0.,0.));
#86615=DIRECTION('ref_axis',(0.,0.,1.));
#86616=DIRECTION('center_axis',(-1.,0.,0.));
#86617=DIRECTION('ref_axis',(0.,0.,1.));
#86618=DIRECTION('center_axis',(1.,0.,0.));
#86619=DIRECTION('ref_axis',(0.,0.,1.));
#86620=DIRECTION('',(1.,0.,0.));
#86621=DIRECTION('center_axis',(-1.,0.,0.));
#86622=DIRECTION('ref_axis',(0.,0.,1.));
#86623=DIRECTION('center_axis',(1.,0.,0.));
#86624=DIRECTION('ref_axis',(0.,0.,1.));
#86625=DIRECTION('center_axis',(1.,0.,6.86169978136685E-18));
#86626=DIRECTION('ref_axis',(6.86169978136685E-18,0.,-1.));
#86627=DIRECTION('',(-0.707106781821139,8.65956055458343E-17,-0.707106780551956));
#86628=DIRECTION('center_axis',(-1.,0.,0.));
#86629=DIRECTION('ref_axis',(0.,0.,1.));
#86630=DIRECTION('center_axis',(1.,0.,0.));
#86631=DIRECTION('ref_axis',(0.,0.,-1.));
#86632=DIRECTION('center_axis',(-1.,0.,0.));
#86633=DIRECTION('ref_axis',(0.,0.,1.));
#86634=DIRECTION('',(1.,0.,0.));
#86635=DIRECTION('center_axis',(-1.,0.,0.));
#86636=DIRECTION('ref_axis',(0.,0.,-1.));
#86637=DIRECTION('center_axis',(-1.,0.,0.));
#86638=DIRECTION('ref_axis',(0.,0.,-1.));
#86639=DIRECTION('center_axis',(-1.,0.,0.));
#86640=DIRECTION('ref_axis',(0.,0.,1.));
#86641=DIRECTION('center_axis',(-1.,0.,-2.79182864590248E-17));
#86642=DIRECTION('ref_axis',(-2.79182864590248E-17,0.,1.));
#86643=DIRECTION('',(-0.500000001036284,-1.0605752379922E-16,-0.86602540318614));
#86644=DIRECTION('center_axis',(-1.,0.,6.88416479379655E-18));
#86645=DIRECTION('ref_axis',(6.88416479379655E-18,0.,1.));
#86646=DIRECTION('',(-0.707106781821139,-8.65956055458343E-17,-0.707106780551956));
#86647=DIRECTION('center_axis',(1.,0.,0.));
#86648=DIRECTION('ref_axis',(0.,0.,1.));
#86649=DIRECTION('center_axis',(-1.,0.,0.));
#86650=DIRECTION('ref_axis',(0.,-0.998325932398639,0.057838851133022));
#86651=DIRECTION('center_axis',(1.,0.,0.));
#86652=DIRECTION('ref_axis',(0.,1.,0.));
#86653=DIRECTION('center_axis',(1.,0.,0.));
#86654=DIRECTION('ref_axis',(0.,1.,0.));
#86655=DIRECTION('center_axis',(0.,-0.0578388511330215,-0.998325932398639));
#86656=DIRECTION('ref_axis',(0.,0.998325932398639,-0.0578388511330215));
#86657=DIRECTION('center_axis',(-1.,0.,0.));
#86658=DIRECTION('ref_axis',(0.,0.,1.));
#86659=DIRECTION('center_axis',(-1.,0.,0.));
#86660=DIRECTION('ref_axis',(0.,1.,0.));
#86661=DIRECTION('center_axis',(-1.,0.,0.));
#86662=DIRECTION('ref_axis',(0.,1.,0.));
#86663=DIRECTION('',(-1.,0.,0.));
#86664=DIRECTION('center_axis',(-1.,1.71983566009223E-17,0.));
#86665=DIRECTION('ref_axis',(-1.29799163280414E-17,-0.754718408812697,0.656048872721561));
#86666=DIRECTION('center_axis',(1.,0.,0.));
#86667=DIRECTION('ref_axis',(0.,0.867366884881976,0.497669254636186));
#86668=DIRECTION('center_axis',(-1.,0.,0.));
#86669=DIRECTION('ref_axis',(0.,1.,0.));
#86670=DIRECTION('center_axis',(-1.,0.,0.));
#86671=DIRECTION('ref_axis',(0.,-0.27343727392181,0.961889836327534));
#86672=DIRECTION('center_axis',(-1.,0.,0.));
#86673=DIRECTION('ref_axis',(0.,0.,1.));
#86674=DIRECTION('',(1.,0.,0.));
#86675=DIRECTION('center_axis',(-1.,0.,0.));
#86676=DIRECTION('ref_axis',(0.,0.,-1.));
#86677=DIRECTION('center_axis',(0.,-1.,0.));
#86678=DIRECTION('ref_axis',(-1.,0.,0.));
#86679=DIRECTION('',(0.,-1.,0.));
#86680=DIRECTION('center_axis',(0.,1.,0.));
#86681=DIRECTION('ref_axis',(-0.951104406813915,0.,0.308869563633505));
#86682=DIRECTION('',(1.424328388566E-10,-1.,4.385942986573E-10));
#86683=DIRECTION('center_axis',(0.,1.,0.));
#86684=DIRECTION('ref_axis',(-0.92054989510347,0.,-0.390624999999987));
#86685=DIRECTION('',(0.,1.,0.));
#86686=DIRECTION('center_axis',(0.,1.,0.));
#86687=DIRECTION('ref_axis',(1.,0.,0.));
#86688=DIRECTION('',(-6.02495790651922E-7,-0.999999999999037,1.25033281170505E-6));
#86689=DIRECTION('center_axis',(0.,1.,0.));
#86690=DIRECTION('ref_axis',(0.916673510305537,0.,0.399636929605016));
#86691=DIRECTION('',(1.22060867629305E-7,-0.999999999999941,3.20447341735213E-7));
#86692=DIRECTION('center_axis',(-1.,0.,0.));
#86693=DIRECTION('ref_axis',(0.,0.,1.));
#86694=DIRECTION('center_axis',(-1.,0.,0.));
#86695=DIRECTION('ref_axis',(0.,0.,1.));
#86696=DIRECTION('',(1.,0.,0.));
#86697=DIRECTION('center_axis',(1.,0.,0.));
#86698=DIRECTION('ref_axis',(0.,0.,1.));
#86699=DIRECTION('center_axis',(-1.,0.,0.));
#86700=DIRECTION('ref_axis',(0.,0.,1.));
#86701=DIRECTION('center_axis',(1.,0.,0.));
#86702=DIRECTION('ref_axis',(0.,0.,1.));
#86703=DIRECTION('',(1.,0.,0.));
#86704=DIRECTION('center_axis',(-1.,0.,0.));
#86705=DIRECTION('ref_axis',(0.,0.,1.));
#86706=DIRECTION('center_axis',(1.,0.,0.));
#86707=DIRECTION('ref_axis',(0.,0.,1.));
#86708=DIRECTION('center_axis',(1.,0.,6.86169978136685E-18));
#86709=DIRECTION('ref_axis',(6.86169978136685E-18,0.,-1.));
#86710=DIRECTION('',(-0.707106781821139,8.65956055458343E-17,-0.707106780551956));
#86711=DIRECTION('center_axis',(-1.,0.,0.));
#86712=DIRECTION('ref_axis',(0.,0.,1.));
#86713=DIRECTION('center_axis',(1.,0.,0.));
#86714=DIRECTION('ref_axis',(0.,0.,-1.));
#86715=DIRECTION('center_axis',(-1.,0.,0.));
#86716=DIRECTION('ref_axis',(0.,0.,1.));
#86717=DIRECTION('',(1.,0.,0.));
#86718=DIRECTION('center_axis',(-1.,0.,0.));
#86719=DIRECTION('ref_axis',(0.,0.,-1.));
#86720=DIRECTION('center_axis',(-1.,0.,0.));
#86721=DIRECTION('ref_axis',(0.,0.,-1.));
#86722=DIRECTION('center_axis',(-1.,0.,0.));
#86723=DIRECTION('ref_axis',(0.,0.,1.));
#86724=DIRECTION('center_axis',(-1.,0.,-2.79182864590248E-17));
#86725=DIRECTION('ref_axis',(-2.79182864590248E-17,0.,1.));
#86726=DIRECTION('',(-0.500000001036284,-1.0605752379922E-16,-0.86602540318614));
#86727=DIRECTION('center_axis',(-1.,0.,6.88416479379655E-18));
#86728=DIRECTION('ref_axis',(6.88416479379655E-18,0.,1.));
#86729=DIRECTION('',(-0.707106781821139,-8.65956055458343E-17,-0.707106780551956));
#86730=DIRECTION('center_axis',(1.,0.,0.));
#86731=DIRECTION('ref_axis',(0.,0.,1.));
#86732=DIRECTION('center_axis',(1.,0.,0.));
#86733=DIRECTION('ref_axis',(0.,1.,0.));
#86734=DIRECTION('',(0.,0.5,0.866025403784439));
#86735=DIRECTION('',(0.,1.,-1.14462064665688E-15));
#86736=DIRECTION('',(0.,0.5,-0.866025403784439));
#86737=DIRECTION('',(0.,-0.5,-0.866025403784438));
#86738=DIRECTION('',(0.,-1.,3.29078435913854E-15));
#86739=DIRECTION('',(0.,-0.5,0.866025403784439));
#86740=DIRECTION('center_axis',(0.,-0.866025403784439,0.5));
#86741=DIRECTION('ref_axis',(-1.,0.,0.));
#86742=DIRECTION('',(-1.,0.,0.));
#86743=DIRECTION('',(-1.,0.,0.));
#86744=DIRECTION('center_axis',(0.,1.14462064665688E-15,1.));
#86745=DIRECTION('ref_axis',(0.,-1.,1.14462064665688E-15));
#86746=DIRECTION('',(-1.,0.,0.));
#86747=DIRECTION('center_axis',(0.,0.866025403784439,0.5));
#86748=DIRECTION('ref_axis',(1.,0.,0.));
#86749=DIRECTION('',(-1.,0.,0.));
#86750=DIRECTION('center_axis',(0.,0.866025403784438,-0.5));
#86751=DIRECTION('ref_axis',(-1.,0.,0.));
#86752=DIRECTION('',(-1.,0.,0.));
#86753=DIRECTION('center_axis',(0.,-3.29078435913854E-15,-1.));
#86754=DIRECTION('ref_axis',(0.,-1.,3.29078435913854E-15));
#86755=DIRECTION('',(-1.,0.,0.));
#86756=DIRECTION('center_axis',(0.,-0.866025403784439,-0.5));
#86757=DIRECTION('ref_axis',(0.,0.5,-0.866025403784439));
#86758=DIRECTION('center_axis',(1.,0.,0.));
#86759=DIRECTION('ref_axis',(0.,1.,0.));
#86760=DIRECTION('center_axis',(-1.,0.,0.));
#86761=DIRECTION('ref_axis',(0.,0.,1.));
#86762=DIRECTION('center_axis',(-0.173648177666902,6.04454757851474E-16,
-0.984807753012213));
#86763=DIRECTION('ref_axis',(-0.463438942593986,-0.882352941176469,0.0817167894903066));
#86764=DIRECTION('',(-0.173648177666902,2.77440767547504E-8,-0.984807753012213));
#86765=DIRECTION('center_axis',(0.173648177666898,0.,0.984807753012214));
#86766=DIRECTION('ref_axis',(-0.984807753012214,0.,0.173648177666898));
#86767=DIRECTION('',(-0.173648117922493,-3.57010191110886E-9,-0.984807763546762));
#86768=DIRECTION('center_axis',(-0.173648177666903,-9.86864910777917E-16,
-0.984807753012213));
#86769=DIRECTION('ref_axis',(0.463439330841621,0.882352730916633,-0.0817168579488417));
#86770=DIRECTION('center_axis',(-0.397579755272508,0.101323258775101,-0.911956103893519));
#86771=DIRECTION('ref_axis',(-0.392477586383088,-0.917154287992033,0.0692051746962059));
#86772=DIRECTION('center_axis',(0.393372356615379,-0.17691820058078,-0.902196286488767));
#86773=DIRECTION('ref_axis',(-0.916656540587377,-7.20245669423595E-6,-0.3996758518431));
#86774=DIRECTION('center_axis',(-0.173648177666902,0.,-0.984807753012213));
#86775=DIRECTION('ref_axis',(-0.984807753012213,0.,0.173648177666902));
#86776=DIRECTION('center_axis',(0.173648177666902,0.,0.984807753012213));
#86777=DIRECTION('ref_axis',(-0.984807753012213,0.,0.173648177666902));
#86778=DIRECTION('center_axis',(0.868839692726475,-0.434335125464283,0.237635407990666));
#86779=DIRECTION('ref_axis',(0.469231632397537,0.569298297750996,-0.675071198715632));
#86780=DIRECTION('center_axis',(0.,-1.,0.));
#86781=DIRECTION('ref_axis',(0.263820822858805,0.,-0.964571704657618));
#86782=DIRECTION('center_axis',(-0.868840214246772,0.434332901506587,-0.237637566004393));
#86783=DIRECTION('ref_axis',(0.463438490098785,0.882353178018822,-0.081716798365105));
#86784=DIRECTION('center_axis',(-0.984807753012213,0.,0.173648177666902));
#86785=DIRECTION('ref_axis',(0.,1.,0.));
#86786=DIRECTION('',(0.,-1.,0.));
#86787=DIRECTION('',(1.76688803752592E-7,-0.999999999999454,1.02989646555295E-6));
#86788=DIRECTION('center_axis',(-0.984807753012216,-2.97655366217181E-14,
0.173648177666884));
#86789=DIRECTION('ref_axis',(0.171669242031833,-0.150541017827785,0.97358465132293));
#86790=DIRECTION('',(0.173648177666902,0.,0.984807753012213));
#86791=DIRECTION('center_axis',(0.159542862636401,-0.394791526125702,0.904812536319608));
#86792=DIRECTION('ref_axis',(0.116378695458399,-0.902639656840687,-0.414364150406293));
#86793=DIRECTION('center_axis',(0.173648177666902,0.,0.984807753012213));
#86794=DIRECTION('ref_axis',(0.,1.,0.));
#86795=DIRECTION('',(0.173648177666902,0.,0.984807753012213));
#86796=DIRECTION('center_axis',(0.173648177666907,0.,0.984807753012212));
#86797=DIRECTION('ref_axis',(-0.984807753012212,0.,0.173648177666907));
#86798=DIRECTION('center_axis',(-0.173648177666902,0.,-0.984807753012213));
#86799=DIRECTION('ref_axis',(-0.984807753012213,0.,0.173648177666902));
#86800=DIRECTION('center_axis',(-0.173648177666902,0.,-0.984807753012213));
#86801=DIRECTION('ref_axis',(-0.984807753012213,0.,0.173648177666902));
#86802=DIRECTION('',(-0.984807753012213,0.,0.173648177666902));
#86803=DIRECTION('center_axis',(0.984805369615038,-5.94830521183634E-6,
-0.173661693939703));
#86804=DIRECTION('ref_axis',(5.14708112789013E-6,0.999999999973931,-5.06405332903727E-6));
#86805=DIRECTION('center_axis',(0.984807753012213,0.,-0.173648177666902));
#86806=DIRECTION('ref_axis',(-0.173648177666902,0.,-0.984807753012213));
#86807=DIRECTION('',(0.984791886359845,5.81942005172826E-8,-0.173738137896708));
#86808=DIRECTION('center_axis',(0.984807753012213,0.,-0.173648177666902));
#86809=DIRECTION('ref_axis',(0.173648177666902,0.,0.984807753012213));
#86810=DIRECTION('',(0.984807753012213,0.,-0.173648177666902));
#86811=DIRECTION('center_axis',(0.173648177666902,0.,0.984807753012213));
#86812=DIRECTION('ref_axis',(0.984807753012213,0.,-0.173648177666902));
#86813=DIRECTION('',(-0.173648177666902,0.,-0.984807753012213));
#86814=DIRECTION('center_axis',(0.173648177666902,0.,0.984807753012213));
#86815=DIRECTION('ref_axis',(-0.984807753012213,0.,0.173648177666902));
#86816=DIRECTION('center_axis',(0.984807753012213,0.,-0.173648177666902));
#86817=DIRECTION('ref_axis',(0.173648177666902,0.,0.984807753012213));
#86818=DIRECTION('center_axis',(0.984807753016654,-6.51848275878855E-11,
-0.173648177641717));
#86819=DIRECTION('ref_axis',(6.55053788989343E-11,1.,-3.8902214782866E-12));
#86820=DIRECTION('',(0.984807727666866,-1.33909143097295E-7,-0.173648321407394));
#86821=DIRECTION('',(0.984807753012213,0.,-0.173648177666902));
#86822=DIRECTION('center_axis',(0.951179035368867,7.0777324670319E-6,-0.308639664697617));
#86823=DIRECTION('ref_axis',(1.4524932914303E-5,-0.999999999656205,2.18315400864325E-5));
#86824=DIRECTION('center_axis',(0.982743786584323,1.24231498930631E-20,
-0.184972024722405));
#86825=DIRECTION('ref_axis',(0.184972024692575,-1.79592168335814E-5,0.98274378642584));
#86826=DIRECTION('center_axis',(0.810538528342403,0.460364015539678,-0.362066661360467));
#86827=DIRECTION('ref_axis',(-0.407745277886695,-0.000235138511653656,-0.913095686700459));
#86828=DIRECTION('center_axis',(0.,1.,0.));
#86829=DIRECTION('ref_axis',(-0.394380038568694,0.,-0.918947433305385));
#86830=DIRECTION('center_axis',(0.399636929605016,-2.01051104928073E-15,
-0.916673510305537));
#86831=DIRECTION('ref_axis',(-1.61907524424502E-14,1.,-9.25185853854296E-15));
#86832=DIRECTION('center_axis',(0.,1.,0.));
#86833=DIRECTION('ref_axis',(0.407236366022499,0.,0.913322802840698));
#86834=DIRECTION('center_axis',(0.913322802840698,0.,-0.407236366022499));
#86835=DIRECTION('ref_axis',(0.,1.,0.));
#86836=DIRECTION('center_axis',(0.,1.,0.));
#86837=DIRECTION('ref_axis',(0.407236366022499,0.,0.913322802840698));
#86838=DIRECTION('center_axis',(0.,1.,0.));
#86839=DIRECTION('ref_axis',(-0.897582332306211,0.,-0.440846863130206));
#86840=DIRECTION('center_axis',(-0.399636929605016,0.,-0.916673510305537));
#86841=DIRECTION('ref_axis',(0.,1.,0.));
#86842=DIRECTION('center_axis',(0.,1.,0.));
#86843=DIRECTION('ref_axis',(0.916673510305537,0.,0.399636929605016));
#86844=DIRECTION('center_axis',(0.,1.,0.));
#86845=DIRECTION('ref_axis',(-0.922191781452919,0.,0.386732877087908));
#86846=DIRECTION('center_axis',(-0.913322802840698,2.13360716298275E-16,
-0.407236366022499));
#86847=DIRECTION('ref_axis',(-4.10189821923682E-14,1.,9.25185853854296E-14));
#86848=DIRECTION('center_axis',(0.,1.,0.));
#86849=DIRECTION('ref_axis',(0.916673510305537,0.,-0.399636929605016));
#86850=DIRECTION('center_axis',(0.,1.,0.));
#86851=DIRECTION('ref_axis',(0.916673510305537,0.,-0.399636929605016));
#86852=DIRECTION('center_axis',(-0.622024016430491,0.134731225190498,-0.77131940202639));
#86853=DIRECTION('ref_axis',(-0.266840017955903,-0.962591712338371,0.0470489123654965));
#86854=DIRECTION('center_axis',(0.,-1.,0.));
#86855=DIRECTION('ref_axis',(0.738951779496096,0.,-0.67375831540661));
#86856=DIRECTION('',(-6.43993943992487E-5,-0.999999997767879,-1.78033415409196E-5));
#86857=DIRECTION('center_axis',(0.,-1.,0.));
#86858=DIRECTION('ref_axis',(-0.278163242525689,0.,0.960533815389961));
#86859=DIRECTION('center_axis',(0.,1.,0.));
#86860=DIRECTION('ref_axis',(0.263821366478493,0.,-0.964571555971573));
#86861=DIRECTION('center_axis',(-0.998752834435612,0.,0.0499277048023606));
#86862=DIRECTION('ref_axis',(-0.0499277048023606,0.,-0.998752834435612));
#86863=DIRECTION('center_axis',(0.,1.,0.));
#86864=DIRECTION('ref_axis',(0.271911425253992,0.,-0.962322283237972));
#86865=DIRECTION('center_axis',(0.,1.,0.));
#86866=DIRECTION('ref_axis',(1.,0.,0.));
#86867=DIRECTION('center_axis',(0.,1.,0.));
#86868=DIRECTION('ref_axis',(-0.0499277048023506,0.,-0.998752834435612));
#86869=DIRECTION('center_axis',(0.,1.,0.));
#86870=DIRECTION('ref_axis',(-0.92054989510347,0.,-0.390624999999987));
#86871=DIRECTION('center_axis',(0.,-1.,0.));
#86872=DIRECTION('ref_axis',(-0.515104509808459,0.,0.857127379083755));
#86873=DIRECTION('center_axis',(0.308869563633509,0.,0.951104406813913));
#86874=DIRECTION('ref_axis',(-0.951104406813913,0.,0.308869563633509));
#86875=DIRECTION('center_axis',(0.,1.,0.));
#86876=DIRECTION('ref_axis',(-0.951104406813913,0.,0.308869563633509));
#86877=DIRECTION('center_axis',(-0.173648177666902,0.,-0.984807753012213));
#86878=DIRECTION('ref_axis',(-0.984807753012213,0.,0.173648177666902));
#86879=DIRECTION('',(-6.30405482876974E-6,-0.999999999979658,9.7046148712086E-7));
#86880=DIRECTION('center_axis',(0.970634532808316,-0.169018497876731,-0.171176374232767));
#86881=DIRECTION('ref_axis',(0.160171782561879,0.98499010992977,-0.0643388172994282));
#86882=DIRECTION('center_axis',(0.0431678122391723,-0.0175769693413298,
0.998913204505405));
#86883=DIRECTION('ref_axis',(-0.000608192349912218,-0.999845501768985,-0.0175670912330945));
#86884=DIRECTION('center_axis',(0.,1.,0.));
#86885=DIRECTION('ref_axis',(1.,0.,0.));
#86886=DIRECTION('center_axis',(0.,1.,0.));
#86887=DIRECTION('ref_axis',(-0.926972158432388,0.,0.375130134075095));
#86888=DIRECTION('center_axis',(0.,1.,0.));
#86889=DIRECTION('ref_axis',(-0.92054989510347,0.,0.390624999999989));
#86890=DIRECTION('center_axis',(0.,1.,0.));
#86891=DIRECTION('ref_axis',(0.946765333984011,0.,-0.321924528991104));
#86892=DIRECTION('center_axis',(0.390624999999987,0.,0.92054989510347));
#86893=DIRECTION('ref_axis',(-0.92054989510347,0.,0.390624999999987));
#86894=DIRECTION('center_axis',(0.,1.,0.));
#86895=DIRECTION('ref_axis',(-0.92054989510347,0.,0.390624999999988));
#86896=DIRECTION('center_axis',(0.,1.,0.));
#86897=DIRECTION('ref_axis',(1.,0.,0.));
#86898=DIRECTION('',(1.04371427654077E-6,-0.999999999999347,-4.65377558618838E-7));
#86899=DIRECTION('center_axis',(0.,1.,0.));
#86900=DIRECTION('ref_axis',(0.945670538570915,0.,-0.325126486892404));
#86901=DIRECTION('center_axis',(0.,1.,0.));
#86902=DIRECTION('ref_axis',(-0.92054989510347,0.,0.390624999999988));
#86903=DIRECTION('center_axis',(0.390624999999987,-8.10565941154282E-16,
0.92054989510347));
#86904=DIRECTION('ref_axis',(4.56810515340559E-14,1.,-1.85037170770859E-14));
#86905=DIRECTION('center_axis',(0.,1.,0.));
#86906=DIRECTION('ref_axis',(-0.92054989510347,0.,0.390624999999988));
#86907=DIRECTION('center_axis',(0.,1.,0.));
#86908=DIRECTION('ref_axis',(1.,0.,0.));
#86909=DIRECTION('center_axis',(0.,1.,0.));
#86910=DIRECTION('ref_axis',(-0.92054989510347,0.,-0.390624999999987));
#86911=DIRECTION('center_axis',(0.,1.,0.));
#86912=DIRECTION('ref_axis',(0.407236366022499,0.,-0.913322802840698));
#86913=DIRECTION('center_axis',(0.,-1.,0.));
#86914=DIRECTION('ref_axis',(-0.4961343040974,0.,0.868245790256301));
#86915=DIRECTION('center_axis',(-0.390624999999987,0.,0.92054989510347));
#86916=DIRECTION('ref_axis',(0.,1.,0.));
#86917=DIRECTION('center_axis',(0.,1.,0.));
#86918=DIRECTION('ref_axis',(0.407236366022499,0.,-0.913322802840698));
#86919=DIRECTION('center_axis',(0.,1.,0.));
#86920=DIRECTION('ref_axis',(1.,0.,0.));
#86921=DIRECTION('',(-1.53786555571077E-6,0.999999999998582,-6.8571404094823E-7));
#86922=DIRECTION('center_axis',(0.,-1.,0.));
#86923=DIRECTION('ref_axis',(-1.,0.,0.));
#86924=DIRECTION('',(4.22571058986286E-5,0.999999999107167,5.65750982326781E-8));
#86925=DIRECTION('center_axis',(0.,-1.,0.));
#86926=DIRECTION('ref_axis',(-0.467917575539515,0.,0.88377211004943));
#86927=DIRECTION('center_axis',(-0.390624999999987,0.,0.92054989510347));
#86928=DIRECTION('ref_axis',(-0.92054989510347,0.,-0.390624999999987));
#86929=DIRECTION('center_axis',(0.,1.,0.));
#86930=DIRECTION('ref_axis',(-0.0499277048023506,0.,-0.998752834435612));
#86931=DIRECTION('center_axis',(0.,-1.,0.));
#86932=DIRECTION('ref_axis',(0.916639684291378,0.,0.399714509596791));
#86933=DIRECTION('center_axis',(0.,-1.,0.));
#86934=DIRECTION('ref_axis',(-0.515086222159914,0.,0.857138369075278));
#86935=DIRECTION('center_axis',(0.,-1.,0.));
#86936=DIRECTION('ref_axis',(0.91633435450131,0.,0.400413974232504));
#86937=DIRECTION('center_axis',(0.,1.,0.));
#86938=DIRECTION('ref_axis',(1.,0.,0.));
#86939=DIRECTION('',(0.,-1.,0.));
#86940=DIRECTION('center_axis',(0.,-1.,0.));
#86941=DIRECTION('ref_axis',(-1.,0.,0.));
#86942=DIRECTION('center_axis',(0.,1.,0.));
#86943=DIRECTION('ref_axis',(-0.948871785268399,0.,0.3156617416184));
#86944=DIRECTION('center_axis',(0.,-1.,0.));
#86945=DIRECTION('ref_axis',(0.91474129068957,0.,0.404040061265687));
#86946=DIRECTION('center_axis',(0.,1.,0.));
#86947=DIRECTION('ref_axis',(-0.92054989510347,0.,-0.390624999999987));
#86948=DIRECTION('center_axis',(0.,-1.,0.));
#86949=DIRECTION('ref_axis',(-1.,0.,0.));
#86950=DIRECTION('',(0.,1.,0.));
#86951=DIRECTION('center_axis',(0.,-1.,0.));
#86952=DIRECTION('ref_axis',(-1.,0.,0.));
#86953=DIRECTION('center_axis',(-0.224095358856088,0.819067467960532,-0.528119070918561));
#86954=DIRECTION('ref_axis',(0.463977785912221,-0.386881508811817,-0.796898558362032));
#86955=DIRECTION('center_axis',(-0.246837407809856,0.623230767295425,-0.742061119317046));
#86956=DIRECTION('ref_axis',(0.539791218156059,-0.547528396775396,-0.63940448506885));
#86957=DIRECTION('center_axis',(0.246857274377899,-0.623239151827494,-0.742047468640693));
#86958=DIRECTION('ref_axis',(0.948871848468687,1.0093306299581E-7,0.315661551639739));
#86959=DIRECTION('center_axis',(0.000234595565147093,-0.999999938412346,
0.000261036827030693));
#86960=DIRECTION('ref_axis',(0.426145025547988,0.000336119971929968,0.90465479837564));
#86961=DIRECTION('center_axis',(-0.224070766742793,-0.819060243879251,0.528140708890878));
#86962=DIRECTION('ref_axis',(0.463992687595474,0.386903384656539,0.796879261117545));
#86963=DIRECTION('center_axis',(-2.61370721960272E-5,-2.03256955069848E-6,
0.999999999656361));
#86964=DIRECTION('ref_axis',(0.724569107033424,0.689202153739462,2.03389663803666E-5));
#86965=DIRECTION('center_axis',(-0.213402506147939,-0.824296876250407,-0.524398732048048));
#86966=DIRECTION('ref_axis',(8.7042714726054E-6,0.536761814042771,-0.843733817569113));
#86967=DIRECTION('center_axis',(0.213403354295598,-0.824295992344205,0.524399776297312));
#86968=DIRECTION('ref_axis',(-0.463992645966795,0.386850387757512,0.796905014402968));
#86969=DIRECTION('center_axis',(0.166308270996678,-0.675248184444775,0.718596860835149));
#86970=DIRECTION('ref_axis',(1.12997034448066E-5,-0.728744204079672,-0.684786013943481));
#86971=DIRECTION('center_axis',(-0.166317165768798,0.675241121871308,0.718601438702019));
#86972=DIRECTION('ref_axis',(-0.539788588710075,0.547519703716366,-0.639414148686693));
#86973=DIRECTION('center_axis',(-0.213391375091325,0.824299649237854,0.52439890284304));
#86974=DIRECTION('ref_axis',(1.03309119588017E-5,-0.53676035334655,0.843734746806459));
#86975=DIRECTION('center_axis',(0.21337795284944,0.824302204958805,-0.524400347194617));
#86976=DIRECTION('ref_axis',(-4.47031203145252E-5,0.536770362230098,0.843728378231407));
#86977=DIRECTION('center_axis',(-1.,0.,0.));
#86978=DIRECTION('ref_axis',(0.,0.,1.));
#86979=DIRECTION('',(-0.500066124153989,-0.76271838947367,-0.410115264081084));
#86980=DIRECTION('',(-1.,0.,-3.55271367880069E-14));
#86981=DIRECTION('',(-0.500661336716138,0.762431358709554,0.409922735614791));
#86982=DIRECTION('center_axis',(-1.,0.,0.));
#86983=DIRECTION('ref_axis',(0.,0.,1.));
#86984=DIRECTION('center_axis',(1.,0.,0.));
#86985=DIRECTION('ref_axis',(0.,1.,0.));
#86986=DIRECTION('',(0.,0.5,0.866025403784439));
#86987=DIRECTION('',(0.,1.,-1.14462064665688E-15));
#86988=DIRECTION('',(0.,0.5,-0.866025403784439));
#86989=DIRECTION('',(0.,-0.5,-0.866025403784438));
#86990=DIRECTION('',(0.,-1.,3.29078435913854E-15));
#86991=DIRECTION('',(0.,-0.5,0.866025403784439));
#86992=DIRECTION('center_axis',(0.,-0.866025403784439,0.5));
#86993=DIRECTION('ref_axis',(-1.,0.,0.));
#86994=DIRECTION('',(-1.,0.,0.));
#86995=DIRECTION('',(-1.,0.,0.));
#86996=DIRECTION('center_axis',(0.,1.14462064665688E-15,1.));
#86997=DIRECTION('ref_axis',(0.,-1.,1.14462064665688E-15));
#86998=DIRECTION('',(-1.,0.,0.));
#86999=DIRECTION('center_axis',(0.,0.866025403784439,0.5));
#87000=DIRECTION('ref_axis',(1.,0.,0.));
#87001=DIRECTION('',(-1.,0.,0.));
#87002=DIRECTION('center_axis',(0.,0.866025403784438,-0.5));
#87003=DIRECTION('ref_axis',(-1.,0.,0.));
#87004=DIRECTION('',(-1.,0.,0.));
#87005=DIRECTION('center_axis',(0.,-3.29078435913854E-15,-1.));
#87006=DIRECTION('ref_axis',(0.,-1.,3.29078435913854E-15));
#87007=DIRECTION('',(-1.,0.,0.));
#87008=DIRECTION('center_axis',(0.,-0.866025403784439,-0.5));
#87009=DIRECTION('ref_axis',(0.,0.5,-0.866025403784439));
#87010=DIRECTION('center_axis',(1.,0.,0.));
#87011=DIRECTION('ref_axis',(0.,1.,0.));
#87012=DIRECTION('center_axis',(-1.,0.,0.));
#87013=DIRECTION('ref_axis',(0.,0.,1.));
#87014=DIRECTION('center_axis',(0.173648177666902,6.04454757851474E-16,
0.984807753012213));
#87015=DIRECTION('ref_axis',(-0.463438942593986,0.882352941176469,0.0817167894903066));
#87016=DIRECTION('',(0.173648126084303,-1.16611032631002E-8,0.984807762107616));
#87017=DIRECTION('center_axis',(0.173648177666898,0.,0.984807753012214));
#87018=DIRECTION('ref_axis',(-0.984807753012214,0.,0.173648177666898));
#87019=DIRECTION('',(0.173648177666902,2.95597971572804E-8,0.984807753012213));
#87020=DIRECTION('center_axis',(0.173648177666903,-2.0600805012489E-15,
0.984807753012213));
#87021=DIRECTION('ref_axis',(0.4634392991042,-0.882352748104395,-0.0817168523526793));
#87022=DIRECTION('center_axis',(-0.95118330404232,-5.76953425511624E-6,
0.308626509032921));
#87023=DIRECTION('ref_axis',(5.44496996660637E-6,0.999999999355918,3.54755617336676E-5));
#87024=DIRECTION('center_axis',(0.984807753012213,0.,-0.173648177666902));
#87025=DIRECTION('ref_axis',(0.,1.,0.));
#87026=DIRECTION('center_axis',(0.984807753012213,0.,-0.173648177666902));
#87027=DIRECTION('ref_axis',(0.,-1.,0.));
#87028=DIRECTION('',(0.984807768899111,5.32100394428906E-13,-0.173648087567802));
#87029=DIRECTION('center_axis',(0.984807753012207,1.14048525880399E-7,-0.173648177666901));
#87030=DIRECTION('ref_axis',(1.12315871800155E-7,-0.999999999999994,-1.98043226913534E-8));
#87031=DIRECTION('',(0.984807714044911,-4.85499100747805E-8,-0.173648398661302));
#87032=DIRECTION('center_axis',(-0.173648177666902,0.,-0.984807753012213));
#87033=DIRECTION('ref_axis',(0.,-1.,0.));
#87034=DIRECTION('',(-0.173648177666902,0.,-0.984807753012213));
#87035=DIRECTION('center_axis',(0.173648177666907,0.,0.984807753012212));
#87036=DIRECTION('ref_axis',(-0.984807753012212,0.,0.173648177666907));
#87037=DIRECTION('center_axis',(-0.984807753012213,0.,0.173648177666903));
#87038=DIRECTION('ref_axis',(-0.173648177666903,0.,-0.984807753012213));
#87039=DIRECTION('',(-0.984807752772238,-4.00549727818515E-7,0.173648179027407));
#87040=DIRECTION('center_axis',(-0.984807753012213,0.,0.173648177666902));
#87041=DIRECTION('ref_axis',(0.173648177666902,0.,0.984807753012213));
#87042=DIRECTION('',(-0.984807753012213,0.,0.173648177666902));
#87043=DIRECTION('center_axis',(0.159552933030562,0.394801167068611,0.90480655393438));
#87044=DIRECTION('ref_axis',(0.116380632029358,0.902634096597889,-0.414375718578394));
#87045=DIRECTION('center_axis',(0.984807755014784,-3.72227084958571E-8,
-0.173648166309755));
#87046=DIRECTION('ref_axis',(0.173219343573378,0.0702347132572566,0.982375765206817));
#87047=DIRECTION('center_axis',(-0.984807753012213,0.,0.173648177666902));
#87048=DIRECTION('ref_axis',(0.,1.,0.));
#87049=DIRECTION('',(0.,-1.,0.));
#87050=DIRECTION('',(-9.4026263796054E-8,-0.999999999999844,-5.51330525790224E-7));
#87051=DIRECTION('center_axis',(0.868839919953252,0.434334769816394,0.237635227237391));
#87052=DIRECTION('ref_axis',(0.469231347474836,-0.569298881243943,-0.675070904691755));
#87053=DIRECTION('center_axis',(0.,-1.,0.));
#87054=DIRECTION('ref_axis',(0.263820905625295,0.,-0.964571682020081));
#87055=DIRECTION('center_axis',(-0.868839778608605,-0.434333710023902,-0.237637681027702));
#87056=DIRECTION('ref_axis',(0.263821400093756,4.3081659164672E-8,-0.964571546777412));
#87057=DIRECTION('center_axis',(-0.173648177666902,0.,-0.984807753012213));
#87058=DIRECTION('ref_axis',(-0.984807753012213,0.,0.173648177666902));
#87059=DIRECTION('center_axis',(0.173648177666902,0.,0.984807753012213));
#87060=DIRECTION('ref_axis',(-0.984807753012213,0.,0.173648177666902));
#87061=DIRECTION('center_axis',(-0.173648177666902,0.,-0.984807753012213));
#87062=DIRECTION('ref_axis',(-0.984807753012213,0.,0.173648177666902));
#87063=DIRECTION('center_axis',(-0.173648177666902,0.,-0.984807753012213));
#87064=DIRECTION('ref_axis',(-0.984807753012213,0.,0.173648177666902));
#87065=DIRECTION('',(0.984807753012213,0.,-0.173648177666902));
#87066=DIRECTION('center_axis',(0.173648177666902,0.,0.984807753012213));
#87067=DIRECTION('ref_axis',(0.984807753012213,0.,-0.173648177666902));
#87068=DIRECTION('center_axis',(0.173648177666902,0.,0.984807753012213));
#87069=DIRECTION('ref_axis',(-0.984807753012213,0.,0.173648177666902));
#87070=DIRECTION('',(0.173648177666902,0.,0.984807753012213));
#87071=DIRECTION('center_axis',(-0.393409542444277,-0.176889802087537,0.90218564044836));
#87072=DIRECTION('ref_axis',(-0.916641374847507,1.2837746409996E-5,-0.39971063252416));
#87073=DIRECTION('center_axis',(0.39758819974252,0.101304962457168,0.911954455006967));
#87074=DIRECTION('ref_axis',(-0.916670483337923,3.52527253137775E-6,0.399643872672397));
#87075=DIRECTION('center_axis',(-0.810495180234583,0.460325137160707,0.362213101522415));
#87076=DIRECTION('ref_axis',(-0.407809813917888,0.000427669905792924,-0.913066795349995));
#87077=DIRECTION('center_axis',(-0.982739063229984,0.,0.184997117820396));
#87078=DIRECTION('ref_axis',(0.184997117820396,0.,0.982739063229984));
#87079=DIRECTION('center_axis',(0.970623774538595,0.169109840258299,-0.171147159568199));
#87080=DIRECTION('ref_axis',(0.160257422681418,-0.984973277091295,-0.0643832423192878));
#87081=DIRECTION('center_axis',(-0.173654718138959,-9.74544300691725E-6,
-0.984806599679909));
#87082=DIRECTION('ref_axis',(8.88767218123285E-5,0.999999995723609,-2.55677663475359E-5));
#87083=DIRECTION('center_axis',(-0.0432132455015585,-0.0171107728542251,
-0.99891933451383));
#87084=DIRECTION('ref_axis',(-0.000613241581050437,0.999853592022779,-0.0171002471885266));
#87085=DIRECTION('center_axis',(0.,-1.,0.));
#87086=DIRECTION('ref_axis',(0.,0.,-1.));
#87087=DIRECTION('center_axis',(0.,-1.,0.));
#87088=DIRECTION('ref_axis',(0.184998949610495,0.,0.982738718400274));
#87089=DIRECTION('center_axis',(0.,-1.,0.));
#87090=DIRECTION('ref_axis',(-0.92054989510347,0.,0.390624999999987));
#87091=DIRECTION('center_axis',(-0.173648177666902,0.,-0.984807753012213));
#87092=DIRECTION('ref_axis',(-0.984807753012213,0.,0.173648177666902));
#87093=DIRECTION('',(3.02443292467696E-8,-0.999999999999985,1.68898496137498E-7));
#87094=DIRECTION('center_axis',(0.,1.,0.));
#87095=DIRECTION('ref_axis',(-0.515104509808457,0.,0.857127379083756));
#87096=DIRECTION('center_axis',(-0.308869563633509,0.,-0.951104406813913));
#87097=DIRECTION('ref_axis',(-0.951104406813913,0.,0.308869563633509));
#87098=DIRECTION('center_axis',(0.,-1.,0.));
#87099=DIRECTION('ref_axis',(0.173648177666902,0.,0.984807753012213));
#87100=DIRECTION('center_axis',(0.,-1.,0.));
#87101=DIRECTION('ref_axis',(0.,0.,-1.));
#87102=DIRECTION('center_axis',(0.,-1.,0.));
#87103=DIRECTION('ref_axis',(-0.951104406813915,0.,0.308869563633505));
#87104=DIRECTION('center_axis',(0.,-1.,0.));
#87105=DIRECTION('ref_axis',(-0.92054989510347,0.,-0.390624999999987));
#87106=DIRECTION('center_axis',(0.,-1.,0.));
#87107=DIRECTION('ref_axis',(-0.0499277048023606,0.,-0.998752834435612));
#87108=DIRECTION('center_axis',(0.,-1.,0.));
#87109=DIRECTION('ref_axis',(0.0559121723748785,0.,0.998435690958773));
#87110=DIRECTION('center_axis',(0.998752834435612,0.,-0.0499277048023606));
#87111=DIRECTION('ref_axis',(-0.0499277048023606,0.,-0.998752834435612));
#87112=DIRECTION('center_axis',(0.,-1.,0.));
#87113=DIRECTION('ref_axis',(-0.0499277048023606,0.,-0.998752834435612));
#87114=DIRECTION('center_axis',(0.,-1.,0.));
#87115=DIRECTION('ref_axis',(0.738977760494908,0.,-0.673729819359312));
#87116=DIRECTION('',(4.15986094482921E-5,-0.999999999067449,1.16041817154406E-5));
#87117=DIRECTION('center_axis',(0.622026863566978,0.134727224711234,0.771317804748883));
#87118=DIRECTION('ref_axis',(-0.778414735295653,-1.07091660949363E-6,0.627750348365854));
#87119=DIRECTION('center_axis',(0.,1.,0.));
#87120=DIRECTION('ref_axis',(-0.38894989240481,0.,0.921258911055023));
#87121=DIRECTION('center_axis',(0.399636929605016,3.72066793566512E-15,
0.916673510305537));
#87122=DIRECTION('ref_axis',(-5.43546689139399E-14,-1.,2.77555756156289E-14));
#87123=DIRECTION('center_axis',(0.,-1.,0.));
#87124=DIRECTION('ref_axis',(0.407236366022499,0.,-0.913322802840698));
#87125=DIRECTION('center_axis',(0.913322802840698,0.,0.407236366022499));
#87126=DIRECTION('ref_axis',(0.,-1.,0.));
#87127=DIRECTION('center_axis',(0.,-1.,0.));
#87128=DIRECTION('ref_axis',(0.407236366022499,0.,-0.913322802840698));
#87129=DIRECTION('center_axis',(0.,1.,0.));
#87130=DIRECTION('ref_axis',(-0.888996404394544,0.,0.457914176427824));
#87131=DIRECTION('center_axis',(-0.399636929605016,0.,0.916673510305537));
#87132=DIRECTION('ref_axis',(0.,-1.,0.));
#87133=DIRECTION('center_axis',(0.,-1.,0.));
#87134=DIRECTION('ref_axis',(0.916673510305537,0.,-0.399636929605016));
#87135=DIRECTION('center_axis',(0.,1.,0.));
#87136=DIRECTION('ref_axis',(-0.924457470735394,0.,-0.381285175166198));
#87137=DIRECTION('center_axis',(-0.913322802840698,7.76865850722253E-16,
0.407236366022499));
#87138=DIRECTION('ref_axis',(-4.21031843648538E-14,-1.,-9.25185853854296E-14));
#87139=DIRECTION('center_axis',(0.,-1.,0.));
#87140=DIRECTION('ref_axis',(0.916673510305537,0.,0.399636929605016));
#87141=DIRECTION('center_axis',(0.,-1.,0.));
#87142=DIRECTION('ref_axis',(0.916673510305537,0.,0.399636929605016));
#87143=DIRECTION('center_axis',(0.,1.,0.));
#87144=DIRECTION('ref_axis',(1.,0.,0.));
#87145=DIRECTION('',(-1.08852304226319E-6,-0.99999999999929,4.85357233595664E-7));
#87146=DIRECTION('center_axis',(0.,1.,0.));
#87147=DIRECTION('ref_axis',(-0.467905576874307,0.,-0.883778462698612));
#87148=DIRECTION('center_axis',(-0.390624999999987,0.,-0.92054989510347));
#87149=DIRECTION('ref_axis',(-0.92054989510347,0.,0.390624999999987));
#87150=DIRECTION('center_axis',(0.,-1.,0.));
#87151=DIRECTION('ref_axis',(0.184972798800006,0.,0.98274364088713));
#87152=DIRECTION('center_axis',(0.,-1.,0.));
#87153=DIRECTION('ref_axis',(0.915933776184509,0.,-0.401329437799404));
#87154=DIRECTION('center_axis',(0.,-1.,0.));
#87155=DIRECTION('ref_axis',(-0.515104509731028,0.,0.857127379130289));
#87156=DIRECTION('center_axis',(0.,-1.,0.));
#87157=DIRECTION('ref_axis',(0.931383237830313,0.,-0.364040195979405));
#87158=DIRECTION('center_axis',(0.390624999999987,0.,-0.92054989510347));
#87159=DIRECTION('ref_axis',(-0.92054989510347,0.,-0.390624999999987));
#87160=DIRECTION('center_axis',(0.,-1.,0.));
#87161=DIRECTION('ref_axis',(0.946765333984011,0.,0.321924528991104));
#87162=DIRECTION('center_axis',(0.,-1.,0.));
#87163=DIRECTION('ref_axis',(-0.92054989510347,0.,-0.390624999999988));
#87164=DIRECTION('center_axis',(0.,-1.,0.));
#87165=DIRECTION('ref_axis',(-1.,0.,0.));
#87166=DIRECTION('',(3.339300040861E-5,0.999999999434799,-3.912721493535E-6));
#87167=DIRECTION('center_axis',(0.,1.,0.));
#87168=DIRECTION('ref_axis',(1.,0.,0.));
#87169=DIRECTION('',(-1.5281607930716E-6,-0.9999999999986,-6.81386790616307E-7));
#87170=DIRECTION('center_axis',(0.,-1.,0.));
#87171=DIRECTION('ref_axis',(0.945670538570914,0.,0.325126486892405));
#87172=DIRECTION('center_axis',(0.,-1.,0.));
#87173=DIRECTION('ref_axis',(-0.92054989510347,0.,-0.390624999999988));
#87174=DIRECTION('center_axis',(0.390624999999987,5.84690488553155E-16,
-0.92054989510347));
#87175=DIRECTION('ref_axis',(4.5102810375397E-14,-1.,1.85037170770859E-14));
#87176=DIRECTION('center_axis',(0.,-1.,0.));
#87177=DIRECTION('ref_axis',(-0.92054989510347,0.,-0.390624999999988));
#87178=DIRECTION('center_axis',(0.,1.,0.));
#87179=DIRECTION('ref_axis',(1.,0.,0.));
#87180=DIRECTION('center_axis',(0.,-1.,0.));
#87181=DIRECTION('ref_axis',(-0.92054989510347,0.,0.390624999999988));
#87182=DIRECTION('center_axis',(0.,-1.,0.));
#87183=DIRECTION('ref_axis',(0.407236366022499,0.,0.913322802840698));
#87184=DIRECTION('center_axis',(0.,1.,0.));
#87185=DIRECTION('ref_axis',(-0.496122516224214,0.,-0.868252525994226));
#87186=DIRECTION('center_axis',(-0.390624999999987,0.,-0.92054989510347));
#87187=DIRECTION('ref_axis',(0.,-1.,0.));
#87188=DIRECTION('center_axis',(0.,-1.,0.));
#87189=DIRECTION('ref_axis',(0.4072363660225,0.,0.913322802840698));
#87190=DIRECTION('center_axis',(0.,1.,0.));
#87191=DIRECTION('ref_axis',(1.,0.,0.));
#87192=DIRECTION('',(0.,-1.,0.));
#87193=DIRECTION('center_axis',(0.,-1.,0.));
#87194=DIRECTION('ref_axis',(-1.,0.,0.));
#87195=DIRECTION('',(0.,1.,0.));
#87196=DIRECTION('center_axis',(0.,-1.,0.));
#87197=DIRECTION('ref_axis',(-1.,0.,0.));
#87198=DIRECTION('center_axis',(0.,-1.,0.));
#87199=DIRECTION('ref_axis',(-0.948871785268399,0.,-0.3156617416184));
#87200=DIRECTION('center_axis',(0.,-1.,0.));
#87201=DIRECTION('ref_axis',(0.916481355130724,0.,-0.400077399633811));
#87202=DIRECTION('center_axis',(0.,-1.,0.));
#87203=DIRECTION('ref_axis',(-0.92054989510347,0.,0.390624999999987));
#87204=DIRECTION('center_axis',(0.,-1.,0.));
#87205=DIRECTION('ref_axis',(-1.,0.,0.));
#87206=DIRECTION('center_axis',(-0.224058386535214,0.819056424696978,-0.528151884012393));
#87207=DIRECTION('ref_axis',(0.464012190567123,-0.386908739989834,-0.796865304756443));
#87208=DIRECTION('center_axis',(0.000234595565451377,-0.999999938412346,
0.000261036827419178));
#87209=DIRECTION('ref_axis',(0.426145025549655,0.000336119972411781,0.904654798374854));
#87210=DIRECTION('center_axis',(-0.224095509272251,-0.819067663979687,0.528118703083757));
#87211=DIRECTION('ref_axis',(0.463970536020739,0.386884684319262,0.796901237760247));
#87212=DIRECTION('center_axis',(-0.246850867614741,-0.623236588607253,0.742051752763272));
#87213=DIRECTION('ref_axis',(0.539787633059408,0.547517821159986,0.639416567433424));
#87214=DIRECTION('center_axis',(0.0015456208083213,0.00171768113197915,
0.999997330310359));
#87215=DIRECTION('ref_axis',(0.550747471894769,0.834668797317559,-0.00228494769739675));
#87216=DIRECTION('center_axis',(0.246871071069859,0.623239366842138,0.742042698156266));
#87217=DIRECTION('ref_axis',(0.539806900209745,0.547489979087855,-0.639424141931102));
#87218=DIRECTION('center_axis',(-0.213357641816103,-0.824307171415416,-0.524400804568212));
#87219=DIRECTION('ref_axis',(-0.463983424918666,-0.386871231470338,0.796900264563495));
#87220=DIRECTION('center_axis',(0.213374617987456,-0.82430473740624,0.524397723382107));
#87221=DIRECTION('ref_axis',(-1.00295012044401E-5,-0.536760887317295,-0.843734407112664));
#87222=DIRECTION('center_axis',(-0.213391699957863,0.824299991802442,0.524398232170541));
#87223=DIRECTION('ref_axis',(1.69583914793472E-5,-0.536758484410448,0.843735935661041));
#87224=DIRECTION('center_axis',(0.213360527418366,0.824307096359649,-0.52439974850383));
#87225=DIRECTION('ref_axis',(-2.00487952037749E-5,0.53676311541999,0.843732989471594));
#87226=DIRECTION('center_axis',(0.1663438053302,0.675238304245454,-0.718597920194591));
#87227=DIRECTION('ref_axis',(8.19782755311054E-6,0.728750066126856,0.68477977558694));
#87228=DIRECTION('center_axis',(-1.,0.,0.));
#87229=DIRECTION('ref_axis',(0.,0.,1.));
#87230=DIRECTION('',(-0.500066124153987,0.762718389473674,-0.410115264081081));
#87231=DIRECTION('',(-0.500660779556073,-0.762417033624258,0.409950058731417));
#87232=DIRECTION('',(-1.,0.,-3.55271367880069E-14));
#87233=DIRECTION('center_axis',(1.,0.,0.));
#87234=DIRECTION('ref_axis',(0.,1.,0.));
#87235=DIRECTION('',(0.532111185932234,-0.738603577927986,0.413911150463199));
#87236=DIRECTION('',(-0.358455003852291,0.738603577927671,0.570941997829637));
#87237=DIRECTION('center_axis',(-0.839921904894139,-0.522108531837321,0.148100893520862));
#87238=DIRECTION('ref_axis',(-0.527930412690934,0.849287630521003,-5.13852122356239E-18));
#87239=DIRECTION('center_axis',(0.173648177666903,0.,0.984807753012213));
#87240=DIRECTION('ref_axis',(0.,-1.,0.));
#87241=DIRECTION('center_axis',(-0.173648177666902,0.,-0.984807753012213));
#87242=DIRECTION('ref_axis',(-0.984807753012213,0.,0.173648177666902));
#87243=DIRECTION('center_axis',(0.,1.,0.));
#87244=DIRECTION('ref_axis',(1.,0.,0.));
#87245=DIRECTION('',(-0.984807753012213,0.,0.173648177666902));
#87246=DIRECTION('',(-0.173648177666902,0.,-0.984807753012213));
#87247=DIRECTION('',(-0.984807753012213,0.,0.173648177666902));
#87248=DIRECTION('',(-0.173651710791594,1.14934020021696E-8,-0.984807130020469));
#87249=DIRECTION('center_axis',(0.,-1.,0.));
#87250=DIRECTION('ref_axis',(-0.984807753012213,0.,0.173648177666903));
#87251=DIRECTION('center_axis',(0.,-1.,0.));
#87252=DIRECTION('ref_axis',(-0.0499277048023606,0.,-0.998752834435612));
#87253=DIRECTION('center_axis',(0.,-1.,0.));
#87254=DIRECTION('ref_axis',(-0.92054989510347,0.,-0.390624999999987));
#87255=DIRECTION('center_axis',(0.,-1.,0.));
#87256=DIRECTION('ref_axis',(-0.951104406813915,0.,0.308869563633505));
#87257=DIRECTION('center_axis',(0.,-1.,0.));
#87258=DIRECTION('ref_axis',(0.173648177666904,0.,0.984807753012213));
#87259=DIRECTION('center_axis',(0.,-1.,0.));
#87260=DIRECTION('ref_axis',(0.,0.,-1.));
#87261=DIRECTION('',(0.984807753012213,0.,-0.173648177666902));
#87262=DIRECTION('',(0.173648177666902,0.,0.984807753012213));
#87263=DIRECTION('',(0.984807753012213,0.,-0.173648177666902));
#87264=DIRECTION('center_axis',(0.,1.,0.));
#87265=DIRECTION('ref_axis',(-0.951104406813942,0.,0.30886956363342));
#87266=DIRECTION('center_axis',(0.,1.,0.));
#87267=DIRECTION('ref_axis',(-0.92054989510347,0.,-0.390624999999987));
#87268=DIRECTION('center_axis',(0.,1.,0.));
#87269=DIRECTION('ref_axis',(-0.0499277048023606,0.,-0.998752834435612));
#87270=DIRECTION('center_axis',(0.,1.,0.));
#87271=DIRECTION('ref_axis',(0.3114756963496,0.,-0.9502541189511));
#87272=DIRECTION('center_axis',(0.,1.,0.));
#87273=DIRECTION('ref_axis',(-0.874458269240608,0.,-0.485100747635705));
#87274=DIRECTION('',(0.173722816438492,-3.55490858096083E-8,0.984794589266552));
#87275=DIRECTION('center_axis',(-0.173648177666902,0.,-0.984807753012213));
#87276=DIRECTION('ref_axis',(-0.984807753012213,0.,0.173648177666902));
#87277=DIRECTION('',(0.98480779821852,2.86780361313506E-5,-0.173647918920904));
#87278=DIRECTION('',(-2.619623158332E-9,1.,-1.484149674398E-8));
#87279=DIRECTION('center_axis',(-0.173738860884696,-3.29476084001257E-5,
-0.984791758258031));
#87280=DIRECTION('ref_axis',(0.227733791624276,0.972892847856778,-0.0402097841520986));
#87281=DIRECTION('center_axis',(-0.173648177666902,0.,-0.984807753012213));
#87282=DIRECTION('ref_axis',(-0.984807753012213,0.,0.173648177666902));
#87283=DIRECTION('',(-2.619623158332E-9,1.,-1.484149674398E-8));
#87284=DIRECTION('',(-0.984808118285514,2.85919679452004E-5,0.173646103732403));
#87285=DIRECTION('center_axis',(-0.173798222257865,3.70611714430505E-5,
-0.984781283619097));
#87286=DIRECTION('ref_axis',(-0.226415421385525,0.973209345122142,0.0399953438008206));
#87287=DIRECTION('center_axis',(0.984807753012213,0.,-0.173648177666903));
#87288=DIRECTION('ref_axis',(0.13914925430432,-0.598224410459968,0.789154636149579));
#87289=DIRECTION('center_axis',(0.984701214027571,0.00034783784991401,-0.174250962985741));
#87290=DIRECTION('ref_axis',(0.147000879085088,-0.538606975966355,0.829634417673586));
#87291=DIRECTION('center_axis',(0.984796609140205,0.000132133476650577,
-0.173711315597746));
#87292=DIRECTION('ref_axis',(0.0494872421690545,-0.95877571584193,0.279821620991475));
#87293=DIRECTION('',(0.98480819903795,7.61270752104513E-7,-0.173645648108583));
#87294=DIRECTION('center_axis',(0.984804385279843,1.83453921068791E-5,-0.173667274974411));
#87295=DIRECTION('ref_axis',(0.0493756213064273,-0.958761501507835,0.279890034204587));
#87296=DIRECTION('center_axis',(0.984807753012213,0.,-0.173648177666902));
#87297=DIRECTION('ref_axis',(0.,-1.,0.));
#87298=DIRECTION('',(0.,1.,0.));
#87299=DIRECTION('',(-0.173647957746888,-0.00166011264183791,-0.984806392544419));
#87300=DIRECTION('',(-5.36954384231574E-8,0.999999999999952,-3.04520965216585E-7));
#87301=DIRECTION('',(-0.173648177666902,0.,-0.984807753012213));
#87302=DIRECTION('center_axis',(-0.984807753012213,1.47875699429781E-16,
0.173648177666902));
#87303=DIRECTION('ref_axis',(0.118437015122884,0.731304063260744,0.671689690636314));
#87304=DIRECTION('center_axis',(-0.984807753012213,1.10906774572336E-17,
0.173648177666902));
#87305=DIRECTION('ref_axis',(0.173046420789886,0.0831790275611967,0.981395020175762));
#87306=DIRECTION('',(0.984807866755134,-7.84910877958438E-6,-0.173647532420113));
#87307=DIRECTION('center_axis',(0.984807753012213,-5.91502797719126E-17,
-0.173648177666902));
#87308=DIRECTION('ref_axis',(0.0712749837854421,0.911880281676684,0.404220519735993));
#87309=DIRECTION('',(-0.984807701359279,7.21578091369084E-7,0.173648470603496));
#87310=DIRECTION('center_axis',(-0.984807753012213,-2.95751398859563E-17,
0.173648177666903));
#87311=DIRECTION('ref_axis',(0.118437565749294,-0.731301105875289,0.671692813393862));
#87312=DIRECTION('center_axis',(0.984807753012213,2.66176258973607E-16,
-0.173648177666903));
#87313=DIRECTION('ref_axis',(0.119975660912596,-0.722938587260738,0.680415784530337));
#87314=DIRECTION('',(0.984807662516202,-6.24263663490926E-6,-0.173648690782289));
#87315=DIRECTION('center_axis',(-0.984807753012213,2.95751398859563E-16,
0.173648177666902));
#87316=DIRECTION('ref_axis',(0.0174472473523288,-0.994939614274932,0.0989482567116538));
#87317=DIRECTION('center_axis',(-0.984807753012213,-1.51942396384287E-16,
0.173648177666902));
#87318=DIRECTION('ref_axis',(-0.0915532115266896,-0.849720177918111,-0.519224064059017));
#87319=DIRECTION('',(-0.984807753012213,0.,0.173648177666902));
#87320=DIRECTION('center_axis',(-0.984807753012213,-3.08475197493174E-16,
0.173648177666902));
#87321=DIRECTION('ref_axis',(-0.148632496508293,-0.517074437493711,-0.84293677525202));
#87322=DIRECTION('',(0.984807705057875,5.76825355638144E-7,-0.173648449628293));
#87323=DIRECTION('center_axis',(-0.984807753012213,-2.93785902374558E-17,
0.173648177666902));
#87324=DIRECTION('ref_axis',(-0.091553228988867,0.84972011552227,-0.519224163091946));
#87325=DIRECTION('',(0.984807701171163,-6.23576923384803E-7,-0.173648471670733));
#87326=DIRECTION('center_axis',(-0.984807753012213,2.20339426780919E-16,
0.173648177666902));
#87327=DIRECTION('ref_axis',(-0.0751084169313667,0.901618518365397,-0.4259609994432));
#87328=DIRECTION('',(0.984807753012213,0.,-0.173648177666902));
#87329=DIRECTION('center_axis',(-4.5541240007271E-5,0.999999998908222,1.04666705814102E-5));
#87330=DIRECTION('ref_axis',(-0.729107486866968,-4.0367840113073E-5,0.684399204386571));
#87331=DIRECTION('center_axis',(-0.984807753012213,0.,0.173648177666902));
#87332=DIRECTION('ref_axis',(0.122787513031607,-0.707108456623977,0.696362590332343));
#87333=DIRECTION('center_axis',(-0.984807753012213,0.,0.173648177666902));
#87334=DIRECTION('ref_axis',(0.,-1.,0.));
#87335=DIRECTION('',(-0.984807753012213,0.,0.173648177666902));
#87336=DIRECTION('center_axis',(0.984807753012213,0.,-0.173648177666902));
#87337=DIRECTION('ref_axis',(0.122787512666764,0.707108458725017,0.696362588263213));
#87338=DIRECTION('',(0.984807753012213,0.,-0.173648177666902));
#87339=DIRECTION('center_axis',(0.984807753012213,0.,-0.173648177666902));
#87340=DIRECTION('ref_axis',(0.,1.,0.));
#87341=DIRECTION('center_axis',(-0.468047248986744,0.720808604941997,0.511240381579461));
#87342=DIRECTION('ref_axis',(0.149821931102216,-0.505420385471279,0.849766805018216));
#87343=DIRECTION('center_axis',(-0.984807752980486,8.02724707364289E-6,
0.173648177661298));
#87344=DIRECTION('ref_axis',(0.173648177647197,-2.42677927780413E-6,0.984807753012698));
#87345=DIRECTION('center_axis',(-0.984807753012213,0.,0.173648177666903));
#87346=DIRECTION('ref_axis',(0.1391482160283,0.598232419576064,0.789148747793665));
#87347=DIRECTION('center_axis',(0.,1.,0.));
#87348=DIRECTION('ref_axis',(-0.984807753012214,0.,0.173648177666898));
#87349=DIRECTION('center_axis',(5.99767279256134E-6,0.999999998756089,-4.95161662595558E-5));
#87350=DIRECTION('ref_axis',(-0.173665667877379,-4.77221618665076E-5,-0.984804667699793));
#87351=DIRECTION('',(3.128857622442E-9,1.,-1.424668953682E-8));
#87352=DIRECTION('center_axis',(0.325178856357606,0.402282522364151,0.85581977283672));
#87353=DIRECTION('ref_axis',(0.0712965070296305,-0.912858053252779,0.402003709804923));
#87354=DIRECTION('center_axis',(0.00953570295887386,-0.900814846469353,
0.434098701621504));
#87355=DIRECTION('ref_axis',(-0.495353769654611,-0.381364780402071,-0.780503393431346));
#87356=DIRECTION('center_axis',(0.540815948209504,0.356362088464686,0.76192136869059));
#87357=DIRECTION('ref_axis',(-0.235026539236875,-0.805720097908675,0.543670534129239));
#87358=DIRECTION('center_axis',(0.540853504125162,0.356471320596299,0.761843609061508));
#87359=DIRECTION('ref_axis',(0.0676210056074329,-0.921248442444026,0.383051833170259));
#87360=DIRECTION('center_axis',(-0.0822813569473299,-0.880495422945283,
-0.466859281230773));
#87361=DIRECTION('ref_axis',(0.988016782566545,-0.0106874206885076,-0.153976025425647));
#87362=DIRECTION('center_axis',(0.984806655704334,5.35809355578126E-6,-0.173654400611492));
#87363=DIRECTION('ref_axis',(0.140766524539594,0.585557533745896,0.798315201059373));
#87364=DIRECTION('center_axis',(-0.118543194053381,-0.732033583437037,-0.670875803605968));
#87365=DIRECTION('ref_axis',(0.979768502675954,-0.195953546642656,0.0406926126254334));
#87366=DIRECTION('center_axis',(-0.118296406893678,-0.732058422007768,-0.670892261755598));
#87367=DIRECTION('ref_axis',(-0.992860141709842,0.0767780069429456,0.0912900687576806));
#87368=DIRECTION('center_axis',(-0.0825005446561861,0.87918155882871,-0.46929036506938));
#87369=DIRECTION('ref_axis',(0.988854899622876,0.0136564674857691,-0.148254808986559));
#87370=DIRECTION('center_axis',(-0.984807753012326,-4.76834328723365E-13,
0.173648177666263));
#87371=DIRECTION('ref_axis',(0.119869363396271,-0.723523116755521,0.679812941359128));
#87372=DIRECTION('center_axis',(-0.118924556957068,0.728675399195287,-0.674454677765789));
#87373=DIRECTION('ref_axis',(-0.984804485455633,1.76838323664053E-5,0.173666706981354));
#87374=DIRECTION('center_axis',(-0.984806653083073,5.45304870040947E-6,
0.173654415473897));
#87375=DIRECTION('ref_axis',(0.14033160238962,-0.589008723332889,0.79584908444285));
#87376=DIRECTION('center_axis',(-0.119158532281579,0.728650964800672,-0.674439779134912));
#87377=DIRECTION('ref_axis',(0.977813440898981,0.203990901934536,0.0476296832367139));
#87378=DIRECTION('center_axis',(-0.172166082870035,0.000366553130519414,
-0.985067868498405));
#87379=DIRECTION('ref_axis',(-0.985067935878727,-2.329605698763E-5,0.172166085977808));
#87380=DIRECTION('center_axis',(0.,-1.,0.));
#87381=DIRECTION('ref_axis',(0.934249900475282,0.,-0.356619017246593));
#87382=DIRECTION('center_axis',(0.390624999999987,-2.7899036639383E-15,
-0.92054989510347));
#87383=DIRECTION('ref_axis',(1.89084858881472E-13,-1.,8.32667268468867E-14));
#87384=DIRECTION('center_axis',(-0.308869563633505,0.,-0.951104406813915));
#87385=DIRECTION('ref_axis',(0.,-1.,0.));
#87386=DIRECTION('center_axis',(0.,-1.,0.));
#87387=DIRECTION('ref_axis',(0.0556368722626882,0.,0.998451069629767));
#87388=DIRECTION('center_axis',(0.,-1.,0.));
#87389=DIRECTION('ref_axis',(-0.0499277048023606,0.,-0.998752834435612));
#87390=DIRECTION('center_axis',(0.998752834435612,-1.73393901318555E-16,
-0.0499277048023606));
#87391=DIRECTION('ref_axis',(-8.67361737988402E-16,-1.,-1.38777878078145E-14));
#87392=DIRECTION('center_axis',(0.,-1.,0.));
#87393=DIRECTION('ref_axis',(0.945670538570914,0.,0.325126486892406));
#87394=DIRECTION('center_axis',(0.,-1.,0.));
#87395=DIRECTION('ref_axis',(-0.92054989510347,0.,-0.390624999999988));
#87396=DIRECTION('center_axis',(0.,-1.,0.));
#87397=DIRECTION('ref_axis',(-1.,0.,0.));
#87398=DIRECTION('',(-2.877698079828E-14,1.,0.));
#87399=DIRECTION('center_axis',(0.,1.,0.));
#87400=DIRECTION('ref_axis',(-0.0499277048023506,0.,-0.998752834435612));
#87401=DIRECTION('center_axis',(0.,-1.,0.));
#87402=DIRECTION('ref_axis',(-0.496134304097401,0.,0.868245790256301));
#87403=DIRECTION('center_axis',(-0.390624999999987,1.64421355075197E-15,
0.92054989510347));
#87404=DIRECTION('ref_axis',(-1.21430643318377E-14,1.,-6.93889390390721E-15));
#87405=DIRECTION('center_axis',(-0.998752834435612,-8.63521945113378E-17,
0.0499277048023606));
#87406=DIRECTION('ref_axis',(1.30104260698261E-15,1.,2.77555756156289E-14));
#87407=DIRECTION('center_axis',(-0.173648177666902,0.,-0.984807753012213));
#87408=DIRECTION('ref_axis',(-0.984807753012213,0.,0.173648177666902));
#87409=DIRECTION('center_axis',(0.173648177666902,0.,0.984807753012213));
#87410=DIRECTION('ref_axis',(-0.984807753012213,0.,0.173648177666902));
#87411=DIRECTION('',(1.450155551197E-11,-1.,-2.556888034633E-12));
#87412=DIRECTION('center_axis',(0.984807753012213,0.,-0.173648177666902));
#87413=DIRECTION('ref_axis',(0.,-1.,0.));
#87414=DIRECTION('',(0.,1.,0.));
#87415=DIRECTION('',(0.173648177666902,0.,0.984807753012213));
#87416=DIRECTION('',(6.51332343039219E-8,0.99999999999993,3.69388507198911E-7));
#87417=DIRECTION('',(0.173648177370708,-5.92206446015928E-5,0.984807751283846));
#87418=DIRECTION('center_axis',(0.173648177666902,0.,0.984807753012213));
#87419=DIRECTION('ref_axis',(0.,1.,0.));
#87420=DIRECTION('center_axis',(0.173648177666898,0.,0.984807753012214));
#87421=DIRECTION('ref_axis',(-0.984807753012214,0.,0.173648177666898));
#87422=DIRECTION('center_axis',(0.173648177666902,0.,0.984807753012213));
#87423=DIRECTION('ref_axis',(0.,-1.,0.));
#87424=DIRECTION('center_axis',(0.0705615471450538,-0.994935989107725,0.0715782483910466));
#87425=DIRECTION('ref_axis',(-0.173073282542036,-0.0828800320757138,-0.981415579228928));
#87426=DIRECTION('center_axis',(-0.984807753012213,-3.59689602365803E-17,
0.173648177666902));
#87427=DIRECTION('ref_axis',(0.00203933837147199,-0.999931035895442,0.0115656626301812));
#87428=DIRECTION('center_axis',(0.984807753012213,-5.43782705938852E-17,
-0.173648177666902));
#87429=DIRECTION('ref_axis',(0.0865532966445691,0.866923871076506,0.490868137688406));
#87430=DIRECTION('center_axis',(-0.984807753012213,1.47875699429781E-16,
0.173648177666902));
#87431=DIRECTION('ref_axis',(-0.0023628809126313,-0.999907416559164,-0.013400563561729));
#87432=DIRECTION('center_axis',(0.984807753012213,-5.91502797719126E-17,
-0.173648177666902));
#87433=DIRECTION('ref_axis',(0.0467849591103274,0.963021699437997,0.265330688034002));
#87434=DIRECTION('',(-0.984807734026167,4.52289952656485E-7,0.173648285341494));
#87435=DIRECTION('center_axis',(0.984807753012213,3.99726500021128E-16,
-0.173648177666902));
#87436=DIRECTION('ref_axis',(0.00236288091262727,0.999907416559164,0.0134005635617093));
#87437=DIRECTION('',(0.984807753012213,0.,-0.173648177666902));
#87438=DIRECTION('',(0.984809659012493,-8.77532653136194E-6,-0.173637367633499));
#87439=DIRECTION('center_axis',(-0.984807753012213,3.51192997585509E-17,
0.173648177666903));
#87440=DIRECTION('ref_axis',(-0.173365149690665,-0.0570712691222515,-0.983202621596133));
#87441=DIRECTION('center_axis',(-0.172758048290314,0.100499036796366,-0.979823759843537));
#87442=DIRECTION('ref_axis',(0.984808733743122,-5.48978072977703E-5,-0.173642606895596));
#87443=DIRECTION('center_axis',(-0.984807753012213,7.02386062257915E-17,
0.173648177666903));
#87444=DIRECTION('ref_axis',(0.173046305904731,0.0831869535125862,0.981394368629666));
#87445=DIRECTION('center_axis',(-0.0143784831960099,0.996544562420649,-0.0818058331099832));
#87446=DIRECTION('ref_axis',(0.984809079270561,-4.49124382155832E-5,-0.173640650105737));
#87447=DIRECTION('center_axis',(-0.984807753012107,-8.63808404924054E-17,
0.173648177667502));
#87448=DIRECTION('ref_axis',(-0.172276800540999,0.125429352942195,-0.977030286846758));
#87449=DIRECTION('center_axis',(-0.984807753012108,6.73770473281316E-17,
0.1736481776675));
#87450=DIRECTION('ref_axis',(0.173048689248285,-0.0830223701171357,0.981407885239151));
#87451=DIRECTION('center_axis',(0.0144827209458809,0.996537080801731,0.0818785526323483));
#87452=DIRECTION('ref_axis',(0.984806418859583,-4.41489308059733E-5,-0.173655738240447));
#87453=DIRECTION('center_axis',(-0.984807753012107,-2.45183611171223E-18,
0.173648177667501));
#87454=DIRECTION('ref_axis',(0.173048500696551,-0.0830354026532529,0.981406815909125));
#87455=DIRECTION('center_axis',(-0.984807753012107,3.1873869452259E-17,
0.173648177667502));
#87456=DIRECTION('ref_axis',(0.173648177667502,9.94558247889318E-15,0.984807753012107));
#87457=DIRECTION('center_axis',(-0.984787402847089,4.77665004704958E-6,
0.173763549603677));
#87458=DIRECTION('ref_axis',(0.0460456062353661,-0.964243981143723,0.260985338619855));
#87459=DIRECTION('center_axis',(-0.984787403020211,-4.77668398007977E-6,
0.173763548622521));
#87460=DIRECTION('ref_axis',(-0.0460456142525782,-0.964243968000674,-0.260985385764066));
#87461=DIRECTION('',(0.984807753012107,0.,-0.173648177667501));
#87462=DIRECTION('center_axis',(0.778348606443954,9.80121874209452E-8,-0.62783233975859));
#87463=DIRECTION('ref_axis',(0.625005248891585,-0.0947925361689985,0.774843735178015));
#87464=DIRECTION('center_axis',(-0.984807753012107,3.1873869452259E-17,
0.173648177667502));
#87465=DIRECTION('ref_axis',(0.173648177660458,9.0068198248696E-6,0.984807752972162));
#87466=DIRECTION('center_axis',(0.416627933083572,-8.76783794334763E-5,
-0.909077091168297));
#87467=DIRECTION('ref_axis',(0.904296443220308,0.102460377442959,0.414427091094858));
#87468=DIRECTION('center_axis',(0.416694788203033,9.03336795019935E-5,-0.90904644838658));
#87469=DIRECTION('ref_axis',(0.903932694694705,-0.105961771702308,0.414340181975725));
#87470=DIRECTION('center_axis',(-0.173648177666902,0.,-0.984807753012213));
#87471=DIRECTION('ref_axis',(-0.984807753012213,0.,0.173648177666902));
#87472=DIRECTION('',(0.,-1.,0.));
#87473=DIRECTION('',(0.984807752993594,6.14919168343789E-6,-0.173648177663619));
#87474=DIRECTION('center_axis',(-0.173648177666902,3.60825379108868E-16,
-0.984807753012213));
#87475=DIRECTION('ref_axis',(0.791113853674831,0.595550245061522,-0.139494717215097));
#87476=DIRECTION('',(-0.98480775279897,2.08102296353245E-5,0.173648177629302));
#87477=DIRECTION('',(0.,-1.,0.));
#87478=DIRECTION('center_axis',(0.173648177666902,0.,0.984807753012213));
#87479=DIRECTION('ref_axis',(0.,-1.,0.));
#87480=DIRECTION('center_axis',(0.173648177666902,0.,0.984807753012213));
#87481=DIRECTION('ref_axis',(0.,-1.,0.));
#87482=DIRECTION('center_axis',(0.140833149244339,-0.988277940715504,0.0589299242239757));
#87483=DIRECTION('ref_axis',(-0.976574519445544,-0.128890957877333,0.172305916750323));
#87484=DIRECTION('center_axis',(-1.45716096092398E-7,-0.999999999999986,
-8.54998680566197E-8));
#87485=DIRECTION('ref_axis',(0.173652309740699,-1.0950480730089E-7,0.984807024407172));
#87486=DIRECTION('center_axis',(0.397005631927029,-5.6725704996324E-5,-0.91781617168168));
#87487=DIRECTION('ref_axis',(-0.618040008182569,0.739279070835237,-0.26738175650309));
#87488=DIRECTION('center_axis',(-0.984807753012213,2.46716227694479E-17,
0.173648177666903));
#87489=DIRECTION('ref_axis',(0.173648177666902,7.45831290246043E-11,0.984807753012213));
#87490=DIRECTION('center_axis',(0.396684871120988,8.29230411004112E-5,-0.917954849732542));
#87491=DIRECTION('ref_axis',(0.917617038505464,-0.0271629495190743,0.396536435675066));
#87492=DIRECTION('',(0.984807753012213,0.,-0.173648177666902));
#87493=DIRECTION('center_axis',(-0.984807752591731,-1.68263835837692E-10,
0.173648180051576));
#87494=DIRECTION('ref_axis',(0.173648180048437,-6.01398766220049E-6,0.984807752573921));
#87495=DIRECTION('center_axis',(-0.984807753398451,-2.54577945895623E-11,
0.173648175476438));
#87496=DIRECTION('ref_axis',(0.173046505047202,0.0831730633887027,0.981395510799539));
#87497=DIRECTION('',(0.984807753012213,0.,-0.173648177666902));
#87498=DIRECTION('center_axis',(-0.984807753012213,2.46716227694479E-17,
0.173648177666903));
#87499=DIRECTION('ref_axis',(0.173648177666902,1.30076688193796E-8,0.984807753012213));
#87500=DIRECTION('center_axis',(-0.686735486868187,-8.14046591486839E-5,
-0.726907397437388));
#87501=DIRECTION('ref_axis',(0.726646064054819,-0.0268893988940089,-0.686485584568794));
#87502=DIRECTION('',(0.984807753012213,0.,-0.173648177666902));
#87503=DIRECTION('center_axis',(0.516198321513486,-3.61900781727334E-6,
-0.856469084587157));
#87504=DIRECTION('ref_axis',(0.856468926804281,0.00060919642574273,0.516198223842778));
#87505=DIRECTION('',(0.984807753012213,0.,-0.173648177666902));
#87506=DIRECTION('center_axis',(-0.686740422865691,8.08918317377472E-5,
-0.726902734249063));
#87507=DIRECTION('ref_axis',(0.72661180009037,0.0283664668836154,-0.686462406491407));
#87508=DIRECTION('center_axis',(-0.984807753012213,1.09651656753102E-17,
0.173648177666902));
#87509=DIRECTION('ref_axis',(0.118437018843228,0.731304043279059,0.671689711735432));
#87510=DIRECTION('',(-0.984807851409346,7.72996941407336E-9,0.173647619628108));
#87511=DIRECTION('center_axis',(0.112178949404874,0.988278168362575,-0.103547792097819));
#87512=DIRECTION('ref_axis',(0.95746136560598,-0.0796203342802649,0.277359578419478));
#87513=DIRECTION('center_axis',(8.73464525969481E-8,0.999999999999991,-1.05573893634399E-7));
#87514=DIRECTION('ref_axis',(0.17364493317501,8.88027804399136E-8,0.984808325098158));
#87515=DIRECTION('center_axis',(-0.112184478285304,0.988277949487833,0.10354389111859));
#87516=DIRECTION('ref_axis',(0.976611185680797,0.128891163139917,-0.172097821216851));
#87517=DIRECTION('center_axis',(-0.140829727433864,-0.98827813488146,-0.0589348452625973));
#87518=DIRECTION('ref_axis',(0.805607533053029,-0.0797909770181293,-0.587051873921466));
#87519=DIRECTION('center_axis',(-0.984807753012213,-3.0154205607103E-17,
0.173648177666903));
#87520=DIRECTION('ref_axis',(-0.173046420789344,0.083179027598608,-0.981395020172686));
#87521=DIRECTION('',(0.984807681305532,-5.61027557369018E-9,-0.173648584335206));
#87522=DIRECTION('',(0.984807945990428,-1.26003174213104E-13,-0.173647083229505));
#87523=DIRECTION('center_axis',(-0.984807753031958,3.17862934597828E-11,
0.173648177554921));
#87524=DIRECTION('ref_axis',(-0.0511404417972143,-0.955649609771606,-0.290031857829726));
#87525=DIRECTION('center_axis',(-0.984807753012213,-9.71445146547012E-17,
0.173648177666902));
#87526=DIRECTION('ref_axis',(-0.0915527669893199,0.849721766333212,-0.519221542962313));
#87527=DIRECTION('',(0.984807753012213,0.,-0.173648177666902));
#87528=DIRECTION('',(0.984807789518797,4.35503035001299E-7,-0.1736479706271));
#87529=DIRECTION('center_axis',(-0.454554571362216,-0.76693110554782,0.452986557192275));
#87530=DIRECTION('ref_axis',(-0.81199513940023,0.565830688971329,0.143176551881345));
#87531=DIRECTION('center_axis',(-0.984807753012213,-3.5605199344424E-16,
0.173648177666902));
#87532=DIRECTION('ref_axis',(-0.00236288091263331,0.999907416559164,-0.0134005635617392));
#87533=DIRECTION('',(0.984807787586651,-4.14936868640622E-7,-0.173647981584909));
#87534=DIRECTION('',(0.984807753012213,0.,-0.173648177666902));
#87535=DIRECTION('center_axis',(-0.984815825350885,-1.94466018545213E-5,
0.173602389846124));
#87536=DIRECTION('ref_axis',(0.0511700711168919,-0.955605550622165,0.290171768857692));
#87537=DIRECTION('center_axis',(-0.190809912898502,-9.49751800403212E-8,
0.981627005099013));
#87538=DIRECTION('ref_axis',(-4.97747620118824E-7,0.999999999999876,4.04178578453096E-24));
#87539=DIRECTION('center_axis',(0.190809912898503,0.,-0.981627005099017));
#87540=DIRECTION('ref_axis',(0.,-1.,0.));
#87541=DIRECTION('center_axis',(0.190809912898503,0.,-0.981627005099017));
#87542=DIRECTION('ref_axis',(0.,-1.,0.));
#87543=DIRECTION('center_axis',(-0.190809912898503,0.,0.981627005099017));
#87544=DIRECTION('ref_axis',(0.,1.,0.));
#87545=DIRECTION('',(-3.635245538593E-8,0.999999999999999,-1.866361044514E-8));
#87546=DIRECTION('center_axis',(0.190809912898503,0.,-0.981627005099017));
#87547=DIRECTION('ref_axis',(0.,-1.,0.));
#87548=DIRECTION('center_axis',(-8.80448426118404E-5,0.999999995977604,
-1.71142691292802E-5));
#87549=DIRECTION('ref_axis',(0.473468177754614,5.6760866602408E-5,0.880810922634324));
#87550=DIRECTION('center_axis',(-0.976953213978548,0.0974838992373601,-0.189892883190669));
#87551=DIRECTION('ref_axis',(0.190801607119635,-4.66549814768457E-7,-0.981628619550361));
#87552=DIRECTION('center_axis',(-0.800108939388847,-0.588097435439644,-0.118182450217318));
#87553=DIRECTION('ref_axis',(0.596174896320331,-0.757825141935888,-0.265097241115962));
#87554=DIRECTION('center_axis',(-0.675651786267923,-0.735965325320194,-0.0430081810741494));
#87555=DIRECTION('ref_axis',(-0.730667597463077,0.676266554259198,-0.0937465178442656));
#87556=DIRECTION('center_axis',(0.107073044687985,-0.827666229220606,-0.550911949506441));
#87557=DIRECTION('ref_axis',(0.98163660235276,1.75954457808426E-5,0.190760532112199));
#87558=DIRECTION('center_axis',(-0.981627005099017,0.,-0.190809912898503));
#87559=DIRECTION('ref_axis',(-0.190809912898503,0.,0.981627005099017));
#87560=DIRECTION('',(-6.598096137308E-10,1.,-1.279942325608E-10));
#87561=DIRECTION('center_axis',(0.,1.,0.));
#87562=DIRECTION('ref_axis',(0.981627005099017,0.,0.190809912898502));
#87563=DIRECTION('center_axis',(-0.799675205911076,0.588765746219848,-0.117789902492802));
#87564=DIRECTION('ref_axis',(0.596998789463264,0.800603041435647,-0.0512563695884574));
#87565=DIRECTION('center_axis',(0.976958619535709,0.0974612280175059,0.189876709335828));
#87566=DIRECTION('ref_axis',(0.190786976255942,-2.08181573059927E-5,-0.981631463054093));
#87567=DIRECTION('center_axis',(-0.984807753012213,-2.95751398859563E-17,
0.173648177666903));
#87568=DIRECTION('ref_axis',(-0.173046420789344,0.0831790275986082,-0.981395020172686));
#87569=DIRECTION('center_axis',(0.984807753012213,3.03145183831052E-16,
-0.173648177666902));
#87570=DIRECTION('ref_axis',(0.0108577499378729,-0.998043254585349,0.0615773598246225));
#87571=DIRECTION('',(0.984807753012213,0.,-0.173648177666902));
#87572=DIRECTION('center_axis',(0.984807753012213,9.16829336464645E-16,
-0.173648177666903));
#87573=DIRECTION('ref_axis',(0.103441898062484,-0.803208388241305,0.586648155868606));
#87574=DIRECTION('',(-0.984807766253658,9.3962545399306E-8,0.173648102570893));
#87575=DIRECTION('center_axis',(0.172766604332646,0.100486419652285,0.979823545283962));
#87576=DIRECTION('ref_axis',(0.98480822440525,-1.91663112048265E-7,-0.173645504242816));
#87577=DIRECTION('center_axis',(-0.240517466226023,0.0124905486229052,0.970564441258442));
#87578=DIRECTION('ref_axis',(0.957551275334907,0.166737877871554,0.235146837502408));
#87579=DIRECTION('center_axis',(-0.984807753012213,-1.51942396384287E-16,
0.173648177666902));
#87580=DIRECTION('ref_axis',(-0.0915531241012405,-0.849720490306423,-0.519223568244658));
#87581=DIRECTION('center_axis',(0.984807753012213,1.51942396384287E-16,
-0.173648177666902));
#87582=DIRECTION('ref_axis',(0.00236288091262946,-0.999907416559164,0.0134005635617186));
#87583=DIRECTION('center_axis',(-0.984807753012213,-7.51655445223487E-16,
0.173648177666902));
#87584=DIRECTION('ref_axis',(-0.0140997774057779,0.996698041116542,-0.0799638112620634));
#87585=DIRECTION('center_axis',(0.984807753012213,-1.47930621883394E-15,
-0.173648177666902));
#87586=DIRECTION('ref_axis',(0.00236288091262263,-0.999907416559164,0.0134005635616892));
#87587=DIRECTION('center_axis',(-0.984807753012213,-3.50624536671156E-16,
0.173648177666902));
#87588=DIRECTION('ref_axis',(-0.0174417350637655,0.994942819454527,-0.0989169949697339));
#87589=DIRECTION('center_axis',(0.984807753012213,4.05541630188082E-16,
-0.173648177666902));
#87590=DIRECTION('ref_axis',(0.0108576734130155,-0.99804328219437,0.0615769258305894));
#87591=DIRECTION('center_axis',(-0.173295783426445,-0.062517609495443,-0.98288357395451));
#87592=DIRECTION('ref_axis',(-0.984810412796333,3.80932965607098E-5,0.173633088427341));
#87593=DIRECTION('center_axis',(0.984807753012213,-5.38458166943201E-15,
-0.173648177666901));
#87594=DIRECTION('ref_axis',(-0.0407970909149098,0.972009612883567,-0.231371799999089));
#87595=DIRECTION('',(0.984807687628933,-2.59140590676409E-7,-0.173648548473306));
#87596=DIRECTION('center_axis',(0.984807753012213,-5.38458166943201E-15,
-0.173648177666901));
#87597=DIRECTION('ref_axis',(0.0407970909149098,-0.972009612883567,0.231371799999089));
#87598=DIRECTION('center_axis',(-0.167224647446209,-0.269421488102054,-0.948392312830174));
#87599=DIRECTION('ref_axis',(-0.984808093511156,-2.14966491856184E-6,0.173646246577062));
#87600=DIRECTION('center_axis',(-0.984807753012213,-2.02770816388138E-16,
0.173648177666902));
#87601=DIRECTION('ref_axis',(-0.110025883188373,0.7736494953753,-0.623987791013705));
#87602=DIRECTION('center_axis',(0.984807753012213,1.52078009876091E-16,
-0.173648177666902));
#87603=DIRECTION('ref_axis',(0.103441898062483,-0.803208388241305,0.586648155868606));
#87604=DIRECTION('center_axis',(-0.139475672938697,-0.595698149020197,-0.791005848216187));
#87605=DIRECTION('ref_axis',(0.103441898016906,-0.803208388435972,0.586648155610114));
#87606=DIRECTION('center_axis',(-0.984807753012214,3.20576898360514E-15,
0.173648177666899));
#87607=DIRECTION('ref_axis',(-0.109429766257885,0.776448339114792,-0.620607043903488));
#87608=DIRECTION('center_axis',(0.,-1.,0.));
#87609=DIRECTION('ref_axis',(-0.173648177666898,0.,-0.984807753012214));
#87610=DIRECTION('',(-8.565880838752E-11,-1.,1.505910719479E-11));
#87611=DIRECTION('center_axis',(0.984901889102444,0.000257016284667763,
-0.173113265768588));
#87612=DIRECTION('ref_axis',(0.173113399729199,-0.000651956645208656,0.984901683309929));
#87613=DIRECTION('center_axis',(0.139473992434594,-0.595698140751181,0.791006150759866));
#87614=DIRECTION('ref_axis',(0.103440598648708,0.803208394568672,0.586648376325728));
#87615=DIRECTION('center_axis',(-0.984807753012213,3.46400144663069E-16,
0.173648177666902));
#87616=DIRECTION('ref_axis',(-0.0421501634500986,-0.97009310576118,-0.239045455668495));
#87617=DIRECTION('center_axis',(0.984807753012213,-4.22438916266538E-17,
-0.173648177666902));
#87618=DIRECTION('ref_axis',(0.0467849591103272,0.963021699437997,0.265330688034001));
#87619=DIRECTION('center_axis',(0.167232170899728,-0.269429194209485,0.948388797025667));
#87620=DIRECTION('ref_axis',(-0.984803328168082,7.04152060432668E-5,0.17367325606082));
#87621=DIRECTION('center_axis',(-0.9848077750298,-7.05368960287473E-8,0.1736480527989));
#87622=DIRECTION('ref_axis',(0.0407970401597095,0.972009548712139,0.231372078537215));
#87623=DIRECTION('center_axis',(-0.984807753012213,-5.38458166943201E-15,
0.173648177666901));
#87624=DIRECTION('ref_axis',(-0.0407970909149098,-0.972009612883567,-0.231371799999089));
#87625=DIRECTION('',(-0.984807701505426,-2.26153704840706E-7,0.173648469776005));
#87626=DIRECTION('center_axis',(-0.984803957534525,-0.000225618307817559,
0.173669554962053));
#87627=DIRECTION('ref_axis',(0.172048805725959,-0.13757327250827,0.975434673947793));
#87628=DIRECTION('center_axis',(0.173311955176598,-0.0625216763371239,0.982880463831111));
#87629=DIRECTION('ref_axis',(-0.984807591131402,-4.20708473535737E-5,0.173649090639741));
#87630=DIRECTION('center_axis',(-0.984807753012213,3.73594668215124E-16,
0.173648177666902));
#87631=DIRECTION('ref_axis',(0.00180597749651713,-0.999945916354496,0.0102422073426411));
#87632=DIRECTION('center_axis',(0.984807753012213,-2.14387893151549E-16,
-0.173648177666902));
#87633=DIRECTION('ref_axis',(0.00236288091262434,0.999907416559164,0.0134005635616892));
#87634=DIRECTION('center_axis',(0.173632090960341,-0.0136072847582164,0.984716577899575));
#87635=DIRECTION('ref_axis',(-0.984807754634243,4.27085877774405E-8,0.173648168467909));
#87636=DIRECTION('center_axis',(-0.984807753012213,-4.38922887721939E-17,
0.173648177666902));
#87637=DIRECTION('ref_axis',(0.161562458752702,-0.366542983040298,0.916266235057094));
#87638=DIRECTION('center_axis',(0.984807753012213,4.55368148680565E-16,
-0.173648177666903));
#87639=DIRECTION('ref_axis',(-0.156740864913815,0.43040754996901,-0.888921617577019));
#87640=DIRECTION('center_axis',(-0.984807753012213,-2.93785902374558E-17,
0.173648177666902));
#87641=DIRECTION('ref_axis',(-0.0917700003358048,0.848944277013721,-0.520453534490849));
#87642=DIRECTION('center_axis',(-0.984807753012145,-1.27114520028174E-13,
0.17364817766729));
#87643=DIRECTION('ref_axis',(-0.166072447287528,0.29214804337792,-0.941843651038953));
#87644=DIRECTION('center_axis',(0.984807753012145,1.27328329737158E-13,
-0.173648177667291));
#87645=DIRECTION('ref_axis',(-0.162244947343955,0.356405400048795,-0.920136820194375));
#87646=DIRECTION('center_axis',(-0.201501638275048,0.96280516344127,0.180009185941446));
#87647=DIRECTION('ref_axis',(0.976016676961642,0.181908483442498,0.119585743064987));
#87648=DIRECTION('center_axis',(1.21185977076882E-11,1.,-3.61798710391132E-11));
#87649=DIRECTION('ref_axis',(0.996578836186276,-9.08695904165718E-12,0.0826475847536266));
#87650=DIRECTION('center_axis',(0.201484553848451,0.962823392583096,-0.179930790181304));
#87651=DIRECTION('ref_axis',(0.976087907632447,-0.182066474456054,0.118761085599849));
#87652=DIRECTION('center_axis',(-0.984807753012213,-1.44182084052305E-14,
0.173648177666903));
#87653=DIRECTION('ref_axis',(-0.166064612600648,-0.292295700970649,-0.941799218324094));
#87654=DIRECTION('center_axis',(0.984807753012213,1.47249787968311E-14,
-0.173648177666902));
#87655=DIRECTION('ref_axis',(-0.156683846646441,-0.431095489042511,-0.888598250913917));
#87656=DIRECTION('',(0.984807776058194,5.24229513912697E-14,-0.173648046966599));
#87657=DIRECTION('center_axis',(-0.0771912637911887,-0.914517936634286,
0.397112644432895));
#87658=DIRECTION('ref_axis',(-0.141744409590102,-0.384189181042076,-0.912308717222505));
#87659=DIRECTION('center_axis',(-3.05340545697296E-8,-0.999999999999987,
1.57083313648698E-7));
#87660=DIRECTION('ref_axis',(-0.173648189854594,-1.49394681507557E-7,-0.984807750863183));
#87661=DIRECTION('center_axis',(0.0771819226456397,-0.914539590865797,-0.3970645886449));
#87662=DIRECTION('ref_axis',(-0.141611064558104,0.384159300577726,-0.912342007239803));
#87663=DIRECTION('center_axis',(0.084142908898196,-0.897541669062807,-0.432826666436));
#87664=DIRECTION('ref_axis',(0.981622833089212,-3.42192540777386E-7,0.190831374668297));
#87665=DIRECTION('center_axis',(-0.0841377180325195,-0.897531445507195,
0.432848875163198));
#87666=DIRECTION('ref_axis',(-0.135188302065196,-0.420091172265935,-0.89735585470256));
#87667=DIRECTION('center_axis',(-0.677112882379002,0.734636173451785,-0.0427532124233805));
#87668=DIRECTION('ref_axis',(-0.733973201133508,-0.678397144997567,-0.0325676784094527));
#87669=DIRECTION('center_axis',(-0.190686705650736,-0.0313546077358391,
0.98115007458686));
#87670=DIRECTION('ref_axis',(0.981632739712338,-3.22581837650991E-6,0.19078040862322));
#87671=DIRECTION('center_axis',(-0.984807753012213,-1.44799683600039E-14,
0.173648177666903));
#87672=DIRECTION('ref_axis',(0.155662080843755,0.443201134484021,0.882803529093234));
#87673=DIRECTION('center_axis',(0.984807753012213,1.44399655486805E-14,
-0.173648177666903));
#87674=DIRECTION('ref_axis',(-0.15668505394005,-0.431080936724009,-0.888605097816209));
#87675=DIRECTION('center_axis',(0.984807753012213,0.,-0.173648177666902));
#87676=DIRECTION('ref_axis',(0.,-1.,0.));
#87677=DIRECTION('center_axis',(0.984807753012145,1.27057714228674E-13,
-0.17364817766729));
#87678=DIRECTION('ref_axis',(-0.162245431570886,0.356398089659788,-0.920139566381769));
#87679=DIRECTION('',(8.81218894669602E-8,0.999999999999902,4.32820325270801E-7));
#87680=DIRECTION('center_axis',(0.,1.,0.));
#87681=DIRECTION('ref_axis',(-0.173648177666898,0.,-0.984807753012214));
#87682=DIRECTION('',(-7.10683480609823E-7,0.999999999999732,1.76068375849406E-7));
#87683=DIRECTION('center_axis',(0.173648177666902,0.,0.984807753012213));
#87684=DIRECTION('ref_axis',(0.,-1.,0.));
#87685=DIRECTION('',(2.81021024324399E-5,-0.999999999592795,-4.96817573254497E-6));
#87686=DIRECTION('',(-2.79857101008889E-5,-0.999999999596161,4.94759277264081E-6));
#87687=DIRECTION('center_axis',(0.,-1.,0.));
#87688=DIRECTION('ref_axis',(0.984807753012214,0.,-0.173648177666898));
#87689=DIRECTION('',(0.,-1.,0.));
#87690=DIRECTION('center_axis',(0.984807753012213,0.,-0.173648177666902));
#87691=DIRECTION('ref_axis',(0.,-1.,0.));
#87692=DIRECTION('center_axis',(0.173648177666902,0.,0.984807753012213));
#87693=DIRECTION('ref_axis',(0.,-1.,0.));
#87694=DIRECTION('center_axis',(0.173648177666902,0.,0.984807753012213));
#87695=DIRECTION('ref_axis',(0.,-1.,0.));
#87696=DIRECTION('center_axis',(-0.173648177666903,8.36511531019332E-17,
-0.984807753012213));
#87697=DIRECTION('ref_axis',(-0.975914789972338,0.134084894844204,0.17208010834453));
#87698=DIRECTION('',(0.,1.,0.));
#87699=DIRECTION('center_axis',(0.,1.,0.));
#87700=DIRECTION('ref_axis',(-0.819141634169878,0.,-0.573591303254767));
#87701=DIRECTION('',(1.39364876480604E-5,0.999999999901329,-1.76500621154505E-6));
#87702=DIRECTION('',(-7.60889122223396E-8,0.999999999999997,1.313139806872E-8));
#87703=DIRECTION('',(-3.71082567177192E-8,0.999999999999977,-2.10540427148495E-7));
#87704=DIRECTION('center_axis',(0.173648177666902,0.,0.984807753012213));
#87705=DIRECTION('ref_axis',(0.984807753012213,-1.22464679914735E-16,-0.173648177666902));
#87706=DIRECTION('center_axis',(0.173648177666902,8.44686595599678E-23,
0.984807753012213));
#87707=DIRECTION('ref_axis',(0.984807753012137,3.91820935308914E-7,-0.173648177666889));
#87708=DIRECTION('center_axis',(0.173648177666902,-2.4603280324098E-16,
0.984807753012213));
#87709=DIRECTION('ref_axis',(-0.829311792010217,-0.539313198208507,0.146230044351063));
#87710=DIRECTION('center_axis',(-0.173648177666902,0.,-0.984807753012213));
#87711=DIRECTION('ref_axis',(-0.984807753012213,0.,0.173648177666902));
#87712=DIRECTION('',(-1.090258469048E-7,0.999999999999801,-6.20717966282101E-7));
#87713=DIRECTION('center_axis',(-0.173648177666903,6.47634049830965E-16,
-0.984807753012213));
#87714=DIRECTION('ref_axis',(-0.681789982854665,0.721602424588165,0.12021796915402));
#87715=DIRECTION('center_axis',(0.173648177666902,-2.87247579347555E-16,
0.984807753012213));
#87716=DIRECTION('ref_axis',(-0.606044361063923,-0.788219989143623,0.106861972361774));
#87717=DIRECTION('center_axis',(0.173648177666903,2.73912803682029E-16,
0.984807753012213));
#87718=DIRECTION('ref_axis',(-0.750334089213524,-0.647683848740426,0.132304144473635));
#87719=DIRECTION('center_axis',(-0.173648177666902,0.,-0.984807753012213));
#87720=DIRECTION('ref_axis',(-0.984807753012213,0.,0.173648177666902));
#87721=DIRECTION('center_axis',(-0.173648177666902,-1.61124207346389E-16,
-0.984807753012213));
#87722=DIRECTION('ref_axis',(-0.750329716580782,0.647689071844487,0.132303373460505));
#87723=DIRECTION('center_axis',(-0.173648177666902,-2.87247456824783E-16,
-0.984807753012213));
#87724=DIRECTION('ref_axis',(-0.606044921708883,0.788219544673781,0.106862071218607));
#87725=DIRECTION('center_axis',(0.173648177666903,6.10624530269016E-16,
0.984807753012213));
#87726=DIRECTION('ref_axis',(-0.681789982854614,-0.721602424588215,0.120217969154011));
#87727=DIRECTION('',(8.2153927947679E-8,0.999999999999888,4.67122875809294E-7));
#87728=DIRECTION('center_axis',(-0.173648177666902,1.77232881935626E-16,
-0.984807753012213));
#87729=DIRECTION('ref_axis',(0.801893974638295,0.580494060044092,-0.141395543396257));
#87730=DIRECTION('center_axis',(0.659077833040731,-0.743026690968582,-0.116308841033747));
#87731=DIRECTION('ref_axis',(-0.173639109027328,0.000135049773334708,-0.984809342755111));
#87732=DIRECTION('center_axis',(0.173648177666902,-1.20886287747465E-16,
0.984807753012213));
#87733=DIRECTION('ref_axis',(-0.750329716580742,-0.647689071844535,0.132303373460498));
#87734=DIRECTION('center_axis',(0.637849218735937,-0.761904762558937,-0.112470026887006));
#87735=DIRECTION('ref_axis',(-0.750329717224971,-0.64768907107501,0.132303373574089));
#87736=DIRECTION('center_axis',(-0.173668324352799,-6.63106817671438E-6,
-0.98480420037311));
#87737=DIRECTION('ref_axis',(-0.984804200395333,1.62419221665202E-6,0.17366832434578));
#87738=DIRECTION('center_axis',(-0.173648177666903,0.,-0.984807753012213));
#87739=DIRECTION('ref_axis',(0.984807753012213,0.,-0.173648177666903));
#87740=DIRECTION('',(-0.173878181060975,0.000322054883223046,-0.984767116851278));
#87741=DIRECTION('center_axis',(-0.173648177666903,0.,-0.984807753012213));
#87742=DIRECTION('ref_axis',(0.984807753012213,0.,-0.173648177666903));
#87743=DIRECTION('',(-0.173877367546055,-0.00032091573288183,-0.984767260863371));
#87744=DIRECTION('center_axis',(-0.173648177666902,-1.20886287747465E-16,
-0.984807753012213));
#87745=DIRECTION('ref_axis',(-0.750329716580742,0.647689071844535,0.132303373460498));
#87746=DIRECTION('center_axis',(-0.173648177666897,3.28903571045203E-15,
-0.984807753012214));
#87747=DIRECTION('ref_axis',(-0.936719925941306,-0.308666459146836,0.165168996310654));
#87748=DIRECTION('',(-0.173636642897303,-6.51718399708411E-5,-0.984809784677217));
#87749=DIRECTION('center_axis',(-0.984807753012213,0.,0.173648177666902));
#87750=DIRECTION('ref_axis',(0.,1.,0.));
#87751=DIRECTION('',(2.35372139113308E-6,0.999999999974235,6.78157916925224E-6));
#87752=DIRECTION('center_axis',(-0.984807753012213,-2.26576147468896E-16,
0.173648177666902));
#87753=DIRECTION('ref_axis',(0.0174469104577598,-0.994939810195265,0.0989463460876066));
#87754=DIRECTION('',(-1.35344856793906E-6,0.999999999998245,-1.29536058899606E-6));
#87755=DIRECTION('',(-0.173639122016199,6.67188537162898E-5,-0.984809347464796));
#87756=DIRECTION('center_axis',(-0.173648177666907,-1.19615497498102E-14,
-0.984807753012212));
#87757=DIRECTION('ref_axis',(-0.936720096114287,0.308665926660553,0.165169026316749));
#87758=DIRECTION('center_axis',(-0.172153314886262,-0.000369434897238181,
-0.985070098871917));
#87759=DIRECTION('ref_axis',(-0.938950108420514,0.302462075571974,0.163979836375689));
#87760=DIRECTION('center_axis',(-0.173642877220662,-1.74636676018426E-6,
-0.984808687607639));
#87761=DIRECTION('ref_axis',(-0.797231544682396,0.587079646333193,0.140567965855004));
#87762=DIRECTION('center_axis',(0.637849235778954,0.761904751719864,-0.112470003658296));
#87763=DIRECTION('ref_axis',(-0.750329430917128,0.647689083824637,0.132304934881434));
#87764=DIRECTION('center_axis',(-0.173648177666902,-3.38353683695286E-16,
-0.984807753012213));
#87765=DIRECTION('ref_axis',(0.785231832909193,-0.603523382437399,-0.138457558253028));
#87766=DIRECTION('center_axis',(-0.173648177666902,1.43623595195129E-16,
-0.984807753012213));
#87767=DIRECTION('ref_axis',(0.630875084425314,-0.767868624027015,-0.111240298840895));
#87768=DIRECTION('center_axis',(-0.173648177666902,-2.93948484863116E-16,
-0.984807753012213));
#87769=DIRECTION('ref_axis',(-0.606035537815208,0.788226983978802,0.106860416584968));
#87770=DIRECTION('center_axis',(0.710639662326888,-0.692307692307688,-0.125304946029797));
#87771=DIRECTION('ref_axis',(-0.173648177665894,1.11610884899936E-12,-0.984807753012391));
#87772=DIRECTION('center_axis',(-0.173648177666902,3.88578058618862E-16,
-0.984807753012213));
#87773=DIRECTION('ref_axis',(0.889587405855847,0.428986868317277,-0.156858261350812));
#87774=DIRECTION('center_axis',(-0.173648177666898,0.,-0.984807753012214));
#87775=DIRECTION('ref_axis',(0.915664591049666,-0.36808992979761,-0.161456372681408));
#87776=DIRECTION('',(0.173648177666902,7.6637955192051E-11,0.984807753012213));
#87777=DIRECTION('center_axis',(-0.984807753012213,0.,0.173648177666902));
#87778=DIRECTION('ref_axis',(0.,1.,0.));
#87779=DIRECTION('',(4.437051728155E-11,-1.,2.516170452507E-10));
#87780=DIRECTION('',(-1.351043146217E-10,-1.,-1.097321493067E-11));
#87781=DIRECTION('',(1.996062744186E-11,-1.,1.132315338918E-10));
#87782=DIRECTION('',(-0.173648177666902,1.00328634318001E-11,-0.984807753012213));
#87783=DIRECTION('',(0.,1.,0.));
#87784=DIRECTION('center_axis',(0.,1.,0.));
#87785=DIRECTION('ref_axis',(0.819151987079672,0.,0.573576518054414));
#87786=DIRECTION('center_axis',(-4.06837822689946E-10,1.,-2.53848971472811E-9));
#87787=DIRECTION('ref_axis',(0.312566484770769,2.53846366149446E-9,0.949895885135863));
#87788=DIRECTION('center_axis',(0.173648177666903,-1.19205647900064E-29,
0.984807753012213));
#87789=DIRECTION('ref_axis',(0.984807753012213,-1.04083408558608E-14,-0.173648177666903));
#87790=DIRECTION('center_axis',(4.41761171680438E-10,-1.,2.56294060048864E-9));
#87791=DIRECTION('ref_axis',(-3.11479720759106E-33,2.56294060048864E-9,
1.));
#87792=DIRECTION('center_axis',(-0.710639662326888,-0.692307692307688,0.125304946029795));
#87793=DIRECTION('ref_axis',(0.173648177387696,2.95556609701271E-10,0.984807753061445));
#87794=DIRECTION('center_axis',(-0.173648177666899,-3.16105230837517E-15,
-0.984807753012214));
#87795=DIRECTION('ref_axis',(-0.681789982854612,0.721602424588218,0.120217969154005));
#87796=DIRECTION('center_axis',(-0.173648177666901,-4.0708177569595E-16,
-0.984807753012213));
#87797=DIRECTION('ref_axis',(0.893467078353688,-0.420591235207693,-0.157542352288493));
#87798=DIRECTION('center_axis',(0.71063966232689,0.692307692307686,-0.125304946029799));
#87799=DIRECTION('ref_axis',(0.633285392360227,-0.707023094958418,-0.314750623539612));
#87800=DIRECTION('center_axis',(-0.173648177666903,-3.98954431097579E-16,
-0.984807753012213));
#87801=DIRECTION('ref_axis',(0.629931807325388,0.768666696624785,-0.111073973637894));
#87802=DIRECTION('center_axis',(0.173648177666902,-1.87058128807964E-16,
0.984807753012213));
#87803=DIRECTION('ref_axis',(-0.606035677048363,-0.78822687359976,0.10686044113553));
#87804=DIRECTION('center_axis',(-0.173648177666902,1.05109872153861E-16,
-0.984807753012213));
#87805=DIRECTION('ref_axis',(-0.709980153735304,0.693005037133797,0.125188656871057));
#87806=DIRECTION('center_axis',(-0.173648177666902,4.20439473358018E-17,
-0.984807753012213));
#87807=DIRECTION('ref_axis',(0.681789982854614,-0.721602424588215,-0.12021796915401));
#87808=DIRECTION('center_axis',(0.,1.,0.));
#87809=DIRECTION('ref_axis',(-0.819128681345575,0.,-0.573609800645926));
#87810=DIRECTION('',(-0.000104732033721804,0.999999994335537,1.89770173025207E-5));
#87811=DIRECTION('center_axis',(-0.173648177666902,0.,-0.984807753012213));
#87812=DIRECTION('ref_axis',(-0.984807753012213,0.,0.173648177666902));
#87813=DIRECTION('',(-2.965055618919E-10,-1.,5.228312595822E-11));
#87814=DIRECTION('',(-0.984807721882561,4.36142738440383E-7,0.173648354211293));
#87815=DIRECTION('center_axis',(-0.173648177666902,0.,-0.984807753012213));
#87816=DIRECTION('ref_axis',(-0.984807753012213,0.,0.173648177666902));
#87817=DIRECTION('',(0.000104623869886698,0.999999994344178,-1.91177692657596E-5));
#87818=DIRECTION('',(0.984807722792198,4.31673701686499E-7,-0.1736483490525));
#87819=DIRECTION('',(-9.024447313596E-12,-1.,1.598357449676E-12));
#87820=DIRECTION('center_axis',(-0.173648177666902,6.30659209509215E-17,
-0.984807753012213));
#87821=DIRECTION('ref_axis',(-0.606056619441591,0.788210270758188,0.106864133844497));
#87822=DIRECTION('center_axis',(-0.984807753012213,1.8503717077086E-15,
0.173648177666903));
#87823=DIRECTION('ref_axis',(0.0751084169313687,0.901618518365398,0.425960999443198));
#87824=DIRECTION('center_axis',(-0.984807753012213,1.2335811384724E-15,
0.173648177666903));
#87825=DIRECTION('ref_axis',(-0.0751084169313687,-0.901618518365396,-0.425960999443203));
#87826=DIRECTION('center_axis',(0.,0.,1.));
#87827=DIRECTION('ref_axis',(1.,0.,0.));
#87828=DIRECTION('center_axis',(0.,-1.,0.));
#87829=DIRECTION('ref_axis',(0.984807753012213,0.,-0.173648177666903));
#87830=DIRECTION('center_axis',(0.156564412664908,-0.432532134460022,0.887920907145648));
#87831=DIRECTION('ref_axis',(-0.075108416931378,-0.901618518365421,-0.425960999443147));
#87832=DIRECTION('center_axis',(-0.984807753012213,2.98614490958382E-16,
0.173648177666903));
#87833=DIRECTION('ref_axis',(0.161725191946745,0.364155244606999,0.917189140861908));
#87834=DIRECTION('center_axis',(-0.730811865748475,-0.554283463095025,0.398351427034748));
#87835=DIRECTION('ref_axis',(0.656406878005312,-0.410641643559799,0.632853419902134));
#87836=DIRECTION('center_axis',(0.926024209527167,0.340292288158955,-0.163341121549745));
#87837=DIRECTION('ref_axis',(-0.180419693350444,0.779131598163688,0.600335478706889));
#87838=DIRECTION('center_axis',(0.925983753120755,-0.340399802521857,-0.163346452056609));
#87839=DIRECTION('ref_axis',(-0.173594778761283,0.000353804681334812,-0.984817103633496));
#87840=DIRECTION('center_axis',(-0.695347255811973,0.70213706029504,-0.153283209762188));
#87841=DIRECTION('ref_axis',(0.620272016580331,0.478605536989138,-0.621449406959817));
#87842=DIRECTION('center_axis',(-0.984807753012196,2.8194560172209E-16,
0.173648177666999));
#87843=DIRECTION('ref_axis',(0.156623827406739,0.43181818181821,0.888257864890415));
#87844=DIRECTION('',(0.622150730667944,0.75432770888201,0.209566638428358));
#87845=DIRECTION('center_axis',(0.224487892977242,-0.241948423367666,0.943963000512488));
#87846=DIRECTION('ref_axis',(-0.18733184772302,-0.961334023585974,-0.201850622799835));
#87847=DIRECTION('center_axis',(1.55730139623408E-6,0.999999999997948,1.29560869156906E-6));
#87848=DIRECTION('ref_axis',(0.729105700774769,-2.48721301333868E-7,-0.684401108340475));
#87849=DIRECTION('center_axis',(-0.173648177666901,-9.49857476623745E-16,
-0.984807753012213));
#87850=DIRECTION('ref_axis',(-0.315917116162589,-0.947150125830322,0.0557047112470661));
#87851=DIRECTION('center_axis',(-0.173648177666902,0.,-0.984807753012213));
#87852=DIRECTION('ref_axis',(-0.984807753012213,0.,0.173648177666902));
#87853=DIRECTION('center_axis',(-0.173648177666902,0.,-0.984807753012213));
#87854=DIRECTION('ref_axis',(-0.984807753012213,0.,0.173648177666902));
#87855=DIRECTION('',(-0.622131158824598,0.754172855889872,-0.210181171036981));
#87856=DIRECTION('',(0.174534476450797,-0.00122572414799798,0.984650300426684));
#87857=DIRECTION('center_axis',(-0.0707686828235114,-0.994894683248916,
-0.0719469441634933));
#87858=DIRECTION('ref_axis',(-0.173001180656409,0.0832765703625063,-0.981394724012793));
#87859=DIRECTION('center_axis',(-6.73423872643482E-7,-0.99999999999248,
-3.81917657283092E-6));
#87860=DIRECTION('ref_axis',(0.679405139203387,-3.25989944411653E-6,0.733763352051191));
#87861=DIRECTION('center_axis',(0.938200139829041,-9.39842509682406E-5,
-0.346093179348754));
#87862=DIRECTION('ref_axis',(0.342337059059529,0.147180963465246,0.927977964171518));
#87863=DIRECTION('center_axis',(-2.61574989044999E-8,-1.,-1.99490763817199E-8));
#87864=DIRECTION('ref_axis',(-0.679404928955814,3.24094387247223E-8,-0.733763546730515));
#87865=DIRECTION('center_axis',(-1.,0.,0.));
#87866=DIRECTION('ref_axis',(0.,0.,1.));
#87867=DIRECTION('center_axis',(-1.,0.,0.));
#87868=DIRECTION('ref_axis',(0.,-0.748331477354783,0.663324958071086));
#87869=DIRECTION('center_axis',(-1.,0.,0.));
#87870=DIRECTION('ref_axis',(0.,0.748331477354783,-0.663324958071086));
#87871=DIRECTION('center_axis',(-0.20258578429475,-0.48430305448073,-0.851122524330261));
#87872=DIRECTION('ref_axis',(0.972820028468568,1.76583649998364E-5,-0.231562501063097));
#87873=DIRECTION('center_axis',(-0.224959803675515,-0.646322642471482,-0.729150278446738));
#87874=DIRECTION('ref_axis',(0.955555444304602,4.45507300384497E-7,-0.29481145306727));
#87875=DIRECTION('center_axis',(0.198384291592322,0.861437385015848,0.467513961873302));
#87876=DIRECTION('ref_axis',(-3.79004033482016E-6,0.476995229637716,-0.878905882838714));
#87877=DIRECTION('center_axis',(-0.198384293344405,0.861437385923514,-0.467513959457367));
#87878=DIRECTION('ref_axis',(3.70182108121826E-6,-0.476993894565724,-0.878906607401105));
#87879=DIRECTION('center_axis',(1.,0.,0.));
#87880=DIRECTION('ref_axis',(0.,-1.,0.));
#87881=DIRECTION('center_axis',(-0.224959803616002,0.646322642426279,-0.729150278505167));
#87882=DIRECTION('ref_axis',(7.58238768779224E-7,-0.748331361275018,-0.663325089026266));
#87883=DIRECTION('center_axis',(0.224959803662862,-0.646322642460983,-0.729150278459948));
#87884=DIRECTION('ref_axis',(2.66897615120205E-13,-0.748331477359025,0.663324958066301));
#87885=DIRECTION('center_axis',(0.198384291071427,-0.861437384747512,-0.467513962588771));
#87886=DIRECTION('ref_axis',(5.22391162033877E-6,-0.476993626757997,0.878906752736013));
#87887=DIRECTION('center_axis',(1.,0.,0.));
#87888=DIRECTION('ref_axis',(0.,-1.,0.));
#87889=DIRECTION('center_axis',(0.198384291487557,0.861437384962546,-0.46751396201597));
#87890=DIRECTION('ref_axis',(0.920549900482293,-4.9913569769151E-9,0.390624987324212));
#87891=DIRECTION('center_axis',(0.224959803665131,0.646322642464532,-0.729150278456101));
#87892=DIRECTION('ref_axis',(0.955555562815279,-2.90698700666896E-8,0.294811068945476));
#87893=DIRECTION('center_axis',(0.202585776058526,0.484303048332413,-0.851122529789159));
#87894=DIRECTION('ref_axis',(0.972822293955169,4.34825508932484E-9,0.231552983966525));
#87895=DIRECTION('center_axis',(0.,1.,0.));
#87896=DIRECTION('ref_axis',(-1.,0.,0.));
#87897=DIRECTION('center_axis',(0.,-1.,0.));
#87898=DIRECTION('ref_axis',(-0.972822292136262,0.,-0.231552991608291));
#87899=DIRECTION('center_axis',(0.390624999999987,0.,-0.92054989510347));
#87900=DIRECTION('ref_axis',(0.,-1.,0.));
#87901=DIRECTION('center_axis',(0.,-1.,0.));
#87902=DIRECTION('ref_axis',(-1.,0.,0.));
#87903=DIRECTION('center_axis',(0.390624999999979,0.,0.920549895103474));
#87904=DIRECTION('ref_axis',(-0.920549895103474,0.,0.390624999999979));
#87905=DIRECTION('center_axis',(0.,-1.,0.));
#87906=DIRECTION('ref_axis',(-0.92054989510347,0.,0.390624999999988));
#87907=DIRECTION('center_axis',(0.,-1.,0.));
#87908=DIRECTION('ref_axis',(-1.,0.,0.));
#87909=DIRECTION('',(0.,-1.,0.));
#87910=DIRECTION('center_axis',(0.,1.,0.));
#87911=DIRECTION('ref_axis',(1.,0.,0.));
#87912=DIRECTION('center_axis',(0.,-1.,0.));
#87913=DIRECTION('ref_axis',(0.407236366022499,0.,0.913322802840698));
#87914=DIRECTION('',(0.,-1.,0.));
#87915=DIRECTION('',(0.,-1.,0.));
#87916=DIRECTION('center_axis',(0.,1.,0.));
#87917=DIRECTION('ref_axis',(-0.920549895103471,0.,0.390624999999986));
#87918=DIRECTION('',(0.,-1.,0.));
#87919=DIRECTION('center_axis',(0.,-1.,0.));
#87920=DIRECTION('ref_axis',(-1.,0.,0.));
#87921=DIRECTION('center_axis',(0.,1.,0.));
#87922=DIRECTION('ref_axis',(-0.972822292136262,0.,0.231552991608291));
#87923=DIRECTION('center_axis',(0.,1.,0.));
#87924=DIRECTION('ref_axis',(-1.,0.,0.));
#87925=DIRECTION('center_axis',(0.390624999999987,0.,0.92054989510347));
#87926=DIRECTION('ref_axis',(0.,1.,0.));
#87927=DIRECTION('center_axis',(0.,1.,0.));
#87928=DIRECTION('ref_axis',(-0.92054989510347,0.,-0.390624999999987));
#87929=DIRECTION('center_axis',(0.390624999999991,0.,-0.920549895103469));
#87930=DIRECTION('ref_axis',(-0.920549895103469,0.,-0.390624999999991));
#87931=DIRECTION('center_axis',(0.,1.,0.));
#87932=DIRECTION('ref_axis',(-0.92054989510347,0.,-0.390624999999987));
#87933=DIRECTION('center_axis',(0.,-1.,0.));
#87934=DIRECTION('ref_axis',(-1.,0.,0.));
#87935=DIRECTION('',(2.849630032705E-13,1.,-6.731484522631E-13));
#87936=DIRECTION('center_axis',(0.,-1.,0.));
#87937=DIRECTION('ref_axis',(-1.,0.,0.));
#87938=DIRECTION('center_axis',(0.,1.,0.));
#87939=DIRECTION('ref_axis',(0.407236366022499,0.,-0.913322802840698));
#87940=DIRECTION('',(2.490857672745E-11,-1.,-3.242137599245E-11));
#87941=DIRECTION('',(5.04906701331786E-7,0.999999999999872,-2.70515465025393E-8));
#87942=DIRECTION('',(0.,-1.,0.));
#87943=DIRECTION('center_axis',(0.,-1.,0.));
#87944=DIRECTION('ref_axis',(-0.92054989510347,0.,-0.390624999999987));
#87945=DIRECTION('',(0.,1.,0.));
#87946=DIRECTION('center_axis',(-0.224959803790892,-0.646322642561247,0.729150278331572));
#87947=DIRECTION('ref_axis',(-3.99311694827824E-11,0.748331477256131,0.66332495818238));
#87948=DIRECTION('center_axis',(-0.198384293281608,-0.86143738589211,0.467513959541878));
#87949=DIRECTION('ref_axis',(-8.58600511532262E-6,0.476996080598531,0.878905420975386));
#87950=DIRECTION('center_axis',(0.198384288808409,-0.861437383575475,-0.467513965708642));
#87951=DIRECTION('ref_axis',(5.22459482121113E-6,-0.476993629596688,0.878906751195416));
#87952=DIRECTION('center_axis',(-0.224959800409593,0.646322639913861,0.729150281721439));
#87953=DIRECTION('ref_axis',(0.955555445223718,-4.48148750110284E-7,0.294811450088189));
#87954=DIRECTION('center_axis',(-0.202585784297521,0.484303054482622,0.851122524328525));
#87955=DIRECTION('ref_axis',(0.972820028467264,-1.76583687795184E-5,0.231562501068576));
#87956=DIRECTION('center_axis',(0.202585775073753,-0.48430304759702,0.851122530442007));
#87957=DIRECTION('ref_axis',(0.972822294179919,-4.88508078433452E-9,-0.231552983022287));
#87958=DIRECTION('center_axis',(0.224959803667178,-0.646322642467156,0.729150278453144));
#87959=DIRECTION('ref_axis',(0.955555562814303,2.90703354721545E-8,-0.294811068948639));
#87960=DIRECTION('center_axis',(0.198384289460816,-0.861437383911164,0.467513964813263));
#87961=DIRECTION('ref_axis',(0.920549901087734,2.47085567722425E-9,-0.390624985897424));
#87962=DIRECTION('center_axis',(0.198384289851298,0.861437384113648,0.467513964274471));
#87963=DIRECTION('ref_axis',(-3.78951340993614E-6,0.476995231822333,-0.878905881653092));
#87964=DIRECTION('center_axis',(0.224959803669713,0.646322642466345,0.729150278453081));
#87965=DIRECTION('ref_axis',(-7.87814258274064E-13,0.748331477353354,-0.663324958072698));
#87966=DIRECTION('center_axis',(-1.,0.,0.));
#87967=DIRECTION('ref_axis',(0.,0.,1.));
#87968=DIRECTION('center_axis',(-1.,0.,0.));
#87969=DIRECTION('ref_axis',(0.,0.748331477354783,-0.663324958071086));
#87970=DIRECTION('center_axis',(-1.,0.,0.));
#87971=DIRECTION('ref_axis',(0.,-0.748331477354783,0.663324958071086));
#87972=DIRECTION('center_axis',(1.,0.,0.));
#87973=DIRECTION('ref_axis',(0.,-1.,0.));
#87974=DIRECTION('center_axis',(1.,0.,0.));
#87975=DIRECTION('ref_axis',(0.,-1.,0.));
#87976=DIRECTION('center_axis',(0.,-1.,0.));
#87977=DIRECTION('ref_axis',(-1.,0.,0.));
#87978=DIRECTION('center_axis',(0.,1.,0.));
#87979=DIRECTION('ref_axis',(1.,0.,0.));
#87980=DIRECTION('center_axis',(0.,-1.,0.));
#87981=DIRECTION('ref_axis',(-0.92054989510347,0.,-0.390624999999987));
#87982=DIRECTION('center_axis',(0.913322802840698,0.,0.407236366022499));
#87983=DIRECTION('ref_axis',(0.,-1.,0.));
#87984=DIRECTION('center_axis',(0.,1.,0.));
#87985=DIRECTION('ref_axis',(1.,0.,0.));
#87986=DIRECTION('center_axis',(0.,-1.,0.));
#87987=DIRECTION('ref_axis',(0.407236366022499,0.,-0.913322802840698));
#87988=DIRECTION('center_axis',(0.,-1.,0.));
#87989=DIRECTION('ref_axis',(0.407236366022499,0.,-0.913322802840698));
#87990=DIRECTION('center_axis',(0.,1.,0.));
#87991=DIRECTION('ref_axis',(1.,0.,0.));
#87992=DIRECTION('center_axis',(0.,-1.,0.));
#87993=DIRECTION('ref_axis',(0.916673510305537,0.,0.399636929605016));
#87994=DIRECTION('center_axis',(0.9133228028407,0.,-0.407236366022496));
#87995=DIRECTION('ref_axis',(0.407236366022496,0.,0.9133228028407));
#87996=DIRECTION('center_axis',(0.,-1.,0.));
#87997=DIRECTION('ref_axis',(0.916673510305537,0.,0.399636929605016));
#87998=DIRECTION('center_axis',(0.,1.,0.));
#87999=DIRECTION('ref_axis',(1.,0.,0.));
#88000=DIRECTION('center_axis',(0.,-1.,0.));
#88001=DIRECTION('ref_axis',(0.4072363660225,0.,0.913322802840698));
#88002=DIRECTION('center_axis',(0.,1.,0.));
#88003=DIRECTION('ref_axis',(1.,0.,0.));
#88004=DIRECTION('center_axis',(0.,1.,0.));
#88005=DIRECTION('ref_axis',(1.,0.,0.));
#88006=DIRECTION('center_axis',(0.397580169372953,0.101324582793625,0.91195577625402));
#88007=DIRECTION('ref_axis',(-0.916673679426937,4.1861421552281E-6,0.399636541657988));
#88008=DIRECTION('center_axis',(0.,1.,0.));
#88009=DIRECTION('ref_axis',(1.,0.,0.));
#88010=DIRECTION('center_axis',(0.,1.,0.));
#88011=DIRECTION('ref_axis',(0.407236366022499,0.,0.913322802840698));
#88012=DIRECTION('center_axis',(0.,1.,0.));
#88013=DIRECTION('ref_axis',(1.,0.,0.));
#88014=DIRECTION('center_axis',(0.,1.,0.));
#88015=DIRECTION('ref_axis',(0.916673510305537,0.,-0.399636929605016));
#88016=DIRECTION('center_axis',(-0.397580166491966,0.101324584811521,-0.911955777285825));
#88017=DIRECTION('ref_axis',(-0.916673138003703,9.14519632467006E-6,0.399637783472497));
#88018=DIRECTION('center_axis',(0.,1.,0.));
#88019=DIRECTION('ref_axis',(1.,0.,0.));
#88020=DIRECTION('center_axis',(0.9133228028407,0.,0.407236366022496));
#88021=DIRECTION('ref_axis',(0.407236366022496,0.,-0.9133228028407));
#88022=DIRECTION('center_axis',(0.,1.,0.));
#88023=DIRECTION('ref_axis',(0.916673510305537,0.,-0.399636929605016));
#88024=DIRECTION('center_axis',(0.,1.,0.));
#88025=DIRECTION('ref_axis',(1.,0.,0.));
#88026=DIRECTION('center_axis',(0.,1.,0.));
#88027=DIRECTION('ref_axis',(0.407236366022499,0.,0.913322802840698));
#88028=DIRECTION('center_axis',(0.913322802840698,0.,-0.407236366022499));
#88029=DIRECTION('ref_axis',(0.,1.,0.));
#88030=DIRECTION('center_axis',(0.,1.,0.));
#88031=DIRECTION('ref_axis',(1.,0.,0.));
#88032=DIRECTION('center_axis',(0.,1.,0.));
#88033=DIRECTION('ref_axis',(-0.92054989510347,0.,0.390624999999987));
#88034=DIRECTION('center_axis',(0.,1.,0.));
#88035=DIRECTION('ref_axis',(1.,0.,0.));
#88036=DIRECTION('center_axis',(0.,1.,0.));
#88037=DIRECTION('ref_axis',(0.407236366022499,0.,-0.913322802840698));
#88038=DIRECTION('center_axis',(0.,1.,0.));
#88039=DIRECTION('ref_axis',(1.,0.,0.));
#88040=DIRECTION('center_axis',(-0.173648177666902,0.,-0.984807753012213));
#88041=DIRECTION('ref_axis',(-0.984807753012213,0.,0.173648177666902));
#88042=DIRECTION('center_axis',(0.404936583198885,-0.815730022456604,-0.413050716075109));
#88043=DIRECTION('ref_axis',(-0.853071505689579,-0.499641512218464,0.15042395237648));
#88044=DIRECTION('center_axis',(-0.984807753012213,2.368475785867E-17,0.173648177666902));
#88045=DIRECTION('ref_axis',(0.156623827406651,0.43181818181821,0.888257864890431));
#88046=DIRECTION('center_axis',(-0.822942767980762,0.55434158079449,-0.124380916665012));
#88047=DIRECTION('ref_axis',(0.566224638055893,0.818181846626126,-0.0998404983457853));
#88048=DIRECTION('center_axis',(-0.730772467313229,-0.554341581231179,0.398342832664342));
#88049=DIRECTION('ref_axis',(-0.566224585875474,0.818181842406769,0.0998408288527907));
#88050=DIRECTION('center_axis',(0.601034283802093,0.702059042596753,-0.381930478493975));
#88051=DIRECTION('ref_axis',(0.161931824632277,0.360993841660879,0.918401617188353));
#88052=DIRECTION('center_axis',(-0.984807753012213,2.368475785867E-17,0.173648177666902));
#88053=DIRECTION('ref_axis',(-0.166064467486216,-0.292298435122346,-0.941798395339229));
#88054=DIRECTION('center_axis',(0.201526976551162,0.962806257988152,-0.179974962983743));
#88055=DIRECTION('ref_axis',(0.171766241992109,0.146158578916091,0.974235098896122));
#88056=DIRECTION('center_axis',(-0.601034543449881,0.702058555044682,0.381930966103257));
#88057=DIRECTION('ref_axis',(0.161932171293584,-0.360994252463314,0.918401394592037));
#88058=DIRECTION('center_axis',(-0.984807753012213,2.368475785867E-17,0.173648177666902));
#88059=DIRECTION('ref_axis',(0.156623827406651,0.43181818181821,0.888257864890431));
#88060=DIRECTION('center_axis',(-0.73077246730534,0.554341581255442,0.39834283264505));
#88061=DIRECTION('ref_axis',(0.156623827039417,-0.431818181546998,0.888257865087031));
#88062=DIRECTION('center_axis',(0.822942767728722,0.554341581230101,0.124380916391147));
#88063=DIRECTION('ref_axis',(0.566224639647915,-0.818181842407621,-0.0998405238871412));
#88064=DIRECTION('center_axis',(-0.173648177666902,0.,-0.984807753012213));
#88065=DIRECTION('ref_axis',(-0.984807753012213,0.,0.173648177666902));
#88066=DIRECTION('center_axis',(-0.173648177666902,1.05109872153861E-17,
-0.984807753012213));
#88067=DIRECTION('ref_axis',(0.71842372566634,-0.68397380420233,-0.126677486416051));
#88068=DIRECTION('center_axis',(-0.173648177666903,4.8350541190776E-16,
-0.984807753012213));
#88069=DIRECTION('ref_axis',(-0.718423725666291,0.683973804202383,0.126677486416043));
#88070=DIRECTION('center_axis',(0.173648177666902,0.,0.984807753012213));
#88071=DIRECTION('ref_axis',(0.984807753012213,0.,-0.173648177666902));
#88072=DIRECTION('center_axis',(0.173648177666902,0.,0.984807753012213));
#88073=DIRECTION('ref_axis',(0.984807753012213,0.,-0.173648177666902));
#88074=DIRECTION('center_axis',(0.173648177666902,0.,0.984807753012213));
#88075=DIRECTION('ref_axis',(0.,-1.,0.));
#88076=DIRECTION('center_axis',(0.173648177666902,0.,0.984807753012213));
#88077=DIRECTION('ref_axis',(0.,-1.,0.));
#88078=DIRECTION('center_axis',(0.173648177666902,0.,0.984807753012213));
#88079=DIRECTION('ref_axis',(0.984807753012213,0.,-0.173648177666902));
#88080=DIRECTION('center_axis',(-0.173648177666902,-4.06038199430382E-17,
-0.984807753012213));
#88081=DIRECTION('ref_axis',(1.13553386910767E-16,1.,-6.12527251775702E-17));
#88082=DIRECTION('center_axis',(0.,-1.,0.));
#88083=DIRECTION('ref_axis',(0.173648177666898,0.,0.984807753012214));
#88084=DIRECTION('',(-1.726015970809E-11,-1.,3.043153626436E-12));
#88085=DIRECTION('center_axis',(0.,-1.,0.));
#88086=DIRECTION('ref_axis',(-0.173648177666898,0.,-0.984807753012214));
#88087=DIRECTION('center_axis',(0.,1.,0.));
#88088=DIRECTION('ref_axis',(0.984807678492017,0.,-0.173648600291403));
#88089=DIRECTION('',(2.443314655013E-11,-1.,-4.308252333139E-12));
#88090=DIRECTION('center_axis',(0.173648177666902,0.,0.984807753012213));
#88091=DIRECTION('ref_axis',(0.,-1.,0.));
#88092=DIRECTION('',(3.24463096977915E-7,0.999999999999946,-5.82194489842227E-8));
#88093=DIRECTION('center_axis',(0.920222040575711,0.356178462119004,-0.162259973996103));
#88094=DIRECTION('ref_axis',(0.12376266272234,-0.658093616333623,-0.742694819866687));
#88095=DIRECTION('center_axis',(0.241714278350237,-0.0321281187450775,0.969815442044272));
#88096=DIRECTION('ref_axis',(0.384280518492239,-0.914567435308961,-0.126074935572958));
#88097=DIRECTION('center_axis',(0.118051334199801,-0.733369237422903,0.669502385429205));
#88098=DIRECTION('ref_axis',(0.123762664959406,-0.658093610311519,-0.742694824830021));
#88099=DIRECTION('center_axis',(-1.92083386233814E-10,1.,-2.71332586028924E-11));
#88100=DIRECTION('ref_axis',(0.573562007104527,8.79450586429204E-11,-0.819162147566785));
#88101=DIRECTION('center_axis',(-0.926044070670311,-0.340292292317125,0.163228474739905));
#88102=DIRECTION('ref_axis',(0.374865784447703,-0.779130469521357,0.502425472198452));
#88103=DIRECTION('center_axis',(-0.730732981967633,0.554399311899593,0.398334924441667));
#88104=DIRECTION('ref_axis',(0.656438883269888,0.410464961352669,0.632934837114481));
#88105=DIRECTION('center_axis',(-0.984807753012213,-1.18056891774303E-16,
0.173648177666902));
#88106=DIRECTION('ref_axis',(0.0583004691281475,-0.941955046662688,0.330638390641696));
#88107=DIRECTION('center_axis',(-0.156564412664908,-0.432532134460024,-0.887920907145647));
#88108=DIRECTION('ref_axis',(-0.0751084169313595,0.901618518365421,-0.425960999443152));
#88109=DIRECTION('center_axis',(0.,0.,1.));
#88110=DIRECTION('ref_axis',(1.,0.,0.));
#88111=DIRECTION('center_axis',(0.,1.,0.));
#88112=DIRECTION('ref_axis',(0.173648177666898,0.,0.984807753012214));
#88113=DIRECTION('center_axis',(0.984807753012213,-2.19577442648087E-15,
-0.173648177666901));
#88114=DIRECTION('ref_axis',(-0.0751084169313502,0.901618518365437,-0.425960999443119));
#88115=DIRECTION('center_axis',(0.984807753012213,-2.96059473233375E-15,
-0.173648177666901));
#88116=DIRECTION('ref_axis',(0.0924969807172837,0.846323733445026,0.524576445111539));
#88117=DIRECTION('center_axis',(0.,1.,0.));
#88118=DIRECTION('ref_axis',(-0.81912263281209,0.,-0.573618438001247));
#88119=DIRECTION('center_axis',(-0.173648177666903,3.36351590892355E-16,
-0.984807753012213));
#88120=DIRECTION('ref_axis',(0.636767654207682,-0.762837013608687,-0.112279317879234));
#88121=DIRECTION('center_axis',(0.,-1.,0.));
#88122=DIRECTION('ref_axis',(-0.984807753012214,0.,0.173648177666898));
#88123=DIRECTION('center_axis',(-0.118051264626697,-0.733369608829381,-0.669501990859981));
#88124=DIRECTION('ref_axis',(0.123762305293398,0.65809327391301,-0.742695182843486));
#88125=DIRECTION('center_axis',(0.241762412222673,0.0322470771212345,0.969799495799731));
#88126=DIRECTION('ref_axis',(0.367434395505702,0.921979202041583,-0.122255126690558));
#88127=DIRECTION('center_axis',(-0.926007889327754,0.340399724817355,0.163209730858875));
#88128=DIRECTION('ref_axis',(-0.17347623837402,0.000278443640092277,-0.984838015710573));
#88129=DIRECTION('center_axis',(-0.920222117579503,0.356178256986601,0.162259987573902));
#88130=DIRECTION('ref_axis',(0.123762302773065,0.65809328252365,-0.742695175633689));
#88131=DIRECTION('center_axis',(-5.77150179500071E-11,-1.,-1.59649478822151E-10));
#88132=DIRECTION('ref_axis',(0.573570749823452,9.76712044575835E-11,-0.819156026009065));
#88133=DIRECTION('center_axis',(0.,1.,0.));
#88134=DIRECTION('ref_axis',(0.984807753012213,0.,-0.173648177666903));
#88135=DIRECTION('center_axis',(0.,-1.,0.));
#88136=DIRECTION('ref_axis',(-1.,0.,0.));
#88137=DIRECTION('center_axis',(0.,1.,0.));
#88138=DIRECTION('ref_axis',(1.,0.,0.));
#88139=DIRECTION('center_axis',(0.,1.,0.));
#88140=DIRECTION('ref_axis',(-0.638049918300179,0.,-0.76999500112477));
#88141=DIRECTION('',(1.42678478092006E-6,0.999999999998742,6.93297741290229E-7));
#88142=DIRECTION('center_axis',(0.,1.,0.));
#88143=DIRECTION('ref_axis',(0.353583464998389,0.,-0.935402979084273));
#88144=DIRECTION('center_axis',(0.,1.,0.));
#88145=DIRECTION('ref_axis',(-0.581942537871004,0.,0.813229907600707));
#88146=DIRECTION('center_axis',(-0.950253372983717,2.30324546582274E-6,
-0.311477972138905));
#88147=DIRECTION('ref_axis',(0.311477972127205,-4.36632101694612E-6,-0.950253372980312));
#88148=DIRECTION('center_axis',(0.,-1.,0.));
#88149=DIRECTION('ref_axis',(-1.,0.,0.));
#88150=DIRECTION('',(-1.37512520730395E-6,0.999999999998864,-6.16668900731678E-7));
#88151=DIRECTION('center_axis',(0.,1.,0.));
#88152=DIRECTION('ref_axis',(0.31147569764019,0.,-0.950254118528069));
#88153=DIRECTION('center_axis',(0.,-1.,0.));
#88154=DIRECTION('ref_axis',(-0.173648177666902,0.,-0.984807753012213));
#88155=DIRECTION('center_axis',(0.,1.,0.));
#88156=DIRECTION('ref_axis',(-0.951104406813913,0.,0.308869563633509));
#88157=DIRECTION('center_axis',(0.,-1.,0.));
#88158=DIRECTION('ref_axis',(0.173648177905701,0.,0.984807752970106));
#88159=DIRECTION('center_axis',(-0.173648177666902,0.,-0.984807753012213));
#88160=DIRECTION('ref_axis',(0.,-1.,0.));
#88161=DIRECTION('center_axis',(0.173648177666898,0.,0.984807753012214));
#88162=DIRECTION('ref_axis',(-0.984807753012214,0.,0.173648177666898));
#88163=DIRECTION('center_axis',(-0.173648177666902,0.,-0.984807753012213));
#88164=DIRECTION('ref_axis',(0.,1.,0.));
#88165=DIRECTION('center_axis',(0.,1.,0.));
#88166=DIRECTION('ref_axis',(0.855993839943912,0.,-0.516986021066407));
#88167=DIRECTION('center_axis',(0.,-1.,0.));
#88168=DIRECTION('ref_axis',(-0.984807753012213,0.,0.173648177666903));
#88169=DIRECTION('center_axis',(0.,1.,0.));
#88170=DIRECTION('ref_axis',(-0.638049654090004,0.,-0.769995220060246));
#88171=DIRECTION('center_axis',(0.308869563633505,0.,0.951104406813915));
#88172=DIRECTION('ref_axis',(0.,1.,0.));
#88173=DIRECTION('center_axis',(0.,-1.,0.));
#88174=DIRECTION('ref_axis',(0.91474129068957,0.,0.404040061265687));
#88175=DIRECTION('center_axis',(0.,-1.,0.));
#88176=DIRECTION('ref_axis',(-0.330689828029415,0.,0.943739496703341));
#88177=DIRECTION('center_axis',(0.173648177666901,-9.49857476623745E-16,
0.984807753012213));
#88178=DIRECTION('ref_axis',(-0.315957255971813,0.947136320160717,0.0557117889784327));
#88179=DIRECTION('center_axis',(0.173648177330704,6.22302969527983E-5,0.984807751105318));
#88180=DIRECTION('ref_axis',(0.782059007286606,0.607747668930201,-0.137936507248064));
#88181=DIRECTION('center_axis',(-0.468012284071803,0.720824709793966,0.511249684311236));
#88182=DIRECTION('ref_axis',(-0.526462193329491,-0.69207313268382,0.493834322432033));
#88183=DIRECTION('center_axis',(0.938122107850457,9.54847915278239E-5,-0.346304637053663));
#88184=DIRECTION('ref_axis',(0.342789334776549,-0.142378604065038,0.928560070791299));
#88185=DIRECTION('center_axis',(0.984807753012213,0.,-0.173648177666902));
#88186=DIRECTION('ref_axis',(0.,-1.,0.));
#88187=DIRECTION('center_axis',(0.984807753012213,4.71278345147005E-16,
-0.173648177666903));
#88188=DIRECTION('ref_axis',(0.119983582797752,-0.72289498517529,0.680460711773598));
#88189=DIRECTION('center_axis',(-0.984807753012213,-1.35945676484713E-17,
0.173648177666902));
#88190=DIRECTION('ref_axis',(-0.173356956027276,0.0578907986824709,-0.983156153021921));
#88191=DIRECTION('center_axis',(0.,-1.,0.));
#88192=DIRECTION('ref_axis',(0.819152071792271,0.,0.573576397072291));
#88193=DIRECTION('center_axis',(0.173648177666903,0.,0.984807753012213));
#88194=DIRECTION('ref_axis',(-0.984807753012213,0.,0.173648177666903));
#88195=DIRECTION('center_axis',(-0.984807753012213,-4.67879703234887E-16,
0.173648177666902));
#88196=DIRECTION('ref_axis',(0.00218187333490138,0.999921058430618,0.0123740185769414));
#88197=DIRECTION('center_axis',(-0.984807753012145,-1.27187584978315E-13,
0.17364817766729));
#88198=DIRECTION('ref_axis',(0.172089384615116,-0.133689495210303,0.975967398314721));
#88199=DIRECTION('center_axis',(4.0599214194867E-7,0.999999999999808,4.68423390877839E-7));
#88200=DIRECTION('ref_axis',(-0.984810514839275,3.18491799434328E-7,0.173632513838568));
#88201=DIRECTION('center_axis',(0.984807753012213,-2.13717932240342E-15,
-0.173648177666903));
#88202=DIRECTION('ref_axis',(-0.109429766257892,-0.776448339114791,-0.620607043903487));
#88203=DIRECTION('center_axis',(-0.442012531356003,-0.893567484242663,0.078498874058781));
#88204=DIRECTION('ref_axis',(0.273297331194067,-0.217505218314496,-0.937016568032905));
#88205=DIRECTION('center_axis',(-0.173648177666902,2.91433543964104E-16,
-0.984807753012213));
#88206=DIRECTION('ref_axis',(-0.595306851389017,-0.796612410881215,0.10496865970047));
#88207=DIRECTION('center_axis',(-0.173648177666902,0.,-0.984807753012213));
#88208=DIRECTION('ref_axis',(-0.984807753012213,0.,0.173648177666902));
#88209=DIRECTION('center_axis',(-0.173648177666902,0.,-0.984807753012213));
#88210=DIRECTION('ref_axis',(-0.984807753012213,0.,0.173648177666902));
#88211=DIRECTION('center_axis',(0.173648177666902,0.,0.984807753012213));
#88212=DIRECTION('ref_axis',(-0.984807753012213,-1.01064309961486E-15,0.173648177666902));
#106596=CARTESIAN_POINT('',(0.,0.,0.));
#106597=CARTESIAN_POINT('Origin',(31.9617040371891,10.34163775063,83.3647327807));
#106598=CARTESIAN_POINT('',(32.421019273976,10.3416377503736,81.9367868757674));
#106599=CARTESIAN_POINT('',(33.4389250502851,10.3415988823771,83.1043137625697));
#106600=CARTESIAN_POINT('Origin',(31.9617040310391,10.34163775061,83.36473278179));
#106601=CARTESIAN_POINT('',(32.4699883443439,11.6438812726382,83.90861341978));
#106602=CARTESIAN_POINT('Origin',(31.9617228057091,10.34158590019,83.36483925822));
#106603=CARTESIAN_POINT('',(31.9729372056209,11.0982732621064,82.0695976383883));
#106604=CARTESIAN_POINT('Origin',(31.9617047093191,10.34163562137,83.36473266219));
#106605=CARTESIAN_POINT('Ctrl Pts',(32.4210192738911,10.3416377499008,81.9367868736946));
#106606=CARTESIAN_POINT('Ctrl Pts',(32.3549889539164,10.4466228903284,81.9155474612096));
#106607=CARTESIAN_POINT('Ctrl Pts',(32.2886439073279,10.5550142815435,81.9117786873653));
#106608=CARTESIAN_POINT('Ctrl Pts',(32.1430793277252,10.7979905465623,81.9374456501848));
#106609=CARTESIAN_POINT('Ctrl Pts',(32.050142777925,10.9583234002542,81.9885060907966));
#106610=CARTESIAN_POINT('Ctrl Pts',(31.9729370250153,11.0982734359973,82.0695971663286));
#106611=CARTESIAN_POINT('Origin',(36.3793934194391,111.0724296188,99.78053857024));
#106612=CARTESIAN_POINT('',(33.438915661672,8.83176086632608,83.1042605178143));
#106613=CARTESIAN_POINT('',(33.4389156626291,10.3416377002,83.10426051803));
#106614=CARTESIAN_POINT('',(33.9717701135603,8.83176086676542,86.1262282870246));
#106615=CARTESIAN_POINT('',(30.0527761960508,8.83176086632608,63.9005093315515));
#106616=CARTESIAN_POINT('Origin',(33.6200489988073,9.47404346582926,84.1315187227546));
#106617=CARTESIAN_POINT('Ctrl Pts',(24.1636631729991,13.15706499277,83.51582887991));
#106618=CARTESIAN_POINT('Ctrl Pts',(24.5647380964491,12.88709995962,83.42585917656));
#106619=CARTESIAN_POINT('Ctrl Pts',(25.4508459341791,12.34148054708,83.2280134562701));
#106620=CARTESIAN_POINT('Ctrl Pts',(26.8687546205291,11.61824835454,82.916179282399));
#106621=CARTESIAN_POINT('Ctrl Pts',(28.4012687778591,10.9828277336,82.586899286296));
#106622=CARTESIAN_POINT('Ctrl Pts',(29.9889244426091,10.45524575259,82.256303592466));
#106623=CARTESIAN_POINT('Ctrl Pts',(31.1186113700191,10.16416102927,82.030294447124));
#106624=CARTESIAN_POINT('Ctrl Pts',(31.7224785782191,10.03238128861,81.9125938256419));
#106625=CARTESIAN_POINT('Ctrl Pts',(31.7734801582891,10.0214207908,81.902675068567));
#106626=CARTESIAN_POINT('Ctrl Pts',(24.7567927563091,14.20870211163,82.429604786895));
#106627=CARTESIAN_POINT('Ctrl Pts',(25.1496452921491,13.97393099452,82.369217803208));
#106628=CARTESIAN_POINT('Ctrl Pts',(26.0172627104391,13.5023674652,82.23949810871));
#106629=CARTESIAN_POINT('Ctrl Pts',(27.4045007518391,12.88486233543,82.046577005672));
#106630=CARTESIAN_POINT('Ctrl Pts',(28.9020017624291,12.3485388144,81.8573104046351));
#106631=CARTESIAN_POINT('Ctrl Pts',(30.4496606056791,11.90711756859,81.682769592993));
#106632=CARTESIAN_POINT('Ctrl Pts',(31.5457868459891,11.6648961111,81.574632069656));
#106633=CARTESIAN_POINT('Ctrl Pts',(32.1290979354391,11.55534512451,81.521562061191));
#106634=CARTESIAN_POINT('Ctrl Pts',(32.1783435389591,11.54623433425,81.517112921513));
#106635=CARTESIAN_POINT('Ctrl Pts',(25.7080286493391,15.3150149528,83.14294079435));
#106636=CARTESIAN_POINT('Ctrl Pts',(26.0688989135491,15.0850238123,83.11779004187));
#106637=CARTESIAN_POINT('Ctrl Pts',(26.8689813841791,14.6149583415,83.06541100723));
#106638=CARTESIAN_POINT('Ctrl Pts',(28.1588544048491,13.97195308165,82.99307250027));
#106639=CARTESIAN_POINT('Ctrl Pts',(29.5625282155191,13.3798239155,82.9283215114359));
#106640=CARTESIAN_POINT('Ctrl Pts',(31.0232600341691,12.85540818655,82.874068928702));
#106641=CARTESIAN_POINT('Ctrl Pts',(32.0637075460491,12.53884471205,82.843263250066));
#106642=CARTESIAN_POINT('Ctrl Pts',(32.6188587936791,12.38578792754,82.828526454707));
#106643=CARTESIAN_POINT('Ctrl Pts',(32.6657375309591,12.37297656687,82.827293324418));
#106644=CARTESIAN_POINT('Ctrl Pts',(25.8021387379591,15.06265599365,84.7445289598801));
#106645=CARTESIAN_POINT('Ctrl Pts',(26.1481251487091,14.80092432819,84.71525261791));
#106646=CARTESIAN_POINT('Ctrl Pts',(26.9179060455191,14.25788527696,84.6506238864801));
#106647=CARTESIAN_POINT('Ctrl Pts',(28.1681063763591,13.49072986795,84.54648965191));
#106648=CARTESIAN_POINT('Ctrl Pts',(29.5390059693791,12.75918568124,84.4316840985199));
#106649=CARTESIAN_POINT('Ctrl Pts',(30.9769324167991,12.08864816876,84.30828130528));
#106650=CARTESIAN_POINT('Ctrl Pts',(32.0107143886891,11.66951152981,84.21547396494));
#106651=CARTESIAN_POINT('Ctrl Pts',(32.5660771059891,11.46279434478,84.16380116418));
#106652=CARTESIAN_POINT('Ctrl Pts',(32.6130018292691,11.44545972437,84.15942188772));
#106653=CARTESIAN_POINT('',(31.7476216575109,11.9111986398664,83.9673641909233));
#106654=CARTESIAN_POINT('Ctrl Pts',(31.9729374161714,11.0982730962909,82.0695981250249));
#106655=CARTESIAN_POINT('Ctrl Pts',(31.8773816796382,11.271485744938,82.1699618473536));
#106656=CARTESIAN_POINT('Ctrl Pts',(31.7859691125908,11.4387437257982,82.2941296376232));
#106657=CARTESIAN_POINT('Ctrl Pts',(31.6474513598846,11.7051229822608,82.5594239510954));
#106658=CARTESIAN_POINT('Ctrl Pts',(31.5929885036314,11.8155387095055,82.6976241757693));
#106659=CARTESIAN_POINT('Ctrl Pts',(31.532073047221,11.9664225268417,82.9716240612167));
#106660=CARTESIAN_POINT('Ctrl Pts',(31.51764374752,12.0171944655651,83.1016289408218));
#106661=CARTESIAN_POINT('Ctrl Pts',(31.5267010611325,12.0648278916674,83.3521318330441));
#106662=CARTESIAN_POINT('Ctrl Pts',(31.5440498678541,12.0682904053271,83.4651019787565));
#106663=CARTESIAN_POINT('Ctrl Pts',(31.5950376430365,12.0429521873511,83.6482075907876));
#106664=CARTESIAN_POINT('Ctrl Pts',(31.6203585852615,12.0251659449056,83.7174101258522));
#106665=CARTESIAN_POINT('Ctrl Pts',(31.6790720264413,11.9766646105216,83.8487103915418));
#106666=CARTESIAN_POINT('Ctrl Pts',(31.7121562819556,11.9462064447579,83.910154915883));
#106667=CARTESIAN_POINT('Ctrl Pts',(31.7476258558315,11.9111910957313,83.9673569696238));
#106668=CARTESIAN_POINT('Ctrl Pts',(31.7476216518526,11.9111986410501,83.9673641947199));
#106669=CARTESIAN_POINT('Ctrl Pts',(31.9883196141856,11.8187715270328,83.9478615827402));
#106670=CARTESIAN_POINT('Ctrl Pts',(32.2291184983712,11.7297634578707,83.9280729607192));
#106671=CARTESIAN_POINT('Ctrl Pts',(32.4699886792762,11.6438823126913,83.9086129755005));
#106672=CARTESIAN_POINT('Ctrl Pts',(16.7315271092291,25.77957474242,75.8056538642681));
#106673=CARTESIAN_POINT('Ctrl Pts',(16.8902739491491,25.78276104928,76.726755143248));
#106674=CARTESIAN_POINT('Ctrl Pts',(17.4170423638691,25.68741378017,79.011155596728));
#106675=CARTESIAN_POINT('Ctrl Pts',(18.6971928491291,25.1486541372,82.327981456666));
#106676=CARTESIAN_POINT('Ctrl Pts',(20.3541926191191,24.21296098443,85.29757061493));
#106677=CARTESIAN_POINT('Ctrl Pts',(21.9876235905991,23.12636897321,87.62326197554));
#106678=CARTESIAN_POINT('Ctrl Pts',(23.5303110581191,21.96974605327,89.49482082956));
#106679=CARTESIAN_POINT('Ctrl Pts',(25.0147293345491,20.73535636643,91.08394632963));
#106680=CARTESIAN_POINT('Ctrl Pts',(26.4477039632491,19.42122041898,92.4661164628101));
#106681=CARTESIAN_POINT('Ctrl Pts',(27.8040593501691,18.0525443245,93.66246634875));
#106682=CARTESIAN_POINT('Ctrl Pts',(29.0976297887891,16.61722673478,94.7173081814599));
#106683=CARTESIAN_POINT('Ctrl Pts',(30.3859883571291,15.03805899871,95.692928827));
#106684=CARTESIAN_POINT('Ctrl Pts',(31.6846191544191,13.2490375268,96.6017522016999));
#106685=CARTESIAN_POINT('Ctrl Pts',(32.9283641549091,11.27078505501,97.39922069443));
#106686=CARTESIAN_POINT('Ctrl Pts',(34.0024905191591,9.24026551673301,98.0256740975701));
#106687=CARTESIAN_POINT('Ctrl Pts',(34.8835248980591,7.19980133487202,98.4916705583199));
#106688=CARTESIAN_POINT('Ctrl Pts',(35.5865206621291,5.09129120886101,98.8275149094299));
#106689=CARTESIAN_POINT('Ctrl Pts',(36.0644764908891,2.94897602587201,99.0360923986901));
#106690=CARTESIAN_POINT('Ctrl Pts',(36.2175390832591,1.50759720120401,99.1082321058299));
#106691=CARTESIAN_POINT('Ctrl Pts',(36.2511547877691,0.817200229439614,
99.1309346670101));
#106692=CARTESIAN_POINT('Ctrl Pts',(16.5657307648391,19.34436604072,75.8499470296021));
#106693=CARTESIAN_POINT('Ctrl Pts',(16.7027032210391,19.34727467235,76.647687526976));
#106694=CARTESIAN_POINT('Ctrl Pts',(17.1758927443291,19.26031994756,78.623309386718));
#106695=CARTESIAN_POINT('Ctrl Pts',(18.3744374416091,18.77127275203,81.451029832546));
#106696=CARTESIAN_POINT('Ctrl Pts',(19.9464727370091,17.9342387447,83.90371085737));
#106697=CARTESIAN_POINT('Ctrl Pts',(21.5011129654591,16.97934371574,85.75395997948));
#106698=CARTESIAN_POINT('Ctrl Pts',(22.9701058542891,15.98027083986,87.18714704112));
#106699=CARTESIAN_POINT('Ctrl Pts',(24.3829496628191,14.93205005415,88.35697360021));
#106700=CARTESIAN_POINT('Ctrl Pts',(25.7455828440791,13.83506997747,89.33304121868));
#106701=CARTESIAN_POINT('Ctrl Pts',(27.0338235509591,12.71200151814,90.14134599812));
#106702=CARTESIAN_POINT('Ctrl Pts',(28.2606989614091,11.55431815225,90.82076231519));
#106703=CARTESIAN_POINT('Ctrl Pts',(29.4805515038791,10.30341122855,91.41513380966));
#106704=CARTESIAN_POINT('Ctrl Pts',(30.7073346580191,8.91606547149402,91.92891446662));
#106705=CARTESIAN_POINT('Ctrl Pts',(31.8785519228191,7.42186252822301,92.33283454608));
#106706=CARTESIAN_POINT('Ctrl Pts',(32.8858034194691,5.93611159812901,92.60136415471));
#106707=CARTESIAN_POINT('Ctrl Pts',(33.7077479385191,4.49637949617201,92.75525280737));
#106708=CARTESIAN_POINT('Ctrl Pts',(34.3594477230791,3.06936714330901,92.82352537927));
#106709=CARTESIAN_POINT('Ctrl Pts',(34.7987841186091,1.68933111557601,92.83289655037));
#106710=CARTESIAN_POINT('Ctrl Pts',(34.9379185776691,0.799874261541514,
92.83329103801));
#106711=CARTESIAN_POINT('Ctrl Pts',(34.9680789093591,0.377412282680914,
92.8379453280101));
#106712=CARTESIAN_POINT('Ctrl Pts',(21.0648245475691,14.80356751578,75.088574197736));
#106713=CARTESIAN_POINT('Ctrl Pts',(21.1562893009191,14.80542149402,75.624814594272));
#106714=CARTESIAN_POINT('Ctrl Pts',(21.4915191590391,14.74994267437,76.949273101324));
#106715=CARTESIAN_POINT('Ctrl Pts',(22.4029329257891,14.43645292234,78.850401178621));
#106716=CARTESIAN_POINT('Ctrl Pts',(23.6728411634791,13.89196197301,80.525093828825));
#106717=CARTESIAN_POINT('Ctrl Pts',(24.9938756020691,13.25961078348,81.813737319686));
#106718=CARTESIAN_POINT('Ctrl Pts',(26.2936708744891,12.5864534242,82.832583999374));
#106719=CARTESIAN_POINT('Ctrl Pts',(27.5870975206191,11.86798256843,83.68225710374));
#106720=CARTESIAN_POINT('Ctrl Pts',(28.8717832775691,11.10303997034,84.4077907698501));
#106721=CARTESIAN_POINT('Ctrl Pts',(30.1179515221891,10.306293006,85.0241310085501));
#106722=CARTESIAN_POINT('Ctrl Pts',(31.3323143284891,9.47069299188402,85.55730149859));
#106723=CARTESIAN_POINT('Ctrl Pts',(32.5667384548491,8.55128051724301,86.04034306038));
#106724=CARTESIAN_POINT('Ctrl Pts',(33.8387497469191,7.50960072681501,86.47900335892));
#106725=CARTESIAN_POINT('Ctrl Pts',(35.0880429676691,6.35762147075602,86.85127259704));
#106726=CARTESIAN_POINT('Ctrl Pts',(36.1977391360291,5.17506491544101,87.13119140558));
#106727=CARTESIAN_POINT('Ctrl Pts',(37.1355508905091,3.98655984369701,87.32815521361));
#106728=CARTESIAN_POINT('Ctrl Pts',(37.9083300473991,2.75824145710901,87.46012871543));
#106729=CARTESIAN_POINT('Ctrl Pts',(38.4524854874891,1.51002426311401,87.5351100622101));
#106730=CARTESIAN_POINT('Ctrl Pts',(38.6303209632591,0.670091817760814,
87.56162468684));
#106731=CARTESIAN_POINT('Ctrl Pts',(38.6686985395891,0.267767345835414,
87.57156379687));
#106732=CARTESIAN_POINT('Ctrl Pts',(27.4060955579191,15.00605745049,73.9992175459301));
#106733=CARTESIAN_POINT('Ctrl Pts',(27.4568706345291,15.00674148237,74.299882608077));
#106734=CARTESIAN_POINT('Ctrl Pts',(27.6563153791591,14.98607407549,75.03933020766));
#106735=CARTESIAN_POINT('Ctrl Pts',(28.2552178354491,14.86384274642,76.157719195735));
#106736=CARTESIAN_POINT('Ctrl Pts',(29.1953897033191,14.62223845856,77.28144993045));
#106737=CARTESIAN_POINT('Ctrl Pts',(30.2745666151391,14.3009152899,78.274673456111));
#106738=CARTESIAN_POINT('Ctrl Pts',(31.4158151207291,13.9175608677,79.163166612491));
#106739=CARTESIAN_POINT('Ctrl Pts',(32.6169037455491,13.46553722345,79.992694706598));
#106740=CARTESIAN_POINT('Ctrl Pts',(33.8649399941491,12.93919476597,80.780446952018));
#106741=CARTESIAN_POINT('Ctrl Pts',(35.1214740837291,12.3447503952,81.5213409775531));
#106742=CARTESIAN_POINT('Ctrl Pts',(36.3853570661891,11.67360909312,82.229199358404));
#106743=CARTESIAN_POINT('Ctrl Pts',(37.7082882345091,10.88094645291,82.940678146904));
#106744=CARTESIAN_POINT('Ctrl Pts',(39.1142274982291,9.91205347783502,83.67127064968));
#106745=CARTESIAN_POINT('Ctrl Pts',(40.5432158335391,8.74576233655301,84.3936442258099));
#106746=CARTESIAN_POINT('Ctrl Pts',(41.8604028480391,7.43460302127903,85.0471196915701));
#106747=CARTESIAN_POINT('Ctrl Pts',(43.0163443071791,5.99020112655302,85.6153164434601));
#106748=CARTESIAN_POINT('Ctrl Pts',(44.0066134889891,4.35311312370201,86.1022978834));
#106749=CARTESIAN_POINT('Ctrl Pts',(44.7332634147991,2.52355184883601,86.4665423458501));
#106750=CARTESIAN_POINT('Ctrl Pts',(44.9781481988991,1.19967484028401,86.60065479763));
#106751=CARTESIAN_POINT('Ctrl Pts',(45.0312601718991,0.557056200456914,
86.6358961446099));
#106752=CARTESIAN_POINT('',(33.0354774640918,10.5124754612176,86.002764223517));
#106753=CARTESIAN_POINT('Ctrl Pts',(33.0354780894153,10.5124757937565,86.0027640773287));
#106754=CARTESIAN_POINT('Ctrl Pts',(32.9691045419567,10.6496448112258,85.7569864680321));
#106755=CARTESIAN_POINT('Ctrl Pts',(32.902549203369,10.7855491860502,85.510603787654));
#106756=CARTESIAN_POINT('Ctrl Pts',(32.8358217036925,10.9202489626629,85.2636140420121));
#106757=CARTESIAN_POINT('Ctrl Pts',(32.7745997949839,11.0438348525407,85.0370030685314));
#106758=CARTESIAN_POINT('Ctrl Pts',(32.7132325472932,11.1664063529086,84.8098803739346));
#106759=CARTESIAN_POINT('Ctrl Pts',(32.6517508198401,11.2879736864104,84.582215596186));
#106760=CARTESIAN_POINT('Ctrl Pts',(32.5912567207905,11.40758819008,84.3582079733403));
#106761=CARTESIAN_POINT('Ctrl Pts',(32.5306515604465,11.5262302794122,84.1336755607773));
#106762=CARTESIAN_POINT('Ctrl Pts',(32.4699952977599,11.6438781598893,83.9086117339545));
#106763=CARTESIAN_POINT('Ctrl Pts',(33.0354771921691,10.5124760026091,86.0027648146029));
#106764=CARTESIAN_POINT('Ctrl Pts',(32.8495032264868,10.7349756256776,85.71341610164));
#106765=CARTESIAN_POINT('Ctrl Pts',(32.6612298048798,10.9502089020156,85.4190598393288));
#106766=CARTESIAN_POINT('Ctrl Pts',(32.2322622376353,11.4204983429167,84.7433742626294));
#106767=CARTESIAN_POINT('Ctrl Pts',(31.9898460045153,11.6720717461064,84.3579809310497));
#106768=CARTESIAN_POINT('Ctrl Pts',(31.7476174649718,11.9112061826963,83.967371408625));
#106769=CARTESIAN_POINT('Ctrl Pts',(34.9120188309791,1.82413434249001,99.4682297448801));
#106770=CARTESIAN_POINT('Ctrl Pts',(34.8888109995891,1.96245987573901,99.3366115926799));
#106771=CARTESIAN_POINT('Ctrl Pts',(34.8360618828891,2.26922408414201,99.0374564860999));
#106772=CARTESIAN_POINT('Ctrl Pts',(34.7492177463391,2.74567423970901,98.54493891335));
#106773=CARTESIAN_POINT('Ctrl Pts',(34.6484936587391,3.26480374793701,97.9737042265299));
#106774=CARTESIAN_POINT('Ctrl Pts',(34.5359614399391,3.81065575291701,97.3355022999601));
#106775=CARTESIAN_POINT('Ctrl Pts',(34.4101441832991,4.38332781361301,96.6219571797501));
#106776=CARTESIAN_POINT('Ctrl Pts',(34.2705880299791,4.97863539521901,95.8304949046499));
#106777=CARTESIAN_POINT('Ctrl Pts',(34.1165979297191,5.59573370623801,94.9571736486099));
#106778=CARTESIAN_POINT('Ctrl Pts',(33.9472609320191,6.23487974368301,93.99681581216));
#106779=CARTESIAN_POINT('Ctrl Pts',(33.7618129557691,6.89641662361901,92.9450880759699));
#106780=CARTESIAN_POINT('Ctrl Pts',(33.5583897547991,7.58563568723501,91.79141777467));
#106781=CARTESIAN_POINT('Ctrl Pts',(33.3359577127391,8.30505069308301,90.52994297838));
#106782=CARTESIAN_POINT('Ctrl Pts',(33.1018473233491,9.03167481851102,89.2022369832699));
#106783=CARTESIAN_POINT('Ctrl Pts',(32.8669035260691,9.73654502702002,87.86980449715));
#106784=CARTESIAN_POINT('Ctrl Pts',(32.6426145809191,10.39144635472,86.5977986801901));
#106785=CARTESIAN_POINT('Ctrl Pts',(32.4344532189191,10.98582291601,85.4172569323101));
#106786=CARTESIAN_POINT('Ctrl Pts',(32.2728252408591,11.4384757794,84.5006191187901));
#106787=CARTESIAN_POINT('Ctrl Pts',(32.1812853801191,11.6913539044,83.9814707708001));
#106788=CARTESIAN_POINT('Ctrl Pts',(32.1528289263991,11.76961293267,83.8200862021699));
#106789=CARTESIAN_POINT('Ctrl Pts',(35.8569731920691,1.77503969967301,99.2500041970801));
#106790=CARTESIAN_POINT('Ctrl Pts',(35.8338338435991,1.91295717426201,99.11877443079));
#106791=CARTESIAN_POINT('Ctrl Pts',(35.7812545230591,2.21873308346601,98.82058228613));
#106792=CARTESIAN_POINT('Ctrl Pts',(35.6946777064391,2.69371897512001,98.3295807600601));
#106793=CARTESIAN_POINT('Ctrl Pts',(35.5942347622291,3.21140170079501,97.75994051661));
#106794=CARTESIAN_POINT('Ctrl Pts',(35.4819850014691,3.75588538366201,97.1233404892));
#106795=CARTESIAN_POINT('Ctrl Pts',(35.3564735177891,4.32716670554801,96.41152949362));
#106796=CARTESIAN_POINT('Ctrl Pts',(35.2172185777891,4.92119264231101,95.62177548413));
#106797=CARTESIAN_POINT('Ctrl Pts',(35.0635160609991,5.53714074858301,94.7500851949999));
#106798=CARTESIAN_POINT('Ctrl Pts',(34.8944557496991,6.17524495260401,93.7912965251));
#106799=CARTESIAN_POINT('Ctrl Pts',(34.7092578581891,6.83589212217101,92.74098708999));
#106800=CARTESIAN_POINT('Ctrl Pts',(34.5060627443091,7.52434013691602,91.58861033481));
#106801=CARTESIAN_POINT('Ctrl Pts',(34.2838298479891,8.243112828341,90.32826495015));
#106802=CARTESIAN_POINT('Ctrl Pts',(34.0498859524991,8.96922127464301,89.00150318887));
#106803=CARTESIAN_POINT('Ctrl Pts',(33.8150764760691,9.67368911335601,87.6698324741));
#106804=CARTESIAN_POINT('Ctrl Pts',(33.5908950508691,10.32827676712,86.39843643309));
#106805=CARTESIAN_POINT('Ctrl Pts',(33.3828234160891,10.92239720819,85.21840355359));
#106806=CARTESIAN_POINT('Ctrl Pts',(33.2212636287591,11.37485908179,84.30215246888));
#106807=CARTESIAN_POINT('Ctrl Pts',(33.1297640948691,11.62762578662,83.78323282584));
#106808=CARTESIAN_POINT('Ctrl Pts',(33.1013204765891,11.7058495157,83.62192105062));
#106809=CARTESIAN_POINT('Ctrl Pts',(36.3377183773691,1.23722166550801,98.59992195691));
#106810=CARTESIAN_POINT('Ctrl Pts',(36.3153292400091,1.37066897199701,98.47294684921));
#106811=CARTESIAN_POINT('Ctrl Pts',(36.2646099888591,1.66561834083701,98.1853036822601));
#106812=CARTESIAN_POINT('Ctrl Pts',(36.1809615870791,2.12456363225101,97.710910022));
#106813=CARTESIAN_POINT('Ctrl Pts',(36.0835984897391,2.62639726107801,97.1587364582));
#106814=CARTESIAN_POINT('Ctrl Pts',(35.9744429775691,3.15589135920801,96.53968478651));
#106815=CARTESIAN_POINT('Ctrl Pts',(35.8522811508591,3.71193752772301,95.84687063963));
#106816=CARTESIAN_POINT('Ctrl Pts',(35.7163259182091,4.29192340492101,95.07583020039));
#106817=CARTESIAN_POINT('Ctrl Pts',(35.5657737976391,4.89527134097302,94.22200669614));
#106818=CARTESIAN_POINT('Ctrl Pts',(35.3997445082091,5.52196255221501,93.28040780544));
#106819=CARTESIAN_POINT('Ctrl Pts',(35.2172862249291,6.17286319437901,92.2456354606199));
#106820=CARTESIAN_POINT('Ctrl Pts',(35.0165897410091,6.85286458512201,91.10742914014));
#106821=CARTESIAN_POINT('Ctrl Pts',(34.7965384304091,7.56460090229802,89.85945614293));
#106822=CARTESIAN_POINT('Ctrl Pts',(34.5644184288691,8.28506022851301,88.54303819824));
#106823=CARTESIAN_POINT('Ctrl Pts',(34.3310803995691,8.98512021902701,87.21971247486));
#106824=CARTESIAN_POINT('Ctrl Pts',(34.1080768252691,9.63627166286102,85.9549963582099));
#106825=CARTESIAN_POINT('Ctrl Pts',(33.9009881270591,10.22758637869,84.78053798901));
#106826=CARTESIAN_POINT('Ctrl Pts',(33.7401753499791,10.67795601284,83.8685234099599));
#106827=CARTESIAN_POINT('Ctrl Pts',(33.6491175854391,10.92950214096,83.35210916544));
#106828=CARTESIAN_POINT('Ctrl Pts',(33.6208145758291,11.00733917725,83.1915948215801));
#106829=CARTESIAN_POINT('Ctrl Pts',(36.0275410752391,0.576180127216414,
97.95977740531));
#106830=CARTESIAN_POINT('Ctrl Pts',(36.0060740354391,0.704133072025914,
97.83803177278));
#106831=CARTESIAN_POINT('Ctrl Pts',(35.9576410280591,0.985775351029713,
97.56335453857));
#106832=CARTESIAN_POINT('Ctrl Pts',(35.8775919920991,1.42500486055401,97.1093738962301));
#106833=CARTESIAN_POINT('Ctrl Pts',(35.7840143883591,1.90735808765601,96.5786689334199));
#106834=CARTESIAN_POINT('Ctrl Pts',(35.6786620711491,2.41842822540601,95.9811862522101));
#106835=CARTESIAN_POINT('Ctrl Pts',(35.5606173663291,2.95574860084301,95.31172146382));
#106836=CARTESIAN_POINT('Ctrl Pts',(35.4287178615891,3.51847759563302,94.5636822006001));
#106837=CARTESIAN_POINT('Ctrl Pts',(35.2820379480591,4.10633844242001,93.73181907368));
#106838=CARTESIAN_POINT('Ctrl Pts',(35.1197341405291,4.71900174491701,92.8113484407899));
#106839=CARTESIAN_POINT('Ctrl Pts',(34.9406431575591,5.35792276003501,91.79567300499));
#106840=CARTESIAN_POINT('Ctrl Pts',(34.7430177833691,6.02754225770801,90.6748838132699));
#106841=CARTESIAN_POINT('Ctrl Pts',(34.5256478978791,6.73063004441001,89.44211793354));
#106842=CARTESIAN_POINT('Ctrl Pts',(34.2957696762391,7.44414593846902,88.1384137544699));
#106843=CARTESIAN_POINT('Ctrl Pts',(34.0642402283191,8.13878816578302,86.82534500575));
#106844=CARTESIAN_POINT('Ctrl Pts',(33.8426843711191,8.785716103976,85.5688393007899));
#106845=CARTESIAN_POINT('Ctrl Pts',(33.6368038174091,9.37358225391602,84.4012326595499));
#106846=CARTESIAN_POINT('Ctrl Pts',(33.4769092036691,9.82138028003303,83.49442524359));
#106847=CARTESIAN_POINT('Ctrl Pts',(33.3863944255791,10.07142617598,82.981090428146));
#106848=CARTESIAN_POINT('Ctrl Pts',(33.3582642405291,10.14878792142,82.821556221103));
#106849=CARTESIAN_POINT('Ctrl Pts',(33.0354776265489,10.5124749757193,86.0027637457613));
#106850=CARTESIAN_POINT('Ctrl Pts',(33.3173179037196,10.1752792325235,86.4412617191918));
#106851=CARTESIAN_POINT('Ctrl Pts',(33.5525634430571,9.85417994660021,86.750215496027));
#106852=CARTESIAN_POINT('Ctrl Pts',(33.772028026241,9.50836650597176,86.9414312064967));
#106853=CARTESIAN_POINT('Ctrl Pts',(33.8248976959827,9.42095261698334,86.9789367692075));
#106854=CARTESIAN_POINT('Ctrl Pts',(33.9013819844101,9.28133355483486,87.0015489199111));
#106855=CARTESIAN_POINT('Ctrl Pts',(33.9294254915404,9.22693873504601,87.0021052933605));
#106856=CARTESIAN_POINT('Ctrl Pts',(33.9721748577027,9.13459135675974,86.9784254921267));
#106857=CARTESIAN_POINT('Ctrl Pts',(33.9877318762359,9.09759012230128,86.9609410997307));
#106858=CARTESIAN_POINT('Ctrl Pts',(34.0126495147909,9.02972409352531,86.9096124910328));
#106859=CARTESIAN_POINT('Ctrl Pts',(34.0212542780569,9.00101992606884,86.8775770431024));
#106860=CARTESIAN_POINT('Ctrl Pts',(34.0348285005369,8.94246589968673,86.7903234150622));
#106861=CARTESIAN_POINT('Ctrl Pts',(34.0368443275895,8.91728874581814,86.7317483654917));
#106862=CARTESIAN_POINT('Ctrl Pts',(34.0324568799591,8.84706856689204,86.5120214361058));
#106863=CARTESIAN_POINT('Ctrl Pts',(34.0047398726329,8.83176059863746,86.313208346417));
#106864=CARTESIAN_POINT('Ctrl Pts',(33.9717701135441,8.83176086632613,86.1262282870275));
#106865=CARTESIAN_POINT('Origin',(31.9617040310391,11.38539957172,83.36473278179));
#106866=CARTESIAN_POINT('Ctrl Pts',(33.4389156605574,8.83176086632183,83.1042605152897));
#106867=CARTESIAN_POINT('Ctrl Pts',(33.4217631809711,8.83176086595217,83.0069839686339));
#106868=CARTESIAN_POINT('Ctrl Pts',(33.3959952397706,8.85207982387865,82.9165557092094));
#106869=CARTESIAN_POINT('Ctrl Pts',(33.3323712217024,8.92179561683953,82.7488570392455));
#106870=CARTESIAN_POINT('Ctrl Pts',(33.2944921671943,8.97119818785721,82.6715977317027));
#106871=CARTESIAN_POINT('Ctrl Pts',(33.1692793088435,9.14763475437354,82.4599992368818));
#106872=CARTESIAN_POINT('Ctrl Pts',(33.0701990377864,9.30262812111028,82.3460559650253));
#106873=CARTESIAN_POINT('Ctrl Pts',(32.8081714962699,9.71888469733861,82.1057109973505));
#106874=CARTESIAN_POINT('Ctrl Pts',(32.6191364880251,10.026640586823,82.0005135599871));
#106875=CARTESIAN_POINT('Ctrl Pts',(32.4210192740185,10.34163775061,81.9367868768039));
#106876=CARTESIAN_POINT('Origin',(11.833832765324,1.4210854715202E-14,67.1130006183894));
#106877=CARTESIAN_POINT('Origin',(31.9617040240391,-10.34163791147,83.36473278302));
#106878=CARTESIAN_POINT('',(31.9729369794551,-11.0982737000556,82.0695978531518));
#106879=CARTESIAN_POINT('',(32.4699922398292,-11.64390462692,83.9085557935526));
#106880=CARTESIAN_POINT('Origin',(31.9617042108291,-10.34163673913,83.36473275008));
#106881=CARTESIAN_POINT('',(33.4389248775025,-10.3415989969539,83.1043127923001));
#106882=CARTESIAN_POINT('Origin',(31.9617224686691,-10.34158709855,83.3648373468));
#106883=CARTESIAN_POINT('',(32.4210191725084,-10.3416379115649,81.9367868456364));
#106884=CARTESIAN_POINT('Origin',(31.9617040310391,-10.34163791149,83.36473278179));
#106885=CARTESIAN_POINT('Ctrl Pts',(31.9729367628468,-11.0982738819268,
82.069597333042));
#106886=CARTESIAN_POINT('Ctrl Pts',(32.0501425538371,-10.9583237686893,
81.9885061566232));
#106887=CARTESIAN_POINT('Ctrl Pts',(32.1430791794419,-10.7979907825697,
81.9374456442463));
#106888=CARTESIAN_POINT('Ctrl Pts',(32.2886438200371,-10.5550144197122,
81.9117786706722));
#106889=CARTESIAN_POINT('Ctrl Pts',(32.3549888593241,-10.446623041826,81.9155474419251));
#106890=CARTESIAN_POINT('Ctrl Pts',(32.4210191729779,-10.3416379122948,
81.9367868477846));
#106891=CARTESIAN_POINT('Ctrl Pts',(31.7735817980591,-10.02140058805,81.9026562156629));
#106892=CARTESIAN_POINT('Ctrl Pts',(31.7357761748391,-10.02952473272,81.910008510489));
#106893=CARTESIAN_POINT('Ctrl Pts',(31.1628542188291,-10.15405062092,82.0216114688509));
#106894=CARTESIAN_POINT('Ctrl Pts',(30.0808930105491,-10.42968733766,82.237676912063));
#106895=CARTESIAN_POINT('Ctrl Pts',(28.5280497869291,-10.93691556809,82.56013369893));
#106896=CARTESIAN_POINT('Ctrl Pts',(26.9921340261691,-11.56119523671,82.889318848888));
#106897=CARTESIAN_POINT('Ctrl Pts',(25.5251460669191,-12.29779125652,83.21142902479));
#106898=CARTESIAN_POINT('Ctrl Pts',(24.5918694655791,-12.86877044185,83.41980202981));
#106899=CARTESIAN_POINT('Ctrl Pts',(24.1635532058191,-13.15708445208,83.5158789747301));
#106900=CARTESIAN_POINT('Ctrl Pts',(32.1784416282891,-11.54621773089,81.5171042031791));
#106901=CARTESIAN_POINT('Ctrl Pts',(32.1419378425891,-11.55297077673,81.5204020721341));
#106902=CARTESIAN_POINT('Ctrl Pts',(31.5885791824291,-11.65648792141,81.57065409752));
#106903=CARTESIAN_POINT('Ctrl Pts',(30.5390466775791,-11.88582952014,81.673590761524));
#106904=CARTESIAN_POINT('Ctrl Pts',(29.0257581845491,-12.31002881764,81.8426957379871));
#106905=CARTESIAN_POINT('Ctrl Pts',(27.5251181140391,-12.83644124757,82.0304770381));
#106906=CARTESIAN_POINT('Ctrl Pts',(26.0900655677491,-13.46474790953,82.2287773907151));
#106907=CARTESIAN_POINT('Ctrl Pts',(25.1761650785191,-13.9579744701,82.365120608326));
#106908=CARTESIAN_POINT('Ctrl Pts',(24.7566393447891,-14.20870689459,82.429615994405));
#106909=CARTESIAN_POINT('Ctrl Pts',(32.6658315200591,-12.37295378417,82.827290215174));
#106910=CARTESIAN_POINT('Ctrl Pts',(32.6310822289791,-12.38244981272,82.828204304523));
#106911=CARTESIAN_POINT('Ctrl Pts',(32.1044073017791,-12.52731765498,82.842152237755));
#106912=CARTESIAN_POINT('Ctrl Pts',(31.1079834548191,-12.82839202105,82.87139447125));
#106913=CARTESIAN_POINT('Ctrl Pts',(29.6790572130991,-13.33539347479,82.923631504117));
#106914=CARTESIAN_POINT('Ctrl Pts',(28.2714383294591,-13.9202137689,82.987255072456));
#106915=CARTESIAN_POINT('Ctrl Pts',(26.9362729380191,-14.57705521407,83.0612022033301));
#106916=CARTESIAN_POINT('Ctrl Pts',(26.0932368319491,-15.06943775184,83.11603253511));
#106917=CARTESIAN_POINT('Ctrl Pts',(25.7078677337091,-15.3150566876,83.14290604076));
#106918=CARTESIAN_POINT('Ctrl Pts',(32.6130962564491,-11.44542862336,84.15941229294));
#106919=CARTESIAN_POINT('Ctrl Pts',(32.5783126975491,-11.4582774734,84.16265859895));
#106920=CARTESIAN_POINT('Ctrl Pts',(32.0513526705791,-11.65402869693,84.21172884833));
#106921=CARTESIAN_POINT('Ctrl Pts',(31.0608695313391,-12.05322295219,84.30085784711));
#106922=CARTESIAN_POINT('Ctrl Pts',(29.6533377532591,-12.70307541124,84.4220131092));
#106923=CARTESIAN_POINT('Ctrl Pts',(28.2776481946291,-13.42796087265,84.53734029307));
#106924=CARTESIAN_POINT('Ctrl Pts',(26.9827128612591,-14.21370720002,84.6452557772899));
#106925=CARTESIAN_POINT('Ctrl Pts',(26.1714980327591,-14.78323258141,84.71322528326));
#106926=CARTESIAN_POINT('Ctrl Pts',(25.8020155523191,-15.06273876079,84.74449966846));
#106927=CARTESIAN_POINT('',(31.7476734280839,-11.9111478604859,83.9674490301228));
#106928=CARTESIAN_POINT('Ctrl Pts',(31.747677586831,-11.9111403866478,83.9674418750385));
#106929=CARTESIAN_POINT('Ctrl Pts',(31.7122146011112,-11.9461515111606,
83.9102588915761));
#106930=CARTESIAN_POINT('Ctrl Pts',(31.6791349693868,-11.9766086818139,
83.8488354653028));
#106931=CARTESIAN_POINT('Ctrl Pts',(31.6204251122535,-12.0251166490527,
83.71758176436));
#106932=CARTESIAN_POINT('Ctrl Pts',(31.5951025357537,-12.0429110201326,
83.6484034469622));
#106933=CARTESIAN_POINT('Ctrl Pts',(31.5440974535816,-12.0682846266406,
83.4653474362906));
#106934=CARTESIAN_POINT('Ctrl Pts',(31.5267301910395,-12.0648516576147,
83.3523970290102));
#106935=CARTESIAN_POINT('Ctrl Pts',(31.5176271818919,-12.0172908463836,
83.1019371589877));
#106936=CARTESIAN_POINT('Ctrl Pts',(31.5320257410619,-11.9665665931259,
82.9719537520677));
#106937=CARTESIAN_POINT('Ctrl Pts',(31.5928693301599,-11.8157968166564,
82.6979996654286));
#106938=CARTESIAN_POINT('Ctrl Pts',(31.6472844110669,-11.7054576729801,
82.5598219677352));
#106939=CARTESIAN_POINT('Ctrl Pts',(31.7857998765308,-11.4390530565216,
82.2943601436417));
#106940=CARTESIAN_POINT('Ctrl Pts',(31.8772946926597,-11.271643725901,82.1700543601994));
#106941=CARTESIAN_POINT('Ctrl Pts',(31.9729371943684,-11.0982735071633,
82.0695983906671));
#106942=CARTESIAN_POINT('Ctrl Pts',(32.4699845397491,-11.64392959724,83.90850213227));
#106943=CARTESIAN_POINT('Ctrl Pts',(32.2291347908734,-11.7297341943093,
83.9281305264186));
#106944=CARTESIAN_POINT('Ctrl Pts',(31.9883508873569,-11.8187156032077,
83.9479776127812));
#106945=CARTESIAN_POINT('Ctrl Pts',(31.7476734278368,-11.9111478582041,
83.9674490379002));
#106946=CARTESIAN_POINT('Origin',(36.3793934194391,111.0724296188,99.78053857024));
#106947=CARTESIAN_POINT('',(33.9717729269383,-8.83176086632605,86.1262442425792));
#106948=CARTESIAN_POINT('Origin',(33.6121664459681,-9.4442782170463,84.0868145463581));
#106949=CARTESIAN_POINT('',(33.4389156594987,-8.83176086632605,83.1042605136998));
#106950=CARTESIAN_POINT('',(30.0527761960508,-8.83176086632605,63.9005093315515));
#106951=CARTESIAN_POINT('',(33.4389156626291,10.3416377002,83.10426051803));
#106952=CARTESIAN_POINT('Ctrl Pts',(32.1527935626691,-11.76968665633,83.8199367020899));
#106953=CARTESIAN_POINT('Ctrl Pts',(32.1877822675091,-11.67346394932,84.01836750773));
#106954=CARTESIAN_POINT('Ctrl Pts',(32.2841012636091,-11.40711317747,84.5646196792199));
#106955=CARTESIAN_POINT('Ctrl Pts',(32.4466951508991,-10.95100845184,85.48673543616));
#106956=CARTESIAN_POINT('Ctrl Pts',(32.6453419112291,-10.38330562976,86.61331719654));
#106957=CARTESIAN_POINT('Ctrl Pts',(32.8601514696091,-9.75625684908599,
87.83156273969));
#106958=CARTESIAN_POINT('Ctrl Pts',(33.0925703565391,-9.05996744084198,
89.1496757476299));
#106959=CARTESIAN_POINT('Ctrl Pts',(33.3361679293591,-8.30506871146998,
90.5311862337));
#106960=CARTESIAN_POINT('Ctrl Pts',(33.5787157856791,-7.51970410304498,
91.90674348165));
#106961=CARTESIAN_POINT('Ctrl Pts',(33.8058023593191,-6.74443968379098,
93.19461543817));
#106962=CARTESIAN_POINT('Ctrl Pts',(34.0112736614491,-5.99939457948999,
94.35990109842));
#106963=CARTESIAN_POINT('Ctrl Pts',(34.1938753301091,-5.29221424379899,
95.39548662213));
#106964=CARTESIAN_POINT('Ctrl Pts',(34.3549807040891,-4.62437962601499,
96.3091606005901));
#106965=CARTESIAN_POINT('Ctrl Pts',(34.4968257910291,-3.99387220682299,
97.11360406338));
#106966=CARTESIAN_POINT('Ctrl Pts',(34.6214195941091,-3.39980514907699,
97.8202106336001));
#106967=CARTESIAN_POINT('Ctrl Pts',(34.7311021597591,-2.84190083195199,
98.44225137414));
#106968=CARTESIAN_POINT('Ctrl Pts',(34.8268721630791,-2.32213954720699,
98.98539005283));
#106969=CARTESIAN_POINT('Ctrl Pts',(34.8855200472191,-1.98268592649499,
99.31799873191));
#106970=CARTESIAN_POINT('Ctrl Pts',(34.9121603553391,-1.82376272593199,
99.469083427));
#106971=CARTESIAN_POINT('Ctrl Pts',(33.1013825708891,-11.70592189092,83.62175380312));
#106972=CARTESIAN_POINT('Ctrl Pts',(33.1363554891591,-11.6097425978,83.82009507874));
#106973=CARTESIAN_POINT('Ctrl Pts',(33.2326322715791,-11.34350858072,84.36610784449));
#106974=CARTESIAN_POINT('Ctrl Pts',(33.3951576120491,-10.8875961498,85.28783485311));
#106975=CARTESIAN_POINT('Ctrl Pts',(33.5937184049891,-10.32013893385,86.4139290682));
#106976=CARTESIAN_POINT('Ctrl Pts',(33.8084250678791,-9.69339027966398,
87.63159106202));
#106977=CARTESIAN_POINT('Ctrl Pts',(34.0407123335591,-8.99749464293698,
88.94895760882));
#106978=CARTESIAN_POINT('Ctrl Pts',(34.2841385092591,-8.24312584709699,
90.32949605346));
#106979=CARTESIAN_POINT('Ctrl Pts',(34.5264675374691,-7.45846750889399,
91.70381226553));
#106980=CARTESIAN_POINT('Ctrl Pts',(34.7532919425091,-6.68409523848699,
92.99019739006));
#106981=CARTESIAN_POINT('Ctrl Pts',(34.9584686160591,-5.94011501678899,
94.15381212856));
#106982=CARTESIAN_POINT('Ctrl Pts',(35.1407525862991,-5.23416156772599,
95.18759589499));
#106983=CARTESIAN_POINT('Ctrl Pts',(35.3015331683191,-4.56766984296199,
96.09942788677));
#106984=CARTESIAN_POINT('Ctrl Pts',(35.4430462540291,-3.93863492368899,
96.90198847698));
#106985=CARTESIAN_POINT('Ctrl Pts',(35.5673227817091,-3.34607958808899,
97.60679568904));
#106986=CARTESIAN_POINT('Ctrl Pts',(35.6767165726691,-2.78964237687799,
98.22719870685));
#106987=CARTESIAN_POINT('Ctrl Pts',(35.7721962938191,-2.27145287258899,
98.76869111359));
#106988=CARTESIAN_POINT('Ctrl Pts',(35.8306532491991,-1.93310428852799,
99.10021698185));
#106989=CARTESIAN_POINT('Ctrl Pts',(35.8572087491291,-1.77468696691499,
99.2508207058));
#106990=CARTESIAN_POINT('Ctrl Pts',(33.6208806990891,-11.00730786661,83.19137758022));
#106991=CARTESIAN_POINT('Ctrl Pts',(33.6556806580191,-10.91160422097,83.38873795465));
#106992=CARTESIAN_POINT('Ctrl Pts',(33.7514949424591,-10.64664938247,83.93212776405));
#106993=CARTESIAN_POINT('Ctrl Pts',(33.9132692761891,-10.19284375433,84.8495956017999));
#106994=CARTESIAN_POINT('Ctrl Pts',(34.1108882006291,-9.62807742703399,
85.97034821521));
#106995=CARTESIAN_POINT('Ctrl Pts',(34.3244675288191,-9.00461699282098,
87.1816167761799));
#106996=CARTESIAN_POINT('Ctrl Pts',(34.5553127372291,-8.31303556163099,
88.49080500981));
#106997=CARTESIAN_POINT('Ctrl Pts',(34.7968610664691,-7.56447277785898,
89.86069365796));
#106998=CARTESIAN_POINT('Ctrl Pts',(35.0367925890191,-6.78755241657298,
91.22141293976));
#106999=CARTESIAN_POINT('Ctrl Pts',(35.2607446450891,-6.02295463041499,
92.49150816386));
#107000=CARTESIAN_POINT('Ctrl Pts',(35.4626933343091,-5.29064138366899,
93.63681609352));
#107001=CARTESIAN_POINT('Ctrl Pts',(35.6414965645091,-4.59812984409599,
94.6508596022301));
#107002=CARTESIAN_POINT('Ctrl Pts',(35.7987186889691,-3.94635100803099,
95.54251057833));
#107003=CARTESIAN_POINT('Ctrl Pts',(35.9365943313691,-3.33344896539199,
96.3244422024101));
#107004=CARTESIAN_POINT('Ctrl Pts',(36.0573947537591,-2.75745622962399,
97.00953544173));
#107005=CARTESIAN_POINT('Ctrl Pts',(36.1636246962091,-2.21709279770699,
97.61199538306));
#107006=CARTESIAN_POINT('Ctrl Pts',(36.2559240529591,-1.71612389891399,
98.13545104697));
#107007=CARTESIAN_POINT('Ctrl Pts',(36.3122891710791,-1.38988222212499,
98.45511351659));
#107008=CARTESIAN_POINT('Ctrl Pts',(36.3379155028391,-1.23700736783499,
98.60044766601));
#107009=CARTESIAN_POINT('Ctrl Pts',(33.3581861538791,-10.14869107751,82.821333853779));
#107010=CARTESIAN_POINT('Ctrl Pts',(33.3927735407891,-10.05357201637,83.01748867236));
#107011=CARTESIAN_POINT('Ctrl Pts',(33.4880194018791,-9.79018932523798,
83.55765479273));
#107012=CARTESIAN_POINT('Ctrl Pts',(33.6488707266591,-9.33897301848499,
84.4698879866199));
#107013=CARTESIAN_POINT('Ctrl Pts',(33.8453320675491,-8.77751387096399,
85.5840756174799));
#107014=CARTESIAN_POINT('Ctrl Pts',(34.0575258688491,-8.15809475395498,
86.78748646502));
#107015=CARTESIAN_POINT('Ctrl Pts',(34.2865987472891,-7.47181560582498,
88.0866233158599));
#107016=CARTESIAN_POINT('Ctrl Pts',(34.5258391490491,-6.73038857837198,
89.44342305689));
#107017=CARTESIAN_POINT('Ctrl Pts',(34.7628240679791,-5.96297841393798,
90.7874313191499));
#107018=CARTESIAN_POINT('Ctrl Pts',(34.9832459243291,-5.21039375089199,
92.03750578569));
#107019=CARTESIAN_POINT('Ctrl Pts',(35.1812273276891,-4.49241955292199,
93.16031411919));
#107020=CARTESIAN_POINT('Ctrl Pts',(35.3557526279591,-3.81642850787699,
94.15009628172));
#107021=CARTESIAN_POINT('Ctrl Pts',(35.5086013054291,-3.18273223645299,
95.01694420737));
#107022=CARTESIAN_POINT('Ctrl Pts',(35.6420064250591,-2.58965796458799,
95.77352223697));
#107023=CARTESIAN_POINT('Ctrl Pts',(35.7585346137691,-2.03402114180199,
96.4343864351));
#107024=CARTESIAN_POINT('Ctrl Pts',(35.8608760951491,-1.51341284832599,
97.01479381783));
#107025=CARTESIAN_POINT('Ctrl Pts',(35.9492666922991,-1.03360857045599,
97.51608180449));
#107026=CARTESIAN_POINT('Ctrl Pts',(36.0030608820791,-0.722246631958186,
97.82116381497));
#107027=CARTESIAN_POINT('Ctrl Pts',(36.0275452393591,-0.576183629892886,
97.9600215052599));
#107028=CARTESIAN_POINT('',(33.0354798288136,-10.5124724840881,86.0027674120725));
#107029=CARTESIAN_POINT('Ctrl Pts',(33.9717729269291,-8.83176086634574,
86.1262442425808));
#107030=CARTESIAN_POINT('Ctrl Pts',(34.00452240054,-8.83176153466786,86.3119775742192));
#107031=CARTESIAN_POINT('Ctrl Pts',(34.0320451313447,-8.84686882170987,
86.5091543621162));
#107032=CARTESIAN_POINT('Ctrl Pts',(34.0369090716926,-8.91605932710747,
86.7286962704357));
#107033=CARTESIAN_POINT('Ctrl Pts',(34.0350299303198,-8.94118685479987,
86.7878948736568));
#107034=CARTESIAN_POINT('Ctrl Pts',(34.0216294684122,-8.99967893519797,
86.8759322099713));
#107035=CARTESIAN_POINT('Ctrl Pts',(34.0131139926901,-9.02830243620887,
86.9082308063866));
#107036=CARTESIAN_POINT('Ctrl Pts',(33.9883890414468,-9.09594990342112,
86.959993287345));
#107037=CARTESIAN_POINT('Ctrl Pts',(33.9729527871185,-9.13279899518379,
86.9777020439548));
#107038=CARTESIAN_POINT('Ctrl Pts',(33.9305535618018,-9.22464467891043,
87.0018535956066));
#107039=CARTESIAN_POINT('Ctrl Pts',(33.9027796998228,-9.27865799813915,
87.0016595140628));
#107040=CARTESIAN_POINT('Ctrl Pts',(33.826939384157,-9.41742371476679,86.9800230277075));
#107041=CARTESIAN_POINT('Ctrl Pts',(33.7745078388006,-9.50429852151224,
86.9432471052056));
#107042=CARTESIAN_POINT('Ctrl Pts',(33.5552084117402,-9.85055375321946,
86.753681284039));
#107043=CARTESIAN_POINT('Ctrl Pts',(33.3189371657181,-10.1733419857233,
86.4437816445647));
#107044=CARTESIAN_POINT('Ctrl Pts',(33.0354799802535,-10.5124720315184,
86.0027669667207));
#107045=CARTESIAN_POINT('Ctrl Pts',(32.4699982866135,-11.6439041840734,
83.9085524108676));
#107046=CARTESIAN_POINT('Ctrl Pts',(32.5078283245398,-11.5705218613496,
84.0489368478963));
#107047=CARTESIAN_POINT('Ctrl Pts',(32.5456303929192,-11.4967563984524,
84.189108156906));
#107048=CARTESIAN_POINT('Ctrl Pts',(32.5833984613449,-11.4226113402587,
84.3290758031173));
#107049=CARTESIAN_POINT('Ctrl Pts',(32.6746058513949,-11.2435559232135,
84.6670884215676));
#107050=CARTESIAN_POINT('Ctrl Pts',(32.7656155737303,-11.0622855248061,
85.0039134635798));
#107051=CARTESIAN_POINT('Ctrl Pts',(32.8563236438861,-10.8787683159464,
85.3396126365442));
#107052=CARTESIAN_POINT('Ctrl Pts',(32.916185525905,-10.7576579727725,85.56115394209));
#107053=CARTESIAN_POINT('Ctrl Pts',(32.9759158306451,-10.6355694329657,
85.7822048579121));
#107054=CARTESIAN_POINT('Ctrl Pts',(33.0354799802617,-10.5124720315087,
86.0027669667333));
#107055=CARTESIAN_POINT('Ctrl Pts',(36.2511910984291,-0.816951121684487,
99.13095237507));
#107056=CARTESIAN_POINT('Ctrl Pts',(36.2200982088991,-1.45683196280799,
99.1098451401801));
#107057=CARTESIAN_POINT('Ctrl Pts',(36.0778630790891,-2.85039942836099,
99.0419676728901));
#107058=CARTESIAN_POINT('Ctrl Pts',(35.6275483510391,-4.94247000735899,
98.84599903898));
#107059=CARTESIAN_POINT('Ctrl Pts',(34.9397597871691,-7.05113172994599,
98.51977184372));
#107060=CARTESIAN_POINT('Ctrl Pts',(34.0734741662491,-9.09163743804897,
98.0649602571899));
#107061=CARTESIAN_POINT('Ctrl Pts',(33.0099168483791,-11.12983443612,97.44906592845));
#107062=CARTESIAN_POINT('Ctrl Pts',(31.7699785170891,-13.12298748389,96.6589115129399));
#107063=CARTESIAN_POINT('Ctrl Pts',(30.4746258290591,-14.92251334854,95.75721789378));
#107064=CARTESIAN_POINT('Ctrl Pts',(29.1968815731991,-16.50069944243,94.7947864407199));
#107065=CARTESIAN_POINT('Ctrl Pts',(27.9225293421991,-17.92619343051,93.76208048801));
#107066=CARTESIAN_POINT('Ctrl Pts',(26.5896727465691,-19.28349187111,92.5956876894801));
#107067=CARTESIAN_POINT('Ctrl Pts',(25.1814694175691,-20.58838494568,91.25117303266));
#107068=CARTESIAN_POINT('Ctrl Pts',(23.7249591534991,-21.81419974781,89.71266771848));
#107069=CARTESIAN_POINT('Ctrl Pts',(22.2142909846591,-22.9637208008,87.91364117654));
#107070=CARTESIAN_POINT('Ctrl Pts',(20.6065395382091,-24.05476593901,85.68623624305));
#107071=CARTESIAN_POINT('Ctrl Pts',(18.9416778012191,-25.02348229969,82.825890425796));
#107072=CARTESIAN_POINT('Ctrl Pts',(17.5339994345191,-25.65356630387,79.417420667109));
#107073=CARTESIAN_POINT('Ctrl Pts',(16.9242179391691,-25.78353110717,76.926255793732));
#107074=CARTESIAN_POINT('Ctrl Pts',(16.7312453442491,-25.77964745785,75.805602355198));
#107075=CARTESIAN_POINT('Ctrl Pts',(34.9680768531591,-0.377262712455286,
92.83793248162));
#107076=CARTESIAN_POINT('Ctrl Pts',(34.9401900659091,-0.768818210978587,
92.83356221903));
#107077=CARTESIAN_POINT('Ctrl Pts',(34.8109275223991,-1.62812620872499,
92.8325719567701));
#107078=CARTESIAN_POINT('Ctrl Pts',(34.3972755661991,-2.97122279462399,
92.8255990532501));
#107079=CARTESIAN_POINT('Ctrl Pts',(33.7599966114291,-4.39375486831299,
92.76261787049));
#107080=CARTESIAN_POINT('Ctrl Pts',(32.9521573659891,-5.82931930270299,
92.61621541888));
#107081=CARTESIAN_POINT('Ctrl Pts',(31.9551618598791,-7.31697565127499,
92.35621163472));
#107082=CARTESIAN_POINT('Ctrl Pts',(30.7878189799691,-8.81951599642399,
91.9596113594201));
#107083=CARTESIAN_POINT('Ctrl Pts',(29.5643467643691,-10.21287137887,91.45281600972));
#107084=CARTESIAN_POINT('Ctrl Pts',(28.3547145027491,-11.46125770319,90.86912642514));
#107085=CARTESIAN_POINT('Ctrl Pts',(27.1462246720591,-12.60932492795,90.2068010813201));
#107086=CARTESIAN_POINT('Ctrl Pts',(25.8804633212691,-13.72121825748,89.42218714027));
#107087=CARTESIAN_POINT('Ctrl Pts',(24.5415426038291,-14.80846467629,88.4770655865801));
#107088=CARTESIAN_POINT('Ctrl Pts',(23.1553900553591,-15.84725088264,87.34998754959));
#107089=CARTESIAN_POINT('Ctrl Pts',(21.7169286490991,-16.83785256507,85.9795861337301));
#107090=CARTESIAN_POINT('Ctrl Pts',(20.1864646779891,-17.79411649535,84.2176273015201));
#107091=CARTESIAN_POINT('Ctrl Pts',(18.6056376920291,-18.65837811088,81.868380902977));
#107092=CARTESIAN_POINT('Ctrl Pts',(17.2833457609491,-19.22934869733,78.9739891356611));
#107093=CARTESIAN_POINT('Ctrl Pts',(16.7318898964791,-19.34793907064,76.820460370021));
#107094=CARTESIAN_POINT('Ctrl Pts',(16.5654152065891,-19.34439445674,75.849914932886));
#107095=CARTESIAN_POINT('Ctrl Pts',(38.6686947048191,-0.267618408180286,
87.57152762521));
#107096=CARTESIAN_POINT('Ctrl Pts',(38.6331457099391,-0.640502714598286,
87.56228047755));
#107097=CARTESIAN_POINT('Ctrl Pts',(38.4681697649291,-1.45257130791499,
87.5371031361401));
#107098=CARTESIAN_POINT('Ctrl Pts',(37.9543196144491,-2.67152049410099,
87.46697907679));
#107099=CARTESIAN_POINT('Ctrl Pts',(37.1964789572891,-3.89993484531899,
87.33954011223));
#107100=CARTESIAN_POINT('Ctrl Pts',(36.2722354399091,-5.08847143352099,
87.1482156939501));
#107101=CARTESIAN_POINT('Ctrl Pts',(35.1711071623791,-6.27550574943099,
86.8740206795701));
#107102=CARTESIAN_POINT('Ctrl Pts',(33.9234036585391,-7.436166673543,86.50611895787));
#107103=CARTESIAN_POINT('Ctrl Pts',(32.6526782149891,-8.48396598041999,
86.07171874038));
#107104=CARTESIAN_POINT('Ctrl Pts',(31.4266015655591,-9.40280963542199,
85.5959755830301));
#107105=CARTESIAN_POINT('Ctrl Pts',(30.2282183070691,-10.23269364386,85.07485106796));
#107106=CARTESIAN_POINT('Ctrl Pts',(29.0009821455491,-11.02282107056,84.4750277186701));
#107107=CARTESIAN_POINT('Ctrl Pts',(27.7349646372491,-11.7823880216,83.77066674245));
#107108=CARTESIAN_POINT('Ctrl Pts',(26.4611997445191,-12.49587308951,82.949856613029));
#107109=CARTESIAN_POINT('Ctrl Pts',(25.1820693516891,-13.16490311603,81.9728674396441));
#107110=CARTESIAN_POINT('Ctrl Pts',(23.8728795301391,-13.79985263807,80.741966022882));
#107111=CARTESIAN_POINT('Ctrl Pts',(22.5850112147791,-14.36356654138,79.133191069062));
#107112=CARTESIAN_POINT('Ctrl Pts',(21.5697113092491,-14.73019815096,77.183930116823));
#107113=CARTESIAN_POINT('Ctrl Pts',(21.1758003549191,-14.80581932552,75.7409655371681));
#107114=CARTESIAN_POINT('Ctrl Pts',(21.0646250899491,-14.8035595922,75.088550558094));
#107115=CARTESIAN_POINT('Ctrl Pts',(45.0312706731691,-0.556809233210386,
86.63588923546));
#107116=CARTESIAN_POINT('Ctrl Pts',(44.9819984429591,-1.15239083593299,
86.6032111113799));
#107117=CARTESIAN_POINT('Ctrl Pts',(44.7550297579291,-2.43387817146999,
86.47794742155));
#107118=CARTESIAN_POINT('Ctrl Pts',(44.0669849657891,-4.23139684260399,
86.1321464635101));
#107119=CARTESIAN_POINT('Ctrl Pts',(43.0931519133991,-5.87949518942999,
85.65298684557));
#107120=CARTESIAN_POINT('Ctrl Pts',(41.9506857162891,-7.33390305288999,
85.0915934778799));
#107121=CARTESIAN_POINT('Ctrl Pts',(40.6400631633491,-8.65884473130499,
84.44202906066));
#107122=CARTESIAN_POINT('Ctrl Pts',(39.2094613534091,-9.84085525044999,
83.71996478425));
#107123=CARTESIAN_POINT('Ctrl Pts',(37.8019957376891,-10.82051536224,82.99003573172));
#107124=CARTESIAN_POINT('Ctrl Pts',(36.4852355554891,-11.6168290835,82.283717786993));
#107125=CARTESIAN_POINT('Ctrl Pts',(35.2348621603691,-12.28740211764,81.586024678646));
#107126=CARTESIAN_POINT('Ctrl Pts',(33.9934103628291,-12.88127932846,80.858065721516));
#107127=CARTESIAN_POINT('Ctrl Pts',(32.7581770629291,-13.40872065919,80.08477919832));
#107128=CARTESIAN_POINT('Ctrl Pts',(31.5683175582891,-13.86272653758,79.272924596943));
#107129=CARTESIAN_POINT('Ctrl Pts',(30.4356778789491,-14.24928723071,78.407307267481));
#107130=CARTESIAN_POINT('Ctrl Pts',(29.3529211006491,-14.57798235441,77.439888248051));
#107131=CARTESIAN_POINT('Ctrl Pts',(28.3831326036191,-14.83361972799,76.336383711929));
#107132=CARTESIAN_POINT('Ctrl Pts',(27.7038229907891,-14.97888942575,75.170329705841));
#107133=CARTESIAN_POINT('Ctrl Pts',(27.4678322792991,-15.00690558171,74.365048202755));
#107134=CARTESIAN_POINT('Ctrl Pts',(27.4060630052191,-15.00607043787,73.999190543978));
#107135=CARTESIAN_POINT('Ctrl Pts',(31.7476692742198,-11.9111553334129,
83.9674561810205));
#107136=CARTESIAN_POINT('Ctrl Pts',(31.9900350122681,-11.6718844892141,
84.3582893314217));
#107137=CARTESIAN_POINT('Ctrl Pts',(32.2325023891363,-11.420244524838,84.7437537826362));
#107138=CARTESIAN_POINT('Ctrl Pts',(32.6614487604326,-10.9499616738916,
85.4194048480172));
#107139=CARTESIAN_POINT('Ctrl Pts',(32.8496143409744,-10.7348422493249,
85.7135871729915));
#107140=CARTESIAN_POINT('Ctrl Pts',(33.0354795753356,-10.5124729887581,
86.002767963063));
#107141=CARTESIAN_POINT('Origin',(31.9617040310391,11.38539957172,83.36473278179));
#107142=CARTESIAN_POINT('Ctrl Pts',(32.4210191728332,-10.34163791149,81.9367868442564));
#107143=CARTESIAN_POINT('Ctrl Pts',(32.5625988328022,-10.1165328327363,
81.9823275610893));
#107144=CARTESIAN_POINT('Ctrl Pts',(32.69839419895,-9.89738949147113,82.049406907544));
#107145=CARTESIAN_POINT('Ctrl Pts',(32.9735010138201,-9.45516064419882,
82.2420387731289));
#107146=CARTESIAN_POINT('Ctrl Pts',(33.1455699418812,-9.17784383559699,
82.409453065027));
#107147=CARTESIAN_POINT('Ctrl Pts',(33.304585399266,-8.95817382749374,82.6925802044263));
#107148=CARTESIAN_POINT('Ctrl Pts',(33.3403472037622,-8.91216026273485,
82.7673290310841));
#107149=CARTESIAN_POINT('Ctrl Pts',(33.400100434177,-8.84867606677267,82.9304931696846));
#107150=CARTESIAN_POINT('Ctrl Pts',(33.423915194776,-8.8317608663218,83.0191886464178));
#107151=CARTESIAN_POINT('Ctrl Pts',(33.4389156605574,-8.8317608663218,83.1042605152897));
#107152=CARTESIAN_POINT('Origin',(11.833832765324,1.4210854715202E-14,67.1130006183894));
#107153=CARTESIAN_POINT('Origin',(11.833832765324,1.4210854715202E-14,67.1130006183894));
#107154=CARTESIAN_POINT('',(-4.35610816560352,-4.33090945180056,90.6854703082044));
#107155=CARTESIAN_POINT('',(5.52231334906584,-17.4578705567949,93.2013353119523));
#107156=CARTESIAN_POINT('Ctrl Pts',(-4.35611010952668,-4.33091289415503,
90.685455311287));
#107157=CARTESIAN_POINT('Ctrl Pts',(-3.98956300814287,-5.77320552148352,
90.9690031198165));
#107158=CARTESIAN_POINT('Ctrl Pts',(-3.45353720107494,-7.14208397764978,
91.3707045991231));
#107159=CARTESIAN_POINT('Ctrl Pts',(-2.19019201912765,-9.58743742151509,
92.1835171115637));
#107160=CARTESIAN_POINT('Ctrl Pts',(-1.47920675948711,-10.6934433015076,
92.5940797795233));
#107161=CARTESIAN_POINT('Ctrl Pts',(0.341152214773563,-13.0620281433899,
93.4022734954383));
#107162=CARTESIAN_POINT('Ctrl Pts',(1.44307216932659,-14.2005867443726,
93.732227499844));
#107163=CARTESIAN_POINT('Ctrl Pts',(3.05159459760781,-15.6229944483531,
93.8400521806102));
#107164=CARTESIAN_POINT('Ctrl Pts',(3.58482881504141,-16.0578814173498,
93.8206256404535));
#107165=CARTESIAN_POINT('Ctrl Pts',(4.76564826470288,-16.9510727199715,
93.5866875535521));
#107166=CARTESIAN_POINT('Ctrl Pts',(5.22912462942103,-17.2624413963519,
93.3669714685417));
#107167=CARTESIAN_POINT('Ctrl Pts',(5.52227383940231,-17.4578559214869,
93.2012481656177));
#107168=CARTESIAN_POINT('',(-3.38209691493766,-8.56599685566968,88.073658572396));
#107169=CARTESIAN_POINT('Ctrl Pts',(-4.35610633752318,-4.33090605764581,
90.6854852128844));
#107170=CARTESIAN_POINT('Ctrl Pts',(-4.54154600199715,-3.60121467706104,
90.5420613441333));
#107171=CARTESIAN_POINT('Ctrl Pts',(-4.66228844482028,-2.97979138225131,
90.3835003204796));
#107172=CARTESIAN_POINT('Ctrl Pts',(-4.76846785957156,-2.41966836721192,
90.1896898800142));
#107173=CARTESIAN_POINT('Ctrl Pts',(-4.79766454744446,-2.26180047015079,
90.1269979540808));
#107174=CARTESIAN_POINT('Ctrl Pts',(-4.83130822577944,-2.10288053743367,
90.0326105277975));
#107175=CARTESIAN_POINT('Ctrl Pts',(-4.84077737827289,-2.06137827664836,
90.0031576448214));
#107176=CARTESIAN_POINT('Ctrl Pts',(-4.85403047519485,-2.01453819592731,
89.9548442851971));
#107177=CARTESIAN_POINT('Ctrl Pts',(-4.85878442471103,-1.99986733184758,
89.9361737747806));
#107178=CARTESIAN_POINT('Ctrl Pts',(-4.86661900096031,-1.98284914892481,
89.9012996077116));
#107179=CARTESIAN_POINT('Ctrl Pts',(-4.86975107961287,-1.97815774911654,
89.8861523758613));
#107180=CARTESIAN_POINT('Ctrl Pts',(-4.87567409040339,-1.97529418204614,
89.8541588802312));
#107181=CARTESIAN_POINT('Ctrl Pts',(-4.87825684110292,-1.97726621084453,
89.8384146145568));
#107182=CARTESIAN_POINT('Ctrl Pts',(-4.88353893083735,-1.98889666576724,
89.8019517129379));
#107183=CARTESIAN_POINT('Ctrl Pts',(-4.88578599526452,-2.00071050952999,
89.7825769301279));
#107184=CARTESIAN_POINT('Ctrl Pts',(-4.89060144205847,-2.04027600096942,
89.7327681179324));
#107185=CARTESIAN_POINT('Ctrl Pts',(-4.89256783986115,-2.07947111499586,
89.6991459647543));
#107186=CARTESIAN_POINT('Ctrl Pts',(-4.89580440699033,-2.4346495038435,
89.4667340267194));
#107187=CARTESIAN_POINT('Ctrl Pts',(-4.85124311607859,-3.16900005450152,
89.2318596900765));
#107188=CARTESIAN_POINT('Ctrl Pts',(-4.48170045661541,-5.56983424992605,
88.5574293003622));
#107189=CARTESIAN_POINT('Ctrl Pts',(-4.00535207593041,-7.18998713465117,
88.1835494250047));
#107190=CARTESIAN_POINT('Ctrl Pts',(-3.38209691507343,-8.56599685566973,
88.0736585716266));
#107191=CARTESIAN_POINT('',(3.67711001798258,-16.9999999999988,86.8289313159581));
#107192=CARTESIAN_POINT('Origin',(14.9594999633274,1.4210854715202E-14,
84.8395401726047));
#107193=CARTESIAN_POINT('',(6.52236793072597,-18.4999999837107,87.8502704807592));
#107194=CARTESIAN_POINT('Ctrl Pts',(3.67710978043326,-17.,86.8289299687314));
#107195=CARTESIAN_POINT('Ctrl Pts',(3.99139559239029,-17.2150671358623,
86.7735129004292));
#107196=CARTESIAN_POINT('Ctrl Pts',(4.34754070270756,-17.4389532379846,
86.7591293140106));
#107197=CARTESIAN_POINT('Ctrl Pts',(5.06665893878612,-17.8504223940439,
86.8312090840392));
#107198=CARTESIAN_POINT('Ctrl Pts',(5.42965862838439,-18.0384248294259,
86.9149877608384));
#107199=CARTESIAN_POINT('Ctrl Pts',(5.91789315169195,-18.2685458496827,
87.1337400811896));
#107200=CARTESIAN_POINT('Ctrl Pts',(6.09300490374504,-18.346334827275,87.2342769515633));
#107201=CARTESIAN_POINT('Ctrl Pts',(6.30672210579366,-18.432901727933,87.4302697426805));
#107202=CARTESIAN_POINT('Ctrl Pts',(6.36972845372232,-18.4567893765268,
87.503098430441));
#107203=CARTESIAN_POINT('Ctrl Pts',(6.46896467655097,-18.490320459441,87.6644868989771));
#107204=CARTESIAN_POINT('Ctrl Pts',(6.50520812449229,-18.4999932787823,
87.7530334383063));
#107205=CARTESIAN_POINT('Ctrl Pts',(6.52236792752664,-18.4999999965284,
87.8502704813229));
#107206=CARTESIAN_POINT('',(7.18082331871055,-18.4999999999755,91.584556528483));
#107207=CARTESIAN_POINT('',(3.13624619141446,-18.5,68.6466197984171));
#107208=CARTESIAN_POINT('',(6.72291618991372,-18.2006285964414,92.4517527605434));
#107209=CARTESIAN_POINT('Ctrl Pts',(7.18082331870226,-18.4999999999971,
91.5845565284845));
#107210=CARTESIAN_POINT('Ctrl Pts',(7.18850613867666,-18.5000000709139,
91.6281271102621));
#107211=CARTESIAN_POINT('Ctrl Pts',(7.1923228389523,-18.4981595928469,91.6719941835109));
#107212=CARTESIAN_POINT('Ctrl Pts',(7.19155915231309,-18.4904703123138,
91.7602655374697));
#107213=CARTESIAN_POINT('Ctrl Pts',(7.18696014363605,-18.4846829765142,
91.8038203409861));
#107214=CARTESIAN_POINT('Ctrl Pts',(7.15984955096027,-18.4606687798121,
91.9378269873827));
#107215=CARTESIAN_POINT('Ctrl Pts',(7.12379243649138,-18.4364837977388,
92.0217596633147));
#107216=CARTESIAN_POINT('Ctrl Pts',(7.03345361994085,-18.3804809940909,
92.1672910669025));
#107217=CARTESIAN_POINT('Ctrl Pts',(6.981424799771,-18.3497232834015,92.2298483634182));
#107218=CARTESIAN_POINT('Ctrl Pts',(6.86282535622547,-18.2807333702774,
92.3477958645267));
#107219=CARTESIAN_POINT('Ctrl Pts',(6.79392622567087,-18.241259822421,92.403017754057));
#107220=CARTESIAN_POINT('Ctrl Pts',(6.72291494162312,-18.200628154702,92.4517505732837));
#107221=CARTESIAN_POINT('Ctrl Pts',(5.52235284477145,-17.4578851823617,
93.2014224682222));
#107222=CARTESIAN_POINT('Ctrl Pts',(5.72370338494148,-17.5920989308729,
93.0876563122291));
#107223=CARTESIAN_POINT('Ctrl Pts',(5.92504705677759,-17.7212905264079,
92.9681277382207));
#107224=CARTESIAN_POINT('Ctrl Pts',(6.32572080308318,-17.9689211252111,
92.7180495304402));
#107225=CARTESIAN_POINT('Ctrl Pts',(6.52475300915694,-18.0872399127614,
92.5877736764462));
#107226=CARTESIAN_POINT('Ctrl Pts',(6.72291744207803,-18.2006290368992,
92.4517549519884));
#107227=CARTESIAN_POINT('Ctrl Pts',(-3.02748297213691,-16.72098536733,90.87050995462));
#107228=CARTESIAN_POINT('Ctrl Pts',(-2.76741589283891,-16.72098536733,90.9223387409));
#107229=CARTESIAN_POINT('Ctrl Pts',(-2.20315940912091,-16.72098536733,91.04438774742));
#107230=CARTESIAN_POINT('Ctrl Pts',(-1.36204058715091,-16.72098536733,91.25306306065));
#107231=CARTESIAN_POINT('Ctrl Pts',(-0.530947724290913,-16.72098536733,
91.4804220205299));
#107232=CARTESIAN_POINT('Ctrl Pts',(0.220249863419087,-16.72098536733,91.6980000211799));
#107233=CARTESIAN_POINT('Ctrl Pts',(0.895988512819086,-16.72098536733,91.8987274439699));
#107234=CARTESIAN_POINT('Ctrl Pts',(1.50513857083909,-16.72098536733,92.0797274483699));
#107235=CARTESIAN_POINT('Ctrl Pts',(2.05850149532909,-16.72098536733,92.24052148621));
#107236=CARTESIAN_POINT('Ctrl Pts',(2.56464571939909,-16.72098536733,92.38151018466));
#107237=CARTESIAN_POINT('Ctrl Pts',(3.03062126430909,-16.72098536733,92.50329230408));
#107238=CARTESIAN_POINT('Ctrl Pts',(3.46055536031908,-16.72098536733,92.6062344343699));
#107239=CARTESIAN_POINT('Ctrl Pts',(3.85857840518909,-16.72098536733,92.69139482375));
#107240=CARTESIAN_POINT('Ctrl Pts',(4.22948852246909,-16.72098536733,92.76008351918));
#107241=CARTESIAN_POINT('Ctrl Pts',(4.57751175258909,-16.72098536733,92.81335828303));
#107242=CARTESIAN_POINT('Ctrl Pts',(4.82900967236909,-16.72098536733,92.84336104984));
#107243=CARTESIAN_POINT('Ctrl Pts',(4.96464306063909,-16.72098536733,92.8564918230699));
#107244=CARTESIAN_POINT('Ctrl Pts',(4.99018242526908,-16.72098536733,92.8588546212399));
#107245=CARTESIAN_POINT('Ctrl Pts',(-3.07030643866891,-17.87841055123,91.0854009342301));
#107246=CARTESIAN_POINT('Ctrl Pts',(-2.81258371044191,-17.87841055123,91.1367624857301));
#107247=CARTESIAN_POINT('Ctrl Pts',(-2.25302994109091,-17.87841055123,91.2577878440801));
#107248=CARTESIAN_POINT('Ctrl Pts',(-1.41756024129091,-17.87841055123,91.4650501435));
#107249=CARTESIAN_POINT('Ctrl Pts',(-0.590567647620912,-17.87841055123,
91.6912794621601));
#107250=CARTESIAN_POINT('Ctrl Pts',(0.158357462979087,-17.87841055123,91.90819507323));
#107251=CARTESIAN_POINT('Ctrl Pts',(0.833361273419087,-17.87841055123,92.10870296934));
#107252=CARTESIAN_POINT('Ctrl Pts',(1.44313497812909,-17.87841055123,92.28988942047));
#107253=CARTESIAN_POINT('Ctrl Pts',(1.99830874984909,-17.87841055123,92.4512124919601));
#107254=CARTESIAN_POINT('Ctrl Pts',(2.50728843127908,-17.87841055123,92.59299586447));
#107255=CARTESIAN_POINT('Ctrl Pts',(2.97716951007909,-17.87841055123,92.71580500278));
#107256=CARTESIAN_POINT('Ctrl Pts',(3.41188248195909,-17.87841055123,92.81989834208));
#107257=CARTESIAN_POINT('Ctrl Pts',(3.81545655558909,-17.87841055123,92.90625460732));
#107258=CARTESIAN_POINT('Ctrl Pts',(4.19272113607909,-17.87841055123,92.97612920327));
#107259=CARTESIAN_POINT('Ctrl Pts',(4.54778442056909,-17.87841055123,93.03048953972));
#107260=CARTESIAN_POINT('Ctrl Pts',(4.80494170520909,-17.87841055123,93.061172168));
#107261=CARTESIAN_POINT('Ctrl Pts',(4.94384757402909,-17.87841055123,93.0746201759801));
#107262=CARTESIAN_POINT('Ctrl Pts',(4.97001116901909,-17.87841055123,93.07704084778));
#107263=CARTESIAN_POINT('Ctrl Pts',(-2.90635108794991,-18.70537143846,90.26266217014));
#107264=CARTESIAN_POINT('Ctrl Pts',(-2.63965269910391,-18.70537143846,90.31581259229));
#107265=CARTESIAN_POINT('Ctrl Pts',(-2.06209396084091,-18.70537143846,90.4407571241401));
#107266=CARTESIAN_POINT('Ctrl Pts',(-1.20499584369091,-18.70537143846,90.6534293353001));
#107267=CARTESIAN_POINT('Ctrl Pts',(-0.362304822780912,-18.70537143846,
90.8839836359601));
#107268=CARTESIAN_POINT('Ctrl Pts',(0.395320769359087,-18.70537143846,91.10343529384));
#107269=CARTESIAN_POINT('Ctrl Pts',(1.07313800872909,-18.70537143846,91.3047836771201));
#107270=CARTESIAN_POINT('Ctrl Pts',(1.68052399893909,-18.70537143846,91.4852562921));
#107271=CARTESIAN_POINT('Ctrl Pts',(2.22876470065909,-18.70537143846,91.64455388772));
#107272=CARTESIAN_POINT('Ctrl Pts',(2.72688845555909,-18.70537143846,91.78329474466));
#107273=CARTESIAN_POINT('Ctrl Pts',(3.18181667720909,-18.70537143846,91.90217180423));
#107274=CARTESIAN_POINT('Ctrl Pts',(3.59823308570909,-18.70537143846,92.00185758637));
#107275=CARTESIAN_POINT('Ctrl Pts',(3.98055430565909,-18.70537143846,92.08363528142));
#107276=CARTESIAN_POINT('Ctrl Pts',(4.33348997659909,-18.70537143846,92.1489694991201));
#107277=CARTESIAN_POINT('Ctrl Pts',(4.66159947439909,-18.70537143846,92.19917357618));
#107278=CARTESIAN_POINT('Ctrl Pts',(4.89708912615909,-18.70537143846,92.2272532641701));
#107279=CARTESIAN_POINT('Ctrl Pts',(5.02346586689909,-18.70537143846,92.23948669662));
#107280=CARTESIAN_POINT('Ctrl Pts',(5.04723951276909,-18.70537143846,92.2416857915));
#107281=CARTESIAN_POINT('Ctrl Pts',(-2.68078525475691,-18.46966542386,89.1307579413));
#107282=CARTESIAN_POINT('Ctrl Pts',(-2.40173836763091,-18.46966542386,89.18636944872));
#107283=CARTESIAN_POINT('Ctrl Pts',(-1.79940882562091,-18.46966542386,89.31670588532));
#107284=CARTESIAN_POINT('Ctrl Pts',(-0.912554851410912,-18.46966542386,
89.5368209230901));
#107285=CARTESIAN_POINT('Ctrl Pts',(-0.0482663113909114,-18.46966542386,
89.7733254300899));
#107286=CARTESIAN_POINT('Ctrl Pts',(0.721329194239087,-18.46966542386,89.99626612027));
#107287=CARTESIAN_POINT('Ctrl Pts',(1.40301708156909,-18.46966542386,90.1987708256));
#107288=CARTESIAN_POINT('Ctrl Pts',(2.00711811150908,-18.46966542386,90.3782613619799));
#107289=CARTESIAN_POINT('Ctrl Pts',(2.54582046205908,-18.46966542386,90.53477235655));
#107290=CARTESIAN_POINT('Ctrl Pts',(3.02900889400909,-18.46966542386,90.66932739364));
#107291=CARTESIAN_POINT('Ctrl Pts',(3.46336533396909,-18.46966542386,90.78279479372));
#107292=CARTESIAN_POINT('Ctrl Pts',(3.85460977005909,-18.46966542386,90.8764167646));
#107293=CARTESIAN_POINT('Ctrl Pts',(4.20769182441909,-18.46966542386,90.9518953727701));
#107294=CARTESIAN_POINT('Ctrl Pts',(4.52715636601909,-18.46966542386,91.01098304712));
#107295=CARTESIAN_POINT('Ctrl Pts',(4.81818349152909,-18.46966542386,91.05546904236));
#107296=CARTESIAN_POINT('Ctrl Pts',(5.02386333443909,-18.46966542386,91.0799676676101));
#107297=CARTESIAN_POINT('Ctrl Pts',(5.13300280174909,-18.46966542386,91.09053011623));
#107298=CARTESIAN_POINT('Ctrl Pts',(5.15348841302909,-18.46966542386,91.0924243709));
#107299=CARTESIAN_POINT('',(4.84744046295298,-18.0488789356219,92.4405620175361));
#107300=CARTESIAN_POINT('',(4.96802222338909,-18.49999999899,91.37511854801));
#107301=CARTESIAN_POINT('Ctrl Pts',(4.84744046295299,-18.0488789356218,
92.440562017536));
#107302=CARTESIAN_POINT('Ctrl Pts',(4.85102555078097,-18.0815232141951,
92.4088329939532));
#107303=CARTESIAN_POINT('Ctrl Pts',(4.85478207102745,-18.1127201945377,
92.3756064273925));
#107304=CARTESIAN_POINT('Ctrl Pts',(4.85868549383694,-18.1422807586517,
92.3410948468652));
#107305=CARTESIAN_POINT('Ctrl Pts',(4.86260561708453,-18.1719677949405,
92.3064356116915));
#107306=CARTESIAN_POINT('Ctrl Pts',(4.86667382820382,-18.2000039257964,
92.2704809975323));
#107307=CARTESIAN_POINT('Ctrl Pts',(4.87086197000954,-18.2262411725814,
92.2334756604867));
#107308=CARTESIAN_POINT('Ctrl Pts',(4.87506446674988,-18.2525683480221,
92.1963434869542));
#107309=CARTESIAN_POINT('Ctrl Pts',(4.87938763195323,-18.2770840322067,
92.1581541306553));
#107310=CARTESIAN_POINT('Ctrl Pts',(4.88380090536888,-18.2996878866408,
92.1191736136303));
#107311=CARTESIAN_POINT('Ctrl Pts',(4.88825477898303,-18.3224996867175,
92.07983449278));
#107312=CARTESIAN_POINT('Ctrl Pts',(4.89280033628601,-18.3433642290032,
92.0396903814176));
#107313=CARTESIAN_POINT('Ctrl Pts',(4.89740535261491,-18.362231073403,91.9990221095588));
#107314=CARTESIAN_POINT('Ctrl Pts',(4.89993844674995,-18.3726092109562,
91.9766516001902));
#107315=CARTESIAN_POINT('Ctrl Pts',(4.90248952589719,-18.382383822476,91.9541225481696));
#107316=CARTESIAN_POINT('Ctrl Pts',(4.9050532720603,-18.3915532115038,91.9314813226531));
#107317=CARTESIAN_POINT('Ctrl Pts',(4.90978228961777,-18.408466821099,91.8897179240253));
#107318=CARTESIAN_POINT('Ctrl Pts',(4.9145543126211,-18.4233184390315,91.8475736367873));
#107319=CARTESIAN_POINT('Ctrl Pts',(4.91933724298231,-18.4361372479446,
91.8053295547132));
#107320=CARTESIAN_POINT('Ctrl Pts',(4.92421230508372,-18.4492029806228,
91.7622717412023));
#107321=CARTESIAN_POINT('Ctrl Pts',(4.9290986181819,-18.4601571995976,91.7191109638508));
#107322=CARTESIAN_POINT('Ctrl Pts',(4.93396478461095,-18.4690800708054,
91.6761221600157));
#107323=CARTESIAN_POINT('Ctrl Pts',(4.93889011969135,-18.4781114369162,
91.6326106470659));
#107324=CARTESIAN_POINT('Ctrl Pts',(4.94379475346279,-18.4850623405295,
91.5892758617947));
#107325=CARTESIAN_POINT('Ctrl Pts',(4.94864984772086,-18.4900585310788,
91.5463702061315));
#107326=CARTESIAN_POINT('Ctrl Pts',(4.95360660584777,-18.4951593400008,
91.5025661219893));
#107327=CARTESIAN_POINT('Ctrl Pts',(4.95851167916532,-18.4982233765136,
91.4592097608613));
#107328=CARTESIAN_POINT('Ctrl Pts',(4.96333909424765,-18.499419121208,91.4165282140099));
#107329=CARTESIAN_POINT('Ctrl Pts',(4.96490856559217,-18.4998078773023,
91.402651747292));
#107330=CARTESIAN_POINT('Ctrl Pts',(4.96646986780409,-18.4999993792627,
91.3888462619152));
#107331=CARTESIAN_POINT('Ctrl Pts',(4.96802222338909,-18.4999999984913,
91.37511854801));
#107332=CARTESIAN_POINT('',(-2.58464131998993,-18.4999999121182,89.4559753223385));
#107333=CARTESIAN_POINT('Ctrl Pts',(-2.58464131998983,-18.4999999284356,
89.4559753223381));
#107334=CARTESIAN_POINT('Ctrl Pts',(-2.42247927437401,-18.4999999283618,
89.4893110383322));
#107335=CARTESIAN_POINT('Ctrl Pts',(-2.26335533538253,-18.4999999529729,
89.5236774280323));
#107336=CARTESIAN_POINT('Ctrl Pts',(-2.10688850553027,-18.4999999715301,
89.5588228176755));
#107337=CARTESIAN_POINT('Ctrl Pts',(-2.04276780678778,-18.4999999791349,
89.5732255312961));
#107338=CARTESIAN_POINT('Ctrl Pts',(-1.97909337321858,-18.499999985739,
89.587759699513));
#107339=CARTESIAN_POINT('Ctrl Pts',(-1.91583913818256,-18.49999999043,89.6024104702437));
#107340=CARTESIAN_POINT('Ctrl Pts',(-1.8205009702631,-18.4999999975004,
89.6244924326495));
#107341=CARTESIAN_POINT('Ctrl Pts',(-1.72611730868866,-18.499999999998,
89.646838986621));
#107342=CARTESIAN_POINT('Ctrl Pts',(-1.63259488358994,-18.499999999998,
89.6694020422784));
#107343=CARTESIAN_POINT('Ctrl Pts',(-1.43742956816962,-18.499999999998,
89.716487282739));
#107344=CARTESIAN_POINT('Ctrl Pts',(-1.24601784666857,-18.4999999972403,
89.7644910558193));
#107345=CARTESIAN_POINT('Ctrl Pts',(-1.06015417158908,-18.4999999985324,
89.8125315836417));
#107346=CARTESIAN_POINT('Ctrl Pts',(-1.02723545567207,-18.4999999987613,
89.8210401450226));
#107347=CARTESIAN_POINT('Ctrl Pts',(-0.994490687489129,-18.4999999990028,
89.8295497600841));
#107348=CARTESIAN_POINT('Ctrl Pts',(-0.961929727974486,-18.4999999992167,
89.8380554342449));
#107349=CARTESIAN_POINT('Ctrl Pts',(-0.889157904801211,-18.499999999695,
89.8570651140955));
#107350=CARTESIAN_POINT('Ctrl Pts',(-0.817304239126653,-18.499999999998,
89.8760550782654));
#107351=CARTESIAN_POINT('Ctrl Pts',(-0.746477846876206,-18.499999999998,
89.8949680126866));
#107352=CARTESIAN_POINT('Ctrl Pts',(-0.60356647905789,-18.499999999998,
89.933129963927));
#107353=CARTESIAN_POINT('Ctrl Pts',(-0.464844365327987,-18.4999999995685,
89.970995089684));
#107354=CARTESIAN_POINT('Ctrl Pts',(-0.329968692827295,-18.4999999996937,
90.0084006617666));
#107355=CARTESIAN_POINT('Ctrl Pts',(-0.252794460947361,-18.4999999997653,
90.0298036786338));
#107356=CARTESIAN_POINT('Ctrl Pts',(-0.176879758684409,-18.4999999998833,
90.0510572704772));
#107357=CARTESIAN_POINT('Ctrl Pts',(-0.102161930483246,-18.4999999999422,
90.0721383232775));
#107358=CARTESIAN_POINT('Ctrl Pts',(-0.0502963668242797,-18.499999999983,
90.086771787771));
#107359=CARTESIAN_POINT('Ctrl Pts',(0.000992469381286637,-18.499999999998,
90.1013222121036));
#107360=CARTESIAN_POINT('Ctrl Pts',(0.0517258844157116,-18.499999999998,
90.1157821369));
#107361=CARTESIAN_POINT('Ctrl Pts',(0.193134512360498,-18.499999999998,
90.1560861086365));
#107362=CARTESIAN_POINT('Ctrl Pts',(0.33022671944429,-18.4999999999633,
90.1956827469086));
#107363=CARTESIAN_POINT('Ctrl Pts',(0.46302310172386,-18.4999999999761,
90.2343586844309));
#107364=CARTESIAN_POINT('Ctrl Pts',(0.531039009910421,-18.4999999999826,
90.2541678009925));
#107365=CARTESIAN_POINT('Ctrl Pts',(0.597927807241826,-18.4999999999913,
90.2737362471997));
#107366=CARTESIAN_POINT('Ctrl Pts',(0.663691145680396,-18.4999999999951,
90.2930404695069));
#107367=CARTESIAN_POINT('Ctrl Pts',(0.697937951951777,-18.4999999999972,
90.3030933040691));
#107368=CARTESIAN_POINT('Ctrl Pts',(0.731879533548189,-18.499999999998,
90.3130745357137));
#107369=CARTESIAN_POINT('Ctrl Pts',(0.765516009892471,-18.499999999998,
90.3229808414617));
#107370=CARTESIAN_POINT('Ctrl Pts',(0.895913684424494,-18.499999999998,
90.3613843656453));
#107371=CARTESIAN_POINT('Ctrl Pts',(1.02172716610423,-18.4999999999955,
90.398659670361));
#107372=CARTESIAN_POINT('Ctrl Pts',(1.14344094134313,-18.4999999999968,
90.4347827934306));
#107373=CARTESIAN_POINT('Ctrl Pts',(1.2104749224429,-18.4999999999976,90.4546776388937));
#107374=CARTESIAN_POINT('Ctrl Pts',(1.27626507277148,-18.499999999998,90.4742240041735));
#107375=CARTESIAN_POINT('Ctrl Pts',(1.34089047774472,-18.499999999998,90.4934241691768));
#107376=CARTESIAN_POINT('Ctrl Pts',(1.36079879604639,-18.499999999998,90.499338917355));
#107377=CARTESIAN_POINT('Ctrl Pts',(1.38059657252599,-18.499999999998,90.5052208381738));
#107378=CARTESIAN_POINT('Ctrl Pts',(1.40028612569937,-18.499999999998,90.5110699428851));
#107379=CARTESIAN_POINT('Ctrl Pts',(1.52644468342528,-18.499999999998,90.548547411666));
#107380=CARTESIAN_POINT('Ctrl Pts',(1.64816139383854,-18.499999999998,90.5846746827562));
#107381=CARTESIAN_POINT('Ctrl Pts',(1.76585682848137,-18.4999999999979,
90.6194412743614));
#107382=CARTESIAN_POINT('Ctrl Pts',(1.82568407703918,-18.4999999999979,
90.6371139183666));
#107383=CARTESIAN_POINT('Ctrl Pts',(1.88447200669,-18.499999999998,90.6544358703474));
#107384=CARTESIAN_POINT('Ctrl Pts',(1.94227444066315,-18.499999999998,90.6714105346848));
#107385=CARTESIAN_POINT('Ctrl Pts',(1.95071832499579,-18.499999999998,90.673890224421));
#107386=CARTESIAN_POINT('Ctrl Pts',(1.95914117746727,-18.499999999998,90.6763625078161));
#107387=CARTESIAN_POINT('Ctrl Pts',(1.96754316566384,-18.499999999998,90.6788273937299));
#107388=CARTESIAN_POINT('Ctrl Pts',(2.09512410234678,-18.499999999998,90.7162557316824));
#107389=CARTESIAN_POINT('Ctrl Pts',(2.21789632546597,-18.4999999999977,
90.7519713117329));
#107390=CARTESIAN_POINT('Ctrl Pts',(2.33648048522128,-18.4999999999979,
90.786049104768));
#107391=CARTESIAN_POINT('Ctrl Pts',(2.38433447329468,-18.499999999998,90.7998010114715));
#107392=CARTESIAN_POINT('Ctrl Pts',(2.43150622941636,-18.499999999998,90.8132868222452));
#107393=CARTESIAN_POINT('Ctrl Pts',(2.47803575426742,-18.499999999998,90.826513582735));
#107394=CARTESIAN_POINT('Ctrl Pts',(2.47881274636391,-18.499999999998,90.8267344551465));
#107395=CARTESIAN_POINT('Ctrl Pts',(2.47958955946783,-18.499999999998,90.8269552553909));
#107396=CARTESIAN_POINT('Ctrl Pts',(2.48036619365538,-18.499999999998,90.8271759834721));
#107397=CARTESIAN_POINT('Ctrl Pts',(2.59599001793783,-18.499999999998,90.8600375614012));
#107398=CARTESIAN_POINT('Ctrl Pts',(2.70764837268176,-18.4999999999976,
90.8912949119218));
#107399=CARTESIAN_POINT('Ctrl Pts',(2.81556632146251,-18.4999999999978,
90.920943621444));
#107400=CARTESIAN_POINT('Ctrl Pts',(2.85790008751792,-18.4999999999979,
90.9325741383964));
#107401=CARTESIAN_POINT('Ctrl Pts',(2.89965825399694,-18.499999999998,90.9439577145226));
#107402=CARTESIAN_POINT('Ctrl Pts',(2.94085432970763,-18.499999999998,90.9550961870934));
#107403=CARTESIAN_POINT('Ctrl Pts',(2.94914642739974,-18.499999999998,90.9573381798343));
#107404=CARTESIAN_POINT('Ctrl Pts',(2.95741575404617,-18.499999999998,90.9595702252726));
#107405=CARTESIAN_POINT('Ctrl Pts',(2.96566243524428,-18.499999999998,90.9617923484759));
#107406=CARTESIAN_POINT('Ctrl Pts',(3.07761262151744,-18.4999999999979,
90.9919580721831));
#107407=CARTESIAN_POINT('Ctrl Pts',(3.18539085749446,-18.499999999998,91.0202907326444));
#107408=CARTESIAN_POINT('Ctrl Pts',(3.28933672475092,-18.499999999998,91.0468531181577));
#107409=CARTESIAN_POINT('Ctrl Pts',(3.31340128417257,-18.499999999998,91.0530025892376));
#107410=CARTESIAN_POINT('Ctrl Pts',(3.33726037793146,-18.499999999998,91.0590573938579));
#107411=CARTESIAN_POINT('Ctrl Pts',(3.36091811406057,-18.499999999998,91.0650186686483));
#107412=CARTESIAN_POINT('Ctrl Pts',(3.3753343264924,-18.499999999998,91.0686512649066));
#107413=CARTESIAN_POINT('Ctrl Pts',(3.3896757551439,-18.499999999998,91.0722490588392));
#107414=CARTESIAN_POINT('Ctrl Pts',(3.40394331686185,-18.499999999998,91.0758123249327));
#107415=CARTESIAN_POINT('Ctrl Pts',(3.52167444174278,-18.499999999998,91.1052151993504));
#107416=CARTESIAN_POINT('Ctrl Pts',(3.63437646858574,-18.499999999998,91.1322618551093));
#107417=CARTESIAN_POINT('Ctrl Pts',(3.74253208016573,-18.499999999998,91.1571146440383));
#107418=CARTESIAN_POINT('Ctrl Pts',(3.7618984974429,-18.499999999998,91.1615648013059));
#107419=CARTESIAN_POINT('Ctrl Pts',(3.78111903871853,-18.499999999998,91.1659445281595));
#107420=CARTESIAN_POINT('Ctrl Pts',(3.80019667602617,-18.499999999998,91.1702549980734));
#107421=CARTESIAN_POINT('Ctrl Pts',(3.90057358324263,-18.499999999998,91.192934517116));
#107422=CARTESIAN_POINT('Ctrl Pts',(3.99699359909732,-18.499999999998,91.213693972243));
#107423=CARTESIAN_POINT('Ctrl Pts',(4.08986202778578,-18.499999999998,91.2326836615883));
#107424=CARTESIAN_POINT('Ctrl Pts',(4.11321407376547,-18.499999999998,91.2374586761438));
#107425=CARTESIAN_POINT('Ctrl Pts',(4.13634181685589,-18.4999999999978,
91.2421216703581));
#107426=CARTESIAN_POINT('Ctrl Pts',(4.15925062103235,-18.4999999999975,
91.2466749152964));
#107427=CARTESIAN_POINT('Ctrl Pts',(4.24476307603062,-18.4999999999964,
91.2636709640594));
#107428=CARTESIAN_POINT('Ctrl Pts',(4.32722530770209,-18.499999999998,91.2791362303439));
#107429=CARTESIAN_POINT('Ctrl Pts',(4.4069358511759,-18.499999999998,91.2931767758584));
#107430=CARTESIAN_POINT('Ctrl Pts',(4.43352619799537,-18.499999999998,91.2978605097597));
#107431=CARTESIAN_POINT('Ctrl Pts',(4.4598108703507,-18.4999999999967,91.3023857892519));
#107432=CARTESIAN_POINT('Ctrl Pts',(4.48581020126748,-18.4999999999932,
91.3067590894636));
#107433=CARTESIAN_POINT('Ctrl Pts',(4.55862954204631,-18.4999999999834,
91.3190078984604));
#107434=CARTESIAN_POINT('Ctrl Pts',(4.62921135945304,-18.499999999998,91.3300662706501));
#107435=CARTESIAN_POINT('Ctrl Pts',(4.6980281630798,-18.499999999998,91.3400811393066));
#107436=CARTESIAN_POINT('Ctrl Pts',(4.72731383018175,-18.499999999998,91.3443430650877));
#107437=CARTESIAN_POINT('Ctrl Pts',(4.75627755155606,-18.4999999999705,
91.3484164128833));
#107438=CARTESIAN_POINT('Ctrl Pts',(4.7849101034947,-18.4999999998331,91.3523016553103));
#107439=CARTESIAN_POINT('Ctrl Pts',(4.84758195043468,-18.4999999995324,
91.3608057984001));
#107440=CARTESIAN_POINT('Ctrl Pts',(4.90866663149108,-18.4999999984913,
91.368407217816));
#107441=CARTESIAN_POINT('Ctrl Pts',(4.96802222338909,-18.4999999984913,
91.37511854801));
#107442=CARTESIAN_POINT('',(-2.88651065708645,-17.0216929393251,90.9254156321813));
#107443=CARTESIAN_POINT('Ctrl Pts',(-2.88651065708645,-17.0216929393251,
90.9254156321813));
#107444=CARTESIAN_POINT('Ctrl Pts',(-2.88640145180437,-17.0995628086248,
90.9240272056507));
#107445=CARTESIAN_POINT('Ctrl Pts',(-2.88729944606883,-17.170132058898,
90.9182441598227));
#107446=CARTESIAN_POINT('Ctrl Pts',(-2.88408965246998,-17.3078577072757,
90.8939618230676));
#107447=CARTESIAN_POINT('Ctrl Pts',(-2.88165190999378,-17.3582840935947,
90.8831196587877));
#107448=CARTESIAN_POINT('Ctrl Pts',(-2.87552901840975,-17.4404493016207,
90.8603531966015));
#107449=CARTESIAN_POINT('Ctrl Pts',(-2.87310852973623,-17.468898354374,
90.8516715121079));
#107450=CARTESIAN_POINT('Ctrl Pts',(-2.86918206784385,-17.5129573190361,
90.8366384861846));
#107451=CARTESIAN_POINT('Ctrl Pts',(-2.86714859023221,-17.5353318776479,
90.8286186440903));
#107452=CARTESIAN_POINT('Ctrl Pts',(-2.86475180509675,-17.5619825690364,
90.8182933829514));
#107453=CARTESIAN_POINT('Ctrl Pts',(-2.863732365432,-17.5735147448426,90.8136508779198));
#107454=CARTESIAN_POINT('Ctrl Pts',(-2.86305596572654,-17.5812266358903,
90.8105064691031));
#107455=CARTESIAN_POINT('Ctrl Pts',(-2.86255639671044,-17.586986281638,
90.8081184917741));
#107456=CARTESIAN_POINT('Ctrl Pts',(-2.85690609956517,-17.6525742813425,
90.7806925204851));
#107457=CARTESIAN_POINT('Ctrl Pts',(-2.85015602453725,-17.7273084397827,
90.7444067214191));
#107458=CARTESIAN_POINT('Ctrl Pts',(-2.83431530931937,-17.8501475630206,
90.6673151810356));
#107459=CARTESIAN_POINT('Ctrl Pts',(-2.82812127750925,-17.8928217227995,
90.6378193587231));
#107460=CARTESIAN_POINT('Ctrl Pts',(-2.8173670861126,-17.9580952571083,
90.5867852678644));
#107461=CARTESIAN_POINT('Ctrl Pts',(-2.81354134391614,-17.9800592712919,
90.5686422926648));
#107462=CARTESIAN_POINT('Ctrl Pts',(-2.80745541916469,-18.0131096158549,
90.539600189903));
#107463=CARTESIAN_POINT('Ctrl Pts',(-2.80432589827305,-18.0296604584008,
90.5246223378286));
#107464=CARTESIAN_POINT('Ctrl Pts',(-2.80052923960525,-18.0489654998569,
90.5063217870538));
#107465=CARTESIAN_POINT('Ctrl Pts',(-2.79887172307984,-18.0572326206646,
90.4982988410398));
#107466=CARTESIAN_POINT('Ctrl Pts',(-2.79776005649735,-18.0627419725255,
90.4929099399053));
#107467=CARTESIAN_POINT('Ctrl Pts',(-2.79688285041213,-18.0670519694588,
90.4886488573163));
#107468=CARTESIAN_POINT('Ctrl Pts',(-2.7809971705961,-18.1447885552345,
90.4114045008268));
#107469=CARTESIAN_POINT('Ctrl Pts',(-2.76011268807195,-18.2451010616449,
90.2967069554987));
#107470=CARTESIAN_POINT('Ctrl Pts',(-2.69081716629771,-18.4229990851704,
89.9576497125368));
#107471=CARTESIAN_POINT('Ctrl Pts',(-2.64099778080791,-18.5000050727964,
89.7303413150615));
#107472=CARTESIAN_POINT('Ctrl Pts',(-2.58464131999691,-18.49999991758,89.45597532234));
#107473=CARTESIAN_POINT('Ctrl Pts',(-2.88654644014915,-17.0216953618235,
90.9255898508946));
#107474=CARTESIAN_POINT('Ctrl Pts',(-2.69742490916333,-17.041410134392,
90.9641774992515));
#107475=CARTESIAN_POINT('Ctrl Pts',(-2.51120236344264,-17.0612039407382,
91.0040506043034));
#107476=CARTESIAN_POINT('Ctrl Pts',(-2.32785216427436,-17.0810959232659,
91.0447708513586));
#107477=CARTESIAN_POINT('Ctrl Pts',(-2.14045947996118,-17.1014264820495,
91.0863888939688));
#107478=CARTESIAN_POINT('Ctrl Pts',(-1.95606671680399,-17.1218596123584,
91.1288915704916));
#107479=CARTESIAN_POINT('Ctrl Pts',(-1.77461315546025,-17.1423912528085,
91.1718473703202));
#107480=CARTESIAN_POINT('Ctrl Pts',(-1.69875208969935,-17.1509750034654,
91.1898060851091));
#107481=CARTESIAN_POINT('Ctrl Pts',(-1.62340441551236,-17.1595756812106,
91.2078444544791));
#107482=CARTESIAN_POINT('Ctrl Pts',(-1.5485643763496,-17.1681917671988,
91.2259329295346));
#107483=CARTESIAN_POINT('Ctrl Pts',(-1.36386673018872,-17.189455395852,
91.27057345622));
#107484=CARTESIAN_POINT('Ctrl Pts',(-1.1822620916855,-17.210814547539,91.3155161541178));
#107485=CARTESIAN_POINT('Ctrl Pts',(-1.00367274643416,-17.2322304456851,
91.360358654297));
#107486=CARTESIAN_POINT('Ctrl Pts',(-0.821153209633123,-17.2541176406033,
91.4061879973085));
#107487=CARTESIAN_POINT('Ctrl Pts',(-0.64178274964877,-17.2760639662355,
91.4519125695349));
#107488=CARTESIAN_POINT('Ctrl Pts',(-0.465462221090628,-17.2980036926607,
91.4971491013743));
#107489=CARTESIAN_POINT('Ctrl Pts',(-0.369787773236968,-17.3099085526844,
91.521695195025));
#107490=CARTESIAN_POINT('Ctrl Pts',(-0.27501108593264,-17.3218110634227,
91.5460983993004));
#107491=CARTESIAN_POINT('Ctrl Pts',(-0.181114947793367,-17.3336980941036,
91.5703031290285));
#107492=CARTESIAN_POINT('Ctrl Pts',(-0.0790942960888194,-17.3466136691308,
91.5966022117184));
#107493=CARTESIAN_POINT('Ctrl Pts',(0.0218789296780678,-17.3595252062434,
91.6226614043843));
#107494=CARTESIAN_POINT('Ctrl Pts',(0.12182234793271,-17.3724259044824,
91.6484080358699));
#107495=CARTESIAN_POINT('Ctrl Pts',(0.30998982251177,-17.39671456551,91.6968822496818));
#107496=CARTESIAN_POINT('Ctrl Pts',(0.494506517524576,-17.4209664306911,
91.7442458924625));
#107497=CARTESIAN_POINT('Ctrl Pts',(0.675467730717484,-17.4451363296152,
91.7900785790369));
#107498=CARTESIAN_POINT('Ctrl Pts',(0.789151121036989,-17.4603203350985,
91.8188715734322));
#107499=CARTESIAN_POINT('Ctrl Pts',(0.901431491157078,-17.4754714086846,
91.8470612859899));
#107500=CARTESIAN_POINT('Ctrl Pts',(1.01233389736521,-17.4905731708789,
91.8745524394624));
#107501=CARTESIAN_POINT('Ctrl Pts',(1.19516693491735,-17.5154698448898,
91.9198741891616));
#107502=CARTESIAN_POINT('Ctrl Pts',(1.37425545371614,-17.5402425452337,
91.9632925176879));
#107503=CARTESIAN_POINT('Ctrl Pts',(1.54966415730625,-17.5648280185183,
92.0043877322477));
#107504=CARTESIAN_POINT('Ctrl Pts',(1.55711643999401,-17.5658725385061,
92.006133672727));
#107505=CARTESIAN_POINT('Ctrl Pts',(1.56456208233662,-17.5669167174875,
92.0078754261942));
#107506=CARTESIAN_POINT('Ctrl Pts',(1.57200108815818,-17.5679605542422,
92.0096129661756));
#107507=CARTESIAN_POINT('Ctrl Pts',(1.66326869021053,-17.5807671684348,
92.0309304797484));
#107508=CARTESIAN_POINT('Ctrl Pts',(1.75353600577784,-17.5935218518874,
92.0516133663183));
#107509=CARTESIAN_POINT('Ctrl Pts',(1.84280452510977,-17.6062185966182,
92.0716139593751));
#107510=CARTESIAN_POINT('Ctrl Pts',(1.88743878477574,-17.6125669689836,
92.0816142559036));
#107511=CARTESIAN_POINT('Ctrl Pts',(1.93182334131449,-17.6189008808474,
92.091443999122));
#107512=CARTESIAN_POINT('Ctrl Pts',(1.97595786838733,-17.6252192062876,
92.1010974690801));
#107513=CARTESIAN_POINT('Ctrl Pts',(1.99802513192375,-17.6283783690077,
92.1059242040592));
#107514=CARTESIAN_POINT('Ctrl Pts',(2.02002988749721,-17.6315336357843,
92.1107068726981));
#107515=CARTESIAN_POINT('Ctrl Pts',(2.04197208025779,-17.6346848579343,
92.115444774685));
#107516=CARTESIAN_POINT('Ctrl Pts',(2.05294317663808,-17.6362604690094,
92.1178137256784));
#107517=CARTESIAN_POINT('Ctrl Pts',(2.06389863227572,-17.6378350689654,
92.1201714851346));
#107518=CARTESIAN_POINT('Ctrl Pts',(2.07483843855079,-17.6394086378195,
92.1225179666464));
#107519=CARTESIAN_POINT('Ctrl Pts',(2.08030834168832,-17.6401954222466,
92.1236912074023));
#107520=CARTESIAN_POINT('Ctrl Pts',(2.08577433248242,-17.6409819489,92.1248616286805));
#107521=CARTESIAN_POINT('Ctrl Pts',(2.09123640974304,-17.6417682151897,
92.1260292197551));
#107522=CARTESIAN_POINT('Ctrl Pts',(2.09669848700366,-17.6425544814794,
92.1271968108297));
#107523=CARTESIAN_POINT('Ctrl Pts',(2.10351059955061,-17.6435355382329,
92.1286500037437));
#107524=CARTESIAN_POINT('Ctrl Pts',(2.10761089969447,-17.6441262303533,
92.1295234916842));
#107525=CARTESIAN_POINT('Ctrl Pts',(2.24213694842401,-17.6635061474786,
92.158181608681));
#107526=CARTESIAN_POINT('Ctrl Pts',(2.37612643197818,-17.6830114011268,
92.1854976283726));
#107527=CARTESIAN_POINT('Ctrl Pts',(2.5096587865986,-17.702596240886,92.2112306127136));
#107528=CARTESIAN_POINT('Ctrl Pts',(2.63660724765655,-17.7212154382676,
92.2356948166873));
#107529=CARTESIAN_POINT('Ctrl Pts',(2.76314226648604,-17.7399063896977,
92.2587286478074));
#107530=CARTESIAN_POINT('Ctrl Pts',(2.88931162583231,-17.7586288569726,
92.2800864466862));
#107531=CARTESIAN_POINT('Ctrl Pts',(2.91200856687956,-17.761996891321,92.283928557834));
#107532=CARTESIAN_POINT('Ctrl Pts',(2.93469327762316,-17.765365993577,92.2877161953679));
#107533=CARTESIAN_POINT('Ctrl Pts',(2.95736544668735,-17.7687356707034,
92.2914478033765));
#107534=CARTESIAN_POINT('Ctrl Pts',(3.06399310547184,-17.7845833287652,
92.3089976295241));
#107535=CARTESIAN_POINT('Ctrl Pts',(3.17034340538539,-17.8004430770719,
92.3253095598612));
#107536=CARTESIAN_POINT('Ctrl Pts',(3.2764152873118,-17.8162938077448,92.3402375054109));
#107537=CARTESIAN_POINT('Ctrl Pts',(3.34072822557292,-17.8259043383081,
92.3492885378152));
#107538=CARTESIAN_POINT('Ctrl Pts',(3.40493909975878,-17.8355114884629,
92.3578306426863));
#107539=CARTESIAN_POINT('Ctrl Pts',(3.4690461953169,-17.8451081528638,92.3658301801403));
#107540=CARTESIAN_POINT('Ctrl Pts',(3.50109974309596,-17.8499064850642,
92.3698299488672));
#107541=CARTESIAN_POINT('Ctrl Pts',(3.5331273495993,-17.8547021827024,92.3736940590896));
#107542=CARTESIAN_POINT('Ctrl Pts',(3.56512883049294,-17.8594942505125,
92.3774182247455));
#107543=CARTESIAN_POINT('Ctrl Pts',(3.58112957093976,-17.8618902844176,
92.3792803075735));
#107544=CARTESIAN_POINT('Ctrl Pts',(3.59712377991582,-17.8642854098686,
92.3811074036578));
#107545=CARTESIAN_POINT('Ctrl Pts',(3.61311160553143,-17.8666795875392,
92.382898941446));
#107546=CARTESIAN_POINT('Ctrl Pts',(3.62110551833924,-17.8678766763745,
92.3837947103401));
#107547=CARTESIAN_POINT('Ctrl Pts',(3.62909783536523,-17.869073528213,92.3846815895001));
#107548=CARTESIAN_POINT('Ctrl Pts',(3.63708856106238,-17.8702701303337,
92.3855595089788));
#107549=CARTESIAN_POINT('Ctrl Pts',(3.64108392391096,-17.870868431394,92.3859984687182));
#107550=CARTESIAN_POINT('Ctrl Pts',(3.64507888892851,-17.8714666700209,
92.3864351885318));
#107551=CARTESIAN_POINT('Ctrl Pts',(3.64907345713086,-17.8720648448385,
92.3868696595651));
#107552=CARTESIAN_POINT('Ctrl Pts',(3.65306802533321,-17.8726630196562,
92.3873041305985));
#107553=CARTESIAN_POINT('Ctrl Pts',(3.658527814823,-17.8734805988681,92.3878941393569));
#107554=CARTESIAN_POINT('Ctrl Pts',(3.66105597228307,-17.8738591764567,
92.3881663174479));
#107555=CARTESIAN_POINT('Ctrl Pts',(3.72371374321079,-17.8832418308994,
92.394911970258));
#107556=CARTESIAN_POINT('Ctrl Pts',(3.78901989206686,-17.8931014191951,
92.4013404584845));
#107557=CARTESIAN_POINT('Ctrl Pts',(3.85701405172134,-17.9033669342938,
92.4073040728435));
#107558=CARTESIAN_POINT('Ctrl Pts',(3.92249284713516,-17.9132526886935,
92.4130470702793));
#107559=CARTESIAN_POINT('Ctrl Pts',(3.99046428990993,-17.9235147273393,
92.4183593456255));
#107560=CARTESIAN_POINT('Ctrl Pts',(4.06094707366189,-17.9340966321926,
92.4230648892938));
#107561=CARTESIAN_POINT('Ctrl Pts',(4.12765142717222,-17.9441112639164,
92.4275181789001));
#107562=CARTESIAN_POINT('Ctrl Pts',(4.19660487502362,-17.9544123001695,
92.4314283106798));
#107563=CARTESIAN_POINT('Ctrl Pts',(4.2678107284946,-17.9649600297792,92.4346013919948));
#107564=CARTESIAN_POINT('Ctrl Pts',(4.28593821212532,-17.967645255593,92.4354091904663));
#107565=CARTESIAN_POINT('Ctrl Pts',(4.30421161719959,-17.9703465160244,
92.4361689716465));
#107566=CARTESIAN_POINT('Ctrl Pts',(4.3226308844424,-17.9730632553954,92.4368770012617));
#107567=CARTESIAN_POINT('Ctrl Pts',(4.39257963099959,-17.9833803060804,
92.4395658044295));
#107568=CARTESIAN_POINT('Ctrl Pts',(4.46463198547307,-17.9939194501827,
92.4415119953763));
#107569=CARTESIAN_POINT('Ctrl Pts',(4.53880237008988,-18.0046684519818,
92.4424903462829));
#107570=CARTESIAN_POINT('Ctrl Pts',(4.60912854064787,-18.0148603383764,
92.4434179897498));
#107571=CARTESIAN_POINT('Ctrl Pts',(4.68135875542199,-18.0252409159418,
92.443475716865));
#107572=CARTESIAN_POINT('Ctrl Pts',(4.75550555857239,-18.0358125205007,
92.4424264461874));
#107573=CARTESIAN_POINT('Ctrl Pts',(4.7858295892246,-18.0401360199243,92.4419973229503));
#107574=CARTESIAN_POINT('Ctrl Pts',(4.81647419910139,-18.0444916218126,
92.4413824851498));
#107575=CARTESIAN_POINT('Ctrl Pts',(4.84744032554683,-18.0488801253806,
92.4405632308584));
#107576=CARTESIAN_POINT('Origin',(-2.58407189360391,-17.,89.45612065267));
#107577=CARTESIAN_POINT('',(-2.84482658273101,-17.,87.9789588497187));
#107578=CARTESIAN_POINT('Ctrl Pts',(-2.844826582731,-17.,87.9789588497187));
#107579=CARTESIAN_POINT('Ctrl Pts',(-2.84474020216979,-17.0600615703758,
87.9789436014661));
#107580=CARTESIAN_POINT('Ctrl Pts',(-2.8440475178467,-17.1201226165087,
87.9824888876553));
#107581=CARTESIAN_POINT('Ctrl Pts',(-2.84275231695818,-17.1797509891795,
87.9895689077724));
#107582=CARTESIAN_POINT('Ctrl Pts',(-2.84145949696887,-17.2392697501704,
87.9966359130634));
#107583=CARTESIAN_POINT('Ctrl Pts',(-2.8395666208452,-17.2983570253343,
88.0072246503357));
#107584=CARTESIAN_POINT('Ctrl Pts',(-2.83708086449162,-17.3565891473593,
88.0212580666932));
#107585=CARTESIAN_POINT('Ctrl Pts',(-2.83460337899347,-17.4146275136843,
88.0352447896741));
#107586=CARTESIAN_POINT('Ctrl Pts',(-2.83153717694925,-17.4718160252179,
88.0526532298416));
#107587=CARTESIAN_POINT('Ctrl Pts',(-2.82788921019877,-17.5277471632685,
88.0733567365258));
#107588=CARTESIAN_POINT('Ctrl Pts',(-2.82687791655771,-17.543252459264,
88.0790961870442));
#107589=CARTESIAN_POINT('Ctrl Pts',(-2.82582190161409,-17.5586612136524,
88.085088574193));
#107590=CARTESIAN_POINT('Ctrl Pts',(-2.82472127710851,-17.5739649677497,
88.0913305259417));
#107591=CARTESIAN_POINT('Ctrl Pts',(-2.82093444903734,-17.6266193338087,
88.1128066951359));
#107592=CARTESIAN_POINT('Ctrl Pts',(-2.81659341444049,-17.67802873488,88.1372352251746));
#107593=CARTESIAN_POINT('Ctrl Pts',(-2.81176864354748,-17.727860714738,
88.1644655245471));
#107594=CARTESIAN_POINT('Ctrl Pts',(-2.80704684540288,-17.7766291547849,
88.1911146608284));
#107595=CARTESIAN_POINT('Ctrl Pts',(-2.80186227329621,-17.8238866061767,
88.2204471003098));
#107596=CARTESIAN_POINT('Ctrl Pts',(-2.79625730851192,-17.8693397954361,
88.2522827608542));
#107597=CARTESIAN_POINT('Ctrl Pts',(-2.79079275113092,-17.9136543576889,
88.2833209208611));
#107598=CARTESIAN_POINT('Ctrl Pts',(-2.78492891390007,-17.9562537995739,
88.3167382778251));
#107599=CARTESIAN_POINT('Ctrl Pts',(-2.77867621237408,-17.996886142221,
88.3523330016412));
#107600=CARTESIAN_POINT('Ctrl Pts',(-2.7753205860046,-18.0186922303374,
88.3714355596884));
#107601=CARTESIAN_POINT('Ctrl Pts',(-2.77185243299703,-18.0399321213815,
88.391164640377));
#107602=CARTESIAN_POINT('Ctrl Pts',(-2.76826940460755,-18.0605694879468,
88.4114850041416));
#107603=CARTESIAN_POINT('Ctrl Pts',(-2.76382050087944,-18.0861940845367,
88.4367159909722));
#107604=CARTESIAN_POINT('Ctrl Pts',(-2.75906875878666,-18.1108870680876,
88.4628338346189));
#107605=CARTESIAN_POINT('Ctrl Pts',(-2.75415514434749,-18.134586226575,
88.4897947333846));
#107606=CARTESIAN_POINT('Ctrl Pts',(-2.74937681705425,-18.1576328732399,
88.5160133144347));
#107607=CARTESIAN_POINT('Ctrl Pts',(-2.74444561035497,-18.1797396741942,
88.543029197706));
#107608=CARTESIAN_POINT('Ctrl Pts',(-2.739443581773,-18.2008531725149,88.5707894736323));
#107609=CARTESIAN_POINT('Ctrl Pts',(-2.73457786914399,-18.2213912829511,
88.5977932228004));
#107610=CARTESIAN_POINT('Ctrl Pts',(-2.72964521534768,-18.2409894988228,
88.6255013502613));
#107611=CARTESIAN_POINT('Ctrl Pts',(-2.72467353158546,-18.2596021255553,
88.6538528266334));
#107612=CARTESIAN_POINT('Ctrl Pts',(-2.71975273425192,-18.2780242473909,
88.6819141185429));
#107613=CARTESIAN_POINT('Ctrl Pts',(-2.71479380706206,-18.2954808490119,
88.7106057229541));
#107614=CARTESIAN_POINT('Ctrl Pts',(-2.70977500459608,-18.3119311025169,
88.7398556806549));
#107615=CARTESIAN_POINT('Ctrl Pts',(-2.70480151656836,-18.3282328277619,
88.7688415424062));
#107616=CARTESIAN_POINT('Ctrl Pts',(-2.69976924048947,-18.3435462913634,
88.7983758543922));
#107617=CARTESIAN_POINT('Ctrl Pts',(-2.69460795995078,-18.3578352494326,
88.82837451494));
#107618=CARTESIAN_POINT('Ctrl Pts',(-2.69107233906138,-18.3676235835986,
88.8489244327543));
#107619=CARTESIAN_POINT('Ctrl Pts',(-2.68747515275225,-18.3769312270556,
88.8696919758207));
#107620=CARTESIAN_POINT('Ctrl Pts',(-2.68378046657837,-18.3857475041723,
88.890645582348));
#107621=CARTESIAN_POINT('Ctrl Pts',(-2.68068893666533,-18.3931245270492,
88.9081785197387));
#107622=CARTESIAN_POINT('Ctrl Pts',(-2.67751265990192,-18.4001570894256,
88.9258375172323));
#107623=CARTESIAN_POINT('Ctrl Pts',(-2.67432824416882,-18.406841537776,
88.9436260880443));
#107624=CARTESIAN_POINT('Ctrl Pts',(-2.67115577032227,-18.4135009187574,
88.961347949886));
#107625=CARTESIAN_POINT('Ctrl Pts',(-2.66797525212034,-18.4198147923675,
88.9791984837008));
#107626=CARTESIAN_POINT('Ctrl Pts',(-2.66481204782588,-18.4257790286698,
88.9971705585405));
#107627=CARTESIAN_POINT('Ctrl Pts',(-2.66165739729203,-18.4317271368171,
89.0150940342978));
#107628=CARTESIAN_POINT('Ctrl Pts',(-2.65851995839964,-18.4373274958245,
89.0331385181964));
#107629=CARTESIAN_POINT('Ctrl Pts',(-2.65537445049633,-18.4425754901149,
89.0512850061412));
#107630=CARTESIAN_POINT('Ctrl Pts',(-2.65256394272583,-18.4472645671053,
89.0674988726912));
#107631=CARTESIAN_POINT('Ctrl Pts',(-2.64974628004101,-18.4516723293873,
89.0837941498156));
#107632=CARTESIAN_POINT('Ctrl Pts',(-2.64686962412422,-18.455795140746,
89.100147404768));
#107633=CARTESIAN_POINT('Ctrl Pts',(-2.64475583480513,-18.458824614853,
89.1121639047076));
#107634=CARTESIAN_POINT('Ctrl Pts',(-2.64259558971588,-18.4616999411796,
89.124207642478));
#107635=CARTESIAN_POINT('Ctrl Pts',(-2.64044693112396,-18.4644212918646,
89.1362892360171));
#107636=CARTESIAN_POINT('Ctrl Pts',(-2.63829611592801,-18.4671453739635,
89.1483829558259));
#107637=CARTESIAN_POINT('Ctrl Pts',(-2.63615687923395,-18.4697151704312,
89.1605147188521));
#107638=CARTESIAN_POINT('Ctrl Pts',(-2.63403658004556,-18.4721299785418,
89.1726830821413));
#107639=CARTESIAN_POINT('Ctrl Pts',(-2.63190762092946,-18.4745546494416,
89.1849011446178));
#107640=CARTESIAN_POINT('Ctrl Pts',(-2.6297976686,-18.4768230613495,89.1971563476236));
#107641=CARTESIAN_POINT('Ctrl Pts',(-2.62766371298307,-18.4789336396701,
89.2094325039168));
#107642=CARTESIAN_POINT('Ctrl Pts',(-2.62709742376013,-18.4794937252444,
89.2126902356863));
#107643=CARTESIAN_POINT('Ctrl Pts',(-2.62652917481738,-18.4800426913482,
89.2159493503241));
#107644=CARTESIAN_POINT('Ctrl Pts',(-2.62595758703253,-18.480580498822,
89.2192093291882));
#107645=CARTESIAN_POINT('Ctrl Pts',(-2.62462385353926,-18.4818354098958,
89.2268161100078));
#107646=CARTESIAN_POINT('Ctrl Pts',(-2.62318817961284,-18.4830281746304,
89.2344037695635));
#107647=CARTESIAN_POINT('Ctrl Pts',(-2.6217508037341,-18.4841603604451,
89.2419984347316));
#107648=CARTESIAN_POINT('Ctrl Pts',(-2.62026232970538,-18.4853327950224,
89.2498630872742));
#107649=CARTESIAN_POINT('Ctrl Pts',(-2.61877225546264,-18.4864402702817,
89.2577354084537));
#107650=CARTESIAN_POINT('Ctrl Pts',(-2.61733491242798,-18.4874835549421,
89.2656311638377));
#107651=CARTESIAN_POINT('Ctrl Pts',(-2.61591966620904,-18.4885108007945,
89.273405534801));
#107652=CARTESIAN_POINT('Ctrl Pts',(-2.61455522039739,-18.4894758080587,
89.2812026800263));
#107653=CARTESIAN_POINT('Ctrl Pts',(-2.61324055925401,-18.4903784200692,
89.2890238126748));
#107654=CARTESIAN_POINT('Ctrl Pts',(-2.61189237703854,-18.4913040467724,
89.2970443676251));
#107655=CARTESIAN_POINT('Ctrl Pts',(-2.61059639061934,-18.492164050674,
89.3050905346638));
#107656=CARTESIAN_POINT('Ctrl Pts',(-2.60929846758452,-18.4929573944076,
89.3131456952514));
#107657=CARTESIAN_POINT('Ctrl Pts',(-2.60800580401295,-18.4937475233419,
89.3211682145961));
#107658=CARTESIAN_POINT('Ctrl Pts',(-2.60671047140018,-18.4944715129502,
89.3292003116569));
#107659=CARTESIAN_POINT('Ctrl Pts',(-2.6053141106307,-18.4951276644591,
89.3372003634645));
#107660=CARTESIAN_POINT('Ctrl Pts',(-2.60359036706128,-18.495937653517,
89.3470760618941));
#107661=CARTESIAN_POINT('Ctrl Pts',(-2.60208835986755,-18.4966913730579,
89.3576070931148));
#107662=CARTESIAN_POINT('Ctrl Pts',(-2.60052610129894,-18.4973293747359,
89.3681774744119));
#107663=CARTESIAN_POINT('Ctrl Pts',(-2.59959542101573,-18.4977094498363,
89.3744745405039));
#107664=CARTESIAN_POINT('Ctrl Pts',(-2.5986409882585,-18.4980492903023,
89.3807838546492));
#107665=CARTESIAN_POINT('Ctrl Pts',(-2.59762776174937,-18.4983445857785,
89.386984983822));
#107666=CARTESIAN_POINT('Ctrl Pts',(-2.5967439113196,-18.4986021757953,
89.3923943080305));
#107667=CARTESIAN_POINT('Ctrl Pts',(-2.59581530167916,-18.4988259903366,
89.3977200824184));
#107668=CARTESIAN_POINT('Ctrl Pts',(-2.59485026613534,-18.4990170956462,
89.4029081198794));
#107669=CARTESIAN_POINT('Ctrl Pts',(-2.59397531173422,-18.4991903622505,
89.4076118805221));
#107670=CARTESIAN_POINT('Ctrl Pts',(-2.59307121798518,-18.4993368371467,
89.4122014131159));
#107671=CARTESIAN_POINT('Ctrl Pts',(-2.59216621619928,-18.4994593854841,
89.4166740656765));
#107672=CARTESIAN_POINT('Ctrl Pts',(-2.5913496748404,-18.4995699551951,
89.4207095337347));
#107673=CARTESIAN_POINT('Ctrl Pts',(-2.59053363947096,-18.4996611364727,
89.4246494796461));
#107674=CARTESIAN_POINT('Ctrl Pts',(-2.58974341667261,-18.4997355651259,
89.4285331822771));
#107675=CARTESIAN_POINT('Ctrl Pts',(-2.58900398229582,-18.4998052101739,
89.4321672753968));
#107676=CARTESIAN_POINT('Ctrl Pts',(-2.58828859201009,-18.4998602719844,
89.4357520928298));
#107677=CARTESIAN_POINT('Ctrl Pts',(-2.58760355029172,-18.49990220908,89.4393608615583));
#107678=CARTESIAN_POINT('Ctrl Pts',(-2.58698361203457,-18.4999401606517,
89.4426266682034));
#107679=CARTESIAN_POINT('Ctrl Pts',(-2.58638959666555,-18.4999674238679,
89.4459127838703));
#107680=CARTESIAN_POINT('Ctrl Pts',(-2.58579704771983,-18.4999835144342,
89.4493030087189));
#107681=CARTESIAN_POINT('Ctrl Pts',(-2.5854174500935,-18.4999938223434,
89.4514748483864));
#107682=CARTESIAN_POINT('Ctrl Pts',(-2.58503785322051,-18.4999995129327,
89.4536900404362));
#107683=CARTESIAN_POINT('Ctrl Pts',(-2.58464131998469,-18.4999998848776,
89.455975322342));
#107684=CARTESIAN_POINT('Ctrl Pts',(-2.844826582731,-17.,87.9789588497187));
#107685=CARTESIAN_POINT('Ctrl Pts',(-2.90394614502961,-17.0023824172101,
87.9893948784988));
#107686=CARTESIAN_POINT('Ctrl Pts',(-2.96243772530833,-17.0047618946116,
88.0033899799603));
#107687=CARTESIAN_POINT('Ctrl Pts',(-3.01987982764382,-17.0071215359131,
88.0208434221831));
#107688=CARTESIAN_POINT('Ctrl Pts',(-3.07731807936984,-17.009481019037,
88.038295694421));
#107689=CARTESIAN_POINT('Ctrl Pts',(-3.1337065942239,-17.0118206522327,
88.0592057220766));
#107690=CARTESIAN_POINT('Ctrl Pts',(-3.18863907715103,-17.0141237898126,
88.0834229295207));
#107691=CARTESIAN_POINT('Ctrl Pts',(-3.24358165494329,-17.016427350637,
88.107644587327));
#107692=CARTESIAN_POINT('Ctrl Pts',(-3.2970672824039,-17.0186943862732,
88.1351744735706));
#107693=CARTESIAN_POINT('Ctrl Pts',(-3.34871044104395,-17.0209087342735,
88.1658142097659));
#107694=CARTESIAN_POINT('Ctrl Pts',(-3.40034592654931,-17.0231227532662,
88.1964493935126));
#107695=CARTESIAN_POINT('Ctrl Pts',(-3.45013913187528,-17.0252840847486,
88.2301932888778));
#107696=CARTESIAN_POINT('Ctrl Pts',(-3.49773127128024,-17.0273773035317,
88.2668027705058));
#107697=CARTESIAN_POINT('Ctrl Pts',(-3.54532853070358,-17.0294707475058,
88.303416190625));
#107698=CARTESIAN_POINT('Ctrl Pts',(-3.59072391869511,-17.0314960493733,
88.3428955594524));
#107699=CARTESIAN_POINT('Ctrl Pts',(-3.63359028942193,-17.0334387366064,
88.3849563386015));
#107700=CARTESIAN_POINT('Ctrl Pts',(-3.66571876688184,-17.0348947866971,
88.416481022682));
#107701=CARTESIAN_POINT('Ctrl Pts',(-3.69642718496859,-17.0363044461387,
88.4494549470133));
#107702=CARTESIAN_POINT('Ctrl Pts',(-3.72559111921561,-17.0376620472082,
88.4837444766152));
#107703=CARTESIAN_POINT('Ctrl Pts',(-3.76450732905361,-17.0394736233711,
88.5295002555828));
#107704=CARTESIAN_POINT('Ctrl Pts',(-3.80067189167083,-17.0411925807839,
88.5775997590202));
#107705=CARTESIAN_POINT('Ctrl Pts',(-3.83382415408655,-17.0428068444602,
88.6276963281322));
#107706=CARTESIAN_POINT('Ctrl Pts',(-3.86697445142636,-17.0444210124521,
88.677789927807));
#107707=CARTESIAN_POINT('Ctrl Pts',(-3.89711257570302,-17.045930487707,
88.7298800079881));
#107708=CARTESIAN_POINT('Ctrl Pts',(-3.92402133297399,-17.0473246982119,
88.7835911939316));
#107709=CARTESIAN_POINT('Ctrl Pts',(-3.950935205338,-17.0487191737428,88.8373125898491));
#107710=CARTESIAN_POINT('Ctrl Pts',(-3.97461829425342,-17.0499983307383,
88.8926553351392));
#107711=CARTESIAN_POINT('Ctrl Pts',(-3.9948998575191,-17.0511532531476,
88.9492204643416));
#107712=CARTESIAN_POINT('Ctrl Pts',(-4.01517844818267,-17.0523080062837,
89.0057773029788));
#107713=CARTESIAN_POINT('Ctrl Pts',(-4.03205637045371,-17.0533385530554,
89.0635557736215));
#107714=CARTESIAN_POINT('Ctrl Pts',(-4.04541197564839,-17.0542377788039,
89.1221394736184));
#107715=CARTESIAN_POINT('Ctrl Pts',(-4.05876899438231,-17.0551370997252,
89.1807293740352));
#107716=CARTESIAN_POINT('Ctrl Pts',(-4.06860285666184,-17.05590506534,89.2401242671352));
#107717=CARTESIAN_POINT('Ctrl Pts',(-4.07484266374113,-17.0565364670105,
89.2998960105598));
#107718=CARTESIAN_POINT('Ctrl Pts',(-4.07951153127009,-17.0570089064177,
89.3446195650669));
#107719=CARTESIAN_POINT('Ctrl Pts',(-4.08216927023329,-17.057404927918,
89.3895538271932));
#107720=CARTESIAN_POINT('Ctrl Pts',(-4.0828051389793,-17.0577230769003,
89.4345172825691));
#107721=CARTESIAN_POINT('Ctrl Pts',(-4.08365488216529,-17.0581482352863,
89.4946041952602));
#107722=CARTESIAN_POINT('Ctrl Pts',(-4.08089198932617,-17.0584343992759,
89.5547429724985));
#107723=CARTESIAN_POINT('Ctrl Pts',(-4.0745363644185,-17.058579722477,89.6145001884501));
#107724=CARTESIAN_POINT('Ctrl Pts',(-4.06818111413334,-17.0587250371122,
89.6742538821047));
#107725=CARTESIAN_POINT('Ctrl Pts',(-4.05823359998992,-17.0587295264416,
89.7336256442276));
#107726=CARTESIAN_POINT('Ctrl Pts',(-4.04476549631919,-17.0585934095053,
89.7921876271694));
#107727=CARTESIAN_POINT('Ctrl Pts',(-4.03129482724969,-17.0584572666415,
89.8507607649733));
#107728=CARTESIAN_POINT('Ctrl Pts',(-4.01430231938096,-17.0581804647287,
89.9085234074744));
#107729=CARTESIAN_POINT('Ctrl Pts',(-3.99391045981778,-17.0577652915182,
89.9650591443483));
#107730=CARTESIAN_POINT('Ctrl Pts',(-3.97352158583064,-17.0573501790932,
90.0215866038142));
#107731=CARTESIAN_POINT('Ctrl Pts',(-3.94973449841905,-17.056796738769,
90.0768871243478));
#107732=CARTESIAN_POINT('Ctrl Pts',(-3.92272061459661,-17.0561092973433,
90.1305621612801));
#107733=CARTESIAN_POINT('Ctrl Pts',(-3.89570386870406,-17.0554217830845,
90.1842428849814));
#107734=CARTESIAN_POINT('Ctrl Pts',(-3.86545982963037,-17.0546002440683,
90.2362974070196));
#107735=CARTESIAN_POINT('Ctrl Pts',(-3.83220649265228,-17.0536509920008,
90.2863504965781));
#107736=CARTESIAN_POINT('Ctrl Pts',(-3.80732503994394,-17.0529407243233,
90.3238021839554));
#107737=CARTESIAN_POINT('Ctrl Pts',(-3.78075977716049,-17.052158996523,
90.3601337988618));
#107738=CARTESIAN_POINT('Ctrl Pts',(-3.75261800855695,-17.0513091504894,
90.3951985771812));
#107739=CARTESIAN_POINT('Ctrl Pts',(-3.7150919602065,-17.0501759110048,
90.4419562129626));
#107740=CARTESIAN_POINT('Ctrl Pts',(-3.6747602537301,-17.0489215300774,
90.4864612103411));
#107741=CARTESIAN_POINT('Ctrl Pts',(-3.63191259383891,-17.0475550414524,
90.5283931856407));
#107742=CARTESIAN_POINT('Ctrl Pts',(-3.58906842455738,-17.0461886641492,
90.5703217449275));
#107743=CARTESIAN_POINT('Ctrl Pts',(-3.54370901311723,-17.044710207171,
90.6096774060446));
#107744=CARTESIAN_POINT('Ctrl Pts',(-3.49616044245401,-17.0431303861969,
90.6461770584101));
#107745=CARTESIAN_POINT('Ctrl Pts',(-3.44860185021139,-17.0415502322517,
90.6826844036286));
#107746=CARTESIAN_POINT('Ctrl Pts',(-3.39885350965945,-17.0398686828611,
90.7163342776236));
#107747=CARTESIAN_POINT('Ctrl Pts',(-3.34727340964406,-17.0380979875471,
90.7468847632878));
#107748=CARTESIAN_POINT('Ctrl Pts',(-3.29569951794632,-17.0363275053587,
90.7774315718144));
#107749=CARTESIAN_POINT('Ctrl Pts',(-3.24229467194259,-17.0344679114925,
90.8048795248662));
#107750=CARTESIAN_POINT('Ctrl Pts',(-3.187443176895,-17.0325327967545,90.8290316882564));
#107751=CARTESIAN_POINT('Ctrl Pts',(-3.13258096101438,-17.0305973037944,
90.8531885722347));
#107752=CARTESIAN_POINT('Ctrl Pts',(-3.07627191706294,-17.0285862743993,
90.8740482084431));
#107753=CARTESIAN_POINT('Ctrl Pts',(-3.01892139861794,-17.026514452939,
90.8914613410692));
#107754=CARTESIAN_POINT('Ctrl Pts',(-2.97530773108157,-17.0249388833572,
90.9047036028257));
#107755=CARTESIAN_POINT('Ctrl Pts',(-2.93109222531984,-17.0233281814062,
90.9159536361465));
#107756=CARTESIAN_POINT('Ctrl Pts',(-2.88645908594721,-17.0216891971845,
90.9251650919679));
#107757=CARTESIAN_POINT('Origin',(17.1910233941991,-17.,85.96920230149));
#107758=CARTESIAN_POINT('',(9.44018183429909,-17.,85.81274487387));
#107759=CARTESIAN_POINT('',(16.4933237498291,-18.49999999514,86.09223866229));
#107760=CARTESIAN_POINT('Origin',(157.369850611169,-18.5,67.852165916321));
#107761=CARTESIAN_POINT('Ctrl Pts',(4.96802222338909,-18.49999999899,91.37511854801));
#107762=CARTESIAN_POINT('Ctrl Pts',(5.22543100101909,-18.49999999899,91.40426861974));
#107763=CARTESIAN_POINT('Ctrl Pts',(5.75020154047909,-18.50000000047,91.46158478716));
#107764=CARTESIAN_POINT('Ctrl Pts',(6.50334881420368,-18.4999999999262,
91.5330830665222));
#107765=CARTESIAN_POINT('Ctrl Pts',(6.98169776546952,-18.4999999999567,
91.5705426281902));
#107766=CARTESIAN_POINT('Ctrl Pts',(7.18082331871055,-18.4999999999755,
91.584556528483));
#107767=CARTESIAN_POINT('Ctrl Pts',(4.67429866745909,-17.81329231081,92.6102332020699));
#107768=CARTESIAN_POINT('Ctrl Pts',(4.92175734799909,-17.81329231081,92.6386607895801));
#107769=CARTESIAN_POINT('Ctrl Pts',(5.44974328288909,-17.81329231081,92.69732199839));
#107770=CARTESIAN_POINT('Ctrl Pts',(6.26767800558908,-17.81329231081,92.77811241642));
#107771=CARTESIAN_POINT('Ctrl Pts',(7.12392866528909,-17.81329231081,92.8472667652099));
#107772=CARTESIAN_POINT('Ctrl Pts',(7.97259535655909,-17.81329231081,92.89672929314));
#107773=CARTESIAN_POINT('Ctrl Pts',(8.78502947769909,-17.81329231081,92.92332784864));
#107774=CARTESIAN_POINT('Ctrl Pts',(9.5332741592491,-17.81329231081,92.9279180420902));
#107775=CARTESIAN_POINT('Ctrl Pts',(10.2041285991891,-17.81329231081,92.9146854325099));
#107776=CARTESIAN_POINT('Ctrl Pts',(10.8004329265091,-17.81329231081,92.8886586089702));
#107777=CARTESIAN_POINT('Ctrl Pts',(11.3349840960491,-17.81329231081,92.8534030050999));
#107778=CARTESIAN_POINT('Ctrl Pts',(11.8178226086691,-17.81329231081,92.8116449801501));
#107779=CARTESIAN_POINT('Ctrl Pts',(12.2554929002391,-17.81329231081,92.7654341535601));
#107780=CARTESIAN_POINT('Ctrl Pts',(12.6533731109991,-17.81329231081,92.71641060703));
#107781=CARTESIAN_POINT('Ctrl Pts',(13.0164525305191,-17.81329231081,92.6657791293399));
#107782=CARTESIAN_POINT('Ctrl Pts',(13.3492734982491,-17.81329231081,92.61435605809));
#107783=CARTESIAN_POINT('Ctrl Pts',(13.6561665865191,-17.81329231081,92.56262780457));
#107784=CARTESIAN_POINT('Ctrl Pts',(13.9403800542091,-17.81329231081,92.51100282361));
#107785=CARTESIAN_POINT('Ctrl Pts',(14.2033497191691,-17.81329231081,92.46001789955));
#107786=CARTESIAN_POINT('Ctrl Pts',(14.4452961696591,-17.81329231081,92.41035496115));
#107787=CARTESIAN_POINT('Ctrl Pts',(14.6666699797891,-17.81329231081,92.36258963016));
#107788=CARTESIAN_POINT('Ctrl Pts',(14.8689728993491,-17.81329231081,92.31698073567));
#107789=CARTESIAN_POINT('Ctrl Pts',(15.0542645826791,-17.81329231081,92.2735532422199));
#107790=CARTESIAN_POINT('Ctrl Pts',(15.2253800918591,-17.81329231082,92.2320415865899));
#107791=CARTESIAN_POINT('Ctrl Pts',(15.3859455327891,-17.81329231077,92.1918578513101));
#107792=CARTESIAN_POINT('Ctrl Pts',(15.5409358917991,-17.81329231096,92.1519372765301));
#107793=CARTESIAN_POINT('Ctrl Pts',(15.6976425511091,-17.81329231023,92.1104475421901));
#107794=CARTESIAN_POINT('Ctrl Pts',(15.8618783881191,-17.81329231324,92.06573309792));
#107795=CARTESIAN_POINT('Ctrl Pts',(16.0323492246791,-17.81329230114,92.0179448915599));
#107796=CARTESIAN_POINT('Ctrl Pts',(16.1990043638691,-17.81329234446,91.96984383322));
#107797=CARTESIAN_POINT('Ctrl Pts',(16.3585633685591,-17.81329220026,91.9225113535201));
#107798=CARTESIAN_POINT('Ctrl Pts',(16.4564706533791,-17.81318796283,91.8929129181599));
#107799=CARTESIAN_POINT('Ctrl Pts',(16.5032491374491,-17.81308325173,91.8786745656599));
#107800=CARTESIAN_POINT('Ctrl Pts',(4.71381130773909,-18.34983158812,92.26627944992));
#107801=CARTESIAN_POINT('Ctrl Pts',(4.96040944056908,-18.34983158812,92.29460814837));
#107802=CARTESIAN_POINT('Ctrl Pts',(5.48608879843909,-18.34983158812,92.35301088002));
#107803=CARTESIAN_POINT('Ctrl Pts',(6.29888635805909,-18.34983158812,92.43328754518));
#107804=CARTESIAN_POINT('Ctrl Pts',(7.14817026536909,-18.34983158812,92.50187169504));
#107805=CARTESIAN_POINT('Ctrl Pts',(7.98856602530908,-18.34983158812,92.55084458026));
#107806=CARTESIAN_POINT('Ctrl Pts',(8.79196326731908,-18.34983158812,92.5771400222));
#107807=CARTESIAN_POINT('Ctrl Pts',(9.53108736363908,-18.34983158812,92.5816705939));
#107808=CARTESIAN_POINT('Ctrl Pts',(10.1933161338291,-18.34983158812,92.5686051930199));
#107809=CARTESIAN_POINT('Ctrl Pts',(10.7815791528391,-18.34983158812,92.54292787439));
#107810=CARTESIAN_POINT('Ctrl Pts',(11.3087547861991,-18.34983158812,92.50815797892));
#107811=CARTESIAN_POINT('Ctrl Pts',(11.7848039744491,-18.34983158812,92.46698641252));
#107812=CARTESIAN_POINT('Ctrl Pts',(12.2161926086191,-18.34983158812,92.42143843311));
#107813=CARTESIAN_POINT('Ctrl Pts',(12.6083398427691,-18.34983158812,92.37312122294));
#107814=CARTESIAN_POINT('Ctrl Pts',(12.9661518810891,-18.34983158812,92.32322406105));
#107815=CARTESIAN_POINT('Ctrl Pts',(13.2940991431591,-18.34983158812,92.27255390755));
#107816=CARTESIAN_POINT('Ctrl Pts',(13.5964793927291,-18.34983158812,92.22158628161));
#107817=CARTESIAN_POINT('Ctrl Pts',(13.8765160809191,-18.34983158812,92.17071999012));
#107818=CARTESIAN_POINT('Ctrl Pts',(14.1356179414191,-18.34983158812,92.12048494285));
#107819=CARTESIAN_POINT('Ctrl Pts',(14.3740019301191,-18.34983158812,92.07155324491));
#107820=CARTESIAN_POINT('Ctrl Pts',(14.5921111933091,-18.34983158812,92.02449226612));
#107821=CARTESIAN_POINT('Ctrl Pts',(14.7914186857591,-18.34983158812,91.9795586751801));
#107822=CARTESIAN_POINT('Ctrl Pts',(14.9739675871691,-18.34983158811,91.93677402423));
#107823=CARTESIAN_POINT('Ctrl Pts',(15.1425533262591,-18.34983158813,91.89587608238));
#107824=CARTESIAN_POINT('Ctrl Pts',(15.3007471565291,-18.34983158809,91.85628587938));
#107825=CARTESIAN_POINT('Ctrl Pts',(15.4534503714491,-18.34983158823,91.81695440386));
#107826=CARTESIAN_POINT('Ctrl Pts',(15.6078464560491,-18.34983158769,91.776076421));
#107827=CARTESIAN_POINT('Ctrl Pts',(15.7696623981791,-18.34983158988,91.73202081673));
#107828=CARTESIAN_POINT('Ctrl Pts',(15.9376211881691,-18.3498315811,91.6849367963501));
#107829=CARTESIAN_POINT('Ctrl Pts',(16.1018113089291,-18.34983161252,91.63754721276));
#107830=CARTESIAN_POINT('Ctrl Pts',(16.2588839577391,-18.34983150793,91.5909515159));
#107831=CARTESIAN_POINT('Ctrl Pts',(16.3563226329691,-18.34975599539,91.56154888587));
#107832=CARTESIAN_POINT('Ctrl Pts',(16.4034488759691,-18.34968013935,91.54726170511));
#107833=CARTESIAN_POINT('Ctrl Pts',(4.78098568915909,-18.59741772268,91.68153288839));
#107834=CARTESIAN_POINT('Ctrl Pts',(5.02612082787908,-18.59741772268,91.7096934681901));
#107835=CARTESIAN_POINT('Ctrl Pts',(5.54787883593908,-18.59741772268,91.76765676975));
#107836=CARTESIAN_POINT('Ctrl Pts',(6.35194284219909,-18.59741772268,91.84706001742));
#107837=CARTESIAN_POINT('Ctrl Pts',(7.18938276036909,-18.59741772268,91.91467478736));
#107838=CARTESIAN_POINT('Ctrl Pts',(8.01571733149909,-18.59741772268,91.9628152441));
#107839=CARTESIAN_POINT('Ctrl Pts',(8.80375121733909,-18.59741772268,91.98859537081));
#107840=CARTESIAN_POINT('Ctrl Pts',(9.52736965098908,-18.59741772268,91.99302458115));
#107841=CARTESIAN_POINT('Ctrl Pts',(10.1749341510891,-18.59741772268,91.98024344731));
#107842=CARTESIAN_POINT('Ctrl Pts',(10.7495263572191,-18.59741772268,91.95516031264));
#107843=CARTESIAN_POINT('Ctrl Pts',(11.2641630390591,-18.59741772268,91.921216157));
#107844=CARTESIAN_POINT('Ctrl Pts',(11.7286698787791,-18.59741772268,91.88104161308));
#107845=CARTESIAN_POINT('Ctrl Pts',(12.1493792354491,-18.59741772268,91.83662052239));
#107846=CARTESIAN_POINT('Ctrl Pts',(12.5317799896291,-18.59741772268,91.78950413574));
#107847=CARTESIAN_POINT('Ctrl Pts',(12.8806370942491,-18.59741772268,91.74085536449));
#107848=CARTESIAN_POINT('Ctrl Pts',(13.2002986998791,-18.59741772268,91.69146522629));
#107849=CARTESIAN_POINT('Ctrl Pts',(13.4950067932391,-18.59741772268,91.64179072293));
#107850=CARTESIAN_POINT('Ctrl Pts',(13.7679426504591,-18.59741772268,91.59221425908));
#107851=CARTESIAN_POINT('Ctrl Pts',(14.0204689601991,-18.59741772268,91.54325405724));
#107852=CARTESIAN_POINT('Ctrl Pts',(14.2527965030291,-18.59741772268,91.49556552163));
#107853=CARTESIAN_POINT('Ctrl Pts',(14.4653557974191,-18.59741772268,91.44970199315));
#107854=CARTESIAN_POINT('Ctrl Pts',(14.6595708444491,-18.59741772268,91.40591646769));
#107855=CARTESIAN_POINT('Ctrl Pts',(14.8374568157691,-18.59741772268,91.36422469606));
#107856=CARTESIAN_POINT('Ctrl Pts',(15.0017417605091,-18.59741772268,91.32437011257));
#107857=CARTESIAN_POINT('Ctrl Pts',(15.1559036790191,-18.59741772267,91.28578895791));
#107858=CARTESIAN_POINT('Ctrl Pts',(15.3047185815191,-18.59741772272,91.24745899426));
#107859=CARTESIAN_POINT('Ctrl Pts',(15.4551865199491,-18.59741772253,91.2076210337));
#107860=CARTESIAN_POINT('Ctrl Pts',(15.6128884636191,-18.5974177233,91.16468550567));
#107861=CARTESIAN_POINT('Ctrl Pts',(15.7765765905091,-18.59741772018,91.11879865301));
#107862=CARTESIAN_POINT('Ctrl Pts',(15.9365759994591,-18.59741773137,91.0726186286001));
#107863=CARTESIAN_POINT('Ctrl Pts',(16.0894216612391,-18.59741769412,91.0272755165199));
#107864=CARTESIAN_POINT('Ctrl Pts',(16.1860844388491,-18.59739084079,90.99814207378));
#107865=CARTESIAN_POINT('Ctrl Pts',(16.2338226818491,-18.59736386515,90.98370815039));
#107866=CARTESIAN_POINT('Ctrl Pts',(4.85238799116909,-18.46968015288,91.05998268273));
#107867=CARTESIAN_POINT('Ctrl Pts',(5.09596805569909,-18.46968015288,91.08796456258));
#107868=CARTESIAN_POINT('Ctrl Pts',(5.6135579062291,-18.46968015288,91.1454607765601));
#107869=CARTESIAN_POINT('Ctrl Pts',(6.40833867382909,-18.46968015288,91.22393563429));
#107870=CARTESIAN_POINT('Ctrl Pts',(7.2331891483591,-18.46968015288,91.2905200120401));
#107871=CARTESIAN_POINT('Ctrl Pts',(8.04457752675909,-18.46968015288,91.3377756476999));
#107872=CARTESIAN_POINT('Ctrl Pts',(8.81628109478909,-18.46968015288,91.3630080254999));
#107873=CARTESIAN_POINT('Ctrl Pts',(9.52341794744909,-18.46968015288,91.36732949485));
#107874=CARTESIAN_POINT('Ctrl Pts',(10.1553952159191,-18.46968015288,91.3548505196701));
#107875=CARTESIAN_POINT('Ctrl Pts',(10.7154561753291,-18.46968015288,91.33039896658));
#107876=CARTESIAN_POINT('Ctrl Pts',(11.2167647105691,-18.46968015288,91.2973325223999));
#107877=CARTESIAN_POINT('Ctrl Pts',(11.6690027323691,-18.46968015288,91.2582177530301));
#107878=CARTESIAN_POINT('Ctrl Pts',(12.0783606633591,-18.46968015288,91.21499447685));
#107879=CARTESIAN_POINT('Ctrl Pts',(12.4504014991991,-18.46968015288,91.16915449294));
#107880=CARTESIAN_POINT('Ctrl Pts',(12.7897400512391,-18.46968015288,91.12183268539));
#107881=CARTESIAN_POINT('Ctrl Pts',(13.1005945055291,-18.46968015288,91.0738031259901));
#107882=CARTESIAN_POINT('Ctrl Pts',(13.3871475611691,-18.46968015288,91.02550313366));
#107883=CARTESIAN_POINT('Ctrl Pts',(13.6525356648191,-18.46968015288,90.97729767853));
#107884=CARTESIAN_POINT('Ctrl Pts',(13.8980725620591,-18.46968015288,90.92969256024));
#107885=CARTESIAN_POINT('Ctrl Pts',(14.1239624694591,-18.46968015288,90.88332543094));
#107886=CARTESIAN_POINT('Ctrl Pts',(14.3306224828991,-18.46968015288,90.83873471968));
#107887=CARTESIAN_POINT('Ctrl Pts',(14.5194245686591,-18.46968015288,90.79616951834));
#107888=CARTESIAN_POINT('Ctrl Pts',(14.6923541275091,-18.46968015288,90.75563941128));
#107889=CARTESIAN_POINT('Ctrl Pts',(14.8520675881291,-18.46968015288,90.71689385458));
#107890=CARTESIAN_POINT('Ctrl Pts',(15.0019438284491,-18.46968015289,90.6793852572301));
#107891=CARTESIAN_POINT('Ctrl Pts',(15.1466256901691,-18.46968015285,90.6421198401));
#107892=CARTESIAN_POINT('Ctrl Pts',(15.2929182469491,-18.46968015302,90.6033873603001));
#107893=CARTESIAN_POINT('Ctrl Pts',(15.4462472592391,-18.4696801523,90.56164240552));
#107894=CARTESIAN_POINT('Ctrl Pts',(15.6053959297191,-18.46968015519,90.5170280697));
#107895=CARTESIAN_POINT('Ctrl Pts',(15.7609408656491,-18.46968014487,90.47213373348));
#107896=CARTESIAN_POINT('Ctrl Pts',(15.9092934960191,-18.4696801792,90.42812204322));
#107897=CARTESIAN_POINT('Ctrl Pts',(16.0051437602991,-18.46970494463,90.39923726359));
#107898=CARTESIAN_POINT('Ctrl Pts',(16.0535447478491,-18.46972982279,90.38460987447));
#107899=CARTESIAN_POINT('Ctrl Pts',(4.84743272606783,-18.0489462436203,
92.4406303885482));
#107900=CARTESIAN_POINT('Ctrl Pts',(5.03040185937532,-18.0650463395508,
92.4454996674276));
#107901=CARTESIAN_POINT('Ctrl Pts',(5.2085737446796,-18.0803746691731,92.4493084336499));
#107902=CARTESIAN_POINT('Ctrl Pts',(5.38188039330711,-18.0949545072779,
92.4520603727252));
#107903=CARTESIAN_POINT('Ctrl Pts',(5.4026891322958,-18.0967050924287,92.452390795028));
#107904=CARTESIAN_POINT('Ctrl Pts',(5.42342773905644,-18.0984448968291,
92.4527060415585));
#107905=CARTESIAN_POINT('Ctrl Pts',(5.44409610243779,-18.1001739686197,
92.4530061664326));
#107906=CARTESIAN_POINT('Ctrl Pts',(5.62803093192004,-18.1155615694235,
92.4556770802594));
#107907=CARTESIAN_POINT('Ctrl Pts',(5.80640080237462,-18.1300984623534,
92.4571460825411));
#107908=CARTESIAN_POINT('Ctrl Pts',(5.97911713546014,-18.1438235369843,
92.4574880960229));
#107909=CARTESIAN_POINT('Ctrl Pts',(6.08580373840904,-18.1523014936513,
92.4576993572041));
#107910=CARTESIAN_POINT('Ctrl Pts',(6.19033366455821,-18.1604698783647,
92.4574816912358));
#107911=CARTESIAN_POINT('Ctrl Pts',(6.29268999604011,-18.1683392495622,
92.4568615559032));
#107912=CARTESIAN_POINT('Ctrl Pts',(6.44065786997315,-18.1797153325893,
92.4559650788082));
#107913=CARTESIAN_POINT('Ctrl Pts',(6.58408260085334,-18.1904664472246,
92.4542269470687));
#107914=CARTESIAN_POINT('Ctrl Pts',(6.72291626644099,-18.2006273153123,
92.4517518039631));
#107915=CARTESIAN_POINT('Ctrl Pts',(20.3703076195591,-17.48636025246,80.6160118299));
#107916=CARTESIAN_POINT('Ctrl Pts',(20.1881103583291,-17.59469264276,81.383197007755));
#107917=CARTESIAN_POINT('Ctrl Pts',(19.7633142133291,-17.81559800981,82.9726719728399));
#107918=CARTESIAN_POINT('Ctrl Pts',(19.0018167096191,-18.10372872761,85.2475673257499));
#107919=CARTESIAN_POINT('Ctrl Pts',(18.1317679720991,-18.32477803286,87.36843783982));
#107920=CARTESIAN_POINT('Ctrl Pts',(17.2370610827991,-18.45951303147,89.2032198305499));
#107921=CARTESIAN_POINT('Ctrl Pts',(16.3494952333791,-18.51446227549,90.7700178089799));
#107922=CARTESIAN_POINT('Ctrl Pts',(15.4867758268391,-18.50123398135,92.10529605495));
#107923=CARTESIAN_POINT('Ctrl Pts',(14.6453959780491,-18.43037008788,93.26267617499));
#107924=CARTESIAN_POINT('Ctrl Pts',(13.8009845953991,-18.30490819777,94.3025568640399));
#107925=CARTESIAN_POINT('Ctrl Pts',(12.9307100320291,-18.12021817286,95.2628709280001));
#107926=CARTESIAN_POINT('Ctrl Pts',(12.0275979803391,-17.86955305763,96.15310194351));
#107927=CARTESIAN_POINT('Ctrl Pts',(11.1010176724691,-17.54986176095,96.96608256951));
#107928=CARTESIAN_POINT('Ctrl Pts',(10.1635981391591,-17.16111541643,97.6955323958101));
#107929=CARTESIAN_POINT('Ctrl Pts',(9.27968364505908,-16.73052720888,98.30286534269));
#107930=CARTESIAN_POINT('Ctrl Pts',(8.71271538374908,-16.41504543997,98.64913661867));
#107931=CARTESIAN_POINT('Ctrl Pts',(8.45819912877909,-16.26514131694,98.79644286584));
#107932=CARTESIAN_POINT('Ctrl Pts',(14.7248846521991,-18.94108804276,77.911688731006));
#107933=CARTESIAN_POINT('Ctrl Pts',(14.5694350031491,-18.93552267139,78.561742613804));
#107934=CARTESIAN_POINT('Ctrl Pts',(14.2134049487491,-18.91245218656,79.908309787637));
#107935=CARTESIAN_POINT('Ctrl Pts',(13.6004443439491,-18.832257487,81.827642780919));
#107936=CARTESIAN_POINT('Ctrl Pts',(12.9289464995691,-18.69869734538,83.60280410874));
#107937=CARTESIAN_POINT('Ctrl Pts',(12.2646619608891,-18.52485132822,85.12309497776));
#107938=CARTESIAN_POINT('Ctrl Pts',(11.6278705382591,-18.32183553005,86.4073429830001));
#107939=CARTESIAN_POINT('Ctrl Pts',(11.0263774792591,-18.09933417041,87.4904580833699));
#107940=CARTESIAN_POINT('Ctrl Pts',(10.4529512601791,-17.86094059021,88.4205103504401));
#107941=CARTESIAN_POINT('Ctrl Pts',(9.88731078157909,-17.60178133109,89.249386304));
#107942=CARTESIAN_POINT('Ctrl Pts',(9.31126387016909,-17.31409529898,90.0096973799401));
#107943=CARTESIAN_POINT('Ctrl Pts',(8.71693645522909,-16.9926399648,90.7110627126001));
#107944=CARTESIAN_POINT('Ctrl Pts',(8.10624510203909,-16.63664836235,91.35001588189));
#107945=CARTESIAN_POINT('Ctrl Pts',(7.48260991328909,-16.24618559887,91.92364883475));
#107946=CARTESIAN_POINT('Ctrl Pts',(6.88447228887909,-15.84456366131,92.40307208249));
#107947=CARTESIAN_POINT('Ctrl Pts',(6.49233429628909,-15.56370842049,92.67816808986));
#107948=CARTESIAN_POINT('Ctrl Pts',(6.31420645011909,-15.43222415467,92.79562051845));
#107949=CARTESIAN_POINT('Ctrl Pts',(12.5063401363191,-24.60762905604,75.845594438731));
#107950=CARTESIAN_POINT('Ctrl Pts',(12.2868497584891,-24.55389093248,76.4322774261809));
#107951=CARTESIAN_POINT('Ctrl Pts',(11.7948949593591,-24.42464703364,77.649532278307));
#107952=CARTESIAN_POINT('Ctrl Pts',(10.9814946228591,-24.17202064863,79.385448634424));
#107953=CARTESIAN_POINT('Ctrl Pts',(10.1222707621991,-23.85736527914,80.987352988331));
#107954=CARTESIAN_POINT('Ctrl Pts',(9.29846527963909,-23.5105055521,82.353880287081));
#107955=CARTESIAN_POINT('Ctrl Pts',(8.52998276490909,-23.14741348718,83.50305548649));
#107956=CARTESIAN_POINT('Ctrl Pts',(7.82085548590909,-22.77957706661,84.4682620618799));
#107957=CARTESIAN_POINT('Ctrl Pts',(7.15797738393909,-22.40870352106,85.2944825448601));
#107958=CARTESIAN_POINT('Ctrl Pts',(6.5147643722091,-22.02537234206,86.0295402695));
#107959=CARTESIAN_POINT('Ctrl Pts',(5.86851416204909,-21.61846160989,86.7038509520601));
#107960=CARTESIAN_POINT('Ctrl Pts',(5.20849832309909,-21.1819420503,87.32752168855));
#107961=CARTESIAN_POINT('Ctrl Pts',(4.53433886995909,-20.71577757791,87.89907590832));
#107962=CARTESIAN_POINT('Ctrl Pts',(3.84677854591909,-20.22008924508,88.41723900531));
#107963=CARTESIAN_POINT('Ctrl Pts',(3.18516755758909,-19.72283039656,88.85636793195));
#107964=CARTESIAN_POINT('Ctrl Pts',(2.74853368799909,-19.38098595465,89.11251172142));
#107965=CARTESIAN_POINT('Ctrl Pts',(2.54938093874909,-19.22185467038,89.22278927536));
#107966=CARTESIAN_POINT('Ctrl Pts',(15.3202955475791,-30.38495224307,75.913018023323));
#107967=CARTESIAN_POINT('Ctrl Pts',(14.9923241307591,-30.38363031797,76.535953769073));
#107968=CARTESIAN_POINT('Ctrl Pts',(14.2581262150091,-30.36285605286,77.831078640661));
#107969=CARTESIAN_POINT('Ctrl Pts',(13.0403732440191,-30.25848525137,79.688467729779));
#107970=CARTESIAN_POINT('Ctrl Pts',(11.7430089211191,-30.06731245317,81.414958143033));
#107971=CARTESIAN_POINT('Ctrl Pts',(10.4851888796891,-29.80822108623,82.899732333371));
#107972=CARTESIAN_POINT('Ctrl Pts',(9.29785820693909,-29.4987931119,84.15906778619));
#107973=CARTESIAN_POINT('Ctrl Pts',(8.19013397563909,-29.15474260213,85.2259540885799));
#107974=CARTESIAN_POINT('Ctrl Pts',(7.14513725765909,-28.78231819477,86.14698476448));
#107975=CARTESIAN_POINT('Ctrl Pts',(6.12414964407909,-28.37420716695,86.97330959057));
#107976=CARTESIAN_POINT('Ctrl Pts',(5.09407323602909,-27.91812922517,87.73786331633));
#107977=CARTESIAN_POINT('Ctrl Pts',(4.04143642525909,-27.40554656753,88.4512402521699));
#107978=CARTESIAN_POINT('Ctrl Pts',(2.97038542110909,-26.83507178681,89.11080249674));
#107979=CARTESIAN_POINT('Ctrl Pts',(1.88745485450909,-26.20680336296,89.71398781054));
#107980=CARTESIAN_POINT('Ctrl Pts',(0.859057681899087,-25.55851947637,90.2295998987501));
#107981=CARTESIAN_POINT('Ctrl Pts',(0.190804675379086,-25.10420966072,90.53273076058));
#107982=CARTESIAN_POINT('Ctrl Pts',(-0.111569990190912,-24.89137338738,
90.6637050372499));
#107983=CARTESIAN_POINT('Origin',(4.09260801170157,-24.6802428299903,99.1716370966873));
#107984=CARTESIAN_POINT('Ctrl Pts',(-3.41678053768791,0.170871362272414,
91.1025096700299));
#107985=CARTESIAN_POINT('Ctrl Pts',(-3.41738790502791,-0.166941914098586,
91.1026167652799));
#107986=CARTESIAN_POINT('Ctrl Pts',(-3.41552781040091,-0.908042807109186,
91.10228878041));
#107987=CARTESIAN_POINT('Ctrl Pts',(-3.39950555870891,-2.09245643556899,
91.0994636251401));
#107988=CARTESIAN_POINT('Ctrl Pts',(-3.36766182185891,-3.42224563324099,
91.09384871517));
#107989=CARTESIAN_POINT('Ctrl Pts',(-3.31682650133491,-4.87342127067699,
91.0848850765899));
#107990=CARTESIAN_POINT('Ctrl Pts',(-3.24468846482291,-6.455970844648,91.07216519442));
#107991=CARTESIAN_POINT('Ctrl Pts',(-3.14948284460091,-8.18752141444799,
91.0553778748601));
#107992=CARTESIAN_POINT('Ctrl Pts',(-3.02972032711291,-10.08904585353,91.03426051175));
#107993=CARTESIAN_POINT('Ctrl Pts',(-2.88692697078091,-12.17223757961,91.00908219036));
#107994=CARTESIAN_POINT('Ctrl Pts',(-2.72810852295691,-14.41821021101,90.98107821297));
#107995=CARTESIAN_POINT('Ctrl Pts',(-2.62472810958691,-16.1057824444,90.96284945682));
#107996=CARTESIAN_POINT('Ctrl Pts',(-2.58507228687091,-17.0405025299,90.95585706533));
#107997=CARTESIAN_POINT('Ctrl Pts',(-2.57998503310891,-17.17969442164,90.9549600452399));
#107998=CARTESIAN_POINT('Ctrl Pts',(-4.30429771344191,0.172489972228314,
91.10115797901));
#107999=CARTESIAN_POINT('Ctrl Pts',(-4.30490948529191,-0.167863353432186,
91.1012658508999));
#108000=CARTESIAN_POINT('Ctrl Pts',(-4.30303535257491,-0.915276061279186,
91.10093539073));
#108001=CARTESIAN_POINT('Ctrl Pts',(-4.28687480850291,-2.10963246135999,
91.0980858507901));
#108002=CARTESIAN_POINT('Ctrl Pts',(-4.25481409995891,-3.44832552765999,
91.09243268285));
#108003=CARTESIAN_POINT('Ctrl Pts',(-4.20362125539891,-4.90968613310399,
91.08340600314));
#108004=CARTESIAN_POINT('Ctrl Pts',(-4.13108944412291,-6.500757297294,91.07061668785));
#108005=CARTESIAN_POINT('Ctrl Pts',(-4.03543691811291,-8.24026573706799,
91.05375056674));
#108006=CARTESIAN_POINT('Ctrl Pts',(-3.91531379550691,-10.1478954092,91.0325696192201));
#108007=CARTESIAN_POINT('Ctrl Pts',(-3.77216277153791,-12.23436059257,91.00732823138));
#108008=CARTESIAN_POINT('Ctrl Pts',(-3.61391434248391,-14.4799922945,90.97942476368));
#108009=CARTESIAN_POINT('Ctrl Pts',(-3.50990930126091,-16.15377302025,90.96108586878));
#108010=CARTESIAN_POINT('Ctrl Pts',(-3.47236980401791,-17.07391474723,90.95446664258));
#108011=CARTESIAN_POINT('Ctrl Pts',(-3.46758380301991,-17.21040361506,90.95362274147));
#108012=CARTESIAN_POINT('Ctrl Pts',(-4.92692319961491,0.173422346322314,
90.4686804169501));
#108013=CARTESIAN_POINT('Ctrl Pts',(-4.92753750861191,-0.168394133661686,
90.4687887362));
#108014=CARTESIAN_POINT('Ctrl Pts',(-4.92565528948092,-0.919442660390486,
90.4684568501801));
#108015=CARTESIAN_POINT('Ctrl Pts',(-4.90941508431792,-2.11952643330099,
90.46559326384));
#108016=CARTESIAN_POINT('Ctrl Pts',(-4.87722939273791,-3.46334842915799,
90.45991805802));
#108017=CARTESIAN_POINT('Ctrl Pts',(-4.82583060223791,-4.93057592074299,
90.4508550644801));
#108018=CARTESIAN_POINT('Ctrl Pts',(-4.75307196337691,-6.52655580919599,
90.43802575337));
#108019=CARTESIAN_POINT('Ctrl Pts',(-4.65716200451291,-8.270648251298,90.4211142399));
#108020=CARTESIAN_POINT('Ctrl Pts',(-4.53683116115991,-10.18179474421,90.39989666561));
#108021=CARTESIAN_POINT('Ctrl Pts',(-4.39347410853091,-12.27014554973,90.37461894936));
#108022=CARTESIAN_POINT('Ctrl Pts',(-4.23555402957291,-14.51558086475,90.34677337864));
#108023=CARTESIAN_POINT('Ctrl Pts',(-4.13118918157491,-16.18141721551,90.3283710401));
#108024=CARTESIAN_POINT('Ctrl Pts',(-4.09486875940191,-17.09316131479,90.32196676972));
#108025=CARTESIAN_POINT('Ctrl Pts',(-4.09025629018791,-17.2280931494,90.32115346695));
#108026=CARTESIAN_POINT('Ctrl Pts',(-4.91434370485591,0.173113944903914,
89.58124990466));
#108027=CARTESIAN_POINT('Ctrl Pts',(-4.91495717464091,-0.168218567462786,
89.58135807593));
#108028=CARTESIAN_POINT('Ctrl Pts',(-4.91307763025291,-0.918064474226685,
89.58102666155));
#108029=CARTESIAN_POINT('Ctrl Pts',(-4.89686377459191,-2.11625380378499,
89.57816772133));
#108030=CARTESIAN_POINT('Ctrl Pts',(-4.86471942365691,-3.45837930339599,
89.57249980499));
#108031=CARTESIAN_POINT('Ctrl Pts',(-4.81338875390391,-4.92366620480499,
89.56344882297));
#108032=CARTESIAN_POINT('Ctrl Pts',(-4.74070514281191,-6.51802243432599,
89.55063274128));
#108033=CARTESIAN_POINT('Ctrl Pts',(-4.64488033502391,-8.26059862578499,
89.5337362422501));
#108034=CARTESIAN_POINT('Ctrl Pts',(-4.52461819947191,-10.17058185974,89.51253078299));
#108035=CARTESIAN_POINT('Ctrl Pts',(-4.38132929495091,-12.25830895794,89.48726508309));
#108036=CARTESIAN_POINT('Ctrl Pts',(-4.22330060761791,-14.50380923186,89.4594003617801));
#108037=CARTESIAN_POINT('Ctrl Pts',(-4.11905477292291,-16.17227334388,89.4410190084999));
#108038=CARTESIAN_POINT('Ctrl Pts',(-4.08233111723691,-17.08679512682,89.4345436371699));
#108039=CARTESIAN_POINT('Ctrl Pts',(-4.07766124890791,-17.22224198138,89.4337202133899));
#108040=CARTESIAN_POINT('Ctrl Pts',(-4.90176421009691,0.172805543485514,
88.69381939237));
#108041=CARTESIAN_POINT('Ctrl Pts',(-4.90237684066891,-0.168043001263886,
88.69392741567));
#108042=CARTESIAN_POINT('Ctrl Pts',(-4.90049997102491,-0.916686288062986,
88.69359647291));
#108043=CARTESIAN_POINT('Ctrl Pts',(-4.88431246486691,-2.11298117426899,
88.69074217883));
#108044=CARTESIAN_POINT('Ctrl Pts',(-4.85220945457491,-3.45341017763399,
88.68508155195));
#108045=CARTESIAN_POINT('Ctrl Pts',(-4.80094690556891,-4.91675648886699,
88.67604258146));
#108046=CARTESIAN_POINT('Ctrl Pts',(-4.72833832224791,-6.50948905945699,
88.66323972919));
#108047=CARTESIAN_POINT('Ctrl Pts',(-4.63259866553591,-8.25054900027199,
88.64635824459));
#108048=CARTESIAN_POINT('Ctrl Pts',(-4.51240523778391,-10.15936897527,88.62516490037));
#108049=CARTESIAN_POINT('Ctrl Pts',(-4.36918448137191,-12.24647236615,88.59991121682));
#108050=CARTESIAN_POINT('Ctrl Pts',(-4.21104718566391,-14.49203759898,88.5720273449301));
#108051=CARTESIAN_POINT('Ctrl Pts',(-4.10692036426991,-16.16312947225,88.5536669769));
#108052=CARTESIAN_POINT('Ctrl Pts',(-4.06979347507191,-17.08042893886,88.54712050463));
#108053=CARTESIAN_POINT('Ctrl Pts',(-4.06506620762691,-17.21639081336,88.54628695983));
#108054=CARTESIAN_POINT('Ctrl Pts',(-4.26146152596491,0.171439791658314,
88.07924489552));
#108055=CARTESIAN_POINT('Ctrl Pts',(-4.26207044009691,-0.167265508546186,
88.07935226351));
#108056=CARTESIAN_POINT('Ctrl Pts',(-4.26020541552291,-0.910583007860386,
88.0790234093601));
#108057=CARTESIAN_POINT('Ctrl Pts',(-4.24413459780491,-2.09848837535599,
88.0761896905901));
#108058=CARTESIAN_POINT('Ctrl Pts',(-4.21221466403891,-3.43140446629699,
88.07056134505));
#108059=CARTESIAN_POINT('Ctrl Pts',(-4.16125378691191,-4.88615689818499,
88.06157556745));
#108060=CARTESIAN_POINT('Ctrl Pts',(-4.08897746313191,-6.47169911548999,
88.0488313015));
#108061=CARTESIAN_POINT('Ctrl Pts',(-3.99361489689491,-8.20604435927999,
88.03201630812));
#108062=CARTESIAN_POINT('Ctrl Pts',(-3.87372574077891,-10.10971285652,88.0108766152));
#108063=CARTESIAN_POINT('Ctrl Pts',(-3.73080677741191,-12.19405416734,87.98567614591));
#108064=CARTESIAN_POINT('Ctrl Pts',(-3.57218851087291,-14.43990706988,87.9577074658801));
#108065=CARTESIAN_POINT('Ctrl Pts',(-3.46858873840091,-16.12263595099,87.9394400308));
#108066=CARTESIAN_POINT('Ctrl Pts',(-3.42967613463191,-17.05223635503,87.9325786888701));
#108067=CARTESIAN_POINT('Ctrl Pts',(-3.42469467592191,-17.19047898892,87.93170032329));
#108068=CARTESIAN_POINT('Ctrl Pts',(-3.37426264989091,0.169828985201214,
88.10305129184));
#108069=CARTESIAN_POINT('Ctrl Pts',(-3.37486718074691,-0.166348511574186,
88.1031578869399));
#108070=CARTESIAN_POINT('Ctrl Pts',(-3.37301612658291,-0.903384626014186,
88.1028314961499));
#108071=CARTESIAN_POINT('Ctrl Pts',(-3.35708293452291,-2.08139515709799,
88.1000220444999));
#108072=CARTESIAN_POINT('Ctrl Pts',(-3.32537892640591,-3.40545030595299,
88.09443177248));
#108073=CARTESIAN_POINT('Ctrl Pts',(-3.27477384965191,-4.85006687269799,
88.0855087320801));
#108074=CARTESIAN_POINT('Ctrl Pts',(-3.20288940220391,-6.42712858331899,
88.0728335645001));
#108075=CARTESIAN_POINT('Ctrl Pts',(-3.10797158717391,-8.15355432291199,
88.05609699276));
#108076=CARTESIAN_POINT('Ctrl Pts',(-2.98844129765691,-10.05114702111,88.0350205777099));
#108077=CARTESIAN_POINT('Ctrl Pts',(-2.84587827757191,-12.13223065634,88.0098828708199));
#108078=CARTESIAN_POINT('Ctrl Pts',(-2.68669274038691,-14.37842284469,87.98181416567));
#108079=CARTESIAN_POINT('Ctrl Pts',(-2.58371458436691,-16.07487674305,87.96365633834));
#108080=CARTESIAN_POINT('Ctrl Pts',(-2.54269585817091,-17.01898522172,87.9564236302));
#108081=CARTESIAN_POINT('Ctrl Pts',(-2.53741459906091,-17.15991784794,87.95549240173));
#108082=CARTESIAN_POINT('Ctrl Pts',(-4.35610804235899,-4.33090944307451,
90.6854704057514));
#108083=CARTESIAN_POINT('Ctrl Pts',(-4.30478949183536,-5.19990479673094,
90.6983684594538));
#108084=CARTESIAN_POINT('Ctrl Pts',(-4.23851111109544,-6.08684801638409,
90.7143224144303));
#108085=CARTESIAN_POINT('Ctrl Pts',(-4.11702828591693,-7.44606667250624,
90.7415669150335));
#108086=CARTESIAN_POINT('Ctrl Pts',(-4.07285971719824,-7.90392354852698,
90.7511901306072));
#108087=CARTESIAN_POINT('Ctrl Pts',(-4.00126272227492,-8.59776393941472,
90.7661321174809));
#108088=CARTESIAN_POINT('Ctrl Pts',(-3.96413053486937,-8.94644949098537,
90.7737290222104));
#108089=CARTESIAN_POINT('Ctrl Pts',(-3.91853774183228,-9.35632602828725,
90.7827359385487));
#108090=CARTESIAN_POINT('Ctrl Pts',(-3.89518250948977,-9.56203226857026,
90.7872649522662));
#108091=CARTESIAN_POINT('Ctrl Pts',(-3.88210036207672,-9.67611777792289,
90.7897776925425));
#108092=CARTESIAN_POINT('Ctrl Pts',(-3.87572411872776,-9.73138466025277,
90.7909950050756));
#108093=CARTESIAN_POINT('Ctrl Pts',(-3.87231200968099,-9.76087630926258,
90.791644554892));
#108094=CARTESIAN_POINT('Ctrl Pts',(-3.87204372056444,-9.76319481202625,
90.7916956195023));
#108095=CARTESIAN_POINT('Ctrl Pts',(-3.72160846660589,-11.0623980380779,
90.8203099123148));
#108096=CARTESIAN_POINT('Ctrl Pts',(-3.5552983746618,-12.3138422799621,
90.8474815345162));
#108097=CARTESIAN_POINT('Ctrl Pts',(-3.21377379456242,-14.7310381632549,
90.8932818883911));
#108098=CARTESIAN_POINT('Ctrl Pts',(-3.03762539304358,-15.893806171053,
90.9116387028507));
#108099=CARTESIAN_POINT('Ctrl Pts',(-2.88651065714691,-17.02169289621,90.92541563295));
#108100=CARTESIAN_POINT('Ctrl Pts',(-3.38209691507323,-8.56599685566967,
88.0736585716266));
#108101=CARTESIAN_POINT('Ctrl Pts',(-3.37193957246855,-8.73337111009727,
88.0718675580392));
#108102=CARTESIAN_POINT('Ctrl Pts',(-3.36148105368786,-8.90295580922593,
88.0700234389496));
#108103=CARTESIAN_POINT('Ctrl Pts',(-3.35072027313829,-9.07482982075256,
88.0681260230053));
#108104=CARTESIAN_POINT('Ctrl Pts',(-3.33169141523008,-9.37876373413238,
88.0647707219443));
#108105=CARTESIAN_POINT('Ctrl Pts',(-3.31172221608685,-9.68986200064915,
88.0612496136998));
#108106=CARTESIAN_POINT('Ctrl Pts',(-3.29083243179542,-10.0082637043351,
88.0575661812411));
#108107=CARTESIAN_POINT('Ctrl Pts',(-3.27269011607683,-10.2847885431281,
88.054367201603));
#108108=CARTESIAN_POINT('Ctrl Pts',(-3.25385379261577,-10.5668216859292,
88.0510458489647));
#108109=CARTESIAN_POINT('Ctrl Pts',(-3.23435072463955,-10.8544713275498,
88.0476069318742));
#108110=CARTESIAN_POINT('Ctrl Pts',(-3.20984726940729,-11.2158713967401,
88.0432863115966));
#108111=CARTESIAN_POINT('Ctrl Pts',(-3.18434819247011,-11.5861270547559,
88.0387901381542));
#108112=CARTESIAN_POINT('Ctrl Pts',(-3.15797463306237,-11.9658298297435,
88.0341397678366));
#108113=CARTESIAN_POINT('Ctrl Pts',(-3.15506081267406,-12.0077803935696,
88.0336259826613));
#108114=CARTESIAN_POINT('Ctrl Pts',(-3.15213636882712,-12.0498462841331,
88.0331103242645));
#108115=CARTESIAN_POINT('Ctrl Pts',(-3.1492015040689,-12.0920283078329,
88.032592828362));
#108116=CARTESIAN_POINT('Ctrl Pts',(-3.13321219304193,-12.3218383850417,
88.0297734810933));
#108117=CARTESIAN_POINT('Ctrl Pts',(-3.11691166401527,-12.5550954111528,
88.0268992568975));
#108118=CARTESIAN_POINT('Ctrl Pts',(-3.1004258518812,-12.791923953235,88.0239923634191));
#108119=CARTESIAN_POINT('Ctrl Pts',(-3.07705345276688,-13.1276824322344,
88.0198711788509));
#108120=CARTESIAN_POINT('Ctrl Pts',(-3.05325235874796,-13.470646096045,
88.0156744064028));
#108121=CARTESIAN_POINT('Ctrl Pts',(-3.02969158386299,-13.8174000592347,
88.0115200063467));
#108122=CARTESIAN_POINT('Ctrl Pts',(-3.01740308839832,-13.998255083096,
88.0093532131704));
#108123=CARTESIAN_POINT('Ctrl Pts',(-3.00518106525742,-14.1801411304469,
88.0071981402658));
#108124=CARTESIAN_POINT('Ctrl Pts',(-2.99312329150158,-14.3625732882036,
88.0050720286504));
#108125=CARTESIAN_POINT('Ctrl Pts',(-2.98190843170579,-14.5322522947031,
88.0030945455627));
#108126=CARTESIAN_POINT('Ctrl Pts',(-2.97083578203845,-14.7024036909771,
88.0011421376712));
#108127=CARTESIAN_POINT('Ctrl Pts',(-2.96001108679389,-14.8726675221283,
87.9992334518416));
#108128=CARTESIAN_POINT('Ctrl Pts',(-2.9388409874884,-15.2056563160088,
87.9955005921496));
#108129=CARTESIAN_POINT('Ctrl Pts',(-2.9187171752877,-15.5390060018737,
87.991952222616));
#108130=CARTESIAN_POINT('Ctrl Pts',(-2.90016396545698,-15.8737256740298,
87.988680790621));
#108131=CARTESIAN_POINT('Ctrl Pts',(-2.88402936386314,-16.1648110767787,
87.9858358245821));
#108132=CARTESIAN_POINT('Ctrl Pts',(-2.86908215708997,-16.4569322750347,
87.9832002282526));
#108133=CARTESIAN_POINT('Ctrl Pts',(-2.85569754787586,-16.7507633239214,
87.9808401604872));
#108134=CARTESIAN_POINT('Ctrl Pts',(-2.85191950242244,-16.8337023952505,
87.9801739891296));
#108135=CARTESIAN_POINT('Ctrl Pts',(-2.84826607231398,-16.9167777891168,
87.9795297908316));
#108136=CARTESIAN_POINT('Ctrl Pts',(-2.84483266429344,-17.,87.978924388362));
#108137=CARTESIAN_POINT('Ctrl Pts',(8.76687408897909,-16.44294428525,98.6115064056));
#108138=CARTESIAN_POINT('Ctrl Pts',(8.50448839268907,-16.29482593816,98.7748340168099));
#108139=CARTESIAN_POINT('Ctrl Pts',(7.73803846225909,-15.84050813694,99.1889282148399));
#108140=CARTESIAN_POINT('Ctrl Pts',(6.5349477692391,-15.02004513321,99.57986765328));
#108141=CARTESIAN_POINT('Ctrl Pts',(5.27236547025909,-14.00812222941,99.71688058005));
#108142=CARTESIAN_POINT('Ctrl Pts',(4.18367013900909,-13.00986029655,99.6525682338999));
#108143=CARTESIAN_POINT('Ctrl Pts',(3.20714073810909,-11.9973978225,99.4540121251699));
#108144=CARTESIAN_POINT('Ctrl Pts',(2.30415558486909,-10.93738557134,99.14726582813));
#108145=CARTESIAN_POINT('Ctrl Pts',(1.48684448748909,-9.84723726948199,
98.7638938018301));
#108146=CARTESIAN_POINT('Ctrl Pts',(0.762911702719089,-8.74553579959698,
98.3366761029799));
#108147=CARTESIAN_POINT('Ctrl Pts',(0.112673674949087,-7.60752902450998,
97.87904754731));
#108148=CARTESIAN_POINT('Ctrl Pts',(-0.488386309690911,-6.37224922945299,
97.3887134898101));
#108149=CARTESIAN_POINT('Ctrl Pts',(-1.04213634100091,-4.97114208044499,
96.8726660516999));
#108150=CARTESIAN_POINT('Ctrl Pts',(-1.51067364081091,-3.36802983074299,
96.3809404461301));
#108151=CARTESIAN_POINT('Ctrl Pts',(-1.81701727702091,-1.61981132427399,
96.0275490175501));
#108152=CARTESIAN_POINT('Ctrl Pts',(-1.87689058580091,-0.403435681896786,
95.95525979127));
#108153=CARTESIAN_POINT('Ctrl Pts',(-1.86852961382091,0.200651371990514,
95.9651297134299));
#108154=CARTESIAN_POINT('Ctrl Pts',(6.48819653156909,-15.56528785696,92.69131734964));
#108155=CARTESIAN_POINT('Ctrl Pts',(6.38630096531909,-15.47758556196,92.78395944648));
#108156=CARTESIAN_POINT('Ctrl Pts',(6.06771745324909,-15.21581444004,93.0220629079301));
#108157=CARTESIAN_POINT('Ctrl Pts',(5.4599981715091,-14.7540110982,93.25770281466));
#108158=CARTESIAN_POINT('Ctrl Pts',(4.67600680749909,-14.1542490297,93.3348504985));
#108159=CARTESIAN_POINT('Ctrl Pts',(3.89225004337909,-13.51762150969,93.2708681228701));
#108160=CARTESIAN_POINT('Ctrl Pts',(3.10219061563909,-12.82180106148,93.10110938746));
#108161=CARTESIAN_POINT('Ctrl Pts',(2.29351899611909,-12.03547497051,92.8361696333));
#108162=CARTESIAN_POINT('Ctrl Pts',(1.49269764718909,-11.16347023105,92.4954481808701));
#108163=CARTESIAN_POINT('Ctrl Pts',(0.723899763099089,-10.21566958806,92.10308906725));
#108164=CARTESIAN_POINT('Ctrl Pts',(-0.0200535606409112,-9.16446753653399,
91.66798555359));
#108165=CARTESIAN_POINT('Ctrl Pts',(-0.760996247700911,-7.93604781061299,
91.18364248321));
#108166=CARTESIAN_POINT('Ctrl Pts',(-1.50146348324091,-6.42271318686499,
90.65003751555));
#108167=CARTESIAN_POINT('Ctrl Pts',(-2.18733220258091,-4.52156727656799,
90.1121766327));
#108168=CARTESIAN_POINT('Ctrl Pts',(-2.67864361223591,-2.24136809065099,
89.70052285778));
#108169=CARTESIAN_POINT('Ctrl Pts',(-2.78026244461691,-0.556674570830786,
89.61294403093));
#108170=CARTESIAN_POINT('Ctrl Pts',(-2.76634006182491,0.277047208448614,
89.6246271184));
#108171=CARTESIAN_POINT('Ctrl Pts',(2.72889798757909,-19.34707978044,89.1447316619801));
#108172=CARTESIAN_POINT('Ctrl Pts',(2.66091020417909,-19.26097438926,89.20317193542));
#108173=CARTESIAN_POINT('Ctrl Pts',(2.42996072068909,-19.00901506437,89.3612231288901));
#108174=CARTESIAN_POINT('Ctrl Pts',(1.89825599140909,-18.57235792605,89.54995470502));
#108175=CARTESIAN_POINT('Ctrl Pts',(1.10699433400909,-17.98310305551,89.64471299023));
#108176=CARTESIAN_POINT('Ctrl Pts',(0.252027388659088,-17.32630382037,89.6293082806));
#108177=CARTESIAN_POINT('Ctrl Pts',(-0.654644487020914,-16.5759732809,89.5211787480401));
#108178=CARTESIAN_POINT('Ctrl Pts',(-1.61859475251091,-15.69330276297,89.32252842609));
#108179=CARTESIAN_POINT('Ctrl Pts',(-2.60190967346991,-14.67920705201,89.04432012876));
#108180=CARTESIAN_POINT('Ctrl Pts',(-3.56872088692091,-13.5426076308,88.7048190356501));
#108181=CARTESIAN_POINT('Ctrl Pts',(-4.52340351538191,-12.24737090716,88.3108681836801));
#108182=CARTESIAN_POINT('Ctrl Pts',(-5.49218708965691,-10.69472182793,87.8542655723));
#108183=CARTESIAN_POINT('Ctrl Pts',(-6.47884434265791,-8.73212611500698,
87.33045821777));
#108184=CARTESIAN_POINT('Ctrl Pts',(-7.41072188100292,-6.20174180863199,
86.77974038575));
#108185=CARTESIAN_POINT('Ctrl Pts',(-8.09046417872891,-3.09478014856899,
86.34080207947));
#108186=CARTESIAN_POINT('Ctrl Pts',(-8.23255272084991,-0.768163226373987,
86.24527748657));
#108187=CARTESIAN_POINT('Ctrl Pts',(-8.21314998798691,0.382355724809714,
86.2578544693));
#108188=CARTESIAN_POINT('Ctrl Pts',(0.196332399109088,-25.06476693734,90.52591274045));
#108189=CARTESIAN_POINT('Ctrl Pts',(0.011250503809089,-24.92028925106,90.61126618974));
#108190=CARTESIAN_POINT('Ctrl Pts',(-0.555409203350912,-24.48834062706,
90.84285524963));
#108191=CARTESIAN_POINT('Ctrl Pts',(-1.58520004181091,-23.72520655934,91.1268519171499));
#108192=CARTESIAN_POINT('Ctrl Pts',(-2.86435733527191,-22.73723822501,91.3040139279599));
#108193=CARTESIAN_POINT('Ctrl Pts',(-4.11539939684391,-21.69298831769,91.35045014482));
#108194=CARTESIAN_POINT('Ctrl Pts',(-5.35778473735791,-20.55625239098,91.29239781524));
#108195=CARTESIAN_POINT('Ctrl Pts',(-6.61477798365991,-19.27659173514,91.13677980334));
#108196=CARTESIAN_POINT('Ctrl Pts',(-7.84814243484691,-17.86250092626,90.8959268123599));
#108197=CARTESIAN_POINT('Ctrl Pts',(-9.02351089959392,-16.33037133773,90.58921613446));
#108198=CARTESIAN_POINT('Ctrl Pts',(-10.1541748021089,-14.63600828855,90.2254084335399));
#108199=CARTESIAN_POINT('Ctrl Pts',(-11.2746720699649,-12.6615424041,89.79831775978));
#108200=CARTESIAN_POINT('Ctrl Pts',(-12.3896921849461,-10.2361987255,89.30460716211));
#108201=CARTESIAN_POINT('Ctrl Pts',(-13.4190864676907,-7.19853323577899,
88.78356996623));
#108202=CARTESIAN_POINT('Ctrl Pts',(-14.1550194975079,-3.56544121650899,
88.3679745890099));
#108203=CARTESIAN_POINT('Ctrl Pts',(-14.3071566503109,-0.885592743395686,
88.2775704089799));
#108204=CARTESIAN_POINT('Ctrl Pts',(-14.2863014408449,0.440736329119914,
88.28947825565));
#108205=CARTESIAN_POINT('Origin',(33.1784433940591,111.0724296188,81.627048885766));
#108206=CARTESIAN_POINT('Origin',(11.833832765324,1.4210854715202E-14,67.1130006183894));
#108207=CARTESIAN_POINT('',(-3.38212037980694,8.56594505080956,88.0736627081359));
#108208=CARTESIAN_POINT('',(3.67711006996132,17.0000002064554,86.8289298464967));
#108209=CARTESIAN_POINT('Origin',(14.9594999633274,1.4210854715202E-14,
84.8395401726047));
#108210=CARTESIAN_POINT('',(-4.35611211213986,4.33088850455625,90.6854742262428));
#108211=CARTESIAN_POINT('Ctrl Pts',(-3.38212037964035,8.56594505080956,
88.0736627090807));
#108212=CARTESIAN_POINT('Ctrl Pts',(-4.01196786573672,7.17537091305373,
88.1847154552553));
#108213=CARTESIAN_POINT('Ctrl Pts',(-4.48931101496871,5.53882790374305,
88.5644810324709));
#108214=CARTESIAN_POINT('Ctrl Pts',(-4.85197636679152,3.15389859767277,
89.2370189724097));
#108215=CARTESIAN_POINT('Ctrl Pts',(-4.89577428506616,2.43186608701334,
89.4685758852254));
#108216=CARTESIAN_POINT('Ctrl Pts',(-4.89257765146922,2.07960258734854,
89.6990122597812));
#108217=CARTESIAN_POINT('Ctrl Pts',(-4.8906158368644,2.04033106029839,89.732655216438));
#108218=CARTESIAN_POINT('Ctrl Pts',(-4.88579454993422,2.00069680433019,
89.7825361835878));
#108219=CARTESIAN_POINT('Ctrl Pts',(-4.88354722702825,1.98887487582002,
89.8019169065442));
#108220=CARTESIAN_POINT('Ctrl Pts',(-4.87826443336458,1.97723449897512,
89.8383892585974));
#108221=CARTESIAN_POINT('Ctrl Pts',(-4.87568144241096,1.97525889172666,
89.8541368575422));
#108222=CARTESIAN_POINT('Ctrl Pts',(-4.86975792746109,1.97811725859756,
89.8861361443495));
#108223=CARTESIAN_POINT('Ctrl Pts',(-4.86662571171048,1.98280632649891,
89.90128551083));
#108224=CARTESIAN_POINT('Ctrl Pts',(-4.85879125914699,1.99981904456653,
89.936162260766));
#108225=CARTESIAN_POINT('Ctrl Pts',(-4.85403768892131,2.01448559580851,
89.9548332706941));
#108226=CARTESIAN_POINT('Ctrl Pts',(-4.84078559510826,2.06131459243085,
90.0031480412483));
#108227=CARTESIAN_POINT('Ctrl Pts',(-4.83131844154325,2.10280479749029,
90.0325972743869));
#108228=CARTESIAN_POINT('Ctrl Pts',(-4.79769422275787,2.26162274419331,
90.1269406929706));
#108229=CARTESIAN_POINT('Ctrl Pts',(-4.76852086425854,2.41936528606566,
90.1895927082715));
#108230=CARTESIAN_POINT('Ctrl Pts',(-4.6623556101869,2.97945480151193,90.3834105370763));
#108231=CARTESIAN_POINT('Ctrl Pts',(-4.54150792694898,3.60135784152189,
90.5420939486474));
#108232=CARTESIAN_POINT('Ctrl Pts',(-4.35610890955664,4.33088267781939,
90.6854997272617));
#108233=CARTESIAN_POINT('',(5.5223959989754,17.4579257767337,93.2012874099244));
#108234=CARTESIAN_POINT('Ctrl Pts',(5.52235604123134,17.4579109754503,93.2011992796923));
#108235=CARTESIAN_POINT('Ctrl Pts',(5.22894280014455,17.2623218249119,93.367079946153));
#108236=CARTESIAN_POINT('Ctrl Pts',(4.76538644319997,16.9508835888659,93.5867638396279));
#108237=CARTESIAN_POINT('Ctrl Pts',(3.58451633043917,16.0576376588373,93.8206675950891));
#108238=CARTESIAN_POINT('Ctrl Pts',(3.05115204928158,15.6226268077262,93.8400596368745));
#108239=CARTESIAN_POINT('Ctrl Pts',(1.44251906803305,14.200046478662,93.7321110206254));
#108240=CARTESIAN_POINT('Ctrl Pts',(0.340389916588458,13.0612424878892,
93.4020444225624));
#108241=CARTESIAN_POINT('Ctrl Pts',(-1.48003977708628,10.6921991318613,
92.5936247707043));
#108242=CARTESIAN_POINT('Ctrl Pts',(-2.19080611119185,9.58637988894192,
92.1831451763138));
#108243=CARTESIAN_POINT('Ctrl Pts',(-3.45378489947922,7.14145905979051,
91.3705187372968));
#108244=CARTESIAN_POINT('Ctrl Pts',(-3.98965312113643,5.77285420037568,
90.9689374055126));
#108245=CARTESIAN_POINT('Ctrl Pts',(-4.35611534545078,4.33089434326653,
90.6854487074141));
#108246=CARTESIAN_POINT('',(6.72284169586273,18.2005858292129,92.4518055721481));
#108247=CARTESIAN_POINT('Ctrl Pts',(6.72284226036562,18.2005860182602,92.4518065521755));
#108248=CARTESIAN_POINT('Ctrl Pts',(6.52447441211948,18.0870793782497,92.5879632910271));
#108249=CARTESIAN_POINT('Ctrl Pts',(6.32523711499546,17.9686329849413,92.7183652975874));
#108250=CARTESIAN_POINT('Ctrl Pts',(5.92461392813651,17.7210119573958,92.9683840841069));
#108251=CARTESIAN_POINT('Ctrl Pts',(5.72352843386396,17.5919809286868,93.087753641798));
#108252=CARTESIAN_POINT('Ctrl Pts',(5.52243594124477,17.4579405679198,93.2013755505527));
#108253=CARTESIAN_POINT('',(7.18082400639694,18.5000000000005,91.584560428554));
#108254=CARTESIAN_POINT('Ctrl Pts',(6.72284115829969,18.2005856294418,92.4518046221571));
#108255=CARTESIAN_POINT('Ctrl Pts',(6.79273197664956,18.240576093798,92.4038466295081));
#108256=CARTESIAN_POINT('Ctrl Pts',(6.86056063905956,18.2794361008248,92.3496148573615));
#108257=CARTESIAN_POINT('Ctrl Pts',(6.97969843358352,18.3487004919864,92.2319577470068));
#108258=CARTESIAN_POINT('Ctrl Pts',(7.0329599010906,18.3801663787552,92.1682058175694));
#108259=CARTESIAN_POINT('Ctrl Pts',(7.12351536852898,18.4363205837614,92.0220852314388));
#108260=CARTESIAN_POINT('Ctrl Pts',(7.15921714211905,18.4602533155557,91.9391925959291));
#108261=CARTESIAN_POINT('Ctrl Pts',(7.18668920593521,18.4843760087887,91.805974202742));
#108262=CARTESIAN_POINT('Ctrl Pts',(7.19146209592983,18.4902813775617,91.7619889127895));
#108263=CARTESIAN_POINT('Ctrl Pts',(7.19239576516467,18.4981238590837,91.6728396062505));
#108264=CARTESIAN_POINT('Ctrl Pts',(7.1885807496804,18.5000000202485,91.6285508614658));
#108265=CARTESIAN_POINT('Ctrl Pts',(7.1808240063969,18.5000000000005,91.584560428554));
#108266=CARTESIAN_POINT('',(6.52234847239187,18.4999999410994,87.8501601928846));
#108267=CARTESIAN_POINT('',(3.13624619141446,18.5,68.6466197984171));
#108268=CARTESIAN_POINT('Ctrl Pts',(6.52234845610643,18.4999999847284,87.8501601957549));
#108269=CARTESIAN_POINT('Ctrl Pts',(6.50518062854233,18.4999859008965,87.7529665002294));
#108270=CARTESIAN_POINT('Ctrl Pts',(6.4689459203091,18.4903141218653,87.664456395585));
#108271=CARTESIAN_POINT('Ctrl Pts',(6.36972845372158,18.4567893765268,87.5030984304372));
#108272=CARTESIAN_POINT('Ctrl Pts',(6.30672210579292,18.432901727933,87.4302697426766));
#108273=CARTESIAN_POINT('Ctrl Pts',(6.09300490374429,18.346334827275,87.2342769515595));
#108274=CARTESIAN_POINT('Ctrl Pts',(5.91789315169122,18.2685458496827,87.1337400811857));
#108275=CARTESIAN_POINT('Ctrl Pts',(5.42965862838366,18.0384248294259,86.9149877608346));
#108276=CARTESIAN_POINT('Ctrl Pts',(5.06665893878539,17.8504223940439,86.8312090840354));
#108277=CARTESIAN_POINT('Ctrl Pts',(4.34754070270684,17.4389532379846,86.7591293140068));
#108278=CARTESIAN_POINT('Ctrl Pts',(3.99139559238964,17.2150671358623,86.7735129004256));
#108279=CARTESIAN_POINT('Ctrl Pts',(3.67710978043254,17.,86.8289299687275));
#108280=CARTESIAN_POINT('Origin',(-2.58324905909591,17.,89.45593823501));
#108281=CARTESIAN_POINT('',(-2.84368888085373,17.0000004240545,87.9787221388565));
#108282=CARTESIAN_POINT('',(-2.58374595121974,18.4999998795018,89.4555997193086));
#108283=CARTESIAN_POINT('Origin',(-2.58324874406691,17.,89.45594000334));
#108284=CARTESIAN_POINT('',(-2.88564989564837,17.021544099749,90.9249820008041));
#108285=CARTESIAN_POINT('Ctrl Pts',(-2.88564989564837,17.021544099749,90.9249820008041));
#108286=CARTESIAN_POINT('Ctrl Pts',(-2.89272275172126,17.0341859203076,
90.9233406649279));
#108287=CARTESIAN_POINT('Ctrl Pts',(-2.89875888973422,17.0483838508755,
90.9216770896837));
#108288=CARTESIAN_POINT('Ctrl Pts',(-2.90373721386657,17.0641913692076,
90.9198941123406));
#108289=CARTESIAN_POINT('Ctrl Pts',(-2.90863603335344,17.0797464389029,
90.9181396094355));
#108290=CARTESIAN_POINT('Ctrl Pts',(-2.91251038467502,17.0968604310834,
90.9162695931292));
#108291=CARTESIAN_POINT('Ctrl Pts',(-2.91533029213212,17.1155732692065,
90.9141442815309));
#108292=CARTESIAN_POINT('Ctrl Pts',(-2.91806979840219,17.1337525669846,
90.912079566806));
#108293=CARTESIAN_POINT('Ctrl Pts',(-2.91981384580904,17.1534411860481,
90.909773888665));
#108294=CARTESIAN_POINT('Ctrl Pts',(-2.92052895027268,17.1746602860845,
90.9070536885397));
#108295=CARTESIAN_POINT('Ctrl Pts',(-2.92116428945037,17.1935125325099,
90.9046369091758));
#108296=CARTESIAN_POINT('Ctrl Pts',(-2.92098715652524,17.2135729063995,
90.9018923789284));
#108297=CARTESIAN_POINT('Ctrl Pts',(-2.91997316350144,17.2348417505946,
90.898666979331));
#108298=CARTESIAN_POINT('Ctrl Pts',(-2.91884217783387,17.2585645547814,
90.8950694390805));
#108299=CARTESIAN_POINT('Ctrl Pts',(-2.91666985230917,17.2838009544818,
90.8908731213832));
#108300=CARTESIAN_POINT('Ctrl Pts',(-2.91338863854326,17.3105273658752,
90.8858265569166));
#108301=CARTESIAN_POINT('Ctrl Pts',(-2.91036157979191,17.3351836130058,
90.8811708873313));
#108302=CARTESIAN_POINT('Ctrl Pts',(-2.9063903424519,17.3611081211397,90.875791137097));
#108303=CARTESIAN_POINT('Ctrl Pts',(-2.90143338018716,17.3882532510825,
90.8694509342227));
#108304=CARTESIAN_POINT('Ctrl Pts',(-2.90101718845782,17.3905323845458,
90.868918604167));
#108305=CARTESIAN_POINT('Ctrl Pts',(-2.90059405731327,17.3928201037254,
90.8683794812995));
#108306=CARTESIAN_POINT('Ctrl Pts',(-2.90016396772038,17.3951163696448,
90.8678334135308));
#108307=CARTESIAN_POINT('Ctrl Pts',(-2.89525968391285,17.4213005413903,
90.8616066380865));
#108308=CARTESIAN_POINT('Ctrl Pts',(-2.88944428307568,17.4485976869347,
90.8544806107943));
#108309=CARTESIAN_POINT('Ctrl Pts',(-2.88266400361103,17.4769183999902,
90.8462258062526));
#108310=CARTESIAN_POINT('Ctrl Pts',(-2.88176772082657,17.4806621051999,
90.8451346065111));
#108311=CARTESIAN_POINT('Ctrl Pts',(-2.88085461529801,17.4844236483625,
90.844023638876));
#108312=CARTESIAN_POINT('Ctrl Pts',(-2.87992459944332,17.4882027778685,
90.8428923335443));
#108313=CARTESIAN_POINT('Ctrl Pts',(-2.87594185832357,17.5043866895776,
90.8380475814458));
#108314=CARTESIAN_POINT('Ctrl Pts',(-2.87164793871547,17.5208931022076,
90.8328303477065));
#108315=CARTESIAN_POINT('Ctrl Pts',(-2.86703278793527,17.5376973896157,
90.8271961656877));
#108316=CARTESIAN_POINT('Ctrl Pts',(-2.86472521254517,17.5460995333198,
90.8243790746783));
#108317=CARTESIAN_POINT('Ctrl Pts',(-2.86233732272639,17.5545761164248,
90.8214577022601));
#108318=CARTESIAN_POINT('Ctrl Pts',(-2.85986784195119,17.563123412719,90.8184264261586));
#108319=CARTESIAN_POINT('Ctrl Pts',(-2.8586331015636,17.567397060866,90.8169107881079));
#108320=CARTESIAN_POINT('Ctrl Pts',(-2.85737796314338,17.5716883855217,
90.8153676717458));
#108321=CARTESIAN_POINT('Ctrl Pts',(-2.85610226614962,17.5759968930406,
90.8137963669988));
#108322=CARTESIAN_POINT('Ctrl Pts',(-2.85546441765275,17.5781511468,90.8130107146253));
#108323=CARTESIAN_POINT('Ctrl Pts',(-2.85482142949836,17.5803096961521,
90.8122180150108));
#108324=CARTESIAN_POINT('Ctrl Pts',(-2.85417328159823,17.5824724768591,
90.8114181792966));
#108325=CARTESIAN_POINT('Ctrl Pts',(-2.85363989194418,17.5842523250277,
90.8107599590126));
#108326=CARTESIAN_POINT('Ctrl Pts',(-2.85275716260682,17.5871762193749,
90.8096706293563));
#108327=CARTESIAN_POINT('Ctrl Pts',(-2.85237889573469,17.5884265878567,
90.809202171474));
#108328=CARTESIAN_POINT('Ctrl Pts',(-2.85229751199868,17.5886956033744,
90.8091013832332));
#108329=CARTESIAN_POINT('Ctrl Pts',(-2.85223948918946,17.5888872233252,
90.8090295090512));
#108330=CARTESIAN_POINT('Ctrl Pts',(-2.85221333854556,17.5889734477422,
90.8089971746851));
#108331=CARTESIAN_POINT('Ctrl Pts',(-2.84981137671696,17.5968932434863,
90.8060272320208));
#108332=CARTESIAN_POINT('Ctrl Pts',(-2.84742439317891,17.6066031853638,
90.8021939861059));
#108333=CARTESIAN_POINT('Ctrl Pts',(-2.84503553822777,17.6180765319828,
90.7973737496568));
#108334=CARTESIAN_POINT('Ctrl Pts',(-2.84267434922401,17.6294170028056,
90.7926093376135));
#108335=CARTESIAN_POINT('Ctrl Pts',(-2.84031138095239,17.6424806348029,
90.78688052455));
#108336=CARTESIAN_POINT('Ctrl Pts',(-2.83791736788481,17.6572145956106,
90.7800277439991));
#108337=CARTESIAN_POINT('Ctrl Pts',(-2.83555953805227,17.6717258665865,
90.7732785367214));
#108338=CARTESIAN_POINT('Ctrl Pts',(-2.83317165642656,17.6878577743391,
90.7654388297756));
#108339=CARTESIAN_POINT('Ctrl Pts',(-2.8307122729031,17.7055277305542,90.7563199402147));
#108340=CARTESIAN_POINT('Ctrl Pts',(-2.82825288937964,17.7231976867694,
90.7472010506538));
#108341=CARTESIAN_POINT('Ctrl Pts',(-2.82572211830423,17.7424062805898,
90.7368026951786));
#108342=CARTESIAN_POINT('Ctrl Pts',(-2.82306354352082,17.7630309283082,
90.7249034888705));
#108343=CARTESIAN_POINT('Ctrl Pts',(-2.82037666239594,17.7838751704968,
90.7128775894938));
#108344=CARTESIAN_POINT('Ctrl Pts',(-2.8175619937707,17.8061702443592,90.6993152921338));
#108345=CARTESIAN_POINT('Ctrl Pts',(-2.81457900890531,17.8297261572579,
90.6839614262744));
#108346=CARTESIAN_POINT('Ctrl Pts',(-2.81183054654266,17.8514301024475,
90.6698146825462));
#108347=CARTESIAN_POINT('Ctrl Pts',(-2.80893917040494,17.8742043080774,
90.6541462654809));
#108348=CARTESIAN_POINT('Ctrl Pts',(-2.80585388277503,17.8978548379212,
90.6367446469575));
#108349=CARTESIAN_POINT('Ctrl Pts',(-2.80559061943676,17.8998729050142,
90.635259790849));
#108350=CARTESIAN_POINT('Ctrl Pts',(-2.80532593181083,17.9018973237863,
90.6337623114634));
#108351=CARTESIAN_POINT('Ctrl Pts',(-2.80505978110586,17.9039279573148,
90.6322520756096));
#108352=CARTESIAN_POINT('Ctrl Pts',(-2.80205444120059,17.9268576128145,
90.6151986844556));
#108353=CARTESIAN_POINT('Ctrl Pts',(-2.79886835716004,17.9505812957136,
90.5965189872643));
#108354=CARTESIAN_POINT('Ctrl Pts',(-2.79546721016593,17.9748626055492,
90.5760303547297));
#108355=CARTESIAN_POINT('Ctrl Pts',(-2.79503723540175,17.977932261312,90.5734401711952));
#108356=CARTESIAN_POINT('Ctrl Pts',(-2.79460378775201,17.9810107717434,
90.5708210887861));
#108357=CARTESIAN_POINT('Ctrl Pts',(-2.79416676592282,17.9840976086969,
90.5681727505254));
#108358=CARTESIAN_POINT('Ctrl Pts',(-2.79221980998713,17.9978496346318,
90.5563742600336));
#108359=CARTESIAN_POINT('Ctrl Pts',(-2.79020290218355,18.0117669734879,
90.5439950698029));
#108360=CARTESIAN_POINT('Ctrl Pts',(-2.78811029496996,18.0257981614033,
90.531005677591));
#108361=CARTESIAN_POINT('Ctrl Pts',(-2.78706399136317,18.032813755361,90.5245109814851));
#108362=CARTESIAN_POINT('Ctrl Pts',(-2.78599875847823,18.0398577888693,
90.5178637116599));
#108363=CARTESIAN_POINT('Ctrl Pts',(-2.78491395993615,18.0469231884083,
90.5110605527259));
#108364=CARTESIAN_POINT('Ctrl Pts',(-2.78437156066511,18.0504558881778,
90.5076589732588));
#108365=CARTESIAN_POINT('Ctrl Pts',(-2.78382426979793,18.0539939285704,
90.5042184205558));
#108366=CARTESIAN_POINT('Ctrl Pts',(-2.78327201036165,18.0575364026759,
90.5007384915099));
#108367=CARTESIAN_POINT('Ctrl Pts',(-2.7829958806435,18.0593076397286,90.498998526987));
#108368=CARTESIAN_POINT('Ctrl Pts',(-2.78271850877296,18.0610799851526,
90.4972487183256));
#108369=CARTESIAN_POINT('Ctrl Pts',(-2.782439885476,18.0628533233283,90.4954890167306));
#108370=CARTESIAN_POINT('Ctrl Pts',(-2.78221394952778,18.0642913252708,
90.494062072707));
#108371=CARTESIAN_POINT('Ctrl Pts',(-2.78185106072081,18.0665937852198,
90.4917650752688));
#108372=CARTESIAN_POINT('Ctrl Pts',(-2.78168224811797,18.0676589240395,
90.4906984446302));
#108373=CARTESIAN_POINT('Ctrl Pts',(-2.78164288170219,18.0679073101016,
90.4904497106821));
#108374=CARTESIAN_POINT('Ctrl Pts',(-2.78161413020944,18.0680885676011,
90.490268030535));
#108375=CARTESIAN_POINT('Ctrl Pts',(-2.78160025212524,18.0681761996918,
90.4901801847663));
#108376=CARTESIAN_POINT('Ctrl Pts',(-2.78032215971842,18.0762466154791,
90.4820900904573));
#108377=CARTESIAN_POINT('Ctrl Pts',(-2.7786805815117,18.0856953119116,90.4724605539379));
#108378=CARTESIAN_POINT('Ctrl Pts',(-2.77666920797862,18.0963860070905,
90.4611876416064));
#108379=CARTESIAN_POINT('Ctrl Pts',(-2.77466627508606,18.1070318392374,
90.4499620355554));
#108380=CARTESIAN_POINT('Ctrl Pts',(-2.77229676958671,18.1189095058335,
90.4371062886785));
#108381=CARTESIAN_POINT('Ctrl Pts',(-2.76954033978892,18.1318401729579,
90.422495725083));
#108382=CARTESIAN_POINT('Ctrl Pts',(-2.76682548303308,18.1445758170975,
90.408105521017));
#108383=CARTESIAN_POINT('Ctrl Pts',(-2.7637353738569,18.1583331058328,90.3920123883352));
#108384=CARTESIAN_POINT('Ctrl Pts',(-2.76023529491343,18.1728952424158,
90.3740845319854));
#108385=CARTESIAN_POINT('Ctrl Pts',(-2.75774287675484,18.1832649895654,
90.3613180443053));
#108386=CARTESIAN_POINT('Ctrl Pts',(-2.75504225355344,18.1940419267948,
90.3476208806931));
#108387=CARTESIAN_POINT('Ctrl Pts',(-2.75211568209974,18.2051324832473,
90.3329443703691));
#108388=CARTESIAN_POINT('Ctrl Pts',(-2.74826585928658,18.2197217997621,
90.313637831931));
#108389=CARTESIAN_POINT('Ctrl Pts',(-2.74402945369785,18.2348512605904,
90.2926396949604));
#108390=CARTESIAN_POINT('Ctrl Pts',(-2.73940734219813,18.2502548534008,
90.2698653768146));
#108391=CARTESIAN_POINT('Ctrl Pts',(-2.73478523069841,18.2656584462113,
90.2470910586688));
#108392=CARTESIAN_POINT('Ctrl Pts',(-2.72977787187187,18.2813361189648,
90.2225397489312));
#108393=CARTESIAN_POINT('Ctrl Pts',(-2.72435293204009,18.2969874788806,
90.1961498106201));
#108394=CARTESIAN_POINT('Ctrl Pts',(-2.71975402191694,18.3102556808865,
90.173778142323));
#108395=CARTESIAN_POINT('Ctrl Pts',(-2.71486064322452,18.3235025090161,
90.150086575742));
#108396=CARTESIAN_POINT('Ctrl Pts',(-2.70967491430402,18.3365199956771,
90.1250651320109));
#108397=CARTESIAN_POINT('Ctrl Pts',(-2.70874348358792,18.338858121543,90.120570924618));
#108398=CARTESIAN_POINT('Ctrl Pts',(-2.70780251144841,18.3411888157279,
90.116033885955));
#108399=CARTESIAN_POINT('Ctrl Pts',(-2.70685186153706,18.3435108313772,
90.1114540572454));
#108400=CARTESIAN_POINT('Ctrl Pts',(-2.70373017080596,18.3511357358172,
90.0964150732175));
#108401=CARTESIAN_POINT('Ctrl Pts',(-2.70050598929708,18.3586669961609,
90.0809143766248));
#108402=CARTESIAN_POINT('Ctrl Pts',(-2.69718010601399,18.3660589508997,
90.064956017357));
#108403=CARTESIAN_POINT('Ctrl Pts',(-2.69551716437245,18.3697549282691,
90.0569768377231));
#108404=CARTESIAN_POINT('Ctrl Pts',(-2.69382879758791,18.3734160829511,
90.0488832440363));
#108405=CARTESIAN_POINT('Ctrl Pts',(-2.69211520430522,18.3770365424535,
90.0406762303334));
#108406=CARTESIAN_POINT('Ctrl Pts',(-2.69111684674479,18.3791458604306,
90.0358947373959));
#108407=CARTESIAN_POINT('Ctrl Pts',(-2.68998177548008,18.3815123624915,
90.0304489795216));
#108408=CARTESIAN_POINT('Ctrl Pts',(-2.68893247195787,18.3836575502816,
90.0254316939668));
#108409=CARTESIAN_POINT('Ctrl Pts',(-2.68818073791755,18.3851943893854,
90.0218372484496));
#108410=CARTESIAN_POINT('Ctrl Pts',(-2.68747356905611,18.3866189610764,
90.0184631770783));
#108411=CARTESIAN_POINT('Ctrl Pts',(-2.68689895589015,18.3877699993807,
90.0157159835079));
#108412=CARTESIAN_POINT('Ctrl Pts',(-2.68273502555585,18.3961109904947,
89.995808464294));
#108413=CARTESIAN_POINT('Ctrl Pts',(-2.67857173349699,18.4038633633472,
89.9760659407918));
#108414=CARTESIAN_POINT('Ctrl Pts',(-2.6744950233554,18.411069615988,89.9564946382672));
#108415=CARTESIAN_POINT('Ctrl Pts',(-2.67033515986297,18.4184228557909,
89.9365241365529));
#108416=CARTESIAN_POINT('Ctrl Pts',(-2.66626541080946,18.4252074926367,
89.9167318884532));
#108417=CARTESIAN_POINT('Ctrl Pts',(-2.66232301180073,18.4314664027915,
89.8971312173691));
#108418=CARTESIAN_POINT('Ctrl Pts',(-2.65832134318844,18.4378194087297,
89.8772358718996));
#108419=CARTESIAN_POINT('Ctrl Pts',(-2.65445073071921,18.4436307789762,
89.8575378564482));
#108420=CARTESIAN_POINT('Ctrl Pts',(-2.65069644096881,18.4489427237725,
89.8380584175511));
#108421=CARTESIAN_POINT('Ctrl Pts',(-2.64684123627611,18.4543974531267,
89.8180553732365));
#108422=CARTESIAN_POINT('Ctrl Pts',(-2.64310853898396,18.4593255648351,
89.7982826110807));
#108423=CARTESIAN_POINT('Ctrl Pts',(-2.63942836724829,18.4637697337413,
89.7787726382549));
#108424=CARTESIAN_POINT('Ctrl Pts',(-2.63842739594567,18.4649785049233,
89.7734661133653));
#108425=CARTESIAN_POINT('Ctrl Pts',(-2.63743001768668,18.4661514569317,
89.7681790936903));
#108426=CARTESIAN_POINT('Ctrl Pts',(-2.6364341883642,18.4672894089015,89.76291239117));
#108427=CARTESIAN_POINT('Ctrl Pts',(-2.63412054764574,18.4699332475128,
89.7506761001432));
#108428=CARTESIAN_POINT('Ctrl Pts',(-2.6318089098615,18.4723877734019,89.7385526465792));
#108429=CARTESIAN_POINT('Ctrl Pts',(-2.62955528816091,18.4746640081669,
89.7265334976566));
#108430=CARTESIAN_POINT('Ctrl Pts',(-2.62727008962927,18.4769721366081,
89.7143459413057));
#108431=CARTESIAN_POINT('Ctrl Pts',(-2.62504439302348,18.4790969404991,
89.7022655671137));
#108432=CARTESIAN_POINT('Ctrl Pts',(-2.62288393166343,18.4810488921174,
89.690295347201));
#108433=CARTESIAN_POINT('Ctrl Pts',(-2.62066950419694,18.4830496014828,
89.6780261234856));
#108434=CARTESIAN_POINT('Ctrl Pts',(-2.61852342927454,18.4848687105302,
89.6658723930533));
#108435=CARTESIAN_POINT('Ctrl Pts',(-2.61639927614851,18.4865164796311,
89.6538519002648));
#108436=CARTESIAN_POINT('Ctrl Pts',(-2.61600399982798,18.4868231072933,
89.6516150482686));
#108437=CARTESIAN_POINT('Ctrl Pts',(-2.61560934480965,18.4871237991489,
89.6493828564495));
#108438=CARTESIAN_POINT('Ctrl Pts',(-2.61521482799771,18.4874186178726,
89.6471555062605));
#108439=CARTESIAN_POINT('Ctrl Pts',(-2.61386181693006,18.4884297103889,
89.6395167203683));
#108440=CARTESIAN_POINT('Ctrl Pts',(-2.61245735898484,18.4893710309274,
89.6319494481471));
#108441=CARTESIAN_POINT('Ctrl Pts',(-2.61108133794674,18.4902464545109,
89.6244341372504));
#108442=CARTESIAN_POINT('Ctrl Pts',(-2.60966686342039,18.4911463421755,
89.6167088078211));
#108443=CARTESIAN_POINT('Ctrl Pts',(-2.60828238466218,18.4919765958269,
89.6090383053057));
#108444=CARTESIAN_POINT('Ctrl Pts',(-2.60696055857762,18.4927406253114,
89.6014139729777));
#108445=CARTESIAN_POINT('Ctrl Pts',(-2.60560833229972,18.4935222264298,
89.5936142914267));
#108446=CARTESIAN_POINT('Ctrl Pts',(-2.60432141487863,18.4942345143377,
89.585862782367));
#108447=CARTESIAN_POINT('Ctrl Pts',(-2.60308124819483,18.4948803903919,
89.5781646752645));
#108448=CARTESIAN_POINT('Ctrl Pts',(-2.60178322759524,18.4955563966369,
89.5701074505968));
#108449=CARTESIAN_POINT('Ctrl Pts',(-2.60053598823274,18.4961596313639,
89.5621081813244));
#108450=CARTESIAN_POINT('Ctrl Pts',(-2.59926508718496,18.496692802091,89.554193733652));
#108451=CARTESIAN_POINT('Ctrl Pts',(-2.59892621066429,18.4968349681874,
89.5520834037447));
#108452=CARTESIAN_POINT('Ctrl Pts',(-2.5985853957473,18.4969721506261,89.5499792438945));
#108453=CARTESIAN_POINT('Ctrl Pts',(-2.59824072044925,18.4971043973977,
89.5478820949598));
#108454=CARTESIAN_POINT('Ctrl Pts',(-2.59726065128508,18.4974804353198,
89.541918943509));
#108455=CARTESIAN_POINT('Ctrl Pts',(-2.59625246810505,18.4978217715933,
89.5359236463374));
#108456=CARTESIAN_POINT('Ctrl Pts',(-2.59526777887276,18.4981250455876,
89.5299443033961));
#108457=CARTESIAN_POINT('Ctrl Pts',(-2.59405837501909,18.4984975293373,
89.5226004225468));
#108458=CARTESIAN_POINT('Ctrl Pts',(-2.59288333407229,18.4988123908878,
89.5152823187125));
#108459=CARTESIAN_POINT('Ctrl Pts',(-2.59175342134928,18.4990691230242,
89.5080864873127));
#108460=CARTESIAN_POINT('Ctrl Pts',(-2.59084788868234,18.4992748728413,
89.5023196167698));
#108461=CARTESIAN_POINT('Ctrl Pts',(-2.58996850226688,18.4994434439634,
89.4966331171326));
#108462=CARTESIAN_POINT('Ctrl Pts',(-2.58910961638368,18.4995774188085,
89.4910554511265));
#108463=CARTESIAN_POINT('Ctrl Pts',(-2.58836825370421,18.4996930615873,
89.4862409891632));
#108464=CARTESIAN_POINT('Ctrl Pts',(-2.58764226881396,18.4997830320815,
89.4815087705558));
#108465=CARTESIAN_POINT('Ctrl Pts',(-2.58693155413368,18.4998498277382,
89.4768411884873));
#108466=CARTESIAN_POINT('Ctrl Pts',(-2.58632491345824,18.4999068421258,
89.4728571070868));
#108467=CARTESIAN_POINT('Ctrl Pts',(-2.58573036890802,18.4999470490274,
89.4689203158292));
#108468=CARTESIAN_POINT('Ctrl Pts',(-2.58514232825975,18.4999715297978,
89.4649839703477));
#108469=CARTESIAN_POINT('Ctrl Pts',(-2.58467724319737,18.4999908917938,
89.461870689847));
#108470=CARTESIAN_POINT('Ctrl Pts',(-2.58421667937964,18.5000004361134,
89.4587570869406));
#108471=CARTESIAN_POINT('Ctrl Pts',(-2.58374595121974,18.4999998795018,
89.4555997193086));
#108472=CARTESIAN_POINT('Ctrl Pts',(-2.88564989564837,17.021544099749,90.9249820008041));
#108473=CARTESIAN_POINT('Ctrl Pts',(-2.94425494600512,17.0236905283469,
90.9128867456866));
#108474=CARTESIAN_POINT('Ctrl Pts',(-3.00214169784583,17.0257878045666,
90.8972746305873));
#108475=CARTESIAN_POINT('Ctrl Pts',(-3.05889396442204,17.0278206146711,
90.8782560396643));
#108476=CARTESIAN_POINT('Ctrl Pts',(-3.11563625018334,17.0298530672727,
90.8592407934717));
#108477=CARTESIAN_POINT('Ctrl Pts',(-3.17124404617029,17.0318210616847,
90.8368204011847));
#108478=CARTESIAN_POINT('Ctrl Pts',(-3.22531755484121,17.0337102576852,
90.8111546993795));
#108479=CARTESIAN_POINT('Ctrl Pts',(-3.2793964272523,17.0355996410817,90.7854864517037));
#108480=CARTESIAN_POINT('Ctrl Pts',(-3.33194032250968,17.0374101967068,
90.7565724291325));
#108481=CARTESIAN_POINT('Ctrl Pts',(-3.38257142258566,17.0391287596191,
90.7246197156803));
#108482=CARTESIAN_POINT('Ctrl Pts',(-3.43319372601489,17.0408470239483,
90.6926725536922));
#108483=CARTESIAN_POINT('Ctrl Pts',(-3.48190353970458,17.04247331515,90.6576879833429));
#108484=CARTESIAN_POINT('Ctrl Pts',(-3.52835092027089,17.0439958500997,
90.6199171167676));
#108485=CARTESIAN_POINT('Ctrl Pts',(-3.57480482369066,17.0455185988672,
90.5821409458279));
#108486=CARTESIAN_POINT('Ctrl Pts',(-3.6189953282331,17.0469375512594,90.5415779633663));
#108487=CARTESIAN_POINT('Ctrl Pts',(-3.66060520918311,17.0482424701167,
90.4985198337093));
#108488=CARTESIAN_POINT('Ctrl Pts',(-3.69259236151813,17.0492456125751,
90.4654193556219));
#108489=CARTESIAN_POINT('Ctrl Pts',(-3.72305509711362,17.0501813960177,
90.4308452036344));
#108490=CARTESIAN_POINT('Ctrl Pts',(-3.7518642681655,17.0510458502037,90.3949445258879));
#108491=CARTESIAN_POINT('Ctrl Pts',(-3.78946888608619,17.0521742224611,
90.3480833625686));
#108492=CARTESIAN_POINT('Ctrl Pts',(-3.82425641745817,17.0531809947735,
90.2989589153202));
#108493=CARTESIAN_POINT('Ctrl Pts',(-3.85597615794192,17.0540585932871,
90.2479252300767));
#108494=CARTESIAN_POINT('Ctrl Pts',(-3.88769401396993,17.0549361396629,
90.1968945767219));
#108495=CARTESIAN_POINT('Ctrl Pts',(-3.91634422361392,17.0556845214828,
90.1439552671422));
#108496=CARTESIAN_POINT('Ctrl Pts',(-3.94172033754719,17.0562980686622,
90.0894887958083));
#108497=CARTESIAN_POINT('Ctrl Pts',(-3.96710126713341,17.0569117322751,
90.0350119883125));
#108498=CARTESIAN_POINT('Ctrl Pts',(-3.98920668027896,17.0573905057506,
89.9790078174381));
#108499=CARTESIAN_POINT('Ctrl Pts',(-4.00787722915267,17.0577306973398,
89.921880016422));
#108500=CARTESIAN_POINT('Ctrl Pts',(-4.02654503603207,17.0580708389678,
89.8647606053095));
#108501=CARTESIAN_POINT('Ctrl Pts',(-4.04177885889447,17.0582724371425,
89.806518291553));
#108502=CARTESIAN_POINT('Ctrl Pts',(-4.05346891781446,17.0583338318022,
89.7475728198879));
#108503=CARTESIAN_POINT('Ctrl Pts',(-4.06516020881029,17.0583952329326,
89.6886211356542));
#108504=CARTESIAN_POINT('Ctrl Pts',(-4.07330690665017,17.0583164006063,
89.6289665549535));
#108505=CARTESIAN_POINT('Ctrl Pts',(-4.07785029379567,17.0580977249397,
89.5690390908458));
#108506=CARTESIAN_POINT('Ctrl Pts',(-4.08125199755465,17.0579339991084,
89.524170477762));
#108507=CARTESIAN_POINT('Ctrl Pts',(-4.08263482891519,17.057691923133,89.4791491395646));
#108508=CARTESIAN_POINT('Ctrl Pts',(-4.08199319731286,17.0573724106553,
89.4341571731456));
#108509=CARTESIAN_POINT('Ctrl Pts',(-4.0811362969349,17.0569457010576,89.3740703057139));
#108510=CARTESIAN_POINT('Ctrl Pts',(-4.07666673783311,17.0563806968148,
89.3140361496127));
#108511=CARTESIAN_POINT('Ctrl Pts',(-4.06861674219757,17.0556812172046,
89.2544873773602));
#108512=CARTESIAN_POINT('Ctrl Pts',(-4.0605672245926,17.0549817791313,89.1949421412753));
#108513=CARTESIAN_POINT('Ctrl Pts',(-4.04893775211773,17.054147886678,89.135882645154));
#108514=CARTESIAN_POINT('Ctrl Pts',(-4.03381213850186,17.0531853114299,
89.0777344865986));
#108515=CARTESIAN_POINT('Ctrl Pts',(-4.01868365241601,17.0522225533814,
89.0195752852621));
#108516=CARTESIAN_POINT('Ctrl Pts',(-4.00005780075606,17.051131070441,88.9623281724327));
#108517=CARTESIAN_POINT('Ctrl Pts',(-3.97806886527228,17.0499185028006,
88.9064058416279));
#108518=CARTESIAN_POINT('Ctrl Pts',(-3.95608315669126,17.048706113106,88.8504917174925));
#108519=CARTESIAN_POINT('Ctrl Pts',(-3.93073550530722,17.0473726828737,
88.79590237483));
#108520=CARTESIAN_POINT('Ctrl Pts',(-3.90220859640684,17.0459275976915,
88.743031232164));
#108521=CARTESIAN_POINT('Ctrl Pts',(-3.87367867435884,17.0444823598725,
88.6901545049968));
#108522=CARTESIAN_POINT('Ctrl Pts',(-3.84196902067873,17.042925453691,88.6389967088623));
#108523=CARTESIAN_POINT('Ctrl Pts',(-3.80730821890185,17.0412678759289,
88.5899266093886));
#108524=CARTESIAN_POINT('Ctrl Pts',(-3.78135715586258,17.0400268225547,
88.5531870886763));
#108525=CARTESIAN_POINT('Ctrl Pts',(-3.75375272349364,17.0387293695425,
88.5176173955231));
#108526=CARTESIAN_POINT('Ctrl Pts',(-3.72460657631882,17.0373806672224,
88.4833613981499));
#108527=CARTESIAN_POINT('Ctrl Pts',(-3.68568139893112,17.0355794522373,
88.4376119285427));
#108528=CARTESIAN_POINT('Ctrl Pts',(-3.6440051618024,17.0336866954822,88.3942070434139));
#108529=CARTESIAN_POINT('Ctrl Pts',(-3.59987823703332,17.031715959433,88.3534595674234));
#108530=CARTESIAN_POINT('Ctrl Pts',(-3.55575391791031,17.0297453397537,
88.3127144975263));
#108531=CARTESIAN_POINT('Ctrl Pts',(-3.50917950754176,17.027696763826,88.2746268057133));
#108532=CARTESIAN_POINT('Ctrl Pts',(-3.46049063955607,17.0255848993722,
88.2394709635901));
#108533=CARTESIAN_POINT('Ctrl Pts',(-3.4117925185039,17.0234726335696,88.2043084402816));
#108534=CARTESIAN_POINT('Ctrl Pts',(-3.36097947365895,17.021297069954,88.1720791269206));
#108535=CARTESIAN_POINT('Ctrl Pts',(-3.30841782215132,17.0190737780021,
88.1430153674807));
#108536=CARTESIAN_POINT('Ctrl Pts',(-3.25586388483155,17.0168508123506,
88.1139558735707));
#108537=CARTESIAN_POINT('Ctrl Pts',(-3.20156222001496,17.0145801479348,
88.0880612053631));
#108538=CARTESIAN_POINT('Ctrl Pts',(-3.1459041800945,17.0122780126348,88.065517987308));
#108539=CARTESIAN_POINT('Ctrl Pts',(-3.09024028320291,17.009975635078,88.0429723969993));
#108540=CARTESIAN_POINT('Ctrl Pts',(-3.03322011233942,17.0076417960823,
88.0237791198216));
#108541=CARTESIAN_POINT('Ctrl Pts',(-2.97525469926286,17.0052931566727,
88.0080765148966));
#108542=CARTESIAN_POINT('Ctrl Pts',(-2.93186940227286,17.0035352736024,
87.9963236067048));
#108543=CARTESIAN_POINT('Ctrl Pts',(-2.88795501514177,17.0017691095523,
87.9865252034533));
#108544=CARTESIAN_POINT('Ctrl Pts',(-2.84368904488424,17.0000017248341,
87.9787209138959));
#108545=CARTESIAN_POINT('Ctrl Pts',(4.99091733589909,16.72092210659,92.8589087628099));
#108546=CARTESIAN_POINT('Ctrl Pts',(4.9667657052791,16.72092210659,92.8566764327501));
#108547=CARTESIAN_POINT('Ctrl Pts',(4.83237115732909,16.72092210659,92.84370830857));
#108548=CARTESIAN_POINT('Ctrl Pts',(4.58105099422909,16.72092210659,92.81384884849));
#108549=CARTESIAN_POINT('Ctrl Pts',(4.23026429059909,16.72092210659,92.76024569411));
#108550=CARTESIAN_POINT('Ctrl Pts',(3.85488118854909,16.72092210659,92.69069139225));
#108551=CARTESIAN_POINT('Ctrl Pts',(3.45147771125909,16.72092210659,92.60420128478));
#108552=CARTESIAN_POINT('Ctrl Pts',(3.01590860903909,16.72092210659,92.4996154625501));
#108553=CARTESIAN_POINT('Ctrl Pts',(2.54470817102909,16.72092210659,92.37611183637));
#108554=CARTESIAN_POINT('Ctrl Pts',(2.03458068702909,16.72092210659,92.2336813754001));
#108555=CARTESIAN_POINT('Ctrl Pts',(1.48085160723909,16.72092210659,92.0725401253));
#108556=CARTESIAN_POINT('Ctrl Pts',(0.879179917559089,16.72092210659,91.8936980027499));
#108557=CARTESIAN_POINT('Ctrl Pts',(0.223663970489089,16.72092210659,91.6990548324));
#108558=CARTESIAN_POINT('Ctrl Pts',(-0.496523475400911,16.72092210659,91.49034500414));
#108559=CARTESIAN_POINT('Ctrl Pts',(-1.29838121732091,16.72092210659,91.2700006865301));
#108560=CARTESIAN_POINT('Ctrl Pts',(-2.15052846082091,16.72092210659,91.0563866516499));
#108561=CARTESIAN_POINT('Ctrl Pts',(-2.73844970172191,16.72092210659,90.92810809411));
#108562=CARTESIAN_POINT('Ctrl Pts',(-3.02681279946791,16.72092210659,90.8706313150801));
#108563=CARTESIAN_POINT('Ctrl Pts',(4.97075622012909,17.878482928,93.07717336913));
#108564=CARTESIAN_POINT('Ctrl Pts',(4.94601405284909,17.878482928,93.07488634949));
#108565=CARTESIAN_POINT('Ctrl Pts',(4.80837330780909,17.878482928,93.06160460452));
#108566=CARTESIAN_POINT('Ctrl Pts',(4.55138762180909,17.878482928,93.0310672706));
#108567=CARTESIAN_POINT('Ctrl Pts',(4.19349622708909,17.878482928,92.97637036656));
#108568=CARTESIAN_POINT('Ctrl Pts',(3.81168120185909,17.878482928,92.90561486059));
#108569=CARTESIAN_POINT('Ctrl Pts',(3.40266948939909,17.878482928,92.81791383544));
#108570=CARTESIAN_POINT('Ctrl Pts',(2.96229009133909,17.878482928,92.71216580768));
#108571=CARTESIAN_POINT('Ctrl Pts',(2.48719060390909,17.878482928,92.5876337928));
#108572=CARTESIAN_POINT('Ctrl Pts',(1.97426210470909,17.878482928,92.4444164613201));
#108573=CARTESIAN_POINT('Ctrl Pts',(1.41877633195909,17.878482928,92.28276124204));
#108574=CARTESIAN_POINT('Ctrl Pts',(0.816542904509091,17.878482928,92.10375113626));
#108575=CARTESIAN_POINT('Ctrl Pts',(0.161760017919087,17.878482928,91.90932682469));
#108576=CARTESIAN_POINT('Ctrl Pts',(-0.556279413340908,17.878482928,91.70124310188));
#108577=CARTESIAN_POINT('Ctrl Pts',(-1.35427477140091,17.878482928,91.4819669887));
#108578=CARTESIAN_POINT('Ctrl Pts',(-2.20083077152091,17.878482928,91.26976572553));
#108579=CARTESIAN_POINT('Ctrl Pts',(-2.78389374754391,17.878482928,91.14255536753));
#108580=CARTESIAN_POINT('Ctrl Pts',(-3.06965715457391,17.878482928,91.08559680638));
#108581=CARTESIAN_POINT('Ctrl Pts',(5.0479315220591,18.70551127491,92.2416721455));
#108582=CARTESIAN_POINT('Ctrl Pts',(5.02544988667909,18.70551127491,92.23959447365));
#108583=CARTESIAN_POINT('Ctrl Pts',(4.90023535074909,18.70551127491,92.2275132465));
#108584=CARTESIAN_POINT('Ctrl Pts',(4.66493687916909,18.70551127491,92.1995707649));
#108585=CARTESIAN_POINT('Ctrl Pts',(4.33424173121909,18.70551127491,92.1490606559601));
#108586=CARTESIAN_POINT('Ctrl Pts',(3.97704764559909,18.70551127491,92.0829032729701));
#108587=CARTESIAN_POINT('Ctrl Pts',(3.58950385423909,18.70551127491,91.99983755366));
#108588=CARTESIAN_POINT('Ctrl Pts',(3.16753792284909,18.70551127491,91.8985383651201));
#108589=CARTESIAN_POINT('Ctrl Pts',(2.70736371634909,18.70551127491,91.7779429482401));
#108590=CARTESIAN_POINT('Ctrl Pts',(2.20515730198909,18.70551127491,91.63773770054));
#108591=CARTESIAN_POINT('Ctrl Pts',(1.65639602359909,18.70551127491,91.4780499183101));
#108592=CARTESIAN_POINT('Ctrl Pts',(1.05631288796909,18.70551127491,91.2996828402801));
#108593=CARTESIAN_POINT('Ctrl Pts',(0.398723898549089,18.70551127491,91.10442075303));
#108594=CARTESIAN_POINT('Ctrl Pts',(-0.32753797830091,18.70551127491,90.8939403435401));
#108595=CARTESIAN_POINT('Ctrl Pts',(-1.14031826414091,18.70551127491,90.67057522062));
#108596=CARTESIAN_POINT('Ctrl Pts',(-2.00827714201091,18.70551127491,90.45296596887));
#108597=CARTESIAN_POINT('Ctrl Pts',(-2.60993720675791,18.70551127491,90.3216666198201));
#108598=CARTESIAN_POINT('Ctrl Pts',(-2.90565204297691,18.70551127491,90.2627243579));
#108599=CARTESIAN_POINT('Ctrl Pts',(5.15410013561909,18.46962664964,91.09228880238));
#108600=CARTESIAN_POINT('Ctrl Pts',(5.13472827152909,18.46962664964,91.0904991263699));
#108601=CARTESIAN_POINT('Ctrl Pts',(5.02660823810909,18.46962664964,91.08006942904));
#108602=CARTESIAN_POINT('Ctrl Pts',(4.82114446012908,18.46962664964,91.05569663703));
#108603=CARTESIAN_POINT('Ctrl Pts',(4.52786267812909,18.46962664964,91.0109462235));
#108604=CARTESIAN_POINT('Ctrl Pts',(4.20453915676909,18.46962664964,90.9511143919301));
#108605=CARTESIAN_POINT('Ctrl Pts',(3.84652838130909,18.46962664964,90.87442537583));
#108606=CARTESIAN_POINT('Ctrl Pts',(3.44989351020909,18.46962664964,90.77924637184));
#108607=CARTESIAN_POINT('Ctrl Pts',(3.01025173241909,18.46962664964,90.6640664589099));
#108608=CARTESIAN_POINT('Ctrl Pts',(2.52279548879909,18.46962664964,90.5280048783));
#108609=CARTESIAN_POINT('Ctrl Pts',(1.98328497102909,18.46962664964,90.37102366228));
#108610=CARTESIAN_POINT('Ctrl Pts',(1.38615995146909,18.46962664964,90.1935411854399));
#108611=CARTESIAN_POINT('Ctrl Pts',(0.72471065908909,18.46962664964,89.99712658593));
#108612=CARTESIAN_POINT('Ctrl Pts',(-0.0128626817609094,18.46962664964,
89.7833490995701));
#108613=CARTESIAN_POINT('Ctrl Pts',(-0.845982315090913,18.46962664964,89.55435880276));
#108614=CARTESIAN_POINT('Ctrl Pts',(-1.74338472995091,18.46962664964,89.3293098826599));
#108615=CARTESIAN_POINT('Ctrl Pts',(-2.37062846040091,18.46962664964,89.19238538542));
#108616=CARTESIAN_POINT('Ctrl Pts',(-2.68003329087591,18.46962664964,89.1307141835901));
#108617=CARTESIAN_POINT('',(4.96810338032909,18.4999999989654,91.37512691991));
#108618=CARTESIAN_POINT('Ctrl Pts',(4.96810338032909,18.49999999896,91.37512691991));
#108619=CARTESIAN_POINT('Ctrl Pts',(4.88114290831909,18.49999999896,91.36529516959));
#108620=CARTESIAN_POINT('Ctrl Pts',(4.69919234968909,18.50000000048,91.34173652012));
#108621=CARTESIAN_POINT('Ctrl Pts',(4.40440989175909,18.49999999987,91.29429551851));
#108622=CARTESIAN_POINT('Ctrl Pts',(4.08146866854909,18.50000000003,91.23249710617));
#108623=CARTESIAN_POINT('Ctrl Pts',(3.72713024749909,18.49999999999,91.1550615909));
#108624=CARTESIAN_POINT('Ctrl Pts',(3.33778568867909,18.50000000001,91.0605802439));
#108625=CARTESIAN_POINT('Ctrl Pts',(2.90976010514909,18.49999999999,90.9478782426));
#108626=CARTESIAN_POINT('Ctrl Pts',(2.43912217626909,18.50000000005,90.81636240186));
#108627=CARTESIAN_POINT('Ctrl Pts',(1.92237783813909,18.4999999998,90.66612537853));
#108628=CARTESIAN_POINT('Ctrl Pts',(1.35481786031909,18.50000000073,90.49759288502));
#108629=CARTESIAN_POINT('Ctrl Pts',(0.731044259609088,18.49999999728,90.3121755411));
#108630=CARTESIAN_POINT('Ctrl Pts',(0.0458698878690877,18.50000001013,90.11263961256));
#108631=CARTESIAN_POINT('Ctrl Pts',(-0.714595015070913,18.49999996218,89.9005103584));
#108632=CARTESIAN_POINT('Ctrl Pts',(-1.59425516731442,18.5000001411387,
89.6744034239708));
#108633=CARTESIAN_POINT('Ctrl Pts',(-2.24165009651391,18.4999996959444,
89.5259395502124));
#108634=CARTESIAN_POINT('Ctrl Pts',(-2.58355159951403,18.49999969586,89.455639680019));
#108635=CARTESIAN_POINT('',(4.84756322776217,18.0488923264225,92.4405611323625));
#108636=CARTESIAN_POINT('Ctrl Pts',(4.84756322776218,18.0488923264225,92.4405611323624));
#108637=CARTESIAN_POINT('Ctrl Pts',(4.85108865467572,18.0808891883013,92.4094618791462));
#108638=CARTESIAN_POINT('Ctrl Pts',(4.85480491613432,18.1117722156623,92.3766550456964));
#108639=CARTESIAN_POINT('Ctrl Pts',(4.85869826376457,18.1412880203712,92.342267321212));
#108640=CARTESIAN_POINT('Ctrl Pts',(4.86255042152504,18.170491561119,92.3082434034122));
#108641=CARTESIAN_POINT('Ctrl Pts',(4.86657590878541,18.1983559273946,92.272672132448));
#108642=CARTESIAN_POINT('Ctrl Pts',(4.87075610737188,18.2246553376688,92.2357229972551));
#108643=CARTESIAN_POINT('Ctrl Pts',(4.87491517490048,18.2508218034551,92.198960641302));
#108644=CARTESIAN_POINT('Ctrl Pts',(4.87922734699014,18.2754384318051,92.1608347313778));
#108645=CARTESIAN_POINT('Ctrl Pts',(4.88366957173433,18.2983128308262,92.121553735949));
#108646=CARTESIAN_POINT('Ctrl Pts',(4.88809513870236,18.3211014537688,92.0824200392424));
#108647=CARTESIAN_POINT('Ctrl Pts',(4.89264972013234,18.3421603511356,92.0421404780596));
#108648=CARTESIAN_POINT('Ctrl Pts',(4.89730666423195,18.3613381441414,92.0009551042941));
#108649=CARTESIAN_POINT('Ctrl Pts',(4.89909677213828,18.3687099996225,91.9851236359265));
#108650=CARTESIAN_POINT('Ctrl Pts',(4.90090196980804,18.3758043538445,91.9691586349514));
#108651=CARTESIAN_POINT('Ctrl Pts',(4.90272062489739,18.3826143754992,91.9530747754237));
#108652=CARTESIAN_POINT('Ctrl Pts',(4.90745910576851,18.4003577934409,91.9111685002032));
#108653=CARTESIAN_POINT('Ctrl Pts',(4.91228901451279,18.4161672956054,91.868454656171));
#108654=CARTESIAN_POINT('Ctrl Pts',(4.91718001881137,18.429956549144,91.8252042611727));
#108655=CARTESIAN_POINT('Ctrl Pts',(4.92209115163039,18.443802551206,91.7817758727795));
#108656=CARTESIAN_POINT('Ctrl Pts',(4.92706379558328,18.4556114950119,91.7378072895491));
#108657=CARTESIAN_POINT('Ctrl Pts',(4.93206617755245,18.4653477652398,91.6935821240343));
#108658=CARTESIAN_POINT('Ctrl Pts',(4.93708571018732,18.4751174162685,91.6492053325472));
#108659=CARTESIAN_POINT('Ctrl Pts',(4.94213509559067,18.4828002340483,91.604570987581));
#108660=CARTESIAN_POINT('Ctrl Pts',(4.94718251049573,18.4884127970871,91.5599629899558));
#108661=CARTESIAN_POINT('Ctrl Pts',(4.95227349442145,18.4940738074756,91.5149699384352));
#108662=CARTESIAN_POINT('Ctrl Pts',(4.95736238798444,18.4976289148035,91.4700044479895));
#108663=CARTESIAN_POINT('Ctrl Pts',(4.96241815198147,18.499146125442,91.4253433749732));
#108664=CARTESIAN_POINT('Ctrl Pts',(4.96431840339645,18.4997163818196,91.4085571351005));
#108665=CARTESIAN_POINT('Ctrl Pts',(4.96621399740515,18.4999992365987,91.3918136968969));
#108666=CARTESIAN_POINT('Ctrl Pts',(4.96810338032909,18.4999999984587,91.37512691991));
#108667=CARTESIAN_POINT('Ctrl Pts',(4.84756322776218,18.0488923264225,92.4405611323624));
#108668=CARTESIAN_POINT('Ctrl Pts',(4.77863748925725,18.0391235192895,92.4423846537365));
#108669=CARTESIAN_POINT('Ctrl Pts',(4.70997125933779,18.0293209872038,92.4432370767815));
#108670=CARTESIAN_POINT('Ctrl Pts',(4.64157809200293,18.0194976485252,92.4431933791652));
#108671=CARTESIAN_POINT('Ctrl Pts',(4.52594851367706,18.0028897247599,92.4431195013621));
#108672=CARTESIAN_POINT('Ctrl Pts',(4.41109803083324,17.986222594221,92.4404834705022));
#108673=CARTESIAN_POINT('Ctrl Pts',(4.29724836321367,17.9695550215731,92.435660158109));
#108674=CARTESIAN_POINT('Ctrl Pts',(4.17169109641864,17.951173458328,92.4303408459524));
#108675=CARTESIAN_POINT('Ctrl Pts',(4.04735487367925,17.9327914945713,92.4223623638395));
#108676=CARTESIAN_POINT('Ctrl Pts',(3.92427963714316,17.9144809687944,92.4122312825809));
#108677=CARTESIAN_POINT('Ctrl Pts',(3.80178290438126,17.8962565099517,92.4021478215333));
#108678=CARTESIAN_POINT('Ctrl Pts',(3.68053568025839,17.8781028263318,92.3899325406664));
#108679=CARTESIAN_POINT('Ctrl Pts',(3.56046442767764,17.8600832142125,92.3759622120109));
#108680=CARTESIAN_POINT('Ctrl Pts',(3.54683918999336,17.8580384158713,92.3743769112468));
#108681=CARTESIAN_POINT('Ctrl Pts',(3.53322904170923,17.855995335902,92.3727690020822));
#108682=CARTESIAN_POINT('Ctrl Pts',(3.51963383569171,17.8539540606116,92.3711390280173));
#108683=CARTESIAN_POINT('Ctrl Pts',(3.48008197200912,17.8480154788849,92.3663970247009));
#108684=CARTESIAN_POINT('Ctrl Pts',(3.44065660212661,17.8420921781034,92.3614682762439));
#108685=CARTESIAN_POINT('Ctrl Pts',(3.40135667910275,17.8361862228892,92.3563640314303));
#108686=CARTESIAN_POINT('Ctrl Pts',(3.29331967364858,17.8199505240228,92.3423322654026));
#108687=CARTESIAN_POINT('Ctrl Pts',(3.18623194199405,17.8038461336087,92.3269747296614));
#108688=CARTESIAN_POINT('Ctrl Pts',(3.08005801224797,17.787912355629,92.3105213482678));
#108689=CARTESIAN_POINT('Ctrl Pts',(2.93466117010058,17.7660923004868,92.2879897371368));
#108690=CARTESIAN_POINT('Ctrl Pts',(2.79097894314264,17.7445928313063,92.2634039732281));
#108691=CARTESIAN_POINT('Ctrl Pts',(2.64892471577811,17.7234998276821,92.2372815745539));
#108692=CARTESIAN_POINT('Ctrl Pts',(2.63349649122928,17.7212089588895,92.2344444732583));
#108693=CARTESIAN_POINT('Ctrl Pts',(2.61808742790506,17.7189228682825,92.2315892244038));
#108694=CARTESIAN_POINT('Ctrl Pts',(2.6026973852413,17.7166416540508,92.2287164747354));
#108695=CARTESIAN_POINT('Ctrl Pts',(2.52991459082119,17.7058533053713,92.2151306288017));
#108696=CARTESIAN_POINT('Ctrl Pts',(2.45755743279404,17.6951741066982,92.2011535006045));
#108697=CARTESIAN_POINT('Ctrl Pts',(2.38560353455431,17.6846137707613,92.1868376533435));
#108698=CARTESIAN_POINT('Ctrl Pts',(2.33067763417641,17.6765525541516,92.1759096727931));
#108699=CARTESIAN_POINT('Ctrl Pts',(2.27598664675078,17.6685605757371,92.1647842866499));
#108700=CARTESIAN_POINT('Ctrl Pts',(2.22151959346614,17.6606417338181,92.153484228638));
#108701=CARTESIAN_POINT('Ctrl Pts',(2.19428606682382,17.6566823128585,92.1478341996321));
#108702=CARTESIAN_POINT('Ctrl Pts',(2.16710852539423,17.652741173016,92.142140496716));
#108703=CARTESIAN_POINT('Ctrl Pts',(2.13998550900522,17.6488187657813,92.1364059063002));
#108704=CARTESIAN_POINT('Ctrl Pts',(2.12642400081072,17.646857562164,92.1335386110924));
#108705=CARTESIAN_POINT('Ctrl Pts',(2.11287612398475,17.6449010414981,92.1306610936225));
#108706=CARTESIAN_POINT('Ctrl Pts',(2.09934169429784,17.6429492585768,92.1277736994122));
#108707=CARTESIAN_POINT('Ctrl Pts',(2.09454050070415,17.6422568845445,92.1267494273221));
#108708=CARTESIAN_POINT('Ctrl Pts',(2.08974099961185,17.6415651068035,92.1257239123675));
#108709=CARTESIAN_POINT('Ctrl Pts',(2.08494318251133,17.6408739276938,92.1246971698815));
#108710=CARTESIAN_POINT('Ctrl Pts',(2.08297854388802,17.6405908995695,92.1242767332742));
#108711=CARTESIAN_POINT('Ctrl Pts',(2.08101418763385,17.6403079718227,92.1238560908356));
#108712=CARTESIAN_POINT('Ctrl Pts',(2.07905011346576,17.640025144613,92.1234352434809));
#108713=CARTESIAN_POINT('Ctrl Pts',(2.07566985705564,17.6395383867788,92.1227109470202));
#108714=CARTESIAN_POINT('Ctrl Pts',(2.07229043580454,17.6390519266124,92.121986043553));
#108715=CARTESIAN_POINT('Ctrl Pts',(2.0689118489881,17.6385657651584,92.1212605378308));
#108716=CARTESIAN_POINT('Ctrl Pts',(2.06553326217166,17.6380796037045,92.1205350321085));
#108717=CARTESIAN_POINT('Ctrl Pts',(2.06419545146993,17.637887061752,92.1202479150636));
#108718=CARTESIAN_POINT('Ctrl Pts',(2.05877858970523,17.6371081775176,92.1190822184667));
#108719=CARTESIAN_POINT('Ctrl Pts',(1.93197314754368,17.6188749709064,92.0917939695089));
#108720=CARTESIAN_POINT('Ctrl Pts',(1.80308271629193,17.6005065693028,92.0630007856599));
#108721=CARTESIAN_POINT('Ctrl Pts',(1.67211378071565,17.5820272808739,92.0328432618983));
#108722=CARTESIAN_POINT('Ctrl Pts',(1.6228660587514,17.5750785883871,92.0215032495602));
#108723=CARTESIAN_POINT('Ctrl Pts',(1.57332416328396,17.5681142187702,92.0099707585996));
#108724=CARTESIAN_POINT('Ctrl Pts',(1.52348737127662,17.5611354685922,91.9982548760115));
#108725=CARTESIAN_POINT('Ctrl Pts',(1.39072766294977,17.5425448490759,91.9670450590761));
#108726=CARTESIAN_POINT('Ctrl Pts',(1.25587748125058,17.5238521878038,91.9345310659547));
#108727=CARTESIAN_POINT('Ctrl Pts',(1.11891188088551,17.5050819682797,91.9008811477652));
#108728=CARTESIAN_POINT('Ctrl Pts',(1.05127012774792,17.4958121183903,91.8842628183949));
#108729=CARTESIAN_POINT('Ctrl Pts',(0.983111955639909,17.4865233509836,
91.867368051501));
#108730=CARTESIAN_POINT('Ctrl Pts',(0.914431433187615,17.4772185998306,
91.8502208383066));
#108731=CARTESIAN_POINT('Ctrl Pts',(0.771048344925136,17.4577932386337,
91.8144229105225));
#108732=CARTESIAN_POINT('Ctrl Pts',(0.62539050942459,17.4382982430918,91.7775223526176));
#108733=CARTESIAN_POINT('Ctrl Pts',(0.477413059436499,17.4187600360463,
91.7397211622103));
#108734=CARTESIAN_POINT('Ctrl Pts',(0.403227685597623,17.4089649679875,
91.7207703325931));
#108735=CARTESIAN_POINT('Ctrl Pts',(0.328458829786943,17.3991590329485,
91.7015937659605));
#108736=CARTESIAN_POINT('Ctrl Pts',(0.253097736293403,17.3893455114241,
91.682220803364));
#108737=CARTESIAN_POINT('Ctrl Pts',(0.101000508020681,17.3695394105002,
91.6431213983823));
#108738=CARTESIAN_POINT('Ctrl Pts',(-0.0535077743595639,17.3497024578493,
91.6032193796216));
#108739=CARTESIAN_POINT('Ctrl Pts',(-0.210473329951067,17.3298610909504,
91.5627670240531));
#108740=CARTESIAN_POINT('Ctrl Pts',(-0.295423188605298,17.3191229305482,
91.5408741834561));
#108741=CARTESIAN_POINT('Ctrl Pts',(-0.381093334328116,17.3083837371342,
91.5188207794666));
#108742=CARTESIAN_POINT('Ctrl Pts',(-0.467494193863738,17.2976475111883,
91.4966522549976));
#108743=CARTESIAN_POINT('Ctrl Pts',(-0.630669617962847,17.277371228853,
91.4547850976415));
#108744=CARTESIAN_POINT('Ctrl Pts',(-0.796449849872686,17.2571056016649,
91.4125048865914));
#108745=CARTESIAN_POINT('Ctrl Pts',(-0.964904430483136,17.23687674083,91.3701121771337));
#108746=CARTESIAN_POINT('Ctrl Pts',(-1.06436517031682,17.2249330023022,
91.345082224069));
#108747=CARTESIAN_POINT('Ctrl Pts',(-1.16475869454555,17.2130020596482,
91.3200138638997));
#108748=CARTESIAN_POINT('Ctrl Pts',(-1.26610367830689,17.2010890878669,
91.2949763539329));
#108749=CARTESIAN_POINT('Ctrl Pts',(-1.43884669881289,17.1807833691985,
91.2522997957345));
#108750=CARTESIAN_POINT('Ctrl Pts',(-1.61435350422044,17.1605299420458,
91.2097102767348));
#108751=CARTESIAN_POINT('Ctrl Pts',(-1.79267599243096,17.1403533403081,
91.167573167666));
#108752=CARTESIAN_POINT('Ctrl Pts',(-1.91617722419394,17.1263795830304,
91.1383901693513));
#108753=CARTESIAN_POINT('Ctrl Pts',(-2.04102934044662,17.1124426471024,
91.1094251287446));
#108754=CARTESIAN_POINT('Ctrl Pts',(-2.16725422868345,17.0985502660013,
91.0808133862865));
#108755=CARTESIAN_POINT('Ctrl Pts',(-2.35033670000424,17.0784001078191,
91.039313579147));
#108756=CARTESIAN_POINT('Ctrl Pts',(-2.53630681046979,17.0583437581363,
90.9985550023606));
#108757=CARTESIAN_POINT('Ctrl Pts',(-2.72521885022047,17.0384034578628,
90.9589637064745));
#108758=CARTESIAN_POINT('Ctrl Pts',(-2.77851356008927,17.0327780222411,
90.9477944520936));
#108759=CARTESIAN_POINT('Ctrl Pts',(-2.8320424923009,17.0271618127094,90.9367184053569));
#108760=CARTESIAN_POINT('Ctrl Pts',(-2.88580705358031,17.0215553046092,
90.9257458669384));
#108761=CARTESIAN_POINT('Ctrl Pts',(7.13360610883155,18.0489603905536,92.656111537346));
#108762=CARTESIAN_POINT('Ctrl Pts',(7.08720655217987,18.0489603905536,92.6528812781694));
#108763=CARTESIAN_POINT('Ctrl Pts',(6.78071640479514,18.0489603905535,92.630985806519));
#108764=CARTESIAN_POINT('Ctrl Pts',(6.2119828023362,18.0489603905535,92.583698020234));
#108765=CARTESIAN_POINT('Ctrl Pts',(5.49686859880516,18.0489603905535,92.5126619062047));
#108766=CARTESIAN_POINT('Ctrl Pts',(5.04175854429137,18.0489603905536,92.4626226012838));
#108767=CARTESIAN_POINT('Ctrl Pts',(4.84744750318331,18.0489603905535,92.4406180506049));
#108768=CARTESIAN_POINT('Ctrl Pts',(7.15347472990633,18.3413983276278,92.3707114414248));
#108769=CARTESIAN_POINT('Ctrl Pts',(7.10741885836741,18.3413983276278,92.3675051220259));
#108770=CARTESIAN_POINT('Ctrl Pts',(6.80316531209303,18.3413983276278,92.3457695710735));
#108771=CARTESIAN_POINT('Ctrl Pts',(6.23816628212326,18.3413983276278,92.2987954908767));
#108772=CARTESIAN_POINT('Ctrl Pts',(5.52672801243274,18.3413983276278,92.2281285588862));
#108773=CARTESIAN_POINT('Ctrl Pts',(5.07333129942109,18.3413983276278,92.178278547464));
#108774=CARTESIAN_POINT('Ctrl Pts',(4.87963860009015,18.3413983276278,92.1563440553926));
#108775=CARTESIAN_POINT('Ctrl Pts',(7.17966409107166,18.5000186763427,91.9945179370873));
#108776=CARTESIAN_POINT('Ctrl Pts',(7.1340612400775,18.5000186763427,91.99134317335));
#108777=CARTESIAN_POINT('Ctrl Pts',(6.83275581758214,18.5000186763427,91.9698184181487));
#108778=CARTESIAN_POINT('Ctrl Pts',(6.27267942755774,18.5000186763427,91.9232578423394));
#108779=CARTESIAN_POINT('Ctrl Pts',(5.56608650463578,18.5000186763427,91.8530775390801));
#108780=CARTESIAN_POINT('Ctrl Pts',(5.11494819291141,18.5000186763427,91.8034770404832));
#108781=CARTESIAN_POINT('Ctrl Pts',(4.92207054642514,18.5000186763427,91.7816348945371));
#108782=CARTESIAN_POINT('Ctrl Pts',(7.20807595092437,18.4999999984374,91.5863996536418));
#108783=CARTESIAN_POINT('Ctrl Pts',(7.16296456500068,18.4999999984374,91.5832591234633));
#108784=CARTESIAN_POINT('Ctrl Pts',(6.86485745189238,18.4999999984374,91.5619630527001));
#108785=CARTESIAN_POINT('Ctrl Pts',(6.31012145010241,18.4999999984374,91.5158510723617));
#108786=CARTESIAN_POINT('Ctrl Pts',(5.60878506293612,18.4999999984374,91.4461986944349));
#108787=CARTESIAN_POINT('Ctrl Pts',(5.16009680642433,18.4999999984374,91.3968688829852));
#108788=CARTESIAN_POINT('Ctrl Pts',(4.96810338033001,18.4999999984374,91.3751269199019));
#108789=CARTESIAN_POINT('Ctrl Pts',(6.72284172768286,18.2005852686258,92.4518051511202));
#108790=CARTESIAN_POINT('Ctrl Pts',(6.56248534649459,18.1888402301925,92.4546733255583));
#108791=CARTESIAN_POINT('Ctrl Pts',(6.39755478889078,18.1764291564116,92.4565176179318));
#108792=CARTESIAN_POINT('Ctrl Pts',(6.22811698030556,18.1633144621374,92.4572506935924));
#108793=CARTESIAN_POINT('Ctrl Pts',(6.05247392496364,18.1497194741508,92.4580106163623));
#108794=CARTESIAN_POINT('Ctrl Pts',(5.87198765880911,18.1353682168452,92.4575754540388));
#108795=CARTESIAN_POINT('Ctrl Pts',(5.6867391554217,18.1202251711888,92.4558938992821));
#108796=CARTESIAN_POINT('Ctrl Pts',(5.60442573979155,18.1134965024642,92.4551467163734));
#108797=CARTESIAN_POINT('Ctrl Pts',(5.52117232550561,18.1066116018656,92.4541540424841));
#108798=CARTESIAN_POINT('Ctrl Pts',(5.43698724844798,18.0995678722315,92.4529144738207));
#108799=CARTESIAN_POINT('Ctrl Pts',(5.25646043165824,18.0844632701615,92.4502563378088));
#108800=CARTESIAN_POINT('Ctrl Pts',(5.07164929495735,18.0686277269766,92.4464594893415));
#108801=CARTESIAN_POINT('Ctrl Pts',(4.88262110769245,18.0520415606046,92.441552020789));
#108802=CARTESIAN_POINT('Ctrl Pts',(4.87094861310268,18.0510173644779,92.4412489845013));
#108803=CARTESIAN_POINT('Ctrl Pts',(4.8592600399789,18.0499903089639,92.4409417297409));
#108804=CARTESIAN_POINT('Ctrl Pts',(4.8475554046566,18.0489603905536,92.4406302697285));
#108805=CARTESIAN_POINT('Ctrl Pts',(7.18082400639694,18.5000000000005,91.584560428554));
#108806=CARTESIAN_POINT('Ctrl Pts',(7.14487677550867,18.5000000000002,91.5820310344745));
#108807=CARTESIAN_POINT('Ctrl Pts',(7.10884978221285,18.4999999999997,91.5794443189311));
#108808=CARTESIAN_POINT('Ctrl Pts',(7.07274752685978,18.4999999999993,91.5768011237233));
#108809=CARTESIAN_POINT('Ctrl Pts',(6.88293336141999,18.499999999997,91.5629040447862));
#108810=CARTESIAN_POINT('Ctrl Pts',(6.69103906347306,18.5000000000007,91.5474409142852));
#108811=CARTESIAN_POINT('Ctrl Pts',(6.49769479188341,18.5000000000007,91.5305920653784));
#108812=CARTESIAN_POINT('Ctrl Pts',(6.4366209629962,18.5000000000007,91.5252698300382));
#108813=CARTESIAN_POINT('Ctrl Pts',(6.3754022841721,18.5,91.5198101796099));
#108814=CARTESIAN_POINT('Ctrl Pts',(6.31407521179294,18.4999999999975,91.5142211124991));
#108815=CARTESIAN_POINT('Ctrl Pts',(6.12154672848197,18.4999999999896,91.4966749526676));
#108816=CARTESIAN_POINT('Ctrl Pts',(5.92795006091614,18.5000000000007,91.4778488501071));
#108817=CARTESIAN_POINT('Ctrl Pts',(5.73440041763818,18.5000000000007,91.4580452702999));
#108818=CARTESIAN_POINT('Ctrl Pts',(5.67091376130322,18.5000000000007,91.4515494532882));
#108819=CARTESIAN_POINT('Ctrl Pts',(5.60743228514628,18.4999999999864,91.4449481438494));
#108820=CARTESIAN_POINT('Ctrl Pts',(5.54394144600132,18.499999999908,91.4382493462182));
#108821=CARTESIAN_POINT('Ctrl Pts',(5.35221348028708,18.4999999996713,91.4180204933653));
#108822=CARTESIAN_POINT('Ctrl Pts',(5.1604002946779,18.4999999984373,91.396903250989));
#108823=CARTESIAN_POINT('Ctrl Pts',(4.96810338032909,18.4999999984373,91.37512691991));
#108824=CARTESIAN_POINT('Origin',(155.459720656869,18.5,57.01928063319));
#108825=CARTESIAN_POINT('',(-2.58374595115891,18.49999969586,89.45559971935));
#108826=CARTESIAN_POINT('Origin',(-3.78022426533191,17.,89.66699908298));
#108827=CARTESIAN_POINT('',(-2.84365663233891,17.00000044005,87.97871656704));
#108828=CARTESIAN_POINT('Ctrl Pts',(8.45816176827909,16.26511926842,98.7964653589499));
#108829=CARTESIAN_POINT('Ctrl Pts',(8.71225114275908,16.41477280571,98.6494070076199));
#108830=CARTESIAN_POINT('Ctrl Pts',(9.27881268981909,16.73006084598,98.30341626023));
#108831=CARTESIAN_POINT('Ctrl Pts',(10.1626398113191,17.16069654247,97.6962496853799));
#108832=CARTESIAN_POINT('Ctrl Pts',(11.1008309226691,17.54981639277,96.96627400869));
#108833=CARTESIAN_POINT('Ctrl Pts',(12.0284701745891,17.86984908755,96.1523318668001));
#108834=CARTESIAN_POINT('Ctrl Pts',(12.9325147810891,18.12067756051,95.26102236673));
#108835=CARTESIAN_POINT('Ctrl Pts',(13.8034582743191,18.30536666785,94.2997004316301));
#108836=CARTESIAN_POINT('Ctrl Pts',(14.6483615697391,18.43072561429,93.2588424428));
#108837=CARTESIAN_POINT('Ctrl Pts',(15.4901719996691,18.50141397362,92.10037160054));
#108838=CARTESIAN_POINT('Ctrl Pts',(16.3530907398691,18.51438369082,90.76409474325));
#108839=CARTESIAN_POINT('Ctrl Pts',(17.2403956363891,18.45914837749,89.19684938304));
#108840=CARTESIAN_POINT('Ctrl Pts',(18.1343401599191,18.32423291388,87.36260202144));
#108841=CARTESIAN_POINT('Ctrl Pts',(19.0033848293491,18.10320054974,85.24319884147));
#108842=CARTESIAN_POINT('Ctrl Pts',(19.7639909942691,17.81526535809,82.9702592037509));
#108843=CARTESIAN_POINT('Ctrl Pts',(20.1883444225591,17.59455708305,81.382235884647));
#108844=CARTESIAN_POINT('Ctrl Pts',(20.3703684052891,17.48632437673,80.615759308313));
#108845=CARTESIAN_POINT('Ctrl Pts',(6.31418014116909,15.43220418763,92.79563719768));
#108846=CARTESIAN_POINT('Ctrl Pts',(6.49200941171909,15.56346847277,92.67838236751));
#108847=CARTESIAN_POINT('Ctrl Pts',(6.88387432291909,15.84414338516,92.4035075448201));
#108848=CARTESIAN_POINT('Ctrl Pts',(7.48196966441909,16.24577547329,91.9242120499101));
#108849=CARTESIAN_POINT('Ctrl Pts',(8.10612356461909,16.6365848729,91.3501649846601));
#108850=CARTESIAN_POINT('Ctrl Pts',(8.71750994518909,16.99297183984,90.71045662041));
#108851=CARTESIAN_POINT('Ctrl Pts',(9.3124519476191,17.31472032014,90.0082381109));
#108852=CARTESIAN_POINT('Ctrl Pts',(9.88895414563909,17.60257331209,89.2471181028301));
#108853=CARTESIAN_POINT('Ctrl Pts',(10.4549508437891,17.8618188302,88.41744323317));
#108854=CARTESIAN_POINT('Ctrl Pts',(11.0287137839791,18.10025681166,87.4864837035));
#108855=CARTESIAN_POINT('Ctrl Pts',(11.6304101411391,18.32271215478,86.40251363781));
#108856=CARTESIAN_POINT('Ctrl Pts',(12.2670974264291,18.52555248364,85.11784149556));
#108857=CARTESIAN_POINT('Ctrl Pts',(12.9309003101591,18.69913435731,83.5979370835401));
#108858=CARTESIAN_POINT('Ctrl Pts',(13.6016889453491,18.83244677012,81.8239640921051));
#108859=CARTESIAN_POINT('Ctrl Pts',(14.2139669773891,18.91249476228,79.9062655709491));
#108860=CARTESIAN_POINT('Ctrl Pts',(14.5696327416291,18.93553052461,78.560927762134));
#108861=CARTESIAN_POINT('Ctrl Pts',(14.7249351849991,18.94108956235,77.911474252923));
#108862=CARTESIAN_POINT('Ctrl Pts',(2.54935064044909,19.22183178223,89.2228044174901));
#108863=CARTESIAN_POINT('Ctrl Pts',(2.74816966526909,19.38069675838,89.11271227861));
#108864=CARTESIAN_POINT('Ctrl Pts',(3.18450270870909,19.72231812323,88.8567707992701));
#108865=CARTESIAN_POINT('Ctrl Pts',(3.84607183220909,20.21957457743,88.41774917846));
#108866=CARTESIAN_POINT('Ctrl Pts',(4.53420387286909,20.71569136082,87.89920721743));
#108867=CARTESIAN_POINT('Ctrl Pts',(5.20913049307909,21.18237918094,87.3269794904301));
#108868=CARTESIAN_POINT('Ctrl Pts',(5.86983667115909,21.61932357701,86.70255461879));
#108869=CARTESIAN_POINT('Ctrl Pts',(6.5166169471191,22.02651478544,86.02752892074));
#108870=CARTESIAN_POINT('Ctrl Pts',(7.16026643121909,22.41003287152,85.29176070735));
#108871=CARTESIAN_POINT('Ctrl Pts',(7.82357909374909,22.78105285215,84.46472655768));
#108872=CARTESIAN_POINT('Ctrl Pts',(8.5330095959891,23.14891805727,83.49874325701));
#108873=CARTESIAN_POINT('Ctrl Pts',(9.30144695145909,23.51183300341,82.349167312438));
#108874=CARTESIAN_POINT('Ctrl Pts',(10.1247389211891,23.8583235636,80.982966536629));
#108875=CARTESIAN_POINT('Ctrl Pts',(10.9831261496691,24.1725563834,79.382122199941));
#108876=CARTESIAN_POINT('Ctrl Pts',(11.7956651902091,24.42485648488,77.6476829007421));
#108877=CARTESIAN_POINT('Ctrl Pts',(12.2871279910191,24.55396132786,76.431541471836));
#108878=CARTESIAN_POINT('Ctrl Pts',(12.5064116716291,24.60764795684,75.845400513527));
#108879=CARTESIAN_POINT('Ctrl Pts',(-0.111615554140913,24.89134380645,90.66372486418));
#108880=CARTESIAN_POINT('Ctrl Pts',(0.19025221778909,25.10382403371,90.53297074905));
#108881=CARTESIAN_POINT('Ctrl Pts',(0.85803534504909,25.557842799,90.23007744772));
#108882=CARTESIAN_POINT('Ctrl Pts',(1.88634608190909,26.20614559666,89.71458517922));
#108883=CARTESIAN_POINT('Ctrl Pts',(2.97016886586909,26.83497373368,89.11095423698));
#108884=CARTESIAN_POINT('Ctrl Pts',(4.04244300886909,27.40608121153,88.4506164042799));
#108885=CARTESIAN_POINT('Ctrl Pts',(5.09618479047909,27.91912696323,87.73638641167));
#108886=CARTESIAN_POINT('Ctrl Pts',(6.1271003298391,28.37546235392,86.9710385745999));
#108887=CARTESIAN_POINT('Ctrl Pts',(7.14876251537909,28.78369951161,86.14393771161));
#108888=CARTESIAN_POINT('Ctrl Pts',(8.19441250288909,29.15618061071,85.2220293390399));
#108889=CARTESIAN_POINT('Ctrl Pts',(9.30256349945909,29.50014277728,84.1543224935201));
#108890=CARTESIAN_POINT('Ctrl Pts',(10.4897674388291,29.80928089036,82.894592873641));
#108891=CARTESIAN_POINT('Ctrl Pts',(11.7467525600991,30.0679526902,81.410216850361));
#108892=CARTESIAN_POINT('Ctrl Pts',(13.0428227217091,30.25874444737,79.684901641459));
#108893=CARTESIAN_POINT('Ctrl Pts',(14.2592774845091,30.36290197067,77.829109904896));
#108894=CARTESIAN_POINT('Ctrl Pts',(14.9927419533391,30.38363581186,76.53517273404));
#108895=CARTESIAN_POINT('Ctrl Pts',(15.3204046577991,30.3849546111,75.912812767194));
#108896=CARTESIAN_POINT('Origin',(4.08384678615258,24.7092212049592,99.2019244382985));
#108897=CARTESIAN_POINT('Ctrl Pts',(-1.86852584115091,-0.200657301970986,
95.96514097396));
#108898=CARTESIAN_POINT('Ctrl Pts',(-1.87679361636091,0.397260618019714,
95.95539499753));
#108899=CARTESIAN_POINT('Ctrl Pts',(-1.81764502158091,1.61545674784001,
96.02675082903));
#108900=CARTESIAN_POINT('Ctrl Pts',(-1.51056034305091,3.37210791261202,
96.3812545342701));
#108901=CARTESIAN_POINT('Ctrl Pts',(-1.03549752546091,4.99180633572701,
96.87949059878));
#108902=CARTESIAN_POINT('Ctrl Pts',(-0.47565565201091,6.40141962980201,
97.39996719591));
#108903=CARTESIAN_POINT('Ctrl Pts',(0.128959222729088,7.63825880799903,
97.89143667163));
#108904=CARTESIAN_POINT('Ctrl Pts',(0.78047764573909,8.77397550221601,98.34798763131));
#108905=CARTESIAN_POINT('Ctrl Pts',(1.50402784399909,9.87146117248002,98.77288024243));
#108906=CARTESIAN_POINT('Ctrl Pts',(2.31936621098909,10.95615772036,99.1532466824299));
#108907=CARTESIAN_POINT('Ctrl Pts',(3.21879357943909,12.01000937004,99.45696306809));
#108908=CARTESIAN_POINT('Ctrl Pts',(4.1912683517691,13.0170795927,99.65335362598));
#108909=CARTESIAN_POINT('Ctrl Pts',(5.2757469215191,14.01086777604,99.7165874722901));
#108910=CARTESIAN_POINT('Ctrl Pts',(6.5351502248891,15.02007613619,99.5796055175001));
#108911=CARTESIAN_POINT('Ctrl Pts',(7.73731890968909,15.84006914657,99.1892695249101));
#108912=CARTESIAN_POINT('Ctrl Pts',(8.5044225018091,16.29480837482,98.77493643233));
#108913=CARTESIAN_POINT('Ctrl Pts',(8.76798669870909,16.44357118509,98.6108142135001));
#108914=CARTESIAN_POINT('Ctrl Pts',(-2.76633335145391,-0.277061106735686,
89.62464525754));
#108915=CARTESIAN_POINT('Ctrl Pts',(-2.78010061236391,0.548141406161314,
89.61313564381));
#108916=CARTESIAN_POINT('Ctrl Pts',(-2.67974655644691,2.23539163023501,
89.69951614818));
#108917=CARTESIAN_POINT('Ctrl Pts',(-2.18690829439091,4.52753916756702,
90.11267233159));
#108918=CARTESIAN_POINT('Ctrl Pts',(-1.49193309304091,6.44657897676101,
90.65739218289));
#108919=CARTESIAN_POINT('Ctrl Pts',(-0.744560214060911,7.96637647141302,
91.1950322953901));
#108920=CARTESIAN_POINT('Ctrl Pts',(-0.000714101840911076,9.19387013708703,
91.67997579193));
#108921=CARTESIAN_POINT('Ctrl Pts',(0.743218764159092,10.2409288401,92.11363373692));
#108922=CARTESIAN_POINT('Ctrl Pts',(1.51015059767909,11.1834522333,92.50353807267));
#108923=CARTESIAN_POINT('Ctrl Pts',(2.30766423261909,12.04981733614,92.84138179648));
#108924=CARTESIAN_POINT('Ctrl Pts',(3.11198293474909,12.83069438562,93.10362209738));
#108925=CARTESIAN_POINT('Ctrl Pts',(3.89792431306909,13.52231896489,93.27156799052));
#108926=CARTESIAN_POINT('Ctrl Pts',(4.67814510883909,14.15587807635,93.33468615681));
#108927=CARTESIAN_POINT('Ctrl Pts',(5.4599957395091,14.75400852768,93.25754212455));
#108928=CARTESIAN_POINT('Ctrl Pts',(6.06740744298909,15.2155704877,93.02226348412));
#108929=CARTESIAN_POINT('Ctrl Pts',(6.38629556221909,15.47756556229,92.7840149103));
#108930=CARTESIAN_POINT('Ctrl Pts',(6.48862860801909,15.56565674012,92.69092482342));
#108931=CARTESIAN_POINT('Ctrl Pts',(-8.21314323670391,-0.382376649944286,
86.25787732271));
#108932=CARTESIAN_POINT('Ctrl Pts',(-8.23233050746892,0.756384491850314,
86.2455034223201));
#108933=CARTESIAN_POINT('Ctrl Pts',(-8.09201734092391,3.08654305365901,
86.33967991873));
#108934=CARTESIAN_POINT('Ctrl Pts',(-7.41007493507491,6.21008628532401,
86.78035394901));
#108935=CARTESIAN_POINT('Ctrl Pts',(-6.46595117430891,8.76366891642203,
87.33791220527));
#108936=CARTESIAN_POINT('Ctrl Pts',(-5.47046355413091,10.73360469488,87.86524851897));
#108937=CARTESIAN_POINT('Ctrl Pts',(-4.49835120662891,12.28405501304,88.3219438496));
#108938=CARTESIAN_POINT('Ctrl Pts',(-3.54419140703191,13.57328011442,88.71413997378));
#108939=CARTESIAN_POINT('Ctrl Pts',(-2.58024571757991,14.70275906295,89.05110200106));
#108940=CARTESIAN_POINT('Ctrl Pts',(-1.60151740187091,15.70963613843,89.32658646923));
#108941=CARTESIAN_POINT('Ctrl Pts',(-0.643241151590912,16.5857007526,89.52289696124));
#108942=CARTESIAN_POINT('Ctrl Pts',(0.258320540729089,17.33121239699,89.6296159923701));
#108943=CARTESIAN_POINT('Ctrl Pts',(1.10917349098909,17.98470665617,89.644481026));
#108944=CARTESIAN_POINT('Ctrl Pts',(1.89817703664909,18.57234274478,89.5498507959201));
#108945=CARTESIAN_POINT('Ctrl Pts',(2.42972632590909,19.00878869518,89.36136454575));
#108946=CARTESIAN_POINT('Ctrl Pts',(2.66092298708909,19.26095009207,89.20319983242));
#108947=CARTESIAN_POINT('Ctrl Pts',(2.72918498241909,19.3474423808,89.14448415142));
#108948=CARTESIAN_POINT('Ctrl Pts',(-14.2862958551049,-0.440758245828086,
88.2895013269199));
#108949=CARTESIAN_POINT('Ctrl Pts',(-14.3069203009679,0.872018283434913,
88.2777849287));
#108950=CARTESIAN_POINT('Ctrl Pts',(-14.1566719512549,3.55593252096201,
88.36691425296));
#108951=CARTESIAN_POINT('Ctrl Pts',(-13.4184630337948,7.20801986586801,
88.78415381662));
#108952=CARTESIAN_POINT('Ctrl Pts',(-12.3753852541951,10.27436448968,89.3116591898701));
#108953=CARTESIAN_POINT('Ctrl Pts',(-11.2498853426949,12.71021402121,89.8086449352));
#108954=CARTESIAN_POINT('Ctrl Pts',(-10.1248635377679,14.68333765206,90.23571355337));
#108955=CARTESIAN_POINT('Ctrl Pts',(-8.99406462449291,16.37115120725,90.59773884278));
#108956=CARTESIAN_POINT('Ctrl Pts',(-7.82135743268891,17.89486271208,90.90193228787));
#108957=CARTESIAN_POINT('Ctrl Pts',(-6.59288141698792,19.29990188201,91.1401305760401));
#108958=CARTESIAN_POINT('Ctrl Pts',(-5.34245787553691,20.5707644631,91.2935385755));
#108959=CARTESIAN_POINT('Ctrl Pts',(-4.10638909157991,21.70068773103,91.3503426401699));
#108960=CARTESIAN_POINT('Ctrl Pts',(-2.86088161342491,22.73992455031,91.30356781784));
#108961=CARTESIAN_POINT('Ctrl Pts',(-1.58517092003091,23.72520760639,91.1267204027899));
#108962=CARTESIAN_POINT('Ctrl Pts',(-0.555955217310912,24.48794052554,90.8430628426899));
#108963=CARTESIAN_POINT('Ctrl Pts',(0.0112272501190876,24.92026069551,90.6113068883499));
#108964=CARTESIAN_POINT('Ctrl Pts',(0.19711543522909,25.06537831943,90.52555227838));
#108965=CARTESIAN_POINT('Ctrl Pts',(-2.88573408563691,17.02155009774,90.92539099034));
#108966=CARTESIAN_POINT('Ctrl Pts',(-2.96183724836951,16.4511697392406,
90.9180810733755));
#108967=CARTESIAN_POINT('Ctrl Pts',(-3.04690368141671,15.8694125167351,
90.9103090292122));
#108968=CARTESIAN_POINT('Ctrl Pts',(-3.21791408217198,14.6867343619779,
90.8916484242105));
#108969=CARTESIAN_POINT('Ctrl Pts',(-3.3054459106508,14.0847518433696,90.8810444512336));
#108970=CARTESIAN_POINT('Ctrl Pts',(-3.4784887655845,12.8570207383856,90.8576637353644));
#108971=CARTESIAN_POINT('Ctrl Pts',(-3.56417210664204,12.2314460226776,
90.8449209670427));
#108972=CARTESIAN_POINT('Ctrl Pts',(-3.68821978087207,11.276327570869,90.8246954161696));
#108973=CARTESIAN_POINT('Ctrl Pts',(-3.749143296294,10.794578024796,90.8143068483821));
#108974=CARTESIAN_POINT('Ctrl Pts',(-3.81793083944601,10.2250983369176,
90.8018485621806));
#108975=CARTESIAN_POINT('Ctrl Pts',(-3.8517045182457,9.93848577016983,90.7955508744864));
#108976=CARTESIAN_POINT('Ctrl Pts',(-3.87022234814949,9.77930508945704,
90.7920478215217));
#108977=CARTESIAN_POINT('Ctrl Pts',(-3.87912764195531,9.70212460187384,
90.7903480188845));
#108978=CARTESIAN_POINT('Ctrl Pts',(-3.883863232778,9.66092239636872,90.7894403356581));
#108979=CARTESIAN_POINT('Ctrl Pts',(-3.88463248027389,9.654224946255,90.7892927837586));
#108980=CARTESIAN_POINT('Ctrl Pts',(-4.09696574678048,7.80475446997897,
90.7485457770365));
#108981=CARTESIAN_POINT('Ctrl Pts',(-4.25603208569112,6.03090266346487,
90.7104679588609));
#108982=CARTESIAN_POINT('Ctrl Pts',(-4.35611208131979,4.33088849294624,
90.6854742441241));
#108983=CARTESIAN_POINT('Ctrl Pts',(-2.57931668725691,17.178594621,90.9548069667399));
#108984=CARTESIAN_POINT('Ctrl Pts',(-2.58855911478591,16.91432196328,90.9564366560799));
#108985=CARTESIAN_POINT('Ctrl Pts',(-2.63992248125991,15.8335002163,90.96549340341));
#108986=CARTESIAN_POINT('Ctrl Pts',(-2.75745612978091,13.99840023162,90.98621775678));
#108987=CARTESIAN_POINT('Ctrl Pts',(-2.91746701901391,11.74002179927,91.0144319937601));
#108988=CARTESIAN_POINT('Ctrl Pts',(-3.05666088400791,9.68164557974802,
91.03897562771));
#108989=CARTESIAN_POINT('Ctrl Pts',(-3.17062879146191,7.82843465735002,
91.05907124473));
#108990=CARTESIAN_POINT('Ctrl Pts',(-3.25937285896191,6.15995521921902,
91.0747192182));
#108991=CARTESIAN_POINT('Ctrl Pts',(-3.32585864265091,4.64679437283801,
91.0864424557));
#108992=CARTESIAN_POINT('Ctrl Pts',(-3.37219209949591,3.26397330020801,
91.09461229425));
#108993=CARTESIAN_POINT('Ctrl Pts',(-3.40128627417591,1.99700231674801,
91.09974238223));
#108994=CARTESIAN_POINT('Ctrl Pts',(-3.41591456021491,0.864740186840713,
91.10232174374));
#108995=CARTESIAN_POINT('Ctrl Pts',(-3.41758620937791,0.154606727500314,
91.10261650059));
#108996=CARTESIAN_POINT('Ctrl Pts',(-3.41699227803491,-0.170855566085486,
91.10251177447));
#108997=CARTESIAN_POINT('Ctrl Pts',(-3.46696900914091,17.21014669308,90.95337008737));
#108998=CARTESIAN_POINT('Ctrl Pts',(-3.47583374334891,16.95150699925,90.95493317919));
#108999=CARTESIAN_POINT('Ctrl Pts',(-3.52514838430391,15.88442344691,90.96362868093));
#109000=CARTESIAN_POINT('Ctrl Pts',(-3.64301280433791,14.06098388959,90.98441135825));
#109001=CARTESIAN_POINT('Ctrl Pts',(-3.80271901722991,11.80179697056,91.01257187257));
#109002=CARTESIAN_POINT('Ctrl Pts',(-3.94227500929891,9.73936414453901,
91.03717935929));
#109003=CARTESIAN_POINT('Ctrl Pts',(-4.05662374314791,7.87974649728102,
91.05734212628));
#109004=CARTESIAN_POINT('Ctrl Pts',(-4.14580292510191,6.20322316682401,
91.07306682217));
#109005=CARTESIAN_POINT('Ctrl Pts',(-4.21266473965291,4.68161991703801,
91.08485636406));
#109006=CARTESIAN_POINT('Ctrl Pts',(-4.25933036892191,3.28889700319401,
91.09308477357));
#109007=CARTESIAN_POINT('Ctrl Pts',(-4.28862172007191,2.01347313433601,
91.09824962908));
#109008=CARTESIAN_POINT('Ctrl Pts',(-4.30337790490591,0.871605021979214,
91.1008515426));
#109009=CARTESIAN_POINT('Ctrl Pts',(-4.30506192324491,0.155435836660514,
91.10114848047));
#109010=CARTESIAN_POINT('Ctrl Pts',(-4.30446363595191,-0.172497509604886,
91.10104298627));
#109011=CARTESIAN_POINT('Ctrl Pts',(-4.08960379568891,17.22831955499,90.3208814529201));
#109012=CARTESIAN_POINT('Ctrl Pts',(-4.09825099208891,16.97292424633,90.32240618695));
#109013=CARTESIAN_POINT('Ctrl Pts',(-4.14638564062291,15.91375340138,90.3308936241901));
#109014=CARTESIAN_POINT('Ctrl Pts',(-4.26444057318591,14.09702983202,90.35170989401));
#109015=CARTESIAN_POINT('Ctrl Pts',(-4.42397130343291,11.83737725366,90.3798394660001));
#109016=CARTESIAN_POINT('Ctrl Pts',(-4.56373586770891,9.77260796779402,
90.4044837296301));
#109017=CARTESIAN_POINT('Ctrl Pts',(-4.67830394390391,7.90930027679202,
90.42468517259));
#109018=CARTESIAN_POINT('Ctrl Pts',(-4.76773373617791,6.22814395284801,
90.44045405785));
#109019=CARTESIAN_POINT('Ctrl Pts',(-4.83481213101691,4.70167818148601,
90.45228178868));
#109020=CARTESIAN_POINT('Ctrl Pts',(-4.88166907968991,3.30325216223001,
90.46054393297));
#109021=CARTESIAN_POINT('Ctrl Pts',(-4.91107399741491,2.02295973454401,
90.46572881333));
#109022=CARTESIAN_POINT('Ctrl Pts',(-4.92590384736791,0.875558920813114,
90.46834371599));
#109023=CARTESIAN_POINT('Ctrl Pts',(-4.92759498990891,0.155913373800914,
90.46864191005));
#109024=CARTESIAN_POINT('Ctrl Pts',(-4.92699419374391,-0.173443210183986,
90.4685359734801));
#109025=CARTESIAN_POINT('Ctrl Pts',(-4.07693104810691,17.2223055404,89.4334912894));
#109026=CARTESIAN_POINT('Ctrl Pts',(-4.08565023512491,16.96583655497,89.4350287173199));
#109027=CARTESIAN_POINT('Ctrl Pts',(-4.13417538305591,15.90404712755,89.44358501014));
#109028=CARTESIAN_POINT('Ctrl Pts',(-4.25216726858091,14.08510101065,89.46439016306));
#109029=CARTESIAN_POINT('Ctrl Pts',(-4.41175607196891,11.82560253471,89.49252997492));
#109030=CARTESIAN_POINT('Ctrl Pts',(-4.55145161264891,9.76160646242102,
89.5171620678199));
#109031=CARTESIAN_POINT('Ctrl Pts',(-4.66594710104291,7.89951993168502,
89.5373507115999));
#109032=CARTESIAN_POINT('Ctrl Pts',(-4.75529395788691,6.21989682196801,
89.5531049731));
#109033=CARTESIAN_POINT('Ctrl Pts',(-4.82230067898491,4.69504022343901,
89.5649200659201));
#109034=CARTESIAN_POINT('Ctrl Pts',(-4.86909431359692,3.29850155463401,
89.57317104623));
#109035=CARTESIAN_POINT('Ctrl Pts',(-4.89846164830091,2.01982029771201,
89.57834929969));
#109036=CARTESIAN_POINT('Ctrl Pts',(-4.91326711997491,0.874250441973816,
89.5809599038099));
#109037=CARTESIAN_POINT('Ctrl Pts',(-4.91495590487691,0.155755340611514,
89.58125768215));
#109038=CARTESIAN_POINT('Ctrl Pts',(-4.91435593898191,-0.173130245880086,
89.58115189197));
#109039=CARTESIAN_POINT('Ctrl Pts',(-4.06425830052491,17.21629152582,88.5461011258701));
#109040=CARTESIAN_POINT('Ctrl Pts',(-4.07304947815991,16.95874886361,88.54765124768));
#109041=CARTESIAN_POINT('Ctrl Pts',(-4.12196512548991,15.89434085372,88.55627639609));
#109042=CARTESIAN_POINT('Ctrl Pts',(-4.23989396397591,14.07317218928,88.57707043212));
#109043=CARTESIAN_POINT('Ctrl Pts',(-4.39954084050591,11.81382781576,88.60522048383));
#109044=CARTESIAN_POINT('Ctrl Pts',(-4.53916735758791,9.75060495704802,
88.6298404060201));
#109045=CARTESIAN_POINT('Ctrl Pts',(-4.65359025818291,7.88973958657902,
88.6500162506));
#109046=CARTESIAN_POINT('Ctrl Pts',(-4.74285417959691,6.21164969108801,
88.66575588835));
#109047=CARTESIAN_POINT('Ctrl Pts',(-4.80978922695191,4.68840226539201,
88.67755834316));
#109048=CARTESIAN_POINT('Ctrl Pts',(-4.85651954750292,3.29375094703901,
88.68579815949));
#109049=CARTESIAN_POINT('Ctrl Pts',(-4.88584929918791,2.01668086088001,
88.6909697860501));
#109050=CARTESIAN_POINT('Ctrl Pts',(-4.90063039258292,0.872941963134614,
88.69357609162));
#109051=CARTESIAN_POINT('Ctrl Pts',(-4.90231681984491,0.155597307422214,
88.69387345424));
#109052=CARTESIAN_POINT('Ctrl Pts',(-4.90171768422091,-0.172817281576286,
88.69376781047));
#109053=CARTESIAN_POINT('Ctrl Pts',(-3.42381468683891,17.18966725702,87.9315533205201));
#109054=CARTESIAN_POINT('Ctrl Pts',(-3.43292456964391,16.92737138735,87.93315963865));
#109055=CARTESIAN_POINT('Ctrl Pts',(-3.48356897249791,15.85137081435,87.94208961329));
#109056=CARTESIAN_POINT('Ctrl Pts',(-3.60121869937191,14.02036284834,87.96283443442));
#109057=CARTESIAN_POINT('Ctrl Pts',(-3.76112266788591,11.76170069203,87.99102981839));
#109058=CARTESIAN_POINT('Ctrl Pts',(-3.90044361490791,9.70190087892902,
88.01559586032));
#109059=CARTESIAN_POINT('Ctrl Pts',(-4.01454516658091,7.84644163089602,
88.03571504243));
#109060=CARTESIAN_POINT('Ctrl Pts',(-4.10344192972591,6.17513933245601,
88.05138994027));
#109061=CARTESIAN_POINT('Ctrl Pts',(-4.17005967472791,4.65901577542201,
88.0631364461));
#109062=CARTESIAN_POINT('Ctrl Pts',(-4.21650970155091,3.27271982851301,
88.07132683909));
#109063=CARTESIAN_POINT('Ctrl Pts',(-4.24567307178991,2.00278245593201,
88.0764691281101));
#109064=CARTESIAN_POINT('Ctrl Pts',(-4.26034624162691,0.867149278093414,
88.07905640384));
#109065=CARTESIAN_POINT('Ctrl Pts',(-4.26202223153091,0.154897688548214,
88.07935192608));
#109066=CARTESIAN_POINT('Ctrl Pts',(-4.26142677154591,-0.171431776830586,
88.0792469304201));
#109067=CARTESIAN_POINT('Ctrl Pts',(-2.53648137537091,17.15826657542,87.9553284263299));
#109068=CARTESIAN_POINT('Ctrl Pts',(-2.54596713928091,16.89036476946,87.95700102244));
#109069=CARTESIAN_POINT('Ctrl Pts',(-2.59865043763191,15.80069191927,87.96629050937));
#109070=CARTESIAN_POINT('Ctrl Pts',(-2.71597098007291,13.95807947397,87.9869772863899));
#109071=CARTESIAN_POINT('Ctrl Pts',(-2.87617816305591,11.70022192514,88.01522613526));
#109072=CARTESIAN_POINT('Ctrl Pts',(-3.01513872052991,9.64445925446003,
88.0397286308001));
#109073=CARTESIAN_POINT('Ctrl Pts',(-3.12886127305691,7.79537599108401,
88.05978098512));
#109074=CARTESIAN_POINT('Ctrl Pts',(-3.21732500947791,6.13207898944801,
88.0753795286699));
#109075=CARTESIAN_POINT('Ctrl Pts',(-3.28356852785791,4.62435732819501,
88.08706004825));
#109076=CARTESIAN_POINT('Ctrl Pts',(-3.32968797605691,3.24791571232601,
88.09519215131));
#109077=CARTESIAN_POINT('Ctrl Pts',(-3.35865511590291,1.98639066722401,
88.1002998396201));
#109078=CARTESIAN_POINT('Ctrl Pts',(-3.37320100061691,0.860317381224614,
88.10286467155));
#109079=CARTESIAN_POINT('Ctrl Pts',(-3.37486468069391,0.154072557549214,
88.10315802323));
#109080=CARTESIAN_POINT('Ctrl Pts',(-3.37427355575891,-0.169797711545386,
88.10305379196));
#109081=CARTESIAN_POINT('Ctrl Pts',(-2.84365660865327,16.99999909128,87.978717018185));
#109082=CARTESIAN_POINT('Ctrl Pts',(-2.85128898638368,16.8100157247129,
87.9800628123056));
#109083=CARTESIAN_POINT('Ctrl Pts',(-2.86030160140771,16.62112233734,87.9816519784134));
#109084=CARTESIAN_POINT('Ctrl Pts',(-2.86985949636735,16.433171083534,87.9833372963379));
#109085=CARTESIAN_POINT('Ctrl Pts',(-2.87089428355535,16.4128225078039,
87.983519757581));
#109086=CARTESIAN_POINT('Ctrl Pts',(-2.871935511102,16.3924849781326,87.9837033544802));
#109087=CARTESIAN_POINT('Ctrl Pts',(-2.87298215385083,16.3721583088458,
87.9838879062745));
#109088=CARTESIAN_POINT('Ctrl Pts',(-2.88977696089625,16.0459892421528,
87.9868492909288));
#109089=CARTESIAN_POINT('Ctrl Pts',(-2.90796161402391,15.7226145279182,
87.9900557624761));
#109090=CARTESIAN_POINT('Ctrl Pts',(-2.92728126454367,15.4012022162267,
87.9934623326708));
#109091=CARTESIAN_POINT('Ctrl Pts',(-2.94004101473621,15.1889240074776,
87.9957122172975));
#109092=CARTESIAN_POINT('Ctrl Pts',(-2.95329710436232,14.9775023794641,
87.9980495955924));
#109093=CARTESIAN_POINT('Ctrl Pts',(-2.96698725787661,14.7667019575818,
88.000463539027));
#109094=CARTESIAN_POINT('Ctrl Pts',(-2.98536063308268,14.4837894803185,
88.0037032608026));
#109095=CARTESIAN_POINT('Ctrl Pts',(-3.0041303113058,14.2020331886729,88.0070129077448));
#109096=CARTESIAN_POINT('Ctrl Pts',(-3.02297301800919,13.9229688465034,
88.0103353860029));
#109097=CARTESIAN_POINT('Ctrl Pts',(-3.04601735495912,13.5816775005789,
88.0143987251873));
#109098=CARTESIAN_POINT('Ctrl Pts',(-3.06916808788408,13.2444133997815,
88.0184807898914));
#109099=CARTESIAN_POINT('Ctrl Pts',(-3.09199769385465,12.9141590882853,
88.0225062558434));
#109100=CARTESIAN_POINT('Ctrl Pts',(-3.09890463996465,12.8142428332681,
88.0237241339107));
#109101=CARTESIAN_POINT('Ctrl Pts',(-3.10578251136168,12.7149682011028,
88.0249368870126));
#109102=CARTESIAN_POINT('Ctrl Pts',(-3.1126205328836,12.6164177761549,88.0261426147017));
#109103=CARTESIAN_POINT('Ctrl Pts',(-3.1328805235663,12.3244282460229,88.0297149976884));
#109104=CARTESIAN_POINT('Ctrl Pts',(-3.15280524949456,12.0387689042729,
88.0332282706136));
#109105=CARTESIAN_POINT('Ctrl Pts',(-3.17219919081432,11.759013804942,88.0366479458216));
#109106=CARTESIAN_POINT('Ctrl Pts',(-3.17474417065642,11.7223027993354,
88.0370966944451));
#109107=CARTESIAN_POINT('Ctrl Pts',(-3.17728008219073,11.6856934685625,
88.0375438440236));
#109108=CARTESIAN_POINT('Ctrl Pts',(-3.17980654662979,11.6491848528322,
88.0379893277735));
#109109=CARTESIAN_POINT('Ctrl Pts',(-3.20356570844914,11.3058536364788,
88.0421787081336));
#109110=CARTESIAN_POINT('Ctrl Pts',(-3.22648679759717,10.9714287895626,
88.0462203093649));
#109111=CARTESIAN_POINT('Ctrl Pts',(-3.24849572832879,10.6451066340725,
88.0501010776695));
#109112=CARTESIAN_POINT('Ctrl Pts',(-3.27279220147798,10.2848675299772,
88.0543852014218));
#109113=CARTESIAN_POINT('Ctrl Pts',(-3.29590271860032,9.9345090800762,88.0584602108139));
#109114=CARTESIAN_POINT('Ctrl Pts',(-3.31782060896809,9.59382982703874,
88.0623249255647));
#109115=CARTESIAN_POINT('Ctrl Pts',(-3.33395684807769,9.34301728101119,
88.0651701793853));
#109116=CARTESIAN_POINT('Ctrl Pts',(-3.34944754773256,9.09745133352557,
88.0679016071817));
#109117=CARTESIAN_POINT('Ctrl Pts',(-3.36429765338097,8.85706270226158,
88.0705200814737));
#109118=CARTESIAN_POINT('Ctrl Pts',(-3.37034490299891,8.75917181225816,
88.0715863747404));
#109119=CARTESIAN_POINT('Ctrl Pts',(-3.37628552874775,8.66213886284631,
88.0726338673872));
#109120=CARTESIAN_POINT('Ctrl Pts',(-3.38212037964037,8.56594505080956,
88.0736627090807));
#109121=CARTESIAN_POINT('Origin',(33.1784433940591,111.0724296188,81.627048885766));
#109122=CARTESIAN_POINT('Origin',(-15.9175364833309,75.,72.98888938658));
#109123=CARTESIAN_POINT('',(-11.8763230992193,66.6,72.98888938658));
#109124=CARTESIAN_POINT('',(-12.3474397125099,66.60000000001,72.9889023406097));
#109125=CARTESIAN_POINT('',(-15.9175364833309,66.6,72.98888938658));
#109126=CARTESIAN_POINT('',(-12.9675940002345,76.1753006967198,81.3061780149303));
#109127=CARTESIAN_POINT('Ctrl Pts',(-11.8763230992193,66.6,72.98888938658));
#109128=CARTESIAN_POINT('Ctrl Pts',(-11.8794256424916,66.6,72.8812206761461));
#109129=CARTESIAN_POINT('Ctrl Pts',(-11.8825189875651,66.6020700932764,
72.7735197025896));
#109130=CARTESIAN_POINT('Ctrl Pts',(-11.900761960782,66.626655646913,72.1347020616983));
#109131=CARTESIAN_POINT('Ctrl Pts',(-11.9153598856798,66.6974656030097,
71.6066954305637));
#109132=CARTESIAN_POINT('Ctrl Pts',(-11.9379572243418,66.8792771008636,
70.8237123401298));
#109133=CARTESIAN_POINT('Ctrl Pts',(-11.9456748218442,66.9537189666686,
70.5616499255183));
#109134=CARTESIAN_POINT('Ctrl Pts',(-11.9694331575962,67.2189017455611,
69.7756235539929));
#109135=CARTESIAN_POINT('Ctrl Pts',(-11.9857513677395,67.4491534718115,
69.2666213176648));
#109136=CARTESIAN_POINT('Ctrl Pts',(-12.0167052040164,67.9950043751541,
68.3225914726985));
#109137=CARTESIAN_POINT('Ctrl Pts',(-12.0313527545475,68.305247981938,67.8874572684421));
#109138=CARTESIAN_POINT('Ctrl Pts',(-12.07658598756,69.3568392141455,66.6751650879817));
#109139=CARTESIAN_POINT('Ctrl Pts',(-12.107875343283,70.207495708555,66.0074653700156));
#109140=CARTESIAN_POINT('Ctrl Pts',(-12.1684779816568,72.138815149854,65.0149854075845));
#109141=CARTESIAN_POINT('Ctrl Pts',(-12.2005292908041,73.2062524150642,
64.7092791039551));
#109142=CARTESIAN_POINT('Ctrl Pts',(-12.2520666938747,75.0277649752649,
64.5574415914327));
#109143=CARTESIAN_POINT('Ctrl Pts',(-12.2720637571735,75.7581081018806,
64.5915460803062));
#109144=CARTESIAN_POINT('Ctrl Pts',(-12.3082103090711,76.9989263241938,
64.8128478597517));
#109145=CARTESIAN_POINT('Ctrl Pts',(-12.323785515563,77.5128997370045,64.95591407137));
#109146=CARTESIAN_POINT('Ctrl Pts',(-12.3544290082357,78.5202646589675,
65.3425428320663));
#109147=CARTESIAN_POINT('Ctrl Pts',(-12.3694367591572,79.0103247715392,
65.5877955532602));
#109148=CARTESIAN_POINT('Ctrl Pts',(-12.3925318410277,79.7034362081076,
66.0238511648671));
#109149=CARTESIAN_POINT('Ctrl Pts',(-12.4002783916204,79.9266152453759,
66.1798858198389));
#109150=CARTESIAN_POINT('Ctrl Pts',(-12.4233639007157,80.5619990642387,
66.6717299659978));
#109151=CARTESIAN_POINT('Ctrl Pts',(-12.4389080979838,80.9503678544398,
67.0361195597719));
#109152=CARTESIAN_POINT('Ctrl Pts',(-12.4699035192427,81.6746959344526,
67.8579397968622));
#109153=CARTESIAN_POINT('Ctrl Pts',(-12.4853975164757,82.0041091067518,
68.317628453921));
#109154=CARTESIAN_POINT('Ctrl Pts',(-12.5164577767264,82.5506589458763,
69.2697002216737));
#109155=CARTESIAN_POINT('Ctrl Pts',(-12.5318997793577,82.771643506454,69.7568065604022));
#109156=CARTESIAN_POINT('Ctrl Pts',(-12.5790126465749,83.3011886052007,
71.2994128987627));
#109157=CARTESIAN_POINT('Ctrl Pts',(-12.6085889564851,83.4506698019872,
72.3970740519697));
#109158=CARTESIAN_POINT('Ctrl Pts',(-12.6555902003529,83.3530105295161,
74.0233805265858));
#109159=CARTESIAN_POINT('Ctrl Pts',(-12.671054833758,83.2707593068306,74.5501463571698));
#109160=CARTESIAN_POINT('Ctrl Pts',(-12.7001594794235,83.0144392652775,
75.5547432858472));
#109161=CARTESIAN_POINT('Ctrl Pts',(-12.7141074504808,82.8457938294387,
76.0316455773091));
#109162=CARTESIAN_POINT('Ctrl Pts',(-12.7432694102026,82.4168316491393,
76.9670048874546));
#109163=CARTESIAN_POINT('Ctrl Pts',(-12.7584573263868,82.1541870779306,
77.421990656059));
#109164=CARTESIAN_POINT('Ctrl Pts',(-12.8051857015011,81.2176184601508,
78.7420486803291));
#109165=CARTESIAN_POINT('Ctrl Pts',(-12.8346827098319,80.4160229325183,
79.5022844929333));
#109166=CARTESIAN_POINT('Ctrl Pts',(-12.8830862236364,78.998746325473,80.3989939153691));
#109167=CARTESIAN_POINT('Ctrl Pts',(-12.8999445714155,78.4751645492438,
80.6584971787898));
#109168=CARTESIAN_POINT('Ctrl Pts',(-12.9331626931529,77.3621037193998,
81.0725918226183));
#109169=CARTESIAN_POINT('Ctrl Pts',(-12.9499554666097,76.7741495751895,
81.2216391404873));
#109170=CARTESIAN_POINT('Ctrl Pts',(-12.9672880448682,76.175305272257,81.3062602161754));
#109171=CARTESIAN_POINT('',(-12.9679003706342,82.2015397612608,68.6647904662762));
#109172=CARTESIAN_POINT('Origin',(-12.9678999777142,75.,72.98888938658));
#109173=CARTESIAN_POINT('Ctrl Pts',(-12.9685679372243,82.2015206898752,
68.6647594448114));
#109174=CARTESIAN_POINT('Ctrl Pts',(-12.9512109568237,81.8931531007796,
68.1511958833865));
#109175=CARTESIAN_POINT('Ctrl Pts',(-12.9337253072393,81.5307214119955,
67.6720706009241));
#109176=CARTESIAN_POINT('Ctrl Pts',(-12.9004039599864,80.7129408499974,
66.8021108354724));
#109177=CARTESIAN_POINT('Ctrl Pts',(-12.8840699634639,80.2605796608795,
66.4131592514108));
#109178=CARTESIAN_POINT('Ctrl Pts',(-12.8500679374412,79.2785032522322,
65.7354507606752));
#109179=CARTESIAN_POINT('Ctrl Pts',(-12.8324865342193,78.7511883261723,
65.4492260302083));
#109180=CARTESIAN_POINT('Ctrl Pts',(-12.7926048066351,77.4689065878324,
64.9212923585615));
#109181=CARTESIAN_POINT('Ctrl Pts',(-12.7714181795333,76.7012242270995,
64.7252666633013));
#109182=CARTESIAN_POINT('Ctrl Pts',(-12.7339958847424,75.3905477198483,
64.58124318139));
#109183=CARTESIAN_POINT('Ctrl Pts',(-12.7185507516877,74.8592910802119,
64.5733546507774));
#109184=CARTESIAN_POINT('Ctrl Pts',(-12.6876698145568,73.798389978797,64.6581350928868));
#109185=CARTESIAN_POINT('Ctrl Pts',(-12.6727423882883,73.2711981139356,
64.7513784901045));
#109186=CARTESIAN_POINT('Ctrl Pts',(-12.6274069825214,71.6977037102964,
65.1874891058586));
#109187=CARTESIAN_POINT('Ctrl Pts',(-12.5953164764482,70.7068140489425,
65.6857855976466));
#109188=CARTESIAN_POINT('Ctrl Pts',(-12.552215583075,69.510898997823,66.6167862897298));
#109189=CARTESIAN_POINT('Ctrl Pts',(-12.5407531485254,69.2013466168084,
66.8971280564601));
#109190=CARTESIAN_POINT('Ctrl Pts',(-12.4984264527959,68.1527467713009,
67.999432534347));
#109191=CARTESIAN_POINT('Ctrl Pts',(-12.4657516690204,67.5568226075881,
68.9418400910791));
#109192=CARTESIAN_POINT('Ctrl Pts',(-12.4205238030014,66.9788430599908,
70.4440307130539));
#109193=CARTESIAN_POINT('Ctrl Pts',(-12.4066962527423,66.8403263929509,
70.9309779345929));
#109194=CARTESIAN_POINT('Ctrl Pts',(-12.3777612751823,66.6490141176107,
71.9422119441106));
#109195=CARTESIAN_POINT('Ctrl Pts',(-12.3626760155638,66.6,72.4649816273617));
#109196=CARTESIAN_POINT('Ctrl Pts',(-12.3474400892301,66.6,72.9888893865802));
#109197=CARTESIAN_POINT('Origin',(-15.9175364833309,75.,72.98888938658));
#109198=CARTESIAN_POINT('',(-10.8470411184477,66.6,72.98888938658));
#109199=CARTESIAN_POINT('Ctrl Pts',(-12.3474397125099,66.60000000001,72.9889023406097));
#109200=CARTESIAN_POINT('Ctrl Pts',(-12.3383509580487,66.6000004819755,
73.3014313418396));
#109201=CARTESIAN_POINT('Ctrl Pts',(-12.3292493655496,66.6174420671942,
73.6137087450362));
#109202=CARTESIAN_POINT('Ctrl Pts',(-12.3116088837576,66.6864578250661,
74.2296180169422));
#109203=CARTESIAN_POINT('Ctrl Pts',(-12.3030894322364,66.7373957872832,
74.5328343294614));
#109204=CARTESIAN_POINT('Ctrl Pts',(-12.2774181628908,66.9403542840846,
75.4349814090962));
#109205=CARTESIAN_POINT('Ctrl Pts',(-12.2601792027666,67.1418836663396,
76.0205964076443));
#109206=CARTESIAN_POINT('Ctrl Pts',(-12.2285210830866,67.6106647331949,
77.0122701558534));
#109207=CARTESIAN_POINT('Ctrl Pts',(-12.2144350846763,67.8522989305133,
77.4273838901755));
#109208=CARTESIAN_POINT('Ctrl Pts',(-12.1771390318329,68.6025865050576,
78.4947112709424));
#109209=CARTESIAN_POINT('Ctrl Pts',(-12.1549803016089,69.1740505608182,
79.0962064068379));
#109210=CARTESIAN_POINT('Ctrl Pts',(-12.1154884969256,70.2621959758581,
79.9475357845932));
#109211=CARTESIAN_POINT('Ctrl Pts',(-12.0991485817419,70.7333585456637,
80.2459755813694));
#109212=CARTESIAN_POINT('Ctrl Pts',(-12.0513754127791,72.2171434724447,
80.9910458322196));
#109213=CARTESIAN_POINT('Ctrl Pts',(-12.0219258723555,73.2917784530345,
81.2871298976208));
#109214=CARTESIAN_POINT('Ctrl Pts',(-11.9777841360304,74.8094404338569,
81.3971062763845));
#109215=CARTESIAN_POINT('Ctrl Pts',(-11.9655484061879,75.2276607939307,
81.3961835994181));
#109216=CARTESIAN_POINT('Ctrl Pts',(-11.9389370364639,76.1605855364148,
81.3244399458181));
#109217=CARTESIAN_POINT('Ctrl Pts',(-11.924798111761,76.6723223983046,81.2370235285619));
#109218=CARTESIAN_POINT('Ctrl Pts',(-11.8883656217225,77.9306403582969,
80.9000800766076));
#109219=CARTESIAN_POINT('Ctrl Pts',(-11.865523905305,78.6563677532716,80.5919473838761));
#109220=CARTESIAN_POINT('Ctrl Pts',(-11.8198903226285,80.0097942736113,
79.7781119315346));
#109221=CARTESIAN_POINT('Ctrl Pts',(-11.7984831150536,80.629293919866,79.2740008508438));
#109222=CARTESIAN_POINT('Ctrl Pts',(-11.7571269120672,81.6219728872003,
78.1999760414976));
#109223=CARTESIAN_POINT('Ctrl Pts',(-11.7375490091182,82.0151282350308,
77.6572813161279));
#109224=CARTESIAN_POINT('Ctrl Pts',(-11.6955578934579,82.7236236098708,
76.3842391094113));
#109225=CARTESIAN_POINT('Ctrl Pts',(-11.6743352616283,83.0082997423443,
75.6440530719495));
#109226=CARTESIAN_POINT('Ctrl Pts',(-11.6335629805257,83.331436047082,74.2417196239464));
#109227=CARTESIAN_POINT('Ctrl Pts',(-11.6144948961672,83.4033738342296,
73.5936053899774));
#109228=CARTESIAN_POINT('Ctrl Pts',(-11.56715692772,83.3945360094672,71.9503684339933));
#109229=CARTESIAN_POINT('Ctrl Pts',(-11.5406728190485,83.2130361389485,
70.9658202476124));
#109230=CARTESIAN_POINT('Ctrl Pts',(-11.4939427868069,82.6428557649125,
69.4474468619433));
#109231=CARTESIAN_POINT('Ctrl Pts',(-11.4753999707528,82.3565430009873,
68.8856748376966));
#109232=CARTESIAN_POINT('Ctrl Pts',(-11.4445545009936,81.7515669255104,
67.96924674705));
#109233=CARTESIAN_POINT('Ctrl Pts',(-11.4316851221503,81.4604832241331,
67.5997677967607));
#109234=CARTESIAN_POINT('Ctrl Pts',(-11.3874716606328,80.3846960034667,
66.447465324252));
#109235=CARTESIAN_POINT('Ctrl Pts',(-11.3546465824438,79.4768262218802,
65.7956130795486));
#109236=CARTESIAN_POINT('Ctrl Pts',(-11.3085845959489,77.9678758003413,
65.1114450860482));
#109237=CARTESIAN_POINT('Ctrl Pts',(-11.293383090747,77.4459446868923,64.9340917042076));
#109238=CARTESIAN_POINT('Ctrl Pts',(-11.2618693998766,76.3714034649417,
64.6831288206911));
#109239=CARTESIAN_POINT('Ctrl Pts',(-11.2456263390625,75.8212568036285,
64.6108272221902));
#109240=CARTESIAN_POINT('Ctrl Pts',(-11.2069496675176,74.479608726194,64.5679980523296));
#109241=CARTESIAN_POINT('Ctrl Pts',(-11.1857392457571,73.6915951787152,
64.6540052900576));
#109242=CARTESIAN_POINT('Ctrl Pts',(-11.1482998568107,72.411316536888,64.9800136749814));
#109243=CARTESIAN_POINT('Ctrl Pts',(-11.1328125992985,71.9091107365945,
65.1601119126757));
#109244=CARTESIAN_POINT('Ctrl Pts',(-11.0849228184656,70.4163518701671,
65.8616173735125));
#109245=CARTESIAN_POINT('Ctrl Pts',(-11.0551958568246,69.5102241308512,
66.5336426772762));
#109246=CARTESIAN_POINT('Ctrl Pts',(-11.0088266082509,68.4329835720872,
67.728112221449));
#109247=CARTESIAN_POINT('Ctrl Pts',(-10.9943850016843,68.1365353688722,
68.1212073427534));
#109248=CARTESIAN_POINT('Ctrl Pts',(-10.9552963721232,67.4125776501631,
69.2799215107));
#109249=CARTESIAN_POINT('Ctrl Pts',(-10.9318432305127,67.0677511953457,
70.0897711514179));
#109250=CARTESIAN_POINT('Ctrl Pts',(-10.8868982190948,66.6852367557343,
71.6092142509929));
#109251=CARTESIAN_POINT('Ctrl Pts',(-10.8664411741287,66.6,72.2980067817921));
#109252=CARTESIAN_POINT('Ctrl Pts',(-10.8470411184477,66.6,72.98888938658));
#109253=CARTESIAN_POINT('',(-10.3758119169399,66.6000000000181,72.9888719572421));
#109254=CARTESIAN_POINT('',(-15.9175364833309,66.6,72.98888938658));
#109255=CARTESIAN_POINT('',(-10.4866907823956,67.6032721057859,69.0114531423211));
#109256=CARTESIAN_POINT('Ctrl Pts',(-10.3758119169399,66.6000000000181,
72.9888719572421));
#109257=CARTESIAN_POINT('Ctrl Pts',(-10.3859052171345,66.600000718797,72.6424593122746));
#109258=CARTESIAN_POINT('Ctrl Pts',(-10.3960457745143,66.6214302853707,
72.2963769232993));
#109259=CARTESIAN_POINT('Ctrl Pts',(-10.4157751272758,66.7066657642043,
71.6107443794253));
#109260=CARTESIAN_POINT('Ctrl Pts',(-10.4253085028644,66.7701553475043,
71.2718173942441));
#109261=CARTESIAN_POINT('Ctrl Pts',(-10.4540473375612,67.0231409069194,
70.2671330393793));
#109262=CARTESIAN_POINT('Ctrl Pts',(-10.4734283552966,67.2741698468866,
69.6199504765713));
#109263=CARTESIAN_POINT('Ctrl Pts',(-10.4934825642517,67.6016542759913,
69.0108898204612));
#109264=CARTESIAN_POINT('',(-11.1260798196334,83.4,72.98888938658));
#109265=CARTESIAN_POINT('Ctrl Pts',(-10.4857108324479,67.6017520181465,
69.0107080434282));
#109266=CARTESIAN_POINT('Ctrl Pts',(-10.4924440164462,67.7339470320748,
68.7648641739199));
#109267=CARTESIAN_POINT('Ctrl Pts',(-10.499325309094,67.8783113993465,68.5257670142111));
#109268=CARTESIAN_POINT('Ctrl Pts',(-10.5135966694059,68.1881179038954,
68.0660849034585));
#109269=CARTESIAN_POINT('Ctrl Pts',(-10.5209698190774,68.3530447724227,
67.8455715258234));
#109270=CARTESIAN_POINT('Ctrl Pts',(-10.5358034440303,68.6897328404269,
67.4387099411056));
#109271=CARTESIAN_POINT('Ctrl Pts',(-10.5431999929194,68.8596837833846,
67.2512529638297));
#109272=CARTESIAN_POINT('Ctrl Pts',(-10.5724885452809,69.5391969302741,
66.5665678032324));
#109273=CARTESIAN_POINT('Ctrl Pts',(-10.5964606357472,70.1027165875061,
66.1271814359369));
#109274=CARTESIAN_POINT('Ctrl Pts',(-10.6326053288691,71.0408445180282,
65.5707490580701));
#109275=CARTESIAN_POINT('Ctrl Pts',(-10.6449129433804,71.3796577283306,
65.3996270238521));
#109276=CARTESIAN_POINT('Ctrl Pts',(-10.6807263893499,72.4715428263888,
64.9379895553254));
#109277=CARTESIAN_POINT('Ctrl Pts',(-10.7023444507398,73.2555833569729,
64.7325398660417));
#109278=CARTESIAN_POINT('Ctrl Pts',(-10.7375866509904,74.5047875528942,
64.5913936931575));
#109279=CARTESIAN_POINT('Ctrl Pts',(-10.750356719919,74.9560252480495,64.5769197805323));
#109280=CARTESIAN_POINT('Ctrl Pts',(-10.7784516536322,75.9596370940102,
64.6255129461359));
#109281=CARTESIAN_POINT('Ctrl Pts',(-10.793645490965,76.5090279203329,64.7069929965395));
#109282=CARTESIAN_POINT('Ctrl Pts',(-10.824938254612,77.5819324145609,64.9764908537815));
#109283=CARTESIAN_POINT('Ctrl Pts',(-10.8409642773336,78.1029043627951,
65.1634903643253));
#109284=CARTESIAN_POINT('Ctrl Pts',(-10.8889317335777,79.5973141318404,
65.8727697249272));
#109285=CARTESIAN_POINT('Ctrl Pts',(-10.9185809685849,80.490233907639,66.5366185927917));
#109286=CARTESIAN_POINT('Ctrl Pts',(-10.9648095287159,81.5661897535722,
67.7260919052978));
#109287=CARTESIAN_POINT('Ctrl Pts',(-10.9794537614335,81.8688404238527,
68.1277234058784));
#109288=CARTESIAN_POINT('Ctrl Pts',(-11.0141928601179,82.5190872820912,
69.1736833146776));
#109289=CARTESIAN_POINT('Ctrl Pts',(-11.0342434566204,82.8219593005975,
69.8409625684042));
#109290=CARTESIAN_POINT('Ctrl Pts',(-11.0670101304895,83.1551947333564,
70.9338395463009));
#109291=CARTESIAN_POINT('Ctrl Pts',(-11.0790157657935,83.2463255339559,
71.3370593530283));
#109292=CARTESIAN_POINT('Ctrl Pts',(-11.1028514344624,83.3690627793617,
72.1569958322429));
#109293=CARTESIAN_POINT('Ctrl Pts',(-11.114463408048,83.4,72.5726453795531));
#109294=CARTESIAN_POINT('Ctrl Pts',(-11.1260798196334,83.4,72.98888938658));
#109295=CARTESIAN_POINT('Ctrl Pts',(-11.1260798196334,83.4,72.9888893865797));
#109296=CARTESIAN_POINT('Ctrl Pts',(-11.1554998323271,83.4,74.0430793040412));
#109297=CARTESIAN_POINT('Ctrl Pts',(-11.1862019338463,83.2015541254395,
75.087874801693));
#109298=CARTESIAN_POINT('Ctrl Pts',(-11.2258266429589,82.6880724176838,
76.390877188071));
#109299=CARTESIAN_POINT('Ctrl Pts',(-11.2354316893231,82.5412658088397,
76.7049749887674));
#109300=CARTESIAN_POINT('Ctrl Pts',(-11.2755123268849,81.8551462172399,
77.9637275658652));
#109301=CARTESIAN_POINT('Ctrl Pts',(-11.3074061933692,81.1543949381981,
78.8082936456724));
#109302=CARTESIAN_POINT('Ctrl Pts',(-11.3523708202787,79.9111548984504,
79.8232571031621));
#109303=CARTESIAN_POINT('Ctrl Pts',(-11.3667007821648,79.4807084235242,
80.1128824671349));
#109304=CARTESIAN_POINT('Ctrl Pts',(-11.3964561316438,78.5619975928432,
80.614642384779));
#109305=CARTESIAN_POINT('Ctrl Pts',(-11.4118382800914,78.0747278790574,
80.8238092853373));
#109306=CARTESIAN_POINT('Ctrl Pts',(-11.4423982312788,77.0643921043933,
81.1486390847459));
#109307=CARTESIAN_POINT('Ctrl Pts',(-11.4571319688664,76.5434166536166,
81.2630113542134));
#109308=CARTESIAN_POINT('Ctrl Pts',(-11.5026741622249,74.9276128008205,
81.4597198802285));
#109309=CARTESIAN_POINT('Ctrl Pts',(-11.5348230919039,73.8246440317065,
81.37809373512));
#109310=CARTESIAN_POINT('Ctrl Pts',(-11.5802118851425,72.2603915529493,
80.9470480447898));
#109311=CARTESIAN_POINT('Ctrl Pts',(-11.5948326656458,71.7666205744012,
80.7595392724667));
#109312=CARTESIAN_POINT('Ctrl Pts',(-11.6240674195689,70.8462231857547,
80.3070011735023));
#109313=CARTESIAN_POINT('Ctrl Pts',(-11.6385739156917,70.4192425309839,
80.047591272425));
#109314=CARTESIAN_POINT('Ctrl Pts',(-11.6682293590274,69.5895796955461,
79.4363888042523));
#109315=CARTESIAN_POINT('Ctrl Pts',(-11.6829378663155,69.1922932146571,
79.0809692818794));
#109316=CARTESIAN_POINT('Ctrl Pts',(-11.7285458471771,68.0862449392967,
77.8842805068686));
#109317=CARTESIAN_POINT('Ctrl Pts',(-11.7607556287622,67.5063910632311,
76.9399260467962));
#109318=CARTESIAN_POINT('Ctrl Pts',(-11.8064350524018,66.9381212087432,
75.4082731100625));
#109319=CARTESIAN_POINT('Ctrl Pts',(-11.8213191649983,66.8002007400394,
74.8890464485664));
#109320=CARTESIAN_POINT('Ctrl Pts',(-11.8497371850303,66.6376609935873,
73.9067834969859));
#109321=CARTESIAN_POINT('Ctrl Pts',(-11.8630898072636,66.6,73.4481292277721));
#109322=CARTESIAN_POINT('Ctrl Pts',(-11.8763230992193,66.6,72.98888938658));
#109323=CARTESIAN_POINT('Origin',(-15.9175364833309,75.,72.98888938658));
#109324=CARTESIAN_POINT('',(-8.87591635085981,66.6,72.98888938658));
#109325=CARTESIAN_POINT('',(-9.34771011126149,66.6,72.98888938658));
#109326=CARTESIAN_POINT('',(-15.9175364833309,66.6,72.98888938658));
#109327=CARTESIAN_POINT('Ctrl Pts',(-8.87591635085981,66.6,72.98888938658));
#109328=CARTESIAN_POINT('Ctrl Pts',(-8.88449608043677,66.6,72.6943442545088));
#109329=CARTESIAN_POINT('Ctrl Pts',(-8.89310105129781,66.6154919764157,
72.3996085824049));
#109330=CARTESIAN_POINT('Ctrl Pts',(-8.91696499178457,66.7032110037113,
71.5697455179493));
#109331=CARTESIAN_POINT('Ctrl Pts',(-8.93163466681888,66.8113717174765,
71.0402876251429));
#109332=CARTESIAN_POINT('Ctrl Pts',(-8.97231498264731,67.2393816268824,
69.6453701576608));
#109333=CARTESIAN_POINT('Ctrl Pts',(-8.99937164587288,67.6518739977052,
68.8162145713841));
#109334=CARTESIAN_POINT('Ctrl Pts',(-9.04117877128941,68.5061653281516,
67.6334439600081));
#109335=CARTESIAN_POINT('Ctrl Pts',(-9.05586138994771,68.8631892543803,
67.2277922757505));
#109336=CARTESIAN_POINT('Ctrl Pts',(-9.09678992714188,69.9352207416046,
66.2233315275476));
#109337=CARTESIAN_POINT('Ctrl Pts',(-9.12411309596022,70.7146673702538,
65.7046231506142));
#109338=CARTESIAN_POINT('Ctrl Pts',(-9.16621738663198,72.0550820069518,
65.1035771293466));
#109339=CARTESIAN_POINT('Ctrl Pts',(-9.18090250737464,72.5671309922688,
64.9308598009226));
#109340=CARTESIAN_POINT('Ctrl Pts',(-9.22593400499185,74.141454380223,64.5637061751752));
#109341=CARTESIAN_POINT('Ctrl Pts',(-9.25802141137251,75.2280193048841,
64.5231482682749));
#109342=CARTESIAN_POINT('Ctrl Pts',(-9.3034231618538,76.8271756355542,64.7721894632313));
#109343=CARTESIAN_POINT('Ctrl Pts',(-9.31817680449446,77.3524838278333,
64.9068996005011));
#109344=CARTESIAN_POINT('Ctrl Pts',(-9.34874701182155,78.3732696137243,
65.2767106127798));
#109345=CARTESIAN_POINT('Ctrl Pts',(-9.36450654423863,78.866090679307,65.5115924641901));
#109346=CARTESIAN_POINT('Ctrl Pts',(-9.41173371854036,80.2547458158857,
66.3476528170148));
#109347=CARTESIAN_POINT('Ctrl Pts',(-9.44055676979217,81.0615816358009,
67.0748687131144));
#109348=CARTESIAN_POINT('Ctrl Pts',(-9.48673413389458,82.0354732697045,
68.3676186459088));
#109349=CARTESIAN_POINT('Ctrl Pts',(-9.50264227275593,82.3190421147218,
68.8312901615648));
#109350=CARTESIAN_POINT('Ctrl Pts',(-9.54990550765018,83.0321398232053,
70.2994991511134));
#109351=CARTESIAN_POINT('Ctrl Pts',(-9.57874851143997,83.3129795650303,
71.3633240025041));
#109352=CARTESIAN_POINT('Ctrl Pts',(-9.62583420939872,83.4172951747497,
72.9892902885587));
#109353=CARTESIAN_POINT('Ctrl Pts',(-9.64176296726587,83.3999121453814,
73.5295696880987));
#109354=CARTESIAN_POINT('Ctrl Pts',(-9.68868706052882,83.1881877996304,
75.1695097513576));
#109355=CARTESIAN_POINT('Ctrl Pts',(-9.71876568409483,82.8270554848739,
76.2352539354287));
#109356=CARTESIAN_POINT('Ctrl Pts',(-9.76701768319113,81.9967495730251,
77.6685695133176));
#109357=CARTESIAN_POINT('Ctrl Pts',(-9.7826694323724,81.6802126532702,78.1102864171987));
#109358=CARTESIAN_POINT('Ctrl Pts',(-9.81278076262282,80.9672925865527,
78.9255488299831));
#109359=CARTESIAN_POINT('Ctrl Pts',(-9.82763853111115,80.5727859169826,
79.297341095552));
#109360=CARTESIAN_POINT('Ctrl Pts',(-9.85844211034537,79.7158078402704,
79.9614333002833));
#109361=CARTESIAN_POINT('Ctrl Pts',(-9.87432389642801,79.2550575699069,
80.2517866465711));
#109362=CARTESIAN_POINT('Ctrl Pts',(-9.92193760820865,77.7901137913412,
80.9874131258493));
#109363=CARTESIAN_POINT('Ctrl Pts',(-9.95095877328019,76.723882182416,81.2828240847856));
#109364=CARTESIAN_POINT('Ctrl Pts',(-9.99809891811017,75.0926985586027,
81.4057084587841));
#109365=CARTESIAN_POINT('Ctrl Pts',(-10.0140330284361,74.5517268190234,
81.3942732064712));
#109366=CARTESIAN_POINT('Ctrl Pts',(-10.0612792385604,72.9088747898517,
81.2004123098757));
#109367=CARTESIAN_POINT('Ctrl Pts',(-10.0911063217156,71.8391043920893,
80.8508712653943));
#109368=CARTESIAN_POINT('Ctrl Pts',(-10.1314663963532,70.6317532579358,
80.1688967431122));
#109369=CARTESIAN_POINT('Ctrl Pts',(-10.1394214898618,70.401407398868,80.023591355259));
#109370=CARTESIAN_POINT('Ctrl Pts',(-10.1785641430454,69.2914325261035,
79.2455523637897));
#109371=CARTESIAN_POINT('Ctrl Pts',(-10.2072704941516,68.5329638524829,
78.4579868704499));
#109372=CARTESIAN_POINT('Ctrl Pts',(-10.2501942049362,67.7280848548892,
77.2125051977263));
#109373=CARTESIAN_POINT('Ctrl Pts',(-10.2619173627264,67.5354218102325,
76.8618405428289));
#109374=CARTESIAN_POINT('Ctrl Pts',(-10.2908350061065,67.1162919785189,
75.9505322913265));
#109375=CARTESIAN_POINT('Ctrl Pts',(-10.3072480931363,66.9239555181329,
75.3767085877148));
#109376=CARTESIAN_POINT('Ctrl Pts',(-10.3409113672873,66.6652958693488,
74.1965300373668));
#109377=CARTESIAN_POINT('Ctrl Pts',(-10.3581925699977,66.6,73.5935864999432));
#109378=CARTESIAN_POINT('Ctrl Pts',(-10.3758114091077,66.6,72.9888893865795));
#109379=CARTESIAN_POINT('',(-9.46554775786244,67.6016909082801,69.0108216919104));
#109380=CARTESIAN_POINT('Ctrl Pts',(-10.8470411184477,66.6,72.98888938658));
#109381=CARTESIAN_POINT('Ctrl Pts',(-10.8429974544575,66.6,73.1328939789574));
#109382=CARTESIAN_POINT('Ctrl Pts',(-10.8389830318835,66.6037030877524,
73.2769889125608));
#109383=CARTESIAN_POINT('Ctrl Pts',(-10.8200995945198,66.6386538757395,
73.9554652693975));
#109384=CARTESIAN_POINT('Ctrl Pts',(-10.8052994167985,66.7171918370302,
74.4860408086064));
#109385=CARTESIAN_POINT('Ctrl Pts',(-10.7673672606253,67.0362804855674,
75.776284033232));
#109386=CARTESIAN_POINT('Ctrl Pts',(-10.7438334944375,67.335214583143,76.5161413930023));
#109387=CARTESIAN_POINT('Ctrl Pts',(-10.7000502611941,68.1205210414441,
77.8702571798004));
#109388=CARTESIAN_POINT('Ctrl Pts',(-10.678911890322,68.5975578161451,78.4810410280505));
#109389=CARTESIAN_POINT('Ctrl Pts',(-10.6423478202938,69.5079009543939,
79.3641382481171));
#109390=CARTESIAN_POINT('Ctrl Pts',(-10.6277391305027,69.8945857817826,
79.6778122874029));
#109391=CARTESIAN_POINT('Ctrl Pts',(-10.5997334830968,70.7071291608878,
80.2252111110413));
#109392=CARTESIAN_POINT('Ctrl Pts',(-10.5865090312781,71.1300498424614,
80.4599389249407));
#109393=CARTESIAN_POINT('Ctrl Pts',(-10.5424090237105,72.5750704014388,
81.1061557090216));
#109394=CARTESIAN_POINT('Ctrl Pts',(-10.5097800041221,73.6578460320961,
81.3536303441462));
#109395=CARTESIAN_POINT('Ctrl Pts',(-10.4594583183132,75.453211984091,81.4054804054051));
#109396=CARTESIAN_POINT('Ctrl Pts',(-10.4404402495851,76.148717327638,81.339031228331));
#109397=CARTESIAN_POINT('Ctrl Pts',(-10.3972128535349,77.6224670548347,
81.0104327503222));
#109398=CARTESIAN_POINT('Ctrl Pts',(-10.3731988605783,78.3869641936456,
80.7187680563788));
#109399=CARTESIAN_POINT('Ctrl Pts',(-10.3358043235385,79.5589275625022,
80.0638838608808));
#109400=CARTESIAN_POINT('Ctrl Pts',(-10.3212492026392,79.9949626824068,
79.7630841569993));
#109401=CARTESIAN_POINT('Ctrl Pts',(-10.2838028980019,81.0045835734316,
78.9157996540609));
#109402=CARTESIAN_POINT('Ctrl Pts',(-10.2603558941316,81.534768850004,78.3255639741675));
#109403=CARTESIAN_POINT('Ctrl Pts',(-10.2228371947749,82.2777896155877,
77.2184883213856));
#109404=CARTESIAN_POINT('Ctrl Pts',(-10.207982765868,82.5362805922708,76.738584788694));
#109405=CARTESIAN_POINT('Ctrl Pts',(-10.1685899659626,83.0769591001059,
75.449122455846));
#109406=CARTESIAN_POINT('Ctrl Pts',(-10.1432360276034,83.2851949198924,
74.6153923607755));
#109407=CARTESIAN_POINT('Ctrl Pts',(-10.1054806048686,83.4085236854867,
73.2857075566512));
#109408=CARTESIAN_POINT('Ctrl Pts',(-10.0923185055741,83.4117258184702,
72.8038168581635));
#109409=CARTESIAN_POINT('Ctrl Pts',(-10.0476349101555,83.285332993399,71.2112930426171));
#109410=CARTESIAN_POINT('Ctrl Pts',(-10.0144854685635,82.9759767394019,
70.1270021722388));
#109411=CARTESIAN_POINT('Ctrl Pts',(-9.9686471877387,82.2205249119231,68.6639642151414));
#109412=CARTESIAN_POINT('Ctrl Pts',(-9.95403766156621,81.9333031210872,
68.2170695755514));
#109413=CARTESIAN_POINT('Ctrl Pts',(-9.91654046434544,81.1188692089366,
67.1801816090873));
#109414=CARTESIAN_POINT('Ctrl Pts',(-9.89312700168102,80.5469717865591,
66.6317855236956));
#109415=CARTESIAN_POINT('Ctrl Pts',(-9.85419328296166,79.4225378831116,
65.8224746710984));
#109416=CARTESIAN_POINT('Ctrl Pts',(-9.83790478950418,78.9022466608465,
65.5263947517448));
#109417=CARTESIAN_POINT('Ctrl Pts',(-9.8054291819373,77.8509918913373,65.0684064454306));
#109418=CARTESIAN_POINT('Ctrl Pts',(-9.7894267946388,77.3266785902673,64.898849201525));
#109419=CARTESIAN_POINT('Ctrl Pts',(-9.74144977797055,75.7116660419685,
64.5466924361694));
#109420=CARTESIAN_POINT('Ctrl Pts',(-9.71208081141942,74.5979439719732,
64.5262941293461));
#109421=CARTESIAN_POINT('Ctrl Pts',(-9.66596321343898,73.0231094515633,
64.809720962872));
#109422=CARTESIAN_POINT('Ctrl Pts',(-9.6513603589804,72.5428617473836,64.9409481708741));
#109423=CARTESIAN_POINT('Ctrl Pts',(-9.62320555521004,71.6195450110593,
65.2836536488962));
#109424=CARTESIAN_POINT('Ctrl Pts',(-9.60985108382497,71.1777185616237,
65.4930037924682));
#109425=CARTESIAN_POINT('Ctrl Pts',(-9.58555856277631,70.4248560092225,
65.9336930808021));
#109426=CARTESIAN_POINT('Ctrl Pts',(-9.57474051005098,70.1068634346352,
66.1503993784754));
#109427=CARTESIAN_POINT('Ctrl Pts',(-9.54743719458288,69.3589885197844,
66.7390174365363));
#109428=CARTESIAN_POINT('Ctrl Pts',(-9.53071392835463,68.949851159647,67.134182469978));
#109429=CARTESIAN_POINT('Ctrl Pts',(-9.49779589939924,68.2071166842069,
68.0132323026672));
#109430=CARTESIAN_POINT('Ctrl Pts',(-9.48191110280316,67.8780097698654,
68.4969309030181));
#109431=CARTESIAN_POINT('Ctrl Pts',(-9.46554775786244,67.6016909082801,
69.0108216919104));
#109432=CARTESIAN_POINT('Ctrl Pts',(-9.46562408938853,67.6016900154045,
69.010823352458));
#109433=CARTESIAN_POINT('Ctrl Pts',(-9.44541854529748,67.2454679990037,
69.6733163523391));
#109434=CARTESIAN_POINT('Ctrl Pts',(-9.42553707582171,66.979848802812,70.3806400212566));
#109435=CARTESIAN_POINT('Ctrl Pts',(-9.38575705560963,66.671022391848,71.7292457946473));
#109436=CARTESIAN_POINT('Ctrl Pts',(-9.36658493103693,66.6,72.3582310229932));
#109437=CARTESIAN_POINT('Ctrl Pts',(-9.34771011126149,66.6,72.98888938658));
#109438=CARTESIAN_POINT('Origin',(-15.9175364833309,-75.,72.98888938658));
#109439=CARTESIAN_POINT('',(-9.34771011126148,-66.6,72.98888938658));
#109440=CARTESIAN_POINT('',(-8.87591635085981,-66.6,72.98888938658));
#109441=CARTESIAN_POINT('',(-15.9175364833309,-66.6,72.98888938658));
#109442=CARTESIAN_POINT('',(-8.56753648333097,-72.6784966214785,81.06172173115));
#109443=CARTESIAN_POINT('Ctrl Pts',(-8.87591635085981,-66.6,72.9888893865799));
#109444=CARTESIAN_POINT('Ctrl Pts',(-8.85294957915599,-66.6,73.7773467317762));
#109445=CARTESIAN_POINT('Ctrl Pts',(-8.83059301219102,-66.7110222695729,
74.5635770776098));
#109446=CARTESIAN_POINT('Ctrl Pts',(-8.79362233623142,-67.0818223436479,
75.8448230515217));
#109447=CARTESIAN_POINT('Ctrl Pts',(-8.77850802983328,-67.2825837564249,
76.3497484918026));
#109448=CARTESIAN_POINT('Ctrl Pts',(-8.7470324735349,-67.7779596867464,
77.312601823614));
#109449=CARTESIAN_POINT('Ctrl Pts',(-8.73122077996138,-68.0711761988425,
77.7684057885426));
#109450=CARTESIAN_POINT('Ctrl Pts',(-8.69128771667201,-68.9417992746947,
78.8715534955591));
#109451=CARTESIAN_POINT('Ctrl Pts',(-8.66821704523819,-69.579004898322,
79.4634820331365));
#109452=CARTESIAN_POINT('Ctrl Pts',(-8.61776368352287,-71.0262048035655,
80.4419034519592));
#109453=CARTESIAN_POINT('Ctrl Pts',(-8.59210212382877,-71.8304934245268,
80.8178615588208));
#109454=CARTESIAN_POINT('Ctrl Pts',(-8.56753648333109,-72.6784966214791,
81.0617217311488));
#109455=CARTESIAN_POINT('',(-8.56920282870944,-83.3330658671999,71.9536543098738));
#109456=CARTESIAN_POINT('Origin',(-8.56753648333091,-75.,72.98888938658));
#109457=CARTESIAN_POINT('',(-8.59969205422499,-83.3999999999891,72.9889028996933));
#109458=CARTESIAN_POINT('Ctrl Pts',(-8.59969205422499,-83.3999999999891,
72.9889028996933));
#109459=CARTESIAN_POINT('Ctrl Pts',(-8.59443361344606,-83.4000003125319,
72.7946205818928));
#109460=CARTESIAN_POINT('Ctrl Pts',(-8.58911455314039,-83.3932603589226,
72.6003991553237));
#109461=CARTESIAN_POINT('Ctrl Pts',(-8.57948092673193,-83.3692714773426,
72.2551795052892));
#109462=CARTESIAN_POINT('Ctrl Pts',(-8.57520339899112,-83.3546488080667,
72.1040856703524));
#109463=CARTESIAN_POINT('Ctrl Pts',(-8.57086917408796,-83.3359409660147,
71.9534724603524));
#109464=CARTESIAN_POINT('Ctrl Pts',(-8.599692054225,-83.3999999999891,72.9889028996933));
#109465=CARTESIAN_POINT('Ctrl Pts',(-8.6245653979019,-83.3999985216074,
73.9078922092929));
#109466=CARTESIAN_POINT('Ctrl Pts',(-8.64831456326027,-83.2492082149449,
74.8206009565659));
#109467=CARTESIAN_POINT('Ctrl Pts',(-8.70336173029356,-82.6585704764233,
76.5592681833137));
#109468=CARTESIAN_POINT('Ctrl Pts',(-8.73114014016359,-82.2232308308517,
77.3736939600486));
#109469=CARTESIAN_POINT('Ctrl Pts',(-8.78168057817269,-81.105995936845,
78.8301160315007));
#109470=CARTESIAN_POINT('Ctrl Pts',(-8.80454434265513,-80.431498229985,
79.4620648581349));
#109471=CARTESIAN_POINT('Ctrl Pts',(-8.86363004660202,-78.758610123619,
80.5803073614369));
#109472=CARTESIAN_POINT('Ctrl Pts',(-8.89744283053813,-77.7390120598963,
81.0048193525973));
#109473=CARTESIAN_POINT('Ctrl Pts',(-8.94677625803638,-75.9714687934765,
81.362608468677));
#109474=CARTESIAN_POINT('Ctrl Pts',(-8.96482541908273,-75.2614168589107,
81.4147123771282));
#109475=CARTESIAN_POINT('Ctrl Pts',(-8.99989289624195,-74.0131601630423,
81.3482398684911));
#109476=CARTESIAN_POINT('Ctrl Pts',(-9.01641208642739,-73.4770816484086,
81.2673699331499));
#109477=CARTESIAN_POINT('Ctrl Pts',(-9.04925276003734,-72.4207468549019,
81.0018865159534));
#109478=CARTESIAN_POINT('Ctrl Pts',(-9.06543988179121,-71.903296508067,
80.8164779418256));
#109479=CARTESIAN_POINT('Ctrl Pts',(-9.11063813073376,-70.4483117239719,
80.1281016998877));
#109480=CARTESIAN_POINT('Ctrl Pts',(-9.13661289890309,-69.5837422354327,
79.4966102182232));
#109481=CARTESIAN_POINT('Ctrl Pts',(-9.19621508389475,-68.2075509289092,
78.0223409841654));
#109482=CARTESIAN_POINT('Ctrl Pts',(-9.22587045537373,-67.6794386529001,
77.2176855012128));
#109483=CARTESIAN_POINT('Ctrl Pts',(-9.28192979902723,-66.8764390499947,
75.3728996039502));
#109484=CARTESIAN_POINT('Ctrl Pts',(-9.3078635989614,-66.6413166549408,
74.3336028706724));
#109485=CARTESIAN_POINT('Ctrl Pts',(-9.34195635427578,-66.6016563503745,
73.1815483385072));
#109486=CARTESIAN_POINT('Ctrl Pts',(-9.34482767571643,-66.6,73.0851992907596));
#109487=CARTESIAN_POINT('Ctrl Pts',(-9.34771011126147,-66.6,72.98888938658));
#109488=CARTESIAN_POINT('Origin',(-15.9175364833309,-75.,72.98888938658));
#109489=CARTESIAN_POINT('',(-10.8470411184476,-66.6,72.98888938658));
#109490=CARTESIAN_POINT('',(-10.3758114091077,-66.6,72.9888893865795));
#109491=CARTESIAN_POINT('',(-15.9175364833309,-66.6,72.98888938658));
#109492=CARTESIAN_POINT('Ctrl Pts',(-10.3758114091077,-66.6,72.9888893865795));
#109493=CARTESIAN_POINT('Ctrl Pts',(-10.3582032242367,-66.6,73.5932208352387));
#109494=CARTESIAN_POINT('Ctrl Pts',(-10.3409320423887,-66.6652169238319,
74.1958019008719));
#109495=CARTESIAN_POINT('Ctrl Pts',(-10.3072885316604,-66.9235651935971,
75.3752941690252));
#109496=CARTESIAN_POINT('Ctrl Pts',(-10.2908864868318,-67.1156700307945,
75.9488004864642));
#109497=CARTESIAN_POINT('Ctrl Pts',(-10.261988887019,-67.5343032730094,
76.8596586711068));
#109498=CARTESIAN_POINT('Ctrl Pts',(-10.2502728742011,-67.7267405915717,
77.2101667049502));
#109499=CARTESIAN_POINT('Ctrl Pts',(-10.2073631419159,-68.5308733934261,
78.4554491819985));
#109500=CARTESIAN_POINT('Ctrl Pts',(-10.178663586788,-69.2887876200924,
79.2430814255604));
#109501=CARTESIAN_POINT('Ctrl Pts',(-10.1395351689805,-70.3981401823001,
80.0214548742716));
#109502=CARTESIAN_POINT('Ctrl Pts',(-10.1315799689027,-70.6284270331717,
80.1668724205897));
#109503=CARTESIAN_POINT('Ctrl Pts',(-10.091218362305,-71.8354636456972,
80.8494052481719));
#109504=CARTESIAN_POINT('Ctrl Pts',(-10.0613841675067,-72.9050626819587,
81.1994391953708));
#109505=CARTESIAN_POINT('Ctrl Pts',(-10.0141484050549,-74.5477937036023,
81.3940612038461));
#109506=CARTESIAN_POINT('Ctrl Pts',(-9.99821434084186,-75.0887392883698,
81.4057498077921));
#109507=CARTESIAN_POINT('Ctrl Pts',(-9.95107381499787,-76.7198313848376,
81.2836479343613));
#109508=CARTESIAN_POINT('Ctrl Pts',(-9.92205777752795,-77.7860811621063,
80.98880100083));
#109509=CARTESIAN_POINT('Ctrl Pts',(-9.87445272111629,-79.2512592478914,
80.2540079646784));
#109510=CARTESIAN_POINT('Ctrl Pts',(-9.85856994315616,-79.7121317522274,
79.9639154167409));
#109511=CARTESIAN_POINT('Ctrl Pts',(-9.82776141766458,-80.5694853043513,
79.3002607780479));
#109512=CARTESIAN_POINT('Ctrl Pts',(-9.81289998677686,-80.9642323271672,
78.9286291622983));
#109513=CARTESIAN_POINT('Ctrl Pts',(-9.78278800959738,-81.6776414021401,
78.1136437405388));
#109514=CARTESIAN_POINT('Ctrl Pts',(-9.76713950264915,-81.9944277630583,
77.6720447722223));
#109515=CARTESIAN_POINT('Ctrl Pts',(-9.71888511166521,-82.8254614118745,
76.2390944889405));
#109516=CARTESIAN_POINT('Ctrl Pts',(-9.68879677956511,-83.1871168803284,
75.1735273461357));
#109517=CARTESIAN_POINT('Ctrl Pts',(-9.64188376543304,-83.3996442407148,
73.5337033427581));
#109518=CARTESIAN_POINT('Ctrl Pts',(-9.62595552208944,-83.4172930830374,
72.9934457186032));
#109519=CARTESIAN_POINT('Ctrl Pts',(-9.57887456877193,-83.3138029716328,
71.3677448194764));
#109520=CARTESIAN_POINT('Ctrl Pts',(-9.55003901146819,-83.0336270035935,
70.3040682601755));
#109521=CARTESIAN_POINT('Ctrl Pts',(-9.50279219367472,-82.3215645216885,
68.8357389347262));
#109522=CARTESIAN_POINT('Ctrl Pts',(-9.48688325147918,-82.0382993760529,
68.3719286886787));
#109523=CARTESIAN_POINT('Ctrl Pts',(-9.44069579575573,-81.0651421331075,
67.078493779823));
#109524=CARTESIAN_POINT('Ctrl Pts',(-9.4118759893924,-80.2586258546887,
66.350701061303));
#109525=CARTESIAN_POINT('Ctrl Pts',(-9.36464665559067,-78.8703628922013,
65.5138066548259));
#109526=CARTESIAN_POINT('Ctrl Pts',(-9.34888578959923,-78.3777232856237,
65.2786637690214));
#109527=CARTESIAN_POINT('Ctrl Pts',(-9.31831182400894,-77.3571698893145,
64.9082628219543));
#109528=CARTESIAN_POINT('Ctrl Pts',(-9.30355600029347,-76.8319066547898,
64.7732407130955));
#109529=CARTESIAN_POINT('Ctrl Pts',(-9.25814827124965,-75.2323844378279,
64.5232057622288));
#109530=CARTESIAN_POINT('Ctrl Pts',(-9.22604336406828,-74.1453066792442,
64.5632531277902));
#109531=CARTESIAN_POINT('Ctrl Pts',(-9.18099559830346,-72.5703710338625,
64.9298824555297));
#109532=CARTESIAN_POINT('Ctrl Pts',(-9.16631182716657,-72.0582549323504,
65.1023930613214));
#109533=CARTESIAN_POINT('Ctrl Pts',(-9.12434353015912,-70.7217192794661,
65.7010534404074));
#109534=CARTESIAN_POINT('Ctrl Pts',(-9.09714179453877,-69.9454865696347,
66.2162767140583));
#109535=CARTESIAN_POINT('Ctrl Pts',(-9.05632554412384,-68.8747503124929,
67.2155027246282));
#109536=CARTESIAN_POINT('Ctrl Pts',(-9.04164869831569,-68.516913096469,
67.6204391047425));
#109537=CARTESIAN_POINT('Ctrl Pts',(-9.00049457750973,-67.6729590190129,
68.7839745058294));
#109538=CARTESIAN_POINT('Ctrl Pts',(-8.97402578865247,-67.265570842812,
69.5910103927026));
#109539=CARTESIAN_POINT('Ctrl Pts',(-8.93387272636529,-66.830570845959,
70.9612572108593));
#109540=CARTESIAN_POINT('Ctrl Pts',(-8.91921129277492,-66.7172708014753,
71.4898077375009));
#109541=CARTESIAN_POINT('Ctrl Pts',(-8.89466879617357,-66.6184301835754,
72.3459818232941));
#109542=CARTESIAN_POINT('Ctrl Pts',(-8.88527448264431,-66.6,72.6676214331228));
#109543=CARTESIAN_POINT('Ctrl Pts',(-8.87591635085981,-66.6,72.9888893865799));
#109544=CARTESIAN_POINT('',(-9.46554776533453,-67.6016910344572,69.0108214572493));
#109545=CARTESIAN_POINT('Ctrl Pts',(-9.34771011126148,-66.6,72.98888938658));
#109546=CARTESIAN_POINT('Ctrl Pts',(-9.36658462513265,-66.6,72.3582412440757));
#109547=CARTESIAN_POINT('Ctrl Pts',(-9.38575644244071,-66.6710200899113,
71.7292661134848));
#109548=CARTESIAN_POINT('Ctrl Pts',(-9.42553652362212,-66.9798415869828,
70.3806592999566));
#109549=CARTESIAN_POINT('Ctrl Pts',(-9.44541826576314,-67.2454630876286,
69.6733255319622));
#109550=CARTESIAN_POINT('Ctrl Pts',(-9.46562408291506,-67.6016899012779,
69.0108235647079));
#109551=CARTESIAN_POINT('Ctrl Pts',(-9.46554776533453,-67.6016910344572,
69.0108214572493));
#109552=CARTESIAN_POINT('Ctrl Pts',(-9.48496609064942,-67.9295977010525,
68.4009890274292));
#109553=CARTESIAN_POINT('Ctrl Pts',(-9.50382515141497,-68.3316390992661,
67.8340483629832));
#109554=CARTESIAN_POINT('Ctrl Pts',(-9.54381168935438,-69.2636569651681,
66.8139762343873));
#109555=CARTESIAN_POINT('Ctrl Pts',(-9.56393837215954,-69.7895316897335,
66.3642193638286));
#109556=CARTESIAN_POINT('Ctrl Pts',(-9.59578124995521,-70.733377952405,
65.7396362524334));
#109557=CARTESIAN_POINT('Ctrl Pts',(-9.60794544192018,-71.1210391147184,
65.5250166898597));
#109558=CARTESIAN_POINT('Ctrl Pts',(-9.65053370411021,-72.5113857746416,
64.8929838099454));
#109559=CARTESIAN_POINT('Ctrl Pts',(-9.68276932829838,-73.5766360222517,
64.639583181404));
#109560=CARTESIAN_POINT('Ctrl Pts',(-9.72645125455699,-75.1374200423614,
64.5764667995703));
#109561=CARTESIAN_POINT('Ctrl Pts',(-9.73951499541836,-75.6150181377391,
64.5978537338206));
#109562=CARTESIAN_POINT('Ctrl Pts',(-9.77652195402752,-76.9122512082918,
64.7673359949956));
#109563=CARTESIAN_POINT('Ctrl Pts',(-9.8011822115001,-77.7157749353004,
64.9966897689716));
#109564=CARTESIAN_POINT('Ctrl Pts',(-9.8381660531439,-78.9091070172569,
65.5384675429136));
#109565=CARTESIAN_POINT('Ctrl Pts',(-9.85134595007298,-79.3279246808202,
65.7736992106172));
#109566=CARTESIAN_POINT('Ctrl Pts',(-9.88711752027425,-80.3877596955818,
66.4946051587608));
#109567=CARTESIAN_POINT('Ctrl Pts',(-9.91085166060931,-80.9830638831558,
67.0385469351782));
#109568=CARTESIAN_POINT('Ctrl Pts',(-9.95325056715723,-81.9242945269183,
68.1849397024771));
#109569=CARTESIAN_POINT('Ctrl Pts',(-9.97185214123004,-82.2908245884359,
68.7618751612809));
#109570=CARTESIAN_POINT('Ctrl Pts',(-10.0130713776169,-82.9232271672781,
70.0895844055562));
#109571=CARTESIAN_POINT('Ctrl Pts',(-10.0365015998053,-83.160564716385,
70.8467766916736));
#109572=CARTESIAN_POINT('Ctrl Pts',(-10.0741925591459,-83.3751732762724,
72.1518753417865));
#109573=CARTESIAN_POINT('Ctrl Pts',(-10.0889121225787,-83.4114029662636,
72.6848775572873));
#109574=CARTESIAN_POINT('Ctrl Pts',(-10.1348078381706,-83.3664488347047,
74.334518176599));
#109575=CARTESIAN_POINT('Ctrl Pts',(-10.1679540153276,-83.1135172714937,
75.434090013385));
#109576=CARTESIAN_POINT('Ctrl Pts',(-10.2131067043693,-82.448898112568,
76.9028173560589));
#109577=CARTESIAN_POINT('Ctrl Pts',(-10.2266396820162,-82.2054284024345,
77.33477306549));
#109578=CARTESIAN_POINT('Ctrl Pts',(-10.2654764363646,-81.427322458614,
78.4683014836411));
#109579=CARTESIAN_POINT('Ctrl Pts',(-10.2915976540544,-80.8183581845854,
79.1110775103155));
#109580=CARTESIAN_POINT('Ctrl Pts',(-10.3361756194551,-79.5622038415008,
80.077102840578));
#109581=CARTESIAN_POINT('Ctrl Pts',(-10.3552431054305,-78.9518458281728,
80.4346528318297));
#109582=CARTESIAN_POINT('Ctrl Pts',(-10.3888191919241,-77.8810753502658,
80.8927515485621));
#109583=CARTESIAN_POINT('Ctrl Pts',(-10.4023024920715,-77.4439700459721,
81.0386502139542));
#109584=CARTESIAN_POINT('Ctrl Pts',(-10.4368868675726,-76.2758307719957,
81.3245766780089));
#109585=CARTESIAN_POINT('Ctrl Pts',(-10.4572104458872,-75.5343220112447,
81.4047026315808));
#109586=CARTESIAN_POINT('Ctrl Pts',(-10.5087059409012,-73.6948718203082,
81.3591355804513));
#109587=CARTESIAN_POINT('Ctrl Pts',(-10.5412791004055,-72.613667306826,
81.1172234537493));
#109588=CARTESIAN_POINT('Ctrl Pts',(-10.5842616617643,-71.2030947285683,
80.494946788034));
#109589=CARTESIAN_POINT('Ctrl Pts',(-10.5964449208363,-70.8114820507407,
80.2836610881585));
#109590=CARTESIAN_POINT('Ctrl Pts',(-10.6239200527003,-69.9977607466304,
79.7574197422417));
#109591=CARTESIAN_POINT('Ctrl Pts',(-10.6393725027132,-69.5847744400246,
79.4317713352398));
#109592=CARTESIAN_POINT('Ctrl Pts',(-10.6773931560393,-68.6316145595861,
78.5233971989891));
#109593=CARTESIAN_POINT('Ctrl Pts',(-10.6991172465038,-68.1384856218894,
77.8987486456542));
#109594=CARTESIAN_POINT('Ctrl Pts',(-10.7434898581446,-67.3401635464417,
76.5271293521389));
#109595=CARTESIAN_POINT('Ctrl Pts',(-10.7670506978084,-67.0397922124725,
75.7866174143636));
#109596=CARTESIAN_POINT('Ctrl Pts',(-10.8050362051295,-66.7188429847764,
74.4952819336274));
#109597=CARTESIAN_POINT('Ctrl Pts',(-10.8198511362895,-66.6396689067076,
73.964414260643));
#109598=CARTESIAN_POINT('Ctrl Pts',(-10.8388232541245,-66.6038519551218,
73.2827238758526));
#109599=CARTESIAN_POINT('Ctrl Pts',(-10.8429169758835,-66.6,73.1357600143794));
#109600=CARTESIAN_POINT('Ctrl Pts',(-10.8470411184476,-66.6,72.98888938658));
#109601=CARTESIAN_POINT('Origin',(-15.9175364833309,-75.,72.98888938658));
#109602=CARTESIAN_POINT('',(-12.3474397125752,-66.60000000001,72.9889023383631));
#109603=CARTESIAN_POINT('',(-11.8763230992193,-66.6,72.98888938658));
#109604=CARTESIAN_POINT('',(-15.9175364833309,-66.6,72.98888938658));
#109605=CARTESIAN_POINT('',(-12.9679003706341,-82.2015397612608,68.6647904662762));
#109606=CARTESIAN_POINT('Ctrl Pts',(-12.3474400892301,-66.6,72.9888893865802));
#109607=CARTESIAN_POINT('Ctrl Pts',(-12.3626760155633,-66.6,72.4649816273803));
#109608=CARTESIAN_POINT('Ctrl Pts',(-12.3777612751813,-66.6490141176073,
71.9422119441476));
#109609=CARTESIAN_POINT('Ctrl Pts',(-12.4066962527405,-66.8403263929348,
70.9309779346599));
#109610=CARTESIAN_POINT('Ctrl Pts',(-12.4205238029993,-66.9788430599666,
70.4440307131329));
#109611=CARTESIAN_POINT('Ctrl Pts',(-12.4657516690178,-67.5568226075387,
68.9418400911724));
#109612=CARTESIAN_POINT('Ctrl Pts',(-12.4984264527936,-68.1527467712344,
67.9994325344402));
#109613=CARTESIAN_POINT('Ctrl Pts',(-12.5407531485241,-69.2013466167469,
66.8971280565159));
#109614=CARTESIAN_POINT('Ctrl Pts',(-12.5522155830747,-69.5108989977885,
66.616786289757));
#109615=CARTESIAN_POINT('Ctrl Pts',(-12.5953164764488,-70.7068140489397,
65.6857855976481));
#109616=CARTESIAN_POINT('Ctrl Pts',(-12.6274069825217,-71.6977037102949,
65.187489105859));
#109617=CARTESIAN_POINT('Ctrl Pts',(-12.6727423882884,-73.2711981139386,
64.7513784901037));
#109618=CARTESIAN_POINT('Ctrl Pts',(-12.687669814557,-73.7983899788031,
64.6581350928857));
#109619=CARTESIAN_POINT('Ctrl Pts',(-12.718550751688,-74.8592910802199,
64.5733546507773));
#109620=CARTESIAN_POINT('Ctrl Pts',(-12.7339958847427,-75.3905477198548,
64.5812431813904));
#109621=CARTESIAN_POINT('Ctrl Pts',(-12.7714181795336,-76.7012242271057,
64.7252666633024));
#109622=CARTESIAN_POINT('Ctrl Pts',(-12.7926048066354,-77.4689065878398,
64.9212923585636));
#109623=CARTESIAN_POINT('Ctrl Pts',(-12.8324865342203,-78.7511883261983,
65.4492260302197));
#109624=CARTESIAN_POINT('Ctrl Pts',(-12.8500679374427,-79.2785032522741,
65.7354507606983));
#109625=CARTESIAN_POINT('Ctrl Pts',(-12.8840699634655,-80.2605796609222,
66.4131592514461));
#109626=CARTESIAN_POINT('Ctrl Pts',(-12.9004039599877,-80.7129408500286,
66.8021108355024));
#109627=CARTESIAN_POINT('Ctrl Pts',(-12.9337253072399,-81.530721412008,
67.6720706009407));
#109628=CARTESIAN_POINT('Ctrl Pts',(-12.951210956824,-81.8931531007849,
68.1511958833952));
#109629=CARTESIAN_POINT('Ctrl Pts',(-12.9685679372243,-82.2015206898752,
68.6647594448114));
#109630=CARTESIAN_POINT('',(-12.9675940210686,-76.1752999551703,81.3061781097492));
#109631=CARTESIAN_POINT('Origin',(-12.9678999777142,-75.,72.98888938658));
#109632=CARTESIAN_POINT('Ctrl Pts',(-12.9672881034143,-76.1753032494785,
81.3062605020086));
#109633=CARTESIAN_POINT('Ctrl Pts',(-12.9456997237206,-76.9211863996156,
81.2008619478354));
#109634=CARTESIAN_POINT('Ctrl Pts',(-12.9250931772649,-77.6494936947553,
80.9956117455372));
#109635=CARTESIAN_POINT('Ctrl Pts',(-12.8827991508676,-79.0202689687081,
80.4014544074433));
#109636=CARTESIAN_POINT('Ctrl Pts',(-12.8610339737836,-79.6579587132031,
80.0182650931779));
#109637=CARTESIAN_POINT('Ctrl Pts',(-12.8264255828997,-80.6134893801562,
79.2563033741515));
#109638=CARTESIAN_POINT('Ctrl Pts',(-12.8131104264417,-80.9633694694468,
78.9243728348466));
#109639=CARTESIAN_POINT('Ctrl Pts',(-12.7846753651269,-81.6362980936601,
78.1660556733353));
#109640=CARTESIAN_POINT('Ctrl Pts',(-12.7692207392664,-81.9510335467936,
77.735109896772));
#109641=CARTESIAN_POINT('Ctrl Pts',(-12.7222821677812,-82.781285547952,
76.3367388231498));
#109642=CARTESIAN_POINT('Ctrl Pts',(-12.6927985335859,-83.1506594241578,
75.2961069719951));
#109643=CARTESIAN_POINT('Ctrl Pts',(-12.646115702509,-83.3865027676399,
73.6962723693769));
#109644=CARTESIAN_POINT('Ctrl Pts',(-12.6309515956989,-83.4142790606389,
73.1725797116149));
#109645=CARTESIAN_POINT('Ctrl Pts',(-12.6017435937532,-83.3726721322348,
72.1429828209544));
#109646=CARTESIAN_POINT('Ctrl Pts',(-12.5877313565474,-83.306346769762,
71.6391498446068));
#109647=CARTESIAN_POINT('Ctrl Pts',(-12.5585622960045,-83.0781712073388,
70.6253840143067));
#109648=CARTESIAN_POINT('Ctrl Pts',(-12.5430982084136,-82.912318620317,
70.1186636650525));
#109649=CARTESIAN_POINT('Ctrl Pts',(-12.4960994835157,-82.2610964223792,
68.6253809566896));
#109650=CARTESIAN_POINT('Ctrl Pts',(-12.4665274681307,-81.6297184639939,
67.7153177363067));
#109651=CARTESIAN_POINT('Ctrl Pts',(-12.4194435134014,-80.4583362182937,
66.5818216027056));
#109652=CARTESIAN_POINT('Ctrl Pts',(-12.4040232416618,-80.0409972621814,
66.2485396381113));
#109653=CARTESIAN_POINT('Ctrl Pts',(-12.3751276187305,-79.186146298515,
65.689943901073));
#109654=CARTESIAN_POINT('Ctrl Pts',(-12.3616365734621,-78.7548794823978,
65.4589954364309));
#109655=CARTESIAN_POINT('Ctrl Pts',(-12.3329899953647,-77.8171230685113,
65.0575196182307));
#109656=CARTESIAN_POINT('Ctrl Pts',(-12.3175212803872,-77.3094826241488,
64.8951218378516));
#109657=CARTESIAN_POINT('Ctrl Pts',(-12.2705039573595,-75.7168016277099,
64.5477663236539));
#109658=CARTESIAN_POINT('Ctrl Pts',(-12.2408979718944,-74.6081372569116,
64.5264545930802));
#109659=CARTESIAN_POINT('Ctrl Pts',(-12.1935275275859,-72.9940114982936,
64.8139948810565));
#109660=CARTESIAN_POINT('Ctrl Pts',(-12.1778786286812,-72.4716137046989,
64.9601802674696));
#109661=CARTESIAN_POINT('Ctrl Pts',(-12.1468429563381,-71.4477448127881,
65.3566266280318));
#109662=CARTESIAN_POINT('Ctrl Pts',(-12.1315521837551,-70.9498506072715,
65.6087655502416));
#109663=CARTESIAN_POINT('Ctrl Pts',(-12.1007394784222,-70.0325547170444,
66.194260241545));
#109664=CARTESIAN_POINT('Ctrl Pts',(-12.0851889193739,-69.6126902487047,
66.5220985011274));
#109665=CARTESIAN_POINT('Ctrl Pts',(-12.0621049879559,-69.0288807199379,
67.0745129171562));
#109666=CARTESIAN_POINT('Ctrl Pts',(-12.0543598138416,-68.840346558027,
67.2711287936886));
#109667=CARTESIAN_POINT('Ctrl Pts',(-12.0316473743537,-68.3116677833476,
67.8790251409699));
#109668=CARTESIAN_POINT('Ctrl Pts',(-12.0169935993769,-68.0007787500592,
68.3139146928697));
#109669=CARTESIAN_POINT('Ctrl Pts',(-11.9857968177324,-67.4492373973459,
69.2651114990225));
#109670=CARTESIAN_POINT('Ctrl Pts',(-11.9692137356407,-67.2154872687839,
69.7823487810449));
#109671=CARTESIAN_POINT('Ctrl Pts',(-11.9452118668441,-66.9490366567213,
70.5772348364475));
#109672=CARTESIAN_POINT('Ctrl Pts',(-11.9374997910295,-66.8751218618912,
70.839367153819));
#109673=CARTESIAN_POINT('Ctrl Pts',(-11.9149154892498,-66.6948599518037,
71.6224916727647));
#109674=CARTESIAN_POINT('Ctrl Pts',(-11.9003192101525,-66.6250678775911,
72.1504973487997));
#109675=CARTESIAN_POINT('Ctrl Pts',(-11.8822182814411,-66.6018737675323,
72.7839881357388));
#109676=CARTESIAN_POINT('Ctrl Pts',(-11.8792748568318,-66.6,72.8864534468495));
#109677=CARTESIAN_POINT('Ctrl Pts',(-11.8763230992193,-66.6,72.98888938658));
#109678=CARTESIAN_POINT('Origin',(20.412052742069,1.37771738462078E-14,
115.762503617193));
#109679=CARTESIAN_POINT('',(4.63472787570938,-6.63404734029626E-9,124.183946153848));
#109680=CARTESIAN_POINT('',(4.68550323141337,7.30187960605121E-9,124.471907505537));
#109681=CARTESIAN_POINT('',(3.67032094086137,1.16952742876573E-14,118.71452263753));
#109682=CARTESIAN_POINT('',(30.2384437550856,-14.4989439202996,120.376781885352));
#109683=CARTESIAN_POINT('Ctrl Pts',(4.68550323141337,1.46037510969853E-8,
124.471907505537));
#109684=CARTESIAN_POINT('Ctrl Pts',(4.68564827370219,-0.0743379810781902,
124.4727300816));
#109685=CARTESIAN_POINT('Ctrl Pts',(4.68627286904241,-0.148681666873179,
124.473464359407));
#109686=CARTESIAN_POINT('Ctrl Pts',(4.69257555007263,-0.572921405614114,
124.477154396249));
#109687=CARTESIAN_POINT('Ctrl Pts',(4.70840025566492,-0.922591984769783,
124.478256410096));
#109688=CARTESIAN_POINT('Ctrl Pts',(4.79765327972258,-2.10050392452701,
124.475642272939));
#109689=CARTESIAN_POINT('Ctrl Pts',(4.92026554240755,-2.92379093403069,
124.463270047188));
#109690=CARTESIAN_POINT('Ctrl Pts',(5.23049420774179,-4.31005019464808,
124.424904003855));
#109691=CARTESIAN_POINT('Ctrl Pts',(5.38864643116668,-4.87819396260196,
124.403924131801));
#109692=CARTESIAN_POINT('Ctrl Pts',(5.72449970156122,-5.88215598968838,
124.357091151595));
#109693=CARTESIAN_POINT('Ctrl Pts',(5.891563799614,-6.32098936543384,124.333097915783));
#109694=CARTESIAN_POINT('Ctrl Pts',(6.39590073385846,-7.49844651927192,
124.258670844125));
#109695=CARTESIAN_POINT('Ctrl Pts',(6.76776540910955,-8.22049418077532,
124.201991251208));
#109696=CARTESIAN_POINT('Ctrl Pts',(7.55229337962165,-9.5095650593795,124.080723281539));
#109697=CARTESIAN_POINT('Ctrl Pts',(7.95146783756154,-10.0829863563159,
124.018416423071));
#109698=CARTESIAN_POINT('Ctrl Pts',(8.82277626176177,-11.18364055349,123.881264840435));
#109699=CARTESIAN_POINT('Ctrl Pts',(9.29491914946344,-11.7091190057174,
123.806386896715));
#109700=CARTESIAN_POINT('Ctrl Pts',(10.3889305316597,-12.7836098358227,
123.630927636382));
#109701=CARTESIAN_POINT('Ctrl Pts',(11.0210922270172,-13.3192253171763,
123.528559568179));
#109702=CARTESIAN_POINT('Ctrl Pts',(12.262108460875,-14.2225124881724,123.327179453397));
#109703=CARTESIAN_POINT('Ctrl Pts',(12.8600982777439,-14.602348817636,123.229976122717));
#109704=CARTESIAN_POINT('Ctrl Pts',(14.0686669900347,-15.2665387834022,
123.033146520733));
#109705=CARTESIAN_POINT('Ctrl Pts',(14.6760428194664,-15.5541209818477,
122.934038709541));
#109706=CARTESIAN_POINT('Ctrl Pts',(16.0579033604686,-16.1090380798308,
122.707406272866));
#109707=CARTESIAN_POINT('Ctrl Pts',(16.8379981425549,-16.3573452565906,
122.578898903116));
#109708=CARTESIAN_POINT('Ctrl Pts',(18.3253530897156,-16.712404758408,122.334106834635));
#109709=CARTESIAN_POINT('Ctrl Pts',(19.0275441866904,-16.8329062920111,
122.218618283029));
#109710=CARTESIAN_POINT('Ctrl Pts',(20.4144969794751,-16.979830770254,121.990588689274));
#109711=CARTESIAN_POINT('Ctrl Pts',(21.0975413897469,-17.0096851753466,
121.878299745259));
#109712=CARTESIAN_POINT('Ctrl Pts',(22.597464642579,-16.9823965839081,121.63098305236));
#109713=CARTESIAN_POINT('Ctrl Pts',(23.4122980386457,-16.9070459274975,
121.496350274446));
#109714=CARTESIAN_POINT('Ctrl Pts',(24.9340099703691,-16.6517959298589,
121.245655591693));
#109715=CARTESIAN_POINT('Ctrl Pts',(25.6411075310777,-16.4848888458814,
121.129465369349));
#109716=CARTESIAN_POINT('Ctrl Pts',(26.6318113393197,-16.1812956925445,
120.967037051241));
#109717=CARTESIAN_POINT('Ctrl Pts',(26.9257278238795,-16.0821510867243,
120.918889926016));
#109718=CARTESIAN_POINT('Ctrl Pts',(27.5878226962084,-15.8379819205855,
120.810455249672));
#109719=CARTESIAN_POINT('Ctrl Pts',(27.9539936514165,-15.6879134099066,
120.750483768592));
#109720=CARTESIAN_POINT('Ctrl Pts',(28.9770567766332,-15.2254104878708,
120.582852082652));
#109721=CARTESIAN_POINT('Ctrl Pts',(29.6196615370995,-14.8827084382633,
120.477610290641));
#109722=CARTESIAN_POINT('Ctrl Pts',(30.2384437550856,-14.4989439202997,
120.376781885352));
#109723=CARTESIAN_POINT('',(30.1878779053518,-14.4989439202996,120.090008701063));
#109724=CARTESIAN_POINT('',(29.1530537532117,-14.4989439202996,114.221229300528));
#109725=CARTESIAN_POINT('Ctrl Pts',(30.1878779053518,-14.4989439202996,
120.090008701063));
#109726=CARTESIAN_POINT('Ctrl Pts',(29.5701295220062,-14.8820451102276,
120.190460271193));
#109727=CARTESIAN_POINT('Ctrl Pts',(28.9285701908142,-15.2242262275709,
120.294914406511));
#109728=CARTESIAN_POINT('Ctrl Pts',(27.9073160249098,-15.6861599886167,
120.461871165917));
#109729=CARTESIAN_POINT('Ctrl Pts',(27.5418339166123,-15.8360734413756,
120.521789705476));
#109730=CARTESIAN_POINT('Ctrl Pts',(26.8646223178921,-16.0861078665858,
120.633036292489));
#109731=CARTESIAN_POINT('Ctrl Pts',(26.5545570371305,-16.1903051542107,
120.684039716594));
#109732=CARTESIAN_POINT('Ctrl Pts',(25.5570642222654,-16.4930572565071,
120.848181542795));
#109733=CARTESIAN_POINT('Ctrl Pts',(24.8600455730495,-16.6563022852734,
120.962939974118));
#109734=CARTESIAN_POINT('Ctrl Pts',(23.3507635550836,-16.9082118704466,
121.211177868491));
#109735=CARTESIAN_POINT('Ctrl Pts',(22.5380569345925,-16.9828670967508,
121.344681854524));
#109736=CARTESIAN_POINT('Ctrl Pts',(21.0480142701009,-17.0094006459033,
121.590004776062));
#109737=CARTESIAN_POINT('Ctrl Pts',(20.3727177501221,-16.9800894283706,
121.701531418683));
#109738=CARTESIAN_POINT('Ctrl Pts',(18.9896530367671,-16.8349601996727,
121.929735369205));
#109739=CARTESIAN_POINT('Ctrl Pts',(18.2837348045804,-16.7142929021189,
122.046064271911));
#109740=CARTESIAN_POINT('Ctrl Pts',(16.7908971654717,-16.3584520046763,
122.291371962011));
#109741=CARTESIAN_POINT('Ctrl Pts',(16.0089806753838,-16.1097518691709,
122.419412700195));
#109742=CARTESIAN_POINT('Ctrl Pts',(14.6252517891792,-15.5541270414664,
122.646037158988));
#109743=CARTESIAN_POINT('Ctrl Pts',(14.0177604233313,-15.2664441128617,
122.745669266514));
#109744=CARTESIAN_POINT('Ctrl Pts',(12.8092235798815,-14.6021563898349,
122.94325916373));
#109745=CARTESIAN_POINT('Ctrl Pts',(12.2113582116683,-14.2223614982591,
123.040639736479));
#109746=CARTESIAN_POINT('Ctrl Pts',(10.9703857883329,-13.319140548469,123.241587762053));
#109747=CARTESIAN_POINT('Ctrl Pts',(10.3381161873546,-12.783541683539,123.34317782452));
#109748=CARTESIAN_POINT('Ctrl Pts',(9.24412514645092,-11.7091171754883,
123.518306828543));
#109749=CARTESIAN_POINT('Ctrl Pts',(8.77212271484894,-11.1836890435598,
123.593730560265));
#109750=CARTESIAN_POINT('Ctrl Pts',(7.90096264894464,-10.0830689066474,
123.731645860865));
#109751=CARTESIAN_POINT('Ctrl Pts',(7.50180343829981,-9.50962956334363,
123.7941365166));
#109752=CARTESIAN_POINT('Ctrl Pts',(6.71725850540307,-8.22065362099649,
123.915004885026));
#109753=CARTESIAN_POINT('Ctrl Pts',(6.34531547753253,-7.4987275441189,123.970953455009));
#109754=CARTESIAN_POINT('Ctrl Pts',(5.84016412446256,-6.31956294685888,
124.045228617864));
#109755=CARTESIAN_POINT('Ctrl Pts',(5.67248743109575,-5.87882814455977,
124.069518606313));
#109756=CARTESIAN_POINT('Ctrl Pts',(5.33660785118728,-4.87340004955567,
124.116937905333));
#109757=CARTESIAN_POINT('Ctrl Pts',(5.1788295887776,-4.30577333755577,124.138227112189));
#109758=CARTESIAN_POINT('Ctrl Pts',(4.868097817236,-2.91562234570062,124.1768908874));
#109759=CARTESIAN_POINT('Ctrl Pts',(4.74525087389593,-2.0877918727058,124.188805864713));
#109760=CARTESIAN_POINT('Ctrl Pts',(4.65694693069434,-0.908304068096513,
124.190531793008));
#109761=CARTESIAN_POINT('Ctrl Pts',(4.64148162450515,-0.561621361795577,
124.189204435518));
#109762=CARTESIAN_POINT('Ctrl Pts',(4.63545287952606,-0.14314631240032,
124.185455054707));
#109763=CARTESIAN_POINT('Ctrl Pts',(4.63486751849338,-0.0715705611967255,
124.184738107108));
#109764=CARTESIAN_POINT('Ctrl Pts',(4.63472787570938,-1.32681063758668E-8,
124.183946153848));
#109765=CARTESIAN_POINT('Origin',(20.412052742069,1.37771738462078E-14,
115.762503617193));
#109766=CARTESIAN_POINT('',(4.42635006251054,-6.99305973109813E-9,123.002176850242));
#109767=CARTESIAN_POINT('',(4.47712541821256,7.41991074646819E-9,123.290138201919));
#109768=CARTESIAN_POINT('',(3.67032094086137,1.16952742876573E-14,118.71452263753));
#109769=CARTESIAN_POINT('Ctrl Pts',(4.47712541821256,1.48397794296156E-8,
123.290138201919));
#109770=CARTESIAN_POINT('Ctrl Pts',(4.47726710739396,-0.0726194254213628,
123.290941761563));
#109771=CARTESIAN_POINT('Ctrl Pts',(4.47786642876489,-0.145242030801444,
123.291661033145));
#109772=CARTESIAN_POINT('Ctrl Pts',(4.4839900234646,-0.565888684765446,
123.295342776981));
#109773=CARTESIAN_POINT('Ctrl Pts',(4.49956960224922,-0.913695551972098,
123.296467862352));
#109774=CARTESIAN_POINT('Ctrl Pts',(4.5881584050187,-2.09260838461004,123.293981907897));
#109775=CARTESIAN_POINT('Ctrl Pts',(4.71087360778027,-2.91874233122078,
123.281620794682));
#109776=CARTESIAN_POINT('Ctrl Pts',(5.02145288530558,-4.30744933963609,
123.243220534685));
#109777=CARTESIAN_POINT('Ctrl Pts',(5.17941587740385,-4.87527836343719,
123.222269549424));
#109778=CARTESIAN_POINT('Ctrl Pts',(5.51534037461342,-5.88011093708854,
123.175434153231));
#109779=CARTESIAN_POINT('Ctrl Pts',(5.68279148735017,-6.32008300865983,
123.151387016631));
#109780=CARTESIAN_POINT('Ctrl Pts',(6.1928471241179,-7.51085101143989,123.076115498515));
#109781=CARTESIAN_POINT('Ctrl Pts',(6.57167088586724,-8.24429588437859,
123.018351219207));
#109782=CARTESIAN_POINT('Ctrl Pts',(7.37775550214019,-9.56183272718522,
122.893697423682));
#109783=CARTESIAN_POINT('Ctrl Pts',(7.79222255393772,-10.1517879468699,
122.828968417862));
#109784=CARTESIAN_POINT('Ctrl Pts',(8.65107706329844,-11.2228313172068,
122.693663517979));
#109785=CARTESIAN_POINT('Ctrl Pts',(9.08844495476356,-11.7080474871114,
122.6242758755));
#109786=CARTESIAN_POINT('Ctrl Pts',(9.79559488252792,-12.4068905234439,
122.51091543823));
#109787=CARTESIAN_POINT('Ctrl Pts',(10.0460199870314,-12.6397930351342,
122.470590049202));
#109788=CARTESIAN_POINT('Ctrl Pts',(10.9291441118157,-13.4124499277954,
122.328005155286));
#109789=CARTESIAN_POINT('Ctrl Pts',(11.5940608970191,-13.9124565891058,
122.220074715601));
#109790=CARTESIAN_POINT('Ctrl Pts',(12.7826564008686,-14.6752591008048,
122.026875198773));
#109791=CARTESIAN_POINT('Ctrl Pts',(13.2884442990623,-14.9637962926425,
121.944572128034));
#109792=CARTESIAN_POINT('Ctrl Pts',(14.229393597922,-15.4373161629874,121.791102013483));
#109793=CARTESIAN_POINT('Ctrl Pts',(14.659459240168,-15.6313578002585,121.720816239832));
#109794=CARTESIAN_POINT('Ctrl Pts',(15.8542046992472,-16.1105360086866,
121.524865880265));
#109795=CARTESIAN_POINT('Ctrl Pts',(16.6321701366166,-16.357971279845,121.396709931516));
#109796=CARTESIAN_POINT('Ctrl Pts',(18.1175366256271,-16.7125236047627,
121.152245156299));
#109797=CARTESIAN_POINT('Ctrl Pts',(18.8199602692764,-16.833035010911,121.03671845183));
#109798=CARTESIAN_POINT('Ctrl Pts',(20.1759966418076,-16.9765988721232,
120.813771847341));
#109799=CARTESIAN_POINT('Ctrl Pts',(20.827583214368,-17.0068888142712,120.706660954248));
#109800=CARTESIAN_POINT('Ctrl Pts',(21.820209012274,-16.9943992689521,120.543023716793));
#109801=CARTESIAN_POINT('Ctrl Pts',(22.1609957504813,-16.9795708430236,
120.486779729856));
#109802=CARTESIAN_POINT('Ctrl Pts',(23.325454646438,-16.8927916932291,120.294602461011));
#109803=CARTESIAN_POINT('Ctrl Pts',(24.1442118184467,-16.7696892735206,
120.159547596836));
#109804=CARTESIAN_POINT('Ctrl Pts',(25.5176572295265,-16.4567561936441,
119.93376984732));
#109805=CARTESIAN_POINT('Ctrl Pts',(26.0775963611282,-16.2978290350979,
119.841933221202));
#109806=CARTESIAN_POINT('Ctrl Pts',(27.0706331175051,-15.9587349207325,
119.679247215503));
#109807=CARTESIAN_POINT('Ctrl Pts',(27.506582159557,-15.7890434224299,119.607878628462));
#109808=CARTESIAN_POINT('Ctrl Pts',(28.6822938465005,-15.2733798568659,
119.415240504232));
#109809=CARTESIAN_POINT('Ctrl Pts',(29.4050751174609,-14.890910317626,119.296813994894));
#109810=CARTESIAN_POINT('Ctrl Pts',(30.7029291554557,-14.0774185471333,
119.085409354161));
#109811=CARTESIAN_POINT('Ctrl Pts',(31.2838112138742,-13.659438615725,118.991311323907));
#109812=CARTESIAN_POINT('Ctrl Pts',(32.3436767356981,-12.7891934101714,
118.82059023505));
#109813=CARTESIAN_POINT('Ctrl Pts',(32.8262181267685,-12.3434373449856,
118.74329168774));
#109814=CARTESIAN_POINT('Ctrl Pts',(33.5203587225289,-11.6228610168815,
118.632291722921));
#109815=CARTESIAN_POINT('Ctrl Pts',(33.7512839999439,-11.368044617997,118.595420807397));
#109816=CARTESIAN_POINT('Ctrl Pts',(34.5148247305714,-10.4722093879614,
118.473935462488));
#109817=CARTESIAN_POINT('Ctrl Pts',(35.0083733806634,-9.79857835634418,
118.396221496327));
#109818=CARTESIAN_POINT('Ctrl Pts',(35.7623443492901,-8.59329982286537,
118.279671845147));
#109819=CARTESIAN_POINT('Ctrl Pts',(36.047962815817,-8.07969204257989,118.236205745305));
#109820=CARTESIAN_POINT('Ctrl Pts',(36.5145795284203,-7.12849545794011,
118.166340750437));
#109821=CARTESIAN_POINT('Ctrl Pts',(36.7048996527446,-6.69627012201427,
118.138281759079));
#109822=CARTESIAN_POINT('Ctrl Pts',(37.1775286435375,-5.49021941209475,
118.06960451221));
#109823=CARTESIAN_POINT('Ctrl Pts',(37.4225200973712,-4.7028020707478,118.035415526615));
#109824=CARTESIAN_POINT('Ctrl Pts',(37.7742471616853,-3.2005590827442,117.990806851836));
#109825=CARTESIAN_POINT('Ctrl Pts',(37.8942651576518,-2.49078908479819,
117.977949248992));
#109826=CARTESIAN_POINT('Ctrl Pts',(38.0393918667326,-1.11430684535171,
117.968546067397));
#109827=CARTESIAN_POINT('Ctrl Pts',(38.0708575434234,-0.449571596658077,
117.970832686332));
#109828=CARTESIAN_POINT('Ctrl Pts',(38.0601978907253,0.562330993406072,
117.984167448484));
#109829=CARTESIAN_POINT('Ctrl Pts',(38.0460622599845,0.909200456291852,
117.990521993183));
#109830=CARTESIAN_POINT('Ctrl Pts',(37.9623049703988,2.08859751610441,118.018430670423));
#109831=CARTESIAN_POINT('Ctrl Pts',(37.8427218298197,2.91614475365796,118.048807782335));
#109832=CARTESIAN_POINT('Ctrl Pts',(37.5375804721073,4.30605508152657,118.118989196761));
#109833=CARTESIAN_POINT('Ctrl Pts',(37.3820784757013,4.87371622890115,118.153308155663));
#109834=CARTESIAN_POINT('Ctrl Pts',(37.0503498179034,5.87903954221305,118.224203757609));
#109835=CARTESIAN_POINT('Ctrl Pts',(36.8845582822338,6.31964458661868,118.258924257963));
#109836=CARTESIAN_POINT('Ctrl Pts',(36.3772894788796,7.5156312662834,118.363098743256));
#109837=CARTESIAN_POINT('Ctrl Pts',(35.9989345561713,8.25337230171225,118.438899254589));
#109838=CARTESIAN_POINT('Ctrl Pts',(35.1889221097438,9.58454817338106,118.599402767094));
#109839=CARTESIAN_POINT('Ctrl Pts',(34.7693860529488,10.1833906406674,118.681875995441));
#109840=CARTESIAN_POINT('Ctrl Pts',(33.9015402757136,11.2659977141092,118.851253797059));
#109841=CARTESIAN_POINT('Ctrl Pts',(33.4608494056369,11.7543667180551,118.936756265481));
#109842=CARTESIAN_POINT('Ctrl Pts',(32.4088127439031,12.7911693969336,119.139099846695));
#109843=CARTESIAN_POINT('Ctrl Pts',(31.783759835985,13.3228138808301,119.258353971258));
#109844=CARTESIAN_POINT('Ctrl Pts',(30.5529657072893,14.222935742887,119.492760409275));
#109845=CARTESIAN_POINT('Ctrl Pts',(29.9575394264109,14.6028899201329,119.605991973676));
#109846=CARTESIAN_POINT('Ctrl Pts',(28.7548010288241,15.2668114071306,119.834336761636));
#109847=CARTESIAN_POINT('Ctrl Pts',(28.1507279910629,15.5541070166201,119.948832320717));
#109848=CARTESIAN_POINT('Ctrl Pts',(26.7795332931003,16.1071303561815,120.207578457541));
#109849=CARTESIAN_POINT('Ctrl Pts',(26.007001721396,16.3543933621251,120.352791411082));
#109850=CARTESIAN_POINT('Ctrl Pts',(24.5388686012415,16.7076229142211,120.628974248775));
#109851=CARTESIAN_POINT('Ctrl Pts',(23.8483729754278,16.8277840263982,120.758944926695));
#109852=CARTESIAN_POINT('Ctrl Pts',(22.4868589598444,16.9759982442222,121.015307040707));
#109853=CARTESIAN_POINT('Ctrl Pts',(21.8175169347674,17.0076877567862,121.141361231551));
#109854=CARTESIAN_POINT('Ctrl Pts',(20.8012630487746,16.9936341543844,121.332253163968));
#109855=CARTESIAN_POINT('Ctrl Pts',(20.4546880305645,16.9778537650809,121.39728774047));
#109856=CARTESIAN_POINT('Ctrl Pts',(19.2985521900949,16.888455261997,121.61425092934));
#109857=CARTESIAN_POINT('Ctrl Pts',(18.4938436921505,16.7657433432543,121.76534324417));
#109858=CARTESIAN_POINT('Ctrl Pts',(17.1353543843919,16.4541818642168,122.02117199174));
#109859=CARTESIAN_POINT('Ctrl Pts',(16.5765828552586,16.2945175961528,122.126611493036));
#109860=CARTESIAN_POINT('Ctrl Pts',(15.5911296520151,15.9557097573121,122.312747046023));
#109861=CARTESIAN_POINT('Ctrl Pts',(15.16141311943,15.7875404630745,122.393962901539));
#109862=CARTESIAN_POINT('Ctrl Pts',(14.0057919657937,15.2785940527204,122.612212836553));
#109863=CARTESIAN_POINT('Ctrl Pts',(13.2962367064769,14.9025423280946,122.74621669592));
#109864=CARTESIAN_POINT('Ctrl Pts',(12.0297019974583,14.1089057733664,122.986605875152));
#109865=CARTESIAN_POINT('Ctrl Pts',(11.4664028315628,13.7050046544477,123.094008585962));
#109866=CARTESIAN_POINT('Ctrl Pts',(10.3852265119859,12.8230888014638,123.301133501878));
#109867=CARTESIAN_POINT('Ctrl Pts',(9.86908329909161,12.3450451709572,123.400518359888));
#109868=CARTESIAN_POINT('Ctrl Pts',(8.81379677784519,11.2370635297596,123.604040065611));
#109869=CARTESIAN_POINT('Ctrl Pts',(8.28784808843838,10.5966828690373,123.705878681044));
#109870=CARTESIAN_POINT('Ctrl Pts',(7.4011641493878,9.33936280823163,123.879672015218));
#109871=CARTESIAN_POINT('Ctrl Pts',(7.0284410076656,8.73343022202691,123.953633541791));
#109872=CARTESIAN_POINT('Ctrl Pts',(6.37727593432207,7.50919786515016,124.084722821822));
#109873=CARTESIAN_POINT('Ctrl Pts',(6.09559017557435,6.89417277130976,124.142376107457));
#109874=CARTESIAN_POINT('Ctrl Pts',(5.55309807168489,5.49682657683749,124.255024330068));
#109875=CARTESIAN_POINT('Ctrl Pts',(5.31070621857193,4.70892781309154,124.306779935966));
#109876=CARTESIAN_POINT('Ctrl Pts',(4.96510428886854,3.20971846714564,124.385093552756));
#109877=CARTESIAN_POINT('Ctrl Pts',(4.84805761747887,2.50358477454962,124.413992821971));
#109878=CARTESIAN_POINT('Ctrl Pts',(4.71425788489729,1.19668922403474,124.452953463954));
#109879=CARTESIAN_POINT('Ctrl Pts',(4.68433543010682,0.598528962184033,
124.465284572257));
#109880=CARTESIAN_POINT('Ctrl Pts',(4.68550323141337,1.46037466841609E-8,
124.471907505537));
#109881=CARTESIAN_POINT('Ctrl Pts',(4.63472787570938,-1.32681063758668E-8,
124.183946153848));
#109882=CARTESIAN_POINT('Ctrl Pts',(4.63357157043953,0.592636422127183,
124.177388423457));
#109883=CARTESIAN_POINT('Ctrl Pts',(4.66297372869761,1.18491592147218,124.165673028352));
#109884=CARTESIAN_POINT('Ctrl Pts',(4.79535858097764,2.48992208384337,124.127738563659));
#109885=CARTESIAN_POINT('Ctrl Pts',(4.91258361015162,3.1999427312807,124.098981089495));
#109886=CARTESIAN_POINT('Ctrl Pts',(5.25855027326533,4.70347259587108,124.02016279834));
#109887=CARTESIAN_POINT('Ctrl Pts',(5.50069974380765,5.49189538696322,123.967681467881));
#109888=CARTESIAN_POINT('Ctrl Pts',(5.9729331803421,6.70938852304439,123.869335083525));
#109889=CARTESIAN_POINT('Ctrl Pts',(6.16643530167966,7.15174597138867,123.829807597709));
#109890=CARTESIAN_POINT('Ctrl Pts',(6.63427325815816,8.10874803164791,123.735420060841));
#109891=CARTESIAN_POINT('Ctrl Pts',(6.91673549416129,8.61859562765863,123.679122811554));
#109892=CARTESIAN_POINT('Ctrl Pts',(7.66404939373591,9.81809160784466,123.531261478371));
#109893=CARTESIAN_POINT('Ctrl Pts',(8.15418404773268,10.4896091503913,123.435085626319));
#109894=CARTESIAN_POINT('Ctrl Pts',(8.91077529748588,11.3805295719812,123.287890510379));
#109895=CARTESIAN_POINT('Ctrl Pts',(9.13825790805126,11.6325708872509,123.243780892955));
#109896=CARTESIAN_POINT('Ctrl Pts',(9.81917170333162,12.3426106797737,123.112310209786));
#109897=CARTESIAN_POINT('Ctrl Pts',(10.2912190591203,12.7813310244438,123.021909785701));
#109898=CARTESIAN_POINT('Ctrl Pts',(11.3402602602008,13.6493968402062,122.821635047057));
#109899=CARTESIAN_POINT('Ctrl Pts',(11.921991240648,14.0707877586969,122.710903425858));
#109900=CARTESIAN_POINT('Ctrl Pts',(13.2195939591294,14.8886845370294,122.464188312415));
#109901=CARTESIAN_POINT('Ctrl Pts',(13.9411142114959,15.2723924140214,122.327155221566));
#109902=CARTESIAN_POINT('Ctrl Pts',(15.1141058611886,15.7891010123792,122.10534577233));
#109903=CARTESIAN_POINT('Ctrl Pts',(15.5484701412069,15.9588860860178,122.023465292593));
#109904=CARTESIAN_POINT('Ctrl Pts',(16.5375748734356,16.2980065214732,121.837243554514));
#109905=CARTESIAN_POINT('Ctrl Pts',(17.0951546556599,16.4568941708419,121.732399387658));
#109906=CARTESIAN_POINT('Ctrl Pts',(18.4634379763096,16.7698780388701,121.474983543641));
#109907=CARTESIAN_POINT('Ctrl Pts',(19.2794125264515,16.8929924618159,121.321329198961));
#109908=CARTESIAN_POINT('Ctrl Pts',(20.4394063893845,16.9796485897213,121.102938142948));
#109909=CARTESIAN_POINT('Ctrl Pts',(20.7785206470763,16.9944338485635,121.039108612961));
#109910=CARTESIAN_POINT('Ctrl Pts',(21.7659172030619,17.006851832197,120.853452568004));
#109911=CARTESIAN_POINT('Ctrl Pts',(22.4139513849207,16.9766294906685,120.731921604675));
#109912=CARTESIAN_POINT('Ctrl Pts',(23.7640956552689,16.8332861610225,120.478497874152));
#109913=CARTESIAN_POINT('Ctrl Pts',(24.4641618784954,16.7127549740021,120.346946306104));
#109914=CARTESIAN_POINT('Ctrl Pts',(25.9449995939361,16.3579054491669,120.067983022337));
#109915=CARTESIAN_POINT('Ctrl Pts',(26.7207744482822,16.1100930037214,119.921396678967));
#109916=CARTESIAN_POINT('Ctrl Pts',(27.9174338041455,15.6278795962631,119.695311392062));
#109917=CARTESIAN_POINT('Ctrl Pts',(28.351459801186,15.4308092630801,119.613381450854));
#109918=CARTESIAN_POINT('Ctrl Pts',(29.291496151248,14.9540699813087,119.435738308823));
#109919=CARTESIAN_POINT('Ctrl Pts',(29.7927425512057,14.6660643413089,119.340860955432));
#109920=CARTESIAN_POINT('Ctrl Pts',(30.9717280914689,13.904309659069,119.116879611861));
#109921=CARTESIAN_POINT('Ctrl Pts',(31.6315847950258,13.40485592162,118.990775086813));
#109922=CARTESIAN_POINT('Ctrl Pts',(32.5069739183114,12.6339912528137,118.822627782942));
#109923=CARTESIAN_POINT('Ctrl Pts',(32.7546636230453,12.4021788087266,118.774952628272));
#109924=CARTESIAN_POINT('Ctrl Pts',(33.452587944606,11.7082093421025,118.640472513404));
#109925=CARTESIAN_POINT('Ctrl Pts',(33.8838359623335,11.2271475981415,118.557259176847));
#109926=CARTESIAN_POINT('Ctrl Pts',(34.7362228595714,10.158936018922,118.391656022213));
#109927=CARTESIAN_POINT('Ctrl Pts',(35.1496104240714,9.56704498839497,118.310611140704));
#109928=CARTESIAN_POINT('Ctrl Pts',(35.9524576718099,8.24551765601765,118.151124099521));
#109929=CARTESIAN_POINT('Ctrl Pts',(36.3291196246265,7.51002525281455,118.074883742046));
#109930=CARTESIAN_POINT('Ctrl Pts',(36.9168427607941,6.12344419029734,117.953856293388));
#109931=CARTESIAN_POINT('Ctrl Pts',(37.1449006259391,5.4816989161467,117.90612396153));
#109932=CARTESIAN_POINT('Ctrl Pts',(37.5323543182424,4.14422801197669,117.822276593452));
#109933=CARTESIAN_POINT('Ctrl Pts',(37.6878035740198,3.44869736947842,117.786842040869));
#109934=CARTESIAN_POINT('Ctrl Pts',(37.9296721133059,1.92890058915011,117.726415139698));
#109935=CARTESIAN_POINT('Ctrl Pts',(38.0006893590256,1.10391386477906,117.704076319898));
#109936=CARTESIAN_POINT('Ctrl Pts',(38.021701197603,-0.389567927783994,
117.683161829751));
#109937=CARTESIAN_POINT('Ctrl Pts',(37.9925285049393,-1.05603275334111,
117.680953085576));
#109938=CARTESIAN_POINT('Ctrl Pts',(37.8505778491347,-2.44754414582975,
117.690434762363));
#109939=CARTESIAN_POINT('Ctrl Pts',(37.7299864086294,-3.17042983055582,
117.703476486874));
#109940=CARTESIAN_POINT('Ctrl Pts',(37.3754127767892,-4.69161292819189,
117.747983257673));
#109941=CARTESIAN_POINT('Ctrl Pts',(37.1288750518075,-5.4849853461492,117.781610581606));
#109942=CARTESIAN_POINT('Ctrl Pts',(36.6543687488704,-6.69561257472272,
117.850284748281));
#109943=CARTESIAN_POINT('Ctrl Pts',(36.4645789815986,-7.12680305931145,
117.878476313845));
#109944=CARTESIAN_POINT('Ctrl Pts',(35.998595574586,-8.07733625586983,117.948838191852));
#109945=CARTESIAN_POINT('Ctrl Pts',(35.7129648268933,-8.59125722700539,
117.992670610368));
#109946=CARTESIAN_POINT('Ctrl Pts',(34.9601596152666,-9.79506354990021,
118.109288374321));
#109947=CARTESIAN_POINT('Ctrl Pts',(34.4680167975701,-10.4671064186872,
118.186325741409));
#109948=CARTESIAN_POINT('Ctrl Pts',(33.705247540462,-11.3628036701157,118.3069797176));
#109949=CARTESIAN_POINT('Ctrl Pts',(33.4733982350078,-11.6187942389264,
118.34380303707));
#109950=CARTESIAN_POINT('Ctrl Pts',(32.9244829807059,-12.1888654406497,
118.431436221565));
#109951=CARTESIAN_POINT('Ctrl Pts',(32.6025707023191,-12.4977728391668,
118.483182864766));
#109952=CARTESIAN_POINT('Ctrl Pts',(31.8279519028623,-13.184307498477,118.608177692849));
#109953=CARTESIAN_POINT('Ctrl Pts',(31.3670494630096,-13.5515373741682,
118.682876301331));
#109954=CARTESIAN_POINT('Ctrl Pts',(30.2678209441983,-14.3366710872971,
118.861301853471));
#109955=CARTESIAN_POINT('Ctrl Pts',(29.6185613468078,-14.7366042885872,
118.966860616838));
#109956=CARTESIAN_POINT('Ctrl Pts',(28.6050470860586,-15.2692166691634,
119.132039055448));
#109957=CARTESIAN_POINT('Ctrl Pts',(28.2593100844575,-15.4359608484853,
119.188460202513));
#109958=CARTESIAN_POINT('Ctrl Pts',(27.2632907286753,-15.8746670555202,
119.351402760385));
#109959=CARTESIAN_POINT('Ctrl Pts',(26.6014253488124,-16.1173823843318,
119.460260186855));
#109960=CARTESIAN_POINT('Ctrl Pts',(25.2629728430788,-16.5138257147529,
119.680526481603));
#109961=CARTESIAN_POINT('Ctrl Pts',(24.5881053523096,-16.6686070365398,
119.791627848937));
#109962=CARTESIAN_POINT('Ctrl Pts',(23.1047903648245,-16.9123829267381,
120.035588552737));
#109963=CARTESIAN_POINT('Ctrl Pts',(22.2954612659473,-16.9849535060156,
120.168537177851));
#109964=CARTESIAN_POINT('Ctrl Pts',(20.7767940116893,-17.0091783921386,
120.418590169224));
#109965=CARTESIAN_POINT('Ctrl Pts',(20.0694661877503,-16.9751003325265,
120.535428990361));
#109966=CARTESIAN_POINT('Ctrl Pts',(18.6818127374102,-16.8187217732458,
120.764362358282));
#109967=CARTESIAN_POINT('Ctrl Pts',(18.0025818287076,-16.6989230056301,
120.876265683671));
#109968=CARTESIAN_POINT('Ctrl Pts',(16.55159241383,-16.3486215821669,121.114669651962));
#109969=CARTESIAN_POINT('Ctrl Pts',(15.7849805428881,-16.1035399671801,
121.240201911816));
#109970=CARTESIAN_POINT('Ctrl Pts',(14.4169345960471,-15.5541003951089,
121.464257992389));
#109971=CARTESIAN_POINT('Ctrl Pts',(13.8105395415181,-15.2669658625495,
121.563710072064));
#109972=CARTESIAN_POINT('Ctrl Pts',(12.6025112117024,-14.6031918160419,
121.761218343765));
#109973=CARTESIAN_POINT('Ctrl Pts',(12.0041572769462,-14.2231713457374,
121.858679413648));
#109974=CARTESIAN_POINT('Ctrl Pts',(10.762564819961,-13.3196002833448,122.059728813854));
#109975=CARTESIAN_POINT('Ctrl Pts',(10.1301410017152,-12.7839116009468,
122.161343974529));
#109976=CARTESIAN_POINT('Ctrl Pts',(9.03574689592426,-11.7091384543426,
122.336537673811));
#109977=CARTESIAN_POINT('Ctrl Pts',(8.56351023550782,-11.1834393583186,
122.411998858786));
#109978=CARTESIAN_POINT('Ctrl Pts',(7.69225645978352,-10.082607814245,122.549928097048));
#109979=CARTESIAN_POINT('Ctrl Pts',(7.29319076719589,-9.50926708152108,
122.61240366853));
#109980=CARTESIAN_POINT('Ctrl Pts',(6.5087410661157,-8.22039708219152,122.733256775656));
#109981=CARTESIAN_POINT('Ctrl Pts',(6.1368128910113,-7.49846994060657,122.789202773831));
#109982=CARTESIAN_POINT('Ctrl Pts',(5.63207897067354,-6.32022659135211,
122.863416122778));
#109983=CARTESIAN_POINT('Ctrl Pts',(5.46472899018517,-5.88044523697474,
122.887659451084));
#109984=CARTESIAN_POINT('Ctrl Pts',(5.12891853630154,-4.87575600939705,
122.93507439902));
#109985=CARTESIAN_POINT('Ctrl Pts',(4.97098785085551,-4.30787607249436,
122.956387598468));
#109986=CARTESIAN_POINT('Ctrl Pts',(4.66050378214033,-2.91954573294833,
122.995029007191));
#109987=CARTESIAN_POINT('Ctrl Pts',(4.53772711179818,-2.09385284645138,
123.00695774643));
#109988=CARTESIAN_POINT('Ctrl Pts',(4.4489132903695,-0.915098142296885,
123.008781287776));
#109989=CARTESIAN_POINT('Ctrl Pts',(4.43326164955744,-0.566998360719908,
123.007469667049));
#109990=CARTESIAN_POINT('Ctrl Pts',(4.42709678199761,-0.145783148343236,
123.003712137728));
#109991=CARTESIAN_POINT('Ctrl Pts',(4.42649227748553,-0.0728888749453103,
123.002983391098));
#109992=CARTESIAN_POINT('Ctrl Pts',(4.42635006251054,-1.39861311574705E-8,
123.002176850242));
#109993=CARTESIAN_POINT('Origin',(20.412052742069,1.37771738462078E-14,
115.762503617193));
#109994=CARTESIAN_POINT('',(4.21797224931213,-7.48108295635842E-9,121.820407546638));
#109995=CARTESIAN_POINT('',(4.268747604916,3.20880881083766E-8,122.108368897758));
#109996=CARTESIAN_POINT('',(3.67032094086137,1.16952742876573E-14,118.71452263753));
#109997=CARTESIAN_POINT('Ctrl Pts',(4.26874760497861,3.20921647476068E-8,
122.108368898113));
#109998=CARTESIAN_POINT('Ctrl Pts',(4.26922578105566,-0.245077937043624,
122.11108077207));
#109999=CARTESIAN_POINT('Ctrl Pts',(4.27491609622479,-0.490145535982509,
122.112832525391));
#110000=CARTESIAN_POINT('Ctrl Pts',(4.31460988481392,-1.38148983558192,
122.115800970694));
#110001=CARTESIAN_POINT('Ctrl Pts',(4.37970572076675,-2.02582311938549,
122.111446643934));
#110002=CARTESIAN_POINT('Ctrl Pts',(4.65258566839347,-3.75010336431689,
122.082974676197));
#110003=CARTESIAN_POINT('Ctrl Pts',(4.92763931498512,-4.81606470696867,
122.04738051702));
#110004=CARTESIAN_POINT('Ctrl Pts',(5.43041779136617,-6.20151981287087,
121.97589295334));
#110005=CARTESIAN_POINT('Ctrl Pts',(5.5703177277972,-6.55083984830884,121.955550379125));
#110006=CARTESIAN_POINT('Ctrl Pts',(5.90317041322273,-7.30887149178157,
121.90619135937));
#110007=CARTESIAN_POINT('Ctrl Pts',(6.10100653230635,-7.71506902449926,
121.876314022122));
#110008=CARTESIAN_POINT('Ctrl Pts',(6.65087384397907,-8.73909267470954,
121.792330168304));
#110009=CARTESIAN_POINT('Ctrl Pts',(7.02564035484147,-9.34337611439463,
121.734271880608));
#110010=CARTESIAN_POINT('Ctrl Pts',(7.79730458877285,-10.4297829004104,
121.613652762633));
#110011=CARTESIAN_POINT('Ctrl Pts',(8.18525864543109,-10.9169706484482,
121.552603236519));
#110012=CARTESIAN_POINT('Ctrl Pts',(8.8764010067179,-11.6932848732858,121.442933199805));
#110013=CARTESIAN_POINT('Ctrl Pts',(9.16532811656547,-11.9946348163095,
121.39683388151));
#110014=CARTESIAN_POINT('Ctrl Pts',(9.76188543663381,-12.572499963897,121.301060850977));
#110015=CARTESIAN_POINT('Ctrl Pts',(10.069131949181,-12.8490141287323,121.251492205614));
#110016=CARTESIAN_POINT('Ctrl Pts',(10.9409499914763,-13.5774709358778,
121.110486537189));
#110017=CARTESIAN_POINT('Ctrl Pts',(11.5246262249861,-14.004498412734,121.015729503029));
#110018=CARTESIAN_POINT('Ctrl Pts',(12.6325232329256,-14.7100638358718,
120.835630921363));
#110019=CARTESIAN_POINT('Ctrl Pts',(13.147691806078,-15.0010010569616,120.751792961646));
#110020=CARTESIAN_POINT('Ctrl Pts',(14.0999968181132,-15.474074229105,120.596432063886));
#110021=CARTESIAN_POINT('Ctrl Pts',(14.531661680017,-15.6661218708745,120.52585381895));
#110022=CARTESIAN_POINT('Ctrl Pts',(15.3543879492404,-15.9910375019631,
120.390871062148));
#110023=CARTESIAN_POINT('Ctrl Pts',(15.7434360335537,-16.1282026394312,
120.32689518932));
#110024=CARTESIAN_POINT('Ctrl Pts',(16.8214329581016,-16.4637383442564,
120.149525212716));
#110025=CARTESIAN_POINT('Ctrl Pts',(17.5185404773362,-16.6321392771732,
120.03474102879));
#110026=CARTESIAN_POINT('Ctrl Pts',(18.8049764836848,-16.8559396958193,
119.823140172198));
#110027=CARTESIAN_POINT('Ctrl Pts',(19.390668969565,-16.9259000800183,119.726874316849));
#110028=CARTESIAN_POINT('Ctrl Pts',(20.4118125445504,-16.9928945734978,
119.558947212145));
#110029=CARTESIAN_POINT('Ctrl Pts',(20.8457800227687,-17.0042675743559,
119.487541600333));
#110030=CARTESIAN_POINT('Ctrl Pts',(21.6238500200444,-16.9940616799006,
119.35927191314));
#110031=CARTESIAN_POINT('Ctrl Pts',(21.967798567634,-16.9788123479304,119.302505055594));
#110032=CARTESIAN_POINT('Ctrl Pts',(23.1306430468139,-16.8908558569782,
119.110594309425));
#110033=CARTESIAN_POINT('Ctrl Pts',(23.9446521586234,-16.7678978870977,
118.97632734953));
#110034=CARTESIAN_POINT('Ctrl Pts',(25.314065606752,-16.4555105804068,118.751214710938));
#110035=CARTESIAN_POINT('Ctrl Pts',(25.8745803394607,-16.2962279601715,
118.659284895716));
#110036=CARTESIAN_POINT('Ctrl Pts',(26.8658954554874,-15.9573061992548,
118.496882056151));
#110037=CARTESIAN_POINT('Ctrl Pts',(27.2996362454932,-15.7883920250589,
118.425874689034));
#110038=CARTESIAN_POINT('Ctrl Pts',(28.4787023790733,-15.2713218021169,
118.232687005525));
#110039=CARTESIAN_POINT('Ctrl Pts',(29.206605539129,-14.8856848318245,118.113421928544));
#110040=CARTESIAN_POINT('Ctrl Pts',(30.5197274065888,-14.060748716363,117.899547151737));
#110041=CARTESIAN_POINT('Ctrl Pts',(31.1102978616076,-13.6338377179082,
117.803901028091));
#110042=CARTESIAN_POINT('Ctrl Pts',(32.1796635484378,-12.7497983493209,
117.631699377159));
#110043=CARTESIAN_POINT('Ctrl Pts',(32.6628294720299,-12.3002285959972,
117.55431497686));
#110044=CARTESIAN_POINT('Ctrl Pts',(33.6874534434968,-11.2283228924822,
117.390498614205));
#110045=CARTESIAN_POINT('Ctrl Pts',(34.2124853699605,-10.5921788479245,
117.306960192879));
#110046=CARTESIAN_POINT('Ctrl Pts',(35.1016834115052,-9.33977052382531,
117.167549589658));
#110047=CARTESIAN_POINT('Ctrl Pts',(35.4771486772781,-8.73400707182166,
117.109583065626));
#110048=CARTESIAN_POINT('Ctrl Pts',(36.1340523610338,-7.50959849603877,
117.010027222943));
#110049=CARTESIAN_POINT('Ctrl Pts',(36.4186544895027,-6.89419357669269,
116.967833746061));
#110050=CARTESIAN_POINT('Ctrl Pts',(36.9682105400366,-5.49355860504427,
116.887964031573));
#110051=CARTESIAN_POINT('Ctrl Pts',(37.2143795904827,-4.70261592559153,
116.853606363927));
#110052=CARTESIAN_POINT('Ctrl Pts',(37.567202504456,-3.19414006987481,116.808877021735));
#110053=CARTESIAN_POINT('Ctrl Pts',(37.6873336021067,-2.4817292229359,116.796031434694));
#110054=CARTESIAN_POINT('Ctrl Pts',(37.8311967659277,-1.10824752902771,
116.786815832772));
#110055=CARTESIAN_POINT('Ctrl Pts',(37.8622688870937,-0.44924647811183,
116.789102921073));
#110056=CARTESIAN_POINT('Ctrl Pts',(37.8520046164646,0.555001953746123,
116.802283320546));
#110057=CARTESIAN_POINT('Ctrl Pts',(37.8381133692295,0.899951732173469,
116.80857402443));
#110058=CARTESIAN_POINT('Ctrl Pts',(37.7550577179883,2.08029606342998,116.836369510181));
#110059=CARTESIAN_POINT('Ctrl Pts',(37.6354043097739,2.91069438385204,116.866788158877));
#110060=CARTESIAN_POINT('Ctrl Pts',(37.3299675200659,4.30300537692423,116.937048493882));
#110061=CARTESIAN_POINT('Ctrl Pts',(37.1746842275698,4.87030139368984,116.971323685906));
#110062=CARTESIAN_POINT('Ctrl Pts',(36.8428324157756,5.8767783994531,117.042254530924));
#110063=CARTESIAN_POINT('Ctrl Pts',(36.6765399127249,6.31884390923729,117.07708173275));
#110064=CARTESIAN_POINT('Ctrl Pts',(36.1698548571281,7.51332556017059,117.181134700329));
#110065=CARTESIAN_POINT('Ctrl Pts',(35.7931167136252,8.24834462327949,117.256616361301));
#110066=CARTESIAN_POINT('Ctrl Pts',(34.9891371451983,9.57113961632986,117.415936297328));
#110067=CARTESIAN_POINT('Ctrl Pts',(34.5743914697279,10.1645922131245,117.497477088718));
#110068=CARTESIAN_POINT('Ctrl Pts',(33.7111835169657,11.2453580826172,117.665982715174));
#110069=CARTESIAN_POINT('Ctrl Pts',(33.2693802063037,11.7364807138392,117.751719889345));
#110070=CARTESIAN_POINT('Ctrl Pts',(32.5451259901296,12.452103837052,117.891042111501));
#110071=CARTESIAN_POINT('Ctrl Pts',(32.282060619084,12.695883451979,117.941450752898));
#110072=CARTESIAN_POINT('Ctrl Pts',(31.4047118389416,13.4581411858243,118.109194059376));
#110073=CARTESIAN_POINT('Ctrl Pts',(30.7614749911917,13.9404113350938,118.231661276034));
#110074=CARTESIAN_POINT('Ctrl Pts',(29.5955081108851,14.6898098144848,118.45339165233));
#110075=CARTESIAN_POINT('Ctrl Pts',(29.0883285852308,14.9792760205531,118.549749775195));
#110076=CARTESIAN_POINT('Ctrl Pts',(28.1580964293806,15.4470237411149,118.726118052834));
#110077=CARTESIAN_POINT('Ctrl Pts',(27.7407221329023,15.635640853154,118.805112556122));
#110078=CARTESIAN_POINT('Ctrl Pts',(26.5570474418163,16.1124324319238,119.02846759665));
#110079=CARTESIAN_POINT('Ctrl Pts',(25.7767468246243,16.361193587035,119.175136230472));
#110080=CARTESIAN_POINT('Ctrl Pts',(24.2798199157637,16.7184022161233,119.45673831598));
#110081=CARTESIAN_POINT('Ctrl Pts',(23.5680137179802,16.8394956152179,119.590728982892));
#110082=CARTESIAN_POINT('Ctrl Pts',(22.2008319538071,16.9804246455505,119.848158649967));
#110083=CARTESIAN_POINT('Ctrl Pts',(21.5475966526756,17.0085771131263,119.971162418197));
#110084=CARTESIAN_POINT('Ctrl Pts',(20.0808846288693,16.9842460025931,120.246643619123));
#110085=CARTESIAN_POINT('Ctrl Pts',(19.2694064281265,16.9103191445245,120.398766621102));
#110086=CARTESIAN_POINT('Ctrl Pts',(17.7739648420178,16.6611601615662,120.679827743417));
#110087=CARTESIAN_POINT('Ctrl Pts',(17.0892911480912,16.5014931290457,120.808789070103));
#110088=CARTESIAN_POINT('Ctrl Pts',(15.7765516085603,16.1053733008256,121.056538377752));
#110089=CARTESIAN_POINT('Ctrl Pts',(15.1485226021275,15.8733867766072,121.175273743084));
#110090=CARTESIAN_POINT('Ctrl Pts',(13.8024410870976,15.2811026726017,121.429494432319));
#110091=CARTESIAN_POINT('Ctrl Pts',(13.0927751535077,14.9053001636955,121.563517158405));
#110092=CARTESIAN_POINT('Ctrl Pts',(11.8280975477732,14.1134251875143,121.803548531652));
#110093=CARTESIAN_POINT('Ctrl Pts',(11.2666051199481,13.7112976507818,121.910601620428));
#110094=CARTESIAN_POINT('Ctrl Pts',(10.1814656425597,12.8275657510704,122.118473609818));
#110095=CARTESIAN_POINT('Ctrl Pts',(9.66028068805985,12.3450280691722,122.218829316659));
#110096=CARTESIAN_POINT('Ctrl Pts',(8.6145489160732,11.2461578048294,122.420511876081));
#110097=CARTESIAN_POINT('Ctrl Pts',(8.10049093622967,10.6219759350091,122.520039818756));
#110098=CARTESIAN_POINT('Ctrl Pts',(7.2356298339529,9.40367904704014,122.689465305852));
#110099=CARTESIAN_POINT('Ctrl Pts',(6.87269184362794,8.82055580199039,122.761399387814));
#110100=CARTESIAN_POINT('Ctrl Pts',(6.19453999831229,7.56803599931309,122.897674388497));
#110101=CARTESIAN_POINT('Ctrl Pts',(5.88553989068536,6.8967812321402,122.9608959521));
#110102=CARTESIAN_POINT('Ctrl Pts',(5.47759320660585,5.83489147349971,123.045699215811));
#110103=CARTESIAN_POINT('Ctrl Pts',(5.34756315637579,5.4576450533461,123.073061755979));
#110104=CARTESIAN_POINT('Ctrl Pts',(5.01152414200896,4.35990681645709,123.145103436831));
#110105=CARTESIAN_POINT('Ctrl Pts',(4.83924298210524,3.6296981447072,123.183881045035));
#110106=CARTESIAN_POINT('Ctrl Pts',(4.61666920953987,2.30411464104747,123.238613832434));
#110107=CARTESIAN_POINT('Ctrl Pts',(4.54863964978615,1.71309618313185,123.257586231491));
#110108=CARTESIAN_POINT('Ctrl Pts',(4.48777356302406,0.746898958496295,
123.279645302893));
#110109=CARTESIAN_POINT('Ctrl Pts',(4.47639669214102,0.37349133505058,123.286005389121));
#110110=CARTESIAN_POINT('Ctrl Pts',(4.47712541821256,1.48397781563059E-8,
123.290138201919));
#110111=CARTESIAN_POINT('Ctrl Pts',(4.42635006251054,-1.39861311574705E-8,
123.002176850242));
#110112=CARTESIAN_POINT('Ctrl Pts',(4.42518823885667,0.595464723605533,
122.995587823697));
#110113=CARTESIAN_POINT('Ctrl Pts',(4.45487722577497,1.19056805989309,122.983791647929));
#110114=CARTESIAN_POINT('Ctrl Pts',(4.58800175956766,2.49647221385867,122.945715111161));
#110115=CARTESIAN_POINT('Ctrl Pts',(4.70515673536992,3.20461407594884,122.916989531995));
#110116=CARTESIAN_POINT('Ctrl Pts',(5.05108720935585,4.70682566645807,122.838191577909));
#110117=CARTESIAN_POINT('Ctrl Pts',(5.29357530148929,5.49573681876531,122.785643279264));
#110118=CARTESIAN_POINT('Ctrl Pts',(5.83642561318191,6.89417724721876,122.672604724397));
#110119=CARTESIAN_POINT('Ctrl Pts',(6.11826003702824,7.50933148956035,122.615429588997));
#110120=CARTESIAN_POINT('Ctrl Pts',(6.76961792463418,8.73362924750353,122.485072826534));
#110121=CARTESIAN_POINT('Ctrl Pts',(7.14234934471908,9.33950362308899,122.411308921857));
#110122=CARTESIAN_POINT('Ctrl Pts',(8.02891881487089,10.5967482036702,122.237110984286));
#110123=CARTESIAN_POINT('Ctrl Pts',(8.55472085039083,11.2371107144602,122.134500999833));
#110124=CARTESIAN_POINT('Ctrl Pts',(9.60990963140838,12.3450429607679,121.930669263089));
#110125=CARTESIAN_POINT('Ctrl Pts',(10.1261191608978,12.8230593294005,121.831843143575));
#110126=CARTESIAN_POINT('Ctrl Pts',(11.2074112670327,13.7049681910703,121.625487493729));
#110127=CARTESIAN_POINT('Ctrl Pts',(11.7707534210822,14.1088796990682,121.518263708808));
#110128=CARTESIAN_POINT('Ctrl Pts',(13.0372380170141,14.9025317613241,121.277479187999));
#110129=CARTESIAN_POINT('Ctrl Pts',(13.7466757175853,15.2785897683167,121.142749461357));
#110130=CARTESIAN_POINT('Ctrl Pts',(14.9025577128908,15.7876715404586,120.9241762995));
#110131=CARTESIAN_POINT('Ctrl Pts',(15.3326185914562,15.9559470883754,120.843104847876));
#110132=CARTESIAN_POINT('Ctrl Pts',(16.3184072501254,16.2947699017502,120.657503523335));
#110133=CARTESIAN_POINT('Ctrl Pts',(16.8771500368237,16.4543775322675,120.552440811145));
#110134=CARTESIAN_POINT('Ctrl Pts',(18.2365561266768,16.7660811102088,120.296695924692));
#110135=CARTESIAN_POINT('Ctrl Pts',(19.0421840745574,16.8888366537347,120.144994671488));
#110136=CARTESIAN_POINT('Ctrl Pts',(20.1985621184983,16.9780071879278,119.927280061992));
#110137=CARTESIAN_POINT('Ctrl Pts',(20.5444717051969,16.9937026550759,119.86216880481));
#110138=CARTESIAN_POINT('Ctrl Pts',(21.5583159176972,17.0076175455186,119.671532332386));
#110139=CARTESIAN_POINT('Ctrl Pts',(22.226005753672,16.9760474101932,119.546321070406));
#110140=CARTESIAN_POINT('Ctrl Pts',(23.5866935336157,16.8282317911089,119.290910042905));
#110141=CARTESIAN_POINT('Ctrl Pts',(24.2779701576123,16.7080446167473,119.161001259895));
#110142=CARTESIAN_POINT('Ctrl Pts',(25.7471798827798,16.354662299431,118.88422038468));
#110143=CARTESIAN_POINT('Ctrl Pts',(26.5199871827589,16.107304431488,118.738192946537));
#110144=CARTESIAN_POINT('Ctrl Pts',(27.8915679713764,15.5541093609196,118.479060318859));
#110145=CARTESIAN_POINT('Ctrl Pts',(28.4957815409686,15.2667869647624,118.365044885245));
#110146=CARTESIAN_POINT('Ctrl Pts',(29.6986816465838,14.6028370891587,118.137438674895));
#110147=CARTESIAN_POINT('Ctrl Pts',(30.2941171099273,14.2228940492812,118.024404403553));
#110148=CARTESIAN_POINT('Ctrl Pts',(31.5248025858741,13.3227936279907,117.789593515893));
#110149=CARTESIAN_POINT('Ctrl Pts',(32.1497105993425,12.7911564093607,117.669578676146));
#110150=CARTESIAN_POINT('Ctrl Pts',(33.2017300678859,11.7543133945301,117.466902307042));
#110151=CARTESIAN_POINT('Ctrl Pts',(33.642545181654,11.2658923909258,117.381860926172));
#110152=CARTESIAN_POINT('Ctrl Pts',(34.5105334763716,10.1832532918875,117.213274495814));
#110153=CARTESIAN_POINT('Ctrl Pts',(34.930075761167,9.58445085798915,117.131046945627));
#110154=CARTESIAN_POINT('Ctrl Pts',(35.7382201691088,8.2562273634107,116.970531287632));
#110155=CARTESIAN_POINT('Ctrl Pts',(36.115098400205,7.52164509304977,116.894262589128));
#110156=CARTESIAN_POINT('Ctrl Pts',(36.7090499882621,6.12346260200393,116.77197805045));
#110157=CARTESIAN_POINT('Ctrl Pts',(36.9414830724226,5.46854639923365,116.723325208009));
#110158=CARTESIAN_POINT('Ctrl Pts',(37.3290081942046,4.12266167533976,116.639371904947));
#110159=CARTESIAN_POINT('Ctrl Pts',(37.4824241879757,3.43260171775824,116.604356477421));
#110160=CARTESIAN_POINT('Ctrl Pts',(37.7227204437875,1.91667604733677,116.54425048954));
#110161=CARTESIAN_POINT('Ctrl Pts',(37.7932539849284,1.0899329692338,116.521975019881));
#110162=CARTESIAN_POINT('Ctrl Pts',(37.8135153901447,-0.449614347336989,
116.500670877354));
#110163=CARTESIAN_POINT('Ctrl Pts',(37.7790188154657,-1.16036323419767,
116.498936940417));
#110164=CARTESIAN_POINT('Ctrl Pts',(37.623719464608,-2.56296318541711,116.510617543849));
#110165=CARTESIAN_POINT('Ctrl Pts',(37.5043513905107,-3.25359763791229,
116.523778424962));
#110166=CARTESIAN_POINT('Ctrl Pts',(37.1564999871574,-4.72543705329675,
116.567654538254));
#110167=CARTESIAN_POINT('Ctrl Pts',(36.9140292009834,-5.50149868860622,
116.600777237718));
#110168=CARTESIAN_POINT('Ctrl Pts',(36.4460644223716,-6.69541860127829,
116.668504892631));
#110169=CARTESIAN_POINT('Ctrl Pts',(36.2564019608999,-7.1263439271623,116.696677210133));
#110170=CARTESIAN_POINT('Ctrl Pts',(35.7905552454678,-8.07670967684446,
116.767017281745));
#110171=CARTESIAN_POINT('Ctrl Pts',(35.504904359474,-8.5907143095185,116.810852414028));
#110172=CARTESIAN_POINT('Ctrl Pts',(34.7524148658142,-9.79410140326056,
116.927420623407));
#110173=CARTESIAN_POINT('Ctrl Pts',(34.2606879220935,-10.4656966310228,
117.004392176695));
#110174=CARTESIAN_POINT('Ctrl Pts',(33.4981693682653,-11.3613513360252,
117.125004150784));
#110175=CARTESIAN_POINT('Ctrl Pts',(33.2660724455843,-11.6176682910296,
117.161866203193));
#110176=CARTESIAN_POINT('Ctrl Pts',(32.7177335663459,-12.1872171454491,
117.249406404016));
#110177=CARTESIAN_POINT('Ctrl Pts',(32.3967281981065,-12.4953602506554,
117.301005833612));
#110178=CARTESIAN_POINT('Ctrl Pts',(31.6227921700325,-13.1816730404354,
117.425887298958));
#110179=CARTESIAN_POINT('Ctrl Pts',(31.1615657934469,-13.549335617007,117.500637689857));
#110180=CARTESIAN_POINT('Ctrl Pts',(30.0691559510562,-14.3299050013909,
117.677955381894));
#110181=CARTESIAN_POINT('Ctrl Pts',(29.4277185931807,-14.7258749417959,
117.782241291571));
#110182=CARTESIAN_POINT('Ctrl Pts',(28.4178969084008,-15.2588015226943,
117.946806360488));
#110183=CARTESIAN_POINT('Ctrl Pts',(28.0673504512446,-15.4284053136147,
118.004008162687));
#110184=CARTESIAN_POINT('Ctrl Pts',(27.0546732857834,-15.8753556275927,
118.169666944165));
#110185=CARTESIAN_POINT('Ctrl Pts',(26.3804775649806,-16.1222727430435,
118.280557649367));
#110186=CARTESIAN_POINT('Ctrl Pts',(25.0337183560893,-16.5188477748547,
118.502194647031));
#110187=CARTESIAN_POINT('Ctrl Pts',(24.3635262076723,-16.671750021719,118.61252396392));
#110188=CARTESIAN_POINT('Ctrl Pts',(22.8946307203057,-16.9121059059674,
118.854111373357));
#110189=CARTESIAN_POINT('Ctrl Pts',(22.0951339373954,-16.9839494300226,
118.985447737349));
#110190=CARTESIAN_POINT('Ctrl Pts',(20.5695232625194,-17.0099335780774,
119.236633819618));
#110191=CARTESIAN_POINT('Ctrl Pts',(19.8454000325533,-16.9747275626374,
119.35625195382));
#110192=CARTESIAN_POINT('Ctrl Pts',(18.4472366962676,-16.8143918726589,
119.58691123482));
#110193=CARTESIAN_POINT('Ctrl Pts',(17.774006315727,-16.6946639187595,119.697818708374));
#110194=CARTESIAN_POINT('Ctrl Pts',(16.3288919004593,-16.3444236125222,
119.935249124945));
#110195=CARTESIAN_POINT('Ctrl Pts',(15.5623250163285,-16.0985937302408,
120.060769943235));
#110196=CARTESIAN_POINT('Ctrl Pts',(14.4103913286245,-15.6347218299559,
120.249433175712));
#110197=CARTESIAN_POINT('Ctrl Pts',(14.0111484769824,-15.4553678980557,
120.314879599975));
#110198=CARTESIAN_POINT('Ctrl Pts',(12.9309599351056,-14.9180868301962,
120.491774242061));
#110199=CARTESIAN_POINT('Ctrl Pts',(12.2665926131983,-14.5283273120543,
120.600309544538));
#110200=CARTESIAN_POINT('Ctrl Pts',(11.1709308024953,-13.7797306432325,
120.778200256408));
#110201=CARTESIAN_POINT('Ctrl Pts',(10.7267032987619,-13.4426600147459,
120.849987117073));
#110202=CARTESIAN_POINT('Ctrl Pts',(9.83461053574349,-12.6931677986486,
120.993545212399));
#110203=CARTESIAN_POINT('Ctrl Pts',(9.39061182533935,-12.2772483278458,
121.064650320127));
#110204=CARTESIAN_POINT('Ctrl Pts',(8.41027111392335,-11.2541508344559,
121.221396334212));
#110205=CARTESIAN_POINT('Ctrl Pts',(7.89287333866819,-10.6304032098477,
121.30374416078));
#110206=CARTESIAN_POINT('Ctrl Pts',(7.02372265835108,-9.41584385666745,
121.440119166576));
#110207=CARTESIAN_POINT('Ctrl Pts',(6.65952050852146,-8.83628073833126,
121.49644641522));
#110208=CARTESIAN_POINT('Ctrl Pts',(5.97069636036473,-7.57855377714445,
121.60112800413));
#110209=CARTESIAN_POINT('Ctrl Pts',(5.65392176226136,-6.89763556146838,
121.648117648005));
#110210=CARTESIAN_POINT('Ctrl Pts',(5.23660743187802,-5.82109881654923,
121.708659428415));
#110211=CARTESIAN_POINT('Ctrl Pts',(5.10389172906911,-5.43928253380061,
121.727575231636));
#110212=CARTESIAN_POINT('Ctrl Pts',(4.76567825046675,-4.34321696884615,
121.774446822623));
#110213=CARTESIAN_POINT('Ctrl Pts',(4.59272480727977,-3.61965369280211,
121.796617516938));
#110214=CARTESIAN_POINT('Ctrl Pts',(4.36618777270672,-2.30033662389662,
121.821147845938));
#110215=CARTESIAN_POINT('Ctrl Pts',(4.29584625684108,-1.70874879397981,
121.826567012219));
#110216=CARTESIAN_POINT('Ctrl Pts',(4.23145416377887,-0.743617261714217,
121.826607423141));
#110217=CARTESIAN_POINT('Ctrl Pts',(4.21869777333078,-0.371849869633078,
121.824522195929));
#110218=CARTESIAN_POINT('Ctrl Pts',(4.21797224931213,-1.49621590811444E-8,
121.820407546637));
#110219=CARTESIAN_POINT('Origin',(20.412052742069,1.37771738462078E-14,
115.762503617193));
#110220=CARTESIAN_POINT('',(4.00959443613148,-1.25155352558489E-8,120.638638243134));
#110221=CARTESIAN_POINT('',(4.06036979181168,7.51633154241203E-9,120.926599594688));
#110222=CARTESIAN_POINT('',(3.67032094086137,1.16952742876573E-14,118.71452263753));
#110223=CARTESIAN_POINT('Ctrl Pts',(4.06036979181167,1.50326513895498E-8,
120.926599594688));
#110224=CARTESIAN_POINT('Ctrl Pts',(4.06109544462189,-0.371916179869893,
120.930714978172));
#110225=CARTESIAN_POINT('Ctrl Pts',(4.07382447319043,-0.743751311529452,
120.93261993144));
#110226=CARTESIAN_POINT('Ctrl Pts',(4.13813558699207,-1.70892963326076,
120.932035879093));
#110227=CARTESIAN_POINT('Ctrl Pts',(4.20841260663817,-2.30049309592992,
120.926232593849));
#110228=CARTESIAN_POINT('Ctrl Pts',(4.43495233645074,-3.62005035895633,
120.901417407863));
#110229=CARTESIAN_POINT('Ctrl Pts',(4.60804054799553,-4.34386905761117,
120.879516002255));
#110230=CARTESIAN_POINT('Ctrl Pts',(4.94644995248541,-5.43999188903374,
120.833272837139));
#110231=CARTESIAN_POINT('Ctrl Pts',(5.07916398511592,-5.82163057348125,
120.814611024077));
#110232=CARTESIAN_POINT('Ctrl Pts',(5.49633802576137,-6.89760324021201,
120.754383332977));
#110233=CARTESIAN_POINT('Ctrl Pts',(5.8128239647134,-7.57814692831025,120.706838878165));
#110234=CARTESIAN_POINT('Ctrl Pts',(6.5013318175681,-8.83567939597569,120.601457736364));
#110235=CARTESIAN_POINT('Ctrl Pts',(6.86556315951656,-9.41537576858684,
120.544981836645));
#110236=CARTESIAN_POINT('Ctrl Pts',(7.73468917633917,-10.6298566517034,
120.409061807226));
#110237=CARTESIAN_POINT('Ctrl Pts',(8.25202139551287,-11.2534276399576,
120.327492256401));
#110238=CARTESIAN_POINT('Ctrl Pts',(9.29791710675212,-12.3450378068388,
120.160585238406));
#110239=CARTESIAN_POINT('Ctrl Pts',(9.8152613163429,-12.821693631004,120.07714587458));
#110240=CARTESIAN_POINT('Ctrl Pts',(10.9007270404882,-13.7030613063849,
119.901428864123));
#110241=CARTESIAN_POINT('Ctrl Pts',(11.467329392624,-14.1075182097664,119.809421046338));
#110242=CARTESIAN_POINT('Ctrl Pts',(12.7403827366668,-14.9017191458757,
119.60242520546));
#110243=CARTESIAN_POINT('Ctrl Pts',(13.4531005949596,-15.2778589958563,
119.486390672741));
#110244=CARTESIAN_POINT('Ctrl Pts',(14.6051338146059,-15.7831725684149,
119.297904325861));
#110245=CARTESIAN_POINT('Ctrl Pts',(15.0277996072462,-15.9483399326344,
119.228511323325));
#110246=CARTESIAN_POINT('Ctrl Pts',(16.0109712043684,-16.2869127197307,
119.066862362756));
#110247=CARTESIAN_POINT('Ctrl Pts',(16.5748809865819,-16.4482975056573,
118.974004987576));
#110248=CARTESIAN_POINT('Ctrl Pts',(17.8933528720093,-16.7511354713472,
118.757020040198));
#110249=CARTESIAN_POINT('Ctrl Pts',(18.6514828656597,-16.8706999705766,
118.632365084318));
#110250=CARTESIAN_POINT('Ctrl Pts',(19.7924944048013,-16.9702626993189,
118.444762699985));
#110251=CARTESIAN_POINT('Ctrl Pts',(20.1709676059958,-16.990232882454,118.382526683596));
#110252=CARTESIAN_POINT('Ctrl Pts',(21.2215668936329,-17.009557256875,118.209558102306));
#110253=CARTESIAN_POINT('Ctrl Pts',(21.8934232023662,-16.9810008623432,
118.098603337571));
#110254=CARTESIAN_POINT('Ctrl Pts',(23.2778320456319,-16.8374273796617,
117.870173739578));
#110255=CARTESIAN_POINT('Ctrl Pts',(23.9884331540669,-16.7165387172295,
117.753068684323));
#110256=CARTESIAN_POINT('Ctrl Pts',(25.4858427290076,-16.3601965710916,
117.507006115782));
#110257=CARTESIAN_POINT('Ctrl Pts',(26.2677773528003,-16.1118164769959,
117.378960611836));
#110258=CARTESIAN_POINT('Ctrl Pts',(27.461378990354,-15.6330692554134,117.183475500784));
#110259=CARTESIAN_POINT('Ctrl Pts',(27.8867428746152,-15.4413547639464,
117.113743690127));
#110260=CARTESIAN_POINT('Ctrl Pts',(28.824741496229,-14.9703264372935,116.960151234113));
#110261=CARTESIAN_POINT('Ctrl Pts',(29.3320277909594,-14.6814098934801,
116.877235529233));
#110262=CARTESIAN_POINT('Ctrl Pts',(30.5200234922694,-13.9200066850356,
116.683877814602));
#110263=CARTESIAN_POINT('Ctrl Pts',(31.1832239089646,-13.4222474326742,
116.576673304186));
#110264=CARTESIAN_POINT('Ctrl Pts',(32.0676524444043,-12.6502865281376,
116.434566029903));
#110265=CARTESIAN_POINT('Ctrl Pts',(32.320665559984,-12.4153959824999,116.394014288617));
#110266=CARTESIAN_POINT('Ctrl Pts',(32.883316441135,-11.8599741383261,116.303953678213));
#110267=CARTESIAN_POINT('Ctrl Pts',(33.1878999803028,-11.5345626300269,
116.255254336194));
#110268=CARTESIAN_POINT('Ctrl Pts',(33.8658480358207,-10.7504542905743,
116.147300651274));
#110269=CARTESIAN_POINT('Ctrl Pts',(34.2289019142407,-10.2833682469229,
116.089858873882));
#110270=CARTESIAN_POINT('Ctrl Pts',(35.0017255995861,-9.17446803628632,
115.968924223625));
#110271=CARTESIAN_POINT('Ctrl Pts',(35.3944932714994,-8.5220283295332,115.90852091134));
#110272=CARTESIAN_POINT('Ctrl Pts',(35.9215227012237,-7.49773719808307,
115.829097564491));
#110273=CARTESIAN_POINT('Ctrl Pts',(36.0883888348419,-7.14421732426023,
115.804260958309));
#110274=CARTESIAN_POINT('Ctrl Pts',(36.5078750567658,-6.17057397482726,
115.742535773449));
#110275=CARTESIAN_POINT('Ctrl Pts',(36.7365888964586,-5.54067853283166,
115.709610892267));
#110276=CARTESIAN_POINT('Ctrl Pts',(37.1364677050348,-4.20035394824862,
115.654676203586));
#110277=CARTESIAN_POINT('Ctrl Pts',(37.3003759135926,-3.48911486135417,
115.633973745358));
#110278=CARTESIAN_POINT('Ctrl Pts',(37.5549425128948,-1.94261459356428,
115.607174294891));
#110279=CARTESIAN_POINT('Ctrl Pts',(37.6306993636554,-1.10678654481858,
115.603764661473));
#110280=CARTESIAN_POINT('Ctrl Pts',(37.6580008868524,0.449255408351833,
115.616876542939));
#110281=CARTESIAN_POINT('Ctrl Pts',(37.6257113101545,1.16734086829877,115.630465228205));
#110282=CARTESIAN_POINT('Ctrl Pts',(37.474126663482,2.57441242725769,115.672949977547));
#110283=CARTESIAN_POINT('Ctrl Pts',(37.357498913966,3.2623082269617,115.701373413403));
#110284=CARTESIAN_POINT('Ctrl Pts',(37.0155854992617,4.73189528757101,115.779098184567));
#110285=CARTESIAN_POINT('Ctrl Pts',(36.775943788676,5.50834935822597,115.83099179919));
#110286=CARTESIAN_POINT('Ctrl Pts',(36.237928244285,6.89413317065628,115.943021002455));
#110287=CARTESIAN_POINT('Ctrl Pts',(35.9564756108636,7.50849876363283,116.000119389192));
#110288=CARTESIAN_POINT('Ctrl Pts',(35.3054756825945,8.73243132318426,116.130407331724));
#110289=CARTESIAN_POINT('Ctrl Pts',(34.932587025956,9.33865756381279,116.204202977392));
#110290=CARTESIAN_POINT('Ctrl Pts',(34.0490423119042,10.5917125048151,116.377807323092));
#110291=CARTESIAN_POINT('Ctrl Pts',(33.5271020059831,11.2280571996377,116.479667474439));
#110292=CARTESIAN_POINT('Ctrl Pts',(32.5096589584696,12.2985478687273,116.676235186642));
#110293=CARTESIAN_POINT('Ctrl Pts',(32.0307840403966,12.7467082442256,116.767975473656));
#110294=CARTESIAN_POINT('Ctrl Pts',(30.9676561601478,13.6308165559435,116.970966648253));
#110295=CARTESIAN_POINT('Ctrl Pts',(30.37874014994,14.0588335895466,117.083068264223));
#110296=CARTESIAN_POINT('Ctrl Pts',(29.0703325658575,14.8848513335703,117.331841683419));
#110297=CARTESIAN_POINT('Ctrl Pts',(28.3455828782913,15.270625341966,117.469490503562));
#110298=CARTESIAN_POINT('Ctrl Pts',(27.1820993001986,15.7831897086887,117.689502444031));
#110299=CARTESIAN_POINT('Ctrl Pts',(26.7611566381927,15.9483682206002,117.768860753313));
#110300=CARTESIAN_POINT('Ctrl Pts',(25.7819669730114,16.2869416279052,117.953229272502));
#110301=CARTESIAN_POINT('Ctrl Pts',(25.220316996997,16.4483197999396,118.058838323665));
#110302=CARTESIAN_POINT('Ctrl Pts',(23.9069281257681,16.7512015630847,118.30592400931));
#110303=CARTESIAN_POINT('Ctrl Pts',(23.1516496604424,16.8707831999228,118.448126679876));
#110304=CARTESIAN_POINT('Ctrl Pts',(22.0151939335348,16.9702998825412,118.662104273353));
#110305=CARTESIAN_POINT('Ctrl Pts',(21.6384049546807,16.9902495533383,118.733039571959));
#110306=CARTESIAN_POINT('Ctrl Pts',(20.5928773358012,17.0095363499679,118.929664362102));
#110307=CARTESIAN_POINT('Ctrl Pts',(19.9243161809923,16.9810415369076,119.055053500864));
#110308=CARTESIAN_POINT('Ctrl Pts',(18.545547260635,16.8376528902263,119.313843191662));
#110309=CARTESIAN_POINT('Ctrl Pts',(17.8373130342597,16.7167427401791,119.44692171617));
#110310=CARTESIAN_POINT('Ctrl Pts',(16.3453737444248,16.360291317995,119.727969834639));
#110311=CARTESIAN_POINT('Ctrl Pts',(15.5665580978345,16.1118423960987,119.875129810112));
#110312=CARTESIAN_POINT('Ctrl Pts',(14.37867728749,15.6333185454838,120.09955675401));
#110313=CARTESIAN_POINT('Ctrl Pts',(13.9559160325654,15.4420006776234,120.179362472352));
#110314=CARTESIAN_POINT('Ctrl Pts',(13.0224523267959,14.9713976198448,120.355752339874));
#110315=CARTESIAN_POINT('Ctrl Pts',(12.5171416344494,14.6824170858708,120.451387438507));
#110316=CARTESIAN_POINT('Ctrl Pts',(11.3360163783748,13.9220584206545,120.675749590544));
#110317=CARTESIAN_POINT('Ctrl Pts',(10.6775849076177,13.4256718427779,120.801559896098));
#110318=CARTESIAN_POINT('Ctrl Pts',(9.79803698539848,12.6545442361247,120.970481932679));
#110319=CARTESIAN_POINT('Ctrl Pts',(9.54537267352967,12.4188408271241,121.019110755335));
#110320=CARTESIAN_POINT('Ctrl Pts',(8.99077749930881,11.8685479042255,121.125969378757));
#110321=CARTESIAN_POINT('Ctrl Pts',(8.69335281993779,11.5496063558978,121.183328850132));
#110322=CARTESIAN_POINT('Ctrl Pts',(8.02140865543179,10.7705783759609,121.313342361084));
#110323=CARTESIAN_POINT('Ctrl Pts',(7.65793145009093,10.3014135595615,121.384041356307));
#110324=CARTESIAN_POINT('Ctrl Pts',(6.90864144572742,9.22154136682129,121.531101377255));
#110325=CARTESIAN_POINT('Ctrl Pts',(6.53551147681524,8.60315882163496,121.605289843067));
#110326=CARTESIAN_POINT('Ctrl Pts',(6.0107063838496,7.5935333625272,121.711189517807));
#110327=CARTESIAN_POINT('Ctrl Pts',(5.83242531068412,7.21760455240921,121.747521818373));
#110328=CARTESIAN_POINT('Ctrl Pts',(5.47996472507408,6.39852644682126,121.819998722905));
#110329=CARTESIAN_POINT('Ctrl Pts',(5.31015689405443,5.9538132267194,121.855290924592));
#110330=CARTESIAN_POINT('Ctrl Pts',(4.96974432108495,4.93727940226185,121.927274640659));
#110331=CARTESIAN_POINT('Ctrl Pts',(4.80995622911867,4.36236813765725,121.962064049053));
#110332=CARTESIAN_POINT('Ctrl Pts',(4.54038106457611,3.1514337907947,122.023640752274));
#110333=CARTESIAN_POINT('Ctrl Pts',(4.43579978837447,2.5151696095759,122.049525683068));
#110334=CARTESIAN_POINT('Ctrl Pts',(4.31712855678972,1.40853117727905,122.083462606372));
#110335=CARTESIAN_POINT('Ctrl Pts',(4.2861748988376,0.940781164514785,122.094433492682));
#110336=CARTESIAN_POINT('Ctrl Pts',(4.27028424358903,0.314887353539518,
122.104488267717));
#110337=CARTESIAN_POINT('Ctrl Pts',(4.26844041796647,0.157441553515873,
122.106626752285));
#110338=CARTESIAN_POINT('Ctrl Pts',(4.26874760497861,3.2092153691432E-8,
122.108368898113));
#110339=CARTESIAN_POINT('Ctrl Pts',(4.21797224931213,-1.49621579481794E-8,
121.820407546637));
#110340=CARTESIAN_POINT('Ctrl Pts',(4.21783007352557,0.0728687587915521,
121.819601228053));
#110341=CARTESIAN_POINT('Ctrl Pts',(4.21814991592475,0.145740700221469,
121.818717063283));
#110342=CARTESIAN_POINT('Ctrl Pts',(4.22266880094517,0.566906322356731,
121.813153004183));
#110343=CARTESIAN_POINT('Ctrl Pts',(4.23695833476989,0.914981990905322,
121.80675828228));
#110344=CARTESIAN_POINT('Ctrl Pts',(4.32115168954176,2.09375351741002,121.778779644602));
#110345=CARTESIAN_POINT('Ctrl Pts',(4.44068155455545,2.91947981692603,121.748430600617));
#110346=CARTESIAN_POINT('Ctrl Pts',(4.74561713539064,4.30783822857224,121.678302906396));
#110347=CARTESIAN_POINT('Ctrl Pts',(4.90124747141045,4.87571418267818,121.643958258756));
#110348=CARTESIAN_POINT('Ctrl Pts',(5.23292063371056,5.88041316543007,121.573079734022));
#110349=CARTESIAN_POINT('Ctrl Pts',(5.39843933003303,6.3202117767867,121.538417493381));
#110350=CARTESIAN_POINT('Ctrl Pts',(5.90493826090496,7.51442804791732,121.434400542965));
#110351=CARTESIAN_POINT('Ctrl Pts',(6.28271877495383,8.25124570795247,121.358712944208));
#110352=CARTESIAN_POINT('Ctrl Pts',(7.0903687141081,9.57914747154308,121.198672867327));
#110353=CARTESIAN_POINT('Ctrl Pts',(7.50793467658244,10.1757668092679,121.116583161096));
#110354=CARTESIAN_POINT('Ctrl Pts',(8.3754602350813,11.2595861350958,120.947254350687));
#110355=CARTESIAN_POINT('Ctrl Pts',(8.81842145140748,11.7508678075734,120.861306141922));
#110356=CARTESIAN_POINT('Ctrl Pts',(9.87127348920574,12.7886305633914,120.658803828637));
#110357=CARTESIAN_POINT('Ctrl Pts',(10.4943313434594,13.3188908012687,120.539927611143));
#110358=CARTESIAN_POINT('Ctrl Pts',(11.7188431948899,14.215372447492,120.306714107406));
#110359=CARTESIAN_POINT('Ctrl Pts',(12.3098477369955,14.5932889240075,120.194321988777));
#110360=CARTESIAN_POINT('Ctrl Pts',(13.517375790144,15.262027798887,119.965058414874));
#110361=CARTESIAN_POINT('Ctrl Pts',(14.1315804472529,15.5544121254239,119.848638715276));
#110362=CARTESIAN_POINT('Ctrl Pts',(15.516280524145,16.1118115997861,119.587354466938));
#110363=CARTESIAN_POINT('Ctrl Pts',(16.2917849850941,16.3592337341959,119.4415850402));
#110364=CARTESIAN_POINT('Ctrl Pts',(17.7752309220187,16.7142811876715,119.16251995002));
#110365=CARTESIAN_POINT('Ctrl Pts',(18.4783003209709,16.8349470402301,119.030177290372));
#110366=CARTESIAN_POINT('Ctrl Pts',(19.8249977354605,16.976833183057,118.776604568924));
#110367=CARTESIAN_POINT('Ctrl Pts',(20.4664967481208,17.0066111080161,118.655800410499));
#110368=CARTESIAN_POINT('Ctrl Pts',(21.4453715317864,16.9946575107851,118.471919832153));
#110369=CARTESIAN_POINT('Ctrl Pts',(21.782415201859,16.9801521685154,118.408670719453));
#110370=CARTESIAN_POINT('Ctrl Pts',(22.93891554042,16.894638106131,118.191639474227));
#110371=CARTESIAN_POINT('Ctrl Pts',(23.7535040221942,16.7724884813998,118.038707528667));
#110372=CARTESIAN_POINT('Ctrl Pts',(25.1180935327818,16.4618282631648,117.781744274011));
#110373=CARTESIAN_POINT('Ctrl Pts',(25.6734094801816,16.3043253562443,117.676964302909));
#110374=CARTESIAN_POINT('Ctrl Pts',(26.6676959571963,15.9650441009021,117.489167290262));
#110375=CARTESIAN_POINT('Ctrl Pts',(27.1092092516129,15.7928567789812,117.405719931934));
#110376=CARTESIAN_POINT('Ctrl Pts',(28.27614666206,15.2789934710198,117.185332752019));
#110377=CARTESIAN_POINT('Ctrl Pts',(28.9856268843385,14.9030339797141,117.051343368819));
#110378=CARTESIAN_POINT('Ctrl Pts',(30.2516948583679,14.1098087462447,116.811043835562));
#110379=CARTESIAN_POINT('Ctrl Pts',(30.8146274662093,13.7062664407844,116.703712047057));
#110380=CARTESIAN_POINT('Ctrl Pts',(31.896593767231,12.8239901004098,116.496438226064));
#110381=CARTESIAN_POINT('Ctrl Pts',(32.4137474342056,12.3450458660301,116.396858793694));
#110382=CARTESIAN_POINT('Ctrl Pts',(33.1490703295368,11.5728759390271,116.255044514662));
#110383=CARTESIAN_POINT('Ctrl Pts',(33.3899025178613,11.3031259146185,116.208530158652));
#110384=CARTESIAN_POINT('Ctrl Pts',(34.1366969902277,10.4105223481146,116.063824153262));
#110385=CARTESIAN_POINT('Ctrl Pts',(34.6075179955994,9.75874629390605,115.971799749524));
#110386=CARTESIAN_POINT('Ctrl Pts',(35.3407421564116,8.57500772105226,115.826415111035));
#110387=CARTESIAN_POINT('Ctrl Pts',(35.6246907724818,8.05853561231405,115.76941529427));
#110388=CARTESIAN_POINT('Ctrl Pts',(36.0828661064104,7.11219814942125,115.676289499588));
#110389=CARTESIAN_POINT('Ctrl Pts',(36.2673549594015,6.68813953265294,115.638368245058));
#110390=CARTESIAN_POINT('Ctrl Pts',(36.7318591556047,5.49018382018588,115.541901750737));
#110391=CARTESIAN_POINT('Ctrl Pts',(36.9738736735577,4.70238708866722,115.490214278083));
#110392=CARTESIAN_POINT('Ctrl Pts',(37.3197824840578,3.19922061230053,115.411800154912));
#110393=CARTESIAN_POINT('Ctrl Pts',(37.43698064961,2.48890638024839,115.382823561136));
#110394=CARTESIAN_POINT('Ctrl Pts',(37.5763106157877,1.11305312917326,115.342076736139));
#110395=CARTESIAN_POINT('Ctrl Pts',(37.6050197380707,0.449510452110751,
115.329194011537));
#110396=CARTESIAN_POINT('Ctrl Pts',(37.5905312631139,-0.560796264490243,
115.320311188467));
#110397=CARTESIAN_POINT('Ctrl Pts',(37.5751276169684,-0.907262466138281,
115.31916957441));
#110398=CARTESIAN_POINT('Ctrl Pts',(37.4870220068825,-2.08686360062308,
115.321562699139));
#110399=CARTESIAN_POINT('Ctrl Pts',(37.3642426354005,-2.91501470291571,
115.333914454204));
#110400=CARTESIAN_POINT('Ctrl Pts',(37.0534327155429,-4.30543659385099,
115.372336136456));
#110401=CARTESIAN_POINT('Ctrl Pts',(36.8956156583974,-4.87302346203984,
115.393264838432));
#110402=CARTESIAN_POINT('Ctrl Pts',(36.55962228171,-5.8785710340372,115.440104022816));
#110403=CARTESIAN_POINT('Ctrl Pts',(36.3918551493605,-6.3194630569091,115.464195304428));
#110404=CARTESIAN_POINT('Ctrl Pts',(35.8812923243715,-7.51135910002527,
115.539542383863));
#110405=CARTESIAN_POINT('Ctrl Pts',(35.5023164122996,-8.24502594434764,
115.597330608199));
#110406=CARTESIAN_POINT('Ctrl Pts',(34.6956101408257,-9.56338991659232,
115.722081992826));
#110407=CARTESIAN_POINT('Ctrl Pts',(34.280625505383,-10.1539171429642,115.786892888107));
#110408=CARTESIAN_POINT('Ctrl Pts',(33.4221029348028,-11.224110773041,115.92214910304));
#110409=CARTESIAN_POINT('Ctrl Pts',(32.9858025621622,-11.7080892166949,
115.991368216351));
#110410=CARTESIAN_POINT('Ctrl Pts',(32.2802501152059,-12.4054779115737,
116.104471010753));
#110411=CARTESIAN_POINT('Ctrl Pts',(32.0302456959124,-12.6380528025974,
116.144727981398));
#110412=CARTESIAN_POINT('Ctrl Pts',(31.1480639693456,-13.4101715841841,
116.287158460895));
#110413=CARTESIAN_POINT('Ctrl Pts',(30.4836903100857,-13.9100111801613,
116.39499994806));
#110414=CARTESIAN_POINT('Ctrl Pts',(29.2963274999843,-14.6724924285829,
116.587997707063));
#110415=CARTESIAN_POINT('Ctrl Pts',(28.7912288149617,-14.9608651822966,
116.670187978247));
#110416=CARTESIAN_POINT('Ctrl Pts',(27.8493300721744,-15.4353386551804,
116.8238100423));
#110417=CARTESIAN_POINT('Ctrl Pts',(27.4175263038477,-15.6302829320919,
116.894378486576));
#110418=CARTESIAN_POINT('Ctrl Pts',(26.2174918118913,-16.1116555507339,
117.091195595799));
#110419=CARTESIAN_POINT('Ctrl Pts',(25.4358484636341,-16.3600132846689,
117.219959307463));
#110420=CARTESIAN_POINT('Ctrl Pts',(23.9392718611159,-16.7162478435817,
117.466268183718));
#110421=CARTESIAN_POINT('Ctrl Pts',(23.2292505514606,-16.8371059063296,
117.583041448304));
#110422=CARTESIAN_POINT('Ctrl Pts',(21.8443102255085,-16.9809423852526,
117.810740120362));
#110423=CARTESIAN_POINT('Ctrl Pts',(21.171323745976,-17.0095872170374,117.921381200104));
#110424=CARTESIAN_POINT('Ctrl Pts',(20.1195190096776,-16.9902089287595,
118.094810677757));
#110425=CARTESIAN_POINT('Ctrl Pts',(19.7408769089898,-16.9702093049175,
118.157314067149));
#110426=CARTESIAN_POINT('Ctrl Pts',(18.6001131992247,-16.8705800755323,
118.345572825384));
#110427=CARTESIAN_POINT('Ctrl Pts',(17.8423841689354,-16.7510401190566,
118.470513173372));
#110428=CARTESIAN_POINT('Ctrl Pts',(16.5241842295137,-16.4482659024811,
118.687194231464));
#110429=CARTESIAN_POINT('Ctrl Pts',(15.9601934378477,-16.2868714560458,
118.779687049748));
#110430=CARTESIAN_POINT('Ctrl Pts',(14.976957725779,-15.9483006906574,118.940759997379));
#110431=CARTESIAN_POINT('Ctrl Pts',(14.5543047309711,-15.7831491857126,
119.009953977652));
#110432=CARTESIAN_POINT('Ctrl Pts',(13.3846165242419,-15.2700698900897,
119.201605219728));
#110433=CARTESIAN_POINT('Ctrl Pts',(12.6554664143251,-14.8835653687048,
119.321073815261));
#110434=CARTESIAN_POINT('Ctrl Pts',(11.3367736332283,-14.0544760261983,
119.535850083452));
#110435=CARTESIAN_POINT('Ctrl Pts',(10.7421480016747,-13.6238745881955,
119.632144648683));
#110436=CARTESIAN_POINT('Ctrl Pts',(9.67542669824277,-12.7396495519746,
119.803901001889));
#110437=CARTESIAN_POINT('Ctrl Pts',(9.19796648560238,-12.2947976368726,
119.880369953539));
#110438=CARTESIAN_POINT('Ctrl Pts',(8.17827012923428,-11.2280299160028,
120.043398424638));
#110439=CARTESIAN_POINT('Ctrl Pts',(7.65308893296738,-10.5916644716746,
120.126960316678));
#110440=CARTESIAN_POINT('Ctrl Pts',(6.76348485086405,-9.33853972082531,
120.266432958544));
#110441=CARTESIAN_POINT('Ctrl Pts',(6.38778879405164,-8.73226459447408,
120.324433377056));
#110442=CARTESIAN_POINT('Ctrl Pts',(5.73140868668388,-7.50838739786742,
120.423905018338));
#110443=CARTESIAN_POINT('Ctrl Pts',(5.4473668784054,-6.89412965705805,120.466015011068));
#110444=CARTESIAN_POINT('Ctrl Pts',(4.90360031729592,-5.50854092235599,
120.54504572343));
#110445=CARTESIAN_POINT('Ctrl Pts',(4.66080535888424,-4.73217529540783,
120.578967518694));
#110446=CARTESIAN_POINT('Ctrl Pts',(4.31302249985493,-3.26283597988525,
120.623265249966));
#110447=CARTESIAN_POINT('Ctrl Pts',(4.19367911309405,-2.57510314607509,
120.636271151057));
#110448=CARTESIAN_POINT('Ctrl Pts',(4.04643707067672,-1.25699276336321,
120.646735609308));
#110449=CARTESIAN_POINT('Ctrl Pts',(4.0108211163763,-0.628705474055431,
120.645595089839));
#110450=CARTESIAN_POINT('Ctrl Pts',(4.00959443610706,-1.25170827869336E-8,
120.638638242996));
#110451=CARTESIAN_POINT('Origin',(20.412052742069,1.37771738462078E-14,
115.762503617193));
#110452=CARTESIAN_POINT('',(3.80489827855296,1.16952742876573E-14,119.477748646113));
#110453=CARTESIAN_POINT('',(3.85199197861135,7.51016167425201E-9,119.744830291073));
#110454=CARTESIAN_POINT('',(3.67032094086137,1.16952742876573E-14,118.71452263753));
#110455=CARTESIAN_POINT('',(17.9811304327022,16.7992135480526,116.97809643255));
#110456=CARTESIAN_POINT('Origin',(20.5466300797608,1.37771738462078E-14,
116.525729625777));
#110457=CARTESIAN_POINT('Ctrl Pts',(17.9811304327023,16.7992135480526,116.97809643255));
#110458=CARTESIAN_POINT('Ctrl Pts',(16.7897846372373,16.6112487406192,117.201949554145));
#110459=CARTESIAN_POINT('Ctrl Pts',(15.6221214752571,16.2926540637075,117.422346711372));
#110460=CARTESIAN_POINT('Ctrl Pts',(13.7984931675232,15.5726780929255,117.766899663695));
#110461=CARTESIAN_POINT('Ctrl Pts',(13.1176819238496,15.2486694483281,117.89535197941));
#110462=CARTESIAN_POINT('Ctrl Pts',(11.8683145822032,14.5460375899264,118.13183797067));
#110463=CARTESIAN_POINT('Ctrl Pts',(11.2964699645734,14.1765810026866,118.240442965548));
#110464=CARTESIAN_POINT('Ctrl Pts',(10.1000199300896,13.2953484678201,118.468781311182));
#110465=CARTESIAN_POINT('Ctrl Pts',(9.48641127866864,12.7710444737475,118.58664290091));
#110466=CARTESIAN_POINT('Ctrl Pts',(8.41106966230483,11.7091865788779,118.793819869014));
#110467=CARTESIAN_POINT('Ctrl Pts',(7.94098286826109,11.1828822588,118.884524327492));
#110468=CARTESIAN_POINT('Ctrl Pts',(7.07488977840765,10.0815779627471,119.052942000803));
#110469=CARTESIAN_POINT('Ctrl Pts',(6.67873017827656,9.50845691218004,119.130682972688));
#110470=CARTESIAN_POINT('Ctrl Pts',(5.90057500006669,8.22000395384214,119.285353401939));
#110471=CARTESIAN_POINT('Ctrl Pts',(5.53205869993802,7.49827075882032,119.35996502358));
#110472=CARTESIAN_POINT('Ctrl Pts',(5.03245268068873,6.32019700437465,119.462841783204));
#110473=CARTESIAN_POINT('Ctrl Pts',(4.86689017575074,5.88037631964747,119.497300359212));
#110474=CARTESIAN_POINT('Ctrl Pts',(4.53511218387901,4.87565684204279,119.567599586156));
#110475=CARTESIAN_POINT('Ctrl Pts',(4.3794227228022,4.30778758820975,119.601585958567));
#110476=CARTESIAN_POINT('Ctrl Pts',(4.07443613362868,2.91937729590652,119.671469568118));
#110477=CARTESIAN_POINT('Ctrl Pts',(3.9549810780892,2.09359099508143,119.702253960006));
#110478=CARTESIAN_POINT('Ctrl Pts',(3.8709218449021,0.914803833709377,119.730912944905));
#110479=CARTESIAN_POINT('Ctrl Pts',(3.85667055737714,0.566765573452197,
119.737496515519));
#110480=CARTESIAN_POINT('Ctrl Pts',(3.85216809223894,0.145671403107022,
119.743133563671));
#110481=CARTESIAN_POINT('Ctrl Pts',(3.85184987052789,0.0728341540194984,
119.744024355712));
#110482=CARTESIAN_POINT('Ctrl Pts',(3.85199197861135,1.50203116532297E-8,
119.744830291073));
#110483=CARTESIAN_POINT('Origin',(20.5162416486691,1.37771738462078E-14,
116.353388269));
#110484=CARTESIAN_POINT('',(21.2294226865383,16.375,120.398038737828));
#110485=CARTESIAN_POINT('',(21.261705303182,16.375,120.581122925479));
#110486=CARTESIAN_POINT('',(20.5162416486691,16.375,116.353388269));
#110487=CARTESIAN_POINT('',(29.803853834021,-13.9658945114651,119.791289468368));
#110488=CARTESIAN_POINT('Ctrl Pts',(21.2617053031124,16.375,120.581122925109));
#110489=CARTESIAN_POINT('Ctrl Pts',(21.1269512056705,16.3749999997303,120.606507815194));
#110490=CARTESIAN_POINT('Ctrl Pts',(20.9921933482164,16.3732778189865,120.63190684463));
#110491=CARTESIAN_POINT('Ctrl Pts',(20.4234668755599,16.3587364271667,120.739138712706));
#110492=CARTESIAN_POINT('Ctrl Pts',(19.9901057026894,16.3297742801148,120.820938220858));
#110493=CARTESIAN_POINT('Ctrl Pts',(18.9074685346542,16.2125102897728,121.025273537121));
#110494=CARTESIAN_POINT('Ctrl Pts',(18.2613381062145,16.1016481834457,121.147187874784));
#110495=CARTESIAN_POINT('Ctrl Pts',(17.040237438277,15.8132755463647,121.377460830846));
#110496=CARTESIAN_POINT('Ctrl Pts',(16.464849099634,15.6424711480854,121.485914365438));
#110497=CARTESIAN_POINT('Ctrl Pts',(15.5273800888505,15.3053767234912,121.662938424917));
#110498=CARTESIAN_POINT('Ctrl Pts',(15.1595706886934,15.1573850569893,121.732498702259));
#110499=CARTESIAN_POINT('Ctrl Pts',(14.4252491828481,14.8295638279538,121.871755302321));
#110500=CARTESIAN_POINT('Ctrl Pts',(14.0593279911024,14.6490727431445,121.941311346875));
#110501=CARTESIAN_POINT('Ctrl Pts',(13.0802953667339,14.1186195775368,122.127631897839));
#110502=CARTESIAN_POINT('Ctrl Pts',(12.4823912340228,13.7415689404671,122.241638539003));
#110503=CARTESIAN_POINT('Ctrl Pts',(11.4207751138345,12.969825138321,122.444387053643));
#110504=CARTESIAN_POINT('Ctrl Pts',(10.9509477020293,12.5859985757552,122.534257344454));
#110505=CARTESIAN_POINT('Ctrl Pts',(10.1918732035576,11.8910283622617,122.68013809973));
#110506=CARTESIAN_POINT('Ctrl Pts',(9.8914274046672,11.5934999012115,122.738110135063));
#110507=CARTESIAN_POINT('Ctrl Pts',(9.30389691116128,10.9642473591434,122.852132975335));
#110508=CARTESIAN_POINT('Ctrl Pts',(9.01790100642259,10.6319450589894,122.907948037655));
#110509=CARTESIAN_POINT('Ctrl Pts',(8.3346946432277,9.77002890623512,123.041852891722));
#110510=CARTESIAN_POINT('Ctrl Pts',(7.95541465582553,9.22672979937164,123.116714236926));
#110511=CARTESIAN_POINT('Ctrl Pts',(7.29353055361505,8.14421917103656,123.24838215676));
#110512=CARTESIAN_POINT('Ctrl Pts',(7.00596235598823,7.6094465227335,123.306085224782));
#110513=CARTESIAN_POINT('Ctrl Pts',(6.57839874640348,6.69652825631077,123.393199208712));
#110514=CARTESIAN_POINT('Ctrl Pts',(6.42160935731405,6.32721063845961,123.42555097996));
#110515=CARTESIAN_POINT('Ctrl Pts',(6.13113819043648,5.56695197763243,123.486544787148));
#110516=CARTESIAN_POINT('Ctrl Pts',(5.99833290099452,5.17597196389945,123.514996189111));
#110517=CARTESIAN_POINT('Ctrl Pts',(5.67612605157289,4.09624359164223,123.585500638579));
#110518=CARTESIAN_POINT('Ctrl Pts',(5.51633769147871,3.39926906699333,123.622255672012));
#110519=CARTESIAN_POINT('Ctrl Pts',(5.30385533983494,2.08939589378513,123.675279010022));
#110520=CARTESIAN_POINT('Ctrl Pts',(5.23927219752487,1.47978403044136,123.693693797234));
#110521=CARTESIAN_POINT('Ctrl Pts',(5.18708047007613,0.441860951021354,
123.714932049854));
#110522=CARTESIAN_POINT('Ctrl Pts',(5.1820715209045,0.0151378861207446,
123.720810605118));
#110523=CARTESIAN_POINT('Ctrl Pts',(5.20533579560537,-0.852946561745866,
123.727133846083));
#110524=CARTESIAN_POINT('Ctrl Pts',(5.23477924860972,-1.29392967011017,
123.727328428485));
#110525=CARTESIAN_POINT('Ctrl Pts',(5.35255986801764,-2.39559987145586,
123.719997679546));
#110526=CARTESIAN_POINT('Ctrl Pts',(5.4631026600747,-3.05308131739314,123.708490076003));
#110527=CARTESIAN_POINT('Ctrl Pts',(5.74965155641503,-4.29561372888164,
123.672923694812));
#110528=CARTESIAN_POINT('Ctrl Pts',(5.91905732867391,-4.88109286318209,
123.650049926354));
#110529=CARTESIAN_POINT('Ctrl Pts',(6.25303511544757,-5.83505987818467,
123.602883613529));
#110530=CARTESIAN_POINT('Ctrl Pts',(6.39958339676622,-6.20936127595935,
123.581748763323));
#110531=CARTESIAN_POINT('Ctrl Pts',(6.72409593944177,-6.95670839164034,
123.534304350866));
#110532=CARTESIAN_POINT('Ctrl Pts',(6.90270537908738,-7.32914786893943,
123.507844941356));
#110533=CARTESIAN_POINT('Ctrl Pts',(7.42744081686339,-8.32566133521726,
123.429010612853));
#110534=CARTESIAN_POINT('Ctrl Pts',(7.80023096658084,-8.93428005939323,
123.371857676562));
#110535=CARTESIAN_POINT('Ctrl Pts',(8.56291104944619,-10.0149755171322,
123.252933560257));
#110536=CARTESIAN_POINT('Ctrl Pts',(8.94210788683628,-10.4932708191696,
123.193097965516));
#110537=CARTESIAN_POINT('Ctrl Pts',(9.62857811287774,-11.2661453947988,
123.084090185315));
#110538=CARTESIAN_POINT('Ctrl Pts',(9.92244097039273,-11.5720938239209,
123.037269574351));
#110539=CARTESIAN_POINT('Ctrl Pts',(10.5439165031095,-12.1704982453563,
122.938112031132));
#110540=CARTESIAN_POINT('Ctrl Pts',(10.8720910784943,-12.4618411075081,
122.88563226067));
#110541=CARTESIAN_POINT('Ctrl Pts',(11.7232110728059,-13.1579209029844,
122.748993988834));
#110542=CARTESIAN_POINT('Ctrl Pts',(12.2596225237396,-13.5444390127188,
122.662394241632));
#110543=CARTESIAN_POINT('Ctrl Pts',(13.3282468833882,-14.2191321682476,
122.488926845304));
#110544=CARTESIAN_POINT('Ctrl Pts',(13.8560919154325,-14.5123516537041,
122.402850562903));
#110545=CARTESIAN_POINT('Ctrl Pts',(14.7571455984442,-14.9485466527617,
122.255693470097));
#110546=CARTESIAN_POINT('Ctrl Pts',(15.1216568623872,-15.1085717248892,
122.196125867526));
#110547=CARTESIAN_POINT('Ctrl Pts',(15.8720373112074,-15.4052214253995,
122.073589452596));
#110548=CARTESIAN_POINT('Ctrl Pts',(16.2579387225977,-15.5409497290459,
122.010578872716));
#110549=CARTESIAN_POINT('Ctrl Pts',(17.323604807395,-15.8705043590967,121.83636387708));
#110550=CARTESIAN_POINT('Ctrl Pts',(18.0114575793266,-16.0342474679337,
121.72365690338));
#110551=CARTESIAN_POINT('Ctrl Pts',(19.3040909184839,-16.2527090462653,
121.511287731991));
#110552=CARTESIAN_POINT('Ctrl Pts',(19.9056432154307,-16.3195087069062,
121.412244869666));
#110553=CARTESIAN_POINT('Ctrl Pts',(20.9298560428971,-16.374595452193,121.243683956606));
#110554=CARTESIAN_POINT('Ctrl Pts',(21.350950315253,-16.3805490867381,121.174429015541));
#110555=CARTESIAN_POINT('Ctrl Pts',(22.2076294821451,-16.3587362487866,
121.033798725361));
#110556=CARTESIAN_POINT('Ctrl Pts',(22.6428343647055,-16.3297738665615,
120.962446622456));
#110557=CARTESIAN_POINT('Ctrl Pts',(23.7567701834067,-16.2096293183694,
120.779796878244));
#110558=CARTESIAN_POINT('Ctrl Pts',(24.4319001791433,-16.092525994299,120.669056267746));
#110559=CARTESIAN_POINT('Ctrl Pts',(25.7011748832876,-15.7872685860135,
120.460728725052));
#110560=CARTESIAN_POINT('Ctrl Pts',(26.2959353891529,-15.6070341040097,
120.363059305307));
#110561=CARTESIAN_POINT('Ctrl Pts',(27.2530063170519,-15.2550803340175,
120.206278780732));
#110562=CARTESIAN_POINT('Ctrl Pts',(27.6218563501888,-15.1036121468542,
120.145985071172));
#110563=CARTESIAN_POINT('Ctrl Pts',(28.6108934709591,-14.6537505947678,
119.984795098443));
#110564=CARTESIAN_POINT('Ctrl Pts',(29.2184750314435,-14.3288893674278,
119.886175468315));
#110565=CARTESIAN_POINT('Ctrl Pts',(29.8038538340209,-13.9658945114651,
119.791289468367));
#110566=CARTESIAN_POINT('',(29.9797471638325,-13.9658945114651,120.78883011192));
#110567=CARTESIAN_POINT('',(28.9358823285198,-13.9658945114651,114.868778449272));
#110568=CARTESIAN_POINT('',(21.4378004997014,16.375,121.57980804145));
#110569=CARTESIAN_POINT('Ctrl Pts',(29.9797471638324,-13.9658945114651,
120.78883011192));
#110570=CARTESIAN_POINT('Ctrl Pts',(29.3944021100277,-14.3288894249513,
120.883908051799));
#110571=CARTESIAN_POINT('Ctrl Pts',(28.7869186269802,-14.6537508697208,
120.983086135754));
#110572=CARTESIAN_POINT('Ctrl Pts',(27.7979459389566,-15.1036132821563,
121.144653755592));
#110573=CARTESIAN_POINT('Ctrl Pts',(27.4290848004083,-15.2550818060388,
121.204892044499));
#110574=CARTESIAN_POINT('Ctrl Pts',(26.4719346799092,-15.6070341116341,
121.361202243655));
#110575=CARTESIAN_POINT('Ctrl Pts',(25.8770929701107,-15.7872689181212,
121.458416794086));
#110576=CARTESIAN_POINT('Ctrl Pts',(24.6077612876369,-16.0925256255625,
121.666406371788));
#110577=CARTESIAN_POINT('Ctrl Pts',(23.932665983966,-16.2096292700361,121.777342911966));
#110578=CARTESIAN_POINT('Ctrl Pts',(22.8188369260007,-16.3297740799414,
121.960622120204));
#110579=CARTESIAN_POINT('Ctrl Pts',(22.3836860223534,-16.3587363282615,
122.032277261078));
#110580=CARTESIAN_POINT('Ctrl Pts',(21.5270543386933,-16.3805491248486,
122.173179027013));
#110581=CARTESIAN_POINT('Ctrl Pts',(21.1059385050175,-16.3745952485427,
122.242325956352));
#110582=CARTESIAN_POINT('Ctrl Pts',(20.0816359839474,-16.3195085930257,
122.410352281758));
#110583=CARTESIAN_POINT('Ctrl Pts',(19.4800062015085,-16.2527088833392,
122.508960347141));
#110584=CARTESIAN_POINT('Ctrl Pts',(18.1873191735067,-16.0342478697915,
122.721001538412));
#110585=CARTESIAN_POINT('Ctrl Pts',(17.4995094847756,-15.8705056928154,
122.833941613525));
#110586=CARTESIAN_POINT('Ctrl Pts',(16.4339496735706,-15.540950150731,123.008779836653));
#110587=CARTESIAN_POINT('Ctrl Pts',(16.0480942764558,-15.4052216747475,
123.072054053034));
#110588=CARTESIAN_POINT('Ctrl Pts',(15.2977511897487,-15.1085719611476,
123.194803313129));
#110589=CARTESIAN_POINT('Ctrl Pts',(14.9332184555073,-14.9485461801693,
123.254257208779));
#110590=CARTESIAN_POINT('Ctrl Pts',(14.0320796358113,-14.5123532582918,
123.400908319161));
#110591=CARTESIAN_POINT('Ctrl Pts',(13.5041600021885,-14.219133267749,123.486568992282));
#110592=CARTESIAN_POINT('Ctrl Pts',(12.4354863194849,-13.5444404384541,
123.659754835075));
#110593=CARTESIAN_POINT('Ctrl Pts',(11.8991092132909,-13.1579220206212,
123.746555154068));
#110594=CARTESIAN_POINT('Ctrl Pts',(11.0480938874283,-12.461839043354,123.883807708687));
#110595=CARTESIAN_POINT('Ctrl Pts',(10.7199733362648,-12.1704965455087,
123.936590510773));
#110596=CARTESIAN_POINT('Ctrl Pts',(10.0985454486913,-11.5720918322731,
124.036019501507));
#110597=CARTESIAN_POINT('Ctrl Pts',(9.80466184291277,-11.2661413923323,
124.082731956147));
#110598=CARTESIAN_POINT('Ctrl Pts',(9.11810056555315,-10.493270010477,124.191205387751));
#110599=CARTESIAN_POINT('Ctrl Pts',(8.73882656970699,-10.0149741521335,
124.250606128712));
#110600=CARTESIAN_POINT('Ctrl Pts',(7.97609112199115,-8.93428178111615,
124.369202557721));
#110601=CARTESIAN_POINT('Ctrl Pts',(7.60334271648535,-8.32566482224343,
124.426588827785));
#110602=CARTESIAN_POINT('Ctrl Pts',(7.07871526636778,-7.32914810760958,
124.506046080878));
#110603=CARTESIAN_POINT('Ctrl Pts',(6.90015222220985,-6.95670839502068,
124.532769062744));
#110604=CARTESIAN_POINT('Ctrl Pts',(6.57567713062222,-6.20936116622651,
124.580426305091));
#110605=CARTESIAN_POINT('Ctrl Pts',(6.42910821308334,-5.83505806167831,
124.601447298829));
#110606=CARTESIAN_POINT('Ctrl Pts',(6.09504272613763,-4.88109526449257,
124.64810808053));
#110607=CARTESIAN_POINT('Ctrl Pts',(5.92556315345833,-4.29561499013365,
124.670566100082));
#110608=CARTESIAN_POINT('Ctrl Pts',(5.63896487902089,-3.05308393470428,
124.705850948283));
#110609=CARTESIAN_POINT('Ctrl Pts',(5.52845704873351,-2.39560234093178,
124.71755902434));
#110610=CARTESIAN_POINT('Ctrl Pts',(5.41078428677368,-1.29392779961911,
124.725503499201));
#110611=CARTESIAN_POINT('Ctrl Pts',(5.38139438319101,-0.852945015804496,
124.725612027869));
#110612=CARTESIAN_POINT('Ctrl Pts',(5.35817798569936,0.0151398450618967,
124.719560192696));
#110613=CARTESIAN_POINT('Ctrl Pts',(5.36316803309009,0.441865208087525,
124.713573158733));
#110614=CARTESIAN_POINT('Ctrl Pts',(5.41526548781392,1.47978373344985,124.691801126435));
#110615=CARTESIAN_POINT('Ctrl Pts',(5.47977197340088,2.08939652759494,124.672951394821));
#110616=CARTESIAN_POINT('Ctrl Pts',(5.6921959618452,3.39926527619464,124.619600905232));
#110617=CARTESIAN_POINT('Ctrl Pts',(5.85202440596573,4.0962373951753,124.58307950803));
#110618=CARTESIAN_POINT('Ctrl Pts',(6.17434178503615,5.1759692947472,124.513197536662));
#110619=CARTESIAN_POINT('Ctrl Pts',(6.30719381190663,5.56695016223244,124.485009638771));
#110620=CARTESIAN_POINT('Ctrl Pts',(6.59770249544839,6.32720904056206,124.424228648833));
#110621=CARTESIAN_POINT('Ctrl Pts',(6.75447232087668,6.69652774090623,124.391762838437));
#110622=CARTESIAN_POINT('Ctrl Pts',(7.18194463766329,7.60944193100352,124.304143958711));
#110623=CARTESIAN_POINT('Ctrl Pts',(7.46944007558031,8.1442161164386,124.246024954014));
#110624=CARTESIAN_POINT('Ctrl Pts',(8.13127492523547,9.22672774730711,124.114075450868));
#110625=CARTESIAN_POINT('Ctrl Pts',(8.51059129421667,9.77002887131228,124.039414303072));
#110626=CARTESIAN_POINT('Ctrl Pts',(9.19390956598191,10.6319490500238,123.906122446443));
#110627=CARTESIAN_POINT('Ctrl Pts',(9.4799582384132,10.9642503171294,123.850610644148));
#110628=CARTESIAN_POINT('Ctrl Pts',(10.0675368529298,11.5935029744899,123.736859168768));
#110629=CARTESIAN_POINT('Ctrl Pts',(10.3679658697001,11.8910333821555,123.678778272639));
#110630=CARTESIAN_POINT('Ctrl Pts',(11.1269433076025,12.5860004639231,123.532364226923));
#110631=CARTESIAN_POINT('Ctrl Pts',(11.5966943771743,12.9698272473745,123.442058941853));
#110632=CARTESIAN_POINT('Ctrl Pts',(12.6582505577837,13.7415691161477,123.238983535326));
#110633=CARTESIAN_POINT('Ctrl Pts',(13.2561952297131,14.1186196962087,123.12521042485));
#110634=CARTESIAN_POINT('Ctrl Pts',(14.2353411786659,14.6490744678662,122.939511854664));
#110635=CARTESIAN_POINT('Ctrl Pts',(14.6013081951695,14.8295650960931,122.870219495883));
#110636=CARTESIAN_POINT('Ctrl Pts',(15.3356672835137,15.1573862653283,122.731175704262));
#110637=CARTESIAN_POINT('Ctrl Pts',(15.7034591555473,15.3053787483099,122.66150101211));
#110638=CARTESIAN_POINT('Ctrl Pts',(16.6408352988461,15.6424715764168,122.483972329681));
#110639=CARTESIAN_POINT('Ctrl Pts',(17.2161508849222,15.8132761446567,122.375102868236));
#110640=CARTESIAN_POINT('Ctrl Pts',(18.4371969010661,16.1016474159221,122.144549354173));
#110641=CARTESIAN_POINT('Ctrl Pts',(19.0833596182917,16.2125094357943,122.022835999945));
#110642=CARTESIAN_POINT('Ctrl Pts',(20.1661074307351,16.3297740472679,121.819113940843));
#110643=CARTESIAN_POINT('Ctrl Pts',(20.5995231439279,16.3587363141683,121.737617351258));
#110644=CARTESIAN_POINT('Ctrl Pts',(21.1682825795621,16.3732778015187,121.630566221165));
#110645=CARTESIAN_POINT('Ctrl Pts',(21.3030457948456,16.3750000002692,121.605193046341));
#110646=CARTESIAN_POINT('Ctrl Pts',(21.4378004997708,16.375,121.579808041818));
#110647=CARTESIAN_POINT('',(21.9054270700044,16.375,124.231850293098));
#110648=CARTESIAN_POINT('',(20.5162416486691,16.375,116.353388269));
#110649=CARTESIAN_POINT('',(38.0316540255793,1.18260248212283E-14,121.388361383802));
#110650=CARTESIAN_POINT('Origin',(21.9054270700043,1.37771738462078E-14,
124.231850293098));
#110651=CARTESIAN_POINT('Origin',(21.9054270700043,1.37771738462078E-14,
124.231850293098));
#110652=CARTESIAN_POINT('Ctrl Pts',(21.4378004997708,16.375,121.579808041818));
#110653=CARTESIAN_POINT('Ctrl Pts',(21.7222361261571,16.3749999994318,121.526226241716));
#110654=CARTESIAN_POINT('Ctrl Pts',(22.0066339771936,16.3673270421196,121.47259248499));
#110655=CARTESIAN_POINT('Ctrl Pts',(22.8920517384166,16.3195086361738,121.305544195588));
#110656=CARTESIAN_POINT('Ctrl Pts',(23.491124819392,16.2527089343712,121.192435949445));
#110657=CARTESIAN_POINT('Ctrl Pts',(24.7783754467992,16.0342479790364,120.949564525856));
#110658=CARTESIAN_POINT('Ctrl Pts',(25.46333266265,15.8705058949884,120.820448760452));
#110659=CARTESIAN_POINT('Ctrl Pts',(26.5244295283424,15.5409504402565,120.620300033193));
#110660=CARTESIAN_POINT('Ctrl Pts',(26.9086562714279,15.4052219085772,120.547787988342));
#110661=CARTESIAN_POINT('Ctrl Pts',(27.6557308815608,15.1085722073146,120.406502106944));
#110662=CARTESIAN_POINT('Ctrl Pts',(28.0186138551774,14.9485465243931,120.337692989708));
#110663=CARTESIAN_POINT('Ctrl Pts',(28.9155649566073,14.5123536902484,120.167292334214));
#110664=CARTESIAN_POINT('Ctrl Pts',(29.4409449496387,14.2191336615093,120.067227862616));
#110665=CARTESIAN_POINT('Ctrl Pts',(30.5044035067849,13.5444404241436,119.864461254712));
#110666=CARTESIAN_POINT('Ctrl Pts',(31.0381211372528,13.157921576383,119.762574991515));
#110667=CARTESIAN_POINT('Ctrl Pts',(31.8847573402336,12.4618382692119,119.600485773276));
#110668=CARTESIAN_POINT('Ctrl Pts',(32.2111423310358,12.1704959589415,119.537861592847));
#110669=CARTESIAN_POINT('Ctrl Pts',(32.8291001932741,11.5720912592585,119.418753436823));
#110670=CARTESIAN_POINT('Ctrl Pts',(33.121237213726,11.266140611681,119.362134640409));
#110671=CARTESIAN_POINT('Ctrl Pts',(33.8034938719758,10.4932691090054,119.229248537044));
#110672=CARTESIAN_POINT('Ctrl Pts',(34.1802109554807,10.0149733658491,119.155347655861));
#110673=CARTESIAN_POINT('Ctrl Pts',(34.9375104429859,8.93428052790522,119.005920908103));
#110674=CARTESIAN_POINT('Ctrl Pts',(35.3074069273513,8.32566292344506,118.932358839238));
#110675=CARTESIAN_POINT('Ctrl Pts',(35.8275713306143,7.32914601069121,118.827591098178));
#110676=CARTESIAN_POINT('Ctrl Pts',(36.0045052055848,6.95670680667804,118.791630388278));
#110677=CARTESIAN_POINT('Ctrl Pts',(36.3257117160693,6.20935960933227,118.72543654362));
#110678=CARTESIAN_POINT('Ctrl Pts',(36.4706311965658,5.8350559938846,118.695060261463));
#110679=CARTESIAN_POINT('Ctrl Pts',(36.8005088957717,4.88109297625686,118.624649943295));
#110680=CARTESIAN_POINT('Ctrl Pts',(36.9674485190917,4.29561302139565,118.587788186366));
#110681=CARTESIAN_POINT('Ctrl Pts',(37.248830317375,3.05308409461299,118.522922850208));
#110682=CARTESIAN_POINT('Ctrl Pts',(37.3566778499744,2.39560434712044,118.49612900573));
#110683=CARTESIAN_POINT('Ctrl Pts',(37.4699713981878,1.29393086671745,118.463347900124));
#110684=CARTESIAN_POINT('Ctrl Pts',(37.4976261147887,0.852947267673733,
118.453397913905));
#110685=CARTESIAN_POINT('Ctrl Pts',(37.5173726205114,-0.0151377222979068,
118.439770558581));
#110686=CARTESIAN_POINT('Ctrl Pts',(37.5106358978946,-0.441862395858203,
118.435851279401));
#110687=CARTESIAN_POINT('Ctrl Pts',(37.4542340612267,-1.47978071072371,
118.433210602794));
#110688=CARTESIAN_POINT('Ctrl Pts',(37.3871708562621,-2.08939398164617,
118.437560151437));
#110689=CARTESIAN_POINT('Ctrl Pts',(37.1693110498983,-3.39926140698662,
118.460080320012));
#110690=CARTESIAN_POINT('Ctrl Pts',(37.0066310088258,-4.09623178047477,
118.480425890428));
#110691=CARTESIAN_POINT('Ctrl Pts',(36.6798512862242,-5.17596354202306,
118.524997254247));
#110692=CARTESIAN_POINT('Ctrl Pts',(36.5453700143859,-5.56694590290851,
118.543947412508));
#110693=CARTESIAN_POINT('Ctrl Pts',(36.2515929072055,-6.32720498028925,
118.586191770913));
#110694=CARTESIAN_POINT('Ctrl Pts',(36.0931741535806,-6.69652246503088,
118.609302228583));
#110695=CARTESIAN_POINT('Ctrl Pts',(35.6615147351133,-7.60943643762439,
118.673171460244));
#110696=CARTESIAN_POINT('Ctrl Pts',(35.3714792670182,-8.14421153955864,
118.716886724508));
#110697=CARTESIAN_POINT('Ctrl Pts',(34.7044258267118,-9.22672823825842,
118.819256011129));
#110698=CARTESIAN_POINT('Ctrl Pts',(34.3224465464673,-9.77003324424218,
118.878831771153));
#110699=CARTESIAN_POINT('Ctrl Pts',(33.6347467080441,-10.6319550936825,
118.987287368102));
#110700=CARTESIAN_POINT('Ctrl Pts',(33.346963979321,-10.9642546314623,119.032957548238));
#110701=CARTESIAN_POINT('Ctrl Pts',(32.7559154858868,-11.5935069059218,
119.127029835159));
#110702=CARTESIAN_POINT('Ctrl Pts',(32.4537383334366,-11.8910384451211,
119.175204642437));
#110703=CARTESIAN_POINT('Ctrl Pts',(31.690455477193,-12.5860054842662,119.297206149842));
#110704=CARTESIAN_POINT('Ctrl Pts',(31.2181484062862,-12.9698312933602,
119.373011148012));
#110705=CARTESIAN_POINT('Ctrl Pts',(30.1511529021958,-13.7415748715436,
119.54525679231));
#110706=CARTESIAN_POINT('Ctrl Pts',(29.5503517047452,-14.1186275058327,
119.642854869179));
#110707=CARTESIAN_POINT('Ctrl Pts',(28.5667415101329,-14.6490814459875,
119.803243155691));
#110708=CARTESIAN_POINT('Ctrl Pts',(28.1991490155244,-14.8295700208867,
119.863297175526));
#110709=CARTESIAN_POINT('Ctrl Pts',(27.4615216312337,-15.1573906711399,
119.98380431688));
#110710=CARTESIAN_POINT('Ctrl Pts',(27.0920767663623,-15.3053841706741,
120.044124306935));
#110711=CARTESIAN_POINT('Ctrl Pts',(26.1505114659207,-15.6424763086833,
120.197903679364));
#110712=CARTESIAN_POINT('Ctrl Pts',(25.5726582382064,-15.8132796665848,
120.292369024202));
#110713=CARTESIAN_POINT('Ctrl Pts',(24.3464105618023,-16.101646690875,120.493339600122));
#110714=CARTESIAN_POINT('Ctrl Pts',(23.6976001202803,-16.2125069155516,
120.599965097211));
#110715=CARTESIAN_POINT('Ctrl Pts',(22.6104800182628,-16.3297725545985,
120.778849374753));
#110716=CARTESIAN_POINT('Ctrl Pts',(22.1753235581518,-16.3587356703288,
120.85050543153));
#110717=CARTESIAN_POINT('Ctrl Pts',(21.3186909946927,-16.3805490143385,
120.991407344687));
#110718=CARTESIAN_POINT('Ctrl Pts',(20.897579861281,-16.3745956486072,121.060553506266));
#110719=CARTESIAN_POINT('Ctrl Pts',(19.8732787757631,-16.3195106073079,
121.228579600857));
#110720=CARTESIAN_POINT('Ctrl Pts',(19.2716457430119,-16.2527112656557,
121.327188197699));
#110721=CARTESIAN_POINT('Ctrl Pts',(17.9789677331887,-16.0342529693121,
121.539227907782));
#110722=CARTESIAN_POINT('Ctrl Pts',(17.2911699400339,-15.8705151299385,
121.65216602469));
#110723=CARTESIAN_POINT('Ctrl Pts',(16.2256110707781,-15.5409636651203,
121.827004102874));
#110724=CARTESIAN_POINT('Ctrl Pts',(15.8397454956958,-15.4052325893497,
121.890279994752));
#110725=CARTESIAN_POINT('Ctrl Pts',(15.089401052641,-15.1085834508617,122.01302948704));
#110726=CARTESIAN_POINT('Ctrl Pts',(14.7248766060145,-14.9485622461053,
122.072482042681));
#110727=CARTESIAN_POINT('Ctrl Pts',(13.8237392726469,-14.5123734185352,
122.219132935716));
#110728=CARTESIAN_POINT('Ctrl Pts',(13.2958133916514,-14.2191516452739,
122.304794627804));
#110729=CARTESIAN_POINT('Ctrl Pts',(12.2271051636115,-13.5444397730029,
122.477986077817));
#110730=CARTESIAN_POINT('Ctrl Pts',(11.6907015942455,-13.1579012925143,
122.564790680211));
#110731=CARTESIAN_POINT('Ctrl Pts',(10.8396748707199,-12.4618029196469,
122.702045035395));
#110732=CARTESIAN_POINT('Ctrl Pts',(10.5115661066434,-12.1704691744574,
122.754825925016));
#110733=CARTESIAN_POINT('Ctrl Pts',(9.89014082440581,-11.5720650916264,
122.854254476866));
#110734=CARTESIAN_POINT('Ctrl Pts',(9.5962494959249,-11.2661049607716,122.900968134615));
#110735=CARTESIAN_POINT('Ctrl Pts',(8.9096884978164,-10.493227939379,123.009441458972));
#110736=CARTESIAN_POINT('Ctrl Pts',(8.53042114646386,-10.0149374565039,
123.068841136596));
#110737=CARTESIAN_POINT('Ctrl Pts',(7.76767401985128,-8.93422328457483,
123.187439341529));
#110738=CARTESIAN_POINT('Ctrl Pts',(7.39491157825789,-8.3255761861697,123.244827724305));
#110739=CARTESIAN_POINT('Ctrl Pts',(6.8702897731879,-7.32905021976876,123.324283926982));
#110740=CARTESIAN_POINT('Ctrl Pts',(6.69174074833573,-6.95663424770594,
123.35100474664));
#110741=CARTESIAN_POINT('Ctrl Pts',(6.36726918610559,-6.20928847661341,
123.398661384592));
#110742=CARTESIAN_POINT('Ctrl Pts',(6.22069329714319,-5.83496151244486,
123.419683291972));
#110743=CARTESIAN_POINT('Ctrl Pts',(5.88663248396758,-4.88098841719496,
123.466343133131));
#110744=CARTESIAN_POINT('Ctrl Pts',(5.71716118231043,-4.29552306043338,
123.488799909125));
#110745=CARTESIAN_POINT('Ctrl Pts',(5.43059202460564,-3.05309143511461,
123.524080882845));
#110746=CARTESIAN_POINT('Ctrl Pts',(5.32009658211262,-2.39569608842982,
123.535787770744));
#110747=CARTESIAN_POINT('Ctrl Pts',(5.20241691740778,-1.29407109911206,
123.543734006921));
#110748=CARTESIAN_POINT('Ctrl Pts',(5.17302116161042,-0.853050225325708,
123.543843135581));
#110749=CARTESIAN_POINT('Ctrl Pts',(5.14980110809517,0.015040685568975,
123.537791891366));
#110750=CARTESIAN_POINT('Ctrl Pts',(5.15478782601776,0.441733852511547,
123.531805857046));
#110751=CARTESIAN_POINT('Ctrl Pts',(5.20687455744126,1.47964255425242,123.510035866345));
#110752=CARTESIAN_POINT('Ctrl Pts',(5.2713785440764,2.08927761857135,123.491186293648));
#110753=CARTESIAN_POINT('Ctrl Pts',(5.48378457540696,3.39908464039202,123.437839706366));
#110754=CARTESIAN_POINT('Ctrl Pts',(5.64358431556042,4.09597530786932,123.401324311695));
#110755=CARTESIAN_POINT('Ctrl Pts',(5.96587458919859,5.17570078817396,123.331447262404));
#110756=CARTESIAN_POINT('Ctrl Pts',(6.09874378158368,5.56675136468612,123.303255532476));
#110757=CARTESIAN_POINT('Ctrl Pts',(6.38924865359715,6.32701960449139,123.242475166738));
#110758=CARTESIAN_POINT('Ctrl Pts',(6.54598818995834,6.69628163084384,123.210015516241));
#110759=CARTESIAN_POINT('Ctrl Pts',(6.9734333383126,7.60918570681968,123.122401728821));
#110760=CARTESIAN_POINT('Ctrl Pts',(7.26094054104113,8.14400264683535,123.064280091628));
#110761=CARTESIAN_POINT('Ctrl Pts',(7.92290138239413,9.22675044927814,122.932305105973));
#110762=CARTESIAN_POINT('Ctrl Pts',(8.30235062028651,9.7702324418394,122.857617947061));
#110763=CARTESIAN_POINT('Ctrl Pts',(8.98577097363052,10.632230507092,122.724306678918));
#110764=CARTESIAN_POINT('Ctrl Pts',(9.2717617017989,10.9644512454239,122.668806212761));
#110765=CARTESIAN_POINT('Ctrl Pts',(9.85933622795868,11.593686162692,122.555055595291));
#110766=CARTESIAN_POINT('Ctrl Pts',(10.1598295101648,11.8912693453428,122.496962296319));
#110767=CARTESIAN_POINT('Ctrl Pts',(10.9188444059412,12.5862344768742,122.350541253647));
#110768=CARTESIAN_POINT('Ctrl Pts',(11.3885598734022,12.9700158503167,122.260242976885));
#110769=CARTESIAN_POINT('Ctrl Pts',(12.4502610211082,13.7418377013528,122.057140090391));
#110770=CARTESIAN_POINT('Ctrl Pts',(13.0484060276627,14.1189842703515,121.943329205423));
#110771=CARTESIAN_POINT('Ctrl Pts',(14.0276136304381,14.6494002917169,121.757619390156));
#110772=CARTESIAN_POINT('Ctrl Pts',(14.3934229711875,14.8297950632316,121.688356927724));
#110773=CARTESIAN_POINT('Ctrl Pts',(15.1277727842966,15.1575922049497,121.549314887423));
#110774=CARTESIAN_POINT('Ctrl Pts',(15.4957235374569,15.3056323090703,121.479610041343));
#110775=CARTESIAN_POINT('Ctrl Pts',(16.4331684038946,15.6426929327914,121.302068450448));
#110776=CARTESIAN_POINT('Ctrl Pts',(17.0083848058396,15.8134409010177,121.193217932046));
#110777=CARTESIAN_POINT('Ctrl Pts',(18.2287678622979,16.1016131421324,120.962789861783));
#110778=CARTESIAN_POINT('Ctrl Pts',(18.8743551492525,16.2123909860811,120.841184733511));
#110779=CARTESIAN_POINT('Ctrl Pts',(19.9567726164627,16.329703915597,120.637524613471));
#110780=CARTESIAN_POINT('Ctrl Pts',(20.3904427658092,16.3587060661075,120.555980224506));
#110781=CARTESIAN_POINT('Ctrl Pts',(20.9596068191691,16.373273991557,120.448853015039));
#110782=CARTESIAN_POINT('Ctrl Pts',(21.0945190072874,16.3750000002698,120.42345180642));
#110783=CARTESIAN_POINT('Ctrl Pts',(21.2294226866078,16.375,120.398038738197));
#110784=CARTESIAN_POINT('Origin',(20.5162416486691,1.37771738462078E-14,
116.353388269));
#110785=CARTESIAN_POINT('',(21.0210448802951,16.375,119.216269432819));
#110786=CARTESIAN_POINT('',(21.0533274904221,16.375,119.399353621776));
#110787=CARTESIAN_POINT('',(20.5162416486691,16.375,116.353388269));
#110788=CARTESIAN_POINT('Ctrl Pts',(21.0533274903535,16.375,119.399353621412));
#110789=CARTESIAN_POINT('Ctrl Pts',(20.9203211694499,16.3749999997375,119.424409266478));
#110790=CARTESIAN_POINT('Ctrl Pts',(20.787310940857,16.3733222029923,119.449478733801));
#110791=CARTESIAN_POINT('Ctrl Pts',(20.223311877966,16.3590887925773,119.555818253589));
#110792=CARTESIAN_POINT('Ctrl Pts',(19.7929163837166,16.3305905185551,119.637057184513));
#110793=CARTESIAN_POINT('Ctrl Pts',(18.706310635637,16.2138830881319,119.842141607053));
#110794=CARTESIAN_POINT('Ctrl Pts',(18.0533556863278,16.1020153840184,119.965344249535));
#110795=CARTESIAN_POINT('Ctrl Pts',(16.8243375113227,15.8112481300296,120.197109812991));
#110796=CARTESIAN_POINT('Ctrl Pts',(16.2477196224269,15.639743939766,120.305795095491));
#110797=CARTESIAN_POINT('Ctrl Pts',(15.3110610197882,15.3022399929439,120.482670398818));
#110798=CARTESIAN_POINT('Ctrl Pts',(14.9451802915709,15.1548230278232,120.551868434007));
#110799=CARTESIAN_POINT('Ctrl Pts',(14.2106624607454,14.8266636041101,120.691164705906));
#110800=CARTESIAN_POINT('Ctrl Pts',(13.8427471830319,14.6449592201731,120.761101545049));
#110801=CARTESIAN_POINT('Ctrl Pts',(12.8644674178109,14.1140035657481,120.947283267502));
#110802=CARTESIAN_POINT('Ctrl Pts',(12.269071580547,13.738151853777,121.060812352906));
#110803=CARTESIAN_POINT('Ctrl Pts',(11.2092537319603,12.967388111256,121.263218700575));
#110804=CARTESIAN_POINT('Ctrl Pts',(10.7389642239055,12.582973013223,121.353178343621));
#110805=CARTESIAN_POINT('Ctrl Pts',(9.98036692713541,11.8879708463641,121.498971884623));
#110806=CARTESIAN_POINT('Ctrl Pts',(9.68074672249082,11.5911190077017,121.556786709824));
#110807=CARTESIAN_POINT('Ctrl Pts',(9.09314685787904,10.9616171643645,121.670825146726));
#110808=CARTESIAN_POINT('Ctrl Pts',(8.80639161607317,10.6282588820644,121.726790240221));
#110809=CARTESIAN_POINT('Ctrl Pts',(8.12450912160487,9.76734771833107,121.86044132184));
#110810=CARTESIAN_POINT('Ctrl Pts',(7.74695906800277,9.2264018404562,121.934962020054));
#110811=CARTESIAN_POINT('Ctrl Pts',(7.08671283228585,8.14695424881023,122.066301029016));
#110812=CARTESIAN_POINT('Ctrl Pts',(6.79929494091541,7.61272789194618,122.12397168301));
#110813=CARTESIAN_POINT('Ctrl Pts',(6.37138053991541,6.69967450997289,122.211150104128));
#110814=CARTESIAN_POINT('Ctrl Pts',(6.21420115195372,6.32962665016487,122.243579672943));
#110815=CARTESIAN_POINT('Ctrl Pts',(5.92367649377749,5.56947388984342,122.304581487186));
#110816=CARTESIAN_POINT('Ctrl Pts',(5.79108858117378,5.17937697230912,122.332983319625));
#110817=CARTESIAN_POINT('Ctrl Pts',(5.46853690991656,4.09956317065931,122.403551083865));
#110818=CARTESIAN_POINT('Ctrl Pts',(5.30838414218357,3.40155243658729,122.440384139609));
#110819=CARTESIAN_POINT('Ctrl Pts',(5.09567395443404,2.09089021655711,122.493457579947));
#110820=CARTESIAN_POINT('Ctrl Pts',(5.03105950660445,1.48155784575182,122.511874950285));
#110821=CARTESIAN_POINT('Ctrl Pts',(4.97873285833206,0.443509922682552,
122.533138202167));
#110822=CARTESIAN_POINT('Ctrl Pts',(4.97368194114913,0.0163812447033533,
122.53902856126));
#110823=CARTESIAN_POINT('Ctrl Pts',(4.99690048968756,-0.851630836139298,
122.545358757691));
#110824=CARTESIAN_POINT('Ctrl Pts',(5.02627073630446,-1.29213789742799,
122.545560310107));
#110825=CARTESIAN_POINT('Ctrl Pts',(5.14396538610984,-2.39443033312803,
122.538252324801));
#110826=CARTESIAN_POINT('Ctrl Pts',(5.25466371609234,-3.05299260799227,
122.526730519826));
#110827=CARTESIAN_POINT('Ctrl Pts',(5.54157816173008,-4.29677235990008,
122.491114630378));
#110828=CARTESIAN_POINT('Ctrl Pts',(5.71108818507745,-4.88243972612774,
122.468224727865));
#110829=CARTESIAN_POINT('Ctrl Pts',(6.04512526822682,-5.83627775691152,
122.421047016773));
#110830=CARTESIAN_POINT('Ctrl Pts',(6.19158602804546,-6.21027903407446,
122.399924203801));
#110831=CARTESIAN_POINT('Ctrl Pts',(6.51614407093082,-6.95764641941092,
122.352472395808));
#110832=CARTESIAN_POINT('Ctrl Pts',(6.6949310428006,-7.3303863901784,122.325986002426));
#110833=CARTESIAN_POINT('Ctrl Pts',(7.21973815462455,-8.32678334842395,
122.247138095185));
#110834=CARTESIAN_POINT('Ctrl Pts',(7.59235085335232,-8.93502113634534,
122.19001118376));
#110835=CARTESIAN_POINT('Ctrl Pts',(8.35488375627462,-10.0154414310004,
122.071109242689));
#110836=CARTESIAN_POINT('Ctrl Pts',(8.73416495622996,-10.4938050238189,
122.01125991514));
#110837=CARTESIAN_POINT('Ctrl Pts',(9.42063891439798,-11.2666081456444,
121.902251015821));
#110838=CARTESIAN_POINT('Ctrl Pts',(9.71440388248239,-11.5724336430292,
121.855445961392));
#110839=CARTESIAN_POINT('Ctrl Pts',(10.3359129459459,-12.1708464294893,
121.756282958297));
#110840=CARTESIAN_POINT('Ctrl Pts',(10.6642375415716,-12.4623006592341,
121.70377905762));
#110841=CARTESIAN_POINT('Ctrl Pts',(11.5152127959518,-13.1581848632437,
121.567163350992));
#110842=CARTESIAN_POINT('Ctrl Pts',(12.0512878497855,-13.5444479422492,
121.480617765594));
#110843=CARTESIAN_POINT('Ctrl Pts',(13.1194733942859,-14.2188990982748,
121.307221926128));
#110844=CARTESIAN_POINT('Ctrl Pts',(13.6472392606898,-14.5120959898824,
121.221158734329));
#110845=CARTESIAN_POINT('Ctrl Pts',(14.5483118791373,-14.9483429681753,
121.0739986727));
#110846=CARTESIAN_POINT('Ctrl Pts',(14.9129282941774,-15.1084261115253,
121.014413846435));
#110847=CARTESIAN_POINT('Ctrl Pts',(15.6632918186689,-15.4050832054591,
120.891880185983));
#110848=CARTESIAN_POINT('Ctrl Pts',(16.0490643426953,-15.5407785915894,
120.828890670378));
#110849=CARTESIAN_POINT('Ctrl Pts',(17.1147424581502,-15.870384877501,120.654673919081));
#110850=CARTESIAN_POINT('Ctrl Pts',(17.8027459788404,-16.0341829287138,
120.541942393758));
#110851=CARTESIAN_POINT('Ctrl Pts',(19.0954936622483,-16.252678919039,120.329554519236));
#110852=CARTESIAN_POINT('Ctrl Pts',(19.6970048808091,-16.3194832338718,
120.230518462596));
#110853=CARTESIAN_POINT('Ctrl Pts',(20.7212358750149,-16.374590393029,120.061954524187));
#110854=CARTESIAN_POINT('Ctrl Pts',(21.142389585171,-16.3805504838629,119.99268975654));
#110855=CARTESIAN_POINT('Ctrl Pts',(21.9990576940155,-16.3587445618759,
119.852061246133));
#110856=CARTESIAN_POINT('Ctrl Pts',(22.4341923546796,-16.3297931391106,
119.780720637706));
#110857=CARTESIAN_POINT('Ctrl Pts',(23.5215147846586,-16.2125421285139,
119.602434637965));
#110858=CARTESIAN_POINT('Ctrl Pts',(24.1705316150466,-16.1016573271302,
119.495981499937));
#110859=CARTESIAN_POINT('Ctrl Pts',(25.3969283948824,-15.8132309897795,
119.294696800569));
#110860=CARTESIAN_POINT('Ctrl Pts',(25.974736828262,-15.6424112777742,119.199810956528));
#110861=CARTESIAN_POINT('Ctrl Pts',(26.9161967631457,-15.3053081163725,
119.045529009866));
#110862=CARTESIAN_POINT('Ctrl Pts',(27.2855724649651,-15.157329304571,118.985103169793));
#110863=CARTESIAN_POINT('Ctrl Pts',(28.023240228696,-14.8295014890817,118.864808434484));
#110864=CARTESIAN_POINT('Ctrl Pts',(28.3909261992793,-14.6489844107888,
118.805010368604));
#110865=CARTESIAN_POINT('Ctrl Pts',(29.3746246089003,-14.1185207132103,
118.645248345325));
#110866=CARTESIAN_POINT('Ctrl Pts',(29.97540876194,-13.7414960737775,118.547893137023));
#110867=CARTESIAN_POINT('Ctrl Pts',(31.0423062514426,-12.9697738961824,
118.375326725267));
#110868=CARTESIAN_POINT('Ctrl Pts',(31.5145467914741,-12.5859349926871,
118.299085183482));
#110869=CARTESIAN_POINT('Ctrl Pts',(32.2777274600128,-11.8909642364878,
118.176551214403));
#110870=CARTESIAN_POINT('Ctrl Pts',(32.579864222179,-11.5934501033141,118.128271439765));
#110871=CARTESIAN_POINT('Ctrl Pts',(33.1709615602311,-10.964192702631,118.034470457708));
#110872=CARTESIAN_POINT('Ctrl Pts',(33.4588155505253,-10.6318684935042,
117.98910063556));
#110873=CARTESIAN_POINT('Ctrl Pts',(34.1465898024254,-9.76997349919565,
117.881264190221));
#110874=CARTESIAN_POINT('Ctrl Pts',(34.5285641225073,-9.22672356489209,
117.821895117977));
#110875=CARTESIAN_POINT('Ctrl Pts',(35.1955302645163,-8.14427712583293,
117.719250046472));
#110876=CARTESIAN_POINT('Ctrl Pts',(35.4854883493288,-7.60951608184327,
117.675119523227));
#110877=CARTESIAN_POINT('Ctrl Pts',(35.9170688595763,-6.6965950582735,117.610743271828));
#110878=CARTESIAN_POINT('Ctrl Pts',(36.0754759458669,-6.3272620461677,117.587517590566));
#110879=CARTESIAN_POINT('Ctrl Pts',(36.3692917044827,-5.56700589872329,
117.545485814655));
#110880=CARTESIAN_POINT('Ctrl Pts',(36.5038140735533,-5.17604479014849,
117.526799897119));
#110881=CARTESIAN_POINT('Ctrl Pts',(36.8307107840002,-4.09631466879815,
117.482849928519));
#110882=CARTESIAN_POINT('Ctrl Pts',(36.9934415693796,-3.39931804535262,
117.462736428478));
#110883=CARTESIAN_POINT('Ctrl Pts',(37.21124965804,-2.08942811743555,117.439888163318));
#110884=CARTESIAN_POINT('Ctrl Pts',(37.278236841777,-1.47982228835419,117.435103488774));
#110885=CARTESIAN_POINT('Ctrl Pts',(37.3345478505745,-0.441896543833017,
117.437209807254));
#110886=CARTESIAN_POINT('Ctrl Pts',(37.3412662450185,-0.015164752207746,
117.441020610151));
#110887=CARTESIAN_POINT('Ctrl Pts',(37.3215686369823,0.852918063577151,
117.454919165428));
#110888=CARTESIAN_POINT('Ctrl Pts',(37.2939689355986,1.29389085507792,117.465171866321));
#110889=CARTESIAN_POINT('Ctrl Pts',(37.1807860154667,2.3955744835109,117.498566385078));
#110890=CARTESIAN_POINT('Ctrl Pts',(37.0729706758541,3.05307929587065,117.525561497503));
#110891=CARTESIAN_POINT('Ctrl Pts',(36.7915305971816,4.29563864808195,117.590147220212));
#110892=CARTESIAN_POINT('Ctrl Pts',(36.6245157295591,4.88112182644342,117.626593535732));
#110893=CARTESIAN_POINT('Ctrl Pts',(36.2945461623767,5.8350860514661,117.696499034697));
#110894=CARTESIAN_POINT('Ctrl Pts',(36.1496091413967,6.20938098297544,117.726760834597));
#110895=CARTESIAN_POINT('Ctrl Pts',(35.8284391994415,6.95672849750201,117.793167678135));
#110896=CARTESIAN_POINT('Ctrl Pts',(35.6515478044601,7.3291744126154,117.829392749982));
#110897=CARTESIAN_POINT('Ctrl Pts',(35.1314933200213,8.32568537129509,117.934783053638));
#110898=CARTESIAN_POINT('Ctrl Pts',(34.7616414812724,8.93429592342269,118.008577823979));
#110899=CARTESIAN_POINT('Ctrl Pts',(34.0042853307297,10.0149854708791,118.15767702614));
#110900=CARTESIAN_POINT('Ctrl Pts',(33.6274900889191,10.4932822310832,118.231143256561));
#110901=CARTESIAN_POINT('Ctrl Pts',(32.9451361461289,11.2661552772443,118.363496099272));
#110902=CARTESIAN_POINT('Ctrl Pts',(32.6529838762402,11.5721010779937,118.420005729933));
#110903=CARTESIAN_POINT('Ctrl Pts',(32.0350733220317,12.1705056711608,118.539385402889));
#110904=CARTESIAN_POINT('Ctrl Pts',(31.7087377748204,12.4618509079776,118.602313475707));
#110905=CARTESIAN_POINT('Ctrl Pts',(30.862216626452,13.1579265271975,118.765015077745));
#110906=CARTESIAN_POINT('Ctrl Pts',(30.3285430287005,13.5444391942604,118.867100086278));
#110907=CARTESIAN_POINT('Ctrl Pts',(29.2650445871458,14.219127183877,119.069583341767));
#110908=CARTESIAN_POINT('Ctrl Pts',(28.7395943704859,14.5123461858667,119.169231411785));
#110909=CARTESIAN_POINT('Ctrl Pts',(27.8425497836647,14.9485422955191,119.339127565797));
#110910=CARTESIAN_POINT('Ctrl Pts',(27.479645681317,15.1085686088602,119.407822946635));
#110911=CARTESIAN_POINT('Ctrl Pts',(26.7326091546206,15.4052184655695,119.549321540871));
#110912=CARTESIAN_POINT('Ctrl Pts',(26.3484323068186,15.5409460642146,119.622096499745));
#110913=CARTESIAN_POINT('Ctrl Pts',(25.2874484596572,15.8705017999792,119.822867273445));
#110914=CARTESIAN_POINT('Ctrl Pts',(24.6025270182626,16.0342460851285,119.952217475419));
#110915=CARTESIAN_POINT('Ctrl Pts',(23.3152120382096,16.2527084003158,120.194762832753));
#110916=CARTESIAN_POINT('Ctrl Pts',(22.7160640075198,16.3195081607478,120.307435824552));
#110917=CARTESIAN_POINT('Ctrl Pts',(21.8305604320732,16.3673270491397,120.474021465835));
#110918=CARTESIAN_POINT('Ctrl Pts',(21.5461413107245,16.3750000005693,120.527541053192));
#110919=CARTESIAN_POINT('Ctrl Pts',(21.2617053031124,16.375,120.581122925109));
#110920=CARTESIAN_POINT('Ctrl Pts',(21.2294226866078,16.375,120.398038738197));
#110921=CARTESIAN_POINT('Ctrl Pts',(21.5134950186656,16.3749999994318,120.344525375246));
#110922=CARTESIAN_POINT('Ctrl Pts',(21.7975297616614,16.367346630148,120.290960168832));
#110923=CARTESIAN_POINT('Ctrl Pts',(22.6827331462377,16.3196009721879,120.123952511932));
#110924=CARTESIAN_POINT('Ctrl Pts',(23.2819546901568,16.2528181429115,120.010816176577));
#110925=CARTESIAN_POINT('Ctrl Pts',(24.5687969606972,16.0344811631837,119.768021711038));
#110926=CARTESIAN_POINT('Ctrl Pts',(25.2532141858301,15.8709368925073,119.639007509549));
#110927=CARTESIAN_POINT('Ctrl Pts',(26.3142694095287,15.5415672362654,119.438867076751));
#110928=CARTESIAN_POINT('Ctrl Pts',(26.6989591193503,15.4057199974352,119.366267956656));
#110929=CARTESIAN_POINT('Ctrl Pts',(27.446098706323,15.1090952657638,119.224970259076));
#110930=CARTESIAN_POINT('Ctrl Pts',(27.8086081227856,14.9492770272043,119.156232507818));
#110931=CARTESIAN_POINT('Ctrl Pts',(28.7054937632722,14.5132695459897,118.985845409194));
#110932=CARTESIAN_POINT('Ctrl Pts',(29.2311566231379,14.2199683764795,118.885727302902));
#110933=CARTESIAN_POINT('Ctrl Pts',(30.2961682586649,13.5444157137362,118.682664981306));
#110934=CARTESIAN_POINT('Ctrl Pts',(30.8310736797733,13.156992257377,118.580552014395));
#110935=CARTESIAN_POINT('Ctrl Pts',(31.6782227121215,12.4602135473578,118.41836290964));
#110936=CARTESIAN_POINT('Ctrl Pts',(32.0040804852523,12.1692646809031,118.355839149194));
#110937=CARTESIAN_POINT('Ctrl Pts',(32.6219255216258,11.5708843841068,118.236751742782));
#110938=CARTESIAN_POINT('Ctrl Pts',(32.9144108478208,11.2644938878675,118.180064331312));
#110939=CARTESIAN_POINT('Ctrl Pts',(33.5966555831746,10.4913653907742,118.047177677072));
#110940=CARTESIAN_POINT('Ctrl Pts',(33.9730740610909,10.0133124755201,117.973334340165));
#110941=CARTESIAN_POINT('Ctrl Pts',(34.7309110549308,8.93161365123495,117.823799708292));
#110942=CARTESIAN_POINT('Ctrl Pts',(35.1014474999196,8.32161139607146,117.750108148327));
#110943=CARTESIAN_POINT('Ctrl Pts',(35.6213560086873,7.32466447116878,117.645382917825));
#110944=CARTESIAN_POINT('Ctrl Pts',(35.7976539053324,6.9533107674858,117.609548510462));
#110945=CARTESIAN_POINT('Ctrl Pts',(36.1187085349124,6.20600803773903,117.543381981358));
#110946=CARTESIAN_POINT('Ctrl Pts',(36.2639492666251,5.83059064731746,117.512934325067));
#110947=CARTESIAN_POINT('Ctrl Pts',(36.5936120273196,4.87614005920006,117.442556383083));
#110948=CARTESIAN_POINT('Ctrl Pts',(36.760172508637,4.29134926168896,117.405771407614));
#110949=CARTESIAN_POINT('Ctrl Pts',(37.0402072941495,3.05350876708511,117.341202943854));
#110950=CARTESIAN_POINT('Ctrl Pts',(37.1474869706935,2.40011050524573,117.314556358608));
#110951=CARTESIAN_POINT('Ctrl Pts',(37.2611212435697,1.30076518070404,117.281740711355));
#110952=CARTESIAN_POINT('Ctrl Pts',(37.2890488080266,0.857962089651411,
117.271721981588));
#110953=CARTESIAN_POINT('Ctrl Pts',(37.3089695168339,-0.0104534301986359,
117.258060854832));
#110954=CARTESIAN_POINT('Ctrl Pts',(37.30239556291,-0.435681649274366,117.254132065725));
#110955=CARTESIAN_POINT('Ctrl Pts',(37.2464983072271,-1.47315699711677,
117.25140928359));
#110956=CARTESIAN_POINT('Ctrl Pts',(37.1795476867236,-2.0838190717909,117.255725714679));
#110957=CARTESIAN_POINT('Ctrl Pts',(36.9625138030023,-3.39095251483045,
117.278132817292));
#110958=CARTESIAN_POINT('Ctrl Pts',(36.8011462652692,-4.08425517116368,
117.298289335757));
#110959=CARTESIAN_POINT('Ctrl Pts',(36.4755879127764,-5.16374285414751,
117.342651212008));
#110960=CARTESIAN_POINT('Ctrl Pts',(36.3403113393078,-5.55790844978006,
117.361704829998));
#110961=CARTESIAN_POINT('Ctrl Pts',(36.046651535411,-6.31873447366145,117.403924538607));
#110962=CARTESIAN_POINT('Ctrl Pts',(35.889561717105,-6.68559912228108,117.426836200389));
#110963=CARTESIAN_POINT('Ctrl Pts',(35.4590773767904,-7.59812727527399,
117.490510771011));
#110964=CARTESIAN_POINT('Ctrl Pts',(35.1685081090666,-8.13480279741698,
117.534295347848));
#110965=CARTESIAN_POINT('Ctrl Pts',(34.4960675767682,-9.22738818677147,
117.637475357967));
#110966=CARTESIAN_POINT('Ctrl Pts',(34.1084526938852,-9.77833358789352,
117.697935793953));
#110967=CARTESIAN_POINT('Ctrl Pts',(33.416383995336,-10.6436219415005,117.807101069928));
#110968=CARTESIAN_POINT('Ctrl Pts',(33.131012518227,-10.9725954024996,117.852392309609));
#110969=CARTESIAN_POINT('Ctrl Pts',(32.539977143262,-11.6012786268155,117.94646524767));
#110970=CARTESIAN_POINT('Ctrl Pts',(32.2349583370586,-11.9011408908722,
117.995094008439));
#110971=CARTESIAN_POINT('Ctrl Pts',(31.4699808953676,-12.5960909724161,
118.117376241431));
#110972=CARTESIAN_POINT('Ctrl Pts',(30.9992033483422,-12.9779742156819,
118.192942771545));
#110973=CARTESIAN_POINT('Ctrl Pts',(29.9250603095167,-13.7537834162604,
118.366353178728));
#110974=CARTESIAN_POINT('Ctrl Pts',(29.3146540222838,-14.135455454452,118.46552758637));
#110975=CARTESIAN_POINT('Ctrl Pts',(28.327869273885,-14.664258237489,118.62645404104));
#110976=CARTESIAN_POINT('Ctrl Pts',(27.9676056914279,-14.8403204286184,
118.685312586953));
#110977=CARTESIAN_POINT('Ctrl Pts',(27.2292288878491,-15.1675370351931,
118.805941883212));
#110978=CARTESIAN_POINT('Ctrl Pts',(26.8511828923902,-15.3181436920486,
118.86766342998));
#110979=CARTESIAN_POINT('Ctrl Pts',(25.9055255215102,-15.6537839281739,
119.022116858353));
#110980=CARTESIAN_POINT('Ctrl Pts',(25.3326509320719,-15.8217348348208,
119.115777143231));
#110981=CARTESIAN_POINT('Ctrl Pts',(24.0065756121728,-16.1312006587827,
119.333123395314));
#110982=CARTESIAN_POINT('Ctrl Pts',(23.2499989853418,-16.2513106809087,
119.457537478582));
#110983=CARTESIAN_POINT('Ctrl Pts',(22.1227437429084,-16.3479883612805,
119.643070487807));
#110984=CARTESIAN_POINT('Ctrl Pts',(21.7566465286155,-16.3667080583793,
119.703340805535));
#110985=CARTESIAN_POINT('Ctrl Pts',(20.8509494577884,-16.3817609729779,
119.85227071464));
#110986=CARTESIAN_POINT('Ctrl Pts',(20.3115332160797,-16.3633578094981,
119.940752286598));
#110987=CARTESIAN_POINT('Ctrl Pts',(19.0644156927292,-16.2573254768737,
120.145251878545));
#110988=CARTESIAN_POINT('Ctrl Pts',(18.3595019569084,-16.1495300631213,
120.260835762513));
#110989=CARTESIAN_POINT('Ctrl Pts',(17.0462771970741,-15.8577388354913,
120.476353311716));
#110990=CARTESIAN_POINT('Ctrl Pts',(16.4371244339281,-15.6838853730086,
120.576395890592));
#110991=CARTESIAN_POINT('Ctrl Pts',(15.4086815197983,-15.3231972943878,
120.744975702729));
#110992=CARTESIAN_POINT('Ctrl Pts',(14.984286088183,-15.1536732490818,120.814411242365));
#110993=CARTESIAN_POINT('Ctrl Pts',(14.019459617361,-14.7196821609465,120.971700053072));
#110994=CARTESIAN_POINT('Ctrl Pts',(13.4853391346778,-14.4424664880218,
121.05844865307));
#110995=CARTESIAN_POINT('Ctrl Pts',(12.4106527360227,-13.8059228770537,
121.232750503302));
#110996=CARTESIAN_POINT('Ctrl Pts',(11.8736392465029,-13.4425311238772,
121.319713505817));
#110997=CARTESIAN_POINT('Ctrl Pts',(10.8962105912107,-12.6917782189329,
121.477620651626));
#110998=CARTESIAN_POINT('Ctrl Pts',(10.4522088180043,-12.3109009030544,
121.549177682248));
#110999=CARTESIAN_POINT('Ctrl Pts',(9.7323682879697,-11.6227014300553,121.664410347319));
#111000=CARTESIAN_POINT('Ctrl Pts',(9.44606700080452,-11.3274815466299,
121.709959799127));
#111001=CARTESIAN_POINT('Ctrl Pts',(8.44457766653677,-10.2135459013248,
121.868335081255));
#111002=CARTESIAN_POINT('Ctrl Pts',(7.79952923274599,-9.3338974006903,121.968794657567));
#111003=CARTESIAN_POINT('Ctrl Pts',(6.98470864934987,-7.95388116015941,
122.093722028873));
#111004=CARTESIAN_POINT('Ctrl Pts',(6.74444855758325,-7.49973829971881,
122.130172937738));
#111005=CARTESIAN_POINT('Ctrl Pts',(6.35676924302653,-6.67615368529231,
122.187960184991));
#111006=CARTESIAN_POINT('Ctrl Pts',(6.20080184169789,-6.31130816008181,
122.210811075314));
#111007=CARTESIAN_POINT('Ctrl Pts',(5.90711967765701,-5.54973986342869,
122.252802015243));
#111008=CARTESIAN_POINT('Ctrl Pts',(5.77107244244981,-5.15267225547731,
122.271679117935));
#111009=CARTESIAN_POINT('Ctrl Pts',(5.44648629185545,-4.07332177614223,
122.315236415625));
#111010=CARTESIAN_POINT('Ctrl Pts',(5.28625235340208,-3.38326786220082,
122.33500205284));
#111011=CARTESIAN_POINT('Ctrl Pts',(5.07001927447514,-2.07846844334889,
122.357637112328));
#111012=CARTESIAN_POINT('Ctrl Pts',(5.00325407383151,-1.46679183650972,
122.362360869277));
#111013=CARTESIAN_POINT('Ctrl Pts',(4.9479330168173,-0.429702895801508,
122.360087896895));
#111014=CARTESIAN_POINT('Ctrl Pts',(4.94153372538027,-0.00588754931961123,
122.356252426584));
#111015=CARTESIAN_POINT('Ctrl Pts',(4.96158031325555,0.862936647225923,
122.342281629526));
#111016=CARTESIAN_POINT('Ctrl Pts',(4.98972630475043,1.30755231507119,122.331887164767));
#111017=CARTESIAN_POINT('Ctrl Pts',(5.10874054183148,2.45421185624014,122.296916007331));
#111018=CARTESIAN_POINT('Ctrl Pts',(5.22667370910118,3.152369041336,122.267652327832));
#111019=CARTESIAN_POINT('Ctrl Pts',(5.53647173456419,4.46763733519119,122.197199906973));
#111020=CARTESIAN_POINT('Ctrl Pts',(5.72058753228943,5.08529560591196,122.15735274927));
#111021=CARTESIAN_POINT('Ctrl Pts',(6.06783396324989,6.04232408048288,122.084251450398));
#111022=CARTESIAN_POINT('Ctrl Pts',(6.20746183008263,6.38981961711627,122.055196857674));
#111023=CARTESIAN_POINT('Ctrl Pts',(6.56731607752931,7.20417263369571,121.980998791448));
#111024=CARTESIAN_POINT('Ctrl Pts',(6.79783575642474,7.66587204476267,121.934030527408));
#111025=CARTESIAN_POINT('Ctrl Pts',(7.35679082933926,8.66475997968274,121.821582389694));
#111026=CARTESIAN_POINT('Ctrl Pts',(7.69513997257765,9.19526362312,121.754408161279));
#111027=CARTESIAN_POINT('Ctrl Pts',(8.45821567499527,10.2519815156924,121.604552448363));
#111028=CARTESIAN_POINT('Ctrl Pts',(8.88677888690755,10.7738515475117,121.521233898674));
#111029=CARTESIAN_POINT('Ctrl Pts',(9.63158800698643,11.5738169376985,121.37703187855));
#111030=CARTESIAN_POINT('Ctrl Pts',(9.92874292365523,11.8691743884886,121.319581877576));
#111031=CARTESIAN_POINT('Ctrl Pts',(11.0050331535403,12.859006320224,121.11192815584));
#111032=CARTESIAN_POINT('Ctrl Pts',(11.8386494501844,13.4883431855134,120.952137861313));
#111033=CARTESIAN_POINT('Ctrl Pts',(13.2599293459805,14.3585888964025,120.681820147208));
#111034=CARTESIAN_POINT('Ctrl Pts',(13.8120274687105,14.6536137994961,120.577218345849));
#111035=CARTESIAN_POINT('Ctrl Pts',(14.7577228673034,15.0896958540015,120.398154731455));
#111036=CARTESIAN_POINT('Ctrl Pts',(15.1423785142069,15.2491169886058,120.325302905041));
#111037=CARTESIAN_POINT('Ctrl Pts',(16.5514679300861,15.7693902158067,120.05841558232));
#111038=CARTESIAN_POINT('Ctrl Pts',(17.6050970628226,16.0398471248037,119.859235114274));
#111039=CARTESIAN_POINT('Ctrl Pts',(19.2551233974631,16.2869590738737,119.548520591475));
#111040=CARTESIAN_POINT('Ctrl Pts',(19.8369249065093,16.3414155687272,119.439137578772));
#111041=CARTESIAN_POINT('Ctrl Pts',(20.6204999588461,16.3711961105069,119.291694285519));
#111042=CARTESIAN_POINT('Ctrl Pts',(20.820774550801,16.3750000004889,119.253996228967));
#111043=CARTESIAN_POINT('Ctrl Pts',(21.0210448803799,16.375,119.216269433269));
#111044=CARTESIAN_POINT('Origin',(20.5162416486691,1.37771738462078E-14,
116.353388269));
#111045=CARTESIAN_POINT('',(20.8126670601567,16.375,118.034500130595));
#111046=CARTESIAN_POINT('',(20.8449496768525,16.375,118.217584318235));
#111047=CARTESIAN_POINT('',(20.5162416486691,16.375,116.353388269));
#111048=CARTESIAN_POINT('',(4.53968745634911,0.597925404686674,119.982827120865));
#111049=CARTESIAN_POINT('Ctrl Pts',(20.8126670602263,16.375,118.034500130964));
#111050=CARTESIAN_POINT('Ctrl Pts',(20.9474177181623,16.3749999997303,118.009115888811));
#111051=CARTESIAN_POINT('Ctrl Pts',(21.0821721364041,16.3732779069003,117.983717507935));
#111052=CARTESIAN_POINT('Ctrl Pts',(21.650889271568,16.3587371251268,117.876487402412));
#111053=CARTESIAN_POINT('Ctrl Pts',(22.0842445742341,16.3297758982501,117.794689003852));
#111054=CARTESIAN_POINT('Ctrl Pts',(23.1668893823753,16.2125130218164,117.590352245407));
#111055=CARTESIAN_POINT('Ctrl Pts',(23.8130331065345,16.1016489691972,117.46843539781));
#111056=CARTESIAN_POINT('Ctrl Pts',(25.0341491046181,15.8132717274978,117.238159551688));
#111057=CARTESIAN_POINT('Ctrl Pts',(25.6095397444326,15.6424660168222,117.129705583372));
#111058=CARTESIAN_POINT('Ctrl Pts',(26.5470071663356,15.3053708438713,116.952681815915));
#111059=CARTESIAN_POINT('Ctrl Pts',(26.9148128865843,15.1573802795131,116.883122229806));
#111060=CARTESIAN_POINT('Ctrl Pts',(27.6491346185028,14.8295584874304,116.743865582365));
#111061=CARTESIAN_POINT('Ctrl Pts',(28.0150594719487,14.649065175926,116.674308838569));
#111062=CARTESIAN_POINT('Ctrl Pts',(28.9940906684615,14.1186111085074,116.487988551128));
#111063=CARTESIAN_POINT('Ctrl Pts',(29.5919901526024,13.741562699019,116.373982795026));
#111064=CARTESIAN_POINT('Ctrl Pts',(30.6536029107296,12.9698207503721,116.171234920188));
#111065=CARTESIAN_POINT('Ctrl Pts',(31.1234311515611,12.5859931310865,116.081364469071));
#111066=CARTESIAN_POINT('Ctrl Pts',(31.8825047789103,11.8910228713346,115.935483873129));
#111067=CARTESIAN_POINT('Ctrl Pts',(32.1829490827144,11.5934956373737,115.877512122518));
#111068=CARTESIAN_POINT('Ctrl Pts',(32.7704796731808,10.9642426798957,115.763489259629));
#111069=CARTESIAN_POINT('Ctrl Pts',(33.0564769270319,10.6319385041319,115.707673930753));
#111070=CARTESIAN_POINT('Ctrl Pts',(33.7396809151958,9.77002416324843,115.573769532027));
#111071=CARTESIAN_POINT('Ctrl Pts',(34.1189578101089,9.22672926659155,115.498908795801));
#111072=CARTESIAN_POINT('Ctrl Pts',(34.7808389790396,8.14422413452029,115.367241465105));
#111073=CARTESIAN_POINT('Ctrl Pts',(35.0684069028315,7.6094524801085,115.309538456126));
#111074=CARTESIAN_POINT('Ctrl Pts',(35.4959711448949,6.69653397773241,115.222424356109));
#111075=CARTESIAN_POINT('Ctrl Pts',(35.6527612389367,6.32721504158711,115.19007244426));
#111076=CARTESIAN_POINT('Ctrl Pts',(35.9432324953718,5.56695659646977,115.129078624169));
#111077=CARTESIAN_POINT('Ctrl Pts',(36.0760373863462,5.17597820217734,115.100627313078));
#111078=CARTESIAN_POINT('Ctrl Pts',(36.3982448654725,4.09624968022862,115.030122748054));
#111079=CARTESIAN_POINT('Ctrl Pts',(36.5580338919987,3.39927326271342,114.993367571957));
#111080=CARTESIAN_POINT('Ctrl Pts',(36.7705166607077,2.08939865451389,114.940344142336));
#111081=CARTESIAN_POINT('Ctrl Pts',(36.8350998608482,1.47978730816307,114.921929350359));
#111082=CARTESIAN_POINT('Ctrl Pts',(36.8872918374902,0.441864000461987,
114.900691051595));
#111083=CARTESIAN_POINT('Ctrl Pts',(36.8923008642108,0.0151401879435104,
114.894812474543));
#111084=CARTESIAN_POINT('Ctrl Pts',(36.8690366745017,-0.852944119966995,
114.888489220714));
#111085=CARTESIAN_POINT('Ctrl Pts',(36.8395933574814,-1.29392634435125,
114.88829462536));
#111086=CARTESIAN_POINT('Ctrl Pts',(36.7218128980036,-2.3955976960719,114.895625332039));
#111087=CARTESIAN_POINT('Ctrl Pts',(36.6112698181393,-3.05308114401722,
114.907132961835));
#111088=CARTESIAN_POINT('Ctrl Pts',(36.3247202460831,-4.29561586371514,
114.942699434511));
#111089=CARTESIAN_POINT('Ctrl Pts',(36.1553142818853,-4.88109534446592,
114.965573232676));
#111090=CARTESIAN_POINT('Ctrl Pts',(35.821336386373,-5.83506212042791,115.012739566429));
#111091=CARTESIAN_POINT('Ctrl Pts',(35.6747882667282,-6.20936296421926,
115.033874394396));
#111092=CARTESIAN_POINT('Ctrl Pts',(35.3502756418419,-6.95671011401383,
115.081318820238));
#111093=CARTESIAN_POINT('Ctrl Pts',(35.1716658764011,-7.32915014280427,
115.107778279266));
#111094=CARTESIAN_POINT('Ctrl Pts',(34.6469303075316,-8.32566339425024,
115.186612632623));
#111095=CARTESIAN_POINT('Ctrl Pts',(34.2741404840464,-8.93428141835405,
115.243765521066));
#111096=CARTESIAN_POINT('Ctrl Pts',(33.5114606724523,-10.0149763697651,
115.362689596489));
#111097=CARTESIAN_POINT('Ctrl Pts',(33.1322636807448,-10.4932717967061,
115.422525216352));
#111098=CARTESIAN_POINT('Ctrl Pts',(32.4457934481117,-11.2661462413179,
115.531532998563));
#111099=CARTESIAN_POINT('Ctrl Pts',(32.1519307699161,-11.5720944452931,
115.578353581029));
#111100=CARTESIAN_POINT('Ctrl Pts',(31.5304551765431,-12.1704988814298,
115.677511134126));
#111101=CARTESIAN_POINT('Ctrl Pts',(31.2022803271675,-12.4618419469874,
115.729990948659));
#111102=CARTESIAN_POINT('Ctrl Pts',(30.3511605977657,-13.157921384732,115.866629179193));
#111103=CARTESIAN_POINT('Ctrl Pts',(29.8147497618534,-13.5444390282589,
115.953228827373));
#111104=CARTESIAN_POINT('Ctrl Pts',(28.7461262048072,-14.2191317412877,
116.126696092821));
#111105=CARTESIAN_POINT('Ctrl Pts',(28.2182813178402,-14.5123511853317,
116.212772351232));
#111106=CARTESIAN_POINT('Ctrl Pts',(27.3172276003375,-14.9485462795208,
116.359929449445));
#111107=CARTESIAN_POINT('Ctrl Pts',(26.952716143915,-15.108571457968,116.419497083543));
#111108=CARTESIAN_POINT('Ctrl Pts',(26.2023357266079,-15.4052211718541,
116.542033493345));
#111109=CARTESIAN_POINT('Ctrl Pts',(25.8164345516943,-15.5409494151087,
116.605044034577));
#111110=CARTESIAN_POINT('Ctrl Pts',(24.7507684449807,-15.8705041398745,
116.779259033408));
#111111=CARTESIAN_POINT('Ctrl Pts',(24.0629153966277,-16.0342473494753,
116.891966052128));
#111112=CARTESIAN_POINT('Ctrl Pts',(22.7702818479534,-16.2527089909263,
117.104335257787));
#111113=CARTESIAN_POINT('Ctrl Pts',(22.1687296264827,-16.3195086601159,
117.203378107608));
#111114=CARTESIAN_POINT('Ctrl Pts',(21.144516765698,-16.3745954429001,117.371939026216));
#111115=CARTESIAN_POINT('Ctrl Pts',(20.7234223841939,-16.3805490893052,
117.441193985326));
#111116=CARTESIAN_POINT('Ctrl Pts',(19.8667432377462,-16.3587362640687,
117.581824272215));
#111117=CARTESIAN_POINT('Ctrl Pts',(19.4315384842745,-16.3297739019914,
117.65317635399));
#111118=CARTESIAN_POINT('Ctrl Pts',(18.3443073251155,-16.2125096513466,
117.831447390598));
#111119=CARTESIAN_POINT('Ctrl Pts',(17.6954492902166,-16.1016479997975,
117.937874497409));
#111120=CARTESIAN_POINT('Ctrl Pts',(16.4692356109282,-15.8132764386314,
118.13912913472));
#111121=CARTESIAN_POINT('Ctrl Pts',(15.8914546814622,-15.6424723469864,
118.234010461954));
#111122=CARTESIAN_POINT('Ctrl Pts',(14.9499758033932,-15.3053780972287,
118.388295607853));
#111123=CARTESIAN_POINT('Ctrl Pts',(14.5805561449671,-15.157386173201,118.448728694602));
#111124=CARTESIAN_POINT('Ctrl Pts',(13.8428911356548,-14.8295650756713,
118.569023034157));
#111125=CARTESIAN_POINT('Ctrl Pts',(13.47524898342,-14.6490745110845,118.628814011724));
#111126=CARTESIAN_POINT('Ctrl Pts',(12.4915335346939,-14.1186215561567,
118.788578899634));
#111127=CARTESIAN_POINT('Ctrl Pts',(11.890693774203,-13.7415703986437,118.885943134522));
#111128=CARTESIAN_POINT('Ctrl Pts',(10.8237560746531,-12.9698261634361,
119.058516077216));
#111129=CARTESIAN_POINT('Ctrl Pts',(10.3515254677957,-12.5859998477385,
119.134756035788));
#111130=CARTESIAN_POINT('Ctrl Pts',(9.58833440215207,-11.8910296450469,
119.25729176993));
#111131=CARTESIAN_POINT('Ctrl Pts',(9.28617974718461,-11.5935008973214,
119.30557444827));
#111132=CARTESIAN_POINT('Ctrl Pts',(8.69508359286318,-10.9642484522917,
119.399375287481));
#111133=CARTESIAN_POINT('Ctrl Pts',(8.40724579345633,-10.6319465903103,
119.44474259634));
#111134=CARTESIAN_POINT('Ctrl Pts',(7.71944310032966,-9.77003001425979,
119.552583621157));
#111135=CARTESIAN_POINT('Ctrl Pts',(7.33743167938567,-9.2267299238087,119.611958476547));
#111136=CARTESIAN_POINT('Ctrl Pts',(6.6704303008902,-8.14421801142984,119.714608904431));
#111137=CARTESIAN_POINT('Ctrl Pts',(6.38046891117741,-7.60944513092628,
119.758739882301));
#111138=CARTESIAN_POINT('Ctrl Pts',(5.94889595319164,-6.69652691962459,
119.823114856413));
#111139=CARTESIAN_POINT('Ctrl Pts',(5.79049732980452,-6.32720960975904,
119.846339239568));
#111140=CARTESIAN_POINT('Ctrl Pts',(5.49668262775027,-5.5669508985232,119.888370794844));
#111141=CARTESIAN_POINT('Ctrl Pts',(5.36215542994127,-5.1759705064359,119.907057318389));
#111142=CARTESIAN_POINT('Ctrl Pts',(5.04268487019767,-4.12074621802567,
119.950008615385));
#111143=CARTESIAN_POINT('Ctrl Pts',(4.88425103526154,-3.44916259355946,
119.969665869807));
#111144=CARTESIAN_POINT('Ctrl Pts',(4.67427441302864,-2.2214623544002,119.992076449368));
#111145=CARTESIAN_POINT('Ctrl Pts',(4.60811190145251,-1.66895874402597,
119.997342580495));
#111146=CARTESIAN_POINT('Ctrl Pts',(4.54679574234008,-0.782153931310234,
119.99788609547));
#111147=CARTESIAN_POINT('Ctrl Pts',(4.53381034943788,-0.449528224858523,
119.996321834545));
#111148=CARTESIAN_POINT('Ctrl Pts',(4.5286489093189,0.121525185001767,119.990497869703));
#111149=CARTESIAN_POINT('Ctrl Pts',(4.53161016399367,0.359801506295293,
119.987124333779));
#111150=CARTESIAN_POINT('Ctrl Pts',(4.53968745733423,0.597925404661066,
119.982827121192));
#111151=CARTESIAN_POINT('',(12.1252604242132,13.8967357372103,118.645285943241));
#111152=CARTESIAN_POINT('Origin',(20.6551601908026,1.37771738462078E-14,
117.14123447141));
#111153=CARTESIAN_POINT('Ctrl Pts',(12.1252604242941,13.8967357370058,118.645285942984));
#111154=CARTESIAN_POINT('Ctrl Pts',(11.1597404820724,13.284169320124,118.829378902758));
#111155=CARTESIAN_POINT('Ctrl Pts',(10.2608304550041,12.5690806535172,119.000961473646));
#111156=CARTESIAN_POINT('Ctrl Pts',(9.14198063508577,11.4657858073982,119.216854573139));
#111157=CARTESIAN_POINT('Ctrl Pts',(8.85173726715739,11.1561735043244,119.273187269843));
#111158=CARTESIAN_POINT('Ctrl Pts',(8.18795432151583,10.3900038555159,119.402623091456));
#111159=CARTESIAN_POINT('Ctrl Pts',(7.8262818696854,9.92361049551718,119.473627072773));
#111160=CARTESIAN_POINT('Ctrl Pts',(7.10391730568458,8.87989942007041,119.616258849931));
#111161=CARTESIAN_POINT('Ctrl Pts',(6.75224905246574,8.29746930661533,119.686228287655));
#111162=CARTESIAN_POINT('Ctrl Pts',(6.24680245725592,7.32914896187816,119.788031668799));
#111163=CARTESIAN_POINT('Ctrl Pts',(6.06986816280178,6.95670904209967,119.823992462004));
#111164=CARTESIAN_POINT('Ctrl Pts',(5.74866154596584,6.20936180049674,119.89018632596));
#111165=CARTESIAN_POINT('Ctrl Pts',(5.60374227229688,5.83505890408794,119.920562562136));
#111166=CARTESIAN_POINT('Ctrl Pts',(5.27386443097109,4.88109619671092,119.990972901856));
#111167=CARTESIAN_POINT('Ctrl Pts',(5.10692456055938,4.29561579219025,120.02783470883));
#111168=CARTESIAN_POINT('Ctrl Pts',(4.82554189788938,3.05308386956103,120.092700235354));
#111169=CARTESIAN_POINT('Ctrl Pts',(4.71769400230651,2.39560152362369,120.119494173849));
#111170=CARTESIAN_POINT('Ctrl Pts',(4.60440066759678,1.29392655010024,120.152275258206));
#111171=CARTESIAN_POINT('Ctrl Pts',(4.57674612282201,0.852944098403716,
120.162225201117));
#111172=CARTESIAN_POINT('Ctrl Pts',(4.55699972666702,-0.015140709895495,
120.175852535511));
#111173=CARTESIAN_POINT('Ctrl Pts',(4.56373655386578,-0.441866353833341,
120.179771808684));
#111174=CARTESIAN_POINT('Ctrl Pts',(4.62013871523287,-1.47978496496699,
120.182412432585));
#111175=CARTESIAN_POINT('Ctrl Pts',(4.68720199259863,-2.08939756486391,
120.178062862687));
#111176=CARTESIAN_POINT('Ctrl Pts',(4.90506234807178,-3.39926685260381,
120.155542619496));
#111177=CARTESIAN_POINT('Ctrl Pts',(5.06774326451499,-4.09623968274988,
120.135196923117));
#111178=CARTESIAN_POINT('Ctrl Pts',(5.39452380613574,-5.17597163856225,
120.090625419194));
#111179=CARTESIAN_POINT('Ctrl Pts',(5.5290045520822,-5.56695189759738,120.071675329381));
#111180=CARTESIAN_POINT('Ctrl Pts',(5.82278177455425,-6.32721069485949,
120.02943094923));
#111181=CARTESIAN_POINT('Ctrl Pts',(5.981201450926,-6.69652989050191,120.006320353581));
#111182=CARTESIAN_POINT('Ctrl Pts',(6.41286169276523,-7.60944416923135,
119.942450985857));
#111183=CARTESIAN_POINT('Ctrl Pts',(6.70289680019166,-8.14421798124779,
119.898735768352));
#111184=CARTESIAN_POINT('Ctrl Pts',(7.36994640105912,-9.22672754721024,
119.796367060064));
#111185=CARTESIAN_POINT('Ctrl Pts',(7.75192164063493,-9.77002708947801,
119.736791934498));
#111186=CARTESIAN_POINT('Ctrl Pts',(8.43961838140779,-10.6319465874527,
119.628336841119));
#111187=CARTESIAN_POINT('Ctrl Pts',(8.72740287301182,-10.9642485591961,
119.582666383961));
#111188=CARTESIAN_POINT('Ctrl Pts',(9.31845149407982,-11.5935013725925,
119.488594078722));
#111189=CARTESIAN_POINT('Ctrl Pts',(9.62062669594056,-11.8910313192151,
119.440419583059));
#111190=CARTESIAN_POINT('Ctrl Pts',(10.3839084183464,-12.5859984183609,
119.31841826376));
#111191=CARTESIAN_POINT('Ctrl Pts',(10.8562165720411,-12.9698255988242,
119.242613096732));
#111192=CARTESIAN_POINT('Ctrl Pts',(11.9232076920776,-13.7415667711839,
119.070368167729));
#111193=CARTESIAN_POINT('Ctrl Pts',(12.5240028290975,-14.1186165143113,
118.972771085672));
#111194=CARTESIAN_POINT('Ctrl Pts',(13.5076111657763,-14.6490716247697,
118.812383115556));
#111195=CARTESIAN_POINT('Ctrl Pts',(13.8752084354256,-14.8295630895892,
118.752328316877));
#111196=CARTESIAN_POINT('Ctrl Pts',(14.6128361148113,-15.1573844703328,
118.631821127168));
#111197=CARTESIAN_POINT('Ctrl Pts',(14.9822761825338,-15.3053765391856,
118.571501918693));
#111198=CARTESIAN_POINT('Ctrl Pts',(15.9238394137623,-15.6424696484626,
118.417722887415));
#111199=CARTESIAN_POINT('Ctrl Pts',(16.5016956420056,-15.8132747098046,
118.323257057273));
#111200=CARTESIAN_POINT('Ctrl Pts',(17.7279633038988,-16.1016477112175,
118.122283213894));
#111201=CARTESIAN_POINT('Ctrl Pts',(18.3767910765389,-16.2125104624114,
118.015654863716));
#111202=CARTESIAN_POINT('Ctrl Pts',(19.4639211362957,-16.3297746553102,
117.836768941188));
#111203=CARTESIAN_POINT('Ctrl Pts',(19.8990699440025,-16.3587365764383,
117.765114145799));
#111204=CARTESIAN_POINT('Ctrl Pts',(20.7557012960041,-16.3805491665361,
117.624212435363));
#111205=CARTESIAN_POINT('Ctrl Pts',(21.1768189028637,-16.3745950976222,
117.555065216385));
#111206=CARTESIAN_POINT('Ctrl Pts',(22.2011219655674,-16.3195078331578,
117.387038803892));
#111207=CARTESIAN_POINT('Ctrl Pts',(22.802750521889,-16.2527079846344,117.288430938992));
#111208=CARTESIAN_POINT('Ctrl Pts',(24.0954409527593,-16.0342459459005,
117.076389188818));
#111209=CARTESIAN_POINT('Ctrl Pts',(24.7832551297753,-15.8705021323465,
116.963448374861));
#111210=CARTESIAN_POINT('Ctrl Pts',(25.8488152966293,-15.540945051873,116.788610097004));
#111211=CARTESIAN_POINT('Ctrl Pts',(26.2346668537666,-15.4052175567522,
116.725336512761));
#111212=CARTESIAN_POINT('Ctrl Pts',(26.9850094295564,-15.1085676258394,
116.602587340136));
#111213=CARTESIAN_POINT('Ctrl Pts',(27.3495452913619,-14.9485401179305,
116.543132938794));
#111214=CARTESIAN_POINT('Ctrl Pts',(28.2506846722699,-14.5123456509191,
116.39648174634));
#111215=CARTESIAN_POINT('Ctrl Pts',(28.7786019485646,-14.2191263330367,
116.310821457708));
#111216=CARTESIAN_POINT('Ctrl Pts',(29.8472625934313,-13.5444406910131,
116.137637731149));
#111217=CARTESIAN_POINT('Ctrl Pts',(30.3836297116358,-13.1579298455225,
116.050839028838));
#111218=CARTESIAN_POINT('Ctrl Pts',(31.2346407361918,-12.4618526787663,
115.913587153723));
#111219=CARTESIAN_POINT('Ctrl Pts',(31.5627657366584,-12.170506877048,115.860803629732));
#111220=CARTESIAN_POINT('Ctrl Pts',(32.1841946087007,-11.5721019248384,
115.761374473169));
#111221=CARTESIAN_POINT('Ctrl Pts',(32.4780753003173,-11.2661551418455,
115.714662472521));
#111222=CARTESIAN_POINT('Ctrl Pts',(33.1646366834815,-10.4932858878529,
115.606189000377));
#111223=CARTESIAN_POINT('Ctrl Pts',(33.5439131870178,-10.0149880007349,
115.546787858102));
#111224=CARTESIAN_POINT('Ctrl Pts',(34.3066442306287,-8.93430385228874,
115.428192098782));
#111225=CARTESIAN_POINT('Ctrl Pts',(34.6793873416775,-8.32569826259176,
115.370806625637));
#111226=CARTESIAN_POINT('Ctrl Pts',(35.204016922313,-7.32918503662734,115.291348976133));
#111227=CARTESIAN_POINT('Ctrl Pts',(35.3825852556302,-6.95673636736924,
115.264625178516));
#111228=CARTESIAN_POINT('Ctrl Pts',(35.7070616810594,-6.20938858312028,
115.216967707811));
#111229=CARTESIAN_POINT('Ctrl Pts',(35.8536279703331,-5.83509447451018,
115.19594705851));
#111230=CARTESIAN_POINT('Ctrl Pts',(36.187695220726,-4.88113555837382,115.149285921989));
#111231=CARTESIAN_POINT('Ctrl Pts',(36.3571779127582,-4.2956496577634,115.126827433441));
#111232=CARTESIAN_POINT('Ctrl Pts',(36.6437871634858,-3.05308112414139,
115.091541124607));
#111233=CARTESIAN_POINT('Ctrl Pts',(36.7542996631356,-2.39556702471343,
115.079832600655));
#111234=CARTESIAN_POINT('Ctrl Pts',(36.8719698247605,-1.29387380383542,
115.071888789447));
#111235=CARTESIAN_POINT('Ctrl Pts',(36.9013575233924,-0.852905371791337,
115.071780486834));
#111236=CARTESIAN_POINT('Ctrl Pts',(36.9245725434912,0.015177219437159,
115.077832544763));
#111237=CARTESIAN_POINT('Ctrl Pts',(36.9195812409251,0.441914723418851,
115.083819955621));
#111238=CARTESIAN_POINT('Ctrl Pts',(36.8674797434211,1.47983695648695,115.105592757666));
#111239=CARTESIAN_POINT('Ctrl Pts',(36.8029723157261,2.08944135597091,115.124442549207));
#111240=CARTESIAN_POINT('Ctrl Pts',(36.5905415507011,3.39933341551244,115.17779451164));
#111241=CARTESIAN_POINT('Ctrl Pts',(36.4307022732685,4.09633627939259,115.214318174334));
#111242=CARTESIAN_POINT('Ctrl Pts',(36.1083746625847,5.17607061333654,115.2842020038));
#111243=CARTESIAN_POINT('Ctrl Pts',(35.9755291125928,5.56702517943654,115.312388455803));
#111244=CARTESIAN_POINT('Ctrl Pts',(35.6850189760879,6.32728056310422,115.373169684351));
#111245=CARTESIAN_POINT('Ctrl Pts',(35.5282377047074,6.69662068296697,115.405637822536));
#111246=CARTESIAN_POINT('Ctrl Pts',(35.1007551184061,7.60953870969189,115.493258627251));
#111247=CARTESIAN_POINT('Ctrl Pts',(34.8132641225272,8.14429674990551,115.551376637967));
#111248=CARTESIAN_POINT('Ctrl Pts',(34.1514769290961,9.22671906732955,115.683316502601));
#111249=CARTESIAN_POINT('Ctrl Pts',(33.7722108273899,9.76995177071023,115.757967809877));
#111250=CARTESIAN_POINT('Ctrl Pts',(33.0889311609431,10.6318425093477,115.891252325604));
#111251=CARTESIAN_POINT('Ctrl Pts',(32.8028605527277,10.9641742629319,115.946768419396));
#111252=CARTESIAN_POINT('Ctrl Pts',(32.2152803445484,11.5934336842087,116.060520228445));
#111253=CARTESIAN_POINT('Ctrl Pts',(31.914875607173,11.8909441565963,116.118596438801));
#111254=CARTESIAN_POINT('Ctrl Pts',(31.1559123088391,12.5859119951017,116.265007843428));
#111255=CARTESIAN_POINT('Ctrl Pts',(30.6861477754281,12.9697559499969,116.355315778851));
#111256=CARTESIAN_POINT('Ctrl Pts',(29.624646174555,13.7414677420151,116.558380839602));
#111257=CARTESIAN_POINT('Ctrl Pts',(29.0267769981518,14.1184821586303,116.672139714958));
#111258=CARTESIAN_POINT('Ctrl Pts',(28.0476542264764,14.6489515843629,116.857834058432));
#111259=CARTESIAN_POINT('Ctrl Pts',(27.6816277312548,14.8294783740573,116.927137694783));
#111260=CARTESIAN_POINT('Ctrl Pts',(26.9472648962211,15.1573087139211,117.066182193985));
#111261=CARTESIAN_POINT('Ctrl Pts',(26.5795327025556,15.3052833195346,117.135845559782));
#111262=CARTESIAN_POINT('Ctrl Pts',(25.6421822967489,15.642388302828,117.313369407985));
#111263=CARTESIAN_POINT('Ctrl Pts',(25.066829375572,15.8132141715895,117.422245999975));
#111264=CARTESIAN_POINT('Ctrl Pts',(23.8455348165031,16.1016601203548,117.652846543175));
#111265=CARTESIAN_POINT('Ctrl Pts',(23.1991565265732,16.2125536994563,117.774600442061));
#111266=CARTESIAN_POINT('Ctrl Pts',(22.1162847810566,16.3298002668299,117.978345738686));
#111267=CARTESIAN_POINT('Ctrl Pts',(21.6829642090882,16.358747623884,118.059824454681));
#111268=CARTESIAN_POINT('Ctrl Pts',(21.1143561097026,16.3732792260656,118.166847129352));
#111269=CARTESIAN_POINT('Ctrl Pts',(20.9796486377732,16.375000000269,118.192209814351));
#111270=CARTESIAN_POINT('Ctrl Pts',(20.8449496767831,16.375,118.217584317867));
#111271=CARTESIAN_POINT('Ctrl Pts',(1.80489434143683,2.28935384663574E-14,
119.652703644671));
#111272=CARTESIAN_POINT('Ctrl Pts',(1.80489434143683,-19.,119.652703644671));
#111273=CARTESIAN_POINT('Ctrl Pts',(20.5162416486687,-19.,116.353388268999));
#111274=CARTESIAN_POINT('Ctrl Pts',(39.2275889559007,-19.,113.054072893327));
#111275=CARTESIAN_POINT('Ctrl Pts',(39.2275889559007,2.28935384663574E-14,
113.054072893327));
#111276=CARTESIAN_POINT('Ctrl Pts',(39.2275889559007,19.0000000000001,113.054072893327));
#111277=CARTESIAN_POINT('Ctrl Pts',(20.5162416486688,19.0000000000001,116.353388268999));
#111278=CARTESIAN_POINT('Ctrl Pts',(1.80489434143685,19.0000000000001,119.652703644671));
#111279=CARTESIAN_POINT('Ctrl Pts',(1.80489434143683,2.28935384663574E-14,
119.652703644671));
#111280=CARTESIAN_POINT('Ctrl Pts',(2.8899419709034,4.93317397042308E-15,
125.818834058975));
#111281=CARTESIAN_POINT('Ctrl Pts',(2.8899419709034,-19.0021739918144,125.818834058975));
#111282=CARTESIAN_POINT('Ctrl Pts',(21.6034302421291,-19.0021739918144,
122.519141173586));
#111283=CARTESIAN_POINT('Ctrl Pts',(40.3169185133548,-19.0021739918144,
119.219448288197));
#111284=CARTESIAN_POINT('Ctrl Pts',(40.3169185133548,4.93317397042304E-15,
119.219448288197));
#111285=CARTESIAN_POINT('Ctrl Pts',(40.3169185133548,19.0021739918144,119.219448288197));
#111286=CARTESIAN_POINT('Ctrl Pts',(21.6034302421291,19.0021739918144,122.519141173586));
#111287=CARTESIAN_POINT('Ctrl Pts',(2.88994197090342,19.0021739918144,125.818834058975));
#111288=CARTESIAN_POINT('Ctrl Pts',(2.8899419709034,4.93317397042308E-15,
125.818834058975));
#111289=CARTESIAN_POINT('Ctrl Pts',(6.3506918559717,-1.15304933939532E-14,
131.036276236652));
#111290=CARTESIAN_POINT('Ctrl Pts',(6.35069185597169,-16.4999999999995,
131.036276236652));
#111291=CARTESIAN_POINT('Ctrl Pts',(22.6000197806726,-16.4999999999995,
128.171081305148));
#111292=CARTESIAN_POINT('Ctrl Pts',(38.8493477053735,-16.4999999999995,
125.305886373643));
#111293=CARTESIAN_POINT('Ctrl Pts',(38.8493477053735,-1.15304933939532E-14,
125.305886373643));
#111294=CARTESIAN_POINT('Ctrl Pts',(38.8493477053735,16.4999999999995,125.305886373643));
#111295=CARTESIAN_POINT('Ctrl Pts',(22.6000197806726,16.4999999999995,128.171081305148));
#111296=CARTESIAN_POINT('Ctrl Pts',(6.35069185597171,16.4999999999995,131.036276236652));
#111297=CARTESIAN_POINT('Ctrl Pts',(6.3506918559717,-1.15304933939532E-14,
131.036276236652));
#111298=CARTESIAN_POINT('',(6.35069185597038,-1.35511606125414E-14,131.036276236651));
#111299=CARTESIAN_POINT('Origin',(22.6000197806719,1.4210854715202E-14,
128.171081305147));
#111300=CARTESIAN_POINT('',(1.80489434143704,2.05667095479774E-14,119.652703644671));
#111301=CARTESIAN_POINT('Origin',(31.3509340513116,2.42107666709492E-14,
114.453517413878));
#111302=CARTESIAN_POINT('Origin',(20.5162416486691,1.4210854715202E-14,
116.353388269));
#111303=CARTESIAN_POINT('Origin',(11.833832765324,1.4210854715202E-14,67.1130006183894));
#111304=CARTESIAN_POINT('',(30.8903745807654,6.7681155228249,63.7528181373285));
#111305=CARTESIAN_POINT('',(30.8903812387965,-6.76809619335572,63.752816963338));
#111306=CARTESIAN_POINT('Origin',(11.833832765324,1.4210854715202E-14,67.1130006183894));
#111307=CARTESIAN_POINT('',(29.6607179812714,9.94038463627826,64.9669467867612));
#111308=CARTESIAN_POINT('Ctrl Pts',(29.6610694362665,9.94001765225634,64.9677683546378));
#111309=CARTESIAN_POINT('Ctrl Pts',(29.8626606590662,9.4922765200743,64.6815301868754));
#111310=CARTESIAN_POINT('Ctrl Pts',(30.0620247360424,9.02635699468926,64.4486981628682));
#111311=CARTESIAN_POINT('Ctrl Pts',(30.4831429543247,7.96380978435469,64.036809917008));
#111312=CARTESIAN_POINT('Ctrl Pts',(30.6973043635228,7.37286267557426,63.8759507130258));
#111313=CARTESIAN_POINT('Ctrl Pts',(30.8903745807654,6.76811552282492,63.7528181373285));
#111314=CARTESIAN_POINT('',(29.4810298430695,10.3418191817547,65.2638887238806));
#111315=CARTESIAN_POINT('Ctrl Pts',(29.4810568782271,10.3417884885121,65.2639387748332));
#111316=CARTESIAN_POINT('Ctrl Pts',(29.5093629970405,10.277887407849,65.2094624539339));
#111317=CARTESIAN_POINT('Ctrl Pts',(29.5383983492446,10.212682227821,65.157394501546));
#111318=CARTESIAN_POINT('Ctrl Pts',(29.5982881786419,10.0787826880955,65.0578607606596));
#111319=CARTESIAN_POINT('Ctrl Pts',(29.6289217697167,10.0105820158188,65.0107648292185));
#111320=CARTESIAN_POINT('Ctrl Pts',(29.6603665235238,9.94075156122962,64.9661252283734));
#111321=CARTESIAN_POINT('',(27.2015660631669,14.9604792914755,73.5557281547034));
#111322=CARTESIAN_POINT('Ctrl Pts',(27.2015705014209,14.9604739009962,73.5557285683884));
#111323=CARTESIAN_POINT('Ctrl Pts',(27.1654392493044,14.8743896900466,72.8216543486108));
#111324=CARTESIAN_POINT('Ctrl Pts',(27.2634348909743,14.6533579394755,72.0350130048608));
#111325=CARTESIAN_POINT('Ctrl Pts',(27.5421046041987,14.1098263590445,70.5236291817684));
#111326=CARTESIAN_POINT('Ctrl Pts',(27.7602914012229,13.7295898281507,69.7103575348371));
#111327=CARTESIAN_POINT('Ctrl Pts',(28.4255514554632,12.52946564147,67.586530187656));
#111328=CARTESIAN_POINT('Ctrl Pts',(28.9609479436267,11.5159364690254,66.2649476939623));
#111329=CARTESIAN_POINT('Ctrl Pts',(29.4810028050673,10.3418498799905,65.2638386757534));
#111330=CARTESIAN_POINT('',(27.2861971804113,14.998680114819,74.2711694581623));
#111331=CARTESIAN_POINT('Ctrl Pts',(27.2015616815609,14.9604819552268,73.5557280582404));
#111332=CARTESIAN_POINT('Ctrl Pts',(27.2121892020169,14.9857764789281,73.7714865315729));
#111333=CARTESIAN_POINT('Ctrl Pts',(27.236302938614,14.998378496898,73.9863406668699));
#111334=CARTESIAN_POINT('Ctrl Pts',(27.2778506876385,14.998378496898,74.2219696605585));
#111335=CARTESIAN_POINT('Ctrl Pts',(27.2823600271523,14.9982089721856,74.2464956078967));
#111336=CARTESIAN_POINT('Ctrl Pts',(27.2870497423904,14.9978696111192,74.2709950325846));
#111337=CARTESIAN_POINT('',(27.6070995425304,14.9199507410733,75.6071390537838));
#111338=CARTESIAN_POINT('Ctrl Pts',(27.2853446200354,14.9994906183976,74.2713438920009));
#111339=CARTESIAN_POINT('Ctrl Pts',(27.3712939315444,14.9932698714981,74.7203331224154));
#111340=CARTESIAN_POINT('Ctrl Pts',(27.4789460295974,14.9667633499927,75.1665245541753));
#111341=CARTESIAN_POINT('Ctrl Pts',(27.6070861523114,14.9199505879433,75.6071429300643));
#111342=CARTESIAN_POINT('',(28.5837286483844,14.4236088234574,78.2159945046497));
#111343=CARTESIAN_POINT('Ctrl Pts',(28.5837271422992,14.4236103938593,78.2159956036932));
#111344=CARTESIAN_POINT('Ctrl Pts',(28.3970080708632,14.5362294106934,77.799204136978));
#111345=CARTESIAN_POINT('Ctrl Pts',(28.2181098367699,14.6364962450901,77.3714384121405));
#111346=CARTESIAN_POINT('Ctrl Pts',(27.8891286847039,14.8042078675273,76.5021371343503));
#111347=CARTESIAN_POINT('Ctrl Pts',(27.738486650416,14.8719150396164,76.0587797395723));
#111348=CARTESIAN_POINT('Ctrl Pts',(27.6071124825729,14.9199244469508,75.6071324936865));
#111349=CARTESIAN_POINT('',(29.8215734155925,13.2678234653359,79.1320791187414));
#111350=CARTESIAN_POINT('Ctrl Pts',(28.5837298611721,14.4236073308178,78.2159935579633));
#111351=CARTESIAN_POINT('Ctrl Pts',(28.633171177856,14.3937861564346,78.3263512175926));
#111352=CARTESIAN_POINT('Ctrl Pts',(28.6946666043271,14.3500018857306,78.4264750537417));
#111353=CARTESIAN_POINT('Ctrl Pts',(28.8785087936175,14.2067869650545,78.6665485169518));
#111354=CARTESIAN_POINT('Ctrl Pts',(29.0141762283142,14.0893218683042,78.7878804462047));
#111355=CARTESIAN_POINT('Ctrl Pts',(29.2616910886977,13.8583103887882,78.9544730956887));
#111356=CARTESIAN_POINT('Ctrl Pts',(29.3748367764198,13.7470705966664,79.0119053447665));
#111357=CARTESIAN_POINT('Ctrl Pts',(29.5992739331012,13.5150320471622,79.0951625262152));
#111358=CARTESIAN_POINT('Ctrl Pts',(29.7118528383796,13.3929287157044,79.1214954015636));
#111359=CARTESIAN_POINT('Ctrl Pts',(29.8215734564531,13.2678235744527,79.1320799848902));
#111360=CARTESIAN_POINT('',(30.1098517192201,12.9238074747324,79.1218447623392));
#111361=CARTESIAN_POINT('Ctrl Pts',(29.8215733551035,13.2678233399104,79.1320782633696));
#111362=CARTESIAN_POINT('Ctrl Pts',(29.9225981941962,13.15263341247,79.14182474059));
#111363=CARTESIAN_POINT('Ctrl Pts',(30.0199654553166,13.0361914615023,79.1376939286814));
#111364=CARTESIAN_POINT('Ctrl Pts',(30.1098481430753,12.92381190166,79.1218451857309));
#111365=CARTESIAN_POINT('',(33.6423066138275,6.32455532063251,78.4989774482698));
#111366=CARTESIAN_POINT('Origin',(14.4385554303262,1.4210854715202E-14,
81.8851169135651));
#111367=CARTESIAN_POINT('',(33.6423066138211,-6.32455532067118,78.4989774483005));
#111368=CARTESIAN_POINT('Ctrl Pts',(33.6423066139704,6.3245553206325,78.49897744908));
#111369=CARTESIAN_POINT('Ctrl Pts',(33.6665909588537,6.24852627328648,78.4946954638666));
#111370=CARTESIAN_POINT('Ctrl Pts',(33.6906077282209,6.17214997068385,78.4910778646682));
#111371=CARTESIAN_POINT('Ctrl Pts',(33.9161865198445,5.44288016546143,78.4625119450618));
#111372=CARTESIAN_POINT('Ctrl Pts',(34.096465981114,4.76669862057734,78.4810806785018));
#111373=CARTESIAN_POINT('Ctrl Pts',(34.3912241285691,3.39678433761039,78.5498773566916));
#111374=CARTESIAN_POINT('Ctrl Pts',(34.5056891678386,2.70299030631043,78.6000742831831));
#111375=CARTESIAN_POINT('Ctrl Pts',(34.6569683004298,1.33087702156853,78.6768075863797));
#111376=CARTESIAN_POINT('Ctrl Pts',(34.6934420688607,0.65241734777343,78.7014923606593));
#111377=CARTESIAN_POINT('Ctrl Pts',(34.6934420688607,1.33226762955019E-14,
78.7014923606593));
#111378=CARTESIAN_POINT('Ctrl Pts',(34.6934420688607,-0.652417347773404,
78.7014923606593));
#111379=CARTESIAN_POINT('Ctrl Pts',(34.6569683004298,-1.3308770215685,78.6768075863797));
#111380=CARTESIAN_POINT('Ctrl Pts',(34.5056891678386,-2.70299030631041,
78.6000742831831));
#111381=CARTESIAN_POINT('Ctrl Pts',(34.3912241285691,-3.39678433761036,
78.5498773566916));
#111382=CARTESIAN_POINT('Ctrl Pts',(34.096465981114,-4.76669862057732,78.4810806785018));
#111383=CARTESIAN_POINT('Ctrl Pts',(33.9161865198445,-5.4428801654614,78.4625119450618));
#111384=CARTESIAN_POINT('Ctrl Pts',(33.6906077282169,-6.17214997069675,
78.4910778646687));
#111385=CARTESIAN_POINT('Ctrl Pts',(33.6665909588457,-6.24852627331219,
78.4946954638678));
#111386=CARTESIAN_POINT('Ctrl Pts',(33.6423066139581,-6.3245553206709,78.4989774490822));
#111387=CARTESIAN_POINT('',(30.109851949332,-12.9238077427022,79.1218473206622));
#111388=CARTESIAN_POINT('Origin',(14.4385554303262,1.4210854715202E-14,
81.8851169135651));
#111389=CARTESIAN_POINT('',(29.8216059073926,-13.2677862231535,79.1320814034235));
#111390=CARTESIAN_POINT('Ctrl Pts',(30.1098481430752,-12.92381190166,79.1218451857304));
#111391=CARTESIAN_POINT('Ctrl Pts',(30.0199751912077,-13.0361794164536,
79.1376925283409));
#111392=CARTESIAN_POINT('Ctrl Pts',(29.9226191337965,-13.1526083961398,
79.1418238949043));
#111393=CARTESIAN_POINT('Ctrl Pts',(29.8216059073926,-13.2677862231535,
79.1320814034235));
#111394=CARTESIAN_POINT('',(28.5838100706278,-14.4235289931938,78.2160017787004));
#111395=CARTESIAN_POINT('Ctrl Pts',(29.8216061616813,-13.2677868117196,
79.1320857232078));
#111396=CARTESIAN_POINT('Ctrl Pts',(29.7118038601082,-13.3929843766212,
79.1214868546364));
#111397=CARTESIAN_POINT('Ctrl Pts',(29.5991328833806,-13.5151805798363,
79.0951067676584));
#111398=CARTESIAN_POINT('Ctrl Pts',(29.3745120791704,-13.7473861843611,
79.0116991693966));
#111399=CARTESIAN_POINT('Ctrl Pts',(29.2612652340829,-13.8587081819794,
78.9541551381127));
#111400=CARTESIAN_POINT('Ctrl Pts',(29.0138299095263,-14.0895961234492,
78.7874271059373));
#111401=CARTESIAN_POINT('Ctrl Pts',(28.8783329260922,-14.2068946013881,
78.666154980642));
#111402=CARTESIAN_POINT('Ctrl Pts',(28.6947017762484,-14.3499295063546,
78.4262685171615));
#111403=CARTESIAN_POINT('Ctrl Pts',(28.6332644595127,-14.3936694520259,
78.3262180844277));
#111404=CARTESIAN_POINT('Ctrl Pts',(28.5838650340229,-14.4234670709579,
78.2159604183534));
#111405=CARTESIAN_POINT('',(27.60718386578,-14.9199168893285,75.6074591138482));
#111406=CARTESIAN_POINT('Ctrl Pts',(27.6071889912212,-14.9199064677107,
75.6074565146134));
#111407=CARTESIAN_POINT('Ctrl Pts',(27.7385049392646,-14.871907393202,76.0588374809969));
#111408=CARTESIAN_POINT('Ctrl Pts',(27.8893213549521,-14.8041048629894,
76.502615799427));
#111409=CARTESIAN_POINT('Ctrl Pts',(28.2182237838036,-14.6364415875546,
77.3717619195238));
#111410=CARTESIAN_POINT('Ctrl Pts',(28.3970555586945,-14.53619934482,77.7993003034521));
#111411=CARTESIAN_POINT('Ctrl Pts',(28.5837551075604,-14.4235909146646,
78.2160431338438));
#111412=CARTESIAN_POINT('',(27.286197390388,-14.9986800996203,74.2711705550149));
#111413=CARTESIAN_POINT('Ctrl Pts',(27.607178555543,-14.9199168285301,75.6074606516617));
#111414=CARTESIAN_POINT('Ctrl Pts',(27.4789995375747,-14.9667499667782,
75.1667448437143));
#111415=CARTESIAN_POINT('Ctrl Pts',(27.3713177919504,-14.9932681141233,
74.7204575783766));
#111416=CARTESIAN_POINT('Ctrl Pts',(27.2853448300283,-14.9994906031988,
74.2713449889783));
#111417=CARTESIAN_POINT('',(27.2015513600941,-14.9604539661155,73.555495291127));
#111418=CARTESIAN_POINT('Ctrl Pts',(27.2870499522845,-14.9978695959315,
74.2709961290926));
#111419=CARTESIAN_POINT('Ctrl Pts',(27.2823583510579,-14.998209098153,74.246486880775));
#111420=CARTESIAN_POINT('Ctrl Pts',(27.2778490441633,-14.998378496899,74.2219603399536));
#111421=CARTESIAN_POINT('Ctrl Pts',(27.2735220998427,-14.998378496899,74.1974210192936));
#111422=CARTESIAN_POINT('Ctrl Pts',(27.2361828882004,-14.998378496899,73.9856598271479));
#111423=CARTESIAN_POINT('Ctrl Pts',(27.2121477368108,-14.9857096904479,
73.7708402126313));
#111424=CARTESIAN_POINT('Ctrl Pts',(27.2015502202211,-14.9604546588834,
73.5554952659763));
#111425=CARTESIAN_POINT('',(29.4810598079121,-10.3417456735051,65.2638113433947));
#111426=CARTESIAN_POINT('Ctrl Pts',(29.4810610160957,-10.3417443046597,
65.2638135766404));
#111427=CARTESIAN_POINT('Ctrl Pts',(28.9598726194414,-11.518367656918,66.266975312665));
#111428=CARTESIAN_POINT('Ctrl Pts',(28.4243894486928,-12.5316424744244,
67.5898019444641));
#111429=CARTESIAN_POINT('Ctrl Pts',(27.758603110063,-13.7325957068466,69.7160102001576));
#111430=CARTESIAN_POINT('Ctrl Pts',(27.5414584630106,-14.1111311675135,
70.5272572949658));
#111431=CARTESIAN_POINT('Ctrl Pts',(27.2515878014758,-14.6764247608876,
72.0991554516062));
#111432=CARTESIAN_POINT('Ctrl Pts',(27.1675460400784,-14.879596606879,72.8656112330152));
#111433=CARTESIAN_POINT('Ctrl Pts',(27.2015525140621,-14.9604525641422,
73.5554953985588));
#111434=CARTESIAN_POINT('',(29.6609510243113,-9.94007378487892,64.9665024957973));
#111435=CARTESIAN_POINT('Ctrl Pts',(29.6605379238539,-9.94033539790784,
64.9657684968317));
#111436=CARTESIAN_POINT('Ctrl Pts',(29.6290590195802,-10.0102283533256,
65.0104017735973));
#111437=CARTESIAN_POINT('Ctrl Pts',(29.5983883914081,-10.0784994646189,
65.0575068363893));
#111438=CARTESIAN_POINT('Ctrl Pts',(29.5384375241501,-10.2125277434113,
65.1571032917546));
#111439=CARTESIAN_POINT('Ctrl Pts',(29.5093737895855,-10.2778012664117,
65.2092349779954));
#111440=CARTESIAN_POINT('Ctrl Pts',(29.4810586060414,-10.3417470414456,
65.2638091169701));
#111441=CARTESIAN_POINT('Ctrl Pts',(30.8903812387965,-6.76809619335574,
63.752816963338));
#111442=CARTESIAN_POINT('Ctrl Pts',(30.7097331720569,-7.33393380168619,
63.8680233812832));
#111443=CARTESIAN_POINT('Ctrl Pts',(30.5107179020567,-7.88750373573765,
64.0162157526285));
#111444=CARTESIAN_POINT('Ctrl Pts',(30.0922727058573,-8.95553598274615,
64.4139142005288));
#111445=CARTESIAN_POINT('Ctrl Pts',(29.8782495861902,-9.45763958307992,
64.6594445903658));
#111446=CARTESIAN_POINT('Ctrl Pts',(29.6612765321668,-9.93956440248096,
64.9674957905432));
#111447=CARTESIAN_POINT('Origin',(24.4068934345791,10.33198790001,60.67496948644));
#111448=CARTESIAN_POINT('',(24.9372762730815,10.3319816626968,59.2718678127106));
#111449=CARTESIAN_POINT('',(25.4229129967449,10.8757238874463,59.714731596499));
#111450=CARTESIAN_POINT('Origin',(24.4069004573991,10.33198058441,60.67497202932));
#111451=CARTESIAN_POINT('',(23.4739833876933,11.4523981580514,60.322322782081));
#111452=CARTESIAN_POINT('Origin',(24.4068934345791,10.33198790001,60.67496948644));
#111453=CARTESIAN_POINT('',(25.5799750648999,11.2436334983186,60.4681263249483));
#111454=CARTESIAN_POINT('Origin',(24.4069004573991,10.33198058441,60.67497202932));
#111455=CARTESIAN_POINT('',(22.9296818101862,10.3319887778349,60.9354417820097));
#111456=CARTESIAN_POINT('Origin',(24.4068934339491,10.33198915989,60.67496948286));
#111457=CARTESIAN_POINT('Origin',(24.4068932609991,10.33198790252,60.67496850203));
#111458=CARTESIAN_POINT('Origin',(6.43246351666909,-92.5,72.98888938658));
#111459=CARTESIAN_POINT('',(16.5158721300291,-92.,68.592883160925));
#111460=CARTESIAN_POINT('',(16.5158721300291,-92.,77.384895612235));
#111461=CARTESIAN_POINT('Origin',(6.43246351666909,-92.,72.98888938658));
#111462=CARTESIAN_POINT('',(16.5158709386063,-25.6802783436,68.5928804239554));
#111463=CARTESIAN_POINT('',(16.5158709400891,-25.6802783436,68.592880423309));
#111464=CARTESIAN_POINT('',(17.4324750363818,-25.5800482337938,72.9889222937213));
#111465=CARTESIAN_POINT('Ctrl Pts',(17.4324635166199,-25.5800482332938,
72.9889222889149));
#111466=CARTESIAN_POINT('Ctrl Pts',(17.4324645777424,-25.5354140613111,
72.6341648714431));
#111467=CARTESIAN_POINT('Ctrl Pts',(17.4152996369824,-25.5033048623799,
72.2793470851132));
#111468=CARTESIAN_POINT('Ctrl Pts',(17.3809768139068,-25.4836548570278,
71.9258481925477));
#111469=CARTESIAN_POINT('Ctrl Pts',(17.3480073399888,-25.4647796515264,
71.5862877638267));
#111470=CARTESIAN_POINT('Ctrl Pts',(17.2992064827594,-25.4574004780469,
71.2479437277912));
#111471=CARTESIAN_POINT('Ctrl Pts',(17.2346272733976,-25.4614590353976,
70.9120508823093));
#111472=CARTESIAN_POINT('Ctrl Pts',(17.1719357280398,-25.4653989602551,
70.5859762560326));
#111473=CARTESIAN_POINT('Ctrl Pts',(17.0943746508061,-25.4801177337986,
70.2622112095332));
#111474=CARTESIAN_POINT('Ctrl Pts',(17.0020368595677,-25.5055620193224,
69.9419040979565));
#111475=CARTESIAN_POINT('Ctrl Pts',(16.9137689448968,-25.5298848235974,
69.6357148290351));
#111476=CARTESIAN_POINT('Ctrl Pts',(16.8119981402997,-25.5640085017763,
69.3326851862224));
#111477=CARTESIAN_POINT('Ctrl Pts',(16.6968477217908,-25.6078864634696,
69.0338398433192));
#111478=CARTESIAN_POINT('Ctrl Pts',(16.6397990529275,-25.6296248065816,
68.8857836813928));
#111479=CARTESIAN_POINT('Ctrl Pts',(16.5794670519359,-25.6537573217834,
68.7387549080006));
#111480=CARTESIAN_POINT('Ctrl Pts',(16.5158709370957,-25.6802783436,68.592880424614));
#111481=CARTESIAN_POINT('',(16.5158721346073,-26.62691877498,77.3848956151154));
#111482=CARTESIAN_POINT('Ctrl Pts',(16.5158721453875,-26.6269187749801,
77.3848956198152));
#111483=CARTESIAN_POINT('Ctrl Pts',(16.8127630709596,-26.408358380933,76.703897373734));
#111484=CARTESIAN_POINT('Ctrl Pts',(17.0412431892719,-26.1956003393225,
75.9870348538324));
#111485=CARTESIAN_POINT('Ctrl Pts',(17.1956813601443,-26.0131972847863,
75.2521770695883));
#111486=CARTESIAN_POINT('Ctrl Pts',(17.3501194912107,-25.8307942772641,
74.5173194747521));
#111487=CARTESIAN_POINT('Ctrl Pts',(17.4305157170817,-25.6787462270838,
73.7644666170394));
#111488=CARTESIAN_POINT('Ctrl Pts',(17.4324409979989,-25.5828615251574,
73.0111529932187));
#111489=CARTESIAN_POINT('Ctrl Pts',(17.4324599365955,-25.5819183268572,
73.0037428004011));
#111490=CARTESIAN_POINT('Ctrl Pts',(17.432471282139,-25.5809805630684,72.9963325629999));
#111491=CARTESIAN_POINT('Ctrl Pts',(17.4324750363818,-25.5800482337938,
72.9889222937213));
#111492=CARTESIAN_POINT('',(16.5158721336291,-26.62691877498,77.384895614689));
#111493=CARTESIAN_POINT('Origin',(82.8534541851791,9.38083151964701,62.64107301909));
#111494=CARTESIAN_POINT('',(83.1139265236516,9.38085957612367,64.1182846358727));
#111495=CARTESIAN_POINT('',(84.3306658152022,9.38085639185424,62.3806007557379));
#111496=CARTESIAN_POINT('Origin',(82.8534541851791,9.38088126242801,62.64107301909));
#111497=CARTESIAN_POINT('',(83.9303998448743,8.3540709653061,62.4514288517342));
#111498=CARTESIAN_POINT('Ctrl Pts',(84.3306658154406,9.38085639185472,62.3806007579587));
#111499=CARTESIAN_POINT('Ctrl Pts',(84.3306679192988,9.34196946191789,62.3806089762619));
#111500=CARTESIAN_POINT('Ctrl Pts',(84.3291773724665,9.30344979713916,62.3808354481103));
#111501=CARTESIAN_POINT('Ctrl Pts',(84.3262566203095,9.26521743471116,62.3812916153508));
#111502=CARTESIAN_POINT('Ctrl Pts',(84.3233100507629,9.22664712515764,62.381751814788));
#111503=CARTESIAN_POINT('Ctrl Pts',(84.3189078623632,9.18836848325348,62.3824457913877));
#111504=CARTESIAN_POINT('Ctrl Pts',(84.3130622625201,9.15029712543912,62.3833944459789));
#111505=CARTESIAN_POINT('Ctrl Pts',(84.3072340119843,9.11233876059393,62.3843402850336));
#111506=CARTESIAN_POINT('Ctrl Pts',(84.2999707739129,9.07458573152475,62.385539315736));
#111507=CARTESIAN_POINT('Ctrl Pts',(84.2912345465586,9.0369630513843,62.3870210874909));
#111508=CARTESIAN_POINT('Ctrl Pts',(84.2826299686156,8.99990732119721,62.3884805298844));
#111509=CARTESIAN_POINT('Ctrl Pts',(84.2725962251058,8.96297738491442,62.3902142976612));
#111510=CARTESIAN_POINT('Ctrl Pts',(84.2610511945124,8.92612011196809,62.3922587022747));
#111511=CARTESIAN_POINT('Ctrl Pts',(84.253721429992,8.90271998934595,62.3935566637032));
#111512=CARTESIAN_POINT('Ctrl Pts',(84.2457815887353,8.87934955357341,62.3949799965243));
#111513=CARTESIAN_POINT('Ctrl Pts',(84.2372015097695,8.85600103677115,62.3965396057256));
#111514=CARTESIAN_POINT('Ctrl Pts',(84.2213960220003,8.81299039570091,62.3994125844308));
#111515=CARTESIAN_POINT('Ctrl Pts',(84.2033988237252,8.77003483830633,62.4026755011808));
#111516=CARTESIAN_POINT('Ctrl Pts',(84.1830317439484,8.72727946222033,62.4063534010779));
#111517=CARTESIAN_POINT('Ctrl Pts',(84.1641545930883,8.6876518036017,62.4097622486872));
#111518=CARTESIAN_POINT('Ctrl Pts',(84.1432409919603,8.64819608240158,62.4135276940112));
#111519=CARTESIAN_POINT('Ctrl Pts',(84.1201358387748,8.60907405684465,62.4176720128793));
#111520=CARTESIAN_POINT('Ctrl Pts',(84.0976541007213,8.57100760804725,62.4217045111906));
#111521=CARTESIAN_POINT('Ctrl Pts',(84.0730969576522,8.53325678692265,62.426095805446));
#111522=CARTESIAN_POINT('Ctrl Pts',(84.046316430218,8.49601897319737,62.4308673152347));
#111523=CARTESIAN_POINT('Ctrl Pts',(84.0205599190037,8.46020503453727,62.4354563751659));
#111524=CARTESIAN_POINT('Ctrl Pts',(83.9927462711912,8.42486550657697,62.4403972238464));
#111525=CARTESIAN_POINT('Ctrl Pts',(83.9627466674285,8.3902241733661,62.4457084182725));
#111526=CARTESIAN_POINT('Ctrl Pts',(83.9522334255182,8.37808425581839,62.4475697052506));
#111527=CARTESIAN_POINT('Ctrl Pts',(83.941451784926,8.36603053885286,62.4494764640261));
#111528=CARTESIAN_POINT('Ctrl Pts',(83.9303964859696,8.35407416969622,62.451429443095));
#111529=CARTESIAN_POINT('',(83.2009909796241,7.9420820879518,62.8844210194974));
#111530=CARTESIAN_POINT('Ctrl Pts',(83.2009909626467,7.942082062319,62.8844208921972));
#111531=CARTESIAN_POINT('Ctrl Pts',(83.222046508233,7.94653931462841,62.8807031398782));
#111532=CARTESIAN_POINT('Ctrl Pts',(83.2429357698035,7.95132157984317,62.8761972279364));
#111533=CARTESIAN_POINT('Ctrl Pts',(83.2635687047957,7.95643767493921,62.871090966125));
#111534=CARTESIAN_POINT('Ctrl Pts',(83.2842193969547,7.96155817306146,62.8659803097501));
#111535=CARTESIAN_POINT('Ctrl Pts',(83.3046143507272,7.96701310580604,62.8602693081362));
#111536=CARTESIAN_POINT('Ctrl Pts',(83.3247033968147,7.97280522806796,62.8541132564984));
#111537=CARTESIAN_POINT('Ctrl Pts',(83.3446240476281,7.97854879819796,62.8480088076095));
#111538=CARTESIAN_POINT('Ctrl Pts',(83.3642448422555,7.98462393869616,62.8414672964301));
#111539=CARTESIAN_POINT('Ctrl Pts',(83.383541384477,7.99102707214922,62.8345960380203));
#111540=CARTESIAN_POINT('Ctrl Pts',(83.4026576805979,7.99737039489514,62.8277889630026));
#111541=CARTESIAN_POINT('Ctrl Pts',(83.421456488262,8.0040356111001,62.8206585172748));
#111542=CARTESIAN_POINT('Ctrl Pts',(83.4399258027391,8.01101300250228,62.8132597545955));
#111543=CARTESIAN_POINT('Ctrl Pts',(83.4582588180922,8.01793890242455,62.8059155930153));
#111544=CARTESIAN_POINT('Ctrl Pts',(83.4762677324473,8.02517237978557,62.7983071209058));
#111545=CARTESIAN_POINT('Ctrl Pts',(83.4939429395274,8.03269780909502,62.7904371848953));
#111546=CARTESIAN_POINT('Ctrl Pts',(83.5116060615294,8.04021809303896,62.7825726298001));
#111547=CARTESIAN_POINT('Ctrl Pts',(83.5289363689357,8.04802992154145,62.7744469479267));
#111548=CARTESIAN_POINT('Ctrl Pts',(83.5459191289626,8.05611167223378,62.7660115139603));
#111549=CARTESIAN_POINT('Ctrl Pts',(83.5629790145414,8.06423012541038,62.7575377712915));
#111550=CARTESIAN_POINT('Ctrl Pts',(83.5796886050667,8.07262094713688,62.7487513653927));
#111551=CARTESIAN_POINT('Ctrl Pts',(83.5960214164399,8.08125626970302,62.7395518330078));
#111552=CARTESIAN_POINT('Ctrl Pts',(83.6086053828994,8.08790954004676,62.7324638550516));
#111553=CARTESIAN_POINT('Ctrl Pts',(83.6209655150557,8.09470782886237,62.725129557547));
#111554=CARTESIAN_POINT('Ctrl Pts',(83.6330826272214,8.1016360813663,62.7174832477284));
#111555=CARTESIAN_POINT('Ctrl Pts',(83.6567703444014,8.11518010766737,62.7025354926875));
#111556=CARTESIAN_POINT('Ctrl Pts',(83.6795771016034,8.12928191424406,62.6868902425315));
#111557=CARTESIAN_POINT('Ctrl Pts',(83.7014877431072,8.14391670430066,62.6707517017523));
#111558=CARTESIAN_POINT('Ctrl Pts',(83.7244532122668,8.15925604612889,62.6538362152531));
#111559=CARTESIAN_POINT('Ctrl Pts',(83.7464350423128,8.17518092904151,62.6363791547347));
#111560=CARTESIAN_POINT('Ctrl Pts',(83.7674378978759,8.19166080634232,62.6185610768498));
#111561=CARTESIAN_POINT('Ctrl Pts',(83.7886019840947,8.20826719317491,62.6006062165939));
#111562=CARTESIAN_POINT('Ctrl Pts',(83.8087728368686,8.22543711768918,62.5822846068703));
#111563=CARTESIAN_POINT('Ctrl Pts',(83.827964089698,8.24313741331777,62.5637259673144));
#111564=CARTESIAN_POINT('Ctrl Pts',(83.8477357437988,8.26137301918273,62.5446060586172));
#111565=CARTESIAN_POINT('Ctrl Pts',(83.8664683468657,8.28017155560093,62.5252344585607));
#111566=CARTESIAN_POINT('Ctrl Pts',(83.8841744418319,8.29949484755758,62.5056966765476));
#111567=CARTESIAN_POINT('Ctrl Pts',(83.9004482213411,8.31725500265072,62.4877393823397));
#111568=CARTESIAN_POINT('Ctrl Pts',(83.9158551085819,8.33545841735704,62.4696407985449));
#111569=CARTESIAN_POINT('Ctrl Pts',(83.930396470504,8.35407418254754,62.4514294460597));
#111570=CARTESIAN_POINT('',(81.9035260502888,8.32029685538484,63.1131988121113));
#111571=CARTESIAN_POINT('Origin',(82.9055487053591,9.38083151964701,62.93651572428));
#111572=CARTESIAN_POINT('Origin',(82.8534541851791,9.38083151964701,62.64107301909));
#111573=CARTESIAN_POINT('Origin',(72.4794067363791,-4.5075054799778E-14,
55.63586067514));
#111574=CARTESIAN_POINT('',(63.1758688215082,1.34031149749143E-14,57.5808113821829));
#111575=CARTESIAN_POINT('',(81.8872355012805,1.51070582845848E-14,54.28158621401));
#111576=CARTESIAN_POINT('Origin',(72.5314653386492,-4.5075054799778E-14,
55.9310996797491));
#111577=CARTESIAN_POINT('',(82.3736337596115,-2.14063710640059E-14,53.5869134266698));
#111578=CARTESIAN_POINT('',(81.8871110497795,1.47525070273786E-14,54.2817578235612));
#111579=CARTESIAN_POINT('',(62.4811376251638,-1.81697385251322E-14,57.0943371416662));
#111580=CARTESIAN_POINT('Origin',(72.4273508090685,-4.5075054799778E-14,
55.3406368409801));
#111581=CARTESIAN_POINT('',(63.1760167402064,1.34099672619711E-14,57.58091496094));
#111582=CARTESIAN_POINT('Origin',(71.6139524734691,1.4210854715202E-14,
50.72762564822));
#111583=CARTESIAN_POINT('',(82.5073599491905,1.54967338543067E-14,52.0401193459587));
#111584=CARTESIAN_POINT('',(82.5003366733922,-0.386927879893151,52.0413577389749));
#111585=CARTESIAN_POINT('Origin',(72.1668785425691,1.4210854715202E-14,
53.86342521146));
#111586=CARTESIAN_POINT('',(82.7678322156911,1.54967338543067E-14,53.5173309754786));
#111587=CARTESIAN_POINT('',(81.9544338800974,1.54967338543067E-14,48.9043197827175));
#111588=CARTESIAN_POINT('Origin',(72.4273508090691,1.4210854715202E-14,
55.34063684098));
#111589=CARTESIAN_POINT('Origin',(72.1668785425691,1.4210854715202E-14,
53.86342521146));
#111590=CARTESIAN_POINT('Origin',(72.1668785425691,1.4210854715202E-14,
53.86342521146));
#111591=CARTESIAN_POINT('',(82.9055752351331,-0.405352763000806,51.4621899410204));
#111592=CARTESIAN_POINT('Origin',(72.0800544537391,1.4210854715202E-14,
53.371021335));
#111593=CARTESIAN_POINT('Origin',(82.9924061081933,-0.405353017030921,51.9545926212376));
#111594=CARTESIAN_POINT('Origin',(71.6139524734691,1.4210854715202E-14,
50.72762564822));
#111595=CARTESIAN_POINT('',(83.072317586283,1.55885823642428E-14,50.925075459698));
#111596=CARTESIAN_POINT('',(83.0657624332148,-0.386939173054244,50.9262313100466));
#111597=CARTESIAN_POINT('Origin',(71.9932303648991,1.4210854715202E-14,
52.87861745845));
#111598=CARTESIAN_POINT('',(83.1591416751154,1.55885823642428E-14,51.4174793361976));
#111599=CARTESIAN_POINT('',(82.6930396948565,1.55885823642428E-14,48.7740836494674));
#111600=CARTESIAN_POINT('Origin',(72.0800544537291,1.4210854715202E-14,
53.37102133495));
#111601=CARTESIAN_POINT('Origin',(71.9932303648991,1.4210854715202E-14,
52.87861745845));
#111602=CARTESIAN_POINT('Origin',(71.9932303648991,1.4210854715202E-14,
52.87861745845));
#111603=CARTESIAN_POINT('',(83.4710450568977,-0.404136266114647,50.3470557427728));
#111604=CARTESIAN_POINT('Origin',(71.9064062760691,1.4210854715202E-14,
52.38621358198));
#111605=CARTESIAN_POINT('Origin',(83.5578749695843,-0.404136469634433,50.8394585923398));
#111606=CARTESIAN_POINT('Origin',(6.43246351666909,92.,72.98888938658));
#111607=CARTESIAN_POINT('',(16.5158721300291,92.,77.384895612235));
#111608=CARTESIAN_POINT('',(16.5158721300291,92.,68.592883160925));
#111609=CARTESIAN_POINT('Origin',(6.43246351666909,92.,72.98888938658));
#111610=CARTESIAN_POINT('',(16.0575353748791,92.5,68.792701625727));
#111611=CARTESIAN_POINT('Origin',(16.0575353748791,92.,68.792701625727));
#111612=CARTESIAN_POINT('',(16.0575353748791,92.5,77.185077147433));
#111613=CARTESIAN_POINT('Origin',(6.43246351666909,92.5,72.98888938658));
#111614=CARTESIAN_POINT('Origin',(16.0575353748791,92.,77.185077147433));
#111615=CARTESIAN_POINT('Origin',(6.43246351666909,-92.5,72.98888938658));
#111616=CARTESIAN_POINT('',(17.4324600236772,25.5801002023223,72.9888894061479));
#111617=CARTESIAN_POINT('',(16.5158721312486,26.62691877866,77.3848956129324));
#111618=CARTESIAN_POINT('Ctrl Pts',(17.4324565306852,25.5801002023224,72.9888894061479));
#111619=CARTESIAN_POINT('Ctrl Pts',(17.4331138485723,25.6746776183602,73.745453096432));
#111620=CARTESIAN_POINT('Ctrl Pts',(17.3542127226475,25.8261249661036,74.4979998452865));
#111621=CARTESIAN_POINT('Ctrl Pts',(17.0463140803605,26.1912967232894,75.9719859573303));
#111622=CARTESIAN_POINT('Ctrl Pts',(16.8173238247368,26.405009893619,76.6934360403765));
#111623=CARTESIAN_POINT('Ctrl Pts',(16.5158721306991,26.62691877866,77.384895612693));
#111624=CARTESIAN_POINT('',(16.5158747362626,25.68037166863,68.5928891373664));
#111625=CARTESIAN_POINT('Ctrl Pts',(16.515874735658,25.68037166863,68.59288913763));
#111626=CARTESIAN_POINT('Ctrl Pts',(16.5986513774045,25.6458493068531,68.7827596723862));
#111627=CARTESIAN_POINT('Ctrl Pts',(16.6762707643978,25.6153134130533,68.9754506479589));
#111628=CARTESIAN_POINT('Ctrl Pts',(16.748483349918,25.588832917128,69.1705474951282));
#111629=CARTESIAN_POINT('Ctrl Pts',(16.8206436166596,25.5623716066008,69.3655029925774));
#111630=CARTESIAN_POINT('Ctrl Pts',(16.8874047263992,25.5399598197198,69.5628605425677));
#111631=CARTESIAN_POINT('Ctrl Pts',(16.948563454897,25.5216663366697,69.7621817628245));
#111632=CARTESIAN_POINT('Ctrl Pts',(17.0096942990628,25.503381194237,69.9614121057976));
#111633=CARTESIAN_POINT('Ctrl Pts',(17.0652277220566,25.4892106011433,70.1626039740258));
#111634=CARTESIAN_POINT('Ctrl Pts',(17.1150090469596,25.4792232435384,70.3653000526195));
#111635=CARTESIAN_POINT('Ctrl Pts',(17.1457649251256,25.4730528582726,70.4905296625209));
#111636=CARTESIAN_POINT('Ctrl Pts',(17.1743261824005,25.4684792184117,70.6163330668643));
#111637=CARTESIAN_POINT('Ctrl Pts',(17.2006658845956,25.465518521688,70.742599609329));
#111638=CARTESIAN_POINT('Ctrl Pts',(17.2467648332579,25.4603367999942,70.9635874859473));
#111639=CARTESIAN_POINT('Ctrl Pts',(17.286051845598,25.4600965467122,71.1859717032842));
#111640=CARTESIAN_POINT('Ctrl Pts',(17.3184481782116,25.4648114312984,71.4092255145296));
#111641=CARTESIAN_POINT('Ctrl Pts',(17.3508491400659,25.4695269896132,71.6325112273989));
#111642=CARTESIAN_POINT('Ctrl Pts',(17.3763574227755,25.4791991020161,71.8566664110209));
#111643=CARTESIAN_POINT('Ctrl Pts',(17.3949461950319,25.4938414438245,72.0811595112339));
#111644=CARTESIAN_POINT('Ctrl Pts',(17.4135468568908,25.508493151051,72.3057961999368));
#111645=CARTESIAN_POINT('Ctrl Pts',(17.4252191627864,25.5281214477534,72.5307708650725));
#111646=CARTESIAN_POINT('Ctrl Pts',(17.4299884033709,25.5527400355065,72.755551934862));
#111647=CARTESIAN_POINT('Ctrl Pts',(17.4316393110341,25.5612619405056,72.8333615534126));
#111648=CARTESIAN_POINT('Ctrl Pts',(17.4324635168074,25.5703818066716,72.9111480090886));
#111649=CARTESIAN_POINT('Ctrl Pts',(17.4324635166691,25.5801002023223,72.9888894061479));
#111650=CARTESIAN_POINT('',(16.5158721300291,92.,68.592883160925));
#111651=CARTESIAN_POINT('',(16.5158721300291,92.,77.384895612235));
#111652=CARTESIAN_POINT('Origin',(17.7894674803291,1.4210854715202E-14,
100.88908350184));
#111653=CARTESIAN_POINT('',(-4.38226888389591,-1.31660223688345E-7,96.08109859282));
#111654=CARTESIAN_POINT('',(7.33390977337979,-18.5189601959142,98.6155810268129));
#111655=CARTESIAN_POINT('Ctrl Pts',(-4.38226888389591,-1.31660223688345E-7,
96.08109859282));
#111656=CARTESIAN_POINT('Ctrl Pts',(-4.38226740849383,-0.395879795914794,
96.0811066634897));
#111657=CARTESIAN_POINT('Ctrl Pts',(-4.36836546848751,-0.794239500360881,
96.0954673000493));
#111658=CARTESIAN_POINT('Ctrl Pts',(-4.32606480122498,-1.39451379175889,
96.1384318258752));
#111659=CARTESIAN_POINT('Ctrl Pts',(-4.29955327484655,-1.69533351275973,
96.1652701131746));
#111660=CARTESIAN_POINT('Ctrl Pts',(-4.2591188739944,-2.04725725181565,
96.2059329439757));
#111661=CARTESIAN_POINT('Ctrl Pts',(-4.2365109977993,-2.22343172549005,
96.228599658187));
#111662=CARTESIAN_POINT('Ctrl Pts',(-4.22630807341278,-2.29897747604772,
96.2388141126869));
#111663=CARTESIAN_POINT('Ctrl Pts',(-4.21939176836248,-2.34935038034874,
96.2457348631364));
#111664=CARTESIAN_POINT('Ctrl Pts',(-4.21611286433566,-2.37287399529721,
96.2490144430748));
#111665=CARTESIAN_POINT('Ctrl Pts',(-4.15135954270303,-2.82954021094412,
96.313747497813));
#111666=CARTESIAN_POINT('Ctrl Pts',(-4.07099976598698,-3.27913917903879,
96.3943244434559));
#111667=CARTESIAN_POINT('Ctrl Pts',(-3.91545475344492,-3.98089845402761,
96.5436302590383));
#111668=CARTESIAN_POINT('Ctrl Pts',(-3.85776822453298,-4.21936941677387,
96.5981382309613));
#111669=CARTESIAN_POINT('Ctrl Pts',(-3.76171544626494,-4.58352350096052,
96.6868742257576));
#111670=CARTESIAN_POINT('Ctrl Pts',(-3.7113080371269,-4.76721148175515,
96.7329856841091));
#111671=CARTESIAN_POINT('Ctrl Pts',(-3.648162566933,-4.98423966769277,96.7898034593372));
#111672=CARTESIAN_POINT('Ctrl Pts',(-3.61548421214779,-5.0934226157687,
96.8189638396919));
#111673=CARTESIAN_POINT('Ctrl Pts',(-3.60123998781038,-5.14035727020337,
96.8316217747574));
#111674=CARTESIAN_POINT('Ctrl Pts',(-3.59169042377515,-5.17167843320581,
96.8400960484506));
#111675=CARTESIAN_POINT('Ctrl Pts',(-3.58636743023429,-5.18904958358344,
96.8448125091018));
#111676=CARTESIAN_POINT('Ctrl Pts',(-3.44424236895454,-5.65095142284287,
96.9705842863248));
#111677=CARTESIAN_POINT('Ctrl Pts',(-3.2720713912644,-6.15256771946993,
97.1189231221924));
#111678=CARTESIAN_POINT('Ctrl Pts',(-2.9441812821162,-6.97785834618417,
97.3778065444133));
#111679=CARTESIAN_POINT('Ctrl Pts',(-2.82324375543532,-7.26505900893829,
97.4701573369327));
#111680=CARTESIAN_POINT('Ctrl Pts',(-2.62183713875804,-7.71262231887509,
97.6173202930935));
#111681=CARTESIAN_POINT('Ctrl Pts',(-2.55136652007071,-7.86460046030084,
97.6678137746956));
#111682=CARTESIAN_POINT('Ctrl Pts',(-2.44032705660128,-8.09654677529307,
97.7456543920469));
#111683=CARTESIAN_POINT('Ctrl Pts',(-2.38347381396219,-8.21351435473895,
97.7850997770581));
#111684=CARTESIAN_POINT('Ctrl Pts',(-2.31473776421149,-8.35166775047382,
97.8320252948431));
#111685=CARTESIAN_POINT('Ctrl Pts',(-2.27975863749924,-8.42116082762791,
97.8557128919944));
#111686=CARTESIAN_POINT('Ctrl Pts',(-2.26463563642141,-8.45103210312728,
97.8659127232834));
#111687=CARTESIAN_POINT('Ctrl Pts',(-2.25452420328234,-8.47096588156003,
97.8727232587939));
#111688=CARTESIAN_POINT('Ctrl Pts',(-2.24889450428614,-8.48204086843337,
97.8765095288148));
#111689=CARTESIAN_POINT('Ctrl Pts',(-2.09953854167641,-8.77534963713818,
97.9768370423297));
#111690=CARTESIAN_POINT('Ctrl Pts',(-1.94846674521134,-9.05697686800579,
98.073135296074));
#111691=CARTESIAN_POINT('Ctrl Pts',(-1.63409619546405,-9.61408890046589,
98.2637989826697));
#111692=CARTESIAN_POINT('Ctrl Pts',(-1.47017163101268,-9.89057982332896,
98.3585098232659));
#111693=CARTESIAN_POINT('Ctrl Pts',(-0.964233481725216,-10.7039866099445,
98.6377449207042));
#111694=CARTESIAN_POINT('Ctrl Pts',(-0.612751142896682,-11.2209512901646,
98.8036853265539));
#111695=CARTESIAN_POINT('Ctrl Pts',(0.10450987898053,-12.1973811850675,
99.0945813177457));
#111696=CARTESIAN_POINT('Ctrl Pts',(0.463979741155269,-12.6487435089947,
99.2162585783067));
#111697=CARTESIAN_POINT('Ctrl Pts',(0.994936356724773,-13.2742324080916,
99.3647947432687));
#111698=CARTESIAN_POINT('Ctrl Pts',(1.17056338743409,-13.4741453696707,
99.4086406561457));
#111699=CARTESIAN_POINT('Ctrl Pts',(1.43092046996534,-13.7616699130789,
99.4660946977389));
#111700=CARTESIAN_POINT('Ctrl Pts',(1.51719322763612,-13.8554543000973,
99.4838600685593));
#111701=CARTESIAN_POINT('Ctrl Pts',(1.68855009682205,-14.0390007881235,
99.516647558742));
#111702=CARTESIAN_POINT('Ctrl Pts',(1.77440983548494,-14.1295696360823,
99.5317952307266));
#111703=CARTESIAN_POINT('Ctrl Pts',(2.19259251099756,-14.5645253456288,
99.5994883737387));
#111704=CARTESIAN_POINT('Ctrl Pts',(2.52711263534736,-14.8925987630755,
99.6339837749765));
#111705=CARTESIAN_POINT('Ctrl Pts',(3.02526127117294,-15.356361515315,99.6568716664454));
#111706=CARTESIAN_POINT('Ctrl Pts',(3.1907097246831,-15.5062274705087,99.6596910271714));
#111707=CARTESIAN_POINT('Ctrl Pts',(3.43756894799691,-15.7241533429341,
99.6567777784696));
#111708=CARTESIAN_POINT('Ctrl Pts',(3.56067058119804,-15.8313982301523,
99.6535355136471));
#111709=CARTESIAN_POINT('Ctrl Pts',(3.70362915460082,-15.9535585987621,
99.6466431710621));
#111710=CARTESIAN_POINT('Ctrl Pts',(3.76474672461133,-16.0052842994467,
99.6430245258013));
#111711=CARTESIAN_POINT('Ctrl Pts',(3.80545736235971,-16.0396289661334,
99.6404645401892));
#111712=CARTESIAN_POINT('Ctrl Pts',(3.82721096178525,-16.0579182564491,
99.6390113352449));
#111713=CARTESIAN_POINT('Ctrl Pts',(5.05603156831833,-17.0879713083793,
99.5526895815698));
#111714=CARTESIAN_POINT('Ctrl Pts',(6.24087891321929,-17.8883939937044,
99.2080656541756));
#111715=CARTESIAN_POINT('Ctrl Pts',(7.33390977282909,-18.51896019696,98.61558102691));
#111716=CARTESIAN_POINT('',(20.8003130802284,-19.9701890893778,80.5583314866612));
#111717=CARTESIAN_POINT('Ctrl Pts',(20.8003130790713,-19.9701890857655,
80.5583314868652));
#111718=CARTESIAN_POINT('Ctrl Pts',(20.7653319117175,-19.987994824802,80.6751964237543));
#111719=CARTESIAN_POINT('Ctrl Pts',(20.7262218203834,-20.0075988348333,
80.8048120490032));
#111720=CARTESIAN_POINT('Ctrl Pts',(20.6825233107631,-20.0289315329255,
80.9468047609331));
#111721=CARTESIAN_POINT('Ctrl Pts',(20.6406279657392,-20.0493839637894,
81.0829383203812));
#111722=CARTESIAN_POINT('Ctrl Pts',(20.5945149707442,-20.0714254468934,
81.2304486066214));
#111723=CARTESIAN_POINT('Ctrl Pts',(20.5437688867959,-20.0949485475054,
81.3890082378651));
#111724=CARTESIAN_POINT('Ctrl Pts',(20.4940782529224,-20.1179823993643,
81.5442700427224));
#111725=CARTESIAN_POINT('Ctrl Pts',(20.4399451680258,-20.1424370973425,
81.7101263638527));
#111726=CARTESIAN_POINT('Ctrl Pts',(20.3809704781416,-20.1681641667881,
81.8862714296551));
#111727=CARTESIAN_POINT('Ctrl Pts',(20.3223276737648,-20.1937464547771,
82.0614252228514));
#111728=CARTESIAN_POINT('Ctrl Pts',(20.2588975070578,-20.220587175818,82.2467523019759));
#111729=CARTESIAN_POINT('Ctrl Pts',(20.1902797183793,-20.2484884442895,
82.4419534052279));
#111730=CARTESIAN_POINT('Ctrl Pts',(20.1216619297008,-20.2763897127609,
82.63715450848));
#111731=CARTESIAN_POINT('Ctrl Pts',(20.0478563792751,-20.3053519379154,
82.8422296605058));
#111732=CARTESIAN_POINT('Ctrl Pts',(19.9684567327649,-20.3351194882471,
83.0568806706376));
#111733=CARTESIAN_POINT('Ctrl Pts',(19.898207261829,-20.361456565977,83.2467948649744));
#111734=CARTESIAN_POINT('Ctrl Pts',(19.823519635129,-20.3884370978636,83.4441575159233));
#111735=CARTESIAN_POINT('Ctrl Pts',(19.7439596888234,-20.4158699133918,
83.6486878978924));
#111736=CARTESIAN_POINT('Ctrl Pts',(19.6670364254486,-20.4423935825492,
83.8464399725348));
#111737=CARTESIAN_POINT('Ctrl Pts',(19.5855582997632,-20.4693401437796,
84.0508925855895));
#111738=CARTESIAN_POINT('Ctrl Pts',(19.4991306420753,-20.4964891051933,
84.261792405076));
#111739=CARTESIAN_POINT('Ctrl Pts',(19.4171160814392,-20.5222518089578,
84.4619234336858));
#111740=CARTESIAN_POINT('Ctrl Pts',(19.3306444054264,-20.5481966833614,
84.6678600984616));
#111741=CARTESIAN_POINT('Ctrl Pts',(19.2393782527093,-20.5740918708992,
84.879385946047));
#111742=CARTESIAN_POINT('Ctrl Pts',(19.1500280070395,-20.5994434530497,
85.0864713318617));
#111743=CARTESIAN_POINT('Ctrl Pts',(19.0560658076384,-20.624751139383,85.2989083256206));
#111744=CARTESIAN_POINT('Ctrl Pts',(18.9571047420586,-20.6497644783627,
85.5164798154753));
#111745=CARTESIAN_POINT('Ctrl Pts',(18.8971764585829,-20.664911914986,85.6482355301482));
#111746=CARTESIAN_POINT('Ctrl Pts',(18.8354150145491,-20.6799504595488,
85.7818741643341));
#111747=CARTESIAN_POINT('Ctrl Pts',(18.7717350493916,-20.6948151419852,
85.9173474032424));
#111748=CARTESIAN_POINT('Ctrl Pts',(18.6873169113696,-20.7145206931811,
86.0969391877568));
#111749=CARTESIAN_POINT('Ctrl Pts',(18.5995231590073,-20.7339224297437,
86.2797556801146));
#111750=CARTESIAN_POINT('Ctrl Pts',(18.5081361122369,-20.7528508611175,
86.4656796928624));
#111751=CARTESIAN_POINT('Ctrl Pts',(18.4624425888517,-20.7623150768044,
86.5586416992363));
#111752=CARTESIAN_POINT('Ctrl Pts',(18.4158514891404,-20.771660387363,86.6523786905016));
#111753=CARTESIAN_POINT('Ctrl Pts',(18.3683406589989,-20.7808622225757,
86.7468635635245));
#111754=CARTESIAN_POINT('Ctrl Pts',(18.3445852439282,-20.7854631401821,
86.7941060000359));
#111755=CARTESIAN_POINT('Ctrl Pts',(18.3205998936028,-20.7900281673136,
86.8415354074536));
#111756=CARTESIAN_POINT('Ctrl Pts',(18.2963818441927,-20.7945540934904,
86.8891482101765));
#111757=CARTESIAN_POINT('Ctrl Pts',(18.2842728194877,-20.7968170565788,
86.9129546115379));
#111758=CARTESIAN_POINT('Ctrl Pts',(18.2721056198366,-20.7990702430506,
86.9368068617565));
#111759=CARTESIAN_POINT('Ctrl Pts',(18.2598798995501,-20.8013132430092,
86.9607045083562));
#111760=CARTESIAN_POINT('Ctrl Pts',(18.2537670394069,-20.8024347429884,
86.972653331656));
#111761=CARTESIAN_POINT('Ctrl Pts',(18.2476395490946,-20.8035536962519,
86.9846135040529));
#111762=CARTESIAN_POINT('Ctrl Pts',(18.2414973854199,-20.8046700510096,
86.9965849683362));
#111763=CARTESIAN_POINT('Ctrl Pts',(18.2368907626639,-20.8055073170779,
87.0055635665487));
#111764=CARTESIAN_POINT('Ctrl Pts',(18.2322758861407,-20.8063431214795,
87.0145485164474));
#111765=CARTESIAN_POINT('Ctrl Pts',(18.2276527376309,-20.8071774422296,
87.0235397937539));
#111766=CARTESIAN_POINT('Ctrl Pts',(18.2261116881277,-20.8074555491462,
87.0265368861894));
#111767=CARTESIAN_POINT('Ctrl Pts',(18.2236400469036,-20.8079008663174,
87.0313414365281));
#111768=CARTESIAN_POINT('Ctrl Pts',(18.2230268311186,-20.8080112676088,
87.0325331792842));
#111769=CARTESIAN_POINT('Ctrl Pts',(18.1533013936453,-20.8205643990277,
87.1680397775557));
#111770=CARTESIAN_POINT('Ctrl Pts',(18.0784123332618,-20.8333737895828,
87.311317704187));
#111771=CARTESIAN_POINT('Ctrl Pts',(17.9980045836939,-20.8461945100127,
87.4619762758188));
#111772=CARTESIAN_POINT('Ctrl Pts',(17.9200700604966,-20.8586208835789,
87.6080008071459));
#111773=CARTESIAN_POINT('Ctrl Pts',(17.8369509634185,-20.8710579465556,
87.7609589579823));
#111774=CARTESIAN_POINT('Ctrl Pts',(17.7483263582346,-20.8832340293166,
87.9204945809405));
#111775=CARTESIAN_POINT('Ctrl Pts',(17.6611683978886,-20.8952086105995,
88.0773900556306));
#111776=CARTESIAN_POINT('Ctrl Pts',(17.5686854591308,-20.9069309183669,
88.2406471355186));
#111777=CARTESIAN_POINT('Ctrl Pts',(17.4705771026812,-20.9180932140501,
88.4099262132584));
#111778=CARTESIAN_POINT('Ctrl Pts',(17.3748863402747,-20.9289804475415,
88.5750339022932));
#111779=CARTESIAN_POINT('Ctrl Pts',(17.2738437991793,-20.939334975306,88.7458704901516));
#111780=CARTESIAN_POINT('Ctrl Pts',(17.1671780469306,-20.9488226713765,
88.9221195676893));
#111781=CARTESIAN_POINT('Ctrl Pts',(17.0925185791883,-20.9554634752315,
89.0454830844847));
#111782=CARTESIAN_POINT('Ctrl Pts',(17.0151043630113,-20.9616786102941,
89.1714982304492));
#111783=CARTESIAN_POINT('Ctrl Pts',(16.9348453643333,-20.9673385492286,
89.3000559693276));
#111784=CARTESIAN_POINT('Ctrl Pts',(16.825042534418,-20.9750819465099,89.4759366028872));
#111785=CARTESIAN_POINT('Ctrl Pts',(16.7098893736243,-20.9817890778163,
89.6565138298478));
#111786=CARTESIAN_POINT('Ctrl Pts',(16.5891011991341,-20.9870881773623,
89.8413160432456));
#111787=CARTESIAN_POINT('Ctrl Pts',(16.4711138718983,-20.9922644009027,
90.021833045991));
#111788=CARTESIAN_POINT('Ctrl Pts',(16.3477496186044,-20.9960971507281,
90.2063814056935));
#111789=CARTESIAN_POINT('Ctrl Pts',(16.2187573001304,-20.9981925841403,
90.3945190644661));
#111790=CARTESIAN_POINT('Ctrl Pts',(16.1458501215178,-20.9993769348045,
90.5008555196454));
#111791=CARTESIAN_POINT('Ctrl Pts',(16.0711452907451,-21.0000054222429,
90.6083385543735));
#111792=CARTESIAN_POINT('Ctrl Pts',(15.9945999617102,-20.9999999647811,
90.7168879103833));
#111793=CARTESIAN_POINT('Ctrl Pts',(15.8639252795662,-20.9999906480521,
90.9021984025108));
#111794=CARTESIAN_POINT('Ctrl Pts',(15.7278791641397,-20.9981364242747,
91.0905957924792));
#111795=CARTESIAN_POINT('Ctrl Pts',(15.5862297149464,-20.9940124499549,
91.2815743670219));
#111796=CARTESIAN_POINT('Ctrl Pts',(15.5378464502222,-20.9926038222309,
91.3468070028096));
#111797=CARTESIAN_POINT('Ctrl Pts',(15.4888096188265,-20.9909299770618,
91.4123407552541));
#111798=CARTESIAN_POINT('Ctrl Pts',(15.4391105631588,-20.9889727067707,
91.4781553681437));
#111799=CARTESIAN_POINT('Ctrl Pts',(15.3415102205454,-20.9851289667152,
91.6074038755989));
#111800=CARTESIAN_POINT('Ctrl Pts',(15.241354021653,-20.9801928015274,91.7377286021338));
#111801=CARTESIAN_POINT('Ctrl Pts',(15.1385783549149,-20.9740185000755,
91.8689881476138));
#111802=CARTESIAN_POINT('Ctrl Pts',(15.0871905215459,-20.9709313493496,
91.9346179203538));
#111803=CARTESIAN_POINT('Ctrl Pts',(15.0351478300591,-20.9675344999767,
92.0004813962707));
#111804=CARTESIAN_POINT('Ctrl Pts',(14.9824426596947,-20.9638087425081,
92.0665607210304));
#111805=CARTESIAN_POINT('Ctrl Pts',(14.9560900745125,-20.9619458637738,
92.0996003834102));
#111806=CARTESIAN_POINT('Ctrl Pts',(14.9295718702518,-20.9600007473097,
92.1326940078877));
#111807=CARTESIAN_POINT('Ctrl Pts',(14.9028870985181,-20.9579709275709,
92.1658392895054));
#111808=CARTESIAN_POINT('Ctrl Pts',(14.8895447126513,-20.9569560177015,
92.1824119303143));
#111809=CARTESIAN_POINT('Ctrl Pts',(14.8761606849662,-20.9559199313282,
92.1989974853993));
#111810=CARTESIAN_POINT('Ctrl Pts',(14.8627348982699,-20.954862356187,92.2155956664944));
#111811=CARTESIAN_POINT('Ctrl Pts',(14.8560220049218,-20.9543335686164,
92.2238947570419));
#111812=CARTESIAN_POINT('Ctrl Pts',(14.8492986718242,-20.9537994088106,
92.2321970040914));
#111813=CARTESIAN_POINT('Ctrl Pts',(14.8425648843961,-20.9532598374809,
92.2405023714394));
#111814=CARTESIAN_POINT('Ctrl Pts',(14.8358310969679,-20.9527202661512,
92.2488077387874));
#111815=CARTESIAN_POINT('Ctrl Pts',(14.8277837298359,-20.9520690930638,
92.2587197029694));
#111816=CARTESIAN_POINT('Ctrl Pts',(14.8223321445671,-20.9516248494587,
92.265427798123));
#111817=CARTESIAN_POINT('Ctrl Pts',(14.6197148893987,-20.9351137952504,
92.5147453379572));
#111818=CARTESIAN_POINT('Ctrl Pts',(14.4184351440027,-20.9145672747272,
92.7538762471074));
#111819=CARTESIAN_POINT('Ctrl Pts',(14.2190755019638,-20.8903363637757,
92.9833072479781));
#111820=CARTESIAN_POINT('Ctrl Pts',(14.0175137590704,-20.8658378013116,
93.2152725140488));
#111821=CARTESIAN_POINT('Ctrl Pts',(13.8179149930755,-20.8375732619276,
93.437322361534));
#111822=CARTESIAN_POINT('Ctrl Pts',(13.6208541261277,-20.8059516975061,
93.6499646150171));
#111823=CARTESIAN_POINT('Ctrl Pts',(13.4198692877072,-20.773700469171,93.8668411040918));
#111824=CARTESIAN_POINT('Ctrl Pts',(13.2215246559016,-20.7379574539372,
94.0739315713755));
#111825=CARTESIAN_POINT('Ctrl Pts',(13.0263985330229,-20.6992003520432,
94.2717803668916));
#111826=CARTESIAN_POINT('Ctrl Pts',(12.950382145547,-20.6841015286179,94.3488574413484));
#111827=CARTESIAN_POINT('Ctrl Pts',(12.8748538757691,-20.6685457010464,
94.4245319769535));
#111828=CARTESIAN_POINT('Ctrl Pts',(12.7998465499645,-20.6525627178891,
94.4988363996149));
#111829=CARTESIAN_POINT('Ctrl Pts',(12.5995488236742,-20.6098821510059,
94.6972571105621));
#111830=CARTESIAN_POINT('Ctrl Pts',(12.4030580629536,-20.564173130271,94.8857858123521));
#111831=CARTESIAN_POINT('Ctrl Pts',(12.2109457221164,-20.5160407252881,
95.0649321222251));
#111832=CARTESIAN_POINT('Ctrl Pts',(12.0946798390561,-20.4869111204706,
95.1733509974708));
#111833=CARTESIAN_POINT('Ctrl Pts',(11.9800168330081,-20.4568946482348,
95.2783335792123));
#111834=CARTESIAN_POINT('Ctrl Pts',(11.8670762772347,-20.4261311415844,
95.3799940814724));
#111835=CARTESIAN_POINT('Ctrl Pts',(11.7172971370492,-20.3853332940472,
95.5148138768514));
#111836=CARTESIAN_POINT('Ctrl Pts',(11.5705393370016,-20.3432198853979,
95.6437907033954));
#111837=CARTESIAN_POINT('Ctrl Pts',(11.4270094765659,-20.3001074782512,
95.7672229849734));
#111838=CARTESIAN_POINT('Ctrl Pts',(11.3552445463481,-20.2785512746779,
95.8289391257624));
#111839=CARTESIAN_POINT('Ctrl Pts',(11.2842843329623,-20.2567446980296,
95.8892731513699));
#111840=CARTESIAN_POINT('Ctrl Pts',(11.2141462900269,-20.2347248452646,
95.9482742817537));
#111841=CARTESIAN_POINT('Ctrl Pts',(11.1790772685592,-20.2237149188821,
95.9777748469456));
#111842=CARTESIAN_POINT('Ctrl Pts',(11.1442137907282,-20.212651672305,96.006942188151));
#111843=CARTESIAN_POINT('Ctrl Pts',(11.1095578622534,-20.2015396909313,
96.0357822745056));
#111844=CARTESIAN_POINT('Ctrl Pts',(11.092229898016,-20.1959837002445,96.0502023176828));
#111845=CARTESIAN_POINT('Ctrl Pts',(11.0749538211899,-20.1904155257147,
96.0645405471347));
#111846=CARTESIAN_POINT('Ctrl Pts',(11.0577298778451,-20.1848357384477,
96.0787977035608));
#111847=CARTESIAN_POINT('Ctrl Pts',(11.0405059345003,-20.1792559511808,
96.0930548599869));
#111848=CARTESIAN_POINT('Ctrl Pts',(11.0223622512192,-20.1733464993521,
96.1080311634234));
#111849=CARTESIAN_POINT('Ctrl Pts',(11.0062146916286,-20.1680621081994,
96.121326691339));
#111850=CARTESIAN_POINT('Ctrl Pts',(10.8884352616903,-20.1295180437516,
96.2183035558513));
#111851=CARTESIAN_POINT('Ctrl Pts',(10.7650451892595,-20.0878025554444,
96.3182483504631));
#111852=CARTESIAN_POINT('Ctrl Pts',(10.6359923950788,-20.0424861616342,
96.4207018070726));
#111853=CARTESIAN_POINT('Ctrl Pts',(10.5090870124052,-19.9979238231403,
96.5214504595896));
#111854=CARTESIAN_POINT('Ctrl Pts',(10.3767055579604,-19.9498793225477,
96.6246250229459));
#111855=CARTESIAN_POINT('Ctrl Pts',(10.2388294415599,-19.8979046255969,
96.7297833218371));
#111856=CARTESIAN_POINT('Ctrl Pts',(10.2093519003149,-19.8867925757868,
96.7522658820785));
#111857=CARTESIAN_POINT('Ctrl Pts',(10.179623323687,-19.8755007363343,96.7748390959961));
#111858=CARTESIAN_POINT('Ctrl Pts',(10.1496437342186,-19.8640244953124,
96.7974986064136));
#111859=CARTESIAN_POINT('Ctrl Pts',(10.0131088563521,-19.8117586973457,
96.900695933069));
#111860=CARTESIAN_POINT('Ctrl Pts',(9.87136065174339,-19.7556701351067,
97.0056761354688));
#111861=CARTESIAN_POINT('Ctrl Pts',(9.72439985909457,-19.6952952121385,
97.1119880032428));
#111862=CARTESIAN_POINT('Ctrl Pts',(9.70301722964254,-19.6865107289933,
97.127456260007));
#111863=CARTESIAN_POINT('Ctrl Pts',(9.68152431320116,-19.6776354405432,
97.1429526968982));
#111864=CARTESIAN_POINT('Ctrl Pts',(9.65992117791659,-19.6686678541629,
97.1584759124834));
#111865=CARTESIAN_POINT('Ctrl Pts',(9.57488145606972,-19.6333673738679,
97.2195823175561));
#111866=CARTESIAN_POINT('Ctrl Pts',(9.48813335101792,-19.5966369901423,
97.2811030929347));
#111867=CARTESIAN_POINT('Ctrl Pts',(9.39968075361787,-19.5583821832216,
97.3429497450282));
#111868=CARTESIAN_POINT('Ctrl Pts',(9.35545445491785,-19.5392547797613,
97.373873071075));
#111869=CARTESIAN_POINT('Ctrl Pts',(9.31080177844068,-19.5197460783091,
97.404877982857));
#111870=CARTESIAN_POINT('Ctrl Pts',(9.26572212530421,-19.4998432260331,
97.4359539001361));
#111871=CARTESIAN_POINT('Ctrl Pts',(9.24318229873596,-19.4898917998951,
97.4514918587756));
#111872=CARTESIAN_POINT('Ctrl Pts',(9.2205357302005,-19.4798418302812,97.4670475684018));
#111873=CARTESIAN_POINT('Ctrl Pts',(9.19778234848026,-19.4696916719074,
97.4826196977618));
#111874=CARTESIAN_POINT('Ctrl Pts',(9.17759947653245,-19.4606882037976,
97.4964326024408));
#111875=CARTESIAN_POINT('Ctrl Pts',(9.15850227514913,-19.4521318460541,
97.509463956387));
#111876=CARTESIAN_POINT('Ctrl Pts',(9.13737792818021,-19.442622036599,97.5238269917626));
#111877=CARTESIAN_POINT('Ctrl Pts',(9.13468751125341,-19.4414108582195,
97.5256562816125));
#111878=CARTESIAN_POINT('Ctrl Pts',(9.13196423804468,-19.4401841502082,
97.5275071678908));
#111879=CARTESIAN_POINT('Ctrl Pts',(9.12920170123955,-19.438938961009,97.5293840121857));
#111880=CARTESIAN_POINT('Ctrl Pts',(8.97159247985769,-19.3678979888895,
97.6364623929759));
#111881=CARTESIAN_POINT('Ctrl Pts',(8.82132163286598,-19.297661080258,97.7355501748584));
#111882=CARTESIAN_POINT('Ctrl Pts',(8.67847795146037,-19.2289123285112,
97.827347023819));
#111883=CARTESIAN_POINT('Ctrl Pts',(8.53637141728977,-19.1605183558611,
97.9186701535871));
#111884=CARTESIAN_POINT('Ctrl Pts',(8.40161506174884,-19.0935973385942,
98.0027774994623));
#111885=CARTESIAN_POINT('Ctrl Pts',(8.2742860773703,-19.0287724910504,98.0803597553401));
#111886=CARTESIAN_POINT('Ctrl Pts',(8.21188246514141,-18.9970019977204,
98.118382622131));
#111887=CARTESIAN_POINT('Ctrl Pts',(8.15126276779457,-18.9657342161231,
98.1548382102798));
#111888=CARTESIAN_POINT('Ctrl Pts',(8.09243574634408,-18.9350379362716,
98.189807885219));
#111889=CARTESIAN_POINT('Ctrl Pts',(7.97432291785049,-18.8734059795942,
98.2600199598188));
#111890=CARTESIAN_POINT('Ctrl Pts',(7.86344177255187,-18.8140842306675,
98.3242349742202));
#111891=CARTESIAN_POINT('Ctrl Pts',(7.75982152702706,-18.7575887951892,
98.3829026523117));
#111892=CARTESIAN_POINT('Ctrl Pts',(7.65766080209592,-18.7018891139683,
98.4407439794915));
#111893=CARTESIAN_POINT('Ctrl Pts',(7.56255748665104,-18.6489366720524,
98.4931932096756));
#111894=CARTESIAN_POINT('Ctrl Pts',(7.47454698907051,-18.599176189517,98.5406800232808));
#111895=CARTESIAN_POINT('Ctrl Pts',(7.42545862910158,-18.5714219948916,
98.5671660660156));
#111896=CARTESIAN_POINT('Ctrl Pts',(7.37857695068473,-18.5446598983877,
98.5921083139664));
#111897=CARTESIAN_POINT('Ctrl Pts',(7.3339097744812,-18.5189601938225,98.6155810266187));
#111898=CARTESIAN_POINT('',(20.1853266918894,-19.2601884204994,66.2798123698034));
#111899=CARTESIAN_POINT('Ctrl Pts',(20.8003130805373,-19.9701890903422,
80.5583314866067));
#111900=CARTESIAN_POINT('Ctrl Pts',(20.8693517674825,-19.9348504256637,
80.3241935365105));
#111901=CARTESIAN_POINT('Ctrl Pts',(20.9340572556619,-19.8998450129912,
80.0878996375295));
#111902=CARTESIAN_POINT('Ctrl Pts',(20.9945301042509,-19.8653108990239,
79.8495426717956));
#111903=CARTESIAN_POINT('Ctrl Pts',(21.0567390479627,-19.8297853565356,
79.6043427943189));
#111904=CARTESIAN_POINT('Ctrl Pts',(21.114469100563,-19.7947582593351,79.3569593518495));
#111905=CARTESIAN_POINT('Ctrl Pts',(21.1677909493497,-19.7603764178263,
79.1074541702422));
#111906=CARTESIAN_POINT('Ctrl Pts',(21.2217202654601,-19.7256028823736,
78.8551065094565));
#111907=CARTESIAN_POINT('Ctrl Pts',(21.2711405458537,-19.69148904593,78.6005880097649));
#111908=CARTESIAN_POINT('Ctrl Pts',(21.3160825670536,-19.6581882435229,
78.3439294715529));
#111909=CARTESIAN_POINT('Ctrl Pts',(21.3613562815535,-19.6246416654977,
78.0853766723521));
#111910=CARTESIAN_POINT('Ctrl Pts',(21.4020855646709,-19.5919198042393,
77.8246516127711));
#111911=CARTESIAN_POINT('Ctrl Pts',(21.4382564880266,-19.5601862163097,
77.5617598999891));
#111912=CARTESIAN_POINT('Ctrl Pts',(21.457389480998,-19.5434003989049,77.4227005444004));
#111913=CARTESIAN_POINT('Ctrl Pts',(21.4752462723882,-19.526891246666,77.2830345749271));
#111914=CARTESIAN_POINT('Ctrl Pts',(21.4918194609359,-19.5106842624389,
77.1427606810275));
#111915=CARTESIAN_POINT('Ctrl Pts',(21.4944245268027,-19.5081367586021,
77.1207116509367));
#111916=CARTESIAN_POINT('Ctrl Pts',(21.4969978707424,-19.5055967227096,
77.0986475982832));
#111917=CARTESIAN_POINT('Ctrl Pts',(21.4995394653114,-19.5030642620853,
77.0765685070557));
#111918=CARTESIAN_POINT('Ctrl Pts',(21.530476373452,-19.4722385345451,76.8078164309129));
#111919=CARTESIAN_POINT('Ctrl Pts',(21.5565518241076,-19.4427769274193,
76.5394083958368));
#111920=CARTESIAN_POINT('Ctrl Pts',(21.5778555625257,-19.4148397515947,
76.2713465444692));
#111921=CARTESIAN_POINT('Ctrl Pts',(21.5996338853268,-19.3862802179901,
75.9973130666279));
#111922=CARTESIAN_POINT('Ctrl Pts',(21.616425632465,-19.3593134816969,75.7236407970041));
#111923=CARTESIAN_POINT('Ctrl Pts',(21.6282776573137,-19.3341145590584,
75.4503097843522));
#111924=CARTESIAN_POINT('Ctrl Pts',(21.6308381967374,-19.3286705243326,
75.3912587072136));
#111925=CARTESIAN_POINT('Ctrl Pts',(21.6331679963451,-19.3233090247849,
75.3322234956698));
#111926=CARTESIAN_POINT('Ctrl Pts',(21.6352672286914,-19.318031869621,75.2732038565701));
#111927=CARTESIAN_POINT('Ctrl Pts',(21.6449021796313,-19.2938110485219,
75.0023184883027));
#111928=CARTESIAN_POINT('Ctrl Pts',(21.6496981660391,-19.2713608165736,
74.7317683257853));
#111929=CARTESIAN_POINT('Ctrl Pts',(21.6497200847025,-19.2508299383448,
74.461543434535));
#111930=CARTESIAN_POINT('Ctrl Pts',(21.6497224177521,-19.248644606381,74.432780364311));
#111931=CARTESIAN_POINT('Ctrl Pts',(21.6496706180902,-19.2464810275705,
74.4040209596642));
#111932=CARTESIAN_POINT('Ctrl Pts',(21.649564732648,-19.2443393870614,74.3752651953395));
#111933=CARTESIAN_POINT('Ctrl Pts',(21.6490144007076,-19.2332083651463,
74.2258091864862));
#111934=CARTESIAN_POINT('Ctrl Pts',(21.6470044611232,-19.2226694685617,
74.0764521542778));
#111935=CARTESIAN_POINT('Ctrl Pts',(21.6435453264523,-19.2127466707316,
73.9271922751806));
#111936=CARTESIAN_POINT('Ctrl Pts',(21.6418157591168,-19.2077852718166,
73.852562335632));
#111937=CARTESIAN_POINT('Ctrl Pts',(21.6397238894754,-19.2029778865437,
73.7779566852953));
#111938=CARTESIAN_POINT('Ctrl Pts',(21.6372710124363,-19.1983274454553,
73.7033751000254));
#111939=CARTESIAN_POINT('Ctrl Pts',(21.6360445739167,-19.1960022249111,
73.6660843073905));
#111940=CARTESIAN_POINT('Ctrl Pts',(21.6347278833634,-19.1937162398297,
73.6287995310882));
#111941=CARTESIAN_POINT('Ctrl Pts',(21.6333211017679,-19.1914698531506,
73.591520743483));
#111942=CARTESIAN_POINT('Ctrl Pts',(21.63240594926,-19.1900085130181,73.5672698035514));
#111943=CARTESIAN_POINT('Ctrl Pts',(21.631475228432,-19.1885975748809,73.5435881702707));
#111944=CARTESIAN_POINT('Ctrl Pts',(21.6304856119411,-19.1871711967383,
73.5193697745296));
#111945=CARTESIAN_POINT('Ctrl Pts',(21.6299539800565,-19.1864049321227,
73.5063594099209));
#111946=CARTESIAN_POINT('Ctrl Pts',(21.6294051186618,-19.1856343118572,
73.4931941227504));
#111947=CARTESIAN_POINT('Ctrl Pts',(21.6288306371666,-19.1848498327995,
73.4797023206213));
#111948=CARTESIAN_POINT('Ctrl Pts',(21.6157703631309,-19.1670154698935,
73.1729794156769));
#111949=CARTESIAN_POINT('Ctrl Pts',(21.5968588497906,-19.1518257309308,
72.8673669315517));
#111950=CARTESIAN_POINT('Ctrl Pts',(21.5721718462519,-19.1392405801733,
72.56284336669));
#111951=CARTESIAN_POINT('Ctrl Pts',(21.5481808736999,-19.1270102580157,
72.2669056084043));
#111952=CARTESIAN_POINT('Ctrl Pts',(21.5187351461639,-19.1172400266441,
71.9719958689088));
#111953=CARTESIAN_POINT('Ctrl Pts',(21.4838572420696,-19.1099176660947,
71.6781041186082));
#111954=CARTESIAN_POINT('Ctrl Pts',(21.4474615106792,-19.1022766488198,
71.3714226972449));
#111955=CARTESIAN_POINT('Ctrl Pts',(21.4051507480994,-19.0973011977332,
71.0658491976107));
#111956=CARTESIAN_POINT('Ctrl Pts',(21.356898873141,-19.0950025685149,70.7613904286314));
#111957=CARTESIAN_POINT('Ctrl Pts',(21.3086469981827,-19.0927039392965,
70.4569316596521));
#111958=CARTESIAN_POINT('Ctrl Pts',(21.2544538761582,-19.0930823045507,
70.1535870956215));
#111959=CARTESIAN_POINT('Ctrl Pts',(21.1942425951636,-19.0961719049028,
69.8513897421172));
#111960=CARTESIAN_POINT('Ctrl Pts',(21.1925947750517,-19.0962564589185,
69.8431194168786));
#111961=CARTESIAN_POINT('Ctrl Pts',(21.1909424444303,-19.096343044904,69.8348499527977));
#111962=CARTESIAN_POINT('Ctrl Pts',(21.1892856007267,-19.0964316635041,
69.8265813512942));
#111963=CARTESIAN_POINT('Ctrl Pts',(21.1291719765333,-19.099646924672,69.5265798470562));
#111964=CARTESIAN_POINT('Ctrl Pts',(21.0631154256295,-19.1055357127208,
69.2276730546282));
#111965=CARTESIAN_POINT('Ctrl Pts',(20.9911889415531,-19.1140355588776,
68.9298794956225));
#111966=CARTESIAN_POINT('Ctrl Pts',(20.9222243626543,-19.1221853846119,
68.6443489617823));
#111967=CARTESIAN_POINT('Ctrl Pts',(20.8478629914071,-19.132735653614,68.3598413343251));
#111968=CARTESIAN_POINT('Ctrl Pts',(20.7681210589116,-19.1456510231459,
68.0763599944801));
#111969=CARTESIAN_POINT('Ctrl Pts',(20.6884849972535,-19.1585492453508,
67.7932550238287));
#111970=CARTESIAN_POINT('Ctrl Pts',(20.6034826469697,-19.1738061512652,
67.5111732148898));
#111971=CARTESIAN_POINT('Ctrl Pts',(20.5130832815626,-19.1914078429555,
67.230111460685));
#111972=CARTESIAN_POINT('Ctrl Pts',(20.4232562861313,-19.2088980882899,
66.9508292688561));
#111973=CARTESIAN_POINT('Ctrl Pts',(20.3281003670252,-19.2287033836298,
66.6725538637127));
#111974=CARTESIAN_POINT('Ctrl Pts',(20.2275394059576,-19.2508331871437,
66.3952817249783));
#111975=CARTESIAN_POINT('Ctrl Pts',(20.2135729243897,-19.2539067008572,
66.3567725841169));
#111976=CARTESIAN_POINT('Ctrl Pts',(20.1995021111998,-19.2570250911829,
66.3182828002111));
#111977=CARTESIAN_POINT('Ctrl Pts',(20.185326692289,-19.2601884214332,66.279812369733));
#111978=CARTESIAN_POINT('',(13.2733353822638,-20.6712011577472,53.9604717079333));
#111979=CARTESIAN_POINT('Ctrl Pts',(20.1853266911301,-19.2601884187249,
66.2798123699373));
#111980=CARTESIAN_POINT('Ctrl Pts',(19.9639238128775,-19.3096532241205,
65.6797118301511));
#111981=CARTESIAN_POINT('Ctrl Pts',(19.7324395957548,-19.3632476924122,
65.0873419883912));
#111982=CARTESIAN_POINT('Ctrl Pts',(19.4905820811039,-19.4200461661253,
64.5026985997605));
#111983=CARTESIAN_POINT('Ctrl Pts',(19.2540984564514,-19.4755826209582,
63.9310455424963));
#111984=CARTESIAN_POINT('Ctrl Pts',(19.0076974411245,-19.5341827396344,
63.3667794154196));
#111985=CARTESIAN_POINT('Ctrl Pts',(18.7510919294293,-19.5949556358985,
62.8099349966494));
#111986=CARTESIAN_POINT('Ctrl Pts',(18.5010868593336,-19.6541653235239,
62.2674138051626));
#111987=CARTESIAN_POINT('Ctrl Pts',(18.2413954218763,-19.7154377803506,
61.7319375615219));
#111988=CARTESIAN_POINT('Ctrl Pts',(17.9717387621731,-19.7779188948128,
61.2035744117988));
#111989=CARTESIAN_POINT('Ctrl Pts',(17.7264912021937,-19.8347442700271,
60.7230382611426));
#111990=CARTESIAN_POINT('Ctrl Pts',(17.4730006172305,-19.8925692715409,
60.2483861746423));
#111991=CARTESIAN_POINT('Ctrl Pts',(17.2110485793565,-19.9507253148562,
59.7796949716318));
#111992=CARTESIAN_POINT('Ctrl Pts',(16.8765459538633,-20.0249883339003,
59.1811944246422));
#111993=CARTESIAN_POINT('Ctrl Pts',(16.5282261267346,-20.0997910946465,
58.5923244407021));
#111994=CARTESIAN_POINT('Ctrl Pts',(16.1659512285725,-20.1735844006505,
58.0131600374827));
#111995=CARTESIAN_POINT('Ctrl Pts',(15.8003816564756,-20.2480488127208,
57.4287284797547));
#111996=CARTESIAN_POINT('Ctrl Pts',(15.4206023598391,-20.3214850259089,
56.8541798870247));
#111997=CARTESIAN_POINT('Ctrl Pts',(15.02646619411,-20.3922681421323,56.2895497896133));
#111998=CARTESIAN_POINT('Ctrl Pts',(14.633836087486,-20.4627807844282,55.7270772366576));
#111999=CARTESIAN_POINT('Ctrl Pts',(14.2269592157691,-20.5306601412776,
55.174447565923));
#112000=CARTESIAN_POINT('Ctrl Pts',(13.8056778443051,-20.5942727051615,
54.6316544273006));
#112001=CARTESIAN_POINT('Ctrl Pts',(13.6307190985375,-20.6206910923631,
54.4062316738221));
#112002=CARTESIAN_POINT('Ctrl Pts',(13.4532757341929,-20.6463732760865,
54.1825049800934));
#112003=CARTESIAN_POINT('Ctrl Pts',(13.2733353822638,-20.6712011577472,
53.9604717079333));
#112004=CARTESIAN_POINT('',(28.7710188797691,-10.4923807534,58.41162797882));
#112005=CARTESIAN_POINT('Ctrl Pts',(13.2733141368383,-20.6710805729304,
53.9604754110713));
#112006=CARTESIAN_POINT('Ctrl Pts',(13.9841764899668,-20.5495789480866,
54.0805152897853));
#112007=CARTESIAN_POINT('Ctrl Pts',(14.7282334585067,-20.3881365720002,
54.2176652013888));
#112008=CARTESIAN_POINT('Ctrl Pts',(15.8847581423893,-20.0711689328545,
54.4507042540058));
#112009=CARTESIAN_POINT('Ctrl Pts',(16.2769694543064,-19.9530421498621,
54.5329427913844));
#112010=CARTESIAN_POINT('Ctrl Pts',(16.873811067161,-19.7552656153632,54.6634086502063));
#112011=CARTESIAN_POINT('Ctrl Pts',(17.1743591090601,-19.6512310990377,
54.7304192850255));
#112012=CARTESIAN_POINT('Ctrl Pts',(17.528343737373,-19.5204462814834,54.8117758920654));
#112013=CARTESIAN_POINT('Ctrl Pts',(17.7061218899511,-19.4526510713967,
54.8532574786262));
#112014=CARTESIAN_POINT('Ctrl Pts',(17.8047452127824,-19.4144496322295,
54.8764440875232));
#112015=CARTESIAN_POINT('Ctrl Pts',(17.8525287220213,-19.3957608171072,
54.8877312234457));
#112016=CARTESIAN_POINT('Ctrl Pts',(17.8780285888305,-19.3857423884871,
54.8937679482584));
#112017=CARTESIAN_POINT('Ctrl Pts',(17.8826006853678,-19.3839445927825,
54.8948507695666));
#112018=CARTESIAN_POINT('Ctrl Pts',(18.3461491916568,-19.2015909106345,
55.004658230301));
#112019=CARTESIAN_POINT('Ctrl Pts',(18.9423634053891,-18.9517707804932,
55.1520850386185));
#112020=CARTESIAN_POINT('Ctrl Pts',(20.0118215345656,-18.4256300462586,
55.4349797018328));
#112021=CARTESIAN_POINT('Ctrl Pts',(20.3973067217419,-18.2248068595463,
55.5396038906132));
#112022=CARTESIAN_POINT('Ctrl Pts',(21.0135595061523,-17.877726763274,55.7129942885508));
#112023=CARTESIAN_POINT('Ctrl Pts',(21.2252972341605,-17.7543836707307,
55.7735365026662));
#112024=CARTESIAN_POINT('Ctrl Pts',(21.5515283692713,-17.5568701641081,
55.8686188214076));
#112025=CARTESIAN_POINT('Ctrl Pts',(21.7167981636613,-17.4549881517412,
55.9172275667681));
#112026=CARTESIAN_POINT('Ctrl Pts',(21.9131746404238,-17.3304278318108,
55.9758427529778));
#112027=CARTESIAN_POINT('Ctrl Pts',(21.9980755025342,-17.2757991118417,
56.0013759384972));
#112028=CARTESIAN_POINT('Ctrl Pts',(22.0548377387607,-17.239100387009,56.0184901764203));
#112029=CARTESIAN_POINT('Ctrl Pts',(22.0850046758637,-17.2194983132274,
56.0276100469492));
#112030=CARTESIAN_POINT('Ctrl Pts',(22.970607285989,-16.6414242908076,56.2959916733566));
#112031=CARTESIAN_POINT('Ctrl Pts',(23.6941088994417,-16.0887360872919,
56.5305409235564));
#112032=CARTESIAN_POINT('Ctrl Pts',(24.6061141279826,-15.3253454244035,
56.838587368009));
#112033=CARTESIAN_POINT('Ctrl Pts',(24.881279478639,-15.0816052976648,56.9339665526185));
#112034=CARTESIAN_POINT('Ctrl Pts',(25.2544866897691,-14.7370181148781,
57.0654260457647));
#112035=CARTESIAN_POINT('Ctrl Pts',(25.372297233081,-14.6256479916899,57.1073113002769));
#112036=CARTESIAN_POINT('Ctrl Pts',(25.5395659314602,-14.4643497436218,
57.1671596145233));
#112037=CARTESIAN_POINT('Ctrl Pts',(25.6208381919006,-14.3851388691851,
57.1963389343571));
#112038=CARTESIAN_POINT('Ctrl Pts',(25.7116149185979,-14.295346440036,57.2290616554915));
#112039=CARTESIAN_POINT('Ctrl Pts',(25.7560043421324,-14.2511174768788,
57.2450910710458));
#112040=CARTESIAN_POINT('Ctrl Pts',(25.779518318372,-14.2276037293349,57.253589079426));
#112041=CARTESIAN_POINT('Ctrl Pts',(25.7904192795905,-14.216679956226,57.2575305044926));
#112042=CARTESIAN_POINT('Ctrl Pts',(25.7966307490415,-14.210449915369,57.2597767868312));
#112043=CARTESIAN_POINT('Ctrl Pts',(25.7972859739144,-14.2097928030817,
57.2600137336337));
#112044=CARTESIAN_POINT('Ctrl Pts',(27.052134281417,-12.950440255771,57.7138669097972));
#112045=CARTESIAN_POINT('Ctrl Pts',(28.0205851764319,-11.680375794482,58.1013187451067));
#112046=CARTESIAN_POINT('Ctrl Pts',(28.7710188797691,-10.4923807534,58.41162797882));
#112047=CARTESIAN_POINT('',(28.0568193669707,-11.8824454183442,59.4053060271813));
#112048=CARTESIAN_POINT('Ctrl Pts',(28.7710784579986,-10.4924156479171,
58.4116174735707));
#112049=CARTESIAN_POINT('Ctrl Pts',(28.6520180730878,-10.7462094425941,
58.5794007290748));
#112050=CARTESIAN_POINT('Ctrl Pts',(28.5266025564978,-11.0009695937572,
58.7551107743632));
#112051=CARTESIAN_POINT('Ctrl Pts',(28.3944692472976,-11.2561596613471,
58.9388115563428));
#112052=CARTESIAN_POINT('Ctrl Pts',(28.2864693695974,-11.4647406486609,
59.0889603879079));
#112053=CARTESIAN_POINT('Ctrl Pts',(28.173981775152,-11.6736080079964,59.2444475481057));
#112054=CARTESIAN_POINT('Ctrl Pts',(28.0568192479267,-11.8824453353875,
59.4053060481747));
#112055=CARTESIAN_POINT('',(23.3999522636103,-18.464444554609,75.101511144554));
#112056=CARTESIAN_POINT('Ctrl Pts',(23.3999522655726,-18.464444558287,75.101511144208));
#112057=CARTESIAN_POINT('Ctrl Pts',(23.2442504171342,-18.4724359023458,
74.3034287395727));
#112058=CARTESIAN_POINT('Ctrl Pts',(23.1780163711756,-18.4339280942775,
73.5030778454822));
#112059=CARTESIAN_POINT('Ctrl Pts',(23.1802594857303,-18.3571062469603,
72.7196600622127));
#112060=CARTESIAN_POINT('Ctrl Pts',(23.180481137904,-18.3495151369095,72.6422470499488));
#112061=CARTESIAN_POINT('Ctrl Pts',(23.1813714219944,-18.3415498815759,
72.5649993563833));
#112062=CARTESIAN_POINT('Ctrl Pts',(23.1829100823713,-18.3332183575115,
72.4879354920009));
#112063=CARTESIAN_POINT('Ctrl Pts',(23.1861430175238,-18.3157126899674,
72.326013810071));
#112064=CARTESIAN_POINT('Ctrl Pts',(23.1922383893482,-18.2965900320351,
72.1649036942477));
#112065=CARTESIAN_POINT('Ctrl Pts',(23.2009883276532,-18.2759250242208,
72.0047382896764));
#112066=CARTESIAN_POINT('Ctrl Pts',(23.2101646253119,-18.2542530699494,
71.8367684851189));
#112067=CARTESIAN_POINT('Ctrl Pts',(23.2222604923313,-18.2308847946912,
71.6698377009382));
#112068=CARTESIAN_POINT('Ctrl Pts',(23.2370361194293,-18.2059062397654,
71.5040994657693));
#112069=CARTESIAN_POINT('Ctrl Pts',(23.2444239329783,-18.1934169623025,
71.4212303481849));
#112070=CARTESIAN_POINT('Ctrl Pts',(23.2524816860625,-18.1805251140686,
71.3386593679393));
#112071=CARTESIAN_POINT('Ctrl Pts',(23.2611793963984,-18.167241446654,71.2564057115819));
#112072=CARTESIAN_POINT('Ctrl Pts',(23.2655282515664,-18.1605996129467,
71.2152788834032));
#112073=CARTESIAN_POINT('Ctrl Pts',(23.2700370960191,-18.1538598243939,
71.1742313862016));
#112074=CARTESIAN_POINT('Ctrl Pts',(23.2747021816155,-18.1470234247457,
71.1332656182255));
#112075=CARTESIAN_POINT('Ctrl Pts',(23.2770347244138,-18.1436052249216,
71.1127827342374));
#112076=CARTESIAN_POINT('Ctrl Pts',(23.2794063274962,-18.1401628723206,
71.092320282556));
#112077=CARTESIAN_POINT('Ctrl Pts',(23.2818165223192,-18.1366965349008,
71.0718785629479));
#112078=CARTESIAN_POINT('Ctrl Pts',(23.2840165943302,-18.1335323956928,
71.0532189696487));
#112079=CARTESIAN_POINT('Ctrl Pts',(23.2863812828526,-18.1301605764761,
71.0334842977952));
#112080=CARTESIAN_POINT('Ctrl Pts',(23.2885475771853,-18.1270951478395,
71.0156661841902));
#112081=CARTESIAN_POINT('Ctrl Pts',(23.2887544739842,-18.1268023772022,
71.013964425287));
#112082=CARTESIAN_POINT('Ctrl Pts',(23.2889595309406,-18.1265124201898,
71.0122801319039));
#112083=CARTESIAN_POINT('Ctrl Pts',(23.2891624134535,-18.1262257361339,
71.0106159001072));
#112084=CARTESIAN_POINT('Ctrl Pts',(23.308094929816,-18.0994730579322,70.8553137241134));
#112085=CARTESIAN_POINT('Ctrl Pts',(23.3295344879901,-18.0708858315582,
70.6984480982839));
#112086=CARTESIAN_POINT('Ctrl Pts',(23.3534887181918,-18.0403985244464,
70.5402898531891));
#112087=CARTESIAN_POINT('Ctrl Pts',(23.3768886626381,-18.0106166743629,
70.3857912899808));
#112088=CARTESIAN_POINT('Ctrl Pts',(23.4026883528905,-17.9790216141216,
70.2300592039702));
#112089=CARTESIAN_POINT('Ctrl Pts',(23.4308580534758,-17.9455637192767,
70.0733780640497));
#112090=CARTESIAN_POINT('Ctrl Pts',(23.434960689978,-17.9406909099168,70.0505590155512));
#112091=CARTESIAN_POINT('Ctrl Pts',(23.4391135300745,-17.9357786088941,
70.0277198937643));
#112092=CARTESIAN_POINT('Ctrl Pts',(23.4433164126347,-17.9308266847173,
70.0048616365201));
#112093=CARTESIAN_POINT('Ctrl Pts',(23.4736395632365,-17.8950993141736,
69.8399428297306));
#112094=CARTESIAN_POINT('Ctrl Pts',(23.5065711797814,-17.8573088992603,
69.6740301896288));
#112095=CARTESIAN_POINT('Ctrl Pts',(23.5420629608149,-17.8173624707892,
69.5071378111653));
#112096=CARTESIAN_POINT('Ctrl Pts',(23.5766664919729,-17.7784157782876,
69.3444222344871));
#112097=CARTESIAN_POINT('Ctrl Pts',(23.6137037244022,-17.7374196096513,
69.1807754044067));
#112098=CARTESIAN_POINT('Ctrl Pts',(23.6530876871092,-17.6942940673088,
69.016184996999));
#112099=CARTESIAN_POINT('Ctrl Pts',(23.6666626215029,-17.6794294785841,
68.959453682301));
#112100=CARTESIAN_POINT('Ctrl Pts',(23.680515979294,-17.6643119662137,68.902610035373));
#112101=CARTESIAN_POINT('Ctrl Pts',(23.69464296705,-17.6489384467432,68.8456528067277));
#112102=CARTESIAN_POINT('Ctrl Pts',(23.7421345988904,-17.5972562665504,
68.6541759129838));
#112103=CARTESIAN_POINT('Ctrl Pts',(23.7927217955473,-17.5426802486052,
68.4614134562826));
#112104=CARTESIAN_POINT('Ctrl Pts',(23.8463804832646,-17.4850732140897,
68.2676445481524));
#112105=CARTESIAN_POINT('Ctrl Pts',(23.8950188452369,-17.4328559140378,
68.0920047273971));
#112106=CARTESIAN_POINT('Ctrl Pts',(23.9461804840968,-17.378148278424,67.9155381604963));
#112107=CARTESIAN_POINT('Ctrl Pts',(23.9998135602292,-17.3208544174594,
67.7384663116596));
#112108=CARTESIAN_POINT('Ctrl Pts',(24.0090663139398,-17.3109701068276,
67.7079179574627));
#112109=CARTESIAN_POINT('Ctrl Pts',(24.0183925442965,-17.3010088373864,
67.6773516204896));
#112110=CARTESIAN_POINT('Ctrl Pts',(24.0277914314848,-17.2909703431112,
67.6467683916423));
#112111=CARTESIAN_POINT('Ctrl Pts',(24.0532747215613,-17.2637528804033,
67.5638477993878));
#112112=CARTESIAN_POINT('Ctrl Pts',(24.0792923072638,-17.2359676727507,
67.4808029949137));
#112113=CARTESIAN_POINT('Ctrl Pts',(24.1058261298632,-17.2076098987618,
67.3976560725148));
#112114=CARTESIAN_POINT('Ctrl Pts',(24.1190930411629,-17.1934310117674,
67.3560826113154));
#112115=CARTESIAN_POINT('Ctrl Pts',(24.1324890037314,-17.1791089716587,
67.3144836220376));
#112116=CARTESIAN_POINT('Ctrl Pts',(24.1460114838888,-17.1646432685094,
67.2728619224439));
#112117=CARTESIAN_POINT('Ctrl Pts',(24.1527727239675,-17.1574104169348,
67.252051072647));
#112118=CARTESIAN_POINT('Ctrl Pts',(24.159565592941,-17.1501416488662,67.2312345453598));
#112119=CARTESIAN_POINT('Ctrl Pts',(24.1663897642528,-17.1428369009422,
67.2104126946916));
#112120=CARTESIAN_POINT('Ctrl Pts',(24.1698018499088,-17.1391845269801,
67.2000017693575));
#112121=CARTESIAN_POINT('Ctrl Pts',(24.1732217611164,-17.135523158007,67.189589513184));
#112122=CARTESIAN_POINT('Ctrl Pts',(24.1766494560711,-17.1318527863852,
67.1791759706309));
#112123=CARTESIAN_POINT('Ctrl Pts',(24.1792202272872,-17.1291000076689,
67.1713658137161));
#112124=CARTESIAN_POINT('Ctrl Pts',(24.1817953768583,-17.1263421649588,
67.1635549332133));
#112125=CARTESIAN_POINT('Ctrl Pts',(24.1843748869266,-17.1235792550871,
67.1557433479229));
#112126=CARTESIAN_POINT('Ctrl Pts',(24.1852347236161,-17.1226582851298,
67.1531394861594));
#112127=CARTESIAN_POINT('Ctrl Pts',(24.1856906524357,-17.1221699380917,
67.1517588717565));
#112128=CARTESIAN_POINT('Ctrl Pts',(24.1869558498151,-17.1208146560523,
67.1479315284031));
#112129=CARTESIAN_POINT('Ctrl Pts',(24.2387975889492,-17.0652816782834,
66.991105298017));
#112130=CARTESIAN_POINT('Ctrl Pts',(24.2917423143794,-17.0084117511973,
66.8360284700413));
#112131=CARTESIAN_POINT('Ctrl Pts',(24.3455586218895,-16.9502826065249,
66.6827206321942));
#112132=CARTESIAN_POINT('Ctrl Pts',(24.4660146818045,-16.8201732018215,
66.3395744938665));
#112133=CARTESIAN_POINT('Ctrl Pts',(24.590837042828,-16.6837553719516,66.0052910913828));
#112134=CARTESIAN_POINT('Ctrl Pts',(24.7188691138333,-16.5407604417291,
65.6781616273983));
#112135=CARTESIAN_POINT('Ctrl Pts',(24.8016663349788,-16.4482868703236,
65.4666098625941));
#112136=CARTESIAN_POINT('Ctrl Pts',(24.8858059845019,-16.3530626625801,
65.2580498152435));
#112137=CARTESIAN_POINT('Ctrl Pts',(24.971082998648,-16.2551183064043,65.0525478755764));
#112138=CARTESIAN_POINT('Ctrl Pts',(25.0170926495023,-16.2022742232019,
64.9416730684712));
#112139=CARTESIAN_POINT('Ctrl Pts',(25.0634333874147,-16.1486383100985,
64.8316884608845));
#112140=CARTESIAN_POINT('Ctrl Pts',(25.1100730529789,-16.0942152806723,
64.7226044908374));
#112141=CARTESIAN_POINT('Ctrl Pts',(25.133392885761,-16.0670037659592,64.6680625058139));
#112142=CARTESIAN_POINT('Ctrl Pts',(25.1567874502383,-16.0395954719033,
64.6137456802135));
#112143=CARTESIAN_POINT('Ctrl Pts',(25.1802527304421,-16.0119909817087,
64.5596553197284));
#112144=CARTESIAN_POINT('Ctrl Pts',(25.2007848506203,-15.9878370527884,
64.5123262543039));
#112145=CARTESIAN_POINT('Ctrl Pts',(25.2213711125132,-15.963532911182,64.4651705762356));
#112146=CARTESIAN_POINT('Ctrl Pts',(25.2420088260471,-15.9390789460828,
64.4181891604787));
#112147=CARTESIAN_POINT('Ctrl Pts',(25.2449570708376,-15.9355855224972,
64.4114775296563));
#112148=CARTESIAN_POINT('Ctrl Pts',(25.2485512358567,-15.9313241295077,
64.4033040151405));
#112149=CARTESIAN_POINT('Ctrl Pts',(25.2508567027187,-15.9285895035509,
64.3980649396906));
#112150=CARTESIAN_POINT('Ctrl Pts',(25.3407766308797,-15.8219311196724,
64.1937257249921));
#112151=CARTESIAN_POINT('Ctrl Pts',(25.4304975710006,-15.7138504718903,
63.9955752199972));
#112152=CARTESIAN_POINT('Ctrl Pts',(25.5197348311737,-15.6046045178627,
63.8034270030152));
#112153=CARTESIAN_POINT('Ctrl Pts',(25.6111577516963,-15.4926828367948,
63.6065725597521));
#112154=CARTESIAN_POINT('Ctrl Pts',(25.7020723508946,-15.3795390166899,
63.4160187616832));
#112155=CARTESIAN_POINT('Ctrl Pts',(25.7921676115896,-15.2654993087428,
63.2316090580315));
#112156=CARTESIAN_POINT('Ctrl Pts',(25.8305858240952,-15.2168707604686,
63.1529734990873));
#112157=CARTESIAN_POINT('Ctrl Pts',(25.8688556221805,-15.1680790293793,
63.0754549574394));
#112158=CARTESIAN_POINT('Ctrl Pts',(25.9069553595192,-15.1191481839815,
62.9990405418654));
#112159=CARTESIAN_POINT('Ctrl Pts',(25.9427321045609,-15.0732007181261,
62.9272852161212));
#112160=CARTESIAN_POINT('Ctrl Pts',(25.9783589090034,-15.0271305776088,
62.856503476091));
#112161=CARTESIAN_POINT('Ctrl Pts',(26.0138189917453,-14.9809571170856,
62.7866843092614));
#112162=CARTESIAN_POINT('Ctrl Pts',(26.0315490331163,-14.957870386824,62.7517747258466));
#112163=CARTESIAN_POINT('Ctrl Pts',(26.0492373984288,-14.9347578310493,
62.7171057849726));
#112164=CARTESIAN_POINT('Ctrl Pts',(26.0668821056934,-14.9116218032023,
62.6826760758216));
#112165=CARTESIAN_POINT('Ctrl Pts',(26.0757044593257,-14.9000537892788,
62.6654612212461));
#112166=CARTESIAN_POINT('Ctrl Pts',(26.0845158987059,-14.8884799076072,
62.6483061745562));
#112167=CARTESIAN_POINT('Ctrl Pts',(26.0933161800254,-14.8769004515561,
62.6312107583831));
#112168=CARTESIAN_POINT('Ctrl Pts',(26.099916391015,-14.8682158595178,62.6183891962533));
#112169=CARTESIAN_POINT('Ctrl Pts',(26.1065103256176,-14.8595281319135,
62.6056011762853));
#112170=CARTESIAN_POINT('Ctrl Pts',(26.1130978824016,-14.8508373918367,
62.5928466232461));
#112171=CARTESIAN_POINT('Ctrl Pts',(26.1152937346629,-14.8479404784777,
62.5885951055664));
#112172=CARTESIAN_POINT('Ctrl Pts',(26.1183068164103,-14.8439632058128,
62.5827653942718));
#112173=CARTESIAN_POINT('Ctrl Pts',(26.1196833095973,-14.8421456520831,
62.580103223031));
#112174=CARTESIAN_POINT('Ctrl Pts',(26.1495148755876,-14.8027553561176,
62.5224082501823));
#112175=CARTESIAN_POINT('Ctrl Pts',(26.182170738001,-14.7594242261849,62.4597989844644));
#112176=CARTESIAN_POINT('Ctrl Pts',(26.2176473167757,-14.7119972228234,
62.3925134181239));
#112177=CARTESIAN_POINT('Ctrl Pts',(26.2526277367343,-14.6652335113195,
62.3261688762026));
#112178=CARTESIAN_POINT('Ctrl Pts',(26.2903508399422,-14.6144875115488,
62.2552778627649));
#112179=CARTESIAN_POINT('Ctrl Pts',(26.3308008173732,-14.5595899140302,
62.1801130968392));
#112180=CARTESIAN_POINT('Ctrl Pts',(26.3415601610262,-14.544987628567,62.1601199201168));
#112181=CARTESIAN_POINT('Ctrl Pts',(26.3525123514416,-14.5300915053854,
62.1398246195584));
#112182=CARTESIAN_POINT('Ctrl Pts',(26.3636568951483,-14.5148981324929,
62.1192328782769));
#112183=CARTESIAN_POINT('Ctrl Pts',(26.4046448515626,-14.4590191909865,
62.0434995493625));
#112184=CARTESIAN_POINT('Ctrl Pts',(26.4482349442434,-14.3991219719376,
61.9637532974569));
#112185=CARTESIAN_POINT('Ctrl Pts',(26.4944163670492,-14.3350007186598,
61.8802978336112));
#112186=CARTESIAN_POINT('Ctrl Pts',(26.5412166875894,-14.2700201480208,
61.7957239460714));
#112187=CARTESIAN_POINT('Ctrl Pts',(26.5906783534958,-14.2007018204385,
61.7073405613577));
#112188=CARTESIAN_POINT('Ctrl Pts',(26.6427848634371,-14.126797388866,61.6155069626122));
#112189=CARTESIAN_POINT('Ctrl Pts',(26.6948913733785,-14.0528929572935,
61.5236733638667));
#112190=CARTESIAN_POINT('Ctrl Pts',(26.7496428216296,-13.9744026194313,
61.4283894311402));
#112191=CARTESIAN_POINT('Ctrl Pts',(26.8070160790248,-13.8910407683245,
61.3300596385221));
#112192=CARTESIAN_POINT('Ctrl Pts',(26.8286817045993,-13.8595611777403,
61.2929277661759));
#112193=CARTESIAN_POINT('Ctrl Pts',(26.8507211285977,-13.8273865079625,
61.2553620201456));
#112194=CARTESIAN_POINT('Ctrl Pts',(26.8731328192345,-13.7944999020021,
61.2173859214206));
#112195=CARTESIAN_POINT('Ctrl Pts',(26.8843386645529,-13.7780565990218,
61.1983978720581));
#112196=CARTESIAN_POINT('Ctrl Pts',(26.895637567286,-13.7614353038493,61.1793072361356));
#112197=CARTESIAN_POINT('Ctrl Pts',(26.9070293274744,-13.7446338246987,
61.1601170608852));
#112198=CARTESIAN_POINT('Ctrl Pts',(26.9127252075685,-13.7362330851234,
61.1505219732599));
#112199=CARTESIAN_POINT('Ctrl Pts',(26.9184443014333,-13.7277872990275,
61.1409020009062));
#112200=CARTESIAN_POINT('Ctrl Pts',(26.9241865818617,-13.7192961882546,
61.1312575281269));
#112201=CARTESIAN_POINT('Ctrl Pts',(26.927057722076,-13.7150506328682,61.1264352917372));
#112202=CARTESIAN_POINT('Ctrl Pts',(26.9299346588935,-13.7107937462796,
61.1216069302478));
#112203=CARTESIAN_POINT('Ctrl Pts',(26.9328173888506,-13.7065254933995,
61.1167724920681));
#112204=CARTESIAN_POINT('Ctrl Pts',(26.9342587538292,-13.7043913669594,
61.1143552729782));
#112205=CARTESIAN_POINT('Ctrl Pts',(26.9357015670903,-13.7022543989444,
61.1119365347162));
#112206=CARTESIAN_POINT('Ctrl Pts',(26.9371458281976,-13.7001145849478,
61.1095162833576));
#112207=CARTESIAN_POINT('Ctrl Pts',(26.9385900893049,-13.6979747709512,
61.107096031999));
#112208=CARTESIAN_POINT('Ctrl Pts',(26.9393230538677,-13.6968888043132,
61.1058677620329));
#112209=CARTESIAN_POINT('Ctrl Pts',(26.9414829546153,-13.6936866005958,
61.1022509960756));
#112210=CARTESIAN_POINT('Ctrl Pts',(27.0187193827629,-13.5791782012597,
60.9729181624769));
#112211=CARTESIAN_POINT('Ctrl Pts',(27.0923797168953,-13.4679359954866,
60.8520372952937));
#112212=CARTESIAN_POINT('Ctrl Pts',(27.1624720225538,-13.3603870981355,
60.7389430187677));
#112213=CARTESIAN_POINT('Ctrl Pts',(27.2311829274812,-13.2549578075519,
60.6280776390487));
#112214=CARTESIAN_POINT('Ctrl Pts',(27.296465288087,-13.1530780797369,60.5246948441136));
#112215=CARTESIAN_POINT('Ctrl Pts',(27.3583354933923,-13.0551344576139,
60.4282135322513));
#112216=CARTESIAN_POINT('Ctrl Pts',(27.4185576656764,-12.9597997539951,
60.3343021874207));
#112217=CARTESIAN_POINT('Ctrl Pts',(27.4755472245224,-12.8681945215141,
60.246929548252));
#112218=CARTESIAN_POINT('Ctrl Pts',(27.5293246809172,-12.7806553500093,
60.1656041894029));
#112219=CARTESIAN_POINT('Ctrl Pts',(27.5656780519623,-12.7214791785048,
60.11062853336));
#112220=CARTESIAN_POINT('Ctrl Pts',(27.600563690595,-12.6641606650941,60.0584172229083));
#112221=CARTESIAN_POINT('Ctrl Pts',(27.6339887949749,-12.6087975633783,
60.0088304806025));
#112222=CARTESIAN_POINT('Ctrl Pts',(27.6818519320055,-12.529520272461,59.9378246577062));
#112223=CARTESIAN_POINT('Ctrl Pts',(27.7267202670337,-12.4542537088115,
59.8721985660002));
#112224=CARTESIAN_POINT('Ctrl Pts',(27.7686161579487,-12.3832641878405,
59.8115780830282));
#112225=CARTESIAN_POINT('Ctrl Pts',(27.8100628946962,-12.3130357257345,
59.7516074953553));
#112226=CARTESIAN_POINT('Ctrl Pts',(27.848600669005,-12.2469932419356,59.6965357243602));
#112227=CARTESIAN_POINT('Ctrl Pts',(27.8842512191725,-12.1853682390402,
59.6460434001692));
#112228=CARTESIAN_POINT('Ctrl Pts',(27.91939608697,-12.1246173510566,59.5962672803017));
#112229=CARTESIAN_POINT('Ctrl Pts',(27.9517351264143,-12.0681596070252,
59.5509416213708));
#112230=CARTESIAN_POINT('Ctrl Pts',(27.9812880817654,-12.0161893006359,
59.5098025229151));
#112231=CARTESIAN_POINT('Ctrl Pts',(28.0088908883515,-11.9676484255036,
59.4713781229079));
#112232=CARTESIAN_POINT('Ctrl Pts',(28.0340632047671,-11.9230221225772,
59.4366063232373));
#112233=CARTESIAN_POINT('Ctrl Pts',(28.0568195157664,-11.8824455220351,
59.4053060009392));
#112234=CARTESIAN_POINT('',(38.6333985430991,-1.20459248512199,98.36583228337));
#112235=CARTESIAN_POINT('Ctrl Pts',(38.6333985430991,-1.20459248512199,
98.36583228337));
#112236=CARTESIAN_POINT('Ctrl Pts',(38.5366002152195,-2.46830688119351,
98.2349959150518));
#112237=CARTESIAN_POINT('Ctrl Pts',(38.0688555603353,-4.89683171878626,
97.6805363924601));
#112238=CARTESIAN_POINT('Ctrl Pts',(37.1095611647792,-7.15936829257837,
96.5833073808643));
#112239=CARTESIAN_POINT('Ctrl Pts',(36.2609354234713,-8.73058637062551,
95.6084465035992));
#112240=CARTESIAN_POINT('Ctrl Pts',(35.6521334167721,-9.73616974679085,
94.9078930628315));
#112241=CARTESIAN_POINT('Ctrl Pts',(34.9681261465269,-10.6688054360461,
94.1123973243883));
#112242=CARTESIAN_POINT('Ctrl Pts',(33.8978354227833,-12.0086232552646,
92.8564947258115));
#112243=CARTESIAN_POINT('Ctrl Pts',(33.1279964816629,-12.8209446465096,
91.9377075741904));
#112244=CARTESIAN_POINT('Ctrl Pts',(31.5241780468789,-14.2851195759495,
89.9695310692828));
#112245=CARTESIAN_POINT('Ctrl Pts',(30.6848812388159,-14.9412747048976,
88.91639447817));
#112246=CARTESIAN_POINT('Ctrl Pts',(29.4134476720632,-15.813447849705,87.2192561730067));
#112247=CARTESIAN_POINT('Ctrl Pts',(28.5629570853225,-16.3564140531643,
86.0495465015485));
#112248=CARTESIAN_POINT('Ctrl Pts',(27.308980739206,-17.0508777267664,84.1836367945689));
#112249=CARTESIAN_POINT('Ctrl Pts',(26.0883942100227,-17.6290940152154,
82.178465418237));
#112250=CARTESIAN_POINT('Ctrl Pts',(24.5910880959154,-18.2270657215307,
79.2772309226755));
#112251=CARTESIAN_POINT('Ctrl Pts',(23.7402842168438,-18.4469370871498,
76.8455281617186));
#112252=CARTESIAN_POINT('Ctrl Pts',(23.3999522626291,-18.46444455277,75.101511144727));
#112253=CARTESIAN_POINT('',(38.6794466444702,5.17649275224089E-11,98.4280216145082));
#112254=CARTESIAN_POINT('Origin',(31.1126367795517,0.000775488753213954,
88.2087611921047));
#112255=CARTESIAN_POINT('',(41.1972044619337,1.16390964369926E-14,112.706776537994));
#112256=CARTESIAN_POINT('',(38.4704302935856,1.16390964369926E-14,97.2424717708351));
#112257=CARTESIAN_POINT('Origin',(20.5162416486691,1.4210854715202E-14,
116.353388269));
#112258=CARTESIAN_POINT('',(38.6333954984551,1.20463046397926,98.3658274732794));
#112259=CARTESIAN_POINT('Origin',(31.1126367795517,0.000775488753213954,
88.2087611921047));
#112260=CARTESIAN_POINT('',(23.3999522626816,18.4644445525526,75.101511144713));
#112261=CARTESIAN_POINT('Ctrl Pts',(23.3999522612866,18.4644445499379,75.101511144959));
#112262=CARTESIAN_POINT('Ctrl Pts',(23.45961890053,18.461375785637,75.4072770176154));
#112263=CARTESIAN_POINT('Ctrl Pts',(23.5261343935816,18.4542914438561,75.7091799541492));
#112264=CARTESIAN_POINT('Ctrl Pts',(23.5991425426504,18.4433532934531,76.0075409544095));
#112265=CARTESIAN_POINT('Ctrl Pts',(23.676959267289,18.4316947176801,76.3255530680745));
#112266=CARTESIAN_POINT('Ctrl Pts',(23.7621520465881,18.4156577543503,76.6395413160084));
#112267=CARTESIAN_POINT('Ctrl Pts',(23.8542600959466,18.3953847954478,76.949899589864));
#112268=CARTESIAN_POINT('Ctrl Pts',(23.9198098214053,18.3809573170726,77.1707695332269));
#112269=CARTESIAN_POINT('Ctrl Pts',(23.9888612270989,18.3643832927569,77.3898011465229));
#112270=CARTESIAN_POINT('Ctrl Pts',(24.0612402519916,18.3457004295971,77.6071378070134));
#112271=CARTESIAN_POINT('Ctrl Pts',(24.1957690600846,18.3109751301561,78.0110951956914));
#112272=CARTESIAN_POINT('Ctrl Pts',(24.3417937836676,18.2689668465408,78.4091970786755));
#112273=CARTESIAN_POINT('Ctrl Pts',(24.4971961404488,18.2202185729628,78.8006560385329));
#112274=CARTESIAN_POINT('Ctrl Pts',(24.6531129926202,18.1713089069675,79.1934110136793));
#112275=CARTESIAN_POINT('Ctrl Pts',(24.818467695171,18.1156103124022,79.5794793560188));
#112276=CARTESIAN_POINT('Ctrl Pts',(24.9910976581544,18.0536592348641,79.9580698919787));
#112277=CARTESIAN_POINT('Ctrl Pts',(25.1634427984296,17.9918103705998,80.3360357902462));
#112278=CARTESIAN_POINT('Ctrl Pts',(25.3430368339901,17.9237286179672,80.7065489563957));
#112279=CARTESIAN_POINT('Ctrl Pts',(25.528086338763,17.8498440729799,81.0694906196872));
#112280=CARTESIAN_POINT('Ctrl Pts',(25.6880971184625,17.7859567166441,81.3833232808445));
#112281=CARTESIAN_POINT('Ctrl Pts',(25.8521862832049,17.7177302616557,81.6914949014036));
#112282=CARTESIAN_POINT('Ctrl Pts',(26.0192052724661,17.6454844942854,81.993926765999));
#112283=CARTESIAN_POINT('Ctrl Pts',(26.0453406526073,17.6341793690289,82.0412517545107));
#112284=CARTESIAN_POINT('Ctrl Pts',(26.0715478076392,17.6227759234653,82.0884361907658));
#112285=CARTESIAN_POINT('Ctrl Pts',(26.0978223780965,17.6112754976626,82.1354797658442));
#112286=CARTESIAN_POINT('Ctrl Pts',(26.302079891663,17.5218716239349,82.501194733113));
#112287=CARTESIAN_POINT('Ctrl Pts',(26.5104101217341,17.4266045074234,82.8583970920815));
#112288=CARTESIAN_POINT('Ctrl Pts',(26.7220462389472,17.3255160396653,83.2087303809841));
#112289=CARTESIAN_POINT('Ctrl Pts',(26.9128055892252,17.2343994066253,83.524505171468));
#112290=CARTESIAN_POINT('Ctrl Pts',(27.1062503495027,17.1385532496861,83.8346993201741));
#112291=CARTESIAN_POINT('Ctrl Pts',(27.3018210400026,17.0380447426029,84.1405160230136));
#112292=CARTESIAN_POINT('Ctrl Pts',(27.5080933913095,16.9320363932463,84.4630670668454));
#112293=CARTESIAN_POINT('Ctrl Pts',(27.7167216246146,16.8208468487113,84.7807500887177));
#112294=CARTESIAN_POINT('Ctrl Pts',(27.926810630039,16.7045966516856,85.0934841667746));
#112295=CARTESIAN_POINT('Ctrl Pts',(28.1227320257951,16.5961859292292,85.3851286388382));
#112296=CARTESIAN_POINT('Ctrl Pts',(28.3199235433799,16.4833742725223,85.6724691858054));
#112297=CARTESIAN_POINT('Ctrl Pts',(28.5176729072871,16.3663061368233,85.9554377650852));
#112298=CARTESIAN_POINT('Ctrl Pts',(28.711664099302,16.2514628486201,86.2330286048869));
#112299=CARTESIAN_POINT('Ctrl Pts',(28.9061918146068,16.1325232534556,86.5064121306224));
#112300=CARTESIAN_POINT('Ctrl Pts',(29.1006016876849,16.0096699843988,86.775520920119));
#112301=CARTESIAN_POINT('Ctrl Pts',(29.2910029919315,15.8893498469027,87.0390809116622));
#112302=CARTESIAN_POINT('Ctrl Pts',(29.481290996414,15.7652757942784,87.2985406796168));
#112303=CARTESIAN_POINT('Ctrl Pts',(29.6708727721434,15.6376644893672,87.5538330451626));
#112304=CARTESIAN_POINT('Ctrl Pts',(29.7251711571417,15.6011151547197,87.6269516932932));
#112305=CARTESIAN_POINT('Ctrl Pts',(29.7794117619617,15.5642759399319,87.699728456207));
#112306=CARTESIAN_POINT('Ctrl Pts',(29.8335810411833,15.5271526278358,87.7721616876146));
#112307=CARTESIAN_POINT('Ctrl Pts',(30.0748187458443,15.3618275076167,88.0947361567057));
#112308=CARTESIAN_POINT('Ctrl Pts',(30.3146457647922,15.19086977782,88.4104967426328));
#112309=CARTESIAN_POINT('Ctrl Pts',(30.5529445467657,15.0139252472042,88.719987132609));
#112310=CARTESIAN_POINT('Ctrl Pts',(30.7879734861698,14.8394086801468,89.0252308166492));
#112311=CARTESIAN_POINT('Ctrl Pts',(31.0215160082487,14.6590682647923,89.3243751689556));
#112312=CARTESIAN_POINT('Ctrl Pts',(31.2534107667758,14.4725553129748,89.61795036547));
#112313=CARTESIAN_POINT('Ctrl Pts',(31.4804877752156,14.2899172775012,89.9054263644965));
#112314=CARTESIAN_POINT('Ctrl Pts',(31.7059848681178,14.1013602822068,90.187562192574));
#112315=CARTESIAN_POINT('Ctrl Pts',(31.9297018364177,13.9065516870498,90.4648642524105));
#112316=CARTESIAN_POINT('Ctrl Pts',(32.056649470055,13.796008037387,90.6222186121021));
#112317=CARTESIAN_POINT('Ctrl Pts',(32.183023011221,13.6834513153511,90.7780166729506));
#112318=CARTESIAN_POINT('Ctrl Pts',(32.3087784870946,13.5688204265169,90.9323522662342));
#112319=CARTESIAN_POINT('Ctrl Pts',(32.5174358981477,13.3786212775358,91.1884307002285));
#112320=CARTESIAN_POINT('Ctrl Pts',(32.724388686809,13.1827084851237,91.4404834298436));
#112321=CARTESIAN_POINT('Ctrl Pts',(32.9289295915244,12.9812207204148,91.6880188239592));
#112322=CARTESIAN_POINT('Ctrl Pts',(33.1315961155715,12.7815793578794,91.9332858426707));
#112323=CARTESIAN_POINT('Ctrl Pts',(33.3318944302162,12.5764647539265,92.1741179965264));
#112324=CARTESIAN_POINT('Ctrl Pts',(33.529153850941,12.3660592360816,92.4100339942283));
#112325=CARTESIAN_POINT('Ctrl Pts',(33.7240072615387,12.1582200737743,92.6430724802884));
#112326=CARTESIAN_POINT('Ctrl Pts',(33.9158951642116,11.9452183770992,92.8713140571761));
#112327=CARTESIAN_POINT('Ctrl Pts',(34.1041926695823,11.7272754394601,93.0942910306846));
#112328=CARTESIAN_POINT('Ctrl Pts',(34.2734101142786,11.5314165143814,93.2946738961344));
#112329=CARTESIAN_POINT('Ctrl Pts',(34.4397280338224,11.3315676163555,93.4908050009544));
#112330=CARTESIAN_POINT('Ctrl Pts',(34.6027109913217,11.127920264297,93.6823417145347));
#112331=CARTESIAN_POINT('Ctrl Pts',(34.7990850568156,10.8825506927515,93.9131194824327));
#112332=CARTESIAN_POINT('Ctrl Pts',(34.9906219329704,10.6316734309369,94.1372267151763));
#112333=CARTESIAN_POINT('Ctrl Pts',(35.1769653584792,10.3750945491389,94.3544033086576));
#112334=CARTESIAN_POINT('Ctrl Pts',(35.3608788294736,10.1218615058667,94.5687478771169));
#112335=CARTESIAN_POINT('Ctrl Pts',(35.5397334897653,9.8630742641629,94.7763413681739));
#112336=CARTESIAN_POINT('Ctrl Pts',(35.7131380216892,9.59855363349448,94.9769423280029));
#112337=CARTESIAN_POINT('Ctrl Pts',(35.8829721861427,9.33947943403824,95.1734129509049));
#112338=CARTESIAN_POINT('Ctrl Pts',(36.047578338922,9.07490522105732,95.3631760292744));
#112339=CARTESIAN_POINT('Ctrl Pts',(36.2065413023706,8.80467404873674,95.5460131008675));
#112340=CARTESIAN_POINT('Ctrl Pts',(36.3181117639983,8.61500838078534,95.6743399515864));
#112341=CARTESIAN_POINT('Ctrl Pts',(36.4269013338651,8.42255624048273,95.7992551285144));
#112342=CARTESIAN_POINT('Ctrl Pts',(36.5327520178202,8.22726805508603,95.9206856461797));
#112343=CARTESIAN_POINT('Ctrl Pts',(36.6634217362688,7.9861902344369,96.0705882350107));
#112344=CARTESIAN_POINT('Ctrl Pts',(36.7896095664863,7.74078502350917,96.2151810512529));
#112345=CARTESIAN_POINT('Ctrl Pts',(36.9107931256386,7.49140320525122,96.354049383852));
#112346=CARTESIAN_POINT('Ctrl Pts',(37.0308658560298,7.24430734474327,96.491644780263));
#112347=CARTESIAN_POINT('Ctrl Pts',(37.1460254141818,6.99330765368619,96.6236201984513));
#112348=CARTESIAN_POINT('Ctrl Pts',(37.2558003327317,6.73878044478437,96.7495657595519));
#112349=CARTESIAN_POINT('Ctrl Pts',(37.3650785385787,6.48540492790448,96.874941438562));
#112350=CARTESIAN_POINT('Ctrl Pts',(37.4690205017941,6.22853395672561,96.9943417443013));
#112351=CARTESIAN_POINT('Ctrl Pts',(37.5672010075701,5.96857059401915,97.1073553044701));
#112352=CARTESIAN_POINT('Ctrl Pts',(37.6648629078788,5.70998040025437,97.2197719085555));
#112353=CARTESIAN_POINT('Ctrl Pts',(37.7568238718426,5.44833064182346,97.3258690929956));
#112354=CARTESIAN_POINT('Ctrl Pts',(37.8427079581854,5.18404618060724,97.4252344635266));
#112355=CARTESIAN_POINT('Ctrl Pts',(37.8758234340989,5.08214248596012,97.4635480985035));
#112356=CARTESIAN_POINT('Ctrl Pts',(37.9080358982251,4.97984735659777,97.5008608021213));
#112357=CARTESIAN_POINT('Ctrl Pts',(37.9393255877055,4.87718615189641,97.5371486179259));
#112358=CARTESIAN_POINT('Ctrl Pts',(38.0405433699397,4.54509147042374,97.6545346418482));
#112359=CARTESIAN_POINT('Ctrl Pts',(38.1321140636492,4.2091457966541,97.7611943001836));
#112360=CARTESIAN_POINT('Ctrl Pts',(38.2136417514429,3.86940501031531,97.8567832599188));
#112361=CARTESIAN_POINT('Ctrl Pts',(38.294046705557,3.53434286056575,97.9510558454578));
#112362=CARTESIAN_POINT('Ctrl Pts',(38.3646832865444,3.19558900540544,98.0345605588972));
#112363=CARTESIAN_POINT('Ctrl Pts',(38.4251283250865,2.85322082336216,98.1069747477039));
#112364=CARTESIAN_POINT('Ctrl Pts',(38.484275895867,2.5182016593606,98.1778345479666));
#112365=CARTESIAN_POINT('Ctrl Pts',(38.5336646070965,2.17972133100617,98.2380748616099));
#112366=CARTESIAN_POINT('Ctrl Pts',(38.5728578338096,1.83788060811413,98.2874004459044));
#112367=CARTESIAN_POINT('Ctrl Pts',(38.5969153115092,1.62805288384956,98.3176773392277));
#112368=CARTESIAN_POINT('Ctrl Pts',(38.6171306416519,1.41695963082921,98.3438420099546));
#112369=CARTESIAN_POINT('Ctrl Pts',(38.6333954797472,1.20463046288776,98.365827476578));
#112370=CARTESIAN_POINT('',(28.0568193311413,11.8824453975844,59.4053060263899));
#112371=CARTESIAN_POINT('Ctrl Pts',(28.0568193741291,11.88244542754,59.40530601881));
#112372=CARTESIAN_POINT('Ctrl Pts',(27.7243204687509,12.4753479870479,59.8627458820805));
#112373=CARTESIAN_POINT('Ctrl Pts',(27.3871488482182,13.0249815959646,60.3740379473461));
#112374=CARTESIAN_POINT('Ctrl Pts',(26.7070209696829,14.050902424375,61.4995241253409));
#112375=CARTESIAN_POINT('Ctrl Pts',(26.3632478725192,14.528011115418,62.1138216849645));
#112376=CARTESIAN_POINT('Ctrl Pts',(25.9349524358028,15.083850920924,62.9426971932013));
#112377=CARTESIAN_POINT('Ctrl Pts',(25.8387793290717,15.2065182721143,63.132611768099));
#112378=CARTESIAN_POINT('Ctrl Pts',(25.7430785079378,15.3263951382971,63.326297480956));
#112379=CARTESIAN_POINT('Ctrl Pts',(25.7218241106203,15.3529652490661,63.3694316382038));
#112380=CARTESIAN_POINT('Ctrl Pts',(25.7127984000554,15.3642261876238,63.3878072603337));
#112381=CARTESIAN_POINT('Ctrl Pts',(25.6840150790617,15.4000878249556,63.4465935348418));
#112382=CARTESIAN_POINT('Ctrl Pts',(25.6265681449639,15.4714305157428,63.5646879742171));
#112383=CARTESIAN_POINT('Ctrl Pts',(25.5695017601332,15.5416253702554,63.6843333208089));
#112384=CARTESIAN_POINT('Ctrl Pts',(25.3802203896199,15.7730314350455,64.0865319974358));
#112385=CARTESIAN_POINT('Ctrl Pts',(25.2318102003903,15.9499041554838,64.4191291739736));
#112386=CARTESIAN_POINT('Ctrl Pts',(25.0153167124731,16.2025590137327,64.9319759177368));
#112387=CARTESIAN_POINT('Ctrl Pts',(24.9085991289255,16.3257238429192,65.1918868774778));
#112388=CARTESIAN_POINT('Ctrl Pts',(24.7914467284545,16.4588957048741,65.4896866658859));
#112389=CARTESIAN_POINT('Ctrl Pts',(24.7442899524852,16.5121400547645,65.6119756838965));
#112390=CARTESIAN_POINT('Ctrl Pts',(24.7293361171015,16.528993566515,65.6509679401623));
#112391=CARTESIAN_POINT('Ctrl Pts',(24.726687619279,16.5319774138165,65.6578821834526));
#112392=CARTESIAN_POINT('Ctrl Pts',(24.724218261392,16.5347587713352,65.6643313770844));
#112393=CARTESIAN_POINT('Ctrl Pts',(24.7130624479885,16.5473202637082,65.6934702352849));
#112394=CARTESIAN_POINT('Ctrl Pts',(24.7015138760334,16.5602890191069,65.7236674345157));
#112395=CARTESIAN_POINT('Ctrl Pts',(24.606377727762,16.6668599454623,65.972849716348));
#112396=CARTESIAN_POINT('Ctrl Pts',(24.5020068601432,16.7818280567286,66.2480874865797));
#112397=CARTESIAN_POINT('Ctrl Pts',(24.2621677955456,17.0412413761153,66.9193266199932));
#112398=CARTESIAN_POINT('Ctrl Pts',(24.1265333019407,17.1856918201085,67.3151772540794));
#112399=CARTESIAN_POINT('Ctrl Pts',(23.9662642473337,17.3560993520012,67.8417223220284));
#112400=CARTESIAN_POINT('Ctrl Pts',(23.9461197147708,17.3775202437756,67.9088199119513));
#112401=CARTESIAN_POINT('Ctrl Pts',(23.9258821889579,17.3990529752298,67.97739921814));
#112402=CARTESIAN_POINT('Ctrl Pts',(23.922507629734,17.4026437778802,67.9888566520998));
#112403=CARTESIAN_POINT('Ctrl Pts',(23.9224051106616,17.4027528840716,67.9892061353641));
#112404=CARTESIAN_POINT('Ctrl Pts',(23.9219433244521,17.4032442896881,67.9907754120686));
#112405=CARTESIAN_POINT('Ctrl Pts',(23.9207864672607,17.4044753791621,67.994707681693));
#112406=CARTESIAN_POINT('Ctrl Pts',(23.9177475773,17.4077096634628,68.0050496368859));
#112407=CARTESIAN_POINT('Ctrl Pts',(23.9072108398732,17.4189272136881,68.0410135841617));
#112408=CARTESIAN_POINT('Ctrl Pts',(23.8968763662478,17.4299398638417,68.0766263973682));
#112409=CARTESIAN_POINT('Ctrl Pts',(23.8706760779252,17.4578852510944,68.1677733316712));
#112410=CARTESIAN_POINT('Ctrl Pts',(23.851342654348,17.4785377378293,68.2361021100229));
#112411=CARTESIAN_POINT('Ctrl Pts',(23.7882754916749,17.5460872093337,68.4645044517986));
#112412=CARTESIAN_POINT('Ctrl Pts',(23.7394076875455,17.5986140173638,68.6479150520402));
#112413=CARTESIAN_POINT('Ctrl Pts',(23.6590361667568,17.6860971594474,68.9739302125424));
#112414=CARTESIAN_POINT('Ctrl Pts',(23.6310851470077,17.7166965723575,69.0911012373308));
#112415=CARTESIAN_POINT('Ctrl Pts',(23.5880604984235,17.76430278348,69.2802207229952));
#112416=CARTESIAN_POINT('Ctrl Pts',(23.5662763612532,17.7885312912849,69.3781224134856));
#112417=CARTESIAN_POINT('Ctrl Pts',(23.5442320193917,17.8133002545793,69.4811630348402));
#112418=CARTESIAN_POINT('Ctrl Pts',(23.5331803275671,17.8257659416173,69.5335508954396));
#112419=CARTESIAN_POINT('Ctrl Pts',(23.5281273300357,17.8314746765208,69.557653479824));
#112420=CARTESIAN_POINT('Ctrl Pts',(23.5189906281387,17.841816471269,69.6015838168922));
#112421=CARTESIAN_POINT('Ctrl Pts',(23.5144489689002,17.8469662730383,69.6235792677627));
#112422=CARTESIAN_POINT('Ctrl Pts',(23.4377049240434,17.9341505450947,69.9980191665425));
#112423=CARTESIAN_POINT('Ctrl Pts',(23.3722679640801,18.0108631114948,70.3586080252768));
#112424=CARTESIAN_POINT('Ctrl Pts',(23.2896219181467,18.1156770894603,70.9095876822499));
#112425=CARTESIAN_POINT('Ctrl Pts',(23.2646831375625,18.1488918983225,71.0948845703221));
#112426=CARTESIAN_POINT('Ctrl Pts',(23.2318893863806,18.1958368605783,71.3749305704336));
#112427=CARTESIAN_POINT('Ctrl Pts',(23.2166390354395,18.2185942366947,71.5154862756931));
#112428=CARTESIAN_POINT('Ctrl Pts',(23.2009542680947,18.2438603952527,71.6803782636731));
#112429=CARTESIAN_POINT('Ctrl Pts',(23.1946945650232,18.2544101672144,71.7512390465093));
#112430=CARTESIAN_POINT('Ctrl Pts',(23.1916426671543,18.2596383402766,71.7867013803973));
#112431=CARTESIAN_POINT('Ctrl Pts',(23.1912659007525,18.2602959595756,71.791207649484));
#112432=CARTESIAN_POINT('Ctrl Pts',(23.1900739387607,18.262401303487,71.8057153804048));
#112433=CARTESIAN_POINT('Ctrl Pts',(23.1894717408811,18.2634825402461,71.8132266082456));
#112434=CARTESIAN_POINT('Ctrl Pts',(23.1791487916456,18.2823374133391,71.9452992336258));
#112435=CARTESIAN_POINT('Ctrl Pts',(23.1676231854454,18.3074993310288,72.1355250601407));
#112436=CARTESIAN_POINT('Ctrl Pts',(23.15971483603,18.3494862191041,72.5228176091576));
#112437=CARTESIAN_POINT('Ctrl Pts',(23.158735305727,18.3641388360826,72.6689234206449));
#112438=CARTESIAN_POINT('Ctrl Pts',(23.1623186709509,18.3856996206964,72.913972835298));
#112439=CARTESIAN_POINT('Ctrl Pts',(23.1643636747112,18.3928126370994,72.9999703254755));
#112440=CARTESIAN_POINT('Ctrl Pts',(23.1691109587509,18.4031551990834,73.135474511414));
#112441=CARTESIAN_POINT('Ctrl Pts',(23.1719054695799,18.4082442930824,73.2048534438938));
#112442=CARTESIAN_POINT('Ctrl Pts',(23.1754157853588,18.413165394377,73.2766778839518));
#112443=CARTESIAN_POINT('Ctrl Pts',(23.1772977650755,18.4155939929091,73.3129980290335));
#112444=CARTESIAN_POINT('Ctrl Pts',(23.1781587151562,18.4166627047207,73.3291724630669));
#112445=CARTESIAN_POINT('Ctrl Pts',(23.1797820783799,18.4185769114322,73.3586179279733));
#112446=CARTESIAN_POINT('Ctrl Pts',(23.2072483677226,18.4495082153164,73.8416758352283));
#112447=CARTESIAN_POINT('Ctrl Pts',(23.2554887086179,18.4600321078001,74.2313583768614));
#112448=CARTESIAN_POINT('Ctrl Pts',(23.3412924764406,18.4677758676054,74.8038516240253));
#112449=CARTESIAN_POINT('Ctrl Pts',(23.379899241412,18.4654735461107,74.998722729572));
#112450=CARTESIAN_POINT('Ctrl Pts',(23.3999522633791,18.46444455386,75.10151114459));
#112451=CARTESIAN_POINT('',(28.7709983219891,10.49234437565,58.41163725334));
#112452=CARTESIAN_POINT('Ctrl Pts',(28.0568192451658,11.8824453376732,59.4053060415497));
#112453=CARTESIAN_POINT('Ctrl Pts',(28.2006128658113,11.6261391970008,59.207884342463));
#112454=CARTESIAN_POINT('Ctrl Pts',(28.3373915772597,11.3697415610487,59.0185211727151));
#112455=CARTESIAN_POINT('Ctrl Pts',(28.4674976733393,11.1138285219291,58.8371561766688));
#112456=CARTESIAN_POINT('Ctrl Pts',(28.5730192009864,10.9062722609512,58.6900615206828));
#112457=CARTESIAN_POINT('Ctrl Pts',(28.6741521197716,10.6990338477355,58.5482278784034));
#112458=CARTESIAN_POINT('Ctrl Pts',(28.7710895317811,10.4923978628195,58.4116212007229));
#112459=CARTESIAN_POINT('',(13.2726083411502,20.6713283131467,53.9604380084771));
#112460=CARTESIAN_POINT('Ctrl Pts',(13.2725470758821,20.670980255801,53.9604489574278));
#112461=CARTESIAN_POINT('Ctrl Pts',(13.3983326199236,20.6495706071341,53.9827646797933));
#112462=CARTESIAN_POINT('Ctrl Pts',(13.531387176427,20.6258486398982,54.0065477088826));
#112463=CARTESIAN_POINT('Ctrl Pts',(13.6715832064528,20.5994311438589,54.0319088395874));
#112464=CARTESIAN_POINT('Ctrl Pts',(13.7714197113082,20.5806186962375,54.0499690275135));
#112465=CARTESIAN_POINT('Ctrl Pts',(13.8748772205112,20.5604384421668,54.0688297144999));
#112466=CARTESIAN_POINT('Ctrl Pts',(13.9818997410914,20.5387396048791,54.0885338755379));
#112467=CARTESIAN_POINT('Ctrl Pts',(14.0974696012661,20.5153077927924,54.1098117068175));
#112468=CARTESIAN_POINT('Ctrl Pts',(14.2171963593889,20.4901051805436,54.1320732233102));
#112469=CARTESIAN_POINT('Ctrl Pts',(14.3410132816261,20.4629320551245,54.1553717026691));
#112470=CARTESIAN_POINT('Ctrl Pts',(14.5137202363644,20.4250294190627,54.1878697598603));
#112471=CARTESIAN_POINT('Ctrl Pts',(14.6943870318908,20.3832944228992,54.2223854561454));
#112472=CARTESIAN_POINT('Ctrl Pts',(14.8828092918702,20.3371466051706,54.2590671495918));
#112473=CARTESIAN_POINT('Ctrl Pts',(14.9123065986212,20.3299222128107,54.2648096301451));
#112474=CARTESIAN_POINT('Ctrl Pts',(14.9419939140507,20.3225895875837,54.2706051992886));
#112475=CARTESIAN_POINT('Ctrl Pts',(14.9718703872864,20.3151464087435,54.2764544309475));
#112476=CARTESIAN_POINT('Ctrl Pts',(15.0822307696412,20.2876521306787,54.2980608447053));
#112477=CARTESIAN_POINT('Ctrl Pts',(15.1951724544689,20.2586497117875,54.3203994742456));
#112478=CARTESIAN_POINT('Ctrl Pts',(15.3106502727804,20.2280193281412,54.3434992717584));
#112479=CARTESIAN_POINT('Ctrl Pts',(15.3683891819361,20.212704136318,54.3550491705148));
#112480=CARTESIAN_POINT('Ctrl Pts',(15.4267621027678,20.1969818742966,54.3667893638777));
#112481=CARTESIAN_POINT('Ctrl Pts',(15.4857629994355,20.1808371688332,54.378723458483));
#112482=CARTESIAN_POINT('Ctrl Pts',(15.5152634477693,20.1727648161015,54.3846905057856));
#112483=CARTESIAN_POINT('Ctrl Pts',(15.5449208887949,20.1645868477245,54.3907060285509));
#112484=CARTESIAN_POINT('Ctrl Pts',(15.5747345513607,20.1563013159571,54.3967704764909));
#112485=CARTESIAN_POINT('Ctrl Pts',(15.5896413826436,20.1521585500734,54.3998027004609));
#112486=CARTESIAN_POINT('Ctrl Pts',(15.604587269227,20.1479888930469,54.4028471557349));
#112487=CARTESIAN_POINT('Ctrl Pts',(15.6195721132309,20.1437920999199,54.4059038984308));
#112488=CARTESIAN_POINT('Ctrl Pts',(15.6345569572348,20.1395953067928,54.4089606411267));
#112489=CARTESIAN_POINT('Ctrl Pts',(15.6481522477201,20.1357745629695,54.4117374402641));
#112490=CARTESIAN_POINT('Ctrl Pts',(15.6646434189796,20.1311200661957,54.415111044885));
#112491=CARTESIAN_POINT('Ctrl Pts',(15.8328267221155,20.0836517190703,54.449516361505));
#112492=CARTESIAN_POINT('Ctrl Pts',(15.9934146374075,20.0362881729058,54.4830079349232));
#112493=CARTESIAN_POINT('Ctrl Pts',(16.1465409572366,19.9894925441059,54.5154517122097));
#112494=CARTESIAN_POINT('Ctrl Pts',(16.3017481192989,19.9420610068557,54.5483363698234));
#112495=CARTESIAN_POINT('Ctrl Pts',(16.4492896509013,19.895212890308,54.5801446504592));
#112496=CARTESIAN_POINT('Ctrl Pts',(16.5892991581977,19.8493805976035,54.6107561641212));
#112497=CARTESIAN_POINT('Ctrl Pts',(16.6705959948486,19.8227679733233,54.6285308086712));
#112498=CARTESIAN_POINT('Ctrl Pts',(16.7493532392507,19.7964969186979,54.6459023039302));
#112499=CARTESIAN_POINT('Ctrl Pts',(16.825595914603,19.7706446140519,54.6628498087903));
#112500=CARTESIAN_POINT('Ctrl Pts',(16.9590472852794,19.7253940313014,54.6925138747832));
#112501=CARTESIAN_POINT('Ctrl Pts',(17.0847944325676,19.6814291917678,54.7208780337367));
#112502=CARTESIAN_POINT('Ctrl Pts',(17.2029519193958,19.6391261391975,54.7478438524984));
#112503=CARTESIAN_POINT('Ctrl Pts',(17.3226347922806,19.5962769639204,54.775157793796));
#112504=CARTESIAN_POINT('Ctrl Pts',(17.4345310839538,19.5551327185357,54.8010371418669));
#112505=CARTESIAN_POINT('Ctrl Pts',(17.5387575365312,19.5160331038114,54.8253961014855));
#112506=CARTESIAN_POINT('Ctrl Pts',(17.6201968381364,19.4854818834884,54.8444294333327));
#112507=CARTESIAN_POINT('Ctrl Pts',(17.6969534080328,19.4561779490565,54.8625348551515));
#112508=CARTESIAN_POINT('Ctrl Pts',(17.7690802329903,19.4282623570324,54.8796778113961));
#112509=CARTESIAN_POINT('Ctrl Pts',(17.8037775298157,19.4148332953333,54.8879245939438));
#112510=CARTESIAN_POINT('Ctrl Pts',(17.8374033749867,19.4017252527957,54.8959487237115));
#112511=CARTESIAN_POINT('Ctrl Pts',(17.8699633866476,19.3889524563322,54.9037467823189));
#112512=CARTESIAN_POINT('Ctrl Pts',(17.886243392478,19.3825660581005,54.9076458116227));
#112513=CARTESIAN_POINT('Ctrl Pts',(17.9022569342675,19.376263457397,54.9114883238176));
#112514=CARTESIAN_POINT('Ctrl Pts',(17.9180046971456,19.3700463431641,54.9152739206525));
#112515=CARTESIAN_POINT('Ctrl Pts',(17.9258785785847,19.3669377860476,54.91716671907));
#112516=CARTESIAN_POINT('Ctrl Pts',(17.9336860149447,19.3638505996751,54.9190452886899));
#112517=CARTESIAN_POINT('Ctrl Pts',(17.9414270900674,19.3607849898339,54.9209095806218));
#112518=CARTESIAN_POINT('Ctrl Pts',(17.9482005307998,19.3581025812228,54.9225408360622));
#112519=CARTESIAN_POINT('Ctrl Pts',(17.9549231636888,19.3554366920914,54.9241611601502));
#112520=CARTESIAN_POINT('Ctrl Pts',(17.9615950443003,19.3527874580197,54.9257705207019));
#112521=CARTESIAN_POINT('Ctrl Pts',(17.9620716072011,19.3525982270146,54.925885475027));
#112522=CARTESIAN_POINT('Ctrl Pts',(17.962257232792,19.3525245107963,54.9259302457957));
#112523=CARTESIAN_POINT('Ctrl Pts',(17.9625879435656,19.3523931767217,54.9260100238398));
#112524=CARTESIAN_POINT('Ctrl Pts',(17.9629186543391,19.3522618426471,54.926089801884));
#112525=CARTESIAN_POINT('Ctrl Pts',(17.9633944550144,19.3520729022509,54.9262045866393));
#112526=CARTESIAN_POINT('Ctrl Pts',(17.964451314587,19.3516530920658,54.9264595753351));
#112527=CARTESIAN_POINT('Ctrl Pts',(18.1681663588649,19.2707325491052,54.9756099400571));
#112528=CARTESIAN_POINT('Ctrl Pts',(18.3646898914307,19.189396868016,55.0239377208772));
#112529=CARTESIAN_POINT('Ctrl Pts',(18.5541472030898,19.1081622375069,55.0713015000461));
#112530=CARTESIAN_POINT('Ctrl Pts',(18.7485133668291,19.0248228120894,55.119892478017));
#112531=CARTESIAN_POINT('Ctrl Pts',(18.9354426488189,18.9415897734647,55.1674689038007));
#112532=CARTESIAN_POINT('Ctrl Pts',(19.1150897843592,18.8589725928745,55.213898600522));
#112533=CARTESIAN_POINT('Ctrl Pts',(19.260647254864,18.792032767807,55.2515178433266));
#112534=CARTESIAN_POINT('Ctrl Pts',(19.4014245088014,18.7254962996004,55.2883846896468));
#112535=CARTESIAN_POINT('Ctrl Pts',(19.5375110188955,18.6596119982858,55.324437893159));
#112536=CARTESIAN_POINT('Ctrl Pts',(19.7134947248391,18.5744120508345,55.3710610034204));
#112537=CARTESIAN_POINT('Ctrl Pts',(19.8816351338832,18.4903038972743,55.4163223459423));
#112538=CARTESIAN_POINT('Ctrl Pts',(20.0421640303715,18.407768078151,55.4600957917956));
#112539=CARTESIAN_POINT('Ctrl Pts',(20.2047686202212,18.3241650427472,55.5044352432276));
#112540=CARTESIAN_POINT('Ctrl Pts',(20.3595638260116,18.2421752263657,55.5472482728489));
#112541=CARTESIAN_POINT('Ctrl Pts',(20.5067845132278,18.1622509049083,55.5884287453757));
#112542=CARTESIAN_POINT('Ctrl Pts',(20.6564303125084,18.0810100195911,55.6302875686333));
#112543=CARTESIAN_POINT('Ctrl Pts',(20.7982502424243,18.0019032324527,55.670459795706));
#112544=CARTESIAN_POINT('Ctrl Pts',(20.9324810363312,17.9253574474708,55.7088566072134));
#112545=CARTESIAN_POINT('Ctrl Pts',(21.0676708251577,17.8482647908153,55.7475277398812));
#112546=CARTESIAN_POINT('Ctrl Pts',(21.1951628772056,17.7737697907286,55.78439821155));
#112547=CARTESIAN_POINT('Ctrl Pts',(21.315185457343,17.7022608641087,55.8193969583901));
#112548=CARTESIAN_POINT('Ctrl Pts',(21.4362280291454,17.6301442309302,55.8546931361805));
#112549=CARTESIAN_POINT('Ctrl Pts',(21.5496738518478,17.5610645912574,55.8880858373269));
#112550=CARTESIAN_POINT('Ctrl Pts',(21.6557399270599,17.4953728891182,55.9195190062841));
#112551=CARTESIAN_POINT('Ctrl Pts',(21.7435139199357,17.4410103327208,55.9455312325553));
#112552=CARTESIAN_POINT('Ctrl Pts',(21.8262338218732,17.3889670330136,55.9702018787292));
#112553=CARTESIAN_POINT('Ctrl Pts',(21.9040123380698,17.3394180031356,55.9935063851894));
#112554=CARTESIAN_POINT('Ctrl Pts',(21.9595325848506,17.3040486685032,56.0101417237513));
#112555=CARTESIAN_POINT('Ctrl Pts',(22.0125347737628,17.2699498293013,56.0260810869046));
#112556=CARTESIAN_POINT('Ctrl Pts',(22.0630567118334,17.2371785721442,56.0413172514788));
#112557=CARTESIAN_POINT('Ctrl Pts',(22.0883176808687,17.2207929435656,56.0489353337659));
#112558=CARTESIAN_POINT('Ctrl Pts',(22.1129585339961,17.2047391316149,56.0563776226435));
#112559=CARTESIAN_POINT('Ctrl Pts',(22.1369837451694,17.1890237610659,56.0636433486403));
#112560=CARTESIAN_POINT('Ctrl Pts',(22.1489963507561,17.1811660757914,56.0672762116387));
#112561=CARTESIAN_POINT('Ctrl Pts',(22.160855042549,17.1733929959198,56.0708649343019));
#112562=CARTESIAN_POINT('Ctrl Pts',(22.1725603608703,17.1657053193998,56.0744094244494));
#112563=CARTESIAN_POINT('Ctrl Pts',(22.178413020031,17.1618614811399,56.0761816695231));
#112564=CARTESIAN_POINT('Ctrl Pts',(22.1842273356144,17.1580389934109,56.0779428564926));
#112565=CARTESIAN_POINT('Ctrl Pts',(22.1900033741081,17.1542379539996,56.0796929742694));
#112566=CARTESIAN_POINT('Ctrl Pts',(22.1943354029784,17.1513871744411,56.081005562602));
#112567=CARTESIAN_POINT('Ctrl Pts',(22.1986459009686,17.148548459536,56.0823119245156));
#112568=CARTESIAN_POINT('Ctrl Pts',(22.2029348958593,17.1457218500621,56.0836120554263));
#112569=CARTESIAN_POINT('Ctrl Pts',(22.2036497283411,17.1452507484831,56.0838287439115));
#112570=CARTESIAN_POINT('Ctrl Pts',(22.2039246071545,17.1450695659692,56.0839120788244));
#112571=CARTESIAN_POINT('Ctrl Pts',(22.2044185879296,17.1447439591707,56.0840618283974));
#112572=CARTESIAN_POINT('Ctrl Pts',(22.2049125687048,17.1444183523722,56.0842115779703));
#112573=CARTESIAN_POINT('Ctrl Pts',(22.2056256717387,17.1439483509576,56.0844277397999));
#112574=CARTESIAN_POINT('Ctrl Pts',(22.2072167240695,17.1428992772211,56.0849101091727));
#112575=CARTESIAN_POINT('Ctrl Pts',(22.4232631234304,17.0004472666548,56.1504102590644));
#112576=CARTESIAN_POINT('Ctrl Pts',(22.6313077906992,16.8580575607652,56.2145538222262));
#112577=CARTESIAN_POINT('Ctrl Pts',(22.8316436620993,16.7163048221399,56.2772017465106));
#112578=CARTESIAN_POINT('Ctrl Pts',(23.0350088497684,16.5724086137791,56.3407969818029));
#112579=CARTESIAN_POINT('Ctrl Pts',(23.2304305725263,16.4291687516019,56.4028511969841));
#112580=CARTESIAN_POINT('Ctrl Pts',(23.4182208717324,16.2871422952561,56.4632510848778));
#112581=CARTESIAN_POINT('Ctrl Pts',(23.6104241266593,16.1417783051521,56.5250703327275));
#112582=CARTESIAN_POINT('Ctrl Pts',(23.7946333175536,15.9976854511902,56.5851567549806));
#112583=CARTESIAN_POINT('Ctrl Pts',(23.9711852633733,15.8554150786589,56.6434195964039));
#112584=CARTESIAN_POINT('Ctrl Pts',(24.1202371250588,15.7353050238531,56.6926073011381));
#112585=CARTESIAN_POINT('Ctrl Pts',(24.2638314927311,15.6164930851575,56.7404958867728));
#112586=CARTESIAN_POINT('Ctrl Pts',(24.4021703284857,15.4992863804217,56.7870457428963));
#112587=CARTESIAN_POINT('Ctrl Pts',(24.5657007214818,15.3607362879427,56.8420723464113));
#112588=CARTESIAN_POINT('Ctrl Pts',(24.721886796623,15.2244306559942,56.8952276754609));
#112589=CARTESIAN_POINT('Ctrl Pts',(24.8710398764416,15.0908494029051,56.9464618033456));
#112590=CARTESIAN_POINT('Ctrl Pts',(25.0237389492806,14.9540923642962,56.9989139809019));
#112591=CARTESIAN_POINT('Ctrl Pts',(25.1690669787661,14.8201907764638,57.04935272528));
#112592=CARTESIAN_POINT('Ctrl Pts',(25.3073581524276,14.6896102615281,57.0977484391436));
#112593=CARTESIAN_POINT('Ctrl Pts',(25.3814685192842,14.6196320437577,57.1236837466094));
#112594=CARTESIAN_POINT('Ctrl Pts',(25.4535579439844,14.5506067710419,57.149032702733));
#112595=CARTESIAN_POINT('Ctrl Pts',(25.5236773638562,14.4826005075336,57.1737931672091));
#112596=CARTESIAN_POINT('Ctrl Pts',(25.5817728389014,14.4262558288157,57.1943077543051));
#112597=CARTESIAN_POINT('Ctrl Pts',(25.638516003415,14.370610575918,57.2144184047141));
#112598=CARTESIAN_POINT('Ctrl Pts',(25.6939355208178,14.3157003634769,57.2341246640445));
#112599=CARTESIAN_POINT('Ctrl Pts',(25.7216452795192,14.2882452572563,57.2439777937097));
#112600=CARTESIAN_POINT('Ctrl Pts',(25.7490241095723,14.2609738950902,57.2537298281413));
#112601=CARTESIAN_POINT('Ctrl Pts',(25.7760755746848,14.2338905536095,57.2633807782122));
#112602=CARTESIAN_POINT('Ctrl Pts',(25.7896013072411,14.2203488828692,57.2682062532476));
#112603=CARTESIAN_POINT('Ctrl Pts',(25.8030451974999,14.2068542162773,57.2730064573516));
#112604=CARTESIAN_POINT('Ctrl Pts',(25.816407686443,14.193407080461,57.2777813938924));
#112605=CARTESIAN_POINT('Ctrl Pts',(25.8230889309145,14.1866835125528,57.2801688621628));
#112606=CARTESIAN_POINT('Ctrl Pts',(25.8297498249901,14.1799718272756,57.2825500135525));
#112607=CARTESIAN_POINT('Ctrl Pts',(25.8363904236561,14.1732720898237,57.2849248487048));
#112608=CARTESIAN_POINT('Ctrl Pts',(25.8413708726557,14.1682472867348,57.2867059750689));
#112609=CARTESIAN_POINT('Ctrl Pts',(25.8463399054818,14.1632292042925,57.2884835485503));
#112610=CARTESIAN_POINT('Ctrl Pts',(25.8512975452887,14.1582178698532,57.2902575694684));
#112611=CARTESIAN_POINT('Ctrl Pts',(25.852950091891,14.1565474250401,57.2908489097744));
#112612=CARTESIAN_POINT('Ctrl Pts',(25.8560371622284,14.1534254693535,57.2919537333789));
#112613=CARTESIAN_POINT('Ctrl Pts',(25.8562513882808,14.1532087857527,57.292030406214));
#112614=CARTESIAN_POINT('Ctrl Pts',(25.8620994629914,14.1472936233727,57.2941234684845));
#112615=CARTESIAN_POINT('Ctrl Pts',(25.8735776967432,14.1356810419393,57.2982181067595));
#112616=CARTESIAN_POINT('Ctrl Pts',(25.8906482847789,14.1183340826607,57.304310381592));
#112617=CARTESIAN_POINT('Ctrl Pts',(25.9076983413253,14.1010079872743,57.3103953289983));
#112618=CARTESIAN_POINT('Ctrl Pts',(25.9303273488426,14.0779612618749,57.3184731525455));
#112619=CARTESIAN_POINT('Ctrl Pts',(25.9584601922357,14.0491212848265,57.3285356587346));
#112620=CARTESIAN_POINT('Ctrl Pts',(25.9864949993255,14.0203818082751,57.3385630994702));
#112621=CARTESIAN_POINT('Ctrl Pts',(26.0199954067525,13.9858893157332,57.3505614815991));
#112622=CARTESIAN_POINT('Ctrl Pts',(26.058849163281,13.9455372029293,57.3645176427207));
#112623=CARTESIAN_POINT('Ctrl Pts',(26.0975892260193,13.905303168403,57.3784329653495));
#112624=CARTESIAN_POINT('Ctrl Pts',(26.1416514425737,13.8592436714862,57.3942947188479));
#112625=CARTESIAN_POINT('Ctrl Pts',(26.1908856865504,13.8072195986701,57.4120836267462));
#112626=CARTESIAN_POINT('Ctrl Pts',(26.2397975092592,13.7555362169292,57.4297560400713));
#112627=CARTESIAN_POINT('Ctrl Pts',(26.2938139308273,13.697966004636,57.4493305605161));
#112628=CARTESIAN_POINT('Ctrl Pts',(26.3527480492319,13.6343410642143,57.4707806166182));
#112629=CARTESIAN_POINT('Ctrl Pts',(26.3956365561786,13.5880388750389,57.4863906046022));
#112630=CARTESIAN_POINT('Ctrl Pts',(26.4411286678883,13.5385294399888,57.5029937293787));
#112631=CARTESIAN_POINT('Ctrl Pts',(26.4891385100757,13.485738019396,57.5205766097949));
#112632=CARTESIAN_POINT('Ctrl Pts',(26.554119601433,13.4142850845785,57.5443749541882));
#112633=CARTESIAN_POINT('Ctrl Pts',(26.6237145012724,13.3368210896554,57.5699686138886));
#112634=CARTESIAN_POINT('Ctrl Pts',(26.697678079691,13.2531302347554,57.5973159560468));
#112635=CARTESIAN_POINT('Ctrl Pts',(26.7707907027383,13.1704022481214,57.6243486654059));
#112636=CARTESIAN_POINT('Ctrl Pts',(26.848172101239,13.0815898112931,57.6530950629175));
#112637=CARTESIAN_POINT('Ctrl Pts',(26.9295465905642,12.9864541213655,57.683503211984));
#112638=CARTESIAN_POINT('Ctrl Pts',(26.9791042032982,12.9285158446683,57.7020219798177));
#112639=CARTESIAN_POINT('Ctrl Pts',(27.0301420512111,12.8682317541113,57.7211568382924));
#112640=CARTESIAN_POINT('Ctrl Pts',(27.0825905397635,12.8055423906308,57.7408935664254));
#112641=CARTESIAN_POINT('Ctrl Pts',(27.1351740721451,12.7426916152215,57.7606811124831));
#112642=CARTESIAN_POINT('Ctrl Pts',(27.1891755326363,12.6774231685811,57.7810736474008));
#112643=CARTESIAN_POINT('Ctrl Pts',(27.2445189896879,12.6096728855716,57.8020546543642));
#112644=CARTESIAN_POINT('Ctrl Pts',(27.2721907182137,12.5757977440668,57.812545157846));
#112645=CARTESIAN_POINT('Ctrl Pts',(27.3001978611984,12.5413020791577,57.8231827941772));
#112646=CARTESIAN_POINT('Ctrl Pts',(27.3285303604243,12.5061774672578,57.8339652179499));
#112647=CARTESIAN_POINT('Ctrl Pts',(27.3426966100372,12.4886151613078,57.8393564298362));
#112648=CARTESIAN_POINT('Ctrl Pts',(27.3569441933603,12.4708956144904,57.8447838395127));
#112649=CARTESIAN_POINT('Ctrl Pts',(27.3712718188045,12.453017749092,57.850247147685));
#112650=CARTESIAN_POINT('Ctrl Pts',(27.3784356315265,12.4440788163928,57.8529788017711));
#112651=CARTESIAN_POINT('Ctrl Pts',(27.3856194544388,12.4351003037946,57.8557194305414));
#112652=CARTESIAN_POINT('Ctrl Pts',(27.3928231238543,12.4260820750035,57.8584689956263));
#112653=CARTESIAN_POINT('Ctrl Pts',(27.3964249585621,12.421572960608,57.8598437781688));
#112654=CARTESIAN_POINT('Ctrl Pts',(27.4000317548744,12.4170539171483,57.8612207947937));
#112655=CARTESIAN_POINT('Ctrl Pts',(27.4036434921889,12.4125249274888,57.862600040639));
#112656=CARTESIAN_POINT('Ctrl Pts',(27.4072552295035,12.4079959378294,57.8639792864843));
#112657=CARTESIAN_POINT('Ctrl Pts',(27.4121604782024,12.4018384965928,57.8658530839424));
#112658=CARTESIAN_POINT('Ctrl Pts',(27.4144935064473,12.3989081027107,57.8667444609622));
#112659=CARTESIAN_POINT('Ctrl Pts',(27.5443731982542,12.2357730634706,57.9163674232507));
#112660=CARTESIAN_POINT('Ctrl Pts',(27.6666333539921,12.0773904465288,57.9636925254359));
#112661=CARTESIAN_POINT('Ctrl Pts',(27.7817898329975,11.9242236513042,58.0087751429393));
#112662=CARTESIAN_POINT('Ctrl Pts',(27.8963722738334,11.7718203701043,58.0536330302021));
#112663=CARTESIAN_POINT('Ctrl Pts',(28.0039219461057,11.6245809497874,58.0962710866615));
#112664=CARTESIAN_POINT('Ctrl Pts',(28.1049157238554,11.4829233739343,58.136757159939));
#112665=CARTESIAN_POINT('Ctrl Pts',(28.1713804642806,11.3896974919233,58.1634013395229));
#112666=CARTESIAN_POINT('Ctrl Pts',(28.2350051607492,11.2988883550859,58.1891137418305));
#112667=CARTESIAN_POINT('Ctrl Pts',(28.2959175074842,11.2106061487287,58.2139158100153));
#112668=CARTESIAN_POINT('Ctrl Pts',(28.3897816383863,11.0745658708867,58.2521350660368));
#112669=CARTESIAN_POINT('Ctrl Pts',(28.4772065834014,10.9445274666595,58.2881919157419));
#112670=CARTESIAN_POINT('Ctrl Pts',(28.5586195289291,10.8208529693944,58.3221601998858));
#112671=CARTESIAN_POINT('Ctrl Pts',(28.6344289501963,10.7056907921461,58.3537905007636));
#112672=CARTESIAN_POINT('Ctrl Pts',(28.7050253514017,10.5960464103352,58.3836102317404));
#112673=CARTESIAN_POINT('Ctrl Pts',(28.7707246265959,10.4921843560221,58.4116855396036));
#112674=CARTESIAN_POINT('',(20.1852098213545,19.2602427307108,66.2798693554263));
#112675=CARTESIAN_POINT('Ctrl Pts',(13.2726083411502,20.6713283131467,53.9604380084771));
#112676=CARTESIAN_POINT('Ctrl Pts',(13.6650705206071,20.6171872598987,54.4446995373014));
#112677=CARTESIAN_POINT('Ctrl Pts',(14.0456121743071,20.5589064465633,54.9370237517833));
#112678=CARTESIAN_POINT('Ctrl Pts',(14.4143958822179,20.4977644961702,55.4374033981323));
#112679=CARTESIAN_POINT('Ctrl Pts',(14.792876198402,20.4350149109242,55.9509397683671));
#112680=CARTESIAN_POINT('Ctrl Pts',(15.1589715900071,20.3692518224625,56.4729607208082));
#112681=CARTESIAN_POINT('Ctrl Pts',(15.5128201222323,20.301816719549,57.0034475857769));
#112682=CARTESIAN_POINT('Ctrl Pts',(15.8776473842055,20.2322893322172,57.550393673817));
#112683=CARTESIAN_POINT('Ctrl Pts',(16.2294557289051,20.1609845788745,58.1063392937893));
#112684=CARTESIAN_POINT('Ctrl Pts',(16.5683635307345,20.0893294000026,58.6712517682346));
#112685=CARTESIAN_POINT('Ctrl Pts',(16.7879003420604,20.0429127952516,59.0371892965194));
#112686=CARTESIAN_POINT('Ctrl Pts',(17.0020232495274,19.9963482605702,59.4068892038341));
#112687=CARTESIAN_POINT('Ctrl Pts',(17.2107580475794,19.9500144834406,59.7803395394369));
#112688=CARTESIAN_POINT('Ctrl Pts',(17.4689577772204,19.8927007588496,60.2422882733654));
#112689=CARTESIAN_POINT('Ctrl Pts',(17.7189332343118,19.8357394220478,60.7100397541429));
#112690=CARTESIAN_POINT('Ctrl Pts',(17.9609010912795,19.7797605046363,61.183494134282));
#112691=CARTESIAN_POINT('Ctrl Pts',(18.2082387691999,19.7225392868326,61.667455551523));
#112692=CARTESIAN_POINT('Ctrl Pts',(18.4472096766317,19.6663442139162,62.1573756648184));
#112693=CARTESIAN_POINT('Ctrl Pts',(18.6780286743746,19.6118176263714,62.6531899405673));
#112694=CARTESIAN_POINT('Ctrl Pts',(18.9120250296077,19.5565404486974,63.155829387633));
#112695=CARTESIAN_POINT('Ctrl Pts',(19.1376435950153,19.5029775403519,63.6645263330383));
#112696=CARTESIAN_POINT('Ctrl Pts',(19.3550892404964,19.4517734533484,64.1792577383865));
#112697=CARTESIAN_POINT('Ctrl Pts',(19.5780377759832,19.3992735461504,64.7070154349712));
#112698=CARTESIAN_POINT('Ctrl Pts',(19.7923945453953,19.3492528297393,65.2411168166477));
#112699=CARTESIAN_POINT('Ctrl Pts',(19.9983593229911,19.3023878519598,65.7815843256316));
#112700=CARTESIAN_POINT('Ctrl Pts',(20.0614280643745,19.2880372663985,65.9470815817552));
#112701=CARTESIAN_POINT('Ctrl Pts',(20.1237097797265,19.2739824855875,66.1131760904936));
#112702=CARTESIAN_POINT('Ctrl Pts',(20.1852098210872,19.2602427300862,66.2798693554734));
#112703=CARTESIAN_POINT('',(20.800313080212,19.9701890918763,80.5583314861626));
#112704=CARTESIAN_POINT('Ctrl Pts',(20.1852098218891,19.26024273196,66.279869355332));
#112705=CARTESIAN_POINT('Ctrl Pts',(20.3956147376191,19.2132888033458,66.85086198908));
#112706=CARTESIAN_POINT('Ctrl Pts',(20.583906319848,19.1756806736357,67.4339514479084));
#112707=CARTESIAN_POINT('Ctrl Pts',(20.8337679129635,19.1346807742746,68.3266260967489));
#112708=CARTESIAN_POINT('Ctrl Pts',(20.9116227172105,19.1235746354422,68.6271916025033));
#112709=CARTESIAN_POINT('Ctrl Pts',(21.0203010142702,19.1108571350284,69.0825429169022));
#112710=CARTESIAN_POINT('Ctrl Pts',(21.0551762471562,19.1072744149749,69.2350772354996));
#112711=CARTESIAN_POINT('Ctrl Pts',(21.1222298094364,19.1014326610879,69.5416461155132));
#112712=CARTESIAN_POINT('Ctrl Pts',(21.1548280750446,19.099151918798,69.6977888999547));
#112713=CARTESIAN_POINT('Ctrl Pts',(21.3068854151633,19.0912914655277,70.4611698530622));
#112714=CARTESIAN_POINT('Ctrl Pts',(21.4047375236733,19.0955470327253,71.0692966232455));
#112715=CARTESIAN_POINT('Ctrl Pts',(21.5157574614961,19.1175959029956,71.9776317061673));
#112716=CARTESIAN_POINT('Ctrl Pts',(21.5468008791318,19.1275486653768,72.2797681764848));
#112717=CARTESIAN_POINT('Ctrl Pts',(21.5843815989602,19.1462934155003,72.7320170222064));
#112718=CARTESIAN_POINT('Ctrl Pts',(21.5954108918719,19.1531771101233,72.8826073649739));
#112719=CARTESIAN_POINT('Ctrl Pts',(21.6144651576598,19.1681946363891,73.1834711088403));
#112720=CARTESIAN_POINT('Ctrl Pts',(21.622539704415,19.1763950000682,73.3348863784913));
#112721=CARTESIAN_POINT('Ctrl Pts',(21.6807506561845,19.2545151271669,74.6756524326983));
#112722=CARTESIAN_POINT('Ctrl Pts',(21.6393791641691,19.3636208894343,75.871367916597));
#112723=CARTESIAN_POINT('Ctrl Pts',(21.3604005439774,19.6406666743054,78.2839515090091));
#112724=CARTESIAN_POINT('Ctrl Pts',(21.128772128542,19.8020335869663,79.4438996858326));
#112725=CARTESIAN_POINT('Ctrl Pts',(20.8003130797391,19.9701890904,80.558331486246));
#112726=CARTESIAN_POINT('',(7.33390977237169,18.5189601985662,98.6155810279324));
#112727=CARTESIAN_POINT('Ctrl Pts',(7.33390977041688,18.5189602022785,98.615581028277));
#112728=CARTESIAN_POINT('Ctrl Pts',(7.40300811544448,18.5587169582139,98.5792660235925));
#112729=CARTESIAN_POINT('Ctrl Pts',(7.47743835222588,18.6010470589897,98.5393831952295));
#112730=CARTESIAN_POINT('Ctrl Pts',(7.5571859506456,18.645686168729,98.4956928813854));
#112731=CARTESIAN_POINT('Ctrl Pts',(7.63681402113335,18.6902583721215,98.4520680518063));
#112732=CARTESIAN_POINT('Ctrl Pts',(7.7217435913383,18.737132513752,98.4046472585255));
#112733=CARTESIAN_POINT('Ctrl Pts',(7.81195440394735,18.7860124926477,98.3531522464439));
#112734=CARTESIAN_POINT('Ctrl Pts',(7.89967363447421,18.8335424285046,98.303079503442));
#112735=CARTESIAN_POINT('Ctrl Pts',(7.99238644327563,18.8829686485955,98.249154440664));
#112736=CARTESIAN_POINT('Ctrl Pts',(8.0900680016121,18.9339911668916,98.191083469747));
#112737=CARTESIAN_POINT('Ctrl Pts',(8.19007101100508,18.9862262608367,98.1316324131815));
#112738=CARTESIAN_POINT('Ctrl Pts',(8.29528185234498,19.0401343561057,98.0678363631022));
#112739=CARTESIAN_POINT('Ctrl Pts',(8.40566612380089,19.0953664082598,97.9993377021124));
#112740=CARTESIAN_POINT('Ctrl Pts',(8.51545955489577,19.1503028265776,97.9312056855101));
#112741=CARTESIAN_POINT('Ctrl Pts',(8.63037125665938,19.2065488445754,97.8584213946183));
#112742=CARTESIAN_POINT('Ctrl Pts',(8.75035847762832,19.2637368556886,97.7805882331736));
#112743=CARTESIAN_POINT('Ctrl Pts',(8.78001842642022,19.2778733067826,97.7613484544362));
#112744=CARTESIAN_POINT('Ctrl Pts',(8.80998846475636,19.2920672107585,97.7417999486203));
#112745=CARTESIAN_POINT('Ctrl Pts',(8.84026785415954,19.3063128108983,97.7219362865122));
#112746=CARTESIAN_POINT('Ctrl Pts',(8.88625532412443,19.3279486206511,97.6917679250429));
#112747=CARTESIAN_POINT('Ctrl Pts',(8.93295637404587,19.3497036940079,97.6608726489343));
#112748=CARTESIAN_POINT('Ctrl Pts',(8.98036824142804,19.3715575334906,97.629227137476));
#112749=CARTESIAN_POINT('Ctrl Pts',(9.00407417511912,19.382484453232,97.6134043817468));
#112750=CARTESIAN_POINT('Ctrl Pts',(9.02795781521243,19.393436059536,97.5973940668182));
#112751=CARTESIAN_POINT('Ctrl Pts',(9.05201878813381,19.404409753059,97.5811931647464));
#112752=CARTESIAN_POINT('Ctrl Pts',(9.07122333245306,19.4131685336909,97.5682622270464));
#112753=CARTESIAN_POINT('Ctrl Pts',(9.09148271476123,19.4223679925869,97.5545719375748));
#112754=CARTESIAN_POINT('Ctrl Pts',(9.11054142550903,19.4309848244041,97.5416478040445));
#112755=CARTESIAN_POINT('Ctrl Pts',(9.1153609758434,19.4331638414014,97.5383795603054));
#112756=CARTESIAN_POINT('Ctrl Pts',(9.12010376098745,19.4353057867906,97.535160499116));
#112757=CARTESIAN_POINT('Ctrl Pts',(9.12473333698127,19.4373944771995,97.5320156598431));
#112758=CARTESIAN_POINT('Ctrl Pts',(9.2329304762039,19.486208953356,97.4585180840177));
#112759=CARTESIAN_POINT('Ctrl Pts',(9.33875382586786,19.5327559178126,97.3853580022948));
#112760=CARTESIAN_POINT('Ctrl Pts',(9.44221015358314,19.5772068491388,97.3126744947735));
#112761=CARTESIAN_POINT('Ctrl Pts',(9.59241066674853,19.6417418354786,97.2071507402632));
#112762=CARTESIAN_POINT('Ctrl Pts',(9.7376200143331,19.7018600336085,97.1026331426659));
#112763=CARTESIAN_POINT('Ctrl Pts',(9.87781587225694,19.7580219968163,96.9995654049525));
#112764=CARTESIAN_POINT('Ctrl Pts',(10.0204767735848,19.8151714476646,96.8946854421794));
#112765=CARTESIAN_POINT('Ctrl Pts',(10.1579466148379,19.8682243189159,96.7913069061254));
#112766=CARTESIAN_POINT('Ctrl Pts',(10.2902269366158,19.9176255912408,96.689870740715));
#112767=CARTESIAN_POINT('Ctrl Pts',(10.3939715015546,19.9563699292942,96.6103165734123));
#112768=CARTESIAN_POINT('Ctrl Pts',(10.4945245822998,19.9928673785176,96.5319566228767));
#112769=CARTESIAN_POINT('Ctrl Pts',(10.5918957033378,20.027315787863,96.4549917215766));
#112770=CARTESIAN_POINT('Ctrl Pts',(10.6631576246075,20.0525271627396,96.3986642737818));
#112771=CARTESIAN_POINT('Ctrl Pts',(10.73271539479,20.076640728936,96.3430838227071));
#112772=CARTESIAN_POINT('Ctrl Pts',(10.8005748819127,20.0997291910529,96.2883254403981));
#112773=CARTESIAN_POINT('Ctrl Pts',(10.8345046254741,20.1112734221114,96.2609462492436));
#112774=CARTESIAN_POINT('Ctrl Pts',(10.8680098181274,20.1225613096538,96.2337725716242));
#112775=CARTESIAN_POINT('Ctrl Pts',(10.9010913435032,20.1336015707345,96.2068134459687));
#112776=CARTESIAN_POINT('Ctrl Pts',(10.9176321061911,20.1391217012748,96.193333883141));
#112777=CARTESIAN_POINT('Ctrl Pts',(10.9340669532922,20.1445799211063,96.1799079580775));
#112778=CARTESIAN_POINT('Ctrl Pts',(10.9503960020745,20.1499772958843,96.1665367899462));
#112779=CARTESIAN_POINT('Ctrl Pts',(10.9585605264657,20.1526759832733,96.1598512058805));
#112780=CARTESIAN_POINT('Ctrl Pts',(10.9666986013493,20.1553594591464,96.1531793110346));
#112781=CARTESIAN_POINT('Ctrl Pts',(10.9748102418903,20.1580278552853,96.1465212440585));
#112782=CARTESIAN_POINT('Ctrl Pts',(10.9829218824312,20.1606962514242,96.1398631770824));
#112783=CARTESIAN_POINT('Ctrl Pts',(10.9926014686587,20.1638715521178,96.1319071805507));
#112784=CARTESIAN_POINT('Ctrl Pts',(10.9990658759471,20.165987935302,96.1265886649839));
#112785=CARTESIAN_POINT('Ctrl Pts',(11.0818740054802,20.1930985001283,96.0584592439361));
#112786=CARTESIAN_POINT('Ctrl Pts',(11.1696312337331,20.2211666649735,95.9854307495776));
#112787=CARTESIAN_POINT('Ctrl Pts',(11.2622619314072,20.2499219836152,95.9071881388308));
#112788=CARTESIAN_POINT('Ctrl Pts',(11.3435991454559,20.2751714696509,95.8384848240785));
#112789=CARTESIAN_POINT('Ctrl Pts',(11.428693788411,20.3009503157172,95.7657607532074));
#112790=CARTESIAN_POINT('Ctrl Pts',(11.5174819094351,20.3270576395467,95.6887777177979));
#112791=CARTESIAN_POINT('Ctrl Pts',(11.6214331785391,20.3576235464909,95.5986475952322));
#112792=CARTESIAN_POINT('Ctrl Pts',(11.7304491331547,20.3886400129683,95.5026781603857));
#112793=CARTESIAN_POINT('Ctrl Pts',(11.8443765358371,20.4197639254504,95.4005049410484));
#112794=CARTESIAN_POINT('Ctrl Pts',(11.9559928176839,20.4502564611001,95.3004043982621));
#112795=CARTESIAN_POINT('Ctrl Pts',(12.0723236790256,20.4808519046811,95.1943487770492));
#112796=CARTESIAN_POINT('Ctrl Pts',(12.1931818716125,20.5112046304692,95.0819849448582));
#112797=CARTESIAN_POINT('Ctrl Pts',(12.3094842731162,20.5404131998328,94.9738567059176));
#112798=CARTESIAN_POINT('Ctrl Pts',(12.4299793180954,20.5693967541912,94.8598864746458));
#112799=CARTESIAN_POINT('Ctrl Pts',(12.5544558512573,20.5978293238787,94.7397559166034));
#112800=CARTESIAN_POINT('Ctrl Pts',(12.6759694988279,20.6255851198089,94.6224847979304));
#112801=CARTESIAN_POINT('Ctrl Pts',(12.8012776177519,20.6528156642883,94.4993427834358));
#112802=CARTESIAN_POINT('Ctrl Pts',(12.930137215551,20.6792033322693,94.370035537127));
#112803=CARTESIAN_POINT('Ctrl Pts',(13.0543738883018,20.7046443248505,94.245367275559));
#112804=CARTESIAN_POINT('Ctrl Pts',(13.1819119164582,20.7293016507751,94.114967928198));
#112805=CARTESIAN_POINT('Ctrl Pts',(13.3124870307784,20.7528798152625,93.9785799115993));
#112806=CARTESIAN_POINT('Ctrl Pts',(13.3813266858498,20.7653103057045,93.9066756742));
#112807=CARTESIAN_POINT('Ctrl Pts',(13.4510096790417,20.7774406823677,93.8331070550628));
#112808=CARTESIAN_POINT('Ctrl Pts',(13.5214915861578,20.789226618785,93.7578374459239));
#112809=CARTESIAN_POINT('Ctrl Pts',(13.6749060720465,20.8148804844387,93.5940018055224));
#112810=CARTESIAN_POINT('Ctrl Pts',(13.8321074502674,20.8389019522866,93.4221100941343));
#112811=CARTESIAN_POINT('Ctrl Pts',(13.992732783026,20.8608671652904,93.24164273448));
#112812=CARTESIAN_POINT('Ctrl Pts',(14.065572171761,20.8708278150904,93.1598055053326));
#112813=CARTESIAN_POINT('Ctrl Pts',(14.1391150943112,20.8803656645332,93.0762043821394));
#112814=CARTESIAN_POINT('Ctrl Pts',(14.2133248047303,20.8894415798287,92.9907888952405));
#112815=CARTESIAN_POINT('Ctrl Pts',(14.3109575206791,20.9013821500724,92.8784134941921));
#112816=CARTESIAN_POINT('Ctrl Pts',(14.4097445882159,20.9125230950735,92.7628977570874));
#112817=CARTESIAN_POINT('Ctrl Pts',(14.5095972235387,20.9227764232584,92.6441234712457));
#112818=CARTESIAN_POINT('Ctrl Pts',(14.5595235412001,20.9279030873509,92.5847363283249));
#112819=CARTESIAN_POINT('Ctrl Pts',(14.6097162484685,20.9328078761558,92.5245345486646));
#112820=CARTESIAN_POINT('Ctrl Pts',(14.6601635801387,20.9374799404975,92.4635029456918));
#112821=CARTESIAN_POINT('Ctrl Pts',(14.6853872459738,20.9398159726684,92.4329871442054));
#112822=CARTESIAN_POINT('Ctrl Pts',(14.710674567712,20.9420938259984,92.4022638869283));
#112823=CARTESIAN_POINT('Ctrl Pts',(14.7360240539024,20.9443121571214,92.3713312646967));
#112824=CARTESIAN_POINT('Ctrl Pts',(14.7486987969976,20.9454213226829,92.3558649535809));
#112825=CARTESIAN_POINT('Ctrl Pts',(14.7613890811952,20.9465156078426,92.3403463012285));
#112826=CARTESIAN_POINT('Ctrl Pts',(14.774094717722,20.9475948454575,92.3247750676269));
#112827=CARTESIAN_POINT('Ctrl Pts',(14.7804475359853,20.9481344642649,92.3169894508261));
#112828=CARTESIAN_POINT('Ctrl Pts',(14.7868041923303,20.9486703211959,92.3091906887131));
#112829=CARTESIAN_POINT('Ctrl Pts',(14.7931646630046,20.9492023954075,92.3013787511973));
#112830=CARTESIAN_POINT('Ctrl Pts',(14.7995251336789,20.9497344696191,92.2935668136815));
#112831=CARTESIAN_POINT('Ctrl Pts',(14.8071091475034,20.9503632205178,92.2842403644937));
#112832=CARTESIAN_POINT('Ctrl Pts',(14.8122574942145,20.9507872490788,92.2779033823244));
#112833=CARTESIAN_POINT('Ctrl Pts',(15.0054140661669,20.9666960267569,92.0401513774521));
#112834=CARTESIAN_POINT('Ctrl Pts',(15.1956957611478,20.9785834093345,91.7979202834243));
#112835=CARTESIAN_POINT('Ctrl Pts',(15.3829840419243,20.9866600873303,91.5512433302939));
#112836=CARTESIAN_POINT('Ctrl Pts',(15.8633605515616,21.0073759931469,90.9185405618053));
#112837=CARTESIAN_POINT('Ctrl Pts',(16.3240405690058,21.0030203136065,90.256589250856));
#112838=CARTESIAN_POINT('Ctrl Pts',(16.7623705722965,20.9778487372575,89.5701434912169));
#112839=CARTESIAN_POINT('Ctrl Pts',(16.8643593595663,20.9719919204158,89.410424170097));
#112840=CARTESIAN_POINT('Ctrl Pts',(16.9651383553155,20.9650082821789,89.24937879876));
#112841=CARTESIAN_POINT('Ctrl Pts',(17.0646744743569,20.9569516053128,89.0870673107852));
#112842=CARTESIAN_POINT('Ctrl Pts',(17.5374317754215,20.9186855683457,88.3161517705195));
#112843=CARTESIAN_POINT('Ctrl Pts',(17.9821471685851,20.8562122789627,87.5166739726371));
#112844=CARTESIAN_POINT('Ctrl Pts',(18.3957624236964,20.7754934985282,86.6957101104845));
#112845=CARTESIAN_POINT('Ctrl Pts',(18.4435021572208,20.7661768859983,86.6009539439071));
#112846=CARTESIAN_POINT('Ctrl Pts',(18.4908276334093,20.7566172155477,86.5059115415749));
#112847=CARTESIAN_POINT('Ctrl Pts',(18.537734193146,20.7468236567509,86.4105937818987));
#112848=CARTESIAN_POINT('Ctrl Pts',(18.9662594531666,20.6573524323955,85.5397972882066));
#112849=CARTESIAN_POINT('Ctrl Pts',(19.3598171159288,20.5483617098516,84.6460200651757));
#112850=CARTESIAN_POINT('Ctrl Pts',(19.7197007721944,20.4254862467279,83.7274864709089));
#112851=CARTESIAN_POINT('Ctrl Pts',(20.121198686996,20.2884023826359,82.7027405110613));
#112852=CARTESIAN_POINT('Ctrl Pts',(20.4807861174765,20.1340385981811,81.6471815928633));
#112853=CARTESIAN_POINT('Ctrl Pts',(20.8003130801046,19.9701890915409,80.5583314861816));
#112854=CARTESIAN_POINT('Ctrl Pts',(7.33390977334909,18.51896019671,98.61558102776));
#112855=CARTESIAN_POINT('Ctrl Pts',(6.63322704598623,18.1147877634574,98.9948595799931));
#112856=CARTESIAN_POINT('Ctrl Pts',(5.89295788622676,17.6398039918909,99.2724209778057));
#112857=CARTESIAN_POINT('Ctrl Pts',(4.74849242406141,16.801502773932,99.531723109432));
#112858=CARTESIAN_POINT('Ctrl Pts',(4.36140549410044,16.5011208865675,99.5919699821525));
#112859=CARTESIAN_POINT('Ctrl Pts',(3.77627559787738,16.0169956123106,99.642372183263));
#112860=CARTESIAN_POINT('Ctrl Pts',(3.58048761657308,15.8500313075335,99.6525106426868));
#112861=CARTESIAN_POINT('Ctrl Pts',(3.28622330212731,15.5909646268607,99.657630641654));
#112862=CARTESIAN_POINT('Ctrl Pts',(3.13894605544017,15.4592765754447,99.6576686311094));
#112863=CARTESIAN_POINT('Ctrl Pts',(2.96699089507222,15.3018219412834,99.6532778873175));
#112864=CARTESIAN_POINT('Ctrl Pts',(2.88099605374559,15.2221343132077,99.649970986995));
#112865=CARTESIAN_POINT('Ctrl Pts',(2.83799628675308,15.1820497226923,99.6480393075469));
#112866=CARTESIAN_POINT('Ctrl Pts',(2.8195675244896,15.1648189435875,99.6471517869677));
#112867=CARTESIAN_POINT('Ctrl Pts',(2.80728164201297,15.1533202673855,99.6465468450906));
#112868=CARTESIAN_POINT('Ctrl Pts',(2.80006760744145,15.1465607400022,99.6461826927322));
#112869=CARTESIAN_POINT('Ctrl Pts',(2.47039426792358,14.8373955143149,99.6292382431169));
#112870=CARTESIAN_POINT('Ctrl Pts',(2.13940644347902,14.5110408544986,99.5933956312336));
#112871=CARTESIAN_POINT('Ctrl Pts',(1.63792852770526,13.9860880137101,99.5100852681188));
#112872=CARTESIAN_POINT('Ctrl Pts',(1.46994338013475,13.8052029378049,99.4773895309509));
#112873=CARTESIAN_POINT('Ctrl Pts',(1.21736259553632,13.524741470774,99.4208454099032));
#112874=CARTESIAN_POINT('Ctrl Pts',(1.09092209996242,13.3822276363525,99.3906981037323));
#112875=CARTESIAN_POINT('Ctrl Pts',(0.943291600146698,13.2119084215627,
99.3522188066159));
#112876=CARTESIAN_POINT('Ctrl Pts',(0.869465991839432,13.1257286835316,
99.3321489851273));
#112877=CARTESIAN_POINT('Ctrl Pts',(0.83255296139824,13.0823829352355,99.3219061144348));
#112878=CARTESIAN_POINT('Ctrl Pts',(0.81673329746239,13.0637512650341,99.3174717049452));
#112879=CARTESIAN_POINT('Ctrl Pts',(0.806186929066697,13.051317937016,99.314505514109));
#112880=CARTESIAN_POINT('Ctrl Pts',(0.799877375459519,13.0438709028361,
99.3127240133116));
#112881=CARTESIAN_POINT('Ctrl Pts',(0.524492575138919,12.718570563598,99.2347520082104));
#112882=CARTESIAN_POINT('Ctrl Pts',(0.241494197014471,12.3680862536953,
99.1412693519639));
#112883=CARTESIAN_POINT('Ctrl Pts',(-0.193563578726575,11.7932354542952,
98.9747078038906));
#112884=CARTESIAN_POINT('Ctrl Pts',(-0.340328439984648,11.5934330443894,
98.9147951491503));
#112885=CARTESIAN_POINT('Ctrl Pts',(-0.562058097063683,11.2810031769473,
98.8181552773681));
#112886=CARTESIAN_POINT('Ctrl Pts',(-0.673317085489583,11.1216071368294,
98.7681423666626));
#112887=CARTESIAN_POINT('Ctrl Pts',(-0.803567088169475,10.9299858870827,
98.7067886060777));
#112888=CARTESIAN_POINT('Ctrl Pts',(-0.86877265525937,10.8327494392575,
98.6753548485219));
#112889=CARTESIAN_POINT('Ctrl Pts',(-0.90488651237819,10.7785259673729,
98.6577437530991));
#112890=CARTESIAN_POINT('Ctrl Pts',(-0.922365710419661,10.7521687743111,
98.649158549259));
#112891=CARTESIAN_POINT('Ctrl Pts',(-0.931688985831928,10.738081682025,
98.6445638924));
#112892=CARTESIAN_POINT('Ctrl Pts',(-0.933921641068739,10.7347067958116,
98.6434628273561));
#112893=CARTESIAN_POINT('Ctrl Pts',(-0.959163860730728,10.6965448724609,
98.6310111690001));
#112894=CARTESIAN_POINT('Ctrl Pts',(-1.10562671612739,10.481109110981,98.5580089322338));
#112895=CARTESIAN_POINT('Ctrl Pts',(-1.47832025232363,9.87531424826814,
98.3524972497975));
#112896=CARTESIAN_POINT('Ctrl Pts',(-1.62755303669153,9.62598937210525,
98.2679041093474));
#112897=CARTESIAN_POINT('Ctrl Pts',(-1.88050856857826,9.17685763766061,
98.1154000785185));
#112898=CARTESIAN_POINT('Ctrl Pts',(-1.96964332888882,9.01461246026334,
98.0602902103554));
#112899=CARTESIAN_POINT('Ctrl Pts',(-2.10919509042164,8.75187222534487,
97.9709702151545));
#112900=CARTESIAN_POINT('Ctrl Pts',(-2.18042989056037,8.61565858151007,
97.9246458046577));
#112901=CARTESIAN_POINT('Ctrl Pts',(-2.26575206205299,8.44813945470475,
97.8676283019775));
#112902=CARTESIAN_POINT('Ctrl Pts',(-2.30892174604868,8.36221323615283,
97.838368504093));
#112903=CARTESIAN_POINT('Ctrl Pts',(-2.33217846248433,8.31559886746861,
97.8224913580097));
#112904=CARTESIAN_POINT('Ctrl Pts',(-2.34306616694847,8.29368664839123,
97.8150268158695));
#112905=CARTESIAN_POINT('Ctrl Pts',(-2.34929602204302,8.28112642642193,
97.8107478154731));
#112906=CARTESIAN_POINT('Ctrl Pts',(-2.35141537312412,8.27685034503791,
97.8092910057185));
#112907=CARTESIAN_POINT('Ctrl Pts',(-2.60781128656009,7.75931157392258,
97.6329689188456));
#112908=CARTESIAN_POINT('Ctrl Pts',(-2.81988247376081,7.27975194019941,
97.4744733855343));
#112909=CARTESIAN_POINT('Ctrl Pts',(-3.08696094432641,6.62204013560463,
97.2649027297406));
#112910=CARTESIAN_POINT('Ctrl Pts',(-3.16746394030832,6.41303970283115,
97.1997380332611));
#112911=CARTESIAN_POINT('Ctrl Pts',(-3.27698929875688,6.11558188393791,
97.1093035669909));
#112912=CARTESIAN_POINT('Ctrl Pts',(-3.32894253061792,5.97086114834436,
97.0659140969878));
#112913=CARTESIAN_POINT('Ctrl Pts',(-3.38495455445906,5.80916015520684,
97.0185474333141));
#112914=CARTESIAN_POINT('Ctrl Pts',(-3.41184824305314,5.73010863336922,
96.9956843445836));
#112915=CARTESIAN_POINT('Ctrl Pts',(-3.42596262200767,5.68824330614735,
96.9836568490984));
#112916=CARTESIAN_POINT('Ctrl Pts',(-3.43247025515977,5.66883807128544,
96.9781041851881));
#112917=CARTESIAN_POINT('Ctrl Pts',(-3.43616965951519,5.65778171617176,
96.9749459908604));
#112918=CARTESIAN_POINT('Ctrl Pts',(-3.43672740741094,5.65611434503391,
96.9744698093448));
#112919=CARTESIAN_POINT('Ctrl Pts',(-3.60276935109794,5.15911377442937,
96.8326696635262));
#112920=CARTESIAN_POINT('Ctrl Pts',(-3.74098279039443,4.67976192410362,
96.7084340657658));
#112921=CARTESIAN_POINT('Ctrl Pts',(-3.91397760600031,3.98465723159937,
96.5477461043137));
#112922=CARTESIAN_POINT('Ctrl Pts',(-3.96592027330548,3.75693302543452,
96.4984607795777));
#112923=CARTESIAN_POINT('Ctrl Pts',(-4.03591904901806,3.42163371778403,
96.4310666045399));
#112924=CARTESIAN_POINT('Ctrl Pts',(-4.06893940480704,3.25555499975203,
96.3990029302307));
#112925=CARTESIAN_POINT('Ctrl Pts',(-4.10414338226531,3.06460755890891,
96.3644790924407));
#112926=CARTESIAN_POINT('Ctrl Pts',(-4.12093315304482,2.96984375547221,
96.347941244464));
#112927=CARTESIAN_POINT('Ctrl Pts',(-4.12795661551212,2.92938357525808,
96.3410090871936));
#112928=CARTESIAN_POINT('Ctrl Pts',(-4.13260087720269,2.90244417691176,
96.3364222397417));
#112929=CARTESIAN_POINT('Ctrl Pts',(-4.13456032116638,2.89101293526736,
96.3344859573235));
#112930=CARTESIAN_POINT('Ctrl Pts',(-4.30537073788798,1.88630577984655,
96.1655730269347));
#112931=CARTESIAN_POINT('Ctrl Pts',(-4.3822632519282,0.924422265265613,
96.0811302365448));
#112932=CARTESIAN_POINT('Ctrl Pts',(-4.38226888389591,-1.31660223688345E-7,
96.08109859282));
#112933=CARTESIAN_POINT('Origin',(6.43246351666909,-92.,72.98888938658));
#112934=CARTESIAN_POINT('',(16.0575353748791,-92.5,68.792701625727));
#112935=CARTESIAN_POINT('',(16.0575353748791,-92.5,77.185077147433));
#112936=CARTESIAN_POINT('Origin',(6.43246351666909,-92.5,72.98888938658));
#112937=CARTESIAN_POINT('Origin',(16.0575353748791,-92.,68.792701625727));
#112938=CARTESIAN_POINT('Origin',(16.0575353748791,-92.,77.185077147433));
#112939=CARTESIAN_POINT('Origin',(27.4324635166691,25.,72.98888938658));
#112940=CARTESIAN_POINT('',(-10.7897587056049,60.03337045294,84.7813330856));
#112941=CARTESIAN_POINT('',(-12.5675365956403,55.41742345328,72.9889053195275));
#112942=CARTESIAN_POINT('Ctrl Pts',(-10.7897587055637,60.03337045294,84.7813330855873));
#112943=CARTESIAN_POINT('Ctrl Pts',(-10.868172625638,59.7799388856398,84.5271742059778));
#112944=CARTESIAN_POINT('Ctrl Pts',(-10.9470443127566,59.5350540421005,
84.2625454327982));
#112945=CARTESIAN_POINT('Ctrl Pts',(-11.0257532130399,59.298715922322,83.9873240920612));
#112946=CARTESIAN_POINT('Ctrl Pts',(-11.1037577008792,59.0644929319882,
83.7145658696824));
#112947=CARTESIAN_POINT('Ctrl Pts',(-11.1816022537234,58.8386643706073,
83.4314035267827));
#112948=CARTESIAN_POINT('Ctrl Pts',(-11.2586336094918,58.6212302381791,
83.1377318414606));
#112949=CARTESIAN_POINT('Ctrl Pts',(-11.2788912404733,58.5640496216161,
83.0605023474235));
#112950=CARTESIAN_POINT('Ctrl Pts',(-11.2990923685216,58.507449546707,82.9825461391374));
#112951=CARTESIAN_POINT('Ctrl Pts',(-11.319224547268,58.4514300134518,82.9038615093504));
#112952=CARTESIAN_POINT('Ctrl Pts',(-11.3482132341978,58.3707664781265,
82.7905620931367));
#112953=CARTESIAN_POINT('Ctrl Pts',(-11.377059007869,58.2913066169089,82.675752374104));
#112954=CARTESIAN_POINT('Ctrl Pts',(-11.4057238500298,58.2130504297991,
82.5594276195734));
#112955=CARTESIAN_POINT('Ctrl Pts',(-11.4200562711102,58.1739223362441,
82.5012652423081));
#112956=CARTESIAN_POINT('Ctrl Pts',(-11.4343434459378,58.1350951612161,
82.4427241029007));
#112957=CARTESIAN_POINT('Ctrl Pts',(-11.4485805234591,58.096568904715,82.3838036677011));
#112958=CARTESIAN_POINT('Ctrl Pts',(-11.4606645752162,58.06386884553,82.3337935734635));
#112959=CARTESIAN_POINT('Ctrl Pts',(-11.4730195897738,58.0305659718623,
82.2822208527233));
#112960=CARTESIAN_POINT('Ctrl Pts',(-11.484860368321,57.9987472502754,82.2323682571557));
#112961=CARTESIAN_POINT('Ctrl Pts',(-11.4869700498907,57.9930780816277,
82.2234859778654));
#112962=CARTESIAN_POINT('Ctrl Pts',(-11.4890635377764,57.9874560271675,
82.2146583348573));
#112963=CARTESIAN_POINT('Ctrl Pts',(-11.491136558511,57.9818928907926,82.2059039350897));
#112964=CARTESIAN_POINT('Ctrl Pts',(-11.5941202893394,57.7055268470603,
81.7710019902227));
#112965=CARTESIAN_POINT('Ctrl Pts',(-11.6914739522762,57.452348325549,81.3273738179643));
#112966=CARTESIAN_POINT('Ctrl Pts',(-11.7824236113942,57.2223573262586,
80.875119635137));
#112967=CARTESIAN_POINT('Ctrl Pts',(-11.7883235253147,57.2074377860266,
80.8457818588909));
#112968=CARTESIAN_POINT('Ctrl Pts',(-11.7941964818091,57.192615821914,80.8164077994128));
#112969=CARTESIAN_POINT('Ctrl Pts',(-11.8000422660877,57.1778914339208,
80.7869974908546));
#112970=CARTESIAN_POINT('Ctrl Pts',(-11.8480227721674,57.0570379172761,
80.5456061870847));
#112971=CARTESIAN_POINT('Ctrl Pts',(-11.8941729321993,56.942757763715,80.3017725851317));
#112972=CARTESIAN_POINT('Ctrl Pts',(-11.9383729337204,56.8350509732375,
80.0555178044805));
#112973=CARTESIAN_POINT('Ctrl Pts',(-11.960472934481,56.7811975779987,79.9323904141548));
#112974=CARTESIAN_POINT('Ctrl Pts',(-11.9820853781408,56.7289875235308,
79.8086577260715));
#112975=CARTESIAN_POINT('Ctrl Pts',(-12.0031951051495,56.6784208098339,
79.6843228350869));
#112976=CARTESIAN_POINT('Ctrl Pts',(-12.0137499686538,56.6531374529854,
79.6221553895946));
#112977=CARTESIAN_POINT('Ctrl Pts',(-12.0241791520448,56.6282649313297,
79.5598373931977));
#112978=CARTESIAN_POINT('Ctrl Pts',(-12.0344807519995,56.6038032448667,
79.4973692470241));
#112979=CARTESIAN_POINT('Ctrl Pts',(-12.0442431275652,56.5806219748433,
79.438170917976));
#112980=CARTESIAN_POINT('Ctrl Pts',(-12.0540526293657,56.5574302292912,
79.3778303823676));
#112981=CARTESIAN_POINT('Ctrl Pts',(-12.0634478798237,56.5353067074411,
79.3192118870842));
#112982=CARTESIAN_POINT('Ctrl Pts',(-12.0639668260734,56.5340847156757,
79.3159740970514));
#112983=CARTESIAN_POINT('Ctrl Pts',(-12.0644845215157,56.5328659829544,
79.3127415628864));
#112984=CARTESIAN_POINT('Ctrl Pts',(-12.0650008929351,56.5316506910558,
79.3095147679841));
#112985=CARTESIAN_POINT('Ctrl Pts',(-12.1397505417616,56.3557256897246,
78.8424056741844));
#112986=CARTESIAN_POINT('Ctrl Pts',(-12.2072603484823,56.2006332465385,
78.3674356697261));
#112987=CARTESIAN_POINT('Ctrl Pts',(-12.2667800777976,56.0663733614975,
77.8848119786146));
#112988=CARTESIAN_POINT('Ctrl Pts',(-12.3253653812388,55.9342212802365,
77.4097652047641));
#112989=CARTESIAN_POINT('Ctrl Pts',(-12.376209304955,55.8222527731538,76.9273030816847));
#112990=CARTESIAN_POINT('Ctrl Pts',(-12.4185828867259,55.7304678402495,
76.4376718607956));
#112991=CARTESIAN_POINT('Ctrl Pts',(-12.4605719336758,55.6395158438418,
75.9524839804513));
#112992=CARTESIAN_POINT('Ctrl Pts',(-12.4942434699381,55.5683827571013,
75.4602563976354));
#112993=CARTESIAN_POINT('Ctrl Pts',(-12.5188778974991,55.5170685800279,
74.961278599836));
#112994=CARTESIAN_POINT('Ctrl Pts',(-12.5431986105029,55.4664078788389,
74.4686551854904));
#112995=CARTESIAN_POINT('Ctrl Pts',(-12.5587107041102,55.4350645216717,
73.9694523035646));
#112996=CARTESIAN_POINT('Ctrl Pts',(-12.5647147706704,55.4230385085262,
73.463998901091));
#112997=CARTESIAN_POINT('Ctrl Pts',(-12.5665887310681,55.4192850071033,
73.306239214448));
#112998=CARTESIAN_POINT('Ctrl Pts',(-12.5675364200079,55.4174133220213,
73.1478710057732));
#112999=CARTESIAN_POINT('Ctrl Pts',(-12.5675364833277,55.41742345328,72.9889053195274));
#113000=CARTESIAN_POINT('',(-10.7897587056049,60.03337045294,61.19644568756));
#113001=CARTESIAN_POINT('Ctrl Pts',(-12.5675367079528,55.4174234532799,
72.9889053195275));
#113002=CARTESIAN_POINT('Ctrl Pts',(-12.5675367177603,55.4174203621651,
72.982050838097));
#113003=CARTESIAN_POINT('Ctrl Pts',(-12.5675348841624,55.4174209999673,
72.975196614252));
#113004=CARTESIAN_POINT('Ctrl Pts',(-12.5675312063047,55.4174253640918,
72.9683426483062));
#113005=CARTESIAN_POINT('Ctrl Pts',(-12.5673418846505,55.4176500120605,
72.6155274331763));
#113006=CARTESIAN_POINT('Ctrl Pts',(-12.5622677006653,55.4277450225524,
72.2633971372145));
#113007=CARTESIAN_POINT('Ctrl Pts',(-12.5525370191446,55.4476997595703,
71.9120808674882));
#113008=CARTESIAN_POINT('Ctrl Pts',(-12.5474620952179,55.4581069208906,
71.7288559475002));
#113009=CARTESIAN_POINT('Ctrl Pts',(-12.5411201910958,55.4711966604094,
71.5458521388165));
#113010=CARTESIAN_POINT('Ctrl Pts',(-12.5335411140015,55.4869721096583,
71.3630859763134));
#113011=CARTESIAN_POINT('Ctrl Pts',(-12.5334665414226,55.4871273285483,
71.3612876908618));
#113012=CARTESIAN_POINT('Ctrl Pts',(-12.5333918499186,55.4872828063653,
71.3594894491793));
#113013=CARTESIAN_POINT('Ctrl Pts',(-12.5333170395134,55.4874385430894,
71.3576912509943));
#113014=CARTESIAN_POINT('Ctrl Pts',(-12.52530966692,55.5041079084492,71.1652201257191));
#113015=CARTESIAN_POINT('Ctrl Pts',(-12.5159419633816,55.5237395698145,
70.9732476647015));
#113016=CARTESIAN_POINT('Ctrl Pts',(-12.5052315297495,55.5463351816122,
70.781537963485));
#113017=CARTESIAN_POINT('Ctrl Pts',(-12.494586011557,55.5687938424586,70.5909902058433));
#113018=CARTESIAN_POINT('Ctrl Pts',(-12.4826139196493,55.5941806061267,
70.4007016562411));
#113019=CARTESIAN_POINT('Ctrl Pts',(-12.4693110004844,55.62254352577,70.2104401810274));
#113020=CARTESIAN_POINT('Ctrl Pts',(-12.4587206881529,55.6451229441618,
70.0589750460298));
#113021=CARTESIAN_POINT('Ctrl Pts',(-12.4472865330326,55.6695893954222,
69.9075269903875));
#113022=CARTESIAN_POINT('Ctrl Pts',(-12.4349969289486,55.6959886852669,
69.7559810535915));
#113023=CARTESIAN_POINT('Ctrl Pts',(-12.4348262620416,55.6963552947291,
69.7538765206772));
#113024=CARTESIAN_POINT('Ctrl Pts',(-12.434655430027,55.6967222772554,69.7517719689367));
#113025=CARTESIAN_POINT('Ctrl Pts',(-12.4344844328715,55.6970896329577,
69.7496673980763));
#113026=CARTESIAN_POINT('Ctrl Pts',(-12.4147573136269,55.7394696931722,
69.5068731819895));
#113027=CARTESIAN_POINT('Ctrl Pts',(-12.3930365100942,55.7865471590384,
69.2663150158759));
#113028=CARTESIAN_POINT('Ctrl Pts',(-12.369431751922,55.8382937182926,69.0280167934519));
#113029=CARTESIAN_POINT('Ctrl Pts',(-12.3456145013075,55.8905061053548,
68.7875733861069));
#113030=CARTESIAN_POINT('Ctrl Pts',(-12.3198790436771,55.9474720578215,
68.5494302363846));
#113031=CARTESIAN_POINT('Ctrl Pts',(-12.2923167664104,56.0092105053825,
68.3136166604113));
#113032=CARTESIAN_POINT('Ctrl Pts',(-12.2871240455808,56.0208420015589,
68.2691894871404));
#113033=CARTESIAN_POINT('Ctrl Pts',(-12.2818664270495,56.0326430296357,
68.2248450281788));
#113034=CARTESIAN_POINT('Ctrl Pts',(-12.2765444463086,56.0446139033485,
68.1805835236521));
#113035=CARTESIAN_POINT('Ctrl Pts',(-12.2761514642722,56.0454978483604,
68.1773151961197));
#113036=CARTESIAN_POINT('Ctrl Pts',(-12.2757581312882,56.0463827194888,
68.1740473209075));
#113037=CARTESIAN_POINT('Ctrl Pts',(-12.2753644474245,56.0472685174559,
68.1707798974206));
#113038=CARTESIAN_POINT('Ctrl Pts',(-12.2443292802395,56.117098374705,67.9132000382251));
#113039=CARTESIAN_POINT('Ctrl Pts',(-12.2111136956103,56.1926615310602,
67.6584279769369));
#113040=CARTESIAN_POINT('Ctrl Pts',(-12.1757902067591,56.2739580008499,
67.406503196972));
#113041=CARTESIAN_POINT('Ctrl Pts',(-12.1581284623335,56.3146062357447,
67.2805408069895));
#113042=CARTESIAN_POINT('Ctrl Pts',(-12.1399397377143,56.3566878012821,
67.1552903360582));
#113043=CARTESIAN_POINT('Ctrl Pts',(-12.1212330098288,56.4002027038148,
67.0307566887872));
#113044=CARTESIAN_POINT('Ctrl Pts',(-12.1118796458861,56.4219601550811,
66.9684898651518));
#113045=CARTESIAN_POINT('Ctrl Pts',(-12.1023967812998,56.4440759405653,
66.9064022535711));
#113046=CARTESIAN_POINT('Ctrl Pts',(-12.0927855383316,56.4665500603436,
66.84449448797));
#113047=CARTESIAN_POINT('Ctrl Pts',(-12.0879799168475,56.4777871202328,
66.8135406051694));
#113048=CARTESIAN_POINT('Ctrl Pts',(-12.0831422008074,56.4891137636837,
66.7826316842441));
#113049=CARTESIAN_POINT('Ctrl Pts',(-12.0782725304343,56.5005299906145,
66.7517678045529));
#113050=CARTESIAN_POINT('Ctrl Pts',(-12.0741631291214,56.5101638784021,
66.7257224959376));
#113051=CARTESIAN_POINT('Ctrl Pts',(-12.0701688778298,56.5195377148765,
66.7005734698854));
#113052=CARTESIAN_POINT('Ctrl Pts',(-12.0659408536375,56.5294710194743,
66.6741328100669));
#113053=CARTESIAN_POINT('Ctrl Pts',(-12.0651586384838,56.5313087528999,
66.6692410961496));
#113054=CARTESIAN_POINT('Ctrl Pts',(-12.0643683768756,56.5331657640086,
66.6643052146056));
#113055=CARTESIAN_POINT('Ctrl Pts',(-12.0635677966548,56.535047421687,66.6593113694085));
#113056=CARTESIAN_POINT('Ctrl Pts',(-12.0630538197315,56.536255456309,66.6561052932107));
#113057=CARTESIAN_POINT('Ctrl Pts',(-12.0625394985148,56.5374644904417,
66.652899713093));
#113058=CARTESIAN_POINT('Ctrl Pts',(-12.0620248331215,56.5386745244904,
66.6496946288546));
#113059=CARTESIAN_POINT('Ctrl Pts',(-12.0160725489409,56.6467133186074,
66.3635262879531));
#113060=CARTESIAN_POINT('Ctrl Pts',(-11.967379099974,56.7627198108511,66.0813107384538));
#113061=CARTESIAN_POINT('Ctrl Pts',(-11.9163040906976,56.8866775804625,
65.8030527981967));
#113062=CARTESIAN_POINT('Ctrl Pts',(-11.8771617699855,56.9816750134855,
65.589804446556));
#113063=CARTESIAN_POINT('Ctrl Pts',(-11.8366199972925,57.0813432649774,
65.3788805106926));
#113064=CARTESIAN_POINT('Ctrl Pts',(-11.7948293248868,57.1856921089343,
65.170285466387));
#113065=CARTESIAN_POINT('Ctrl Pts',(-11.7942686561782,57.1870920656284,
65.1674869300781));
#113066=CARTESIAN_POINT('Ctrl Pts',(-11.7937077625437,57.1884928650177,
65.1646888129909));
#113067=CARTESIAN_POINT('Ctrl Pts',(-11.7931466444446,57.1898945067013,
65.1618911157007));
#113068=CARTESIAN_POINT('Ctrl Pts',(-11.7543525232861,57.2868000554267,
64.9684662238414));
#113069=CARTESIAN_POINT('Ctrl Pts',(-11.7144860248049,57.3877303365134,
64.7770433401785));
#113070=CARTESIAN_POINT('Ctrl Pts',(-11.6736515325127,57.4926792079085,
64.5876187494813));
#113071=CARTESIAN_POINT('Ctrl Pts',(-11.6631346852652,57.5197085937856,
64.5388327998231));
#113072=CARTESIAN_POINT('Ctrl Pts',(-11.6525535566606,57.5470047844004,
64.4901794771697));
#113073=CARTESIAN_POINT('Ctrl Pts',(-11.6419097870471,57.5745681821331,
64.4416588980482));
#113074=CARTESIAN_POINT('Ctrl Pts',(-11.6159242509573,57.6418610391336,
64.3232014994337));
#113075=CARTESIAN_POINT('Ctrl Pts',(-11.5895653660488,57.7107441790474,
64.2055345618778));
#113076=CARTESIAN_POINT('Ctrl Pts',(-11.5628547265451,57.7812175829487,
64.0886576456412));
#113077=CARTESIAN_POINT('Ctrl Pts',(-11.5476899162953,57.8212284481947,
64.0223014561138));
#113078=CARTESIAN_POINT('Ctrl Pts',(-11.5325098453544,57.861491635489,63.9566240152157));
#113079=CARTESIAN_POINT('Ctrl Pts',(-11.5171516660184,57.9024467648906,
63.8909009575293));
#113080=CARTESIAN_POINT('Ctrl Pts',(-11.5064596477077,57.9309588029324,
63.8451460460357));
#113081=CARTESIAN_POINT('Ctrl Pts',(-11.4956810919766,57.959807135689,63.7993694871288));
#113082=CARTESIAN_POINT('Ctrl Pts',(-11.4847584588285,57.9891528879259,
63.7533340900277));
#113083=CARTESIAN_POINT('Ctrl Pts',(-11.4837358338686,57.9919003663313,
63.7490240536585));
#113084=CARTESIAN_POINT('Ctrl Pts',(-11.4827119445604,57.9946522124987,
63.7447117530293));
#113085=CARTESIAN_POINT('Ctrl Pts',(-11.4816867427005,57.9974085638167,
63.7403969958321));
#113086=CARTESIAN_POINT('Ctrl Pts',(-11.4356078701281,58.1212959328434,
63.5464652884868));
#113087=CARTESIAN_POINT('Ctrl Pts',(-11.3889411870607,58.2488419536169,
63.3562493137595));
#113088=CARTESIAN_POINT('Ctrl Pts',(-11.3418218316508,58.3799615459157,
63.1697081560175));
#113089=CARTESIAN_POINT('Ctrl Pts',(-11.2938772096396,58.5133776174288,
62.9798998443447));
#113090=CARTESIAN_POINT('Ctrl Pts',(-11.245463670129,58.6504936180663,62.7938957316933));
#113091=CARTESIAN_POINT('Ctrl Pts',(-11.196706025114,58.7912696725781,62.611664155393));
#113092=CARTESIAN_POINT('Ctrl Pts',(-11.1477507289715,58.9326163975128,
62.4286938584979));
#113093=CARTESIAN_POINT('Ctrl Pts',(-11.0984482456183,59.0776530871168,
62.2495262909455));
#113094=CARTESIAN_POINT('Ctrl Pts',(-11.0489114884965,59.226386964476,62.0741478009945));
#113095=CARTESIAN_POINT('Ctrl Pts',(-10.9995158025983,59.3746972761584,
61.8992687554883));
#113096=CARTESIAN_POINT('Ctrl Pts',(-10.949886889216,59.5266839527353,61.728156812183));
#113097=CARTESIAN_POINT('Ctrl Pts',(-10.9001276897382,59.6823984335242,
61.560823247083));
#113098=CARTESIAN_POINT('Ctrl Pts',(-10.8633960277559,59.7973450511166,
61.437299556669));
#113099=CARTESIAN_POINT('Ctrl Pts',(-10.8265931653708,59.9143239540159,
61.3158352677684));
#113100=CARTESIAN_POINT('Ctrl Pts',(-10.7897587056886,60.03337045294,61.1964456875342));
#113101=CARTESIAN_POINT('',(-9.38953228746991,65.4601089375,57.36388938658));
#113102=CARTESIAN_POINT('Ctrl Pts',(-10.7897587055637,60.03337045294,61.1964456875727));
#113103=CARTESIAN_POINT('Ctrl Pts',(-10.6961215374564,60.3360244277033,
60.8929445016431));
#113104=CARTESIAN_POINT('Ctrl Pts',(-10.6017811001726,60.6488111261909,
60.5999839999674));
#113105=CARTESIAN_POINT('Ctrl Pts',(-10.5074126423797,60.9717305484028,
60.3174333914687));
#113106=CARTESIAN_POINT('Ctrl Pts',(-10.4809076023769,61.0624281438025,
60.2380740869275));
#113107=CARTESIAN_POINT('Ctrl Pts',(-10.4544000522521,61.1539250752782,
60.1595358809919));
#113108=CARTESIAN_POINT('Ctrl Pts',(-10.4279042524337,61.2462213428298,
60.081815652062));
#113109=CARTESIAN_POINT('Ctrl Pts',(-10.3674885729892,61.4566751412635,
59.9045981130723));
#113110=CARTESIAN_POINT('Ctrl Pts',(-10.3071345414077,61.6712849314232,
59.7316336177837));
#113111=CARTESIAN_POINT('Ctrl Pts',(-10.2470052704755,61.890050713309,59.5628835799898));
#113112=CARTESIAN_POINT('Ctrl Pts',(-10.2169406350094,61.9994336042519,
59.4785085610928));
#113113=CARTESIAN_POINT('Ctrl Pts',(-10.1869320857492,62.1098554931263,
59.3951871939623));
#113114=CARTESIAN_POINT('Ctrl Pts',(-10.156999204859,62.2213163799322,59.3129143826965));
#113115=CARTESIAN_POINT('Ctrl Pts',(-10.1270663239688,62.3327772667381,
59.2306415714307));
#113116=CARTESIAN_POINT('Ctrl Pts',(-10.0974532818734,62.4443457418673,
59.150075118638));
#113117=CARTESIAN_POINT('Ctrl Pts',(-10.067446726607,62.5588160341445,59.0692366701422));
#113118=CARTESIAN_POINT('Ctrl Pts',(-9.97973504987513,62.8934222954267,
58.8329391078582));
#113119=CARTESIAN_POINT('Ctrl Pts',(-9.89342052728445,63.2348821549413,
58.6072400191336));
#113120=CARTESIAN_POINT('Ctrl Pts',(-9.80904661013946,63.5831956126882,
58.3919745250479));
#113121=CARTESIAN_POINT('Ctrl Pts',(-9.724205933447,63.9334359530241,58.1755181744985));
#113122=CARTESIAN_POINT('Ctrl Pts',(-9.64132737070179,64.2906059300402,
57.9696108949634));
#113123=CARTESIAN_POINT('Ctrl Pts',(-9.56091064477735,64.6547055437366,
57.7740851436321));
#113124=CARTESIAN_POINT('Ctrl Pts',(-9.50242514788926,64.9195080034116,
57.6318831254627));
#113125=CARTESIAN_POINT('Ctrl Pts',(-9.44524070271336,65.1879758013327,
57.4951722686513));
#113126=CARTESIAN_POINT('Ctrl Pts',(-9.38953228746956,65.4601089375,57.3638893865801));
#113127=CARTESIAN_POINT('',(-9.38953228747191,-65.46010893749,57.36388938658));
#113128=CARTESIAN_POINT('',(-9.38953228747191,-65.46010893749,57.36388938658));
#113129=CARTESIAN_POINT('',(-10.7897587056049,-60.03337045294,61.19644568756));
#113130=CARTESIAN_POINT('Ctrl Pts',(-9.38953228746987,-65.46010893749,57.3638893865809));
#113131=CARTESIAN_POINT('Ctrl Pts',(-9.46407446179315,-65.0959614287623,
57.5395560509113));
#113132=CARTESIAN_POINT('Ctrl Pts',(-9.54149305329802,-64.737710655496,
57.72548653469));
#113133=CARTESIAN_POINT('Ctrl Pts',(-9.62133689772822,-64.3853566176911,
57.92184339707));
#113134=CARTESIAN_POINT('Ctrl Pts',(-9.65220875720963,-64.2491178829401,
57.997765360834));
#113135=CARTESIAN_POINT('Ctrl Pts',(-9.68344264578583,-64.1137607131964,
58.0752461350595));
#113136=CARTESIAN_POINT('Ctrl Pts',(-9.71501039923335,-63.9792851084599,
58.1542953015588));
#113137=CARTESIAN_POINT('Ctrl Pts',(-9.79705218697199,-63.6297949542694,
58.3597370650858));
#113138=CARTESIAN_POINT('Ctrl Pts',(-9.88157720980486,-63.2854296652719,
58.5763549087011));
#113139=CARTESIAN_POINT('Ctrl Pts',(-9.9675636085802,-62.9479926546559,
58.803052399267));
#113140=CARTESIAN_POINT('Ctrl Pts',(-10.000231858517,-62.8197924188312,
58.8891800937317));
#113141=CARTESIAN_POINT('Ctrl Pts',(-10.0331114014216,-62.6925922234125,
58.9767623509528));
#113142=CARTESIAN_POINT('Ctrl Pts',(-10.0661477385087,-62.5664909655025,
59.0657376624532));
#113143=CARTESIAN_POINT('Ctrl Pts',(-10.1635313447246,-62.194773144266,
59.3280166395464));
#113144=CARTESIAN_POINT('Ctrl Pts',(-10.2616480241468,-61.834854396424,
59.6006923739533));
#113145=CARTESIAN_POINT('Ctrl Pts',(-10.359861054366,-61.4867347219765,
59.8839207289473));
#113146=CARTESIAN_POINT('Ctrl Pts',(-10.4570476923973,-61.1422531321451,
60.1641891572358));
#113147=CARTESIAN_POINT('Ctrl Pts',(-10.554328628233,-60.8093252878649,
60.4547910987241));
#113148=CARTESIAN_POINT('Ctrl Pts',(-10.651037906848,-60.4879511891359,
60.755863623304));
#113149=CARTESIAN_POINT('Ctrl Pts',(-10.6974363335145,-60.3337648197827,
60.9003098610704));
#113150=CARTESIAN_POINT('Ctrl Pts',(-10.7437024522593,-60.1822379077174,
61.047165996827));
#113151=CARTESIAN_POINT('Ctrl Pts',(-10.7897587055637,-60.03337045294,61.1964456875727));
#113152=CARTESIAN_POINT('',(-12.5675365956403,-55.41742345328,72.9888734536679));
#113153=CARTESIAN_POINT('Ctrl Pts',(-10.7897587055637,-60.03337045294,61.1964456875727));
#113154=CARTESIAN_POINT('Ctrl Pts',(-10.8681726256022,-59.7799388857426,
61.4506045670663));
#113155=CARTESIAN_POINT('Ctrl Pts',(-10.9470443126877,-59.5350540422957,
61.7152333401302));
#113156=CARTESIAN_POINT('Ctrl Pts',(-11.0257532129406,-59.2987159225995,
61.9904546807518));
#113157=CARTESIAN_POINT('Ctrl Pts',(-11.1037577007278,-59.0644929324136,
62.2632129029387));
#113158=CARTESIAN_POINT('Ctrl Pts',(-11.1816022535226,-58.8386643711656,
62.5463752456409));
#113159=CARTESIAN_POINT('Ctrl Pts',(-11.2586336092453,-58.6212302388556,
62.8400469307598));
#113160=CARTESIAN_POINT('Ctrl Pts',(-11.2788912403012,-58.5640496220798,
62.9172764250728));
#113161=CARTESIAN_POINT('Ctrl Pts',(-11.2990923684237,-58.5074495469618,
62.9952326336407));
#113162=CARTESIAN_POINT('Ctrl Pts',(-11.3192245472439,-58.4514300135017,
63.0739172637152));
#113163=CARTESIAN_POINT('Ctrl Pts',(-11.3482132341742,-58.3707664781753,
63.18721667993));
#113164=CARTESIAN_POINT('Ctrl Pts',(-11.3770590078463,-58.291306616956,
63.3020263989648));
#113165=CARTESIAN_POINT('Ctrl Pts',(-11.4057238500081,-58.2130504298437,
63.4183511534986));
#113166=CARTESIAN_POINT('Ctrl Pts',(-11.4200562710891,-58.1739223362876,
63.4765135307655));
#113167=CARTESIAN_POINT('Ctrl Pts',(-11.4343434459173,-58.1350951612583,
63.5350546701748));
#113168=CARTESIAN_POINT('Ctrl Pts',(-11.4485805234392,-58.0965689047557,
63.5939751053765));
#113169=CARTESIAN_POINT('Ctrl Pts',(-11.4606645751704,-58.0638688456409,
63.6439851995063));
#113170=CARTESIAN_POINT('Ctrl Pts',(-11.4730195897036,-58.030565972039,
63.6955579201435));
#113171=CARTESIAN_POINT('Ctrl Pts',(-11.4848603682263,-57.9987472505176,
63.7454105156055));
#113172=CARTESIAN_POINT('Ctrl Pts',(-11.4869700498222,-57.9930780817996,
63.7542927950056));
#113173=CARTESIAN_POINT('Ctrl Pts',(-11.4890635377336,-57.9874560272703,
63.7631204381219));
#113174=CARTESIAN_POINT('Ctrl Pts',(-11.4911365584932,-57.9818928908282,
63.7718748379952));
#113175=CARTESIAN_POINT('Ctrl Pts',(-11.5941202890719,-57.7055268477676,
64.2067767818039));
#113176=CARTESIAN_POINT('Ctrl Pts',(-11.6914739517999,-57.4523483267938,
64.6504049530184));
#113177=CARTESIAN_POINT('Ctrl Pts',(-11.7824236107497,-57.222357327907,
65.1026591348182));
#113178=CARTESIAN_POINT('Ctrl Pts',(-11.7883235248732,-57.2074377871601,
65.1319969120616));
#113179=CARTESIAN_POINT('Ctrl Pts',(-11.7941964815689,-57.1926158225392,
65.1613709725395));
#113180=CARTESIAN_POINT('Ctrl Pts',(-11.800042266047,-57.1778914340443,
65.1907812821003));
#113181=CARTESIAN_POINT('Ctrl Pts',(-11.8480227721297,-57.0570379173963,
65.4321725858791));
#113182=CARTESIAN_POINT('Ctrl Pts',(-11.8941729321676,-56.942757763823,
65.6760061878564));
#113183=CARTESIAN_POINT('Ctrl Pts',(-11.9383729336968,-56.8350509733243,
65.9222609685475));
#113184=CARTESIAN_POINT('Ctrl Pts',(-11.9604729344613,-56.7811975780749,
66.0453883588931));
#113185=CARTESIAN_POINT('Ctrl Pts',(-11.9820853781256,-56.7289875235943,
66.1691210470003));
#113186=CARTESIAN_POINT('Ctrl Pts',(-12.0031951051392,-56.6784208098823,
66.2934559380126));
#113187=CARTESIAN_POINT('Ctrl Pts',(-12.013749968646,-56.6531374530263,
66.3556233835188));
#113188=CARTESIAN_POINT('Ctrl Pts',(-12.0241791520395,-56.6282649313624,
66.4179413799305));
#113189=CARTESIAN_POINT('Ctrl Pts',(-12.0344807519969,-56.6038032448907,
66.4804095261199));
#113190=CARTESIAN_POINT('Ctrl Pts',(-12.0442431275156,-56.5806219749766,
66.539607854883));
#113191=CARTESIAN_POINT('Ctrl Pts',(-12.054052629272,-56.5574302295258,
66.5999483902158));
#113192=CARTESIAN_POINT('Ctrl Pts',(-12.0634478796864,-56.5353067077742,
66.6585668852194));
#113193=CARTESIAN_POINT('Ctrl Pts',(-12.0639668259839,-56.534084715896,
66.6618046755502));
#113194=CARTESIAN_POINT('Ctrl Pts',(-12.0644845214739,-56.5328659830625,
66.6650372100122));
#113195=CARTESIAN_POINT('Ctrl Pts',(-12.0650008929406,-56.5316506910522,
66.6682640052103));
#113196=CARTESIAN_POINT('Ctrl Pts',(-12.1397505417374,-56.3557256897672,
67.1353730988268));
#113197=CARTESIAN_POINT('Ctrl Pts',(-12.2072603484355,-56.2006332466164,
67.6103431031051));
#113198=CARTESIAN_POINT('Ctrl Pts',(-12.2667800777353,-56.0663733615999,
68.0929667940404));
#113199=CARTESIAN_POINT('Ctrl Pts',(-12.3253653811598,-55.9342212803662,
68.5680135677053));
#113200=CARTESIAN_POINT('Ctrl Pts',(-12.3762093048664,-55.8222527732994,
69.0504756906023));
#113201=CARTESIAN_POINT('Ctrl Pts',(-12.4185828866349,-55.7304678403994,
69.5401069113127));
#113202=CARTESIAN_POINT('Ctrl Pts',(-12.4605719335821,-55.6395158439964,
70.0252947914776));
#113203=CARTESIAN_POINT('Ctrl Pts',(-12.4942434698488,-55.568382757249,
70.5175223741176));
#113204=CARTESIAN_POINT('Ctrl Pts',(-12.5188778974211,-55.5170685801572,
71.0165001717449));
#113205=CARTESIAN_POINT('Ctrl Pts',(-12.5431986104359,-55.4664078789505,
71.5091235859169));
#113206=CARTESIAN_POINT('Ctrl Pts',(-12.558710704061,-55.435064521754,72.0083264676726));
#113207=CARTESIAN_POINT('Ctrl Pts',(-12.5647147706456,-55.4230385085677,
72.5137798699802));
#113208=CARTESIAN_POINT('Ctrl Pts',(-12.5665887310599,-55.4192850071141,
72.6715395573251));
#113209=CARTESIAN_POINT('Ctrl Pts',(-12.5675364200081,-55.4174133220182,
72.829907766708));
#113210=CARTESIAN_POINT('Ctrl Pts',(-12.5675364833277,-55.41742345328,72.988873453668));
#113211=CARTESIAN_POINT('',(-10.7897587055989,-60.03337045296,84.78133308562));
#113212=CARTESIAN_POINT('Ctrl Pts',(-12.5675367079528,-55.4174234532799,
72.9888734536678));
#113213=CARTESIAN_POINT('Ctrl Pts',(-12.5675367177603,-55.417420362165,
72.9957279350907));
#113214=CARTESIAN_POINT('Ctrl Pts',(-12.5675348841625,-55.4174209999673,
73.0025821589281));
#113215=CARTESIAN_POINT('Ctrl Pts',(-12.5675312063047,-55.4174253640918,
73.0094361248664));
#113216=CARTESIAN_POINT('Ctrl Pts',(-12.5673418846506,-55.4176500120595,
73.3622513396429));
#113217=CARTESIAN_POINT('Ctrl Pts',(-12.5622677006751,-55.4277450225353,
73.7143816352725));
#113218=CARTESIAN_POINT('Ctrl Pts',(-12.5525370191716,-55.4476997595217,
74.0656979046879));
#113219=CARTESIAN_POINT('Ctrl Pts',(-12.5474620952415,-55.458106920851,
74.2489228249614));
#113220=CARTESIAN_POINT('Ctrl Pts',(-12.5411201911119,-55.4711966603877,
74.4319266339354));
#113221=CARTESIAN_POINT('Ctrl Pts',(-12.5335411140059,-55.4869721096635,
74.6146927967335));
#113222=CARTESIAN_POINT('Ctrl Pts',(-12.5334665414252,-55.4871273285572,
74.6164910822281));
#113223=CARTESIAN_POINT('Ctrl Pts',(-12.5333918499194,-55.487282806378,
74.6182893239537));
#113224=CARTESIAN_POINT('Ctrl Pts',(-12.5333170395124,-55.4874385431059,
74.6200875221817));
#113225=CARTESIAN_POINT('Ctrl Pts',(-12.5253096668512,-55.5041079086092,
74.8125586490817));
#113226=CARTESIAN_POINT('Ctrl Pts',(-12.5159419632214,-55.5237395701696,
75.0045311117337));
#113227=CARTESIAN_POINT('Ctrl Pts',(-12.5052315294745,-55.5463351822132,
75.1962408145872));
#113228=CARTESIAN_POINT('Ctrl Pts',(-12.494586011168,-55.5687938433041,
75.3867885738564));
#113229=CARTESIAN_POINT('Ctrl Pts',(-12.4826139191233,-55.5941806072669,
75.5770771250886));
#113230=CARTESIAN_POINT('Ctrl Pts',(-12.4693109997989,-55.6225435272547,
75.7673386019281));
#113231=CARTESIAN_POINT('Ctrl Pts',(-12.4587206876582,-55.6451229452431,
75.9188037336736));
#113232=CARTESIAN_POINT('Ctrl Pts',(-12.4472865327652,-55.6695893960182,
76.0702517860621));
#113233=CARTESIAN_POINT('Ctrl Pts',(-12.4349969289462,-55.6959886852914,
76.2217977195888));
#113234=CARTESIAN_POINT('Ctrl Pts',(-12.4348262620392,-55.6963552947537,
76.2239022525037));
#113235=CARTESIAN_POINT('Ctrl Pts',(-12.4346554300246,-55.69672227728,76.2260068042449));
#113236=CARTESIAN_POINT('Ctrl Pts',(-12.434484432869,-55.6970896329825,
76.2281113751059));
#113237=CARTESIAN_POINT('Ctrl Pts',(-12.4147573136306,-55.73946969318,76.4709055911142));
#113238=CARTESIAN_POINT('Ctrl Pts',(-12.3930365101054,-55.786547159027,
76.7114637571515));
#113239=CARTESIAN_POINT('Ctrl Pts',(-12.3694317519418,-55.8382937182597,
76.9497619795014));
#113240=CARTESIAN_POINT('Ctrl Pts',(-12.3456145013358,-55.8905061053007,
77.1902053867733));
#113241=CARTESIAN_POINT('Ctrl Pts',(-12.3198790437151,-55.9474720577438,
77.4283485364247));
#113242=CARTESIAN_POINT('Ctrl Pts',(-12.292316766459,-56.0092105052791,
77.6641621123292));
#113243=CARTESIAN_POINT('Ctrl Pts',(-12.2871240456124,-56.020842001493,
77.7085892857489));
#113244=CARTESIAN_POINT('Ctrl Pts',(-12.2818664270638,-56.0326430296083,
77.7529337448585));
#113245=CARTESIAN_POINT('Ctrl Pts',(-12.2765444463052,-56.0446139033609,
77.7971952495328));
#113246=CARTESIAN_POINT('Ctrl Pts',(-12.2761514642688,-56.0454978483726,
77.800463577065));
#113247=CARTESIAN_POINT('Ctrl Pts',(-12.2757581312848,-56.046382719501,
77.8037314522769));
#113248=CARTESIAN_POINT('Ctrl Pts',(-12.2753644474211,-56.0472685174681,
77.8069988757635));
#113249=CARTESIAN_POINT('Ctrl Pts',(-12.2443292802359,-56.1170983747168,
78.064578734961));
#113250=CARTESIAN_POINT('Ctrl Pts',(-12.2111136956062,-56.1926615310725,
78.3193507962519));
#113251=CARTESIAN_POINT('Ctrl Pts',(-12.1757902067544,-56.2739580008635,
78.5712755762204));
#113252=CARTESIAN_POINT('Ctrl Pts',(-12.1581284623285,-56.314606235759,
78.6972379662047));
#113253=CARTESIAN_POINT('Ctrl Pts',(-12.139939737709,-56.3566878012973,
78.822488437138));
#113254=CARTESIAN_POINT('Ctrl Pts',(-12.121233009823,-56.4002027038311,
78.9470220844111));
#113255=CARTESIAN_POINT('Ctrl Pts',(-12.1118796458801,-56.421960155098,
79.0092889080477));
#113256=CARTESIAN_POINT('Ctrl Pts',(-12.1023967812936,-56.4440759405827,
79.0713765196295));
#113257=CARTESIAN_POINT('Ctrl Pts',(-12.0927855383251,-56.4665500603618,
79.1332842852319));
#113258=CARTESIAN_POINT('Ctrl Pts',(-12.0879799168409,-56.4777871202513,
79.1642381680331));
#113259=CARTESIAN_POINT('Ctrl Pts',(-12.0831422008006,-56.4891137637026,
79.195147088959));
#113260=CARTESIAN_POINT('Ctrl Pts',(-12.0782725304274,-56.5005299906337,
79.2260109686509));
#113261=CARTESIAN_POINT('Ctrl Pts',(-12.0741631291138,-56.5101638784231,
79.2520562772707));
#113262=CARTESIAN_POINT('Ctrl Pts',(-12.0701688778214,-56.5195377148995,
79.2772053033278));
#113263=CARTESIAN_POINT('Ctrl Pts',(-12.0659408536283,-56.5294710194992,
79.303645963151));
#113264=CARTESIAN_POINT('Ctrl Pts',(-12.0651586384752,-56.5313087529233,
79.3085376770643));
#113265=CARTESIAN_POINT('Ctrl Pts',(-12.0643683768676,-56.5331657640305,
79.3134735586042));
#113266=CARTESIAN_POINT('Ctrl Pts',(-12.0635677966475,-56.5350474217073,
79.3184674037971));
#113267=CARTESIAN_POINT('Ctrl Pts',(-12.0630538197257,-56.5362554563258,
79.3216734799854));
#113268=CARTESIAN_POINT('Ctrl Pts',(-12.0625394985106,-56.5374644904549,
79.3248790600936));
#113269=CARTESIAN_POINT('Ctrl Pts',(-12.0620248331187,-56.5386745245,79.3280841443224));
#113270=CARTESIAN_POINT('Ctrl Pts',(-12.016072548911,-56.646713318681,79.6142524853919));
#113271=CARTESIAN_POINT('Ctrl Pts',(-11.9673790999134,-56.7627198109995,
79.8964680350565));
#113272=CARTESIAN_POINT('Ctrl Pts',(-11.9163040906032,-56.8866775806963,
80.1747259754764));
#113273=CARTESIAN_POINT('Ctrl Pts',(-11.8771617699198,-56.9816750136521,
80.387974326944));
#113274=CARTESIAN_POINT('Ctrl Pts',(-11.8366199972576,-57.08134326507,80.5988982626393));
#113275=CARTESIAN_POINT('Ctrl Pts',(-11.7948293248845,-57.185692108946,
80.8074933067817));
#113276=CARTESIAN_POINT('Ctrl Pts',(-11.7942686561726,-57.1870920656483,
80.8102918431072));
#113277=CARTESIAN_POINT('Ctrl Pts',(-11.7937077625348,-57.1884928650459,
80.8130899602107));
#113278=CARTESIAN_POINT('Ctrl Pts',(-11.7931466444324,-57.1898945067378,
80.8158876575174));
#113279=CARTESIAN_POINT('Ctrl Pts',(-11.7543525232763,-57.2868000554576,
81.0093125493625));
#113280=CARTESIAN_POINT('Ctrl Pts',(-11.7144860247975,-57.3877303365387,
81.2007354330128));
#113281=CARTESIAN_POINT('Ctrl Pts',(-11.6736515325075,-57.4926792079279,
81.3901600236987));
#113282=CARTESIAN_POINT('Ctrl Pts',(-11.6631346852557,-57.5197085938161,
81.4389459733767));
#113283=CARTESIAN_POINT('Ctrl Pts',(-11.6525535566467,-57.5470047844422,
81.4875992960499));
#113284=CARTESIAN_POINT('Ctrl Pts',(-11.6419097870288,-57.5745681821866,
81.5361198751912));
#113285=CARTESIAN_POINT('Ctrl Pts',(-11.6159242509377,-57.6418610391903,
81.65457727381));
#113286=CARTESIAN_POINT('Ctrl Pts',(-11.5895653660279,-57.7107441791077,
81.7722442113706));
#113287=CARTESIAN_POINT('Ctrl Pts',(-11.5628547265227,-57.7812175830128,
81.8891211276125));
#113288=CARTESIAN_POINT('Ctrl Pts',(-11.5476899162457,-57.8212284483305,
81.9554773172582));
#113289=CARTESIAN_POINT('Ctrl Pts',(-11.5325098452768,-57.8614916356994,
82.0211547582754));
#113290=CARTESIAN_POINT('Ctrl Pts',(-11.5171516659124,-57.9024467651775,
82.0868778160803));
#113291=CARTESIAN_POINT('Ctrl Pts',(-11.5064596476346,-57.930958803132,
82.1326327274308));
#113292=CARTESIAN_POINT('Ctrl Pts',(-11.495681091937,-57.9598071357988,
82.1784092861939));
#113293=CARTESIAN_POINT('Ctrl Pts',(-11.4847584588241,-57.989152887941,
82.2244446831469));
#113294=CARTESIAN_POINT('Ctrl Pts',(-11.4837358338566,-57.9919003663668,
82.2287547195481));
#113295=CARTESIAN_POINT('Ctrl Pts',(-11.4827119445408,-57.9946522125546,
82.2330670202093));
#113296=CARTESIAN_POINT('Ctrl Pts',(-11.4816867426733,-57.9974085638931,
82.2373817774385));
#113297=CARTESIAN_POINT('Ctrl Pts',(-11.43560787011,-58.1212959328948,82.4313134847434));
#113298=CARTESIAN_POINT('Ctrl Pts',(-11.3889411870521,-58.2488419536418,
82.6215294594314));
#113299=CARTESIAN_POINT('Ctrl Pts',(-11.341821831652,-58.3799615459125,
82.8080706171353));
#113300=CARTESIAN_POINT('Ctrl Pts',(-11.2938772096503,-58.5133776173983,
82.9978789287711));
#113301=CARTESIAN_POINT('Ctrl Pts',(-11.2454636701495,-58.6504936180069,
83.1838830413866));
#113302=CARTESIAN_POINT('Ctrl Pts',(-11.1967060251446,-58.7912696724882,
83.366114617652));
#113303=CARTESIAN_POINT('Ctrl Pts',(-11.1477507290122,-58.9326163973922,
83.549084914512));
#113304=CARTESIAN_POINT('Ctrl Pts',(-11.0984482456694,-59.0776530869639,
83.7282524820302));
#113305=CARTESIAN_POINT('Ctrl Pts',(-11.0489114885581,-59.2263869642892,
83.9036309719482));
#113306=CARTESIAN_POINT('Ctrl Pts',(-10.9995158026708,-59.3746972759362,
84.0785100174197));
#113307=CARTESIAN_POINT('Ctrl Pts',(-10.9498868892997,-59.5266839524761,
84.2496219606914));
#113308=CARTESIAN_POINT('Ctrl Pts',(-10.9001276898329,-59.6823984332261,
84.416955525759));
#113309=CARTESIAN_POINT('Ctrl Pts',(-10.863396027817,-59.7973450509208,
84.5404792162896));
#113310=CARTESIAN_POINT('Ctrl Pts',(-10.8265931653981,-59.9143239539261,
84.661943505303));
#113311=CARTESIAN_POINT('Ctrl Pts',(-10.7897587056822,-60.03337045296,84.7813330856457));
#113312=CARTESIAN_POINT('',(-9.38953228746991,-65.4601089375,88.61388938658));
#113313=CARTESIAN_POINT('Ctrl Pts',(-10.7897587055989,-60.03337045296,84.78133308562));
#113314=CARTESIAN_POINT('Ctrl Pts',(-10.670470502179,-60.4185374401732,
85.1679756114817));
#113315=CARTESIAN_POINT('Ctrl Pts',(-10.549981394999,-60.8207041658133,
85.5377156681126));
#113316=CARTESIAN_POINT('Ctrl Pts',(-10.3694938731286,-61.449453861914,
86.0673758482434));
#113317=CARTESIAN_POINT('Ctrl Pts',(-10.2793086657354,-61.7702036118744,
86.325969517694));
#113318=CARTESIAN_POINT('Ctrl Pts',(-10.1895683919245,-62.1005157147001,
86.5752922699324));
#113319=CARTESIAN_POINT('Ctrl Pts',(-10.1298782561999,-62.3228487505539,
86.7394569667994));
#113320=CARTESIAN_POINT('Ctrl Pts',(-10.1003989068031,-62.4339433710822,
86.8197126563052));
#113321=CARTESIAN_POINT('Ctrl Pts',(-9.83051728469071,-63.4637761676075,
87.54725601639));
#113322=CARTESIAN_POINT('Ctrl Pts',(-9.60025786520268,-64.4343560676532,
88.1172918608766));
#113323=CARTESIAN_POINT('Ctrl Pts',(-9.38953228746991,-65.4601089375,88.61388938658));
#113324=CARTESIAN_POINT('',(-9.38953228746991,65.4601089375,88.61388938658));
#113325=CARTESIAN_POINT('',(-9.38953228746991,65.4601089375,88.61388938658));
#113326=CARTESIAN_POINT('Ctrl Pts',(-9.38953228746955,65.4601089375,88.6138893865798));
#113327=CARTESIAN_POINT('Ctrl Pts',(-9.4673250436269,65.0800846589239,88.4305623759675));
#113328=CARTESIAN_POINT('Ctrl Pts',(-9.54819413567023,64.706647013074,88.2361905377287));
#113329=CARTESIAN_POINT('Ctrl Pts',(-9.63163220313212,64.3397959999503,
88.0305916995967));
#113330=CARTESIAN_POINT('Ctrl Pts',(-9.715070270594,63.9729449868266,87.8249928614648));
#113331=CARTESIAN_POINT('Ctrl Pts',(-9.80107740201692,63.6126806064291,
87.6081667119018));
#113332=CARTESIAN_POINT('Ctrl Pts',(-9.88908572874933,63.2590028587578,
87.3799269420104));
#113333=CARTESIAN_POINT('Ctrl Pts',(-9.93149413019431,63.088576849512,87.2699454874521));
#113334=CARTESIAN_POINT('Ctrl Pts',(-9.97461011732333,62.9187650612967,
87.1566690415153));
#113335=CARTESIAN_POINT('Ctrl Pts',(-10.0178349665076,62.7515519635204,
87.0414743274715));
#113336=CARTESIAN_POINT('Ctrl Pts',(-10.0344118943353,62.6874249739302,
86.9972966265224));
#113337=CARTESIAN_POINT('Ctrl Pts',(-10.0510053294605,62.6236801887277,
86.9528369978398));
#113338=CARTESIAN_POINT('Ctrl Pts',(-10.0675834133922,62.5604295403834,
86.9081738596842));
#113339=CARTESIAN_POINT('Ctrl Pts',(-10.1642608210937,62.1915745663972,
86.647714542764));
#113340=CARTESIAN_POINT('Ctrl Pts',(-10.2617150056454,61.8342111001938,
86.3768550872122));
#113341=CARTESIAN_POINT('Ctrl Pts',(-10.3593126521196,61.4883391417732,
86.0954394287602));
#113342=CARTESIAN_POINT('Ctrl Pts',(-10.455900523795,61.1460456793497,85.8169353819112));
#113343=CARTESIAN_POINT('Ctrl Pts',(-10.5526288561325,60.8150071655915,
85.5280921336091));
#113344=CARTESIAN_POINT('Ctrl Pts',(-10.6488346943094,60.4952236004985,
85.2287720071987));
#113345=CARTESIAN_POINT('Ctrl Pts',(-10.6959629091748,60.3385716877694,
85.0821444895936));
#113346=CARTESIAN_POINT('Ctrl Pts',(-10.742964994564,60.1846206385832,84.9330030588417));
#113347=CARTESIAN_POINT('Ctrl Pts',(-10.7897587055637,60.03337045294,84.7813330855873));
#113348=CARTESIAN_POINT('Origin',(24.4068933420691,-10.33199109902,60.67496896178));
#113349=CARTESIAN_POINT('',(25.579982351165,-11.2436243723453,60.4681262431048));
#113350=CARTESIAN_POINT('',(25.4229139949212,-10.8757227763334,59.7147318914574));
#113351=CARTESIAN_POINT('Origin',(24.4069013928191,-10.33197941375,60.67497222926));
#113352=CARTESIAN_POINT('',(23.4739859593054,-11.4524032074963,60.3223210887327));
#113353=CARTESIAN_POINT('Origin',(24.4068933420691,-10.33199109902,60.67496896178));
#113354=CARTESIAN_POINT('',(24.9372779666099,-10.3319811032157,59.2718682957262));
#113355=CARTESIAN_POINT('Origin',(24.4069013928191,-10.33197941375,60.67497222926));
#113356=CARTESIAN_POINT('',(22.9296817484535,-10.3319903259816,60.9354414318888));
#113357=CARTESIAN_POINT('Origin',(24.4068932609991,-10.33199110019,60.67496850203));
#113358=CARTESIAN_POINT('Origin',(24.4068933430391,-10.33198915989,60.67496896729));
#113359=CARTESIAN_POINT('Origin',(71.6139524734691,1.4210854715202E-14,
50.72762564822));
#113360=CARTESIAN_POINT('Origin',(72.5315042041368,1.25011112572802E-13,
55.931320096872));
#113361=CARTESIAN_POINT('',(82.4056897430765,1.53742691743921E-14,57.2222894375664));
#113362=CARTESIAN_POINT('',(80.9696261270861,1.53742691743921E-14,49.0779679603843));
#113363=CARTESIAN_POINT('',(81.8983892080091,3.04138126515101,57.22463037752));
#113364=CARTESIAN_POINT('Ctrl Pts',(82.4056897430765,1.31838984174237E-14,
57.2222894375664));
#113365=CARTESIAN_POINT('Ctrl Pts',(82.4056897430765,0.630938140511888,
57.2222894375664));
#113366=CARTESIAN_POINT('Ctrl Pts',(82.3346727961054,1.31739466653436,57.2050618631517));
#113367=CARTESIAN_POINT('Ctrl Pts',(82.1105250320151,2.34612040996873,57.2005733737953));
#113368=CARTESIAN_POINT('Ctrl Pts',(82.0116225514947,2.70113410021125,57.2046642839492));
#113369=CARTESIAN_POINT('Ctrl Pts',(81.8983892080076,3.04138126515041,57.2246303775219));
#113370=CARTESIAN_POINT('',(81.8983892080091,-3.04138126515099,57.22463037752));
#113371=CARTESIAN_POINT('Origin',(73.0351194308991,1.4210854715202E-14,
58.78746397652));
#113372=CARTESIAN_POINT('Ctrl Pts',(81.8983892080076,-3.04138126515039,
57.2246303775219));
#113373=CARTESIAN_POINT('Ctrl Pts',(82.0116225514947,-2.70113410021123,
57.2046642839493));
#113374=CARTESIAN_POINT('Ctrl Pts',(82.1105250320151,-2.34612040996872,
57.2005733737953));
#113375=CARTESIAN_POINT('Ctrl Pts',(82.3346727961054,-1.31739466653435,
57.2050618631517));
#113376=CARTESIAN_POINT('Ctrl Pts',(82.4056897430765,-0.630938140511861,
57.2222894375664));
#113377=CARTESIAN_POINT('Ctrl Pts',(82.4056897430765,1.36696209906972E-14,
57.2222894375664));
#113378=CARTESIAN_POINT('Origin',(74.1638325857391,1.4210854715202E-14,
65.188714371101));
#113379=CARTESIAN_POINT('',(82.1915345300951,-0.411812550483981,63.2655006193781));
#113380=CARTESIAN_POINT('Origin',(74.0770084969191,1.4210854715202E-14,
64.696310494688));
#113381=CARTESIAN_POINT('',(81.7865781657935,-0.386854671015844,63.8446186582614));
#113382=CARTESIAN_POINT('Origin',(82.2783682032164,-0.411813036887835,63.7579028058202));
#113383=CARTESIAN_POINT('',(81.7960926715764,1.51599559845412E-14,63.8429409941838));
#113384=CARTESIAN_POINT('Origin',(74.1638325857391,1.4210854715202E-14,
65.188714371101));
#113385=CARTESIAN_POINT('Origin',(74.1638325857391,1.4210854715202E-14,
65.188714371101));
#113386=CARTESIAN_POINT('Origin',(71.6139524734691,1.4210854715202E-14,
50.72762564822));
#113387=CARTESIAN_POINT('',(82.0565649380767,1.51599559845412E-14,65.3201526237018));
#113388=CARTESIAN_POINT('',(79.2462125593138,1.51599559845412E-14,49.3818522713015));
#113389=CARTESIAN_POINT('Origin',(74.4243048522391,1.4210854715202E-14,
66.665926000619));
#113390=CARTESIAN_POINT('Origin',(71.6139524734691,1.4210854715202E-14,
50.72762564822));
#113391=CARTESIAN_POINT('',(80.8255552468114,1.50068751346478E-14,65.5372128457854));
#113392=CARTESIAN_POINT('Origin',(74.4243048522391,1.4210854715202E-14,
66.665926000619));
#113393=CARTESIAN_POINT('',(81.0860275133185,1.50068751346486E-14,67.0144244753021));
#113394=CARTESIAN_POINT('',(78.0152028680485,1.50068751346478E-14,49.5989124933851));
#113395=CARTESIAN_POINT('',(69.2683344771676,3.46410161513628,69.0982026073056));
#113396=CARTESIAN_POINT('Origin',(74.6847771187391,1.4210854715202E-14,
68.143137630137));
#113397=CARTESIAN_POINT('',(69.268334477169,-3.46410161513855,69.0982026073053));
#113398=CARTESIAN_POINT('Ctrl Pts',(69.2683344771665,-3.4641016151401,69.0982026073051));
#113399=CARTESIAN_POINT('Ctrl Pts',(68.9648321493424,-2.97479325737662,
69.1517182564088));
#113400=CARTESIAN_POINT('Ctrl Pts',(68.7289781639998,-2.41648059182673,
69.2912781361514));
#113401=CARTESIAN_POINT('Ctrl Pts',(68.4194117007815,-1.22911622864477,
69.5454817189857));
#113402=CARTESIAN_POINT('Ctrl Pts',(68.3498544259377,-0.596312598658473,
69.6480138742419));
#113403=CARTESIAN_POINT('Ctrl Pts',(68.3498544259377,0.5963125986585,69.6480138742419));
#113404=CARTESIAN_POINT('Ctrl Pts',(68.4194117007815,1.2291162286448,69.5454817189857));
#113405=CARTESIAN_POINT('Ctrl Pts',(68.7289781639996,2.41648059182585,69.2912781361516));
#113406=CARTESIAN_POINT('Ctrl Pts',(68.9648321493417,2.97479325737492,69.1517182564092));
#113407=CARTESIAN_POINT('Ctrl Pts',(69.2683344771651,3.46410161513784,69.0982026073054));
#113408=CARTESIAN_POINT('Origin',(74.6847771187391,1.4210854715202E-14,
68.143137630137));
#113409=CARTESIAN_POINT('Origin',(113.044794833869,1.4210854715202E-14,
71.158082873799));
#113410=CARTESIAN_POINT('',(118.579168886261,-8.01332830629138,69.4281578533551));
#113411=CARTESIAN_POINT('',(118.579167675758,8.01332909152356,69.4281576180553));
#113412=CARTESIAN_POINT('Origin',(113.570314823169,1.4210854715202E-14,
68.454530393505));
#113413=CARTESIAN_POINT('',(113.836120912569,9.49997724965368,66.9781228011004));
#113414=CARTESIAN_POINT('Ctrl Pts',(113.836120912568,9.49997724965366,66.9781228011068));
#113415=CARTESIAN_POINT('Ctrl Pts',(114.686038635719,9.50187211507081,67.1433308953068));
#113416=CARTESIAN_POINT('Ctrl Pts',(115.610633133812,9.38050971532904,67.4594549710188));
#113417=CARTESIAN_POINT('Ctrl Pts',(117.387516977032,8.79824955495792,68.2752003940439));
#113418=CARTESIAN_POINT('Ctrl Pts',(118.027127690967,8.42218281811796,68.6679459525273));
#113419=CARTESIAN_POINT('Ctrl Pts',(118.418563176045,8.156345641126,69.0448344935117));
#113420=CARTESIAN_POINT('Ctrl Pts',(118.489716706812,8.10440527523949,69.1261923172504));
#113421=CARTESIAN_POINT('Ctrl Pts',(118.553353478955,8.05159245557175,69.2438470494525));
#113422=CARTESIAN_POINT('Ctrl Pts',(118.56938447916,8.03708381445878,69.2821462693244));
#113423=CARTESIAN_POINT('Ctrl Pts',(118.581302967088,8.02269597530884,69.3399573591882));
#113424=CARTESIAN_POINT('Ctrl Pts',(118.583467017461,8.01916164376496,69.3579848864792));
#113425=CARTESIAN_POINT('Ctrl Pts',(118.583973829246,8.01451405680058,69.3936861214022));
#113426=CARTESIAN_POINT('Ctrl Pts',(118.582509524538,8.01332909160475,69.4109653817901));
#113427=CARTESIAN_POINT('Ctrl Pts',(118.579167675665,8.01332909160488,69.4281576180372));
#113428=CARTESIAN_POINT('',(104.531073144128,1.53742691743937E-14,65.1693957133202));
#113429=CARTESIAN_POINT('Origin',(113.856529692569,1.4210854715202E-14,
66.982089885856));
#113430=CARTESIAN_POINT('',(105.008097926387,1.5374269174392E-14,62.7153282005846));
#113431=CARTESIAN_POINT('',(103.719338285428,1.5374269174392E-14,69.3453887012632));
#113432=CARTESIAN_POINT('Origin',(114.333554474769,1.4210854715202E-14,
64.528022373109));
#113433=CARTESIAN_POINT('',(113.83612107687,-9.49997725001998,66.9781228330329));
#113434=CARTESIAN_POINT('Origin',(113.856529692569,1.4210854715202E-14,
66.982089885856));
#113435=CARTESIAN_POINT('Ctrl Pts',(118.579168886168,-8.01332830637214,
69.428157853337));
#113436=CARTESIAN_POINT('Ctrl Pts',(118.583697953965,-8.01332830637242,
69.4048579356841));
#113437=CARTESIAN_POINT('Ctrl Pts',(118.584755128007,-8.01550606099109,
69.3815157842115));
#113438=CARTESIAN_POINT('Ctrl Pts',(118.58079181303,-8.02388189771212,69.3327838467339));
#113439=CARTESIAN_POINT('Ctrl Pts',(118.575268672964,-8.03030115604168,
69.3081184208139));
#113440=CARTESIAN_POINT('Ctrl Pts',(118.550114989685,-8.05509816333799,
69.2312409077683));
#113441=CARTESIAN_POINT('Ctrl Pts',(118.519917693981,-8.07983477899803,
69.1790179082443));
#113442=CARTESIAN_POINT('Ctrl Pts',(118.365671255634,-8.19683130407594,
68.9686926024889));
#113443=CARTESIAN_POINT('Ctrl Pts',(118.148405235818,-8.34221746197395,
68.7907241087155));
#113444=CARTESIAN_POINT('Ctrl Pts',(117.411981582031,-8.75017745982984,
68.3043581295628));
#113445=CARTESIAN_POINT('Ctrl Pts',(116.685780703193,-9.08337727457682,
67.9164630081501));
#113446=CARTESIAN_POINT('Ctrl Pts',(115.095330683893,-9.4415653031523,67.2939793018252));
#113447=CARTESIAN_POINT('Ctrl Pts',(114.445102020103,-9.50133494336816,
67.0964973277519));
#113448=CARTESIAN_POINT('Ctrl Pts',(113.83612107687,-9.49997725001994,66.9781228330337));
#113449=CARTESIAN_POINT('Origin',(113.044794833869,1.4210854715202E-14,
71.158082873799));
#113450=CARTESIAN_POINT('',(101.08158990599,1.58641278940509E-14,61.9520885489905));
#113451=CARTESIAN_POINT('Origin',(114.333554474769,1.4210854715202E-14,
64.528022373109));
#113452=CARTESIAN_POINT('',(102.016642645058,1.58641278940509E-14,57.1416832303295));
#113453=CARTESIAN_POINT('',(99.7928302650323,1.58641278940509E-14,68.5821490496692));
#113454=CARTESIAN_POINT('',(115.268607213821,13.5000000002585,59.71761705473));
#113455=CARTESIAN_POINT('Origin',(115.268607213895,1.4210854715202E-14,
59.7176170544594));
#113456=CARTESIAN_POINT('Origin',(115.268607213895,1.4210854715202E-14,
59.7176170544594));
#113457=CARTESIAN_POINT('Origin',(115.325809116069,6.8389738316912E-14,
59.42334024732));
#113458=CARTESIAN_POINT('',(115.383008995803,14.0995393124789,59.1290738447923));
#113459=CARTESIAN_POINT('',(115.325809116069,13.7997749560101,59.42334024732));
#113460=CARTESIAN_POINT('Origin',(115.383008995752,2.51354492775102E-13,
59.1290738450566));
#113461=CARTESIAN_POINT('Origin',(113.044794833869,1.4210854715202E-14,
71.158082873799));
#113462=CARTESIAN_POINT('',(101.149417421836,1.59865925739657E-14,56.3623301080323));
#113463=CARTESIAN_POINT('Origin',(115.383008995769,1.4210854715202E-14,
59.12907384506));
#113464=CARTESIAN_POINT('',(102.198871764054,1.59865925739657E-14,50.9633824994358));
#113465=CARTESIAN_POINT('',(98.8112032599333,1.59865925739657E-14,68.3913391367707));
#113466=CARTESIAN_POINT('Origin',(116.432463337969,1.4210854715202E-14,
53.73012623646));
#113467=CARTESIAN_POINT('Origin',(71.6139524734691,1.4210854715202E-14,
50.72762564822));
#113468=CARTESIAN_POINT('',(84.0425654467451,1.50987236445838E-14,79.4627064438384));
#113469=CARTESIAN_POINT('Origin',(76.9027092374091,1.4210854715202E-14,
80.721655731923));
#113470=CARTESIAN_POINT('',(84.4766854941234,2.43409355081298E-8,81.924725896327));
#113471=CARTESIAN_POINT('',(78.7538086828077,1.50987236445838E-14,49.4686763601349));
#113472=CARTESIAN_POINT('',(84.4100541385791,0.934521241357814,81.895304371373));
#113473=CARTESIAN_POINT('Origin',(76.7759739330123,0.0982566280424606,78.5297174321831));
#113474=CARTESIAN_POINT('',(70.2495245506391,0.934521077365814,84.39218780804));
#113475=CARTESIAN_POINT('Ctrl Pts',(70.2495245506391,0.934521077365814,
84.39218780804));
#113476=CARTESIAN_POINT('Ctrl Pts',(70.2969934017684,1.35358127369409,84.3467359130793));
#113477=CARTESIAN_POINT('Ctrl Pts',(70.4869050838629,2.32787641859955,84.1880974727865));
#113478=CARTESIAN_POINT('Ctrl Pts',(71.0685341933312,3.76636998723846,83.7654733575445));
#113479=CARTESIAN_POINT('Ctrl Pts',(72.0301843466196,5.12897761292657,83.1528274066478));
#113480=CARTESIAN_POINT('Ctrl Pts',(73.2668101124888,6.19715034366626,82.4884313637663));
#113481=CARTESIAN_POINT('Ctrl Pts',(74.6880725700381,6.91163507431541,81.8874154360421));
#113482=CARTESIAN_POINT('Ctrl Pts',(76.21258020475,7.26357978151313,81.4299948820006));
#113483=CARTESIAN_POINT('Ctrl Pts',(77.7886661372182,7.26412555002382,81.1517875118529));
#113484=CARTESIAN_POINT('Ctrl Pts',(79.3787551980435,6.91301445740564,81.0596077375714));
#113485=CARTESIAN_POINT('Ctrl Pts',(80.9222078782584,6.19827430998822,81.1380989555079));
#113486=CARTESIAN_POINT('Ctrl Pts',(82.3132368783365,5.12885137030863,81.3397449855469));
#113487=CARTESIAN_POINT('Ctrl Pts',(83.4269049429719,3.7650811278669,81.5867141627659));
#113488=CARTESIAN_POINT('Ctrl Pts',(84.1174814320447,2.3269000879036,81.7848112655805));
#113489=CARTESIAN_POINT('Ctrl Pts',(84.3499684922177,1.35312292207528,81.868858277333));
#113490=CARTESIAN_POINT('Ctrl Pts',(84.4100541385791,0.934521241357814,
81.895304371373));
#113491=CARTESIAN_POINT('',(70.1969737837932,-2.46875951473559E-8,84.4426243475923));
#113492=CARTESIAN_POINT('Origin',(77.2332453430234,0.0370024116887719,77.698216590392));
#113493=CARTESIAN_POINT('',(70.2495210701591,-0.934521544955186,84.39218841976));
#113494=CARTESIAN_POINT('Origin',(76.207146622872,-0.102456625673098,78.6809209731816));
#113495=CARTESIAN_POINT('',(84.4100566843091,-0.934521571518686,81.895303921756));
#113496=CARTESIAN_POINT('Ctrl Pts',(84.4100566843091,-0.934521571518686,
81.895303921756));
#113497=CARTESIAN_POINT('Ctrl Pts',(84.3485694403728,-1.36293966038387,
81.868236180679));
#113498=CARTESIAN_POINT('Ctrl Pts',(84.1118115437881,-2.3450231478546,81.7828932767119));
#113499=CARTESIAN_POINT('Ctrl Pts',(83.4124450771603,-3.78704013149007,
81.5830498021844));
#113500=CARTESIAN_POINT('Ctrl Pts',(82.2982972025616,-5.14249136537986,
81.3370657981871));
#113501=CARTESIAN_POINT('Ctrl Pts',(80.9114749651663,-6.20390890762343,
81.1372668611484));
#113502=CARTESIAN_POINT('Ctrl Pts',(79.3752681809786,-6.91362667787633,
81.0598653963965));
#113503=CARTESIAN_POINT('Ctrl Pts',(77.7914654251769,-7.26346845250041,
81.1516464342562));
#113504=CARTESIAN_POINT('Ctrl Pts',(76.2200481462661,-7.26409591671058,
81.4283837861607));
#113505=CARTESIAN_POINT('Ctrl Pts',(74.698991450041,-6.91521469606571,81.8835971817274));
#113506=CARTESIAN_POINT('Ctrl Pts',(73.2794043860132,-6.2052646895131,82.4824234380684));
#113507=CARTESIAN_POINT('Ctrl Pts',(72.0428187684898,-5.14252677561984,
83.1454232256136));
#113508=CARTESIAN_POINT('Ctrl Pts',(71.0795152379404,-3.78584032635307,
83.758011848655));
#113509=CARTESIAN_POINT('Ctrl Pts',(70.4910989582979,-2.34409180177857,
84.1847388290923));
#113510=CARTESIAN_POINT('Ctrl Pts',(70.2979924693142,-1.36249704964592,
84.3457715729416));
#113511=CARTESIAN_POINT('Ctrl Pts',(70.2495210701591,-0.934521544955186,
84.39218841976));
#113512=CARTESIAN_POINT('Origin',(76.0757054979363,-0.0613886712863647,
78.2217740086092));
#113513=CARTESIAN_POINT('Origin',(76.8158851485791,1.4210854715202E-14,
80.229251855417));
#113514=CARTESIAN_POINT('',(83.2171355431526,1.50068751346478E-14,79.1005387005832));
#113515=CARTESIAN_POINT('',(83.2046721647582,-0.405417357723799,79.1027363304649));
#113516=CARTESIAN_POINT('Origin',(76.8158851485791,1.4210854715202E-14,
80.229251855417));
#113517=CARTESIAN_POINT('Origin',(76.8158851485791,1.4210854715202E-14,
80.229251855417));
#113518=CARTESIAN_POINT('',(83.7829335152822,-0.436602807422093,79.508486558344));
#113519=CARTESIAN_POINT('Origin',(83.6961173198489,-0.436603308317939,79.016081290084));
#113520=CARTESIAN_POINT('Origin',(76.9027092373991,1.4210854715202E-14,
80.72165573186));
#113521=CARTESIAN_POINT('Origin',(71.6139524734691,1.4210854715202E-14,
50.72762564822));
#113522=CARTESIAN_POINT('',(83.0434873654856,1.50068751346478E-14,78.1157309475707));
#113523=CARTESIAN_POINT('Origin',(76.6422369709091,1.4210854715202E-14,
79.244444102405));
#113524=CARTESIAN_POINT('',(78.0152028680485,1.50068751346478E-14,49.5989124933851));
#113525=CARTESIAN_POINT('Origin',(76.5901687245791,3.1641356201812E-14,
78.949150403589));
#113526=CARTESIAN_POINT('',(76.5380973908943,5.50000000026545,78.6538391955389));
#113527=CARTESIAN_POINT('',(81.9545400325016,1.4884410454733E-14,77.6987742186408));
#113528=CARTESIAN_POINT('Origin',(76.5380973909344,1.4210854715202E-14,
78.6538391958088));
#113529=CARTESIAN_POINT('',(76.6422369709602,6.09968496682694,79.2444441026693));
#113530=CARTESIAN_POINT('',(76.5901687245791,5.79985137262403,78.949150403589));
#113531=CARTESIAN_POINT('Origin',(76.6422369709134,3.1641356201812E-14,
79.2444441024043));
#113532=CARTESIAN_POINT('Origin',(76.5380973909344,1.4210854715202E-14,
78.6538391958088));
#113533=CARTESIAN_POINT('Origin',(71.6139524734691,1.4210854715202E-14,
50.72762564822));
#113534=CARTESIAN_POINT('',(70.6108044793244,-6.69216074262907E-7,76.7117291756247));
#113535=CARTESIAN_POINT('',(81.443689908106,1.4884410454733E-14,74.8015991956061));
#113536=CARTESIAN_POINT('Origin',(76.0272472665391,1.4210854715202E-14,
75.756664172774));
#113537=CARTESIAN_POINT('Origin',(76.0272472665391,1.4210854715202E-14,
75.756664172774));
#113538=CARTESIAN_POINT('',(77.0303951150363,1.4884410454733E-14,49.772560671052));
#113539=CARTESIAN_POINT('Origin',(77.1089102519491,1.4210854715202E-14,
81.89107979688));
#113540=CARTESIAN_POINT('',(85.978205710623,0.538566788587397,77.5711572248142));
#113541=CARTESIAN_POINT('',(85.9781969325309,-0.538566277248559,77.5711587732182));
#113542=CARTESIAN_POINT('Origin',(76.9466693241,0.0139589647788434,66.7387412315728));
#113543=CARTESIAN_POINT('',(83.8031819186193,-5.65795202609479,75.9086537965711));
#113544=CARTESIAN_POINT('Ctrl Pts',(85.978196932531,-0.538566277248559,
77.5711587732182));
#113545=CARTESIAN_POINT('Ctrl Pts',(85.9662144643982,-0.701937597578064,
77.5567675886209));
#113546=CARTESIAN_POINT('Ctrl Pts',(85.9493237206406,-0.865436116456894,
77.5389549030835));
#113547=CARTESIAN_POINT('Ctrl Pts',(85.9275097219851,-1.02884991082947,
77.5177470062622));
#113548=CARTESIAN_POINT('Ctrl Pts',(85.9061196526422,-1.18908795101694,
77.4969512598799));
#113549=CARTESIAN_POINT('Ctrl Pts',(85.8799956734439,-1.34924507627592,
77.4728908186415));
#113550=CARTESIAN_POINT('Ctrl Pts',(85.8490864021384,-1.50909866089878,
77.4455664203364));
#113551=CARTESIAN_POINT('Ctrl Pts',(85.8368899917902,-1.57217487820617,
77.4347845558611));
#113552=CARTESIAN_POINT('Ctrl Pts',(85.8239481131521,-1.63520353641687,
77.4234942417378));
#113553=CARTESIAN_POINT('Ctrl Pts',(85.8102560443249,-1.69816965667799,
77.411694547642));
#113554=CARTESIAN_POINT('Ctrl Pts',(85.8027877437963,-1.73251435032291,
77.4052584376016));
#113555=CARTESIAN_POINT('Ctrl Pts',(85.7950962355473,-1.76684042190365,
77.3986707699566));
#113556=CARTESIAN_POINT('Ctrl Pts',(85.7871816196228,-1.80114691080217,
77.391932216887));
#113557=CARTESIAN_POINT('Ctrl Pts',(85.7463561667131,-1.97810786006311,
77.357173173157));
#113558=CARTESIAN_POINT('Ctrl Pts',(85.6995993200506,-2.15452400245472,
77.3183956868117));
#113559=CARTESIAN_POINT('Ctrl Pts',(85.6469330932711,-2.33010254807959,
77.2755957751522));
#113560=CARTESIAN_POINT('Ctrl Pts',(85.6372258054953,-2.36246468172528,
77.2677070182644));
#113561=CARTESIAN_POINT('Ctrl Pts',(85.6273177557924,-2.39479821740101,
77.2596816108375));
#113562=CARTESIAN_POINT('Ctrl Pts',(85.6172090817812,-2.42710112678368,
77.2515195341207));
#113563=CARTESIAN_POINT('Ctrl Pts',(85.5847327845844,-2.53088119569059,
77.225297100901));
#113564=CARTESIAN_POINT('Ctrl Pts',(85.5501853982468,-2.63434715539312,
77.1976640345017));
#113565=CARTESIAN_POINT('Ctrl Pts',(85.5135688065919,-2.73743563372485,
77.1686200026685));
#113566=CARTESIAN_POINT('Ctrl Pts',(85.4952605107644,-2.78897987289072,
77.1540979867519));
#113567=CARTESIAN_POINT('Ctrl Pts',(85.4764348763288,-2.84042973404583,
77.1392232360841));
#113568=CARTESIAN_POINT('Ctrl Pts',(85.4570919373216,-2.89177709254335,
77.123995744836));
#113569=CARTESIAN_POINT('Ctrl Pts',(85.4474204678179,-2.91745077179212,
77.1163819992119));
#113570=CARTESIAN_POINT('Ctrl Pts',(85.4376196696253,-2.94309882414378,
77.1086800688932));
#113571=CARTESIAN_POINT('Ctrl Pts',(85.4276895322232,-2.96872022216433,
77.1008899557592));
#113572=CARTESIAN_POINT('Ctrl Pts',(85.4210724538229,-2.98579337962055,
77.0956989108353));
#113573=CARTESIAN_POINT('Ctrl Pts',(85.4147180597581,-3.00203887736141,
77.0907195487122));
#113574=CARTESIAN_POINT('Ctrl Pts',(85.407988054798,-3.01908814644679,77.085451494958));
#113575=CARTESIAN_POINT('Ctrl Pts',(85.4046184553818,-3.02762442650873,
77.0828138697319));
#113576=CARTESIAN_POINT('Ctrl Pts',(85.4011541048568,-3.03636190537531,
77.0801034885673));
#113577=CARTESIAN_POINT('Ctrl Pts',(85.3975110815366,-3.04550341715496,
77.0772550716083));
#113578=CARTESIAN_POINT('Ctrl Pts',(85.3695874993951,-3.11557262413956,
77.0554221054331));
#113579=CARTESIAN_POINT('Ctrl Pts',(85.3405734858181,-3.18574621766199,
77.0328615317925));
#113580=CARTESIAN_POINT('Ctrl Pts',(85.3104477713276,-3.25598520087038,
77.0095630573215));
#113581=CARTESIAN_POINT('Ctrl Pts',(85.2480342703271,-3.40150410134786,
76.9612940159294));
#113582=CARTESIAN_POINT('Ctrl Pts',(85.1808476668105,-3.54730551159,76.9098558683555));
#113583=CARTESIAN_POINT('Ctrl Pts',(85.108723733047,-3.69312705963221,76.8552039801537));
#113584=CARTESIAN_POINT('Ctrl Pts',(85.0382641434063,-3.83558360491052,
76.8018132481892));
#113585=CARTESIAN_POINT('Ctrl Pts',(84.9630922540674,-3.97805940335467,
76.7453552101207));
#113586=CARTESIAN_POINT('Ctrl Pts',(84.8830768863397,-4.12027618953755,
76.6858154420667));
#113587=CARTESIAN_POINT('Ctrl Pts',(84.805813877074,-4.25760102076219,76.6283237153962));
#113588=CARTESIAN_POINT('Ctrl Pts',(84.7240347343763,-4.3946843146335,76.5679585237037));
#113589=CARTESIAN_POINT('Ctrl Pts',(84.6376444659376,-4.53124394110661,
76.5047344232751));
#113590=CARTESIAN_POINT('Ctrl Pts',(84.5694971390091,-4.63896641585609,
76.4548612891879));
#113591=CARTESIAN_POINT('Ctrl Pts',(84.498480915318,-4.74636245394866,76.4032096693207));
#113592=CARTESIAN_POINT('Ctrl Pts',(84.42456079498,-4.85327902986735,76.3498001953486));
#113593=CARTESIAN_POINT('Ctrl Pts',(84.3281244473085,-4.99276262432044,
76.2801220809546));
#113594=CARTESIAN_POINT('Ctrl Pts',(84.226745450638,-5.13142992615831,76.2074506944152));
#113595=CARTESIAN_POINT('Ctrl Pts',(84.1202967047771,-5.26902674736115,
76.1318569723351));
#113596=CARTESIAN_POINT('Ctrl Pts',(84.0191960638591,-5.39971054921692,
76.0600611640343));
#113597=CARTESIAN_POINT('Ctrl Pts',(83.9135222658985,-5.52942861474292,
75.9856293087662));
#113598=CARTESIAN_POINT('Ctrl Pts',(83.8031865951727,-5.6579465788927,75.9086570590228));
#113599=CARTESIAN_POINT('',(83.8031578769549,5.65797623157721,75.9086520659686));
#113600=CARTESIAN_POINT('Origin',(76.2877195330491,1.4210854715202E-14,
77.233875802293));
#113601=CARTESIAN_POINT('Ctrl Pts',(83.8031631996716,5.65797003185228,75.9086557791601));
#113602=CARTESIAN_POINT('Ctrl Pts',(83.9146383767883,5.52812731488565,75.9864222198002));
#113603=CARTESIAN_POINT('Ctrl Pts',(84.0213782518127,5.39701190664906,76.0615222181351));
#113604=CARTESIAN_POINT('Ctrl Pts',(84.1234507304318,5.26489792169313,76.1339017634367));
#113605=CARTESIAN_POINT('Ctrl Pts',(84.2274634112329,5.13027270309868,76.2076571051687));
#113606=CARTESIAN_POINT('Ctrl Pts',(84.3266296801952,4.994610790924,76.2785877161089));
#113607=CARTESIAN_POINT('Ctrl Pts',(84.4210534082592,4.85818561965194,76.3466763826821));
#113608=CARTESIAN_POINT('Ctrl Pts',(84.4310223939351,4.8437822423851,76.3538649882972));
#113609=CARTESIAN_POINT('Ctrl Pts',(84.4409385446514,4.82937034077388,76.3610219510471));
#113610=CARTESIAN_POINT('Ctrl Pts',(84.4508020021065,4.81495022461278,76.3681472750928));
#113611=CARTESIAN_POINT('Ctrl Pts',(84.5395416903718,4.68521512728899,76.4322524874367));
#113612=CARTESIAN_POINT('Ctrl Pts',(84.6240136534749,4.55481766585984,76.4937943659752));
#113613=CARTESIAN_POINT('Ctrl Pts',(84.7042816981499,4.42405601459424,76.5527860260094));
#113614=CARTESIAN_POINT('Ctrl Pts',(84.7164642319641,4.40420990716007,76.5617393759512));
#113615=CARTESIAN_POINT('Ctrl Pts',(84.7285499856946,4.38435535298269,76.5706340353276));
#113616=CARTESIAN_POINT('Ctrl Pts',(84.7405392429994,4.36449333269502,76.5794701069808));
#113617=CARTESIAN_POINT('Ctrl Pts',(84.8272353310484,4.22086813424354,76.6433650444714));
#113618=CARTESIAN_POINT('Ctrl Pts',(84.9089044311266,4.07680745468572,76.7041670189899));
#113619=CARTESIAN_POINT('Ctrl Pts',(84.9856720925189,3.93260490356097,76.7618449210903));
#113620=CARTESIAN_POINT('Ctrl Pts',(85.0260284014314,3.8567984690074,76.7921658556136));
#113621=CARTESIAN_POINT('Ctrl Pts',(85.0650305614148,3.7809521898354,76.8216239761702));
#113622=CARTESIAN_POINT('Ctrl Pts',(85.1026991261737,3.70510470472398,76.8502180733543));
#113623=CARTESIAN_POINT('Ctrl Pts',(85.1573608628283,3.59504064245878,76.8917116375544));
#113624=CARTESIAN_POINT('Ctrl Pts',(85.2092130179194,3.48497576389758,76.9313826789799));
#113625=CARTESIAN_POINT('Ctrl Pts',(85.2583185901418,3.37502563477719,76.9692200894284));
#113626=CARTESIAN_POINT('Ctrl Pts',(85.2814644688194,3.32320071483382,76.987054727578));
#113627=CARTESIAN_POINT('Ctrl Pts',(85.3040001456757,3.27140131321668,77.0044819961335));
#113628=CARTESIAN_POINT('Ctrl Pts',(85.3259325406226,3.21963888336876,77.0215006470104));
#113629=CARTESIAN_POINT('Ctrl Pts',(85.3272656872237,3.21649253717243,77.0225351148205));
#113630=CARTESIAN_POINT('Ctrl Pts',(85.3285966049385,3.21334632746294,77.0235680730266));
#113631=CARTESIAN_POINT('Ctrl Pts',(85.3299252954779,3.21020025792908,77.0245995217025));
#113632=CARTESIAN_POINT('Ctrl Pts',(85.3415191835484,3.1827482840084,77.0335997366838));
#113633=CARTESIAN_POINT('Ctrl Pts',(85.3529435118309,3.15530692758353,77.0424849792601));
#113634=CARTESIAN_POINT('Ctrl Pts',(85.3641995909304,3.12787797423294,77.051255018393));
#113635=CARTESIAN_POINT('Ctrl Pts',(85.371631741544,3.10976721731019,77.0570456894736));
#113636=CARTESIAN_POINT('Ctrl Pts',(85.3793140484198,3.09086332054833,77.0630385222237));
#113637=CARTESIAN_POINT('Ctrl Pts',(85.3866042826731,3.07274766257864,77.0687323546987));
#113638=CARTESIAN_POINT('Ctrl Pts',(85.3903551935305,3.06342694450479,77.0716618981549));
#113639=CARTESIAN_POINT('Ctrl Pts',(85.394003006187,3.05431525216176,77.0745127386788));
#113640=CARTESIAN_POINT('Ctrl Pts',(85.3974643703546,3.04563007803897,77.0772192980654));
#113641=CARTESIAN_POINT('Ctrl Pts',(85.4649143560354,2.87638614939062,77.1299607557767));
#113642=CARTESIAN_POINT('Ctrl Pts',(85.5266941417952,2.7059554568368,77.1788836210702));
#113643=CARTESIAN_POINT('Ctrl Pts',(85.5828053059658,2.5346255676035,77.2239545594196));
#113644=CARTESIAN_POINT('Ctrl Pts',(85.6402207568679,2.35931316785643,77.2700731578513));
#113645=CARTESIAN_POINT('Ctrl Pts',(85.6917014501738,2.18305900250801,77.3121590342264));
#113646=CARTESIAN_POINT('Ctrl Pts',(85.7372343351277,2.00611866949535,77.3501710657188));
#113647=CARTESIAN_POINT('Ctrl Pts',(85.7663710211512,1.89289380063139,77.3744951257435));
#113648=CARTESIAN_POINT('Ctrl Pts',(85.793071895714,1.77938691442686,77.3971509120166));
#113649=CARTESIAN_POINT('Ctrl Pts',(85.8173291550407,1.66565496084234,77.418125491269));
#113650=CARTESIAN_POINT('Ctrl Pts',(85.8528280677087,1.49921568452159,77.4488204163263));
#113651=CARTESIAN_POINT('Ctrl Pts',(85.8830952727907,1.33229650434879,77.4759159598019));
#113652=CARTESIAN_POINT('Ctrl Pts',(85.9081981255997,1.16521709143556,77.4994608635661));
#113653=CARTESIAN_POINT('Ctrl Pts',(85.9337966630433,0.994838503788336,
77.5234706884732));
#113654=CARTESIAN_POINT('Ctrl Pts',(85.9540251498616,0.824292838675683,
77.54378844342));
#113655=CARTESIAN_POINT('Ctrl Pts',(85.9689234471876,0.653880651746717,
77.5604450953023));
#113656=CARTESIAN_POINT('Ctrl Pts',(85.9722845858547,0.61543471538934,77.5642029285285));
#113657=CARTESIAN_POINT('Ctrl Pts',(85.9753742950457,0.576995436892595,
77.5677743312878));
#113658=CARTESIAN_POINT('Ctrl Pts',(85.9781927942916,0.538566041923533,
77.5711595027625));
#113659=CARTESIAN_POINT('Origin',(27.4324635166691,25.,72.98888938658));
#113660=CARTESIAN_POINT('',(-7.08815755044579,5.,58.3404518883124));
#113661=CARTESIAN_POINT('',(-8.23395173885291,5.,84.57149802283));
#113662=CARTESIAN_POINT('Origin',(27.4324635166691,5.,72.98888938658));
#113663=CARTESIAN_POINT('',(-8.23395173885291,-5.,84.57149802283));
#113664=CARTESIAN_POINT('',(-8.23395173890591,5.,84.57149802267));
#113665=CARTESIAN_POINT('',(-7.08815755044587,-5.,58.3404518883126));
#113666=CARTESIAN_POINT('Origin',(27.4324635166691,-5.,72.98888938658));
#113667=CARTESIAN_POINT('',(-7.08815755167191,-5.,58.3404518912));
#113668=CARTESIAN_POINT('Origin',(20.5162416486691,1.37771738462078E-14,
116.353388269));
#113669=CARTESIAN_POINT('Ctrl Pts',(20.8449496767831,16.375,118.217584317867));
#113670=CARTESIAN_POINT('Ctrl Pts',(20.560377721845,16.3749999994318,118.271191799454));
#113671=CARTESIAN_POINT('Ctrl Pts',(20.2758436122818,16.3673196851251,118.324851280152));
#113672=CARTESIAN_POINT('Ctrl Pts',(19.3903453687992,16.3194739703247,118.491914823905));
#113673=CARTESIAN_POINT('Ctrl Pts',(18.7913279623376,16.2526679348737,118.605012536406));
#113674=CARTESIAN_POINT('Ctrl Pts',(17.5039222623931,16.034160127074,118.847913184993));
#113675=CARTESIAN_POINT('Ctrl Pts',(16.8187606642767,15.8703432356303,118.977067391609));
#113676=CARTESIAN_POINT('Ctrl Pts',(15.7576475272096,15.5407174414681,119.177219354591));
#113677=CARTESIAN_POINT('Ctrl Pts',(15.3735955108468,15.4050337240163,119.249698536666));
#113678=CARTESIAN_POINT('Ctrl Pts',(14.6265437499547,15.1083739087842,119.39098027536));
#113679=CARTESIAN_POINT('Ctrl Pts',(14.2635181721422,14.9482691083237,119.459816635334));
#113680=CARTESIAN_POINT('Ctrl Pts',(13.3665414482046,14.5120054500825,119.630222584242));
#113681=CARTESIAN_POINT('Ctrl Pts',(12.8412688288321,14.2188161913186,119.730266696678));
#113682=CARTESIAN_POINT('Ctrl Pts',(11.7784055359248,13.5444528029723,119.932919961903));
#113683=CARTESIAN_POINT('Ctrl Pts',(11.2451441103364,13.1582815993812,120.034719152112));
#113684=CARTESIAN_POINT('Ctrl Pts',(10.3987038222404,12.462464869475,120.196770206009));
#113685=CARTESIAN_POINT('Ctrl Pts',(10.0721152976126,12.1709707006107,120.259433153701));
#113686=CARTESIAN_POINT('Ctrl Pts',(9.45411172552166,11.5725544403491,120.378549735947));
#113687=CARTESIAN_POINT('Ctrl Pts',(9.16210718307875,11.2667712606362,120.435142432012));
#113688=CARTESIAN_POINT('Ctrl Pts',(8.47984509519864,10.4939970519773,120.568028493558));
#113689=CARTESIAN_POINT('Ctrl Pts',(8.10301362456274,10.0156082338631,120.641951418667));
#113690=CARTESIAN_POINT('Ctrl Pts',(7.34591246341852,8.93528959929101,120.791338336788));
#113691=CARTESIAN_POINT('Ctrl Pts',(6.97625508631526,8.32719027346426,120.864852016916));
#113692=CARTESIAN_POINT('Ctrl Pts',(6.45599262264532,7.33083168892778,120.969636114732));
#113693=CARTESIAN_POINT('Ctrl Pts',(6.27881899880134,6.95798344802511,121.005644436317));
#113694=CARTESIAN_POINT('Ctrl Pts',(5.95755041512535,6.21060783612537,121.071849577373));
#113695=CARTESIAN_POINT('Ctrl Pts',(5.81274808411848,5.83671191490872,121.102199809476));
#113696=CARTESIAN_POINT('Ctrl Pts',(5.48278908801904,4.88292384939799,121.172622486078));
#113697=CARTESIAN_POINT('Ctrl Pts',(5.31570887041526,4.29718792996188,121.209512719585));
#113698=CARTESIAN_POINT('Ctrl Pts',(5.03383788936494,3.05296609408649,121.274485762568));
#113699=CARTESIAN_POINT('Ctrl Pts',(4.92578521641382,2.39401992697441,121.301332717164));
#113700=CARTESIAN_POINT('Ctrl Pts',(4.81261148165586,1.2915016417281,121.334101978111));
#113701=CARTESIAN_POINT('Ctrl Pts',(4.78505336113655,0.85116335348093,121.344027614717));
#113702=CARTESIAN_POINT('Ctrl Pts',(4.76536842121233,-0.0168249872455496,
121.357643273541));
#113703=CARTESIAN_POINT('Ctrl Pts',(4.7721643660596,-0.444100963069227,
121.361559172694));
#113704=CARTESIAN_POINT('Ctrl Pts',(4.8287501723439,-1.48218942359855,121.364170012791));
#113705=CARTESIAN_POINT('Ctrl Pts',(4.89585438918724,-2.0914232995622,121.359808433127));
#113706=CARTESIAN_POINT('Ctrl Pts',(5.11402913302341,-3.4023682566261,121.337245585004));
#113707=CARTESIAN_POINT('Ctrl Pts',(5.27721183480348,-4.10075146847743,
121.316827709394));
#113708=CARTESIAN_POINT('Ctrl Pts',(5.60446279919227,-5.18060140277138,
121.272175811282));
#113709=CARTESIAN_POINT('Ctrl Pts',(5.7386430530597,-5.57038133211787,121.253264839852));
#113710=CARTESIAN_POINT('Ctrl Pts',(6.03249489152454,-6.33050202809045,
121.211006773134));
#113711=CARTESIAN_POINT('Ctrl Pts',(6.19145203607718,-6.70081947829591,
121.187815822064));
#113712=CARTESIAN_POINT('Ctrl Pts',(6.62359354871342,-7.61392061452341,
121.123866996895));
#113713=CARTESIAN_POINT('Ctrl Pts',(6.91342082458287,-8.1479497402729,121.080178706915));
#113714=CARTESIAN_POINT('Ctrl Pts',(7.57820509716986,-9.22626204269762,
120.978151358745));
#113715=CARTESIAN_POINT('Ctrl Pts',(7.95779022242495,-9.76633340359109,
120.918951563827));
#113716=CARTESIAN_POINT('Ctrl Pts',(8.6436636687758,-10.6268782169619,120.810792977168));
#113717=CARTESIAN_POINT('Ctrl Pts',(8.93249980583699,-10.9606327551128,
120.764957268814));
#113718=CARTESIAN_POINT('Ctrl Pts',(9.5236526191515,-11.5902362641935,120.670869569245));
#113719=CARTESIAN_POINT('Ctrl Pts',(9.82469433091606,-11.8868426097135,
120.622876156179));
#113720=CARTESIAN_POINT('Ctrl Pts',(10.5873244522212,-12.5818566432385,
120.500983008873));
#113721=CARTESIAN_POINT('Ctrl Pts',(11.0602699688564,-12.9664901615787,
120.425078437679));
#113722=CARTESIAN_POINT('Ctrl Pts',(12.1248222765698,-13.7369140406902,
120.253231628986));
#113723=CARTESIAN_POINT('Ctrl Pts',(12.7222049932059,-14.1123415385586,
120.156194743627));
#113724=CARTESIAN_POINT('Ctrl Pts',(13.7048000340426,-14.6434851446472,
119.995979681164));
#113725=CARTESIAN_POINT('Ctrl Pts',(14.0751201110258,-14.8256257622507,
119.935480783136));
#113726=CARTESIAN_POINT('Ctrl Pts',(14.813050602275,-15.15392143503,119.8149240473));
#113727=CARTESIAN_POINT('Ctrl Pts',(15.1798936674267,-15.3011443639482,
119.755027934311));
#113728=CARTESIAN_POINT('Ctrl Pts',(16.1203776478522,-15.6387948805931,
119.601426904445));
#113729=CARTESIAN_POINT('Ctrl Pts',(16.6999012936228,-15.8105439418231,
119.506691369404));
#113730=CARTESIAN_POINT('Ctrl Pts',(17.936785303593,-16.1021212889422,119.303982023674));
#113731=CARTESIAN_POINT('Ctrl Pts',(18.5947437481837,-16.2143268134127,
119.195850610668));
#113732=CARTESIAN_POINT('Ctrl Pts',(19.687203546909,-16.3308560109771,119.016084384859));
#113733=CARTESIAN_POINT('Ctrl Pts',(20.1184051367867,-16.3592035165354,
118.94508023839));
#113734=CARTESIAN_POINT('Ctrl Pts',(20.9746338980482,-16.380630176759,118.804246552665));
#113735=CARTESIAN_POINT('Ctrl Pts',(21.3993127608701,-16.3742972727923,
118.734517544012));
#113736=CARTESIAN_POINT('Ctrl Pts',(22.4247777142537,-16.3180078925996,
118.566303953469));
#113737=CARTESIAN_POINT('Ctrl Pts',(23.0240182250927,-16.2509343747199,
118.46808654998));
#113738=CARTESIAN_POINT('Ctrl Pts',(24.3244196987897,-16.0302753659217,
118.254778504253));
#113739=CARTESIAN_POINT('Ctrl Pts',(25.0220284027002,-15.8629945222672,
118.140225379743));
#113740=CARTESIAN_POINT('Ctrl Pts',(26.0886546236702,-15.5300690963237,
117.965220170735));
#113741=CARTESIAN_POINT('Ctrl Pts',(26.4664124402663,-15.3964168081272,
117.903278978449));
#113742=CARTESIAN_POINT('Ctrl Pts',(27.2168327898064,-15.0988355234507,
117.7805254849));
#113743=CARTESIAN_POINT('Ctrl Pts',(27.5890792034858,-14.9346004754354,
117.719823710413));
#113744=CARTESIAN_POINT('Ctrl Pts',(28.4920465230995,-14.4945467777078,
117.57289640398));
#113745=CARTESIAN_POINT('Ctrl Pts',(29.0145808915519,-14.2028410042795,
117.488114142301));
#113746=CARTESIAN_POINT('Ctrl Pts',(30.1677040854385,-13.4721703757075,
117.301251244048));
#113747=CARTESIAN_POINT('Ctrl Pts',(30.7858698634633,-13.0157853524169,
117.201229394986));
#113748=CARTESIAN_POINT('Ctrl Pts',(31.6508239602556,-12.276882594101,117.061942375504));
#113749=CARTESIAN_POINT('Ctrl Pts',(31.9235781977717,-12.0272962337938,
117.018139934069));
#113750=CARTESIAN_POINT('Ctrl Pts',(32.6685048727935,-11.2975278642344,
116.899101386167));
#113751=CARTESIAN_POINT('Ctrl Pts',(33.1200888948291,-10.7967905266924,
116.827755373074));
#113752=CARTESIAN_POINT('Ctrl Pts',(33.8995146291264,-9.81706586470456,
116.705574216279));
#113753=CARTESIAN_POINT('Ctrl Pts',(34.2352669512445,-9.34590300807752,
116.653342387818));
#113754=CARTESIAN_POINT('Ctrl Pts',(34.8931481542072,-8.31112175338087,
116.551834947782));
#113755=CARTESIAN_POINT('Ctrl Pts',(35.2082625859149,-7.744104661659,116.503744836743));
#113756=CARTESIAN_POINT('Ctrl Pts',(35.6897396189397,-6.74306729907632,
116.431728658734));
#113757=CARTESIAN_POINT('Ctrl Pts',(35.8726183337573,-6.31807756200283,
116.404892093368));
#113758=CARTESIAN_POINT('Ctrl Pts',(36.2794399424667,-5.25178640577539,
116.346872057103));
#113759=CARTESIAN_POINT('Ctrl Pts',(36.4822775238642,-4.60316262806885,
116.319429213635));
#113760=CARTESIAN_POINT('Ctrl Pts',(36.8951991037712,-2.92793855495885,
116.267347054293));
#113761=CARTESIAN_POINT('Ctrl Pts',(37.049006831098,-1.89034145061715,116.252247993329));
#113762=CARTESIAN_POINT('Ctrl Pts',(37.1267103121608,-0.420910239128301,
116.255589744507));
#113763=CARTESIAN_POINT('Ctrl Pts',(37.1328878516839,0.00402868902685441,
116.259479566599));
#113764=CARTESIAN_POINT('Ctrl Pts',(37.1066528453196,1.10928849771526,116.277385483572));
#113765=CARTESIAN_POINT('Ctrl Pts',(37.048743919782,1.78810410530278,116.295943789864));
#113766=CARTESIAN_POINT('Ctrl Pts',(36.8573145214258,3.08469646862634,116.345460736456));
#113767=CARTESIAN_POINT('Ctrl Pts',(36.7298396643764,3.7022014920466,116.375366743719));
#113768=CARTESIAN_POINT('Ctrl Pts',(36.4339114898637,4.81193811867991,116.440901050943));
#113769=CARTESIAN_POINT('Ctrl Pts',(36.2767924596985,5.3064543030832,116.474563704631));
#113770=CARTESIAN_POINT('Ctrl Pts',(35.94950740758,6.19025495266907,116.543289610683));
#113771=CARTESIAN_POINT('Ctrl Pts',(35.7870277847551,6.58200030310312,116.577005611126));
#113772=CARTESIAN_POINT('Ctrl Pts',(35.3498426650777,7.53095447632581,116.666765889529));
#113773=CARTESIAN_POINT('Ctrl Pts',(35.0584583250972,8.07946459542988,116.725750167534));
#113774=CARTESIAN_POINT('Ctrl Pts',(34.3446687704117,9.25671145535685,116.86817565282));
#113775=CARTESIAN_POINT('Ctrl Pts',(33.9084059099991,9.87507715868073,116.953951655212));
#113776=CARTESIAN_POINT('Ctrl Pts',(33.0537009768897,10.923666116097,117.120393299594));
#113777=CARTESIAN_POINT('Ctrl Pts',(32.6511232386463,11.3654519807241,117.198308385746));
#113778=CARTESIAN_POINT('Ctrl Pts',(31.9558880781184,12.0486275219986,117.332670334456));
#113779=CARTESIAN_POINT('Ctrl Pts',(31.6772079410402,12.3039234612902,117.386448701375));
#113780=CARTESIAN_POINT('Ctrl Pts',(30.8181950144664,13.0371387092337,117.551776378099));
#113781=CARTESIAN_POINT('Ctrl Pts',(30.2136188341809,13.4840967544494,117.667527990713));
#113782=CARTESIAN_POINT('Ctrl Pts',(29.0761869599664,14.2075608565754,117.884105131791));
#113783=CARTESIAN_POINT('Ctrl Pts',(28.5545753434907,14.4996912570987,117.983034196769));
#113784=CARTESIAN_POINT('Ctrl Pts',(27.6563439774672,14.9385818707944,118.153161433088));
#113785=CARTESIAN_POINT('Ctrl Pts',(27.2880615584285,15.1015661154573,118.222872926722));
#113786=CARTESIAN_POINT('Ctrl Pts',(26.5412221153119,15.3987943846171,118.364333736677));
#113787=CARTESIAN_POINT('Ctrl Pts',(26.1629504867174,15.533003030054,118.435990930457));
#113788=CARTESIAN_POINT('Ctrl Pts',(25.1012520068866,15.8650022450366,118.636906660495));
#113789=CARTESIAN_POINT('Ctrl Pts',(24.4092489289208,16.0313210680016,118.767601207822));
#113790=CARTESIAN_POINT('Ctrl Pts',(23.1164101485355,16.2513860974161,119.011190980202));
#113791=CARTESIAN_POINT('Ctrl Pts',(22.5190413259115,16.3183899512091,119.123531240596));
#113792=CARTESIAN_POINT('Ctrl Pts',(21.6309411126748,16.3670889161068,119.290604045939));
#113793=CARTESIAN_POINT('Ctrl Pts',(21.3421435866636,16.37500000057,119.344946631207));
#113794=CARTESIAN_POINT('Ctrl Pts',(21.0533274903535,16.375,119.399353621412));
#113795=CARTESIAN_POINT('Ctrl Pts',(21.0210448803799,16.375,119.216269433269));
#113796=CARTESIAN_POINT('Ctrl Pts',(21.2091318775354,16.3749999995409,119.180837725885));
#113797=CARTESIAN_POINT('Ctrl Pts',(21.3972151118309,16.3716448489046,119.145380652092));
#113798=CARTESIAN_POINT('Ctrl Pts',(22.129344463814,16.3455117717536,119.007303069283));
#113799=CARTESIAN_POINT('Ctrl Pts',(22.6721403186664,16.2980016429559,118.904821018823));
#113800=CARTESIAN_POINT('Ctrl Pts',(23.8478536836665,16.133620224497,118.682943650173));
#113801=CARTESIAN_POINT('Ctrl Pts',(24.4783842341807,16.0059662313511,118.564026140583));
#113802=CARTESIAN_POINT('Ctrl Pts',(25.677290186071,15.6863267000636,118.337952311273));
#113803=CARTESIAN_POINT('Ctrl Pts',(26.2459811391878,15.4997572265107,118.230729148814));
#113804=CARTESIAN_POINT('Ctrl Pts',(27.2265273202302,15.1155688019718,118.045336237119));
#113805=CARTESIAN_POINT('Ctrl Pts',(27.6428128347225,14.9315226080182,117.966394393069));
#113806=CARTESIAN_POINT('Ctrl Pts',(28.6151484541191,14.4508997439625,117.781617308589));
#113807=CARTESIAN_POINT('Ctrl Pts',(29.1628753749719,14.1386251308742,117.677270394425));
#113808=CARTESIAN_POINT('Ctrl Pts',(30.2121066950332,13.4554895657411,117.477160345643));
#113809=CARTESIAN_POINT('Ctrl Pts',(30.7132868775911,13.0860987775049,117.381461820497));
#113810=CARTESIAN_POINT('Ctrl Pts',(31.6902754071368,12.2746616878511,117.194364546538));
#113811=CARTESIAN_POINT('Ctrl Pts',(32.163404786753,11.8310500365806,117.103433365788));
#113812=CARTESIAN_POINT('Ctrl Pts',(32.8735132979374,11.080184408507,116.96574152817));
#113813=CARTESIAN_POINT('Ctrl Pts',(33.1280659380327,10.7910743327432,116.916135028231));
#113814=CARTESIAN_POINT('Ctrl Pts',(33.844073207513,9.91714487357266,116.77606015033));
#113815=CARTESIAN_POINT('Ctrl Pts',(34.2763750258454,9.30891627341975,116.6908063204));
#113816=CARTESIAN_POINT('Ctrl Pts',(34.9813230114452,8.15805333104755,116.550588458271));
#113817=CARTESIAN_POINT('Ctrl Pts',(35.2681430841832,7.62601541255148,116.493046851121));
#113818=CARTESIAN_POINT('Ctrl Pts',(35.6975270948211,6.71231056108483,116.405597429031));
#113819=CARTESIAN_POINT('Ctrl Pts',(35.856320222466,6.33922267043306,116.37284567988));
#113820=CARTESIAN_POINT('Ctrl Pts',(36.1471447701724,5.57924034963549,116.311793432552));
#113821=CARTESIAN_POINT('Ctrl Pts',(36.2788944480832,5.19254204154739,116.283582673026));
#113822=CARTESIAN_POINT('Ctrl Pts',(36.6027999168374,4.11232940312022,116.212765649901));
#113823=CARTESIAN_POINT('Ctrl Pts',(36.7643736529417,3.41025680340466,116.175628119676));
#113824=CARTESIAN_POINT('Ctrl Pts',(36.9779681886653,2.09643819954386,116.122359176686));
#113825=CARTESIAN_POINT('Ctrl Pts',(37.0426989224839,1.48813747162239,116.10393213763));
#113826=CARTESIAN_POINT('Ctrl Pts',(37.0955271601667,0.449603788305685,
116.082575680149));
#113827=CARTESIAN_POINT('Ctrl Pts',(37.1007337682424,0.0209528223131461,
116.076641323096));
#113828=CARTESIAN_POINT('Ctrl Pts',(37.0776801789711,-0.846849150257792,
116.070285431662));
#113829=CARTESIAN_POINT('Ctrl Pts',(37.0485748538665,-1.28563078188508,
116.070058690432));
#113830=CARTESIAN_POINT('Ctrl Pts',(36.9311891574028,-2.39022465940462,
116.077284079822));
#113831=CARTESIAN_POINT('Ctrl Pts',(36.8199178219872,-3.05274998811974,
116.088858437463));
#113832=CARTESIAN_POINT('Ctrl Pts',(36.5316502460197,-4.30112393281202,
116.124657868899));
#113833=CARTESIAN_POINT('Ctrl Pts',(36.3617472251379,-4.88750193079068,
116.147608578871));
#113834=CARTESIAN_POINT('Ctrl Pts',(36.0274823548541,-5.84086906357453,
116.19482981852));
#113835=CARTESIAN_POINT('Ctrl Pts',(35.8813462638261,-6.21375293713925,
116.215908008467));
#113836=CARTESIAN_POINT('Ctrl Pts',(35.5566013349731,-6.9612282755069,116.263389976612));
#113837=CARTESIAN_POINT('Ctrl Pts',(35.3771346186739,-7.33511832637184,
116.289979693107));
#113838=CARTESIAN_POINT('Ctrl Pts',(34.8520486261734,-8.33107956937099,
116.368880244316));
#113839=CARTESIAN_POINT('Ctrl Pts',(34.4801094096761,-8.93786897760451,
116.425908415246));
#113840=CARTESIAN_POINT('Ctrl Pts',(33.7181280802402,-10.0172495988322,
116.544727350233));
#113841=CARTESIAN_POINT('Ctrl Pts',(33.3385187776704,-10.4958789408354,
116.604630085464));
#113842=CARTESIAN_POINT('Ctrl Pts',(32.6520278465918,-11.2684074249856,
116.71364372183));
#113843=CARTESIAN_POINT('Ctrl Pts',(32.3586408904443,-11.573757717665,116.760388703545));
#113844=CARTESIAN_POINT('Ctrl Pts',(31.7369943050775,-12.1722093244503,
116.85957407915));
#113845=CARTESIAN_POINT('Ctrl Pts',(31.4080817467552,-12.4640999378746,
116.912172552455));
#113846=CARTESIAN_POINT('Ctrl Pts',(30.557667792781,-13.1592229908957,117.048700775769));
#113847=CARTESIAN_POINT('Ctrl Pts',(30.0229043823789,-13.5444910972657,
117.13503518517));
#113848=CARTESIAN_POINT('Ctrl Pts',(28.9564262533286,-14.2179993513951,
117.308152610967));
#113849=CARTESIAN_POINT('Ctrl Pts',(28.4289654111353,-14.5111092739633,
117.39416536399));
#113850=CARTESIAN_POINT('Ctrl Pts',(27.5278176717548,-14.9475578246718,
117.54133721563));
#113851=CARTESIAN_POINT('Ctrl Pts',(27.1627938609599,-15.1078657553674,
117.600988772271));
#113852=CARTESIAN_POINT('Ctrl Pts',(26.4124904929182,-15.4045530984644,
117.723512644894));
#113853=CARTESIAN_POINT('Ctrl Pts',(26.0272117649698,-15.5401223337483,
117.786421458838));
#113854=CARTESIAN_POINT('Ctrl Pts',(24.9614860358582,-15.8699271201329,
117.960645185498));
#113855=CARTESIAN_POINT('Ctrl Pts',(24.2729033574866,-16.0339360814211,
118.073471036143));
#113856=CARTESIAN_POINT('Ctrl Pts',(22.9797149815855,-16.2525640843145,
118.285930997449));
#113857=CARTESIAN_POINT('Ctrl Pts',(22.3783601715876,-16.319386137466,118.384941140902));
#113858=CARTESIAN_POINT('Ctrl Pts',(21.354059431856,-16.374571109063,118.553516692846));
#113859=CARTESIAN_POINT('Ctrl Pts',(20.9326788300833,-16.3805558020248,
118.622818971033));
#113860=CARTESIAN_POINT('Ctrl Pts',(20.0760515029751,-16.3587761243772,
118.763440921684));
#113861=CARTESIAN_POINT('Ctrl Pts',(19.6411834765693,-16.3298663047228,
118.834737885319));
#113862=CARTESIAN_POINT('Ctrl Pts',(18.5535127541741,-16.2126655967384,
119.013080985069));
#113863=CARTESIAN_POINT('Ctrl Pts',(17.9038907796058,-16.1016925093283,
119.119633324013));
#113864=CARTESIAN_POINT('Ctrl Pts',(16.6767957492659,-15.8130571197902,
119.321032664589));
#113865=CARTESIAN_POINT('Ctrl Pts',(16.098882022775,-15.642177621903,119.415935800281));
#113866=CARTESIAN_POINT('Ctrl Pts',(15.1574942497523,-15.3050402551196,
119.57020555807));
#113867=CARTESIAN_POINT('Ctrl Pts',(14.7882864778266,-15.1571115096946,
119.630603712903));
#113868=CARTESIAN_POINT('Ctrl Pts',(14.0506074722251,-14.8292576329358,
119.750900076669));
#113869=CARTESIAN_POINT('Ctrl Pts',(13.6827534072311,-14.6486388375962,
119.810725334464));
#113870=CARTESIAN_POINT('Ctrl Pts',(12.6991201429727,-14.1181338292149,
119.970476404401));
#113871=CARTESIAN_POINT('Ctrl Pts',(12.0985491030648,-13.7412107925646,
120.067797018619));
#113872=CARTESIAN_POINT('Ctrl Pts',(11.0318055770103,-12.9695729735432,
120.240338423157));
#113873=CARTESIAN_POINT('Ctrl Pts',(10.5595268380952,-12.5856856666768,
120.316586053339));
#113874=CARTESIAN_POINT('Ctrl Pts',(9.79638608059639,-11.8907127291724,
120.43911324634));
#113875=CARTESIAN_POINT('Ctrl Pts',(9.4943180599465,-11.5932547346191,120.487381865253));
#113876=CARTESIAN_POINT('Ctrl Pts',(8.9032160382818,-10.9639781252492,120.581183417368));
#113877=CARTESIAN_POINT('Ctrl Pts',(8.61529972165134,-10.6315678888641,
120.626562914325));
#113878=CARTESIAN_POINT('Ctrl Pts',(7.92763484426373,-9.76975584838192,
120.734381748345));
#113879=CARTESIAN_POINT('Ctrl Pts',(7.54580325266375,-9.22669885034435,
120.793728572479));
#113880=CARTESIAN_POINT('Ctrl Pts',(6.8789726410338,-8.14450419205229,120.896353041296));
#113881=CARTESIAN_POINT('Ctrl Pts',(6.58902724562507,-7.60978860165946,
120.940481819028));
#113882=CARTESIAN_POINT('Ctrl Pts',(6.15741770612613,-6.69685673131263,
121.004862979586));
#113883=CARTESIAN_POINT('Ctrl Pts',(5.998978099082,-6.32746337152405,121.028093649019));
#113884=CARTESIAN_POINT('Ctrl Pts',(5.70515824532934,-5.56721695848674,
121.070126277436));
#113885=CARTESIAN_POINT('Ctrl Pts',(5.57065440452245,-5.17632983917947,
121.088809869634));
#113886=CARTESIAN_POINT('Ctrl Pts',(5.24372883810874,-4.096592838739,121.132764719218));
#113887=CARTESIAN_POINT('Ctrl Pts',(5.08096720098151,-3.39950969154844,
121.152882509476));
#113888=CARTESIAN_POINT('Ctrl Pts',(4.8631397704427,-2.08955413269141,121.175733358692));
#113889=CARTESIAN_POINT('Ctrl Pts',(4.79615003176477,-1.47997189837179,
121.180518731692));
#113890=CARTESIAN_POINT('Ctrl Pts',(4.7398276134997,-0.442035720120334,
121.178414324204));
#113891=CARTESIAN_POINT('Ctrl Pts',(4.73310555264194,-0.0152697929301527,
121.174603797263));
#113892=CARTESIAN_POINT('Ctrl Pts',(4.75279931713012,0.85280667069366,121.160706016147));
#113893=CARTESIAN_POINT('Ctrl Pts',(4.78039298773773,1.29373913838167,121.150454881641));
#113894=CARTESIAN_POINT('Ctrl Pts',(4.89356839464253,2.39547527162674,121.117061045922));
#113895=CARTESIAN_POINT('Ctrl Pts',(5.00139648645773,3.05307143673042,121.090062567205));
#113896=CARTESIAN_POINT('Ctrl Pts',(5.28286697461074,4.29573612649765,121.025470220113));
#113897=CARTESIAN_POINT('Ctrl Pts',(5.44989054252997,4.88123512615391,120.989022181531));
#113898=CARTESIAN_POINT('Ctrl Pts',(5.77986510507261,5.83518844406934,120.919115881787));
#113899=CARTESIAN_POINT('Ctrl Pts',(5.92479484405015,6.20945808579371,120.88885565206));
#113900=CARTESIAN_POINT('Ctrl Pts',(6.24596853150438,6.9568071761554,120.822448097083));
#113901=CARTESIAN_POINT('Ctrl Pts',(6.42287468611648,7.32927828513093,120.786220060535));
#113902=CARTESIAN_POINT('Ctrl Pts',(6.94293518901919,8.32577943534677,120.680828775043));
#113903=CARTESIAN_POINT('Ctrl Pts',(7.31277227877049,8.93435801135389,120.607037047274));
#113904=CARTESIAN_POINT('Ctrl Pts',(8.07011615192993,10.0150244357185,120.457940327377));
#113905=CARTESIAN_POINT('Ctrl Pts',(8.44691841369944,10.4933269043719,120.384472763636));
#113906=CARTESIAN_POINT('Ctrl Pts',(9.12927267228777,11.26619396452,120.252119903972));
#113907=CARTESIAN_POINT('Ctrl Pts',(9.42141679712077,11.5721294771388,120.195611852136));
#113908=CARTESIAN_POINT('Ctrl Pts',(10.0393301143943,12.1705347454964,120.076231654595));
#113909=CARTESIAN_POINT('Ctrl Pts',(10.3656781195924,12.4618892800762,120.013301191211));
#113910=CARTESIAN_POINT('Ctrl Pts',(11.2121872463817,13.1579485499713,119.85060195608));
#113911=CARTESIAN_POINT('Ctrl Pts',(11.7458328819303,13.5444399087714,119.748522308693));
#113912=CARTESIAN_POINT('Ctrl Pts',(12.8092948086128,14.2191076742046,119.546045978058));
#113913=CARTESIAN_POINT('Ctrl Pts',(13.3347384211048,14.5123247839378,119.446399145257));
#113914=CARTESIAN_POINT('Ctrl Pts',(14.2317845745067,14.9485252410783,119.276502684149));
#113915=CARTESIAN_POINT('Ctrl Pts',(14.5946974353486,15.1085564130321,119.207805648761));
#113916=CARTESIAN_POINT('Ctrl Pts',(15.3417325317689,15.4052068819475,119.066307326217));
#113917=CARTESIAN_POINT('Ctrl Pts',(15.7258986236758,15.5409317215388,118.993534403211));
#113918=CARTESIAN_POINT('Ctrl Pts',(16.7868834627811,15.870491784824,118.79276342403));
#113919=CARTESIAN_POINT('Ctrl Pts',(17.4718174756613,16.0342406736939,118.663410835333));
#113920=CARTESIAN_POINT('Ctrl Pts',(18.7591419880857,16.2527058726663,118.420863675022));
#113921=CARTESIAN_POINT('Ctrl Pts',(19.358286584221,16.319506023589,118.308191325544));
#113922=CARTESIAN_POINT('Ctrl Pts',(20.2437951232121,16.3673265956352,118.141604753093));
#113923=CARTESIAN_POINT('Ctrl Pts',(20.5282226470002,16.3750000005693,118.088083586325));
#113924=CARTESIAN_POINT('Ctrl Pts',(20.8126670602263,16.375,118.034500130964));
#113925=CARTESIAN_POINT('Origin',(21.9054270700043,1.38313839548321E-14,
124.231850293098));
#113926=CARTESIAN_POINT('',(37.957553020665,1.18719490761447E-14,123.127652630566));
#113927=CARTESIAN_POINT('',(22.2006289720379,16.,125.906023473218));
#113928=CARTESIAN_POINT('Origin',(22.2006289720381,1.38313839548321E-14,
125.906023473218));
#113929=CARTESIAN_POINT('',(22.6000197806719,16.,128.171081305147));
#113930=CARTESIAN_POINT('',(21.9054270700043,16.,124.231850293098));
#113931=CARTESIAN_POINT('Origin',(22.6000197806719,1.38313839548321E-14,
128.171081305147));
#113932=CARTESIAN_POINT('Origin',(22.2006289720381,1.38313839548321E-14,
125.906023473218));
#113933=CARTESIAN_POINT('Origin',(21.9054270700043,1.38313839548321E-14,
124.231850293098));
#113934=CARTESIAN_POINT('',(38.0316540255793,1.18260248212283E-14,121.388361383802));
#113935=CARTESIAN_POINT('Origin',(20.5162416486691,1.37771738462078E-14,
116.353388269));
#113936=CARTESIAN_POINT('',(3.90398359427627,-1.84682113605508,119.460277231561));
#113937=CARTESIAN_POINT('Origin',(20.5466300797608,1.37771738462078E-14,
116.525729625777));
#113938=CARTESIAN_POINT('',(36.9907122711205,-3.93403322697978E-8,113.998798303651));
#113939=CARTESIAN_POINT('Ctrl Pts',(3.90398359410123,-1.84682113607734,
119.460277231708));
#113940=CARTESIAN_POINT('Ctrl Pts',(4.09253341241264,-3.46976715541364,
119.43913879994));
#113941=CARTESIAN_POINT('Ctrl Pts',(4.51057950486753,-5.0605456459531,119.376649209939));
#113942=CARTESIAN_POINT('Ctrl Pts',(5.79266958034729,-8.0927115867017,119.17455671751));
#113943=CARTESIAN_POINT('Ctrl Pts',(6.65971736290921,-9.5201420067015,119.034171523839));
#113944=CARTESIAN_POINT('Ctrl Pts',(9.14067745054749,-12.5154238059216,
118.624373321083));
#113945=CARTESIAN_POINT('Ctrl Pts',(10.8833818913406,-13.924253160688,118.334038478557));
#113946=CARTESIAN_POINT('Ctrl Pts',(14.8090149381498,-15.9767847332362,
117.67364111434));
#113947=CARTESIAN_POINT('Ctrl Pts',(16.9465567801897,-16.5926464636835,
117.313655965925));
#113948=CARTESIAN_POINT('Ctrl Pts',(21.3360110729831,-16.9482149073978,
116.571441632361));
#113949=CARTESIAN_POINT('Ctrl Pts',(23.5360492708532,-16.6801796399091,
116.200471262066));
#113950=CARTESIAN_POINT('Ctrl Pts',(27.7085953562218,-15.2935300241975,
115.496533117316));
#113951=CARTESIAN_POINT('Ctrl Pts',(29.6310311157987,-14.1880688975949,
115.174475049015));
#113952=CARTESIAN_POINT('Ctrl Pts',(32.943669339213,-11.2838229294257,114.622135650669));
#113953=CARTESIAN_POINT('Ctrl Pts',(34.293178901759,-9.51652058353961,114.401130878503));
#113954=CARTESIAN_POINT('Ctrl Pts',(36.2394244838757,-5.55274054743395,
114.089754684589));
#113955=CARTESIAN_POINT('Ctrl Pts',(36.8110750825502,-3.40072162936504,
114.005863757635));
#113956=CARTESIAN_POINT('Ctrl Pts',(36.9812100412032,-0.799638676443703,
113.994632996858));
#113957=CARTESIAN_POINT('Ctrl Pts',(36.9930711830864,-0.399432342122534,
113.995429427058));
#113958=CARTESIAN_POINT('Ctrl Pts',(36.9907122708882,-3.93444676838328E-8,
113.998798303983));
#113959=CARTESIAN_POINT('',(37.4303148066539,1.16738429686722E-14,113.370980817571));
#113960=CARTESIAN_POINT('',(37.4303148066539,1.16738429686722E-14,113.370980817571));
#113961=CARTESIAN_POINT('Origin',(20.5162416486691,1.37771738462078E-14,
116.353388269));
#113962=CARTESIAN_POINT('Ctrl Pts',(36.9907122708882,-3.93444688880656E-8,
113.998798303983));
#113963=CARTESIAN_POINT('Ctrl Pts',(36.9800850306418,1.79950019091975,114.013975581234));
#113964=CARTESIAN_POINT('Ctrl Pts',(36.6819302639181,3.58330630250089,114.080237606053));
#113965=CARTESIAN_POINT('Ctrl Pts',(35.7530800713107,6.33618653414545,114.265066091959));
#113966=CARTESIAN_POINT('Ctrl Pts',(35.2956795589072,7.34652123993085,114.354154457965));
#113967=CARTESIAN_POINT('Ctrl Pts',(34.2285725062847,9.19089883267023,114.558491993484));
#113968=CARTESIAN_POINT('Ctrl Pts',(33.6338727138396,10.0291239704148,114.670864685681));
#113969=CARTESIAN_POINT('Ctrl Pts',(31.5459638144946,12.4575613900211,115.062384361103));
#113970=CARTESIAN_POINT('Ctrl Pts',(29.8207162508918,13.7996252076585,115.383524865064));
#113971=CARTESIAN_POINT('Ctrl Pts',(26.9146848459564,15.2482131474179,115.919866461799));
#113972=CARTESIAN_POINT('Ctrl Pts',(25.895397765369,15.6324963399188,116.108011822642));
#113973=CARTESIAN_POINT('Ctrl Pts',(23.870374682289,16.1689827911728,116.481257071023));
#113974=CARTESIAN_POINT('Ctrl Pts',(22.8723592822232,16.3346562272248,116.664754987268));
#113975=CARTESIAN_POINT('Ctrl Pts',(20.1524185690243,16.5243507431533,117.164544345951));
#113976=CARTESIAN_POINT('Ctrl Pts',(18.4322580304876,16.3641488207914,117.4815548212));
#113977=CARTESIAN_POINT('Ctrl Pts',(15.9758638057878,15.7279853791109,117.933720990333));
#113978=CARTESIAN_POINT('Ctrl Pts',(15.1949824542152,15.4599369840143,118.07740759597));
#113979=CARTESIAN_POINT('Ctrl Pts',(13.63561352332,14.7849825795089,118.365310419915));
#113980=CARTESIAN_POINT('Ctrl Pts',(12.8618917558936,14.3714704128383,118.508675853693));
#113981=CARTESIAN_POINT('Ctrl Pts',(12.125260423911,13.8967357377783,118.645285943585));
#113982=CARTESIAN_POINT('Ctrl Pts',(17.9811304324852,16.7992135487842,116.978096432152));
#113983=CARTESIAN_POINT('Ctrl Pts',(17.0503538967826,16.626385888926,117.167878519795));
#113984=CARTESIAN_POINT('Ctrl Pts',(16.1385226671129,16.3728037819194,117.355201872128));
#113985=CARTESIAN_POINT('Ctrl Pts',(14.3473992740267,15.7021557934855,117.72511490003));
#113986=CARTESIAN_POINT('Ctrl Pts',(13.4658015096741,15.2811885701607,117.90700169916));
#113987=CARTESIAN_POINT('Ctrl Pts',(10.5304702170588,13.5432870163047,118.516688678144));
#113988=CARTESIAN_POINT('Ctrl Pts',(9.15175218320397,12.097625298113,118.817226349984));
#113989=CARTESIAN_POINT('Ctrl Pts',(7.70060472672751,10.3365673810277,119.134906706266));
#113990=CARTESIAN_POINT('Ctrl Pts',(7.14965557029621,9.53339680556488,119.258265584443));
#113991=CARTESIAN_POINT('Ctrl Pts',(6.33485406962454,8.08283642086701,119.44871952037));
#113992=CARTESIAN_POINT('Ctrl Pts',(6.03619407286761,7.46301526240171,119.521139481765));
#113993=CARTESIAN_POINT('Ctrl Pts',(5.36573584063663,5.81988748793478,119.689551381307));
#113994=CARTESIAN_POINT('Ctrl Pts',(5.04916200526517,4.76612292289117,119.77442607934));
#113995=CARTESIAN_POINT('Ctrl Pts',(4.64336725291272,2.67058753533681,119.905000730856));
#113996=CARTESIAN_POINT('Ctrl Pts',(4.54325447090625,1.63745668755726,119.952553699906));
#113997=CARTESIAN_POINT('Ctrl Pts',(4.53968745365174,0.597925404677087,
119.982827119854));
#113998=CARTESIAN_POINT('Origin',(20.412052742069,1.37771738462078E-14,
115.762503617193));
#113999=CARTESIAN_POINT('Ctrl Pts',(3.85199197861135,1.50203116532297E-8,
119.744830291073));
#114000=CARTESIAN_POINT('Ctrl Pts',(3.85271799321469,-0.37210160825748,
119.748947726387));
#114001=CARTESIAN_POINT('Ctrl Pts',(3.86545935605242,-0.744122030987361,
119.750852528501));
#114002=CARTESIAN_POINT('Ctrl Pts',(3.9298097134233,-1.70942059371102,119.750262875271));
#114003=CARTESIAN_POINT('Ctrl Pts',(4.00009513845879,-2.3009195849853,119.74445746699));
#114004=CARTESIAN_POINT('Ctrl Pts',(4.22677607963365,-3.62113055601483,
119.719625040996));
#114005=CARTESIAN_POINT('Ctrl Pts',(4.40009631645244,-4.34564743104804,
119.69769156195));
#114006=CARTESIAN_POINT('Ctrl Pts',(4.73873631394887,-5.4419393116626,119.651410533643));
#114007=CARTESIAN_POINT('Ctrl Pts',(4.87132594088532,-5.82309122877746,
119.63276466704));
#114008=CARTESIAN_POINT('Ctrl Pts',(5.28797586353499,-6.89751614828942,
119.572610144393));
#114009=CARTESIAN_POINT('Ctrl Pts',(5.60395796881511,-7.57704252247497,
119.525142407087));
#114010=CARTESIAN_POINT('Ctrl Pts',(6.29193951357836,-8.83402061782267,
119.419845430246));
#114011=CARTESIAN_POINT('Ctrl Pts',(6.65631953289691,-9.4140855358866,119.363347348149));
#114012=CARTESIAN_POINT('Ctrl Pts',(7.52516386874132,-10.6283481506271,
119.227472650152));
#114013=CARTESIAN_POINT('Ctrl Pts',(8.0419455767051,-11.2514241803914,119.145991033838));
#114014=CARTESIAN_POINT('Ctrl Pts',(9.08935198284955,-12.3450437351211,
118.978848345114));
#114015=CARTESIAN_POINT('Ctrl Pts',(9.60911156584989,-12.823841024795,118.895017827169));
#114016=CARTESIAN_POINT('Ctrl Pts',(10.6964592721647,-13.7060623220113,
118.718992292532));
#114017=CARTESIAN_POINT('Ctrl Pts',(11.262180675743,-14.109662558594,118.627127092461));
#114018=CARTESIAN_POINT('Ctrl Pts',(12.533969198827,-14.9027933258467,118.420336055715));
#114019=CARTESIAN_POINT('Ctrl Pts',(13.2463513125027,-15.2786458153057,
118.304355644959));
#114020=CARTESIAN_POINT('Ctrl Pts',(14.408983687951,-15.7884938562373,118.114134007312));
#114021=CARTESIAN_POINT('Ctrl Pts',(14.8429858589734,-15.9575118233424,
118.042872723305));
#114022=CARTESIAN_POINT('Ctrl Pts',(15.834430410622,-16.2964541964434,117.879851808611));
#114023=CARTESIAN_POINT('Ctrl Pts',(16.3947999294395,-16.4556862701782,
117.787577779365));
#114024=CARTESIAN_POINT('Ctrl Pts',(17.7647960824515,-16.7681638955507,
117.5621158453));
#114025=CARTESIAN_POINT('Ctrl Pts',(18.5796111634086,-16.8911468539739,
117.428162113254));
#114026=CARTESIAN_POINT('Ctrl Pts',(19.742825576758,-16.9789270540022,117.236892774666));
#114027=CARTESIAN_POINT('Ctrl Pts',(20.0863305029633,-16.9941127917336,
117.180394982505));
#114028=CARTESIAN_POINT('Ctrl Pts',(20.8687595384806,-17.0043128978382,
117.051551265545));
#114029=CARTESIAN_POINT('Ctrl Pts',(21.3075047500614,-16.9925873117754,
116.979157735974));
#114030=CARTESIAN_POINT('Ctrl Pts',(22.3314933276495,-16.9244202093205,
116.810165704712));
#114031=CARTESIAN_POINT('Ctrl Pts',(22.9152707581049,-16.8542132352159,
116.713819192822));
#114032=CARTESIAN_POINT('Ctrl Pts',(24.2166311841858,-16.626969122988,116.499475361948));
#114033=CARTESIAN_POINT('Ctrl Pts',(24.9301381832088,-16.4529756777154,
116.382273419367));
#114034=CARTESIAN_POINT('Ctrl Pts',(26.0117157534911,-16.111944864853,116.204986476976));
#114035=CARTESIAN_POINT('Ctrl Pts',(26.3889193678127,-15.9778624640433,
116.143221441321));
#114036=CARTESIAN_POINT('Ctrl Pts',(27.4525780934676,-15.5559612318494,
115.96902314246));
#114037=CARTESIAN_POINT('Ctrl Pts',(28.1253461728596,-15.2354433406124,
115.8586704274));
#114038=CARTESIAN_POINT('Ctrl Pts',(29.3671431107902,-14.5384840938646,
115.655739420418));
#114039=CARTESIAN_POINT('Ctrl Pts',(29.9389426923638,-14.1701502984732,
115.56265904247));
#114040=CARTESIAN_POINT('Ctrl Pts',(31.1382177033198,-13.2902733853208,
115.368530305677));
#114041=CARTESIAN_POINT('Ctrl Pts',(31.7545545940983,-12.7659684716934,
115.269514531316));
#114042=CARTESIAN_POINT('Ctrl Pts',(32.8030425974044,-11.7355072922184,
115.101672402844));
#114043=CARTESIAN_POINT('Ctrl Pts',(33.2473503334598,-11.2444095111543,
115.030665807847));
#114044=CARTESIAN_POINT('Ctrl Pts',(34.1157035321844,-10.1638523206168,
114.89303802056));
#114045=CARTESIAN_POINT('Ctrl Pts',(34.5331004292285,-9.57060514800458,
114.827612323976));
#114046=CARTESIAN_POINT('Ctrl Pts',(35.3429169625275,-8.2481290840788,114.702756888522));
#114047=CARTESIAN_POINT('Ctrl Pts',(35.7228201630239,-7.51321099309242,
114.645587234829));
#114048=CARTESIAN_POINT('Ctrl Pts',(36.2345314732538,-6.31885114286027,
114.570346560497));
#114049=CARTESIAN_POINT('Ctrl Pts',(36.4026661867263,-5.87679790201272,
114.545991015855));
#114050=CARTESIAN_POINT('Ctrl Pts',(36.7386620439605,-4.8703271861914,114.498562365834));
#114051=CARTESIAN_POINT('Ctrl Pts',(36.8962420959419,-4.30302893979826,
114.477304368902));
#114052=CARTESIAN_POINT('Ctrl Pts',(37.207245462913,-2.91072959494826,114.438617875259));
#114053=CARTESIAN_POINT('Ctrl Pts',(37.3301644725751,-2.08034584037984,
114.426721472385));
#114054=CARTESIAN_POINT('Ctrl Pts',(37.4178422211624,-0.90001140238114,
114.425114777429));
#114055=CARTESIAN_POINT('Ctrl Pts',(37.4330817608476,-0.555049444777654,
114.426461153991));
#114056=CARTESIAN_POINT('Ctrl Pts',(37.4472678076631,0.449246104619875,
114.435507171637));
#114057=CARTESIAN_POINT('Ctrl Pts',(37.4187635225561,1.108284042432,114.447795564935));
#114058=CARTESIAN_POINT('Ctrl Pts',(37.2802795982228,2.4817911040431,114.48756930671));
#114059=CARTESIAN_POINT('Ctrl Pts',(37.1629618698992,3.19418405315069,114.516367827871));
#114060=CARTESIAN_POINT('Ctrl Pts',(36.8166970857841,4.70042200423587,114.59526874833));
#114061=CARTESIAN_POINT('Ctrl Pts',(36.5745791108977,5.48923154181531,114.647748596065));
#114062=CARTESIAN_POINT('Ctrl Pts',(36.1067888181912,6.69578234672308,114.745176264061));
#114063=CARTESIAN_POINT('Ctrl Pts',(35.9186866220005,7.12721727996997,114.783620197467));
#114064=CARTESIAN_POINT('Ctrl Pts',(35.4566150813895,8.07790602254515,114.876901575129));
#114065=CARTESIAN_POINT('Ctrl Pts',(35.1732364169441,8.59175099873082,114.93340010801));
#114066=CARTESIAN_POINT('Ctrl Pts',(34.4256662182454,9.79592859903436,115.081344438067));
#114067=CARTESIAN_POINT('Ctrl Pts',(33.9364866331835,10.4683694410871,115.17734737897));
#114068=CARTESIAN_POINT('Ctrl Pts',(33.1782298465971,11.364102886918,115.324893274146));
#114069=CARTESIAN_POINT('Ctrl Pts',(32.9479882125162,11.6198018402333,115.369544650871));
#114070=CARTESIAN_POINT('Ctrl Pts',(32.4018327708539,12.1901923961905,115.475007335694));
#114071=CARTESIAN_POINT('Ctrl Pts',(32.0809814011665,12.4996467427407,115.53660638392));
#114072=CARTESIAN_POINT('Ctrl Pts',(31.3098433945328,13.1863187617331,115.684175017861));
#114073=CARTESIAN_POINT('Ctrl Pts',(30.8514325589148,13.5532197783405,115.771572094959));
#114074=CARTESIAN_POINT('Ctrl Pts',(29.7518229927019,14.3421697557263,115.980939691737));
#114075=CARTESIAN_POINT('Ctrl Pts',(29.0991589453022,14.7453853766348,116.105033475238));
#114076=CARTESIAN_POINT('Ctrl Pts',(28.0871520018169,15.277780253951,116.297041181183));
#114077=CARTESIAN_POINT('Ctrl Pts',(27.7468654774369,15.4422015372312,116.361529641027));
#114078=CARTESIAN_POINT('Ctrl Pts',(26.7683612233073,15.8743439342201,116.54657308316));
#114079=CARTESIAN_POINT('Ctrl Pts',(26.1188324460879,16.1137232616475,116.668838755098));
#114080=CARTESIAN_POINT('Ctrl Pts',(24.7922172442306,16.5100104461845,116.918422555183));
#114081=CARTESIAN_POINT('Ctrl Pts',(24.1163405762553,16.6662611877686,117.04553556975));
#114082=CARTESIAN_POINT('Ctrl Pts',(22.6337691523531,16.9116792603534,117.324602149443));
#114083=CARTESIAN_POINT('Ctrl Pts',(21.8262668366208,16.9846848324341,117.47676301644));
#114084=CARTESIAN_POINT('Ctrl Pts',(20.3085977417149,17.0093357039595,117.762159566835));
#114085=CARTESIAN_POINT('Ctrl Pts',(19.6004264523002,16.9750187446062,117.894949973447));
#114086=CARTESIAN_POINT('Ctrl Pts',(18.2159800951321,16.8178077503574,118.154839084414));
#114087=CARTESIAN_POINT('Ctrl Pts',(17.54073749996,16.6980293030593,118.281752438149));
#114088=CARTESIAN_POINT('Ctrl Pts',(16.0974956406338,16.3478780427604,118.55365975145));
#114089=CARTESIAN_POINT('Ctrl Pts',(15.3346814310107,16.1028393572611,118.697800747025));
#114090=CARTESIAN_POINT('Ctrl Pts',(13.9745337524518,15.5540667308777,118.954773074378));
#114091=CARTESIAN_POINT('Ctrl Pts',(13.3721674714921,15.2676722999989,119.06844030748));
#114092=CARTESIAN_POINT('Ctrl Pts',(12.1701191348142,14.604589514317,119.295882779618));
#114093=CARTESIAN_POINT('Ctrl Pts',(11.5738563299225,14.2242624331316,119.409072544891));
#114094=CARTESIAN_POINT('Ctrl Pts',(10.3375441029528,13.3202174924989,119.644955350538));
#114095=CARTESIAN_POINT('Ctrl Pts',(9.70830067517231,12.7844092305938,119.765808959591));
#114096=CARTESIAN_POINT('Ctrl Pts',(8.61944759326335,11.7091674408892,119.975589220271));
#114097=CARTESIAN_POINT('Ctrl Pts',(8.14956662736872,11.1831025683743,120.066253985677));
#114098=CARTESIAN_POINT('Ctrl Pts',(7.28355580932695,10.0819854007779,120.234654862375));
#114099=CARTESIAN_POINT('Ctrl Pts',(6.88731422728817,9.50877753106153,120.312411527511));
#114100=CARTESIAN_POINT('Ctrl Pts',(6.10903212580853,8.22015947760868,120.467106658173));
#114101=CARTESIAN_POINT('Ctrl Pts',(5.74046962270476,7.49834933045992,120.5417275053));
#114102=CARTESIAN_POINT('Ctrl Pts',(5.24083623071057,6.32021024263145,120.6446099079));
#114103=CARTESIAN_POINT('Ctrl Pts',(5.07527966788584,5.88040718534626,120.67906723405));
#114104=CARTESIAN_POINT('Ctrl Pts',(4.74350280728304,4.87570126780782,120.749366118117));
#114105=CARTESIAN_POINT('Ctrl Pts',(4.5878104871605,4.30782722835296,120.783353049156));
#114106=CARTESIAN_POINT('Ctrl Pts',(4.28282875510673,2.91945271640569,120.85323538363));
#114107=CARTESIAN_POINT('Ctrl Pts',(4.16337497561081,2.09370822520031,120.884019039261));
#114108=CARTESIAN_POINT('Ctrl Pts',(4.07930582718988,0.914935586217559,
120.912679619261));
#114109=CARTESIAN_POINT('Ctrl Pts',(4.06505102882361,0.566869786360458,
120.919264141611));
#114110=CARTESIAN_POINT('Ctrl Pts',(4.06054612858338,0.145722462032777,
120.92490224283));
#114111=CARTESIAN_POINT('Ctrl Pts',(4.06022763391727,0.0728596834798867,
120.925793376835));
#114112=CARTESIAN_POINT('Ctrl Pts',(4.06036979181167,1.50326513895498E-8,
120.926599594688));
#114113=CARTESIAN_POINT('Ctrl Pts',(4.00959443610706,-1.25170851643402E-8,
120.638638242996));
#114114=CARTESIAN_POINT('Ctrl Pts',(4.00941930028957,0.0897616374665513,
120.637644998799));
#114115=CARTESIAN_POINT('Ctrl Pts',(4.00994522096334,0.179531815916759,
120.63653358753));
#114116=CARTESIAN_POINT('Ctrl Pts',(4.02241319275843,1.09160129606617,120.624027713017));
#114117=CARTESIAN_POINT('Ctrl Pts',(4.09245406774986,1.91187325198813,120.602698061528));
#114118=CARTESIAN_POINT('Ctrl Pts',(4.32997148817351,3.41615195095139,120.543651401598));
#114119=CARTESIAN_POINT('Ctrl Pts',(4.48139080798906,4.10102192532192,120.508870155708));
#114120=CARTESIAN_POINT('Ctrl Pts',(4.86894595447833,5.45566394986278,120.424051461169));
#114121=CARTESIAN_POINT('Ctrl Pts',(5.10569304281492,6.1238361677535,120.373942172049));
#114122=CARTESIAN_POINT('Ctrl Pts',(5.53393200045323,7.12952847586363,120.286047843403));
#114123=CARTESIAN_POINT('Ctrl Pts',(5.69680707063255,7.4787675842911,120.253036441261));
#114124=CARTESIAN_POINT('Ctrl Pts',(6.21907007830176,8.5063951264318,120.148079606928));
#114125=CARTESIAN_POINT('Ctrl Pts',(6.61229879522507,9.16583718027728,120.070125792049));
#114126=CARTESIAN_POINT('Ctrl Pts',(7.38379765576326,10.2808484071456,119.918385020826));
#114127=CARTESIAN_POINT('Ctrl Pts',(7.74417176915716,10.7476537005959,119.847880703483));
#114128=CARTESIAN_POINT('Ctrl Pts',(8.41822736444313,11.5323419487485,119.716829141124));
#114129=CARTESIAN_POINT('Ctrl Pts',(8.72169523896559,11.8585311948728,119.658091568323));
#114130=CARTESIAN_POINT('Ctrl Pts',(9.28165636666735,12.4144326952983,119.550341446819));
#114131=CARTESIAN_POINT('Ctrl Pts',(9.53302405607704,12.6490968913906,119.502156238616));
#114132=CARTESIAN_POINT('Ctrl Pts',(10.4128789185094,13.4212897305271,119.333874211133));
#114133=CARTESIAN_POINT('Ctrl Pts',(11.0732209728882,13.9194267380072,119.208147069428));
#114134=CARTESIAN_POINT('Ctrl Pts',(12.2560288088416,14.6811166886917,118.983209706228));
#114135=CARTESIAN_POINT('Ctrl Pts',(12.7609433941091,14.9700149254131,118.887279820164));
#114136=CARTESIAN_POINT('Ctrl Pts',(13.6949513007292,15.4411687009317,118.710186284678));
#114137=CARTESIAN_POINT('Ctrl Pts',(14.1187151926111,15.6330014728069,118.629978501912));
#114138=CARTESIAN_POINT('Ctrl Pts',(15.2925990160622,16.1058440253134,118.408471012262));
#114139=CARTESIAN_POINT('Ctrl Pts',(16.055611923457,16.3504407701573,118.265042740636));
#114140=CARTESIAN_POINT('Ctrl Pts',(17.5028474371416,16.7007056529506,117.992792844911));
#114141=CARTESIAN_POINT('Ctrl Pts',(18.1820204468462,16.8205536260093,117.864958416257));
#114142=CARTESIAN_POINT('Ctrl Pts',(19.5598323485553,16.9752682547864,117.605528693718));
#114143=CARTESIAN_POINT('Ctrl Pts',(20.2572667455539,17.0088668144535,117.474177393979));
#114144=CARTESIAN_POINT('Ctrl Pts',(21.7741415562458,16.9852600946745,117.189265334446));
#114145=CARTESIAN_POINT('Ctrl Pts',(22.5915224717932,16.9111999146883,117.036039392438));
#114146=CARTESIAN_POINT('Ctrl Pts',(24.093168110406,16.6609389494782,116.753811883417));
#114147=CARTESIAN_POINT('Ctrl Pts',(24.7782503198109,16.5011163161582,116.62477315557));
#114148=CARTESIAN_POINT('Ctrl Pts',(26.0904043329047,16.104997532903,116.377133536012));
#114149=CARTESIAN_POINT('Ctrl Pts',(26.7174905868263,15.873336267133,116.258576530814));
#114150=CARTESIAN_POINT('Ctrl Pts',(28.0734795149186,15.2767865408782,116.002484637455));
#114151=CARTESIAN_POINT('Ctrl Pts',(28.7932354201816,14.8947128644818,115.86655500571));
#114152=CARTESIAN_POINT('Ctrl Pts',(30.0811344098328,14.0845853304245,115.622083128316));
#114153=CARTESIAN_POINT('Ctrl Pts',(30.6554519075947,13.6701016283902,115.512550630566));
#114154=CARTESIAN_POINT('Ctrl Pts',(31.7157604337614,12.7973756534496,115.309356867423));
#114155=CARTESIAN_POINT('Ctrl Pts',(32.2040772124031,12.3441134431078,115.215330091604));
#114156=CARTESIAN_POINT('Ctrl Pts',(32.9043392884413,11.612143294737,115.080290415224));
#114157=CARTESIAN_POINT('Ctrl Pts',(33.1362928032818,11.3542166814392,115.035501283874));
#114158=CARTESIAN_POINT('Ctrl Pts',(33.8929474327213,10.4587984692788,114.888957473996));
#114159=CARTESIAN_POINT('Ctrl Pts',(34.3793648001977,9.78944551919494,114.793937144242));
#114160=CARTESIAN_POINT('Ctrl Pts',(35.1247318148005,8.58818303815335,114.646169202786));
#114161=CARTESIAN_POINT('Ctrl Pts',(35.4081786357093,8.07378631833508,114.589283864809));
#114162=CARTESIAN_POINT('Ctrl Pts',(35.8692721662685,7.12416271301863,114.495592266303));
#114163=CARTESIAN_POINT('Ctrl Pts',(36.0565242320879,6.69443153578555,114.457108069221));
#114164=CARTESIAN_POINT('Ctrl Pts',(36.5191404407503,5.50143785511238,114.36103444054));
#114165=CARTESIAN_POINT('Ctrl Pts',(36.7585332602379,4.72505075855716,114.30993383552));
#114166=CARTESIAN_POINT('Ctrl Pts',(37.1005710479695,3.25254145824192,114.232560306386));
#114167=CARTESIAN_POINT('Ctrl Pts',(37.2172154447346,2.56156820931256,114.203915819025));
#114168=CARTESIAN_POINT('Ctrl Pts',(37.3668078416288,1.15951241881491,114.161052857355));
#114169=CARTESIAN_POINT('Ctrl Pts',(37.3984771000427,0.449654850245953,
114.147091391248));
#114170=CARTESIAN_POINT('Ctrl Pts',(37.3722207529235,-1.09396235525398,
114.134271572704));
#114171=CARTESIAN_POINT('Ctrl Pts',(37.297702358504,-1.92563455369374,114.138310420694));
#114172=CARTESIAN_POINT('Ctrl Pts',(37.0481456529654,-3.45388030596479,
114.164862247004));
#114173=CARTESIAN_POINT('Ctrl Pts',(36.8892313015764,-4.15126057687536,
114.184639028468));
#114174=CARTESIAN_POINT('Ctrl Pts',(36.4963490562346,-5.48605687675346,
114.237647904344));
#114175=CARTESIAN_POINT('Ctrl Pts',(36.2670725075451,-6.12351678490518,
114.270099446789));
#114176=CARTESIAN_POINT('Ctrl Pts',(35.6816057623652,-7.49201423894137,
114.356478426261));
#114177=CARTESIAN_POINT('Ctrl Pts',(35.309918173823,-8.21444541962333,114.413124686832));
#114178=CARTESIAN_POINT('Ctrl Pts',(34.5272657296374,-9.50155972380706,
114.534094029113));
#114179=CARTESIAN_POINT('Ctrl Pts',(34.130121517857,-10.072849712436,114.596078870479));
#114180=CARTESIAN_POINT('Ctrl Pts',(33.2567246534963,-11.1781883092315,
114.733542630841));
#114181=CARTESIAN_POINT('Ctrl Pts',(32.7794288768618,-11.7096249860511,
114.809234167398));
#114182=CARTESIAN_POINT('Ctrl Pts',(31.6935580895123,-12.7750858369867,
114.983400478659));
#114183=CARTESIAN_POINT('Ctrl Pts',(31.0773355552952,-13.2985586939205,
115.083171767844));
#114184=CARTESIAN_POINT('Ctrl Pts',(29.8743613895649,-14.1798125471617,
115.278357715051));
#114185=CARTESIAN_POINT('Ctrl Pts',(29.298425482713,-14.5498604120333,115.371968236492));
#114186=CARTESIAN_POINT('Ctrl Pts',(28.0625214018881,-15.2409386847464,
115.573199682369));
#114187=CARTESIAN_POINT('Ctrl Pts',(27.4008044647638,-15.5557999556707,
115.6811530664));
#114188=CARTESIAN_POINT('Ctrl Pts',(26.3541034903535,-15.9718380084046,
115.852858291872));
#114189=CARTESIAN_POINT('Ctrl Pts',(25.9822179651935,-16.1045424611203,
115.914001383399));
#114190=CARTESIAN_POINT('Ctrl Pts',(24.8988200925056,-16.4481814905653,
116.092242525465));
#114191=CARTESIAN_POINT('Ctrl Pts',(24.1776960641974,-16.6247725812183,
116.210989886834));
#114192=CARTESIAN_POINT('Ctrl Pts',(22.8690593008678,-16.8535855084627,
116.426244432939));
#114193=CARTESIAN_POINT('Ctrl Pts',(22.2858720973622,-16.9238823077358,
116.522099685318));
#114194=CARTESIAN_POINT('Ctrl Pts',(21.2608407091994,-16.9924661098353,
116.690663287622));
#114195=CARTESIAN_POINT('Ctrl Pts',(20.8204508694921,-17.0043221651928,
116.763123114258));
#114196=CARTESIAN_POINT('Ctrl Pts',(20.036746452358,-16.9941460515523,116.892321026314));
#114197=CARTESIAN_POINT('Ctrl Pts',(19.6935856990506,-16.979001773077,116.948957606962));
#114198=CARTESIAN_POINT('Ctrl Pts',(18.5303243083283,-16.8913361586865,
117.140937191185));
#114199=CARTESIAN_POINT('Ctrl Pts',(17.7151179108909,-16.7683375808488,
117.275402802738));
#114200=CARTESIAN_POINT('Ctrl Pts',(16.3446787257858,-16.4558041489712,
117.500684601443));
#114201=CARTESIAN_POINT('Ctrl Pts',(15.7843002396079,-16.2966055065796,
117.592592357442));
#114202=CARTESIAN_POINT('Ctrl Pts',(14.7926010507014,-15.9576504725585,
117.755058380267));
#114203=CARTESIAN_POINT('Ctrl Pts',(14.3583603041696,-15.7885620302798,
117.82614752501));
#114204=CARTESIAN_POINT('Ctrl Pts',(13.1827235176851,-15.2729862389073,
118.018773325584));
#114205=CARTESIAN_POINT('Ctrl Pts',(12.4584699152919,-14.8896318770529,
118.137441055054));
#114206=CARTESIAN_POINT('Ctrl Pts',(11.1567694101241,-14.0732459290973,
118.349467910793));
#114207=CARTESIAN_POINT('Ctrl Pts',(10.5735987631925,-13.6531402431575,
118.44393147152));
#114208=CARTESIAN_POINT('Ctrl Pts',(9.51717859125105,-12.7842820492166,
118.614085566742));
#114209=CARTESIAN_POINT('Ctrl Pts',(9.03963203754324,-12.3429421777055,
118.690583911227));
#114210=CARTESIAN_POINT('Ctrl Pts',(8.35137225178435,-11.6289947435209,
118.800645361808));
#114211=CARTESIAN_POINT('Ctrl Pts',(8.12178136911124,-11.3759359997991,
118.837304741581));
#114212=CARTESIAN_POINT('Ctrl Pts',(7.34610584542342,-10.4672517649577,
118.960731741905));
#114213=CARTESIAN_POINT('Ctrl Pts',(6.84144120640024,-9.77700645242168,
119.04018367225));
#114214=CARTESIAN_POINT('Ctrl Pts',(6.07626521479113,-8.54633206248309,
119.158377721677));
#114215=CARTESIAN_POINT('Ctrl Pts',(5.7887332234669,-8.02512483548903,119.202085921422));
#114216=CARTESIAN_POINT('Ctrl Pts',(5.33194267538356,-7.08433436660324,
119.2703842278));
#114217=CARTESIAN_POINT('Ctrl Pts',(5.15110109479715,-6.67117922278847,
119.297027606815));
#114218=CARTESIAN_POINT('Ctrl Pts',(4.84876516523162,-5.89891988503616,
119.340953402027));
#114219=CARTESIAN_POINT('Ctrl Pts',(4.72248360426319,-5.54204249120961,
119.359012018623));
#114220=CARTESIAN_POINT('Ctrl Pts',(4.42063356141633,-4.59024170670288,
119.401126195762));
#114221=CARTESIAN_POINT('Ctrl Pts',(4.26521846397487,-3.9893706433944,119.421616823222));
#114222=CARTESIAN_POINT('Ctrl Pts',(4.04000962269131,-2.87370222757645,
119.448350331979));
#114223=CARTESIAN_POINT('Ctrl Pts',(3.9604302776283,-2.36168632455117,119.456378260556));
#114224=CARTESIAN_POINT('Ctrl Pts',(3.90398359427621,-1.84682113605508,
119.46027723156));
#114225=CARTESIAN_POINT('Origin',(-15.0675364833309,-75.,72.98888938658));
#114226=CARTESIAN_POINT('',(-15.5675364832709,-84.9916953137207,73.3961602849894));
#114227=CARTESIAN_POINT('Origin',(-15.5675364832709,-75.,72.98888938658));
#114228=CARTESIAN_POINT('',(-15.0675364833309,-84.4921179126434,73.3757970402573));
#114229=CARTESIAN_POINT('Origin',(-15.0675364833309,-84.9917030659404,73.3961606009772));
#114230=CARTESIAN_POINT('',(-15.0675364833309,-65.5,72.98888938658));
#114231=CARTESIAN_POINT('Origin',(-15.0675364833309,-75.,72.98888938658));
#114232=CARTESIAN_POINT('Origin',(-15.0675364833309,-75.,72.98888938658));
#114233=CARTESIAN_POINT('Origin',(-15.9175364833309,-75.,72.98888938658));
#114234=CARTESIAN_POINT('',(-13.5675364833309,-65.5,72.98888938658));
#114235=CARTESIAN_POINT('',(-15.9175364833309,-65.5,72.98888938658));
#114236=CARTESIAN_POINT('Origin',(-13.5675364833309,-75.,72.98888938658));
#114237=CARTESIAN_POINT('Origin',(-13.2677182305224,-75.,72.98888938658));
#114238=CARTESIAN_POINT('',(-13.2266934083678,-66.3412177685878,72.9890206473583));
#114239=CARTESIAN_POINT('',(-13.5675364833309,-80.6547445743814,66.0025908482903));
#114240=CARTESIAN_POINT('Ctrl Pts',(-13.2266934083678,-66.3412177685878,
72.9890206473583));
#114241=CARTESIAN_POINT('Ctrl Pts',(-13.2407667008042,-66.3271326547269,
72.1690325463416));
#114242=CARTESIAN_POINT('Ctrl Pts',(-13.2550858955079,-66.4295793336072,
71.3495943325524));
#114243=CARTESIAN_POINT('Ctrl Pts',(-13.2840611221687,-66.8589654028222,
69.7699075933991));
#114244=CARTESIAN_POINT('Ctrl Pts',(-13.2977088950612,-67.1832493356237,
69.0176462295908));
#114245=CARTESIAN_POINT('Ctrl Pts',(-13.3212649090564,-67.8955624618356,
67.8450674617599));
#114246=CARTESIAN_POINT('Ctrl Pts',(-13.3310562007338,-68.2300949998944,
67.3967683499587));
#114247=CARTESIAN_POINT('Ctrl Pts',(-13.3606234486437,-69.3599797236658,
66.1502763569408));
#114248=CARTESIAN_POINT('Ctrl Pts',(-13.3788394562794,-70.2685176026843,
65.4723217468462));
#114249=CARTESIAN_POINT('Ctrl Pts',(-13.4083143132994,-71.7995141325709,
64.7275913681621));
#114250=CARTESIAN_POINT('Ctrl Pts',(-13.4186276870038,-72.3482377586366,
64.5246133683743));
#114251=CARTESIAN_POINT('Ctrl Pts',(-13.4386174214408,-73.4695109564809,
64.232333269707));
#114252=CARTESIAN_POINT('Ctrl Pts',(-13.4484368516908,-74.0392487572431,
64.1418028503483));
#114253=CARTESIAN_POINT('Ctrl Pts',(-13.4742869329458,-75.5285911817388,
64.051052323433));
#114254=CARTESIAN_POINT('Ctrl Pts',(-13.4928531712087,-76.5958501455569,
64.1271300649806));
#114255=CARTESIAN_POINT('Ctrl Pts',(-13.5251748522153,-78.7941276658468,
64.7998965188398));
#114256=CARTESIAN_POINT('Ctrl Pts',(-13.5399964381131,-79.784891548598,
65.3190823617296));
#114257=CARTESIAN_POINT('Ctrl Pts',(-13.5590282940972,-80.6565021394416,
66.0000474243114));
#114258=CARTESIAN_POINT('Ctrl Pts',(-12.9675119086199,-76.1752581060379,
81.3058749742284));
#114259=CARTESIAN_POINT('Ctrl Pts',(-12.9761555362729,-75.7054160823964,
81.3809966173537));
#114260=CARTESIAN_POINT('Ctrl Pts',(-12.984944367006,-75.2297319433566,
81.4162357955362));
#114261=CARTESIAN_POINT('Ctrl Pts',(-13.0018977558637,-74.2930269577767,
81.4058301185759));
#114262=CARTESIAN_POINT('Ctrl Pts',(-13.0099327739343,-73.8336256353453,
81.3626055539312));
#114263=CARTESIAN_POINT('Ctrl Pts',(-13.034703878876,-72.4494579405428,
81.1175572774556));
#114264=CARTESIAN_POINT('Ctrl Pts',(-13.0521103372511,-71.5497303411989,
80.7973636804612));
#114265=CARTESIAN_POINT('Ctrl Pts',(-13.0786991340095,-70.2436949188266,
80.067967843619));
#114266=CARTESIAN_POINT('Ctrl Pts',(-13.0881440974825,-69.7906308676622,
79.7534393148135));
#114267=CARTESIAN_POINT('Ctrl Pts',(-13.1078514587778,-68.9366818033151,
79.0296821594344));
#114268=CARTESIAN_POINT('Ctrl Pts',(-13.1181095048179,-68.5395865522349,
78.6185751098584));
#114269=CARTESIAN_POINT('Ctrl Pts',(-13.14503423917,-67.6118538973413,77.4433982113719));
#114270=CARTESIAN_POINT('Ctrl Pts',(-13.1606202152678,-67.1609530319177,
76.6272467528462));
#114271=CARTESIAN_POINT('Ctrl Pts',(-13.1935425350349,-66.5290168126367,
74.8691112225869));
#114272=CARTESIAN_POINT('Ctrl Pts',(-13.2104360376322,-66.3574887953517,
73.9362652681327));
#114273=CARTESIAN_POINT('Ctrl Pts',(-13.2266934083678,-66.3412177685878,
72.9890206473583));
#114274=CARTESIAN_POINT('',(-13.2736619003202,-83.7052176583754,72.9888947630294));
#114275=CARTESIAN_POINT('Ctrl Pts',(-13.2736619003202,-83.7052176583754,
72.9888947630294));
#114276=CARTESIAN_POINT('Ctrl Pts',(-13.2229688258284,-83.6545977325295,
72.2041789688224));
#114277=CARTESIAN_POINT('Ctrl Pts',(-13.1720553132674,-83.4982142737105,
71.4337103090239));
#114278=CARTESIAN_POINT('Ctrl Pts',(-13.0702284178419,-82.9868581475011,
69.9759204830989));
#114279=CARTESIAN_POINT('Ctrl Pts',(-13.0193150349773,-82.6340458634663,
69.2881849289806));
#114280=CARTESIAN_POINT('Ctrl Pts',(-12.9679003706341,-82.2015397612608,
68.6647904662762));
#114281=CARTESIAN_POINT('',(-13.5669824724428,-82.8099251083261,77.459681895839));
#114282=CARTESIAN_POINT('Ctrl Pts',(-13.5669824724428,-82.8099251083261,
77.459681895839));
#114283=CARTESIAN_POINT('Ctrl Pts',(-13.5187525677101,-83.1543720959849,
76.7599043053519));
#114284=CARTESIAN_POINT('Ctrl Pts',(-13.4698907813316,-83.4052651158459,
76.0216902016215));
#114285=CARTESIAN_POINT('Ctrl Pts',(-13.3719801094319,-83.7042558727909,
74.5139171860312));
#114286=CARTESIAN_POINT('Ctrl Pts',(-13.3229312239106,-83.753373874782,
73.7448830644764));
#114287=CARTESIAN_POINT('Ctrl Pts',(-13.2736619003202,-83.7052176583754,
72.9888947630294));
#114288=CARTESIAN_POINT('Origin',(-13.5675364833309,-75.,72.98888938658));
#114289=CARTESIAN_POINT('Origin',(-15.9175364833309,-75.,72.98888938658));
#114290=CARTESIAN_POINT('',(-11.126080082656,-83.3999999999947,72.9888988113144));
#114291=CARTESIAN_POINT('Ctrl Pts',(-11.8763230992193,-66.6,72.98888938658));
#114292=CARTESIAN_POINT('Ctrl Pts',(-11.8631868209786,-66.6,73.4447625248225));
#114293=CARTESIAN_POINT('Ctrl Pts',(-11.8499323085124,-66.6371108146397,
73.9000553019549));
#114294=CARTESIAN_POINT('Ctrl Pts',(-11.8215505215453,-66.7982238465426,
74.8810309345825));
#114295=CARTESIAN_POINT('Ctrl Pts',(-11.8066118707031,-66.9361797585604,
75.4022143669236));
#114296=CARTESIAN_POINT('Ctrl Pts',(-11.7608748863597,-67.5043835959706,
76.9361908756775));
#114297=CARTESIAN_POINT('Ctrl Pts',(-11.7286576515623,-68.0839240829853,
77.8810612875392));
#114298=CARTESIAN_POINT('Ctrl Pts',(-11.6830410476023,-69.1896027373828,
79.0783996027313));
#114299=CARTESIAN_POINT('Ctrl Pts',(-11.6683360173514,-69.5866997778602,
79.4339675737516));
#114300=CARTESIAN_POINT('Ctrl Pts',(-11.6388063150206,-70.412644761118,
80.0430072438156));
#114301=CARTESIAN_POINT('Ctrl Pts',(-11.6244218669597,-70.8356745762694,
80.3007161607582));
#114302=CARTESIAN_POINT('Ctrl Pts',(-11.5952332387126,-71.7533765643096,
80.754166157821));
#114303=CARTESIAN_POINT('Ctrl Pts',(-11.5805467836055,-72.2489414458553,
80.9432445269332));
#114304=CARTESIAN_POINT('Ctrl Pts',(-11.5350826929847,-73.8155100562091,
81.3769013847141));
#114305=CARTESIAN_POINT('Ctrl Pts',(-11.5029132423661,-74.9191184248915,
81.4597345425669));
#114306=CARTESIAN_POINT('Ctrl Pts',(-11.4573495157567,-76.5357040014433,
81.2644397908755));
#114307=CARTESIAN_POINT('Ctrl Pts',(-11.4426237633509,-77.0566866345932,
81.1505780668194));
#114308=CARTESIAN_POINT('Ctrl Pts',(-11.412347381053,-78.0581362354934,
80.8296613001395));
#114309=CARTESIAN_POINT('Ctrl Pts',(-11.3972392495797,-78.5371113108017,
80.6255613125404));
#114310=CARTESIAN_POINT('Ctrl Pts',(-11.3676835224782,-79.4510244581362,
80.1315843948107));
#114311=CARTESIAN_POINT('Ctrl Pts',(-11.3532974583416,-79.8840076862191,
79.8428064851497));
#114312=CARTESIAN_POINT('Ctrl Pts',(-11.3082195679676,-81.1349701187117,
78.8293990833468));
#114313=CARTESIAN_POINT('Ctrl Pts',(-11.2762215280228,-81.8406359595486,
77.9843984850121));
#114314=CARTESIAN_POINT('Ctrl Pts',(-11.2359873168664,-82.5324799639801,
76.7229153250283));
#114315=CARTESIAN_POINT('Ctrl Pts',(-11.2263351879566,-82.6807503593282,
76.4075549821276));
#114316=CARTESIAN_POINT('Ctrl Pts',(-11.1865296948425,-83.199466595355,
75.0987856006205));
#114317=CARTESIAN_POINT('Ctrl Pts',(-11.1556542565268,-83.3999988110041,
74.0486126652872));
#114318=CARTESIAN_POINT('Ctrl Pts',(-11.126080082656,-83.3999999999947,
72.9888988113141));
#114319=CARTESIAN_POINT('',(-10.4867014633236,-67.603277897842,69.0114834762033));
#114320=CARTESIAN_POINT('Ctrl Pts',(-11.126080082656,-83.3999999999947,
72.9888988113144));
#114321=CARTESIAN_POINT('Ctrl Pts',(-11.1145413077361,-83.400000463896,
72.5754367246302));
#114322=CARTESIAN_POINT('Ctrl Pts',(-11.1030084942769,-83.3694748842814,
72.1625474232924));
#114323=CARTESIAN_POINT('Ctrl Pts',(-11.0793359541153,-83.2483598295159,
71.3479290463103));
#114324=CARTESIAN_POINT('Ctrl Pts',(-11.0674086818258,-83.1584221870653,
70.9472376975009));
#114325=CARTESIAN_POINT('Ctrl Pts',(-11.0345838926802,-82.8268542747668,
69.8521348082208));
#114326=CARTESIAN_POINT('Ctrl Pts',(-11.014410632469,-82.5229520442308,
69.1804710740507));
#114327=CARTESIAN_POINT('Ctrl Pts',(-10.9795609202248,-81.8709899141359,
68.1307930177543));
#114328=CARTESIAN_POINT('Ctrl Pts',(-10.9649269598758,-81.5687066565817,
67.7292622960216));
#114329=CARTESIAN_POINT('Ctrl Pts',(-10.9187102026195,-80.4937138906786,
66.5396188829876));
#114330=CARTESIAN_POINT('Ctrl Pts',(-10.8890682820479,-79.6013444988769,
65.8754091418893));
#114331=CARTESIAN_POINT('Ctrl Pts',(-10.8411103417265,-78.1075663202381,
65.1653414135114));
#114332=CARTESIAN_POINT('Ctrl Pts',(-10.8250822942596,-77.5867180388744,
64.9780354390374));
#114333=CARTESIAN_POINT('Ctrl Pts',(-10.7937856070089,-76.5139839988153,
64.7078973259577));
#114334=CARTESIAN_POINT('Ctrl Pts',(-10.7785899986975,-75.9646383727142,
64.6260880741254));
#114335=CARTESIAN_POINT('Ctrl Pts',(-10.7503632792826,-74.9562112953451,
64.5766577258682));
#114336=CARTESIAN_POINT('Ctrl Pts',(-10.7374549491415,-74.5001098436499,
64.5914093172152));
#114337=CARTESIAN_POINT('Ctrl Pts',(-10.7021819967178,-73.2498417520493,
64.7341073150666));
#114338=CARTESIAN_POINT('Ctrl Pts',(-10.6806528480035,-72.4694504792138,
64.9390080019671));
#114339=CARTESIAN_POINT('Ctrl Pts',(-10.6450022581522,-71.3823104846934,
65.3984426740841));
#114340=CARTESIAN_POINT('Ctrl Pts',(-10.6327525993254,-71.044869025316,
65.568684875407));
#114341=CARTESIAN_POINT('Ctrl Pts',(-10.5965655968264,-70.1050628211244,
66.1251860093398));
#114342=CARTESIAN_POINT('Ctrl Pts',(-10.5724815457644,-69.5389935191861,
66.566396987944));
#114343=CARTESIAN_POINT('Ctrl Pts',(-10.543113335062,-68.8576878872331,
67.2533980030717));
#114344=CARTESIAN_POINT('Ctrl Pts',(-10.5357245337686,-68.6879271709305,
67.4407721722845));
#114345=CARTESIAN_POINT('Ctrl Pts',(-10.5208890369568,-68.3512272796966,
67.8478997193744));
#114346=CARTESIAN_POINT('Ctrl Pts',(-10.5135077658083,-68.1861425191738,
68.0687970134825));
#114347=CARTESIAN_POINT('Ctrl Pts',(-10.4992635891988,-67.8770180063945,
68.5279098299338));
#114348=CARTESIAN_POINT('Ctrl Pts',(-10.4924139281037,-67.733356462548,
68.765962978087));
#114349=CARTESIAN_POINT('Ctrl Pts',(-10.4857110114799,-67.6017555331481,
69.0107015065655));
#114350=CARTESIAN_POINT('Ctrl Pts',(-10.493482781736,-67.6016578275035,
69.0108832153103));
#114351=CARTESIAN_POINT('Ctrl Pts',(-10.4734285229243,-67.2741720795565,
69.61994502055));
#114352=CARTESIAN_POINT('Ctrl Pts',(-10.4540474308237,-67.0231417279012,
70.2671297790049));
#114353=CARTESIAN_POINT('Ctrl Pts',(-10.4253085028645,-66.7701553475053,
71.27181739424));
#114354=CARTESIAN_POINT('Ctrl Pts',(-10.415775127276,-66.7066657642059,
71.6107443794165));
#114355=CARTESIAN_POINT('Ctrl Pts',(-10.3960457754692,-66.6214302894955,
72.2963768901155));
#114356=CARTESIAN_POINT('Ctrl Pts',(-10.3859052190887,-66.600000722933,
72.6424592454741));
#114357=CARTESIAN_POINT('Ctrl Pts',(-10.375811919862,-66.6000000000183,
72.9888718569527));
#114358=CARTESIAN_POINT('Ctrl Pts',(-10.8470411184476,-66.6,72.98888938658));
#114359=CARTESIAN_POINT('Ctrl Pts',(-10.8664020390562,-66.6,72.2994004757708));
#114360=CARTESIAN_POINT('Ctrl Pts',(-10.8868168182513,-66.6848932300671,
71.6119769486083));
#114361=CARTESIAN_POINT('Ctrl Pts',(-10.9317844969506,-67.0668102088584,
70.0917430958867));
#114362=CARTESIAN_POINT('Ctrl Pts',(-10.9552891277897,-67.4123212964733,
69.2799741823665));
#114363=CARTESIAN_POINT('Ctrl Pts',(-10.9944756820166,-68.1382837038421,
68.1186106133782));
#114364=CARTESIAN_POINT('Ctrl Pts',(-11.0089562329978,-68.4357035076209,
67.7245961283561));
#114365=CARTESIAN_POINT('Ctrl Pts',(-11.0553589070755,-69.5146785268516,
66.5298471320123));
#114366=CARTESIAN_POINT('Ctrl Pts',(-11.0850904667867,-70.4213205268241,
65.8584153852941));
#114367=CARTESIAN_POINT('Ctrl Pts',(-11.1329935679342,-71.9148752194113,
65.1578197079955));
#114368=CARTESIAN_POINT('Ctrl Pts',(-11.1484859650805,-72.4174783128085,
64.9780062826356));
#114369=CARTESIAN_POINT('Ctrl Pts',(-11.185933772976,-73.6985502883669,
64.6528906424635));
#114370=CARTESIAN_POINT('Ctrl Pts',(-11.2071539018874,-74.4869117255284,
64.5675243442591));
#114371=CARTESIAN_POINT('Ctrl Pts',(-11.2490784262655,-75.9408195094156,
64.6152465065459));
#114372=CARTESIAN_POINT('Ctrl Pts',(-11.2685950087625,-76.6011304134222,
64.7160749359359));
#114373=CARTESIAN_POINT('Ctrl Pts',(-11.3098734880201,-78.0075842524421,
65.1057089617123));
#114374=CARTESIAN_POINT('Ctrl Pts',(-11.3312503612692,-78.738651161473,
65.4249889856119));
#114375=CARTESIAN_POINT('Ctrl Pts',(-11.3763508683028,-80.0670110840061,
66.2454139502382));
#114376=CARTESIAN_POINT('Ctrl Pts',(-11.3987245609227,-80.6616947373075,
66.7363422965288));
#114377=CARTESIAN_POINT('Ctrl Pts',(-11.4339822674988,-81.5141144062874,
67.6627512081687));
#114378=CARTESIAN_POINT('Ctrl Pts',(-11.4474218230183,-81.8144462479833,
68.0528236096077));
#114379=CARTESIAN_POINT('Ctrl Pts',(-11.47559604091,-82.3515738740102,68.8936705988461));
#114380=CARTESIAN_POINT('Ctrl Pts',(-11.4904764804107,-82.5850359761253,
69.3442130163506));
#114381=CARTESIAN_POINT('Ctrl Pts',(-11.5369186379525,-83.1914900094629,
70.8291880812308));
#114382=CARTESIAN_POINT('Ctrl Pts',(-11.5661250213123,-83.4033109990622,
71.9168916413994));
#114383=CARTESIAN_POINT('Ctrl Pts',(-11.6191785733491,-83.3977024566762,
73.7544760260515));
#114384=CARTESIAN_POINT('Ctrl Pts',(-11.6407895058686,-83.2976786974849,
74.4909279410523));
#114385=CARTESIAN_POINT('Ctrl Pts',(-11.6744017058846,-82.9818552469437,
75.6457821548017));
#114386=CARTESIAN_POINT('Ctrl Pts',(-11.6869510695521,-82.8254210531336,
76.0762625537984));
#114387=CARTESIAN_POINT('Ctrl Pts',(-11.7202337039545,-82.3299737799591,
77.1560894029684));
#114388=CARTESIAN_POINT('Ctrl Pts',(-11.7418620756503,-81.9398414717581,
77.7776918925204));
#114389=CARTESIAN_POINT('Ctrl Pts',(-11.7872345369775,-80.9307048601188,
78.9984197023975));
#114390=CARTESIAN_POINT('Ctrl Pts',(-11.8101222335905,-80.2902003889862,
79.5692736077059));
#114391=CARTESIAN_POINT('Ctrl Pts',(-11.8482492964135,-79.1717122804874,
80.2955831476102));
#114392=CARTESIAN_POINT('Ctrl Pts',(-11.8623691819322,-78.7469382818944,
80.5222429012281));
#114393=CARTESIAN_POINT('Ctrl Pts',(-11.9084582056147,-77.2786902849668,
81.15063602866));
#114394=CARTESIAN_POINT('Ctrl Pts',(-11.9381487200623,-76.1749276675997,
81.3809138810878));
#114395=CARTESIAN_POINT('Ctrl Pts',(-11.9859193414545,-74.5285305330077,
81.3923749598895));
#114396=CARTESIAN_POINT('Ctrl Pts',(-12.0013614799584,-73.9994141424513,
81.3459043724441));
#114397=CARTESIAN_POINT('Ctrl Pts',(-12.0387800059918,-72.7029438625803,
81.107076853382));
#114398=CARTESIAN_POINT('Ctrl Pts',(-12.059962771865,-71.9516445122256,
80.8558430660798));
#114399=CARTESIAN_POINT('Ctrl Pts',(-12.0982159586963,-70.7615118930262,
80.2613730281013));
#114400=CARTESIAN_POINT('Ctrl Pts',(-12.1141384355232,-70.3011839779977,
79.9727953493084));
#114401=CARTESIAN_POINT('Ctrl Pts',(-12.1538537839071,-69.2025439911863,
79.125963032737));
#114402=CARTESIAN_POINT('Ctrl Pts',(-12.1765336606602,-68.6149100195654,
78.5120005903277));
#114403=CARTESIAN_POINT('Ctrl Pts',(-12.2143675660734,-67.8535751690471,
77.4293358979771));
#114404=CARTESIAN_POINT('Ctrl Pts',(-12.2284252541423,-67.612283742812,
77.0151290640062));
#114405=CARTESIAN_POINT('Ctrl Pts',(-12.2600783049814,-67.1431213608927,
76.0239401130097));
#114406=CARTESIAN_POINT('Ctrl Pts',(-12.2773381972661,-66.9411455127516,
75.4377574575907));
#114407=CARTESIAN_POINT('Ctrl Pts',(-12.3030381220826,-66.7377227431684,
74.5346543764784));
#114408=CARTESIAN_POINT('Ctrl Pts',(-12.3115670151115,-66.6866649432039,
74.2310937593356));
#114409=CARTESIAN_POINT('Ctrl Pts',(-12.3292273729659,-66.6174842077814,
73.6144624987546));
#114410=CARTESIAN_POINT('Ctrl Pts',(-12.3383399852619,-66.6000004824736,
73.3018086558167));
#114411=CARTESIAN_POINT('Ctrl Pts',(-12.3474397125752,-66.60000000001,72.9889023383631));
#114412=CARTESIAN_POINT('Origin',(-15.5675364833309,-75.,72.98888938658));
#114413=CARTESIAN_POINT('',(-8.69331175948402,-74.9999999935748,84.9888491626601));
#114414=CARTESIAN_POINT('',(-10.0948640593367,-81.4411229981149,83.1137069660509));
#114415=CARTESIAN_POINT('Ctrl Pts',(-8.69331176731091,-74.99999999459,84.98885921934));
#114416=CARTESIAN_POINT('Ctrl Pts',(-8.69350218303866,-75.3399348100396,
84.98888938658));
#114417=CARTESIAN_POINT('Ctrl Pts',(-8.70999107237271,-75.6865565005233,
84.9744403650337));
#114418=CARTESIAN_POINT('Ctrl Pts',(-8.75917211678321,-76.2144573664476,
84.9285833243014));
#114419=CARTESIAN_POINT('Ctrl Pts',(-8.77964041665495,-76.3917477453332,
84.9092679071993));
#114420=CARTESIAN_POINT('Ctrl Pts',(-8.81645479406493,-76.6593680378655,
84.8739469876302));
#114421=CARTESIAN_POINT('Ctrl Pts',(-8.83638996467051,-76.7935989129425,
84.8546997132077));
#114422=CARTESIAN_POINT('Ctrl Pts',(-8.86232163203638,-76.9508673416978,
84.8294029000445));
#114423=CARTESIAN_POINT('Ctrl Pts',(-8.87692983821257,-77.0352867737512,
84.8150813510417));
#114424=CARTESIAN_POINT('Ctrl Pts',(-8.8839419779519,-77.0747270242531,
84.808187280968));
#114425=CARTESIAN_POINT('Ctrl Pts',(-8.88799666438019,-77.0972749617629,
84.8041960057921));
#114426=CARTESIAN_POINT('Ctrl Pts',(-8.88930142930253,-77.1044975230504,
84.8029110191365));
#114427=CARTESIAN_POINT('Ctrl Pts',(-8.93704494657942,-77.3680116340577,
84.7558764741991));
#114428=CARTESIAN_POINT('Ctrl Pts',(-8.996315423307,-77.646861748394,84.6973356957918));
#114429=CARTESIAN_POINT('Ctrl Pts',(-9.10361335105004,-78.091735186163,
84.584775362276));
#114430=CARTESIAN_POINT('Ctrl Pts',(-9.14244469573966,-78.2444478463605,
84.5431227555126));
#114431=CARTESIAN_POINT('Ctrl Pts',(-9.205289765937,-78.4797206212988,84.4735849437371));
#114432=CARTESIAN_POINT('Ctrl Pts',(-9.2378618143264,-78.5989066168308,
84.4370507663802));
#114433=CARTESIAN_POINT('Ctrl Pts',(-9.27787418570615,-78.740560111277,
84.3911450412213));
#114434=CARTESIAN_POINT('Ctrl Pts',(-9.29838328346071,-78.8120228871968,
84.3673470633219));
#114435=CARTESIAN_POINT('Ctrl Pts',(-9.3095050087037,-78.85047486607,84.3543684906706));
#114436=CARTESIAN_POINT('Ctrl Pts',(-9.31473181782181,-78.868464671978,
84.348248857627));
#114437=CARTESIAN_POINT('Ctrl Pts',(-9.31772754646189,-78.8787556642023,
84.3447364218093));
#114438=CARTESIAN_POINT('Ctrl Pts',(-9.31880032699569,-78.8824378399766,
84.343477834413));
#114439=CARTESIAN_POINT('Ctrl Pts',(-9.34657670740517,-78.9777339923983,
84.3108797837443));
#114440=CARTESIAN_POINT('Ctrl Pts',(-9.37891343386388,-79.0868515499015,
84.2722906472581));
#114441=CARTESIAN_POINT('Ctrl Pts',(-9.43490003601987,-79.2726635673985,
84.202663101968));
#114442=CARTESIAN_POINT('Ctrl Pts',(-9.45480915548319,-79.3382869048505,
84.1774909725898));
#114443=CARTESIAN_POINT('Ctrl Pts',(-9.48654321279514,-79.4421181774566,
84.1364887145665));
#114444=CARTESIAN_POINT('Ctrl Pts',(-9.49743296158528,-79.4776277277984,
84.1222802870086));
#114445=CARTESIAN_POINT('Ctrl Pts',(-9.5198359185379,-79.550419763444,84.0927275962692));
#114446=CARTESIAN_POINT('Ctrl Pts',(-9.53095928417824,-79.5864443608939,
84.0779088489564));
#114447=CARTESIAN_POINT('Ctrl Pts',(-9.59203318603208,-79.7835095778662,
83.9955795484352));
#114448=CARTESIAN_POINT('Ctrl Pts',(-9.63384205469713,-79.9173749817685,
83.9357786815125));
#114449=CARTESIAN_POINT('Ctrl Pts',(-9.68597997846769,-80.0839679014012,
83.8588944861294));
#114450=CARTESIAN_POINT('Ctrl Pts',(-9.70159672318671,-80.1337954519072,
83.8353887160939));
#114451=CARTESIAN_POINT('Ctrl Pts',(-9.72237799545848,-80.2001344713731,
83.8036571761089));
#114452=CARTESIAN_POINT('Ctrl Pts',(-9.73210767039267,-80.231203008154,
83.7886719432529));
#114453=CARTESIAN_POINT('Ctrl Pts',(-9.74230227571295,-80.2638018139171,
83.7727923316102));
#114454=CARTESIAN_POINT('Ctrl Pts',(-9.74711040784735,-80.2791925024508,
83.7652601401528));
#114455=CARTESIAN_POINT('Ctrl Pts',(-9.74910907079229,-80.285594124668,
83.7621201130671));
#114456=CARTESIAN_POINT('Ctrl Pts',(-9.75042774273054,-80.2898187121123,
83.7600464056674));
#114457=CARTESIAN_POINT('Ctrl Pts',(-9.75062835462383,-80.2904612028244,
83.7597313046068));
#114458=CARTESIAN_POINT('Ctrl Pts',(-9.89219342166761,-80.7442018423511,
83.5366773477816));
#114459=CARTESIAN_POINT('Ctrl Pts',(-10.0065728498921,-81.1239733380417,
83.3154687974507));
#114460=CARTESIAN_POINT('Ctrl Pts',(-10.0948640443048,-81.4411228740412,
83.1137067644422));
#114461=CARTESIAN_POINT('',(-10.7325093222838,-83.7451128513012,81.2061270357565));
#114462=CARTESIAN_POINT('Ctrl Pts',(-10.0948643816744,-81.4411242764804,
83.113706293064));
#114463=CARTESIAN_POINT('Ctrl Pts',(-10.1145889408639,-81.5120136748696,
83.0686084401552));
#114464=CARTESIAN_POINT('Ctrl Pts',(-10.134262787638,-81.5824703733078,
83.0227400344558));
#114465=CARTESIAN_POINT('Ctrl Pts',(-10.1538554911333,-81.6524782418569,
82.9761078803152));
#114466=CARTESIAN_POINT('Ctrl Pts',(-10.1630137060671,-81.6852020110595,
82.9543106183625));
#114467=CARTESIAN_POINT('Ctrl Pts',(-10.1721541893806,-81.7178277160856,
82.932346488473));
#114468=CARTESIAN_POINT('Ctrl Pts',(-10.1812743580122,-81.7503538579739,
82.9102160961475));
#114469=CARTESIAN_POINT('Ctrl Pts',(-10.2036036374808,-81.8299889328943,
82.8560333573243));
#114470=CARTESIAN_POINT('Ctrl Pts',(-10.2258097210356,-81.9090267401245,
82.8008544982978));
#114471=CARTESIAN_POINT('Ctrl Pts',(-10.2478613443576,-81.9874661349763,
82.7446731589146));
#114472=CARTESIAN_POINT('Ctrl Pts',(-10.2540851768928,-82.009604807064,
82.7288165826063));
#114473=CARTESIAN_POINT('Ctrl Pts',(-10.2602967017504,-82.0316958025345,
82.7128801399322));
#114474=CARTESIAN_POINT('Ctrl Pts',(-10.2664952398757,-82.0537390094448,
82.6968637096431));
#114475=CARTESIAN_POINT('Ctrl Pts',(-10.2912298513789,-82.1417000977185,
82.6329518367372));
#114476=CARTESIAN_POINT('Ctrl Pts',(-10.3157575691505,-82.2289010075233,
82.5677659776206));
#114477=CARTESIAN_POINT('Ctrl Pts',(-10.34003159336,-82.315327383666,82.5013015554146));
#114478=CARTESIAN_POINT('Ctrl Pts',(-10.3433937280341,-82.3272980859061,
82.4920957337281));
#114479=CARTESIAN_POINT('Ctrl Pts',(-10.346750994044,-82.339253926429,82.4828653808484));
#114480=CARTESIAN_POINT('Ctrl Pts',(-10.3501032905936,-82.3511948681523,
82.4736104792522));
#114481=CARTESIAN_POINT('Ctrl Pts',(-10.3776585818149,-82.4493473202934,
82.397536807088));
#114482=CARTESIAN_POINT('Ctrl Pts',(-10.4048769457379,-82.5464932440241,
82.3198049543937));
#114483=CARTESIAN_POINT('Ctrl Pts',(-10.4317048924259,-82.6426167536869,
82.2403978649875));
#114484=CARTESIAN_POINT('Ctrl Pts',(-10.4585328391139,-82.7387402633496,
82.1609907755813));
#114485=CARTESIAN_POINT('Ctrl Pts',(-10.4849703685669,-82.8338413739666,
82.0799084732329));
#114486=CARTESIAN_POINT('Ctrl Pts',(-10.5109756445671,-82.9278970790637,
81.9971327232997));
#114487=CARTESIAN_POINT('Ctrl Pts',(-10.5129329729522,-82.9349763310343,
81.990902475063));
#114488=CARTESIAN_POINT('Ctrl Pts',(-10.5148878555447,-82.9420496564716,
81.9846626334909));
#114489=CARTESIAN_POINT('Ctrl Pts',(-10.5168402781798,-82.9491170406922,
81.9784131934004));
#114490=CARTESIAN_POINT('Ctrl Pts',(-10.5408279532213,-83.0359476853625,
81.9016318985182));
#114491=CARTESIAN_POINT('Ctrl Pts',(-10.5644444159327,-83.1218817349016,
81.8234018722818));
#114492=CARTESIAN_POINT('Ctrl Pts',(-10.5876709688431,-83.2068866485923,
81.7437172531352));
#114493=CARTESIAN_POINT('Ctrl Pts',(-10.5920344468021,-83.222856175742,
81.728747228067));
#114494=CARTESIAN_POINT('Ctrl Pts',(-10.596384183008,-83.2387929057976,
81.7137258573887));
#114495=CARTESIAN_POINT('Ctrl Pts',(-10.6007198219405,-83.2546967030312,
81.6986530080038));
#114496=CARTESIAN_POINT('Ctrl Pts',(-10.6213409618985,-83.3303382483097,
81.6269636119132));
#114497=CARTESIAN_POINT('Ctrl Pts',(-10.6416433017889,-83.4052350699339,
81.5541098256993));
#114498=CARTESIAN_POINT('Ctrl Pts',(-10.6615921031911,-83.4793719471172,
81.4800761056022));
#114499=CARTESIAN_POINT('Ctrl Pts',(-10.6681626972362,-83.5037906234037,
81.4556914064616));
#114500=CARTESIAN_POINT('Ctrl Pts',(-10.6746950042282,-83.5281267213735,
81.4311787890362));
#114501=CARTESIAN_POINT('Ctrl Pts',(-10.6811897503772,-83.552378548331,
81.4065387716961));
#114502=CARTESIAN_POINT('Ctrl Pts',(-10.6985593874023,-83.617237962661,
81.3406411757519));
#114503=CARTESIAN_POINT('Ctrl Pts',(-10.7156603688218,-83.6814945969358,
81.2738323243309));
#114504=CARTESIAN_POINT('Ctrl Pts',(-10.7325093222788,-83.7451129887462,
81.2061271649026));
#114505=CARTESIAN_POINT('',(-10.728449721964,-86.9999997812556,72.9890778951916));
#114506=CARTESIAN_POINT('Ctrl Pts',(-10.7325093222941,-83.7451125764117,
81.2061267774639));
#114507=CARTESIAN_POINT('Ctrl Pts',(-10.7510222432914,-83.8147824396805,
81.1319806227714));
#114508=CARTESIAN_POINT('Ctrl Pts',(-10.7684192693147,-83.8853352697393,
81.0550084029296));
#114509=CARTESIAN_POINT('Ctrl Pts',(-10.784678148295,-83.9565893449822,
80.9750967182059));
#114510=CARTESIAN_POINT('Ctrl Pts',(-10.8005806758881,-84.0262817203942,
80.8969364850883));
#114511=CARTESIAN_POINT('Ctrl Pts',(-10.8153942348733,-84.0966443465624,
80.8159644628949));
#114512=CARTESIAN_POINT('Ctrl Pts',(-10.829129701094,-84.167505760494,80.7320688051));
#114513=CARTESIAN_POINT('Ctrl Pts',(-10.8366818581569,-84.2064674177918,
80.6859405430965));
#114514=CARTESIAN_POINT('Ctrl Pts',(-10.8439087777216,-84.2455793597819,
80.6389285660367));
#114515=CARTESIAN_POINT('Ctrl Pts',(-10.8508177380832,-84.2848092060794,
80.59101538589));
#114516=CARTESIAN_POINT('Ctrl Pts',(-10.8639725022384,-84.3595034218339,
80.499787972246));
#114517=CARTESIAN_POINT('Ctrl Pts',(-10.8759730630549,-84.4346271026063,
80.4052926427323));
#114518=CARTESIAN_POINT('Ctrl Pts',(-10.8868017876358,-84.5099482633126,
80.3074184901472));
#114519=CARTESIAN_POINT('Ctrl Pts',(-10.8919626453418,-84.5458455464829,
80.2607726852041));
#114520=CARTESIAN_POINT('Ctrl Pts',(-10.8968578239527,-84.5817871757456,
80.2133596100936));
#114521=CARTESIAN_POINT('Ctrl Pts',(-10.9014882826352,-84.6177451464455,
80.1651683767535));
#114522=CARTESIAN_POINT('Ctrl Pts',(-10.9104447521555,-84.687296888652,
80.071954433568));
#114523=CARTESIAN_POINT('Ctrl Pts',(-10.918410184324,-84.7569111066675,
79.9758285647734));
#114524=CARTESIAN_POINT('Ctrl Pts',(-10.9253427541375,-84.8263886683429,
79.8767099737823));
#114525=CARTESIAN_POINT('Ctrl Pts',(-10.9290250056511,-84.8632918461719,
79.8240628903024));
#114526=CARTESIAN_POINT('Ctrl Pts',(-10.9324235557544,-84.9001588458681,
79.7705676777781));
#114527=CARTESIAN_POINT('Ctrl Pts',(-10.9355433881164,-84.9369547938558,
79.7162164675029));
#114528=CARTESIAN_POINT('Ctrl Pts',(-10.9431567626755,-85.0267485076795,
79.5835823790142));
#114529=CARTESIAN_POINT('Ctrl Pts',(-10.9491098324278,-85.1161220781421,
79.4458496824301));
#114530=CARTESIAN_POINT('Ctrl Pts',(-10.9533490201889,-85.2045892224903,
79.3028708304583));
#114531=CARTESIAN_POINT('Ctrl Pts',(-10.9537936745096,-85.213868664729,
79.2878735791283));
#114532=CARTESIAN_POINT('Ctrl Pts',(-10.9542194866345,-85.2231380919539,
79.2728186248596));
#114533=CARTESIAN_POINT('Ctrl Pts',(-10.9546264050554,-85.2323969126946,
79.257705809322));
#114534=CARTESIAN_POINT('Ctrl Pts',(-10.9566325283981,-85.2780432522572,
79.1831990520264));
#114535=CARTESIAN_POINT('Ctrl Pts',(-10.9581789632201,-85.3234320314642,
79.1072859065619));
#114536=CARTESIAN_POINT('Ctrl Pts',(-10.9592926858649,-85.3684954136484,
79.029941852874));
#114537=CARTESIAN_POINT('Ctrl Pts',(-10.9604160766467,-85.4139499874387,
78.9519263816601));
#114538=CARTESIAN_POINT('Ctrl Pts',(-10.9610809172281,-85.4590688918478,
78.8724629550289));
#114539=CARTESIAN_POINT('Ctrl Pts',(-10.9612894216802,-85.5037788116888,
78.7915296637231));
#114540=CARTESIAN_POINT('Ctrl Pts',(-10.9614870058926,-85.5461470882778,
78.7148351833147));
#114541=CARTESIAN_POINT('Ctrl Pts',(-10.9612749276812,-85.5881481125788,
78.6368206735561));
#114542=CARTESIAN_POINT('Ctrl Pts',(-10.960650954875,-85.6297120799806,
78.5574804832683));
#114543=CARTESIAN_POINT('Ctrl Pts',(-10.9600140200044,-85.672139474149,
78.4764921239476));
#114544=CARTESIAN_POINT('Ctrl Pts',(-10.9589490660722,-85.7141130952747,
78.3941194696662));
#114545=CARTESIAN_POINT('Ctrl Pts',(-10.9574560783488,-85.7555582591477,
78.3103522147957));
#114546=CARTESIAN_POINT('Ctrl Pts',(-10.9574460434946,-85.7558368255226,
78.3097891879347));
#114547=CARTESIAN_POINT('Ctrl Pts',(-10.9574359893214,-85.7561153680064,
78.3092260980831));
#114548=CARTESIAN_POINT('Ctrl Pts',(-10.9574259158265,-85.7563938865775,
78.3086629452375));
#114549=CARTESIAN_POINT('Ctrl Pts',(-10.956671510735,-85.7772521716685,
78.2664883693699));
#114550=CARTESIAN_POINT('Ctrl Pts',(-10.9558086563518,-85.7979763919999,
78.2239604082909));
#114551=CARTESIAN_POINT('Ctrl Pts',(-10.9548373526965,-85.8185569657927,
78.1810781497251));
#114552=CARTESIAN_POINT('Ctrl Pts',(-10.9543517008688,-85.8288472526891,
78.1596370204423));
#114553=CARTESIAN_POINT('Ctrl Pts',(-10.9538389367222,-85.8391016262828,
78.138107315856));
#114554=CARTESIAN_POINT('Ctrl Pts',(-10.953299060256,-85.8493188733959,
78.116488926769));
#114555=CARTESIAN_POINT('Ctrl Pts',(-10.953029122023,-85.8544274969525,
78.1056797322255));
#114556=CARTESIAN_POINT('Ctrl Pts',(-10.95275240571,-85.8595268387752,78.0948483664995));
#114557=CARTESIAN_POINT('Ctrl Pts',(-10.9524689113171,-85.8646167459357,
78.0839948168531));
#114558=CARTESIAN_POINT('Ctrl Pts',(-10.9521854169241,-85.8697066530963,
78.0731412672067));
#114559=CARTESIAN_POINT('Ctrl Pts',(-10.9518650103282,-85.8753015385961,
78.0611599992563));
#114560=CARTESIAN_POINT('Ctrl Pts',(-10.9515980938983,-85.8798580098567,
78.0513676035743));
#114561=CARTESIAN_POINT('Ctrl Pts',(-10.9493307066674,-85.9185640751157,
77.968183691148));
#114562=CARTESIAN_POINT('Ctrl Pts',(-10.9466840767295,-85.9568853712228,
77.8833334794079));
#114563=CARTESIAN_POINT('Ctrl Pts',(-10.9436635797958,-85.9947243643778,
77.7968032951168));
#114564=CARTESIAN_POINT('Ctrl Pts',(-10.9409949187626,-86.0281557661588,
77.7203523878379));
#114565=CARTESIAN_POINT('Ctrl Pts',(-10.9380346094849,-86.061210580883,
77.6425901674792));
#114566=CARTESIAN_POINT('Ctrl Pts',(-10.934777888651,-86.0938213085787,
77.5635061522729));
#114567=CARTESIAN_POINT('Ctrl Pts',(-10.9313064850056,-86.1285817331826,
77.4792089242683));
#114568=CARTESIAN_POINT('Ctrl Pts',(-10.9275010633154,-86.1628371480715,
77.3934109785441));
#114569=CARTESIAN_POINT('Ctrl Pts',(-10.9233616235826,-86.1965015630842,
77.306104556324));
#114570=CARTESIAN_POINT('Ctrl Pts',(-10.9221879091295,-86.206046915356,
77.2813493198119));
#114571=CARTESIAN_POINT('Ctrl Pts',(-10.9209875019718,-86.2155447536471,
77.2564727659167));
#114572=CARTESIAN_POINT('Ctrl Pts',(-10.9197600577454,-86.2249930310364,
77.2314748551298));
#114573=CARTESIAN_POINT('Ctrl Pts',(-10.9188230353986,-86.2322057799839,
77.2123916246859));
#114574=CARTESIAN_POINT('Ctrl Pts',(-10.9178702559755,-86.2393896458739,
77.1932376718965));
#114575=CARTESIAN_POINT('Ctrl Pts',(-10.9169019504432,-86.2465437460638,
77.1740128936221));
#114576=CARTESIAN_POINT('Ctrl Pts',(-10.9157835859962,-86.2548065216399,
77.1518088394203));
#114577=CARTESIAN_POINT('Ctrl Pts',(-10.9146443454205,-86.2630295774941,
77.1295103433876));
#114578=CARTESIAN_POINT('Ctrl Pts',(-10.9134842287163,-86.2712115153925,
77.1071173363896));
#114579=CARTESIAN_POINT('Ctrl Pts',(-10.9129041703643,-86.2753024843418,
77.0959208328907));
#114580=CARTESIAN_POINT('Ctrl Pts',(-10.9123188929802,-86.2793831737303,
77.0847007016266));
#114581=CARTESIAN_POINT('Ctrl Pts',(-10.911728396564,-86.2834534078366,
77.0734569352409));
#114582=CARTESIAN_POINT('Ctrl Pts',(-10.911433148356,-86.2854885248897,
77.0678350520481));
#114583=CARTESIAN_POINT('Ctrl Pts',(-10.9111365953899,-86.287521028118,
77.0622072600734));
#114584=CARTESIAN_POINT('Ctrl Pts',(-10.9108387376659,-86.289550895496,
77.056573558484));
#114585=CARTESIAN_POINT('Ctrl Pts',(-10.9105408799419,-86.291580762874,
77.0509398568946));
#114586=CARTESIAN_POINT('Ctrl Pts',(-10.9101335854462,-86.2943365970394,
77.0432685379285));
#114587=CARTESIAN_POINT('Ctrl Pts',(-10.9099412502199,-86.2956325680269,
77.0396547240619));
#114588=CARTESIAN_POINT('Ctrl Pts',(-10.907803220588,-86.3100387921298,
76.9994829818475));
#114589=CARTESIAN_POINT('Ctrl Pts',(-10.9052699371439,-86.326228168735,
76.95367723549));
#114590=CARTESIAN_POINT('Ctrl Pts',(-10.9023364899602,-86.3439953687665,
76.9021729235994));
#114591=CARTESIAN_POINT('Ctrl Pts',(-10.8994201604487,-86.3616588910807,
76.8509691570665));
#114592=CARTESIAN_POINT('Ctrl Pts',(-10.896107836887,-86.3808818716695,
76.7941329967364));
#114593=CARTESIAN_POINT('Ctrl Pts',(-10.8923984096102,-86.4014134015565,
76.7315870902248));
#114594=CARTESIAN_POINT('Ctrl Pts',(-10.8898341614871,-86.4156064111637,
76.6883504363129));
#114595=CARTESIAN_POINT('Ctrl Pts',(-10.8870802112116,-86.4304237153378,
76.6423849924677));
#114596=CARTESIAN_POINT('Ctrl Pts',(-10.8841392492642,-86.4457685531813,
76.5936618749884));
#114597=CARTESIAN_POINT('Ctrl Pts',(-10.8832950114274,-86.4501734699867,
76.5796753290774));
#114598=CARTESIAN_POINT('Ctrl Pts',(-10.8824353843272,-86.4546217860028,
76.5654615226593));
#114599=CARTESIAN_POINT('Ctrl Pts',(-10.8815605246739,-86.4591110286805,
76.5510197661022));
#114600=CARTESIAN_POINT('Ctrl Pts',(-10.8773404009239,-86.4807661130926,
76.4813560210649));
#114601=CARTESIAN_POINT('Ctrl Pts',(-10.8727620467592,-86.5033764055256,
76.4063902509679));
#114602=CARTESIAN_POINT('Ctrl Pts',(-10.8678183023178,-86.5266369525449,
76.3260472126269));
#114603=CARTESIAN_POINT('Ctrl Pts',(-10.8652847021162,-86.5385576590697,
76.2848725239761));
#114604=CARTESIAN_POINT('Ctrl Pts',(-10.8626555235647,-86.5506484475054,
76.242285489306));
#114605=CARTESIAN_POINT('Ctrl Pts',(-10.8599327538662,-86.5628637872285,
76.1982758449494));
#114606=CARTESIAN_POINT('Ctrl Pts',(-10.8559149361761,-86.5808891854308,
76.1333336180234));
#114607=CARTESIAN_POINT('Ctrl Pts',(-10.8516905238557,-86.5991864130687,
76.0652937708498));
#114608=CARTESIAN_POINT('Ctrl Pts',(-10.847259516825,-86.6175965484567,
75.9941250065181));
#114609=CARTESIAN_POINT('Ctrl Pts',(-10.8450440133097,-86.6268016161507,
75.9585406243523));
#114610=CARTESIAN_POINT('Ctrl Pts',(-10.8427768611176,-86.6360346768941,
75.922174040174));
#114611=CARTESIAN_POINT('Ctrl Pts',(-10.8404580602521,-86.6452744508845,
75.8850215613659));
#114612=CARTESIAN_POINT('Ctrl Pts',(-10.8399932126182,-86.6471267389101,
75.8775736420024));
#114613=CARTESIAN_POINT('Ctrl Pts',(-10.8395262919422,-86.648979293872,
75.8700941390403));
#114614=CARTESIAN_POINT('Ctrl Pts',(-10.83905729361,-86.6508319396637,75.8625830239116));
#114615=CARTESIAN_POINT('Ctrl Pts',(-10.8383565390388,-86.6536000731901,
75.8513602798226));
#114616=CARTESIAN_POINT('Ctrl Pts',(-10.8376511456282,-86.6563684098304,
75.8400669618679));
#114617=CARTESIAN_POINT('Ctrl Pts',(-10.8369411224503,-86.6591363571076,
75.8287029780982));
#114618=CARTESIAN_POINT('Ctrl Pts',(-10.8358316521156,-86.6634615051979,
75.8109458072505));
#114619=CARTESIAN_POINT('Ctrl Pts',(-10.8346490644395,-86.6680217558641,
75.792028396447));
#114620=CARTESIAN_POINT('Ctrl Pts',(-10.8335669198333,-86.67215187099,75.7747240707307));
#114621=CARTESIAN_POINT('Ctrl Pts',(-10.833493031196,-86.6724338745012,
75.7735425345117));
#114622=CARTESIAN_POINT('Ctrl Pts',(-10.833419610159,-86.67271389208,75.7723685240432));
#114623=CARTESIAN_POINT('Ctrl Pts',(-10.8333467116477,-86.6729917202779,
75.771202924429));
#114624=CARTESIAN_POINT('Ctrl Pts',(-10.82650931042,-86.6990501791833,75.6618773416835));
#114625=CARTESIAN_POINT('Ctrl Pts',(-10.8200333262671,-86.7226942142122,
75.5558789242882));
#114626=CARTESIAN_POINT('Ctrl Pts',(-10.8139542169689,-86.7442167453786,
75.4533141127769));
#114627=CARTESIAN_POINT('Ctrl Pts',(-10.8076212434149,-86.7666380597528,
75.3464661837463));
#114628=CARTESIAN_POINT('Ctrl Pts',(-10.8017186737899,-86.7867571708465,
75.2433446321614));
#114629=CARTESIAN_POINT('Ctrl Pts',(-10.7962391680734,-86.8048850275004,
75.1440468283543));
#114630=CARTESIAN_POINT('Ctrl Pts',(-10.7947405931986,-86.8098427649171,
75.1168901464188));
#114631=CARTESIAN_POINT('Ctrl Pts',(-10.7932734134942,-86.814651444266,
75.0900193350083));
#114632=CARTESIAN_POINT('Ctrl Pts',(-10.7918369460471,-86.8193171491601,
75.0634361046744));
#114633=CARTESIAN_POINT('Ctrl Pts',(-10.7901112142961,-86.824922396319,
75.0314997564292));
#114634=CARTESIAN_POINT('Ctrl Pts',(-10.7884297963389,-86.8303212963133,
74.9999784843577));
#114635=CARTESIAN_POINT('Ctrl Pts',(-10.7867896150128,-86.8355242020625,
74.9688754749133));
#114636=CARTESIAN_POINT('Ctrl Pts',(-10.7811928432361,-86.8532780171989,
74.8627430353731));
#114637=CARTESIAN_POINT('Ctrl Pts',(-10.7761184458931,-86.8687532514872,
74.7614793995783));
#114638=CARTESIAN_POINT('Ctrl Pts',(-10.77156743064,-86.8823386801257,74.6651789381298));
#114639=CARTESIAN_POINT('Ctrl Pts',(-10.7709185994682,-86.8842755335735,
74.6514495310024));
#114640=CARTESIAN_POINT('Ctrl Pts',(-10.7702803824442,-86.8861739133072,
74.6378209491359));
#114641=CARTESIAN_POINT('Ctrl Pts',(-10.7696527601112,-86.8880348839046,
74.6242934129354));
#114642=CARTESIAN_POINT('Ctrl Pts',(-10.7671378225696,-86.8954919557344,
74.5700873930946));
#114643=CARTESIAN_POINT('Ctrl Pts',(-10.7647934875938,-86.9023486428634,
74.5175042618523));
#114644=CARTESIAN_POINT('Ctrl Pts',(-10.7626197553063,-86.9086708213643,
74.4665573115567));
#114645=CARTESIAN_POINT('Ctrl Pts',(-10.7615328891625,-86.9118319106148,
74.4410838364088));
#114646=CARTESIAN_POINT('Ctrl Pts',(-10.7604886736913,-86.9148593057109,
74.4160193984485));
#114647=CARTESIAN_POINT('Ctrl Pts',(-10.7594871088829,-86.9177608650203,
74.3913654171809));
#114648=CARTESIAN_POINT('Ctrl Pts',(-10.7589863264787,-86.919211644675,
74.379038426547));
#114649=CARTESIAN_POINT('Ctrl Pts',(-10.7584962067405,-86.9206309612238,
74.3668140495618));
#114650=CARTESIAN_POINT('Ctrl Pts',(-10.7580167496668,-86.9220197725852,
74.3546924568402));
#114651=CARTESIAN_POINT('Ctrl Pts',(-10.7577770211299,-86.9227141782659,
74.3486316604794));
#114652=CARTESIAN_POINT('Ctrl Pts',(-10.7575399582592,-86.9234009573923,
74.3425965601559));
#114653=CARTESIAN_POINT('Ctrl Pts',(-10.7573055610544,-86.9240802282338,
74.336587176387));
#114654=CARTESIAN_POINT('Ctrl Pts',(-10.7570711638495,-86.9247594990753,
74.3305777926182));
#114655=CARTESIAN_POINT('Ctrl Pts',(-10.7568941569512,-86.9252725409332,
74.3260174959602));
#114656=CARTESIAN_POINT('Ctrl Pts',(-10.7566103664373,-86.9260956331663,
74.3186361949689));
#114657=CARTESIAN_POINT('Ctrl Pts',(-10.7557717398522,-86.9285279450123,
74.2968237842595));
#114658=CARTESIAN_POINT('Ctrl Pts',(-10.7549515907162,-86.9308930137454,
74.275070955312));
#114659=CARTESIAN_POINT('Ctrl Pts',(-10.754150066911,-86.933191857729,74.2533782531655));
#114660=CARTESIAN_POINT('Ctrl Pts',(-10.7479305549346,-86.9510299900418,
74.085051348921));
#114661=CARTESIAN_POINT('Ctrl Pts',(-10.7428350444671,-86.9648824251588,
73.9203479344601));
#114662=CARTESIAN_POINT('Ctrl Pts',(-10.7388723178175,-86.9752360679132,
73.7594344127732));
#114663=CARTESIAN_POINT('Ctrl Pts',(-10.7365822146096,-86.9812195516561,
73.6664407231237));
#114664=CARTESIAN_POINT('Ctrl Pts',(-10.73466985067,-86.9860341006921,73.5747120535647));
#114665=CARTESIAN_POINT('Ctrl Pts',(-10.7331325040884,-86.9897703599552,
73.4842749393781));
#114666=CARTESIAN_POINT('Ctrl Pts',(-10.7305698086316,-86.9959985551799,
73.3335198758081));
#114667=CARTESIAN_POINT('Ctrl Pts',(-10.7290511142392,-86.9992315626732,
73.1863560058278));
#114668=CARTESIAN_POINT('Ctrl Pts',(-10.7285784258043,-86.9998778669969,
73.0429165819694));
#114669=CARTESIAN_POINT('Ctrl Pts',(-10.728519092563,-86.9999589930147,
73.0249116440121));
#114670=CARTESIAN_POINT('Ctrl Pts',(-10.7284762009538,-86.9999993368467,
73.0069653406822));
#114671=CARTESIAN_POINT('Ctrl Pts',(-10.7284497219417,-86.9999996839437,
72.9890778951898));
#114672=CARTESIAN_POINT('',(-10.7325538919673,-83.7450248445335,64.7715579422181));
#114673=CARTESIAN_POINT('Ctrl Pts',(-10.7284497219764,-86.9999998242331,
72.9890778951925));
#114674=CARTESIAN_POINT('Ctrl Pts',(-10.7284888747654,-87.0000012631274,
72.8882010561864));
#114675=CARTESIAN_POINT('Ctrl Pts',(-10.7291051326801,-86.9987315794751,
72.7849150495473));
#114676=CARTESIAN_POINT('Ctrl Pts',(-10.7302920457223,-86.996004952873,
72.6792651291966));
#114677=CARTESIAN_POINT('Ctrl Pts',(-10.7319888110209,-86.992107072206,
72.5282320608291));
#114678=CARTESIAN_POINT('Ctrl Pts',(-10.7348512590662,-86.9852332530932,
72.3723668347754));
#114679=CARTESIAN_POINT('Ctrl Pts',(-10.7389002092034,-86.9748130428885,
72.2117979770313));
#114680=CARTESIAN_POINT('Ctrl Pts',(-10.7395319821845,-86.9731871381373,
72.1867438117535));
#114681=CARTESIAN_POINT('Ctrl Pts',(-10.7401926355456,-86.9714748188675,
72.1615752029785));
#114682=CARTESIAN_POINT('Ctrl Pts',(-10.7408822399634,-86.9696738375772,
72.1362927230114));
#114683=CARTESIAN_POINT('Ctrl Pts',(-10.7426464435455,-86.9650664169143,
72.071612972457));
#114684=CARTESIAN_POINT('Ctrl Pts',(-10.7446002347412,-86.9598787695624,
72.00618781155));
#114685=CARTESIAN_POINT('Ctrl Pts',(-10.7467361926647,-86.9540740543932,
71.9400335061946));
#114686=CARTESIAN_POINT('Ctrl Pts',(-10.7509385308377,-86.9426537095119,
71.8098798362008));
#114687=CARTESIAN_POINT('Ctrl Pts',(-10.7558549933362,-86.9288446840852,
71.676888006109));
#114688=CARTESIAN_POINT('Ctrl Pts',(-10.7615098162251,-86.9123520250915,
71.5411743141284));
#114689=CARTESIAN_POINT('Ctrl Pts',(-10.7639724035918,-86.9051697287615,
71.482073113272));
#114690=CARTESIAN_POINT('Ctrl Pts',(-10.7665748213442,-86.8974782983634,
71.4224562468907));
#114691=CARTESIAN_POINT('Ctrl Pts',(-10.7693103288981,-86.889252545791,
71.3623303350626));
#114692=CARTESIAN_POINT('Ctrl Pts',(-10.7738188465192,-86.875695299215,
71.2632340146852));
#114693=CARTESIAN_POINT('Ctrl Pts',(-10.7787004449165,-86.8606874728627,
71.1627601820488));
#114694=CARTESIAN_POINT('Ctrl Pts',(-10.7839551238006,-86.8441164950172,
71.0609588802453));
#114695=CARTESIAN_POINT('Ctrl Pts',(-10.7865824632427,-86.8358310060945,
71.0100582293435));
#114696=CARTESIAN_POINT('Ctrl Pts',(-10.7893030728237,-86.8271546776825,
70.958825719308));
#114697=CARTESIAN_POINT('Ctrl Pts',(-10.7921169525352,-86.8180732504146,
70.907268334575));
#114698=CARTESIAN_POINT('Ctrl Pts',(-10.7924606326094,-86.8169640681049,
70.9009712474106));
#114699=CARTESIAN_POINT('Ctrl Pts',(-10.7928057051129,-86.8158488425891,
70.8946693145837));
#114700=CARTESIAN_POINT('Ctrl Pts',(-10.7931521683829,-86.8147275475862,
70.8883625482581));
#114701=CARTESIAN_POINT('Ctrl Pts',(-10.7942240386725,-86.8112585426332,
70.8688509981639));
#114702=CARTESIAN_POINT('Ctrl Pts',(-10.7953092216315,-86.8077314450951,
70.849293184582));
#114703=CARTESIAN_POINT('Ctrl Pts',(-10.7964077247073,-86.8041454871649,
70.8296894990121));
#114704=CARTESIAN_POINT('Ctrl Pts',(-10.7971345121707,-86.801772959199,
70.8167193824761));
#114705=CARTESIAN_POINT('Ctrl Pts',(-10.7978671290185,-86.7993746656645,
70.8037291852011));
#114706=CARTESIAN_POINT('Ctrl Pts',(-10.7986055752513,-86.7969503833673,
70.7907190216704));
#114707=CARTESIAN_POINT('Ctrl Pts',(-10.7992908472177,-86.7947006695452,
70.7786456980492));
#114708=CARTESIAN_POINT('Ctrl Pts',(-10.7998987965539,-86.7927000493644,
70.7679895228104));
#114709=CARTESIAN_POINT('Ctrl Pts',(-10.8006586536161,-86.7901926376231,
70.7547573980053));
#114710=CARTESIAN_POINT('Ctrl Pts',(-10.800717615377,-86.7899980728568,
70.7537306399234));
#114711=CARTESIAN_POINT('Ctrl Pts',(-10.800777495232,-86.789800431358,70.7526883773526));
#114712=CARTESIAN_POINT('Ctrl Pts',(-10.8008384021056,-86.7895993463446,
70.7516287476968));
#114713=CARTESIAN_POINT('Ctrl Pts',(-10.8119753799017,-86.7528304367686,
70.5578727519031));
#114714=CARTESIAN_POINT('Ctrl Pts',(-10.823335768474,-86.7112853942037,
70.3650224851882));
#114715=CARTESIAN_POINT('Ctrl Pts',(-10.8349247208416,-86.6650136200905,
70.1733140719098));
#114716=CARTESIAN_POINT('Ctrl Pts',(-10.8374182920251,-86.6550574170725,
70.1320645646358));
#114717=CARTESIAN_POINT('Ctrl Pts',(-10.8399224267147,-86.6448823906394,
70.0908679706403));
#114718=CARTESIAN_POINT('Ctrl Pts',(-10.8424365917833,-86.6344890661378,
70.0497263415853));
#114719=CARTESIAN_POINT('Ctrl Pts',(-10.8495360058733,-86.6051407487454,
69.9335520041667));
#114720=CARTESIAN_POINT('Ctrl Pts',(-10.8567186108653,-86.5740520420787,
69.8178173284099));
#114721=CARTESIAN_POINT('Ctrl Pts',(-10.8639844065654,-86.5412369311502,
69.7025742433079));
#114722=CARTESIAN_POINT('Ctrl Pts',(-10.8676173044154,-86.5248293756859,
69.644952700757));
#114723=CARTESIAN_POINT('Ctrl Pts',(-10.8712709999796,-86.5079902361993,
69.5874540509201));
#114724=CARTESIAN_POINT('Ctrl Pts',(-10.8749454933449,-86.4907214240387,
69.5300847389974));
#114725=CARTESIAN_POINT('Ctrl Pts',(-10.8767827400276,-86.4820870179584,
69.5014000830361));
#114726=CARTESIAN_POINT('Ctrl Pts',(-10.8786251861658,-86.4733451959164,
69.4727477609269));
#114727=CARTESIAN_POINT('Ctrl Pts',(-10.8804728317814,-86.4644962125682,
69.4441285732381));
#114728=CARTESIAN_POINT('Ctrl Pts',(-10.8807324272481,-86.4632529243844,
69.4401075578871));
#114729=CARTESIAN_POINT('Ctrl Pts',(-10.8809947516596,-86.4619951972876,
69.4360473607439));
#114730=CARTESIAN_POINT('Ctrl Pts',(-10.8812586851527,-86.4607281333618,
69.4319648057151));
#114731=CARTESIAN_POINT('Ctrl Pts',(-10.8826244528261,-86.4541715007429,
69.4108389470075));
#114732=CARTESIAN_POINT('Ctrl Pts',(-10.8840327498243,-86.4473607879374,
69.3891157686244));
#114733=CARTESIAN_POINT('Ctrl Pts',(-10.8853325786385,-86.4410332420026,
69.3691163789735));
#114734=CARTESIAN_POINT('Ctrl Pts',(-10.8855693856182,-86.4398804694023,
69.3654728260624));
#114735=CARTESIAN_POINT('Ctrl Pts',(-10.8858026112128,-86.4387438659352,
69.3618864423125));
#114736=CARTESIAN_POINT('Ctrl Pts',(-10.8860313670693,-86.4376280585935,
69.3583712056871));
#114737=CARTESIAN_POINT('Ctrl Pts',(-10.8956823808273,-86.3905531020374,
69.2100663816831));
#114738=CARTESIAN_POINT('Ctrl Pts',(-10.904504945182,-86.3398056888968,
69.0601907694884));
#114739=CARTESIAN_POINT('Ctrl Pts',(-10.9125092853346,-86.2851319634432,
68.9089620111517));
#114740=CARTESIAN_POINT('Ctrl Pts',(-10.9157955212498,-86.2626852961636,
68.8468740229391));
#114741=CARTESIAN_POINT('Ctrl Pts',(-10.9189433001879,-86.2395768797012,
68.784558218495));
#114742=CARTESIAN_POINT('Ctrl Pts',(-10.9219509878368,-86.2157892384658,
68.722030682055));
#114743=CARTESIAN_POINT('Ctrl Pts',(-10.9221051116491,-86.2145702814525,
68.7188265653326));
#114744=CARTESIAN_POINT('Ctrl Pts',(-10.9222588672882,-86.2133495408695,
68.7156218927447));
#114745=CARTESIAN_POINT('Ctrl Pts',(-10.9224122547845,-86.2121270144323,
68.712416666541));
#114746=CARTESIAN_POINT('Ctrl Pts',(-10.9276310461364,-86.1705322915913,
68.6033634047605));
#114747=CARTESIAN_POINT('Ctrl Pts',(-10.9324274924053,-86.1268703731123,
68.4936690105705));
#114748=CARTESIAN_POINT('Ctrl Pts',(-10.9368015932311,-86.0810510568632,
68.3834248233145));
#114749=CARTESIAN_POINT('Ctrl Pts',(-10.938988643644,-86.0581413987386,
68.3283027296865));
#114750=CARTESIAN_POINT('Ctrl Pts',(-10.9410701077568,-86.0346923515679,
68.2730432024122));
#114751=CARTESIAN_POINT('Ctrl Pts',(-10.9430459856038,-86.0106927200718,
68.2176584839966));
#114752=CARTESIAN_POINT('Ctrl Pts',(-10.9440339245274,-85.9986929043237,
68.1899661247888));
#114753=CARTESIAN_POINT('Ctrl Pts',(-10.9449954668838,-85.9865554403056,
68.1622424687455));
#114754=CARTESIAN_POINT('Ctrl Pts',(-10.9459306126711,-85.9742789254811,
68.1344890742454));
#114755=CARTESIAN_POINT('Ctrl Pts',(-10.9463981855648,-85.9681406680688,
68.1206123769953));
#114756=CARTESIAN_POINT('Ctrl Pts',(-10.946859159316,-85.9619676478248,
68.1067282451965));
#114757=CARTESIAN_POINT('Ctrl Pts',(-10.9473135339246,-85.9557596898088,
68.0928368765541));
#114758=CARTESIAN_POINT('Ctrl Pts',(-10.9475407212289,-85.9526557108008,
68.0858911922329));
#114759=CARTESIAN_POINT('Ctrl Pts',(-10.9477662587475,-85.9495429973423,
68.0789436987048));
#114760=CARTESIAN_POINT('Ctrl Pts',(-10.9479901464804,-85.946421527598,
68.0719944208737));
#114761=CARTESIAN_POINT('Ctrl Pts',(-10.94816823117,-85.943938649401,68.066466829122));
#114762=CARTESIAN_POINT('Ctrl Pts',(-10.9483711709324,-85.9410850462583,
68.0601277871563));
#114763=CARTESIAN_POINT('Ctrl Pts',(-10.9485371095389,-85.9387319835289,
68.0549110128396));
#114764=CARTESIAN_POINT('Ctrl Pts',(-10.9485797886327,-85.9381267802728,
68.053569268413));
#114765=CARTESIAN_POINT('Ctrl Pts',(-10.9486200425959,-85.9375547496877,
68.0523017345745));
#114766=CARTESIAN_POINT('Ctrl Pts',(-10.9486568603221,-85.9370308276724,
68.0511412594396));
#114767=CARTESIAN_POINT('Ctrl Pts',(-10.9535290566002,-85.8676987107813,
67.8975722255995));
#114768=CARTESIAN_POINT('Ctrl Pts',(-10.9571237516371,-85.796390348302,
67.7482490038176));
#114769=CARTESIAN_POINT('Ctrl Pts',(-10.9593857595805,-85.7235058471837,
67.6031289566081));
#114770=CARTESIAN_POINT('Ctrl Pts',(-10.9602457587846,-85.6957956823561,
67.547955355002));
#114771=CARTESIAN_POINT('Ctrl Pts',(-10.9609134980145,-85.6678573736214,
67.4933890699717));
#114772=CARTESIAN_POINT('Ctrl Pts',(-10.9613872778227,-85.6397117577135,
67.4394269159064));
#114773=CARTESIAN_POINT('Ctrl Pts',(-10.9626755897398,-85.5631776130193,
67.2926919032226));
#114774=CARTESIAN_POINT('Ctrl Pts',(-10.9625276751357,-85.4851133229949,
67.1504256856112));
#114775=CARTESIAN_POINT('Ctrl Pts',(-10.9609574725558,-85.4059328878418,
67.0125566511054));
#114776=CARTESIAN_POINT('Ctrl Pts',(-10.9604607636164,-85.3808854000432,
66.9689439461118));
#114777=CARTESIAN_POINT('Ctrl Pts',(-10.9598219500033,-85.3557259460709,
66.9257710771614));
#114778=CARTESIAN_POINT('Ctrl Pts',(-10.9590420630014,-85.3304668763377,
66.8830352992811));
#114779=CARTESIAN_POINT('Ctrl Pts',(-10.9566133192741,-85.2518044457246,
66.7499464643508));
#114780=CARTESIAN_POINT('Ctrl Pts',(-10.9528135993784,-85.1721785314414,
66.6210980796646));
#114781=CARTESIAN_POINT('Ctrl Pts',(-10.9476408198054,-85.0919519597182,
66.496393328091));
#114782=CARTESIAN_POINT('Ctrl Pts',(-10.9461366559269,-85.0686233199461,
66.4601311251219));
#114783=CARTESIAN_POINT('Ctrl Pts',(-10.9445166201651,-85.0452436680095,
66.4242191730408));
#114784=CARTESIAN_POINT('Ctrl Pts',(-10.9427812044943,-85.0218213848203,
66.3886548154653));
#114785=CARTESIAN_POINT('Ctrl Pts',(-10.9388414051909,-84.9686473259792,
66.3079154090165));
#114786=CARTESIAN_POINT('Ctrl Pts',(-10.9343065299015,-84.9152540838332,
66.2289677825578));
#114787=CARTESIAN_POINT('Ctrl Pts',(-10.9291847863793,-84.8617440602333,
66.151785527885));
#114788=CARTESIAN_POINT('Ctrl Pts',(-10.9246671423073,-84.8145454373701,
66.083706766469));
#114789=CARTESIAN_POINT('Ctrl Pts',(-10.9196756195247,-84.7672558795174,
66.017001426963));
#114790=CARTESIAN_POINT('Ctrl Pts',(-10.9142209171807,-84.71993740355,65.9516443212193));
#114791=CARTESIAN_POINT('Ctrl Pts',(-10.9052079494621,-84.6417516714083,
65.8436528219419));
#114792=CARTESIAN_POINT('Ctrl Pts',(-10.8949278585239,-84.5634888687763,
65.7393427125517));
#114793=CARTESIAN_POINT('Ctrl Pts',(-10.8833752888633,-84.4854095252617,
65.6385828033828));
#114794=CARTESIAN_POINT('Ctrl Pts',(-10.8806126706233,-84.4667380586618,
65.6144876305245));
#114795=CARTESIAN_POINT('Ctrl Pts',(-10.8777774550046,-84.4480769262614,
65.590595431077));
#114796=CARTESIAN_POINT('Ctrl Pts',(-10.8748698783256,-84.4294294000177,
65.5669043282896));
#114797=CARTESIAN_POINT('Ctrl Pts',(-10.8628804971574,-84.3525363978144,
65.4692141577535));
#114798=CARTESIAN_POINT('Ctrl Pts',(-10.8496579766825,-84.2758777732863,
65.3749443449109));
#114799=CARTESIAN_POINT('Ctrl Pts',(-10.8352182645738,-84.1996939182158,
65.283979980599));
#114800=CARTESIAN_POINT('Ctrl Pts',(-10.832318642333,-84.1843955245298,
65.2657135295859));
#114801=CARTESIAN_POINT('Ctrl Pts',(-10.8293700476068,-84.1691161545344,
65.2475803268386));
#114802=CARTESIAN_POINT('Ctrl Pts',(-10.8263727699115,-84.153857575543,
65.2295793819169));
#114803=CARTESIAN_POINT('Ctrl Pts',(-10.8122899682069,-84.0821646714902,
65.1450013869506));
#114804=CARTESIAN_POINT('Ctrl Pts',(-10.7971290892607,-84.0109333643218,
65.0633439925102));
#114805=CARTESIAN_POINT('Ctrl Pts',(-10.7808637979447,-83.9403515843494,
64.9845085897367));
#114806=CARTESIAN_POINT('Ctrl Pts',(-10.7774480386293,-83.9255292016602,
64.9679529218317));
#114807=CARTESIAN_POINT('Ctrl Pts',(-10.7739837140888,-83.91073535137,64.9515216712212));
#114808=CARTESIAN_POINT('Ctrl Pts',(-10.7704707982537,-83.8959715976633,
64.9352138692215));
#114809=CARTESIAN_POINT('Ctrl Pts',(-10.758408522074,-83.8452773928997,
64.8792178759091));
#114810=CARTESIAN_POINT('Ctrl Pts',(-10.7457724178086,-83.7949388097837,
64.8246776374892));
#114811=CARTESIAN_POINT('Ctrl Pts',(-10.7325538919668,-83.7450247454837,
64.7715580352908));
#114812=CARTESIAN_POINT('',(-10.0948919410771,-81.441165552193,62.8640987085368));
#114813=CARTESIAN_POINT('Ctrl Pts',(-10.7325538919677,-83.7450249101666,
64.7715578805454));
#114814=CARTESIAN_POINT('Ctrl Pts',(-10.716052847459,-83.6827202146583,
64.7052522272387));
#114815=CARTESIAN_POINT('Ctrl Pts',(-10.6992857379384,-83.6198066549952,
64.6398096456013));
#114816=CARTESIAN_POINT('Ctrl Pts',(-10.682265385291,-83.5563142176879,
64.5752405343746));
#114817=CARTESIAN_POINT('Ctrl Pts',(-10.675408278814,-83.530734582993,64.5492271326563));
#114818=CARTESIAN_POINT('Ctrl Pts',(-10.6685100674777,-83.5050609864359,
64.5233554972818));
#114819=CARTESIAN_POINT('Ctrl Pts',(-10.6615717516232,-83.4792951642798,
64.4976259928887));
#114820=CARTESIAN_POINT('Ctrl Pts',(-10.6419708779072,-83.4065062286275,
64.4249396556047));
#114821=CARTESIAN_POINT('Ctrl Pts',(-10.6220493826656,-83.332982544654,
64.3533885661189));
#114822=CARTESIAN_POINT('Ctrl Pts',(-10.6018193908424,-83.2587410840879,
64.2829606190104));
#114823=CARTESIAN_POINT('Ctrl Pts',(-10.5971136829087,-83.2414717429507,
64.2665783410361));
#114824=CARTESIAN_POINT('Ctrl Pts',(-10.5923912784162,-83.224163554349,
64.250256840545));
#114825=CARTESIAN_POINT('Ctrl Pts',(-10.5876523724971,-83.2068167290645,
64.2339959799492));
#114826=CARTESIAN_POINT('Ctrl Pts',(-10.5648061772901,-83.1231879414425,
64.1556026119974));
#114827=CARTESIAN_POINT('Ctrl Pts',(-10.5415758864884,-83.0386612172355,
64.0786183411402));
#114828=CARTESIAN_POINT('Ctrl Pts',(-10.5179870208428,-82.9532664129503,
64.003036429589));
#114829=CARTESIAN_POINT('Ctrl Pts',(-10.5156479561116,-82.9447986901722,
63.995541750265));
#114830=CARTESIAN_POINT('Ctrl Pts',(-10.5133053645548,-82.9363224295946,
63.9880608612116));
#114831=CARTESIAN_POINT('Ctrl Pts',(-10.5109592781889,-82.9278376552467,
63.9805937523783));
#114832=CARTESIAN_POINT('Ctrl Pts',(-10.4849535148002,-82.8337861159219,
63.8978227732952));
#114833=CARTESIAN_POINT('Ctrl Pts',(-10.4585177019786,-82.7386893008579,
63.8167450927115));
#114834=CARTESIAN_POINT('Ctrl Pts',(-10.4316909758191,-82.6425707375081,
63.7373428936201));
#114835=CARTESIAN_POINT('Ctrl Pts',(-10.4048642496596,-82.5464521741583,
63.6579406945286));
#114836=CARTESIAN_POINT('Ctrl Pts',(-10.3776466101622,-82.4493118573151,
63.5802139880668));
#114837=CARTESIAN_POINT('Ctrl Pts',(-10.3500932814054,-82.3511651955188,
63.5041452967892));
#114838=CARTESIAN_POINT('Ctrl Pts',(-10.347150821168,-82.3406839700988,
63.4960218101001));
#114839=CARTESIAN_POINT('Ctrl Pts',(-10.3442045436766,-82.3301912664879,
63.4879172374884));
#114840=CARTESIAN_POINT('Ctrl Pts',(-10.3412545142997,-82.3196871110276,
63.479831568023));
#114841=CARTESIAN_POINT('Ctrl Pts',(-10.316580337161,-82.2318298867721,
63.4122026683785));
#114842=CARTESIAN_POINT('Ctrl Pts',(-10.2916437834906,-82.143171673775,
63.3458960280496));
#114843=CARTESIAN_POINT('Ctrl Pts',(-10.2664918373664,-82.0537284697427,
63.2809074057432));
#114844=CARTESIAN_POINT('Ctrl Pts',(-10.2607110531259,-82.0331713382295,
63.2659707800927));
#114845=CARTESIAN_POINT('Ctrl Pts',(-10.2549189010341,-82.0125726968343,
63.2511037585608));
#114846=CARTESIAN_POINT('Ctrl Pts',(-10.2491160027292,-81.9919326250545,
63.2363062330404));
#114847=CARTESIAN_POINT('Ctrl Pts',(-10.2266520827284,-81.9120317036672,
63.17902271504));
#114848=CARTESIAN_POINT('Ctrl Pts',(-10.204027171449,-81.8315100262574,
63.1227805141884));
#114849=CARTESIAN_POINT('Ctrl Pts',(-10.1812787454196,-81.7503678787914,
63.0675722165488));
#114850=CARTESIAN_POINT('Ctrl Pts',(-10.1725838287424,-81.7193536798173,
63.0464704687951));
#114851=CARTESIAN_POINT('Ctrl Pts',(-10.1638710839087,-81.6882489050877,
63.0255198497883));
#114852=CARTESIAN_POINT('Ctrl Pts',(-10.1551422412299,-81.6570549439541,
63.0047209448188));
#114853=CARTESIAN_POINT('Ctrl Pts',(-10.135134576849,-81.585554250444,62.9570470978457));
#114854=CARTESIAN_POINT('Ctrl Pts',(-10.1150423492291,-81.5135849718596,
62.9101703633017));
#114855=CARTESIAN_POINT('Ctrl Pts',(-10.0948919410775,-81.4411655389391,
62.8640987293704));
#114856=CARTESIAN_POINT('',(-8.69365830054091,-75.00000003516,60.98889557741));
#114857=CARTESIAN_POINT('Ctrl Pts',(-10.0948919410769,-81.44116555882,62.86409869812));
#114858=CARTESIAN_POINT('Ctrl Pts',(-10.0518048744405,-81.2863646276699,
62.7656178172554));
#114859=CARTESIAN_POINT('Ctrl Pts',(-10.0025424805627,-81.116825889132,
62.6627172439813));
#114860=CARTESIAN_POINT('Ctrl Pts',(-9.91938589888409,-80.8390231510282,
62.5047510738291));
#114861=CARTESIAN_POINT('Ctrl Pts',(-9.89012320651422,-80.7425066983133,
62.4514990831448));
#114862=CARTESIAN_POINT('Ctrl Pts',(-9.8439134202439,-80.5916925981988,
62.3711580712742));
#114863=CARTESIAN_POINT('Ctrl Pts',(-9.82022959017987,-80.5147758129416,
62.3308723952113));
#114864=CARTESIAN_POINT('Ctrl Pts',(-9.79158531547964,-80.4223627831845,
62.2837716277709));
#114865=CARTESIAN_POINT('Ctrl Pts',(-9.77700989322315,-80.3754828784744,
62.260209105959));
#114866=CARTESIAN_POINT('Ctrl Pts',(-9.7696588608683,-80.3518740598891,
62.2484264570357));
#114867=CARTESIAN_POINT('Ctrl Pts',(-9.76649484959624,-80.341719754058,
62.2433766307136));
#114868=CARTESIAN_POINT('Ctrl Pts',(-9.76438249345169,-80.3349421572503,
62.2400100730806));
#114869=CARTESIAN_POINT('Ctrl Pts',(-9.76289144897654,-80.3301595361113,
62.2376380948878));
#114870=CARTESIAN_POINT('Ctrl Pts',(-9.74223890670972,-80.2639262891045,
62.2048169668438));
#114871=CARTESIAN_POINT('Ctrl Pts',(-9.71522129820358,-80.1778496550703,
62.1627985636355));
#114872=CARTESIAN_POINT('Ctrl Pts',(-9.66420853416412,-80.0148712661353,
62.0868410206361));
#114873=CARTESIAN_POINT('Ctrl Pts',(-9.64545655427094,-79.9548962970397,
62.0593795841153));
#114874=CARTESIAN_POINT('Ctrl Pts',(-9.6147069966111,-79.8562873318557,
62.0153863538377));
#114875=CARTESIAN_POINT('Ctrl Pts',(-9.60402021275448,-79.82197637176,62.0002559306572));
#114876=CARTESIAN_POINT('Ctrl Pts',(-9.58177278243454,-79.7504407061777,
61.9691419096399));
#114877=CARTESIAN_POINT('Ctrl Pts',(-9.57055025010918,-79.7143065643979,
61.9536195698955));
#114878=CARTESIAN_POINT('Ctrl Pts',(-9.50887179058622,-79.5153650542099,
61.8694766597471));
#114879=CARTESIAN_POINT('Ctrl Pts',(-9.46580516087099,-79.3743754823427,
61.8138362640074));
#114880=CARTESIAN_POINT('Ctrl Pts',(-9.41061942315287,-79.1916364045872,
61.7445829366495));
#114881=CARTESIAN_POINT('Ctrl Pts',(-9.39379321172261,-79.1355075403693,
61.723875018136));
#114882=CARTESIAN_POINT('Ctrl Pts',(-9.37090744629091,-79.0586241662255,
61.6960459575867));
#114883=CARTESIAN_POINT('Ctrl Pts',(-9.36005295150348,-79.0220094527361,
61.6829405002834));
#114884=CARTESIAN_POINT('Ctrl Pts',(-9.34841905312621,-78.9825136859927,
61.6690033648935));
#114885=CARTESIAN_POINT('Ctrl Pts',(-9.34285952365626,-78.9635738264959,
61.6623657291019));
#114886=CARTESIAN_POINT('Ctrl Pts',(-9.34014411385095,-78.9543062283972,
61.6591287630642));
#114887=CARTESIAN_POINT('Ctrl Pts',(-9.33899415713361,-78.9503777913378,
61.6577589392433));
#114888=CARTESIAN_POINT('Ctrl Pts',(-9.33823058384251,-78.9477684793878,
61.6568495904088));
#114889=CARTESIAN_POINT('Ctrl Pts',(-9.33816091406803,-78.9475306640759,
61.656766554339));
#114890=CARTESIAN_POINT('Ctrl Pts',(-9.29335597623239,-78.7943239964564,
61.6034329332589));
#114891=CARTESIAN_POINT('Ctrl Pts',(-9.25256248254764,-78.6504854818397,
61.5567280406397));
#114892=CARTESIAN_POINT('Ctrl Pts',(-9.19635544814298,-78.445849160099,
61.4940552038252));
#114893=CARTESIAN_POINT('Ctrl Pts',(-9.16949773247126,-78.3463089295506,
61.4645666950856));
#114894=CARTESIAN_POINT('Ctrl Pts',(-9.14034388353282,-78.2351486053617,
61.4331267605316));
#114895=CARTESIAN_POINT('Ctrl Pts',(-9.12631199723324,-78.1808229019596,
61.4181153888453));
#114896=CARTESIAN_POINT('Ctrl Pts',(-9.11943231362586,-78.1539751249433,
61.410782870149));
#114897=CARTESIAN_POINT('Ctrl Pts',(-9.11651307626751,-78.1425366028503,
61.407677047469));
#114898=CARTESIAN_POINT('Ctrl Pts',(-9.11457340657824,-78.1349259754488,
61.4056146047108));
#114899=CARTESIAN_POINT('Ctrl Pts',(-9.11392192730972,-78.1323679828658,
61.4049221056818));
#114900=CARTESIAN_POINT('Ctrl Pts',(-9.07173282663215,-77.9663764800442,
61.3601144269983));
#114901=CARTESIAN_POINT('Ctrl Pts',(-9.0341765477646,-77.8090390324268,
61.3212393125679));
#114902=CARTESIAN_POINT('Ctrl Pts',(-8.98287367578384,-77.5788683170903,
61.2690076535193));
#114903=CARTESIAN_POINT('Ctrl Pts',(-8.9584801263736,-77.4652406052022,
61.2444124341212));
#114904=CARTESIAN_POINT('Ctrl Pts',(-8.93222228691025,-77.3353009481976,
61.2182124618105));
#114905=CARTESIAN_POINT('Ctrl Pts',(-8.91964369255738,-77.2709961531179,
61.2057156191777));
#114906=CARTESIAN_POINT('Ctrl Pts',(-8.91349197672566,-77.2390110591143,
61.1996154368605));
#114907=CARTESIAN_POINT('Ctrl Pts',(-8.91088500880021,-77.2253391220203,
61.1970325667274));
#114908=CARTESIAN_POINT('Ctrl Pts',(-8.90915358167585,-77.2162325005146,
61.1953176217769));
#114909=CARTESIAN_POINT('Ctrl Pts',(-8.90853926942428,-77.2129958721295,
61.1947092630006));
#114910=CARTESIAN_POINT('Ctrl Pts',(-8.76569916465401,-76.4573161571757,
61.0533061035506));
#114911=CARTESIAN_POINT('Ctrl Pts',(-8.69444127090419,-75.7170145006195,
60.9888893886809));
#114912=CARTESIAN_POINT('Ctrl Pts',(-8.69365830054091,-75.00000003516,60.98889557741));
#114913=CARTESIAN_POINT('',(-8.56753648333091,-75.,60.98888938658));
#114914=CARTESIAN_POINT('',(-15.5675364833309,-75.,60.98888938658));
#114915=CARTESIAN_POINT('Origin',(-8.56753648333091,-75.,72.98888938658));
#114916=CARTESIAN_POINT('',(-10.094867738972,-68.5588861609101,62.8640661515342));
#114917=CARTESIAN_POINT('Ctrl Pts',(-8.69365830112879,-75.0000000361644,
60.9889038049696));
#114918=CARTESIAN_POINT('Ctrl Pts',(-8.69384525821713,-74.8245766453446,
60.9889252073937));
#114919=CARTESIAN_POINT('Ctrl Pts',(-8.69827073512056,-74.647732721061,
60.9928047893908));
#114920=CARTESIAN_POINT('Ctrl Pts',(-8.706920554905,-74.4696329007517,61.0006933496487));
#114921=CARTESIAN_POINT('Ctrl Pts',(-8.71504876833194,-74.3022729572094,
61.0081062094544));
#114922=CARTESIAN_POINT('Ctrl Pts',(-8.72690760767029,-74.1338036400519,
61.0190593571933));
#114923=CARTESIAN_POINT('Ctrl Pts',(-8.7425079218425,-73.9643922544561,
61.0337105002916));
#114924=CARTESIAN_POINT('Ctrl Pts',(-8.74350903028094,-73.9535207318819,
61.034650698215));
#114925=CARTESIAN_POINT('Ctrl Pts',(-8.74452555346398,-73.9426453420439,
61.0356061359183));
#114926=CARTESIAN_POINT('Ctrl Pts',(-8.74555749710937,-73.9317661343774,
61.0365768596762));
#114927=CARTESIAN_POINT('Ctrl Pts',(-8.75602275042763,-73.8214367916468,
61.0464212635574));
#114928=CARTESIAN_POINT('Ctrl Pts',(-8.76806128725323,-73.7107058345274,
61.0578380832004));
#114929=CARTESIAN_POINT('Ctrl Pts',(-8.7816935928635,-73.5996352672253,
61.0708786774647));
#114930=CARTESIAN_POINT('Ctrl Pts',(-8.7903528098044,-73.5290834350178,
61.0791620403823));
#114931=CARTESIAN_POINT('Ctrl Pts',(-8.79965520013409,-73.4583948049494,
61.0881006865537));
#114932=CARTESIAN_POINT('Ctrl Pts',(-8.80959015964689,-73.3875752183467,
61.0977035441218));
#114933=CARTESIAN_POINT('Ctrl Pts',(-8.82237800036828,-73.2964193769703,
61.1100639179001));
#114934=CARTESIAN_POINT('Ctrl Pts',(-8.83622370490817,-73.2050527888017,
61.1235239289185));
#114935=CARTESIAN_POINT('Ctrl Pts',(-8.8511272719821,-73.1135030831726,
61.1381012595064));
#114936=CARTESIAN_POINT('Ctrl Pts',(-8.85857905551907,-73.067728230358,
61.1453899248004));
#114937=CARTESIAN_POINT('Ctrl Pts',(-8.86629530475195,-73.0219075951315,
61.1529579327023));
#114938=CARTESIAN_POINT('Ctrl Pts',(-8.87427601982463,-72.9760447470789,
61.1608075542463));
#114939=CARTESIAN_POINT('Ctrl Pts',(-8.87826637736097,-72.9531133230526,
61.1647323650183));
#114940=CARTESIAN_POINT('Ctrl Pts',(-8.88232285135977,-72.9301713457549,
61.1687275800761));
#114941=CARTESIAN_POINT('Ctrl Pts',(-8.88644544184757,-72.907219264802,
61.1727934881509));
#114942=CARTESIAN_POINT('Ctrl Pts',(-8.88953738471342,-72.8900052040874,
61.175842919207));
#114943=CARTESIAN_POINT('Ctrl Pts',(-8.89266651810446,-72.8727854600641,
61.1789321151613));
#114944=CARTESIAN_POINT('Ctrl Pts',(-8.89583284203163,-72.8555602239495,
61.1820611989636));
#114945=CARTESIAN_POINT('Ctrl Pts',(-8.89688828334068,-72.849818478578,
61.1831042268977));
#114946=CARTESIAN_POINT('Ctrl Pts',(-8.89817259108541,-72.8428627810642,
61.1843739259477));
#114947=CARTESIAN_POINT('Ctrl Pts',(-8.89901156280451,-72.8383331643582,
61.1852035833048));
#114948=CARTESIAN_POINT('Ctrl Pts',(-8.9225926824401,-72.7110184634967,
61.2085229025959));
#114949=CARTESIAN_POINT('Ctrl Pts',(-8.948694109248,-72.5807530056447,61.234507052742));
#114950=CARTESIAN_POINT('Ctrl Pts',(-8.97731851831312,-72.4476737333343,
61.2634710838465));
#114951=CARTESIAN_POINT('Ctrl Pts',(-8.9812829872012,-72.429242308828,61.2674825902474));
#114952=CARTESIAN_POINT('Ctrl Pts',(-8.98529579245517,-72.410756960309,
61.2715512808838));
#114953=CARTESIAN_POINT('Ctrl Pts',(-8.98935688116652,-72.3922181029307,
61.2756780155713));
#114954=CARTESIAN_POINT('Ctrl Pts',(-9.00017444305544,-72.3428359664415,
61.2866704392916));
#114955=CARTESIAN_POINT('Ctrl Pts',(-9.01133391949106,-72.2930733728004,
61.2980748567245));
#114956=CARTESIAN_POINT('Ctrl Pts',(-9.02283815818018,-72.2429398737176,
61.3099074330183));
#114957=CARTESIAN_POINT('Ctrl Pts',(-9.02908502354944,-72.2157171058559,
61.3163325875267));
#114958=CARTESIAN_POINT('Ctrl Pts',(-9.03543353648351,-72.1883849945047,
61.3228839886947));
#114959=CARTESIAN_POINT('Ctrl Pts',(-9.04188256206101,-72.1609442733638,
61.3295644679222));
#114960=CARTESIAN_POINT('Ctrl Pts',(-9.05104534349893,-72.1219564716734,
61.3390560989177));
#114961=CARTESIAN_POINT('Ctrl Pts',(-9.0604123756522,-72.0827501093837,
61.3488081304238));
#114962=CARTESIAN_POINT('Ctrl Pts',(-9.06998365852324,-72.0433292790635,
61.3588282522153));
#114963=CARTESIAN_POINT('Ctrl Pts',(-9.07476929995877,-72.0236188639035,
61.363838313111));
#114964=CARTESIAN_POINT('Ctrl Pts',(-9.07960600407186,-72.0038548320136,
61.3689153973613));
#114965=CARTESIAN_POINT('Ctrl Pts',(-9.08449377085193,-71.9840377054465,
61.3740604684296));
#114966=CARTESIAN_POINT('Ctrl Pts',(-9.08693765424197,-71.974129142163,
61.3766330039637));
#114967=CARTESIAN_POINT('Ctrl Pts',(-9.08939430329864,-71.9642073052274,
61.3792225362478));
#114968=CARTESIAN_POINT('Ctrl Pts',(-9.09186371802004,-71.9542722609874,
61.3818291857182));
#114969=CARTESIAN_POINT('Ctrl Pts',(-9.09309842538075,-71.9493047388673,
61.3831325104534));
#114970=CARTESIAN_POINT('Ctrl Pts',(-9.09433632415762,-71.9443339149221,
61.3844401144878));
#114971=CARTESIAN_POINT('Ctrl Pts',(-9.09557741435042,-71.9393597975172,
61.3857520128741));
#114972=CARTESIAN_POINT('Ctrl Pts',(-9.09681850454321,-71.9343856801124,
61.3870639112604));
#114973=CARTESIAN_POINT('Ctrl Pts',(-9.09837281773138,-71.9281704284257,
61.388708285338));
#114974=CARTESIAN_POINT('Ctrl Pts',(-9.09931025917626,-71.9244275733127,
61.3897006061457));
#114975=CARTESIAN_POINT('Ctrl Pts',(-9.11922873284419,-71.8449005144027,
61.4107851399981));
#114976=CARTESIAN_POINT('Ctrl Pts',(-9.14074565379796,-71.7615529692762,
61.4337570806931));
#114977=CARTESIAN_POINT('Ctrl Pts',(-9.16387259792112,-71.6744787276342,
61.458871924867));
#114978=CARTESIAN_POINT('Ctrl Pts',(-9.17557588230001,-71.6304152055975,
61.4715811769815));
#114979=CARTESIAN_POINT('Ctrl Pts',(-9.18769082592326,-71.5853975145052,
61.4848395475597));
#114980=CARTESIAN_POINT('Ctrl Pts',(-9.20021431489938,-71.5394388953521,
61.4986823135457));
#114981=CARTESIAN_POINT('Ctrl Pts',(-9.21884993753997,-71.4710500074589,
61.5192810910676));
#114982=CARTESIAN_POINT('Ctrl Pts',(-9.23839470040588,-71.4005780245766,
61.5411734447155));
#114983=CARTESIAN_POINT('Ctrl Pts',(-9.25884860323448,-71.3280737128276,
61.5644799762425));
#114984=CARTESIAN_POINT('Ctrl Pts',(-9.26907555464878,-71.2918215569531,
61.576133242006));
#114985=CARTESIAN_POINT('Ctrl Pts',(-9.27952979104853,-71.2550613542374,
61.5881401626345));
#114986=CARTESIAN_POINT('Ctrl Pts',(-9.29021131242184,-71.2178001815926,
61.6005162820495));
#114987=CARTESIAN_POINT('Ctrl Pts',(-9.2955520731085,-71.1991695952702,
61.606704341757));
#114988=CARTESIAN_POINT('Ctrl Pts',(-9.30094965503958,-71.1804137683667,
61.612984707645));
#114989=CARTESIAN_POINT('Ctrl Pts',(-9.30640405821832,-71.1615336159611,
61.6193593546832));
#114990=CARTESIAN_POINT('Ctrl Pts',(-9.30913125980769,-71.1520935397583,
61.6225466782022));
#114991=CARTESIAN_POINT('Ctrl Pts',(-9.31187266670901,-71.1426223823034,
61.6257575724023));
#114992=CARTESIAN_POINT('Ctrl Pts',(-9.31462827892278,-71.1331202606396,
61.6289922858397));
#114993=CARTESIAN_POINT('Ctrl Pts',(-9.31600608502967,-71.1283691998077,
61.6306096425584));
#114994=CARTESIAN_POINT('Ctrl Pts',(-9.31738744246467,-71.123610397931,
61.6322329541106));
#114995=CARTESIAN_POINT('Ctrl Pts',(-9.31877235122784,-71.1188438698163,
61.6338622516649));
#114996=CARTESIAN_POINT('Ctrl Pts',(-9.32015725999101,-71.1140773417016,
61.6354915492193));
#114997=CARTESIAN_POINT('Ctrl Pts',(-9.32207922785804,-71.1074703323387,
61.637755884187));
#114998=CARTESIAN_POINT('Ctrl Pts',(-9.32293773150189,-71.1045211216348,
61.6387681335848));
#114999=CARTESIAN_POINT('Ctrl Pts',(-9.32540804075955,-71.0960348879923,
61.6416808399853));
#115000=CARTESIAN_POINT('Ctrl Pts',(-9.32791662688662,-71.087431771361,
61.6446442765875));
#115001=CARTESIAN_POINT('Ctrl Pts',(-9.33046351585559,-71.0787120910557,
61.6476592445136));
#115002=CARTESIAN_POINT('Ctrl Pts',(-9.34717384114147,-71.0215016291683,
61.6674406701609));
#115003=CARTESIAN_POINT('Ctrl Pts',(-9.36553468648594,-70.9592718360005,
61.6894370377311));
#115004=CARTESIAN_POINT('Ctrl Pts',(-9.38555146037108,-70.8921230086149,
61.713900599354));
#115005=CARTESIAN_POINT('Ctrl Pts',(-9.39641198312577,-70.8556899963845,
61.7271738205629));
#115006=CARTESIAN_POINT('Ctrl Pts',(-9.4077596439782,-70.8178092287548,
61.7411740572641));
#115007=CARTESIAN_POINT('Ctrl Pts',(-9.41959197261567,-70.7784990529737,
61.7559466688392));
#115008=CARTESIAN_POINT('Ctrl Pts',(-9.43807399470082,-70.717096808393,
61.7790213941744));
#115009=CARTESIAN_POINT('Ctrl Pts',(-9.457742507847,-70.6522072039607,61.8039793522644));
#115010=CARTESIAN_POINT('Ctrl Pts',(-9.47859751201244,-70.5839139312709,
61.8310082703903));
#115011=CARTESIAN_POINT('Ctrl Pts',(-9.48902501409516,-70.549767294926,
61.8445227294532));
#115012=CARTESIAN_POINT('Ctrl Pts',(-9.49974913892252,-70.5147699709371,
61.8585552215054));
#115013=CARTESIAN_POINT('Ctrl Pts',(-9.51076988645421,-70.478933866873,
61.8731309024725));
#115014=CARTESIAN_POINT('Ctrl Pts',(-9.51628026022006,-70.4610158148409,
61.8804187429561));
#115015=CARTESIAN_POINT('Ctrl Pts',(-9.52186478966094,-70.442888076038,
61.8878424007396));
#115016=CARTESIAN_POINT('Ctrl Pts',(-9.5275234747752,-70.424552245374,61.8954051157619));
#115017=CARTESIAN_POINT('Ctrl Pts',(-9.53249846447252,-70.4084317921585,
61.9020540860722));
#115018=CARTESIAN_POINT('Ctrl Pts',(-9.53721923892211,-70.3931570372304,
61.9083908527476));
#115019=CARTESIAN_POINT('Ctrl Pts',(-9.54250747549523,-70.3760742064197,
61.9155244139028));
#115020=CARTESIAN_POINT('Ctrl Pts',(-9.54323421933363,-70.3737265727875,
61.9165047542382));
#115021=CARTESIAN_POINT('Ctrl Pts',(-9.54397168194754,-70.3713448258,61.9175002152205));
#115022=CARTESIAN_POINT('Ctrl Pts',(-9.54472199713705,-70.3689221118314,
61.9185137476522));
#115023=CARTESIAN_POINT('Ctrl Pts',(-9.56686698111811,-70.2974175457824,
61.9484273889841));
#115024=CARTESIAN_POINT('Ctrl Pts',(-9.587521094413,-70.2309884594451,61.9770285730077));
#115025=CARTESIAN_POINT('Ctrl Pts',(-9.60666602037937,-70.1695285933851,
62.0040558945936));
#115026=CARTESIAN_POINT('Ctrl Pts',(-9.61672698109021,-70.1372304639063,
62.0182591785902));
#115027=CARTESIAN_POINT('Ctrl Pts',(-9.62637177798907,-70.1063049602051,
62.0320284265364));
#115028=CARTESIAN_POINT('Ctrl Pts',(-9.63560123225895,-70.0767385813395,
62.0453297677685));
#115029=CARTESIAN_POINT('Ctrl Pts',(-9.64820959587144,-70.0363479315196,
62.0635007388664));
#115030=CARTESIAN_POINT('Ctrl Pts',(-9.66004264588526,-69.9984935808949,
62.0807981351448));
#115031=CARTESIAN_POINT('Ctrl Pts',(-9.67110723157983,-69.9631454708437,
62.097144337565));
#115032=CARTESIAN_POINT('Ctrl Pts',(-9.68741261949328,-69.9110545329359,
62.1212330091818));
#115033=CARTESIAN_POINT('Ctrl Pts',(-9.70203866039361,-69.8644019000139,
62.1432555275304));
#115034=CARTESIAN_POINT('Ctrl Pts',(-9.7149849350291,-69.8230959229707,
62.1630072776116));
#115035=CARTESIAN_POINT('Ctrl Pts',(-9.7157652165445,-69.8206063812863,
62.1641977301487));
#115036=CARTESIAN_POINT('Ctrl Pts',(-9.71653940047268,-69.8181362679303,
62.1653799476744));
#115037=CARTESIAN_POINT('Ctrl Pts',(-9.71730748819526,-69.815685565258,
62.1665538906621));
#115038=CARTESIAN_POINT('Ctrl Pts',(-9.72406351089009,-69.7941294299548,
62.1768797756291));
#115039=CARTESIAN_POINT('Ctrl Pts',(-9.73034752354787,-69.774074824194,
62.1865652270092));
#115040=CARTESIAN_POINT('Ctrl Pts',(-9.73615952618739,-69.7555102227944,
62.1955855670669));
#115041=CARTESIAN_POINT('Ctrl Pts',(-9.73906552750716,-69.7462279220946,
62.2000957370957));
#115042=CARTESIAN_POINT('Ctrl Pts',(-9.74185352632141,-69.7373181496336,
62.2044396850447));
#115043=CARTESIAN_POINT('Ctrl Pts',(-9.74452352263516,-69.7287795988378,
62.2086146753113));
#115044=CARTESIAN_POINT('Ctrl Pts',(-9.74585852079203,-69.7245103234399,
62.2107021704445));
#115045=CARTESIAN_POINT('Ctrl Pts',(-9.74716401832364,-69.7203338551499,
62.212747429656));
#115046=CARTESIAN_POINT('Ctrl Pts',(-9.74844001523034,-69.7162500405712,
62.2147501321042));
#115047=CARTESIAN_POINT('Ctrl Pts',(-9.74907801368369,-69.7142081332818,
62.2157514833284));
#115048=CARTESIAN_POINT('Ctrl Pts',(-9.74970863698081,-69.7121893895273,
62.2167421955798));
#115049=CARTESIAN_POINT('Ctrl Pts',(-9.75033188512175,-69.7101937906893,
62.2177222301046));
#115050=CARTESIAN_POINT('Ctrl Pts',(-9.7509551332627,-69.7081981918514,
62.2187022646294));
#115051=CARTESIAN_POINT('Ctrl Pts',(-9.75108437475398,-69.7077846654699,
62.2189049711921));
#115052=CARTESIAN_POINT('Ctrl Pts',(-9.75217950407609,-69.7042764107142,
62.2206302626284));
#115053=CARTESIAN_POINT('Ctrl Pts',(-9.78388530258222,-69.6027066543888,
62.2705802927656));
#115054=CARTESIAN_POINT('Ctrl Pts',(-9.81434516651739,-69.5047221369212,
62.3205516446024));
#115055=CARTESIAN_POINT('Ctrl Pts',(-9.84346562989802,-69.4102197139354,
62.3703005384937));
#115056=CARTESIAN_POINT('Ctrl Pts',(-9.86510654357278,-69.3399901042222,
62.4072714995682));
#115057=CARTESIAN_POINT('Ctrl Pts',(-9.88600896198795,-69.2716836485838,
62.4441198786041));
#115058=CARTESIAN_POINT('Ctrl Pts',(-9.90615231348221,-69.2052596148448,
62.480750451818));
#115059=CARTESIAN_POINT('Ctrl Pts',(-9.93783413302433,-69.1007867196179,
62.5383636653202));
#115060=CARTESIAN_POINT('Ctrl Pts',(-9.96763719432755,-69.0009707238969,
62.5954366889229));
#115061=CARTESIAN_POINT('Ctrl Pts',(-9.99559863800527,-68.9056769114017,
62.6516169537898));
#115062=CARTESIAN_POINT('Ctrl Pts',(-10.0249484751374,-68.8056513938114,
62.7105867853512));
#115063=CARTESIAN_POINT('Ctrl Pts',(-10.0522697332514,-68.7106081000212,
62.7685727517803));
#115064=CARTESIAN_POINT('Ctrl Pts',(-10.0776526495244,-68.6203935392705,
62.8251989857031));
#115065=CARTESIAN_POINT('Ctrl Pts',(-10.0834929971886,-68.5996360977893,
62.8382280990432));
#115066=CARTESIAN_POINT('Ctrl Pts',(-10.0892308978382,-68.5791343120549,
62.8511853626773));
#115067=CARTESIAN_POINT('Ctrl Pts',(-10.0948677389681,-68.558886345915,
62.8640664423475));
#115068=CARTESIAN_POINT('',(-10.0948705696752,-68.5588302431943,83.1136771106412));
#115069=CARTESIAN_POINT('Ctrl Pts',(-10.094867738974,-68.5588860050051,
62.8640659064653));
#115070=CARTESIAN_POINT('Ctrl Pts',(-10.1443275500759,-68.3811321371765,
62.9771476730743));
#115071=CARTESIAN_POINT('Ctrl Pts',(-10.192135551363,-68.2091735334229,
63.093117860736));
#115072=CARTESIAN_POINT('Ctrl Pts',(-10.2382917428353,-68.0429516821774,
63.2113907952489));
#115073=CARTESIAN_POINT('Ctrl Pts',(-10.2849968592397,-67.8747529928199,
63.331070322474));
#115074=CARTESIAN_POINT('Ctrl Pts',(-10.3300106430149,-67.7124280221737,
63.4531075205968));
#115075=CARTESIAN_POINT('Ctrl Pts',(-10.373333094161,-67.5558738575396,
63.5769296557302));
#115076=CARTESIAN_POINT('Ctrl Pts',(-10.4175331184007,-67.3961484106037,
63.7032600278475));
#115077=CARTESIAN_POINT('Ctrl Pts',(-10.4599725941102,-67.242429666187,
63.8314481853243));
#115078=CARTESIAN_POINT('Ctrl Pts',(-10.5006515212892,-67.0945688096429,
63.9609240734804));
#115079=CARTESIAN_POINT('Ctrl Pts',(-10.5377636714851,-66.959672569828,
64.0790473609223));
#115080=CARTESIAN_POINT('Ctrl Pts',(-10.5734104720686,-66.8296513193455,
64.1982428928792));
#115081=CARTESIAN_POINT('Ctrl Pts',(-10.6075919230397,-66.7043672961587,
64.3181063744779));
#115082=CARTESIAN_POINT('Ctrl Pts',(-10.6461222346423,-66.5631435530154,
64.4532199277225));
#115083=CARTESIAN_POINT('Ctrl Pts',(-10.6827906078484,-66.4279393536557,
64.5891814235258));
#115084=CARTESIAN_POINT('Ctrl Pts',(-10.717597042658,-66.2985272376477,
64.725453553584));
#115085=CARTESIAN_POINT('Ctrl Pts',(-10.7531375112871,-66.1663859461206,
64.8645995301782));
#115086=CARTESIAN_POINT('Ctrl Pts',(-10.7867366804925,-66.0402832831347,
65.0040692609461));
#115087=CARTESIAN_POINT('Ctrl Pts',(-10.8183945502742,-65.9199491500656,
65.1433379998));
#115088=CARTESIAN_POINT('Ctrl Pts',(-10.8430359460974,-65.8262852041199,
65.2517399909494));
#115089=CARTESIAN_POINT('Ctrl Pts',(-10.8665011999206,-65.736115520797,
65.3600211773868));
#115090=CARTESIAN_POINT('Ctrl Pts',(-10.888790311744,-65.6493033632878,
65.4679537793447));
#115091=CARTESIAN_POINT('Ctrl Pts',(-10.9019518551797,-65.5980414740365,
65.5316871232325));
#115092=CARTESIAN_POINT('Ctrl Pts',(-10.9147033004037,-65.5479501463495,
65.5952992464033));
#115093=CARTESIAN_POINT('Ctrl Pts',(-10.927044647416,-65.4990001414469,
65.6587460259236));
#115094=CARTESIAN_POINT('Ctrl Pts',(-10.9332153209221,-65.4745251389956,
65.6904694156838));
#115095=CARTESIAN_POINT('Ctrl Pts',(-10.9392834698753,-65.4503354754091,
65.7221514757892));
#115096=CARTESIAN_POINT('Ctrl Pts',(-10.9452490942756,-65.4264274089262,
65.7537869102193));
#115097=CARTESIAN_POINT('Ctrl Pts',(-10.9482319064758,-65.4144733756847,
65.7696046274344));
#115098=CARTESIAN_POINT('Ctrl Pts',(-10.9511890875377,-65.4025897422853,
65.7854106886726));
#115099=CARTESIAN_POINT('Ctrl Pts',(-10.9541206374614,-65.3907760409084,
65.8012044391147));
#115100=CARTESIAN_POINT('Ctrl Pts',(-10.9555864124233,-65.3848691902199,
65.8091013143357));
#115101=CARTESIAN_POINT('Ctrl Pts',(-10.9570457796006,-65.378979822572,
65.8169951118837));
#115102=CARTESIAN_POINT('Ctrl Pts',(-10.9584987389933,-65.3731078792483,
65.8248857506646));
#115103=CARTESIAN_POINT('Ctrl Pts',(-10.9595884585378,-65.3687039217556,
65.8308037297502));
#115104=CARTESIAN_POINT('Ctrl Pts',(-10.9606745737036,-65.3643097654482,
65.8367199320315));
#115105=CARTESIAN_POINT('Ctrl Pts',(-10.9617570844905,-65.359925385512,
65.8426343234645));
#115106=CARTESIAN_POINT('Ctrl Pts',(-10.9621179214195,-65.3584639255333,
65.8446057872755));
#115107=CARTESIAN_POINT('Ctrl Pts',(-10.9621766445903,-65.3582264482039,
65.8449252842859));
#115108=CARTESIAN_POINT('Ctrl Pts',(-10.9628383938178,-65.3555442634409,
65.8485481100336));
#115109=CARTESIAN_POINT('Ctrl Pts',(-10.9998963505593,-65.2053419167105,
66.0514263519079));
#115110=CARTESIAN_POINT('Ctrl Pts',(-11.0349672381504,-65.0601785208779,
66.2608881377162));
#115111=CARTESIAN_POINT('Ctrl Pts',(-11.0680510565911,-64.9207073657571,
66.4767576316708));
#115112=CARTESIAN_POINT('Ctrl Pts',(-11.0993629451878,-64.7887061193043,
66.6810654130789));
#115113=CARTESIAN_POINT('Ctrl Pts',(-11.1288949147412,-64.6618040411431,
66.8911126211767));
#115114=CARTESIAN_POINT('Ctrl Pts',(-11.1566469652512,-64.5405622102097,
67.106699222916));
#115115=CARTESIAN_POINT('Ctrl Pts',(-11.1841387787951,-64.4204572900871,
67.3202642225704));
#115116=CARTESIAN_POINT('Ctrl Pts',(-11.2098838981534,-64.3059072327915,
67.5392652961144));
#115117=CARTESIAN_POINT('Ctrl Pts',(-11.2338823233261,-64.1974604243281,
67.7634574698823));
#115118=CARTESIAN_POINT('Ctrl Pts',(-11.2576587098004,-64.0900169895454,
67.9855753684387));
#115119=CARTESIAN_POINT('Ctrl Pts',(-11.2797205741621,-63.9885646684362,
68.2127888114342));
#115120=CARTESIAN_POINT('Ctrl Pts',(-11.300067916411,-63.8936355732867,
68.4448087071646));
#115121=CARTESIAN_POINT('Ctrl Pts',(-11.3202294713136,-63.7995732559436,
68.6747100775266));
#115122=CARTESIAN_POINT('Ctrl Pts',(-11.3387076710504,-63.7119158685469,
68.9093305624892));
#115123=CARTESIAN_POINT('Ctrl Pts',(-11.3555025156215,-63.6311757184616,
69.1483380647638));
#115124=CARTESIAN_POINT('Ctrl Pts',(-11.3720713949053,-63.5515218821634,
69.3841298541042));
#115125=CARTESIAN_POINT('Ctrl Pts',(-11.3870019115129,-63.4786006761391,
69.6241913779256));
#115126=CARTESIAN_POINT('Ctrl Pts',(-11.4002940654443,-63.4128946261226,
69.8681540478078));
#115127=CARTESIAN_POINT('Ctrl Pts',(-11.4134848783109,-63.3476895273517,
70.110256715402));
#115128=CARTESIAN_POINT('Ctrl Pts',(-11.4250622154367,-63.289590271564,
70.3562012670786));
#115129=CARTESIAN_POINT('Ctrl Pts',(-11.4350260768217,-63.2390549508833,
70.6055783385509));
#115130=CARTESIAN_POINT('Ctrl Pts',(-11.4448755988908,-63.1890995433278,
70.8520937078527));
#115131=CARTESIAN_POINT('Ctrl Pts',(-11.4531484633147,-63.1465357405352,
71.1019632110204));
#115132=CARTESIAN_POINT('Ctrl Pts',(-11.4598446700932,-63.1117886989206,
71.3547437196065));
#115133=CARTESIAN_POINT('Ctrl Pts',(-11.4641055045612,-63.0896789586643,
71.5155893952958));
#115134=CARTESIAN_POINT('Ctrl Pts',(-11.4677279741092,-63.070733747897,
71.6776127373646));
#115135=CARTESIAN_POINT('Ctrl Pts',(-11.4707120787369,-63.0550580966133,
71.8406895238746));
#115136=CARTESIAN_POINT('Ctrl Pts',(-11.4737205646426,-63.0392543692532,
72.0050987102059));
#115137=CARTESIAN_POINT('Ctrl Pts',(-11.4760802116421,-63.0267738882719,
72.1705786358204));
#115138=CARTESIAN_POINT('Ctrl Pts',(-11.4777910197354,-63.0177200726439,
72.3369938869189));
#115139=CARTESIAN_POINT('Ctrl Pts',(-11.478646423782,-63.0131931648298,
72.4202015124681));
#115140=CARTESIAN_POINT('Ctrl Pts',(-11.4793396181021,-63.0095228482124,
72.5036429658301));
#115141=CARTESIAN_POINT('Ctrl Pts',(-11.4798706026955,-63.0067216199527,
72.5873004192394));
#115142=CARTESIAN_POINT('Ctrl Pts',(-11.4801360949923,-63.0053210058228,
72.629129145944));
#115143=CARTESIAN_POINT('Ctrl Pts',(-11.4803610348574,-63.0041376585083,
72.6710118723181));
#115144=CARTESIAN_POINT('Ctrl Pts',(-11.4805454222909,-63.0031731096894,
72.7129463418755));
#115145=CARTESIAN_POINT('Ctrl Pts',(-11.4806885551879,-63.0024243674126,
72.7454984632382));
#115146=CARTESIAN_POINT('Ctrl Pts',(-11.4808055767655,-63.001818854722,
72.7774000278934));
#115147=CARTESIAN_POINT('Ctrl Pts',(-11.4809003880803,-63.0013299265603,
72.8102375779043));
#115148=CARTESIAN_POINT('Ctrl Pts',(-11.4809277151094,-63.0011890050454,
72.8197021938854));
#115149=CARTESIAN_POINT('Ctrl Pts',(-11.4809531970458,-63.001058095518,
72.8292445713027));
#115150=CARTESIAN_POINT('Ctrl Pts',(-11.4809769272963,-63.0009373700998,
72.8389027080638));
#115151=CARTESIAN_POINT('Ctrl Pts',(-11.4816147494037,-62.9976925101056,
73.098494284336));
#115152=CARTESIAN_POINT('Ctrl Pts',(-11.480706716154,-63.0028956745713,
73.3564745512392));
#115153=CARTESIAN_POINT('Ctrl Pts',(-11.4782528275472,-63.0162050441979,
73.6123141673606));
#115154=CARTESIAN_POINT('Ctrl Pts',(-11.4757031884669,-63.0300337440175,
73.878136618204));
#115155=CARTESIAN_POINT('Ctrl Pts',(-11.4714847021596,-63.0526134452692,
74.1416477523053));
#115156=CARTESIAN_POINT('Ctrl Pts',(-11.4655973686252,-63.0835298833964,
74.402303678319));
#115157=CARTESIAN_POINT('Ctrl Pts',(-11.4598014315056,-63.1139663671286,
74.6589131175824));
#115158=CARTESIAN_POINT('Ctrl Pts',(-11.4523880601533,-63.1524823556258,
74.9127554294561));
#115159=CARTESIAN_POINT('Ctrl Pts',(-11.4433572545684,-63.1986578291045,
75.1633601188373));
#115160=CARTESIAN_POINT('Ctrl Pts',(-11.4342487987822,-63.2452303363555,
75.4161195998789));
#115161=CARTESIAN_POINT('Ctrl Pts',(-11.4234949745895,-63.299594321962,
75.6655854918157));
#115162=CARTESIAN_POINT('Ctrl Pts',(-11.4110957819905,-63.3612984860316,
75.9113245131054));
#115163=CARTESIAN_POINT('Ctrl Pts',(-11.398588636057,-63.423539876232,76.1592030565097));
#115164=CARTESIAN_POINT('Ctrl Pts',(-11.3844073462561,-63.4932495223862,
76.4032895248276));
#115165=CARTESIAN_POINT('Ctrl Pts',(-11.3685519125877,-63.5699480453472,
76.6431899097907));
#115166=CARTESIAN_POINT('Ctrl Pts',(-11.3524740491355,-63.6477225424026,
76.8864557650327));
#115167=CARTESIAN_POINT('Ctrl Pts',(-11.3346747404995,-63.7326830920559,
77.1254172171987));
#115168=CARTESIAN_POINT('Ctrl Pts',(-11.3151539866796,-63.8243176890293,
77.359715954205));
#115169=CARTESIAN_POINT('Ctrl Pts',(-11.2954837390822,-63.9166540417941,
77.5958089970854));
#115170=CARTESIAN_POINT('Ctrl Pts',(-11.2740655790092,-64.0157667566476,
77.8271676705252));
#115171=CARTESIAN_POINT('Ctrl Pts',(-11.2508995064605,-64.1211241869361,
78.0534783179675));
#115172=CARTESIAN_POINT('Ctrl Pts',(-11.2274340048623,-64.2278433964014,
78.2827141043994));
#115173=CARTESIAN_POINT('Ctrl Pts',(-11.2021751140965,-64.340969500323,
78.5067705421234));
#115174=CARTESIAN_POINT('Ctrl Pts',(-11.1751228341631,-64.4599465123221,
78.7253754605533));
#115175=CARTESIAN_POINT('Ctrl Pts',(-11.1504541131106,-64.5684405367777,
78.9247192410678));
#115176=CARTESIAN_POINT('Ctrl Pts',(-11.1242941090657,-64.6817996566903,
79.1195305579161));
#115177=CARTESIAN_POINT('Ctrl Pts',(-11.0966428220287,-64.7996028657007,
79.3096407899006));
#115178=CARTESIAN_POINT('Ctrl Pts',(-11.0779169478987,-64.8793809990325,
79.438386344138));
#115179=CARTESIAN_POINT('Ctrl Pts',(-11.0585071407615,-64.961197299292,
79.5649766295904));
#115180=CARTESIAN_POINT('Ctrl Pts',(-11.0384134006173,-65.0449218093244,
79.6893683409186));
#115181=CARTESIAN_POINT('Ctrl Pts',(-11.0283665305452,-65.0867840643406,
79.7515641965827));
#115182=CARTESIAN_POINT('Ctrl Pts',(-11.0181486772213,-65.1291233283142,
79.8132104383628));
#115183=CARTESIAN_POINT('Ctrl Pts',(-11.0077598406456,-65.1719235132878,
79.8743024149563));
#115184=CARTESIAN_POINT('Ctrl Pts',(-11.0025654223577,-65.1933236057745,
79.904848403253));
#115185=CARTESIAN_POINT('Ctrl Pts',(-10.9973282582569,-65.2148389261161,
79.935255826801));
#115186=CARTESIAN_POINT('Ctrl Pts',(-10.9920483483432,-65.236467460282,
79.9655241301987));
#115187=CARTESIAN_POINT('Ctrl Pts',(-10.9894083933863,-65.2472817273649,
79.9806582818975));
#115188=CARTESIAN_POINT('Ctrl Pts',(-10.9867577519762,-65.2581242977531,
79.9957576536675));
#115189=CARTESIAN_POINT('Ctrl Pts',(-10.9840964241129,-65.2689949201948,
80.0108221786826));
#115190=CARTESIAN_POINT('Ctrl Pts',(-10.9821004282154,-65.2771478870261,
80.0221205724439));
#115191=CARTESIAN_POINT('Ctrl Pts',(-10.9800984211879,-65.2853166331253,
80.0333993649144));
#115192=CARTESIAN_POINT('Ctrl Pts',(-10.9780904030305,-65.2935010525828,
80.0446585284801));
#115193=CARTESIAN_POINT('Ctrl Pts',(-10.9774210636447,-65.296229192402,
80.0484115830019));
#115194=CARTESIAN_POINT('Ctrl Pts',(-10.9764432355883,-65.3002128087954,
80.053882998953));
#115195=CARTESIAN_POINT('Ctrl Pts',(-10.9760803811631,-65.3016906925888,
80.0559111480989));
#115196=CARTESIAN_POINT('Ctrl Pts',(-10.9506866377528,-65.4051178502617,
80.1978476808771));
#115197=CARTESIAN_POINT('Ctrl Pts',(-10.9232759588804,-65.5140065031049,
80.340734749093));
#115198=CARTESIAN_POINT('Ctrl Pts',(-10.8938483445461,-65.6286728917096,
80.4841030746226));
#115199=CARTESIAN_POINT('Ctrl Pts',(-10.8648132081499,-65.7418099674972,
80.625559287802));
#115200=CARTESIAN_POINT('Ctrl Pts',(-10.8338145775144,-65.8605720396774,
80.7674840000695));
#115201=CARTESIAN_POINT('Ctrl Pts',(-10.8008524526395,-65.9852439685844,
80.9093801348895));
#115202=CARTESIAN_POINT('Ctrl Pts',(-10.7685610860177,-66.1073789031209,
81.0483887737158));
#115203=CARTESIAN_POINT('Ctrl Pts',(-10.7343853237954,-66.2351859267227,
81.1873698930677));
#115204=CARTESIAN_POINT('Ctrl Pts',(-10.6983251659726,-66.3689098151028,
81.3258122133891));
#115205=CARTESIAN_POINT('Ctrl Pts',(-10.6720325297249,-66.4664122601025,
81.4267550208881));
#115206=CARTESIAN_POINT('Ctrl Pts',(-10.6447380840791,-66.5670598666787,
81.5274104787523));
#115207=CARTESIAN_POINT('Ctrl Pts',(-10.6164418290353,-66.6709380618347,
81.6275656295125));
#115208=CARTESIAN_POINT('Ctrl Pts',(-10.5788107064715,-66.8090854275401,
81.7607617272937));
#115209=CARTESIAN_POINT('Ctrl Pts',(-10.5394077560457,-66.9529478270377,
81.893074375948));
#115210=CARTESIAN_POINT('Ctrl Pts',(-10.498232977758,-67.1027000784011,
82.0239684647239));
#115211=CARTESIAN_POINT('Ctrl Pts',(-10.4575611058947,-67.2506232641955,
82.1532638204671));
#115212=CARTESIAN_POINT('Ctrl Pts',(-10.415160423859,-67.4042936052472,
82.2811749400427));
#115213=CARTESIAN_POINT('Ctrl Pts',(-10.371030931651,-67.5638460348357,
82.4071490032168));
#115214=CARTESIAN_POINT('Ctrl Pts',(-10.3277609374189,-67.7202909056594,
82.5306695042285));
#115215=CARTESIAN_POINT('Ctrl Pts',(-10.2828288203227,-67.8823912045507,
82.6523274841528));
#115216=CARTESIAN_POINT('Ctrl Pts',(-10.2362345803624,-68.0502377910592,
82.771568224157));
#115217=CARTESIAN_POINT('Ctrl Pts',(-10.1907005843092,-68.2142650573938,
82.888095661655));
#115218=CARTESIAN_POINT('Ctrl Pts',(-10.1435792474133,-68.3837802585928,
83.0023143992325));
#115219=CARTESIAN_POINT('Ctrl Pts',(-10.0948705696749,-68.5588301155626,
83.1136773112635));
#115220=CARTESIAN_POINT('Ctrl Pts',(-10.0948705696749,-68.55883030701,83.11367701033));
#115221=CARTESIAN_POINT('Ctrl Pts',(-10.0502938077784,-68.718948701588,
83.2155412734439));
#115222=CARTESIAN_POINT('Ctrl Pts',(-9.99901505528794,-68.8951734040083,
83.3223532112927));
#115223=CARTESIAN_POINT('Ctrl Pts',(-9.91204394066144,-69.1852539436349,
83.4865593135653));
#115224=CARTESIAN_POINT('Ctrl Pts',(-9.8813780714708,-69.2862378191267,
83.5419522481948));
#115225=CARTESIAN_POINT('Ctrl Pts',(-9.83286602121212,-69.4443386154877,
83.6255326581122));
#115226=CARTESIAN_POINT('Ctrl Pts',(-9.8079816844646,-69.5250451157206,
83.6674449107169));
#115227=CARTESIAN_POINT('Ctrl Pts',(-9.77785041292734,-69.6221403905299,
83.7164402392164));
#115228=CARTESIAN_POINT('Ctrl Pts',(-9.76250989082578,-69.6714272090312,
83.7409472746058));
#115229=CARTESIAN_POINT('Ctrl Pts',(-9.75477090819175,-69.6962560014835,
83.7532012372322));
#115230=CARTESIAN_POINT('Ctrl Pts',(-9.75143947529504,-69.7069366999104,
83.7584528258423));
#115231=CARTESIAN_POINT('Ctrl Pts',(-9.74921524757422,-69.714066014065,
83.7619538376723));
#115232=CARTESIAN_POINT('Ctrl Pts',(-9.74760316095839,-69.7192316813361,
83.7644863914133));
#115233=CARTESIAN_POINT('Ctrl Pts',(-9.72724051790498,-69.7844701446807,
83.7964427918803));
#115234=CARTESIAN_POINT('Ctrl Pts',(-9.69988686319735,-69.871555510311,
83.8385058175468));
#115235=CARTESIAN_POINT('Ctrl Pts',(-9.64744428897033,-70.0391065537308,
83.9156142440336));
#115236=CARTESIAN_POINT('Ctrl Pts',(-9.62806141553372,-70.1011166189966,
83.9436375961161));
#115237=CARTESIAN_POINT('Ctrl Pts',(-9.59613408233741,-70.2035640260259,
83.9886890950437));
#115238=CARTESIAN_POINT('Ctrl Pts',(-9.57945715997892,-70.2571461972045,
84.0119674793892));
#115239=CARTESIAN_POINT('Ctrl Pts',(-9.5617103539799,-70.3143052101089,
84.0362741519362));
#115240=CARTESIAN_POINT('Ctrl Pts',(-9.54964139806043,-70.353210584381,
84.0526949680574));
#115241=CARTESIAN_POINT('Ctrl Pts',(-9.54306984809565,-70.3744133871288,
84.0615750413791));
#115242=CARTESIAN_POINT('Ctrl Pts',(-9.49038354358189,-70.5445482096079,
84.1323077681235));
#115243=CARTESIAN_POINT('Ctrl Pts',(-9.44837032070452,-70.682363037354,
84.1860064293701));
#115244=CARTESIAN_POINT('Ctrl Pts',(-9.39257905809074,-70.8678500066756,
84.2551971750906));
#115245=CARTESIAN_POINT('Ctrl Pts',(-9.3751867325032,-70.9261439148029,
84.2763632109177));
#115246=CARTESIAN_POINT('Ctrl Pts',(-9.35090538704745,-71.0081767458892,
84.3055226886024));
#115247=CARTESIAN_POINT('Ctrl Pts',(-9.33921650005097,-71.0478414726449,
84.3194545615856));
#115248=CARTESIAN_POINT('Ctrl Pts',(-9.32637009025168,-71.0917316627996,
84.3346257467507));
#115249=CARTESIAN_POINT('Ctrl Pts',(-9.32014454160952,-71.1130781654726,
84.3419466755683));
#115250=CARTESIAN_POINT('Ctrl Pts',(-9.31751880424662,-71.1220981592162,
84.3450281366084));
#115251=CARTESIAN_POINT('Ctrl Pts',(-9.3157777248741,-71.1280829053576,
84.3470700511436));
#115252=CARTESIAN_POINT('Ctrl Pts',(-9.31544127521446,-71.1292389848438,
84.3474647690699));
#115253=CARTESIAN_POINT('Ctrl Pts',(-9.26955439872479,-71.2871697016937,
84.4012099517279));
#115254=CARTESIAN_POINT('Ctrl Pts',(-9.22873605973666,-71.4324726572279,
84.4472137338849));
#115255=CARTESIAN_POINT('Ctrl Pts',(-9.1730255903936,-71.6380168485605,
84.5085326682448));
#115256=CARTESIAN_POINT('Ctrl Pts',(-9.14654961550685,-71.7376891690263,
84.5372682003853));
#115257=CARTESIAN_POINT('Ctrl Pts',(-9.11807468276234,-71.848434346492,
84.567725331802));
#115258=CARTESIAN_POINT('Ctrl Pts',(-9.10444064254594,-71.90240961628,84.5822224138533));
#115259=CARTESIAN_POINT('Ctrl Pts',(-9.0977744789767,-71.9290463969955,
84.5892924535069));
#115260=CARTESIAN_POINT('Ctrl Pts',(-9.09494987813394,-71.9403868187052,
84.5922846825071));
#115261=CARTESIAN_POINT('Ctrl Pts',(-9.09307399455015,-71.9479303399745,
84.5942711555288));
#115262=CARTESIAN_POINT('Ctrl Pts',(-9.09244019876047,-71.9504811837714,
84.5949421765475));
#115263=CARTESIAN_POINT('Ctrl Pts',(-9.05180689196814,-72.1144096422424,
84.637939790309));
#115264=CARTESIAN_POINT('Ctrl Pts',(-9.01546444294639,-72.2711841971463,
84.6755717545402));
#115265=CARTESIAN_POINT('Ctrl Pts',(-8.96554008757908,-72.5027421373977,
84.7264337754863));
#115266=CARTESIAN_POINT('Ctrl Pts',(-8.94172523943675,-72.6176208899744,
84.7504682609118));
#115267=CARTESIAN_POINT('Ctrl Pts',(-8.91594907663469,-72.7500075021818,
84.7761749791267));
#115268=CARTESIAN_POINT('Ctrl Pts',(-8.90356295190799,-72.815783810216,
84.7884586800507));
#115269=CARTESIAN_POINT('Ctrl Pts',(-8.8983621748839,-72.8438835247074,
84.7936025209064));
#115270=CARTESIAN_POINT('Ctrl Pts',(-8.89491889289996,-72.8625965537548,
84.797005110384));
#115271=CARTESIAN_POINT('Ctrl Pts',(-8.89356984042164,-72.8699597621748,
84.7983373347971));
#115272=CARTESIAN_POINT('Ctrl Pts',(-8.75977543568638,-73.6057342558853,
84.9303191698575));
#115273=CARTESIAN_POINT('Ctrl Pts',(-8.693708869803,-74.3160938546077,84.98888938658));
#115274=CARTESIAN_POINT('Ctrl Pts',(-8.69331176731091,-74.99999999459,84.98885921934));
#115275=CARTESIAN_POINT('Origin',(27.4324635166691,25.,72.98888938658));
#115276=CARTESIAN_POINT('',(-8.23395173818595,-10.,84.5714980248889));
#115277=CARTESIAN_POINT('',(-7.08815755488265,-10.,58.3404518987683));
#115278=CARTESIAN_POINT('Origin',(27.4324635166691,-10.,72.98888938658));
#115279=CARTESIAN_POINT('',(-8.23395173885291,-22.5,84.57149802283));
#115280=CARTESIAN_POINT('',(-8.23395173707291,-10.,84.57149802832));
#115281=CARTESIAN_POINT('',(-7.08815755056573,-22.5,87.637326884565));
#115282=CARTESIAN_POINT('Origin',(27.4324635166691,-22.5,72.98888938658));
#115283=CARTESIAN_POINT('',(-7.08838231939817,-64.8259873690431,87.6374222559034));
#115284=CARTESIAN_POINT('',(-7.08815755142093,25.,87.63732688255));
#115285=CARTESIAN_POINT('',(-10.0675288996373,-56.3106244902745,72.9888900918571));
#115286=CARTESIAN_POINT('Ctrl Pts',(-7.08827439219835,-64.8259873732546,
87.6373764712027));
#115287=CARTESIAN_POINT('Ctrl Pts',(-7.14208955312506,-64.5902694889972,
87.5106518782322));
#115288=CARTESIAN_POINT('Ctrl Pts',(-7.19693271715934,-64.3590102276896,
87.3795061726048));
#115289=CARTESIAN_POINT('Ctrl Pts',(-7.25261931495788,-64.1321728080882,
87.2440051558485));
#115290=CARTESIAN_POINT('Ctrl Pts',(-7.30862354726613,-63.9040415153574,
87.1077312457799));
#115291=CARTESIAN_POINT('Ctrl Pts',(-7.36548116596207,-63.6803822131273,
86.9670520486309));
#115292=CARTESIAN_POINT('Ctrl Pts',(-7.42302254145316,-63.4611762104035,
86.8219885103422));
#115293=CARTESIAN_POINT('Ctrl Pts',(-7.4806154753667,-63.2417737939584,
86.6767949917199));
#115294=CARTESIAN_POINT('Ctrl Pts',(-7.53889369791152,-63.0268322400467,
86.5272091019534));
#115295=CARTESIAN_POINT('Ctrl Pts',(-7.59770061678909,-62.8163579553965,
86.3732083557253));
#115296=CARTESIAN_POINT('Ctrl Pts',(-7.61918115792911,-62.7394775199539,
86.3169561420728));
#115297=CARTESIAN_POINT('Ctrl Pts',(-7.64073234701225,-62.6631933984299,
86.2601144748895));
#115298=CARTESIAN_POINT('Ctrl Pts',(-7.6623468788977,-62.5875069082207,
86.2026808795064));
#115299=CARTESIAN_POINT('Ctrl Pts',(-7.72171944494865,-62.3796050594585,
86.044917576859));
#115300=CARTESIAN_POINT('Ctrl Pts',(-7.78156955763312,-62.1762098056603,
85.8826908973321));
#115301=CARTESIAN_POINT('Ctrl Pts',(-7.84171474168083,-61.9772731854025,
85.7159708650554));
#115302=CARTESIAN_POINT('Ctrl Pts',(-7.90063733995764,-61.7823803981647,
85.5526397913863));
#115303=CARTESIAN_POINT('Ctrl Pts',(-7.95984346167794,-61.5917666858401,
85.3849958682327));
#115304=CARTESIAN_POINT('Ctrl Pts',(-8.01916413597774,-61.4054240949616,
85.2129748040599));
#115305=CARTESIAN_POINT('Ctrl Pts',(-8.08033107846091,-61.2132818667592,
85.0355998388838));
#115306=CARTESIAN_POINT('Ctrl Pts',(-8.14162016396233,-61.0256802340243,
84.8535710238742));
#115307=CARTESIAN_POINT('Ctrl Pts',(-8.20284384296533,-60.8426558696489,
84.6667810946507));
#115308=CARTESIAN_POINT('Ctrl Pts',(-8.26406752196834,-60.6596315052735,
84.4799911654272));
#115309=CARTESIAN_POINT('Ctrl Pts',(-8.32522614611897,-60.4811840784473,
84.28843993731));
#115310=CARTESIAN_POINT('Ctrl Pts',(-8.38612459115579,-60.307401135805,
84.0919856472692));
#115311=CARTESIAN_POINT('Ctrl Pts',(-8.40695694934915,-60.2479528443613,
84.0247818601072));
#115312=CARTESIAN_POINT('Ctrl Pts',(-8.42775877187844,-60.1890508569645,
83.9570040220028));
#115313=CARTESIAN_POINT('Ctrl Pts',(-8.44852208912459,-60.1306987436672,
83.8886487292554));
#115314=CARTESIAN_POINT('Ctrl Pts',(-8.46296549103274,-60.0901077815126,
83.8410993442512));
#115315=CARTESIAN_POINT('Ctrl Pts',(-8.4773880041915,-60.0497767660536,
83.7932779384106));
#115316=CARTESIAN_POINT('Ctrl Pts',(-8.49178675063624,-60.0097056972605,
83.7451840627535));
#115317=CARTESIAN_POINT('Ctrl Pts',(-8.49538643724743,-59.9996879300622,
83.7331605938392));
#115318=CARTESIAN_POINT('Ctrl Pts',(-8.49884248469713,-59.9900827858179,
83.7215930957605));
#115319=CARTESIAN_POINT('Ctrl Pts',(-8.50162619849312,-59.9823533344902,
83.712263964152));
#115320=CARTESIAN_POINT('Ctrl Pts',(-8.50440991228911,-59.9746238831625,
83.7029348325435));
#115321=CARTESIAN_POINT('Ctrl Pts',(-8.50719220167007,-59.9669062119242,
83.6935972057491));
#115322=CARTESIAN_POINT('Ctrl Pts',(-8.5099730494076,-59.9592003207754,
83.6842510817912));
#115323=CARTESIAN_POINT('Ctrl Pts',(-8.51553474488267,-59.9437885384776,
83.6655588338753));
#115324=CARTESIAN_POINT('Ctrl Pts',(-8.52109067384868,-59.9284238765374,
83.6468325973273));
#115325=CARTESIAN_POINT('Ctrl Pts',(-8.52664069770649,-59.9131063349545,
83.6280723560549));
#115326=CARTESIAN_POINT('Ctrl Pts',(-8.54884079313775,-59.8518361686228,
83.5530313909652));
#115327=CARTESIAN_POINT('Ctrl Pts',(-8.5709464276222,-59.7913199280025,
83.4774463572037));
#115328=CARTESIAN_POINT('Ctrl Pts',(-8.59294854414954,-59.7315576131294,
83.4013162397247));
#115329=CARTESIAN_POINT('Ctrl Pts',(-8.63695277720424,-59.6120329833831,
83.2490560047667));
#115330=CARTESIAN_POINT('Ctrl Pts',(-8.68054321499461,-59.4955240566604,
83.0946155134775));
#115331=CARTESIAN_POINT('Ctrl Pts',(-8.72364395735391,-59.3820308335148,
82.937986299838));
#115332=CARTESIAN_POINT('Ctrl Pts',(-8.77931417365709,-59.2354395699865,
82.7356792924547));
#115333=CARTESIAN_POINT('Ctrl Pts',(-8.83416874073783,-59.0938841685608,
82.5297174962948));
#115334=CARTESIAN_POINT('Ctrl Pts',(-8.88802887219702,-58.9573534873692,
82.3200954780129));
#115335=CARTESIAN_POINT('Ctrl Pts',(-8.91756743410084,-58.8824758391183,
82.2051322798983));
#115336=CARTESIAN_POINT('Ctrl Pts',(-8.94680683515967,-58.8091101854314,
82.0890675858819));
#115337=CARTESIAN_POINT('Ctrl Pts',(-8.97571685333632,-58.7372599362983,
81.9718964272046));
#115338=CARTESIAN_POINT('Ctrl Pts',(-8.9810958478393,-58.723891487591,81.9500955755213));
#115339=CARTESIAN_POINT('Ctrl Pts',(-8.98646348068979,-58.7105757369594,
81.9282562377321));
#115340=CARTESIAN_POINT('Ctrl Pts',(-8.99181954156358,-58.6973126643615,
81.9063784200908));
#115341=CARTESIAN_POINT('Ctrl Pts',(-9.04421400583836,-58.5675696312296,
81.692363575631));
#115342=CARTESIAN_POINT('Ctrl Pts',(-9.09550157275799,-58.4428643549359,
81.4746692484697));
#115343=CARTESIAN_POINT('Ctrl Pts',(-9.14550683304999,-58.3231561767416,
81.2533245862162));
#115344=CARTESIAN_POINT('Ctrl Pts',(-9.19551814217404,-58.2034335181774,
81.0319531492457));
#115345=CARTESIAN_POINT('Ctrl Pts',(-9.24424716833884,-58.0887087970384,
80.8069302641477));
#115346=CARTESIAN_POINT('Ctrl Pts',(-9.29150993392781,-57.9789829137176,
80.5782535255859));
#115347=CARTESIAN_POINT('Ctrl Pts',(-9.33877269951677,-57.8692570303968,
80.349576787024));
#115348=CARTESIAN_POINT('Ctrl Pts',(-9.38456956736444,-57.7645295954233,
80.1172459456955));
#115349=CARTESIAN_POINT('Ctrl Pts',(-9.4287028391648,-57.6648487671302,
79.8812306242836));
#115350=CARTESIAN_POINT('Ctrl Pts',(-9.43407045269604,-57.6527253024305,
79.8525257723405));
#115351=CARTESIAN_POINT('Ctrl Pts',(-9.43941336419247,-57.6406759877037,
79.8237667794555));
#115352=CARTESIAN_POINT('Ctrl Pts',(-9.44473119037857,-57.6287008573064,
79.7949536339167));
#115353=CARTESIAN_POINT('Ctrl Pts',(-9.4563678165064,-57.6024965192201,
79.7319038480703));
#115354=CARTESIAN_POINT('Ctrl Pts',(-9.46788432996337,-57.5766473867214,
79.6685947689743));
#115355=CARTESIAN_POINT('Ctrl Pts',(-9.4792774035311,-57.5511533674906,
79.6050267292126));
#115356=CARTESIAN_POINT('Ctrl Pts',(-9.48135235335323,-57.5465102998975,
79.5934494764184));
#115357=CARTESIAN_POINT('Ctrl Pts',(-9.48342320871521,-57.541879012395,
79.5818636331032));
#115358=CARTESIAN_POINT('Ctrl Pts',(-9.48548994915482,-57.537259504983,
79.5702692013485));
#115359=CARTESIAN_POINT('Ctrl Pts',(-9.48755668959442,-57.5326399975709,
79.5586747695938));
#115360=CARTESIAN_POINT('Ctrl Pts',(-9.48889802164019,-57.5296438207682,
79.5511269172421));
#115361=CARTESIAN_POINT('Ctrl Pts',(-9.49042437195825,-57.5262355074984,
79.5425266149269));
#115362=CARTESIAN_POINT('Ctrl Pts',(-9.49347707259439,-57.5194188809588,
79.5253260102966));
#115363=CARTESIAN_POINT('Ctrl Pts',(-9.49652001932305,-57.5126304293838,
79.5081104005636));
#115364=CARTESIAN_POINT('Ctrl Pts',(-9.49955316118484,-57.5058701527735,
79.4908797944758));
#115365=CARTESIAN_POINT('Ctrl Pts',(-9.50561944490843,-57.492349599553,
79.4564185823002));
#115366=CARTESIAN_POINT('Ctrl Pts',(-9.51164650964414,-57.4789417461908,
79.4218973848201));
#115367=CARTESIAN_POINT('Ctrl Pts',(-9.51763394201365,-57.4656465926865,
79.3873162705839));
#115368=CARTESIAN_POINT('Ctrl Pts',(-9.54158367149169,-57.4124659786691,
79.2489918136391));
#115369=CARTESIAN_POINT('Ctrl Pts',(-9.5648994423365,-57.3610885623673,
79.1097087217166));
#115370=CARTESIAN_POINT('Ctrl Pts',(-9.58755352231721,-57.3115143438162,
78.9694712267336));
#115371=CARTESIAN_POINT('Ctrl Pts',(-9.62609916515577,-57.2271644110935,
78.7308588267249));
#115372=CARTESIAN_POINT('Ctrl Pts',(-9.66273029453766,-57.1480362853527,
78.48948291296));
#115373=CARTESIAN_POINT('Ctrl Pts',(-9.69729491697327,-57.0741259973634,
78.2453693959728));
#115374=CARTESIAN_POINT('Ctrl Pts',(-9.70335899669416,-57.0611590430911,
78.202541680128));
#115375=CARTESIAN_POINT('Ctrl Pts',(-9.70935942942061,-57.0483528046862,
78.159629649545));
#115376=CARTESIAN_POINT('Ctrl Pts',(-9.71529534017754,-57.0357074057499,
78.1166333803834));
#115377=CARTESIAN_POINT('Ctrl Pts',(-9.72742678734184,-57.0098635217449,
78.0287602655483));
#115378=CARTESIAN_POINT('Ctrl Pts',(-9.73928886456698,-56.9846922496317,
77.9405345025405));
#115379=CARTESIAN_POINT('Ctrl Pts',(-9.75087363454091,-56.9601929819792,
77.8519582094545));
#115380=CARTESIAN_POINT('Ctrl Pts',(-9.78311100811269,-56.8920179517175,
77.6054736390878));
#115381=CARTESIAN_POINT('Ctrl Pts',(-9.81320230114342,-56.8290436401664,
77.3562760559548));
#115382=CARTESIAN_POINT('Ctrl Pts',(-9.84101052750768,-56.7712538627715,
77.1044066262465));
#115383=CARTESIAN_POINT('Ctrl Pts',(-9.86872917611775,-56.7136502417465,
76.8533485355128));
#115384=CARTESIAN_POINT('Ctrl Pts',(-9.89417981525409,-56.661197513563,
76.5996355006453));
#115385=CARTESIAN_POINT('Ctrl Pts',(-9.91720607264976,-56.6139237675165,
76.3432915265767));
#115386=CARTESIAN_POINT('Ctrl Pts',(-9.92060784437707,-56.6069398061206,
76.3054206877135));
#115387=CARTESIAN_POINT('Ctrl Pts',(-9.92395664213361,-56.6000685445888,
76.2674925987102));
#115388=CARTESIAN_POINT('Ctrl Pts',(-9.9272519106857,-56.5933099829211,
76.2295073886416));
#115389=CARTESIAN_POINT('Ctrl Pts',(-9.92950591356342,-56.5886870463661,
76.2035250532258));
#115390=CARTESIAN_POINT('Ctrl Pts',(-9.93150317406151,-56.5845931209331,
76.1802069722421));
#115391=CARTESIAN_POINT('Ctrl Pts',(-9.93346399982777,-56.5805746185882,
76.157082382999));
#115392=CARTESIAN_POINT('Ctrl Pts',(-9.93436982855763,-56.5787182196476,
76.1463996810155));
#115393=CARTESIAN_POINT('Ctrl Pts',(-9.93526760888132,-56.5768786059676,
76.135758163069));
#115394=CARTESIAN_POINT('Ctrl Pts',(-9.93617772172492,-56.5750144321809,
76.124913722644));
#115395=CARTESIAN_POINT('Ctrl Pts',(-9.93748512336717,-56.5723364962664,
76.1093353915387));
#115396=CARTESIAN_POINT('Ctrl Pts',(-9.93878300849999,-56.5696788927295,
76.0937531901985));
#115397=CARTESIAN_POINT('Ctrl Pts',(-9.9400713590507,-56.5670416263439,
76.0781671294405));
#115398=CARTESIAN_POINT('Ctrl Pts',(-9.94445949385756,-56.5580590707693,
76.0250808512716));
#115399=CARTESIAN_POINT('Ctrl Pts',(-9.94873702206621,-56.5493124387524,
75.9719498006223));
#115400=CARTESIAN_POINT('Ctrl Pts',(-9.95290366859442,-56.5408017072184,
75.9187744460697));
#115401=CARTESIAN_POINT('Ctrl Pts',(-9.96368360542344,-56.5187827652024,
75.7811993100327));
#115402=CARTESIAN_POINT('Ctrl Pts',(-9.97372148030912,-56.4983429057096,
75.6433276363244));
#115403=CARTESIAN_POINT('Ctrl Pts',(-9.98301121954607,-56.4794821288461,
75.5051674707858));
#115404=CARTESIAN_POINT('Ctrl Pts',(-10.00159069802,-56.4417605751189,75.2288471397085));
#115405=CARTESIAN_POINT('Ctrl Pts',(-10.0171796586205,-56.4103553524075,
74.9513729078636));
#115406=CARTESIAN_POINT('Ctrl Pts',(-10.0297059689885,-56.3852664608848,
74.672808313959));
#115407=CARTESIAN_POINT('Ctrl Pts',(-10.0349411749523,-56.374780890061,
74.5563859213738));
#115408=CARTESIAN_POINT('Ctrl Pts',(-10.0396410471935,-56.3653997046156,
74.4397728123101));
#115409=CARTESIAN_POINT('Ctrl Pts',(-10.0437985795037,-56.3571233343035,
74.3229742968176));
#115410=CARTESIAN_POINT('Ctrl Pts',(-10.0532545573527,-56.338299385744,
74.0573253269758));
#115411=CARTESIAN_POINT('Ctrl Pts',(-10.0599068555642,-56.3251877634295,
73.7907175155284));
#115412=CARTESIAN_POINT('Ctrl Pts',(-10.0637172608622,-56.3177898385427,
73.5232108702605));
#115413=CARTESIAN_POINT('Ctrl Pts',(-10.0662486708131,-56.3128750908428,
73.345495133801));
#115414=CARTESIAN_POINT('Ctrl Pts',(-10.0675252675775,-56.3104829476421,
73.1673825891876));
#115415=CARTESIAN_POINT('Ctrl Pts',(-10.0675288996373,-56.3106244902745,
72.9888900918571));
#115416=CARTESIAN_POINT('',(-7.08825603872491,-64.825987319,58.34041012264));
#115417=CARTESIAN_POINT('Ctrl Pts',(-10.0675326914397,-56.3106244903022,
72.9888900919343));
#115418=CARTESIAN_POINT('Ctrl Pts',(-10.0675364861884,-56.3106236438183,
72.8373894080529));
#115419=CARTESIAN_POINT('Ctrl Pts',(-10.0665997793874,-56.3125565421587,
72.6820441351514));
#115420=CARTESIAN_POINT('Ctrl Pts',(-10.0627950071674,-56.3200932749138,
72.3728615295497));
#115421=CARTESIAN_POINT('Ctrl Pts',(-10.0599294447923,-56.3257673245125,
72.2179451440282));
#115422=CARTESIAN_POINT('Ctrl Pts',(-10.0484874118121,-56.3485897944341,
71.7544431528985));
#115423=CARTESIAN_POINT('Ctrl Pts',(-10.0141911002797,-56.4173278124564,
70.8296920351912));
#115424=CARTESIAN_POINT('Ctrl Pts',(-9.94612028955057,-56.5553450650161,
69.9125366186336));
#115425=CARTESIAN_POINT('Ctrl Pts',(-9.82621684669285,-56.8009496102399,
68.6978275958031));
#115426=CARTESIAN_POINT('Ctrl Pts',(-9.75383725762295,-56.9508618239222,
68.1137141942851));
#115427=CARTESIAN_POINT('Ctrl Pts',(-9.58475593550578,-57.3152540454977,
66.9627992394608));
#115428=CARTESIAN_POINT('Ctrl Pts',(-9.48823107615905,-57.5285692202934,
66.3988547901617));
#115429=CARTESIAN_POINT('Ctrl Pts',(-9.36773885117348,-57.8035577389473,
65.7777835756058));
#115430=CARTESIAN_POINT('Ctrl Pts',(-9.35418547529567,-57.8345982541729,
65.7089611577416));
#115431=CARTESIAN_POINT('Ctrl Pts',(-9.33875494628785,-57.8700658485987,
65.631745287302));
#115432=CARTESIAN_POINT('Ctrl Pts',(-9.33693933149597,-57.8742404593784,
65.6226733259747));
#115433=CARTESIAN_POINT('Ctrl Pts',(-9.33254286197359,-57.8843567207882,
65.6007616913834));
#115434=CARTESIAN_POINT('Ctrl Pts',(-9.32593778198101,-57.8995651499525,
65.5679186925187));
#115435=CARTESIAN_POINT('Ctrl Pts',(-9.31045372056789,-57.9352897440166,
65.4914562102728));
#115436=CARTESIAN_POINT('Ctrl Pts',(-9.26134090855832,-58.0490646698304,
65.2522216414933));
#115437=CARTESIAN_POINT('Ctrl Pts',(-9.141804444225,-58.3297867322916,64.6952379674525));
#115438=CARTESIAN_POINT('Ctrl Pts',(-9.02454771227377,-58.6150552440629,
64.19989351254));
#115439=CARTESIAN_POINT('Ctrl Pts',(-8.78268079338333,-59.2204462064251,
63.2342091003427));
#115440=CARTESIAN_POINT('Ctrl Pts',(-8.61166284917084,-59.6705120997594,
62.6237793667378));
#115441=CARTESIAN_POINT('Ctrl Pts',(-8.42446623526063,-60.1980835247549,
62.0101821405832));
#115442=CARTESIAN_POINT('Ctrl Pts',(-8.41343432384315,-60.2292986689213,
61.9742166981781));
#115443=CARTESIAN_POINT('Ctrl Pts',(-8.39962032684187,-60.2685445127935,
61.9294203517137));
#115444=CARTESIAN_POINT('Ctrl Pts',(-8.39591465393794,-60.2790823039808,
61.9174185017987));
#115445=CARTESIAN_POINT('Ctrl Pts',(-8.38867784863578,-60.2996915603767,
61.8940265584313));
#115446=CARTESIAN_POINT('Ctrl Pts',(-8.37781951720245,-60.3306539737948,
61.8589894052093));
#115447=CARTESIAN_POINT('Ctrl Pts',(-8.33797279171314,-60.444716640061,
61.7310779500568));
#115448=CARTESIAN_POINT('Ctrl Pts',(-8.24355473748462,-60.7185251372143,
61.4331346970249));
#115449=CARTESIAN_POINT('Ctrl Pts',(-8.15608967698741,-60.9805889765312,
61.1678034254881));
#115450=CARTESIAN_POINT('Ctrl Pts',(-7.98128295927112,-61.5171400341676,
60.6499539622089));
#115451=CARTESIAN_POINT('Ctrl Pts',(-7.86491848259896,-61.8914052445958,
60.3218068716169));
#115452=CARTESIAN_POINT('Ctrl Pts',(-7.52031758516955,-63.063894391892,
59.3876499202851));
#115453=CARTESIAN_POINT('Ctrl Pts',(-7.29670946703427,-63.9118118447716,
58.8319269483214));
#115454=CARTESIAN_POINT('Ctrl Pts',(-7.08825603872491,-64.825987319,58.34041012264));
#115455=CARTESIAN_POINT('',(-7.08815756005477,25.,58.3404519109566));
#115456=CARTESIAN_POINT('Origin',(6.43246351666909,-92.5,72.98888938658));
#115457=CARTESIAN_POINT('',(14.224188353942,-89.,69.5919754841955));
#115458=CARTESIAN_POINT('',(14.2241883540028,-89.,76.3858032888256));
#115459=CARTESIAN_POINT('Origin',(6.43246351666909,-89.,72.98888938658));
#115460=CARTESIAN_POINT('',(14.2241130800822,-26.6269674540304,76.3859511531206));
#115461=CARTESIAN_POINT('',(14.2241160297191,-26.62696745403,76.385952439033));
#115462=CARTESIAN_POINT('',(14.9324318700046,-25.5800517253112,72.9888915205226));
#115463=CARTESIAN_POINT('Ctrl Pts',(14.9324318700046,-25.5800517253112,
72.9888915205226));
#115464=CARTESIAN_POINT('Ctrl Pts',(14.9324322830594,-25.5815074595943,
72.9978095054497));
#115465=CARTESIAN_POINT('Ctrl Pts',(14.932422196367,-25.5836894834383,73.011062863635));
#115466=CARTESIAN_POINT('Ctrl Pts',(14.9323408487722,-25.5866504441077,
73.0286517844855));
#115467=CARTESIAN_POINT('Ctrl Pts',(14.9322592991564,-25.5896187581116,
73.0462843861658));
#115468=CARTESIAN_POINT('Ctrl Pts',(14.9321061543371,-25.5933699393119,
73.0682741904377));
#115469=CARTESIAN_POINT('Ctrl Pts',(14.9317800569268,-25.5979909573379,
73.0946204833495));
#115470=CARTESIAN_POINT('Ctrl Pts',(14.9314522032137,-25.6026368633467,
73.1211086727178));
#115471=CARTESIAN_POINT('Ctrl Pts',(14.9309495708688,-25.6081620793749,
73.152000526072));
#115472=CARTESIAN_POINT('Ctrl Pts',(14.9301281339321,-25.6146882494659,
73.1872928876012));
#115473=CARTESIAN_POINT('Ctrl Pts',(14.9294390067672,-25.6201632419956,
73.2169006687399));
#115474=CARTESIAN_POINT('Ctrl Pts',(14.9285247921834,-25.626343334206,73.2496055449496));
#115475=CARTESIAN_POINT('Ctrl Pts',(14.9272780733121,-25.6333174822889,
73.2854032475674));
#115476=CARTESIAN_POINT('Ctrl Pts',(14.9257812819554,-25.6416905364001,
73.3283814145796));
#115477=CARTESIAN_POINT('Ctrl Pts',(14.9238063101476,-25.6512075171394,
73.3758179348384));
#115478=CARTESIAN_POINT('Ctrl Pts',(14.9211282881862,-25.6620501269969,
73.4276988568622));
#115479=CARTESIAN_POINT('Ctrl Pts',(14.9209004886526,-25.6629724276743,
73.432111983421));
#115480=CARTESIAN_POINT('Ctrl Pts',(14.9206675765875,-25.663904337248,73.4365572627827));
#115481=CARTESIAN_POINT('Ctrl Pts',(14.9204293993517,-25.6648459769638,
73.4410346832428));
#115482=CARTESIAN_POINT('Ctrl Pts',(14.9175353168443,-25.6762878052311,
73.4954396484616));
#115483=CARTESIAN_POINT('Ctrl Pts',(14.9138678415203,-25.6891646855909,
73.5545910535414));
#115484=CARTESIAN_POINT('Ctrl Pts',(14.9091275338572,-25.7036970772543,
73.6184639971648));
#115485=CARTESIAN_POINT('Ctrl Pts',(14.9057789676978,-25.7139627980468,
73.6635840173669));
#115486=CARTESIAN_POINT('Ctrl Pts',(14.9018940489071,-25.7250551143502,
73.71105991217));
#115487=CARTESIAN_POINT('Ctrl Pts',(14.8973527386311,-25.7370561031237,
73.7608788972865));
#115488=CARTESIAN_POINT('Ctrl Pts',(14.8958761541438,-25.7409581650348,
73.7770772929306));
#115489=CARTESIAN_POINT('Ctrl Pts',(14.8943300819425,-25.7449563112392,
73.7935233685791));
#115490=CARTESIAN_POINT('Ctrl Pts',(14.8927101227617,-25.7490534109817,
73.8102165937442));
#115491=CARTESIAN_POINT('Ctrl Pts',(14.8919001431713,-25.751101960853,73.8185632063267));
#115492=CARTESIAN_POINT('Ctrl Pts',(14.8910716896904,-25.753175249109,73.8269716060774));
#115493=CARTESIAN_POINT('Ctrl Pts',(14.890224199929,-25.7552736361177,73.8354417213194));
#115494=CARTESIAN_POINT('Ctrl Pts',(14.8893767101676,-25.7573720231265,
73.8439118365614));
#115495=CARTESIAN_POINT('Ctrl Pts',(14.8887607019875,-25.758878463585,73.849958788021));
#115496=CARTESIAN_POINT('Ctrl Pts',(14.8882268814574,-25.7601790630543,
73.8551710985703));
#115497=CARTESIAN_POINT('Ctrl Pts',(14.8860915993371,-25.7653814609316,
73.8760203407674));
#115498=CARTESIAN_POINT('Ctrl Pts',(14.8838992970071,-25.7705918971331,
73.8966649244407));
#115499=CARTESIAN_POINT('Ctrl Pts',(14.8816544011347,-25.7758047260644,
73.9171044047801));
#115500=CARTESIAN_POINT('Ctrl Pts',(14.8722952428081,-25.7975374451164,
74.00231830488));
#115501=CARTESIAN_POINT('Ctrl Pts',(14.8620235677878,-25.8193217618782,
74.0839701106493));
#115502=CARTESIAN_POINT('Ctrl Pts',(14.8511411867226,-25.8408864029058,
74.1620634102641));
#115503=CARTESIAN_POINT('Ctrl Pts',(14.84114150854,-25.8607018705969,74.2338223258621));
#115504=CARTESIAN_POINT('Ctrl Pts',(14.8306258959872,-25.8803326345716,
74.3025768350749));
#115505=CARTESIAN_POINT('Ctrl Pts',(14.8198094672081,-25.899601248361,74.3683365258879));
#115506=CARTESIAN_POINT('Ctrl Pts',(14.8085156384223,-25.9197203125662,
74.4369986235374));
#115507=CARTESIAN_POINT('Ctrl Pts',(14.7968940012334,-25.9394446013637,
74.5023957862849));
#115508=CARTESIAN_POINT('Ctrl Pts',(14.7851682425416,-25.9586045066459,
74.5645445447822));
#115509=CARTESIAN_POINT('Ctrl Pts',(14.7793053631958,-25.968184459287,74.5956189240309));
#115510=CARTESIAN_POINT('Ctrl Pts',(14.7734161154646,-25.9776238048017,
74.6258812797001));
#115511=CARTESIAN_POINT('Ctrl Pts',(14.7675264323988,-25.9869041150831,
74.6553340710032));
#115512=CARTESIAN_POINT('Ctrl Pts',(14.7645815908659,-25.9915442702239,
74.6700604666547));
#115513=CARTESIAN_POINT('Ctrl Pts',(14.7616366208883,-25.9961446665606,
74.6845844672437));
#115514=CARTESIAN_POINT('Ctrl Pts',(14.7586946352575,-26.0007032008082,
74.6989064097336));
#115515=CARTESIAN_POINT('Ctrl Pts',(14.7563545752567,-26.0043290661229,
74.7102981053299));
#115516=CARTESIAN_POINT('Ctrl Pts',(14.7534682637949,-26.008774456286,74.7242134413493));
#115517=CARTESIAN_POINT('Ctrl Pts',(14.750526882187,-26.0132657974865,74.7381970253182));
#115518=CARTESIAN_POINT('Ctrl Pts',(14.7497702806568,-26.0144210898212,
74.7417939747926));
#115519=CARTESIAN_POINT('Ctrl Pts',(14.7490102658137,-26.0155792891444,
74.7453954749945));
#115520=CARTESIAN_POINT('Ctrl Pts',(14.7482557038702,-26.0167269386934,
74.7489598144109));
#115521=CARTESIAN_POINT('Ctrl Pts',(14.726595823022,-26.0496704931656,74.8512750288573));
#115522=CARTESIAN_POINT('Ctrl Pts',(14.7030251667799,-26.0836746568982,
74.9532932583679));
#115523=CARTESIAN_POINT('Ctrl Pts',(14.6775434815947,-26.1186225857099,
75.0549628614383));
#115524=CARTESIAN_POINT('Ctrl Pts',(14.5807327523832,-26.2513977317848,
75.4412288536748));
#115525=CARTESIAN_POINT('Ctrl Pts',(14.4563370759543,-26.3977958659517,
75.822466523226));
#115526=CARTESIAN_POINT('Ctrl Pts',(14.3044197355888,-26.5490345935639,
76.1954372265989));
#115527=CARTESIAN_POINT('Ctrl Pts',(14.2784528993981,-26.5748854362402,
76.2591881396619));
#115528=CARTESIAN_POINT('Ctrl Pts',(14.2516820244083,-26.6008776840374,
76.322697408171));
#115529=CARTESIAN_POINT('Ctrl Pts',(14.2241074907228,-26.6269674540316,
76.3859487164399));
#115530=CARTESIAN_POINT('',(14.2241195978544,-25.6803288454663,69.5918555673368));
#115531=CARTESIAN_POINT('Ctrl Pts',(14.2241026265127,-25.6803288453497,
69.5918629655995));
#115532=CARTESIAN_POINT('Ctrl Pts',(14.2338993117142,-25.6750456877715,
69.61433611693));
#115533=CARTESIAN_POINT('Ctrl Pts',(14.2453110648062,-25.6689449086916,
69.6407711517479));
#115534=CARTESIAN_POINT('Ctrl Pts',(14.2582172700314,-25.6621326199402,
69.671216979588));
#115535=CARTESIAN_POINT('Ctrl Pts',(14.2711080763947,-25.6553284591778,
69.7016264814059));
#115536=CARTESIAN_POINT('Ctrl Pts',(14.2854898165465,-25.6478143058882,
69.7360373571018));
#115537=CARTESIAN_POINT('Ctrl Pts',(14.3012054317066,-25.6397313603784,
69.7745096285445));
#115538=CARTESIAN_POINT('Ctrl Pts',(14.3169210468667,-25.6316484148687,
69.8129818999871));
#115539=CARTESIAN_POINT('Ctrl Pts',(14.3339706033377,-25.6229964426334,
69.8555157476333));
#115540=CARTESIAN_POINT('Ctrl Pts',(14.3521592952607,-25.6139552487866,
69.9021800432174));
#115541=CARTESIAN_POINT('Ctrl Pts',(14.3697195313874,-25.6052264463257,
69.9472319937706));
#115542=CARTESIAN_POINT('Ctrl Pts',(14.3883414175576,-25.5961348293546,
69.9961341361763));
#115543=CARTESIAN_POINT('Ctrl Pts',(14.4078153200047,-25.5868797326659,
70.0489536868223));
#115544=CARTESIAN_POINT('Ctrl Pts',(14.4269162706787,-25.5778018836928,
70.1007616710847));
#115545=CARTESIAN_POINT('Ctrl Pts',(14.4468368816831,-25.5685666230943,
70.1563386573105));
#115546=CARTESIAN_POINT('Ctrl Pts',(14.4673467945466,-25.5594001158797,
70.2157500959955));
#115547=CARTESIAN_POINT('Ctrl Pts',(14.4746780481005,-25.55612355449,70.2369866718843));
#115548=CARTESIAN_POINT('Ctrl Pts',(14.4820842922524,-25.5528561464829,
70.2587131799805));
#115549=CARTESIAN_POINT('Ctrl Pts',(14.4895539796186,-25.5496094889563,
70.280932595363));
#115550=CARTESIAN_POINT('Ctrl Pts',(14.4978326632631,-25.5460112057556,
70.3055584601015));
#115551=CARTESIAN_POINT('Ctrl Pts',(14.5061892901608,-25.5424383921229,
70.330789784142));
#115552=CARTESIAN_POINT('Ctrl Pts',(14.5146073477813,-25.5389078583163,
70.3566305615356));
#115553=CARTESIAN_POINT('Ctrl Pts',(14.5188163765916,-25.5371425914131,
70.3695509502323));
#115554=CARTESIAN_POINT('Ctrl Pts',(14.5230407515599,-25.5353878944688,
70.3826237059942));
#115555=CARTESIAN_POINT('Ctrl Pts',(14.5272783273136,-25.5336459975768,
70.3958493129143));
#115556=CARTESIAN_POINT('Ctrl Pts',(14.5306261334141,-25.532269849189,70.406297920822));
#115557=CARTESIAN_POINT('Ctrl Pts',(14.5330136918787,-25.5312977314843,
70.4138070161427));
#115558=CARTESIAN_POINT('Ctrl Pts',(14.5353086196189,-25.5303666064219,
70.4210470939523));
#115559=CARTESIAN_POINT('Ctrl Pts',(14.5359185584858,-25.5301191348542,
70.4229713396609));
#115560=CARTESIAN_POINT('Ctrl Pts',(14.5365217515845,-25.529874753799,70.4248766451319));
#115561=CARTESIAN_POINT('Ctrl Pts',(14.5371340949548,-25.529627025719,70.4268132660522));
#115562=CARTESIAN_POINT('Ctrl Pts',(14.5469741685572,-25.5256461505121,
70.4579338649191));
#115563=CARTESIAN_POINT('Ctrl Pts',(14.5565890539903,-25.5218518761061,
70.4889666874341));
#115564=CARTESIAN_POINT('Ctrl Pts',(14.5659829572459,-25.5182420787809,
70.5199083042194));
#115565=CARTESIAN_POINT('Ctrl Pts',(14.6088329330693,-25.5017761088953,
70.6610474553376));
#115566=CARTESIAN_POINT('Ctrl Pts',(14.6470859696426,-25.4891475731015,
70.8002848510483));
#115567=CARTESIAN_POINT('Ctrl Pts',(14.6811698955704,-25.4799462604506,
70.9373334188642));
#115568=CARTESIAN_POINT('Ctrl Pts',(14.6927625606021,-25.4768166991542,
70.9839465391702));
#115569=CARTESIAN_POINT('Ctrl Pts',(14.7038728251073,-25.4740836902524,
71.0303068799569));
#115570=CARTESIAN_POINT('Ctrl Pts',(14.7145171831541,-25.471731357348,71.0764044326882));
#115571=CARTESIAN_POINT('Ctrl Pts',(14.7226506902966,-25.4699339059286,
71.1116282360168));
#115572=CARTESIAN_POINT('Ctrl Pts',(14.730419914814,-25.4683758830105,71.1462827098248));
#115573=CARTESIAN_POINT('Ctrl Pts',(14.7380228251446,-25.467013237196,71.181215845594));
#115574=CARTESIAN_POINT('Ctrl Pts',(14.7456257354751,-25.4656505913816,
71.2161489813631));
#115575=CARTESIAN_POINT('Ctrl Pts',(14.7530624440847,-25.4644832094774,
71.2513608443164));
#115576=CARTESIAN_POINT('Ctrl Pts',(14.7604873173191,-25.4635097754476,
71.2877085029335));
#115577=CARTESIAN_POINT('Ctrl Pts',(14.8052502089818,-25.4576411605043,
71.5068403659952));
#115578=CARTESIAN_POINT('Ctrl Pts',(14.8413639787243,-25.4600534562162,
71.7277141970178));
#115579=CARTESIAN_POINT('Ctrl Pts',(14.8687019433517,-25.4708912995428,
71.9497116025528));
#115580=CARTESIAN_POINT('Ctrl Pts',(14.8776406202561,-25.4744349422813,
72.0222979530274));
#115581=CARTESIAN_POINT('Ctrl Pts',(14.885641027309,-25.4788793646732,72.0950044205385));
#115582=CARTESIAN_POINT('Ctrl Pts',(14.8927019369333,-25.4842038600896,
72.1678085493355));
#115583=CARTESIAN_POINT('Ctrl Pts',(14.9070299012433,-25.4950083009269,
72.315542342079));
#115584=CARTESIAN_POINT('Ctrl Pts',(14.917489429708,-25.5094365505709,72.463678333871));
#115585=CARTESIAN_POINT('Ctrl Pts',(14.924069381774,-25.5273157376696,72.6120282867966));
#115586=CARTESIAN_POINT('Ctrl Pts',(14.9273593578071,-25.5362553312189,
72.6862032632594));
#115587=CARTESIAN_POINT('Ctrl Pts',(14.9296794223991,-25.5460576591347,
72.7604317306291));
#115588=CARTESIAN_POINT('Ctrl Pts',(14.9310280814812,-25.5567011269805,
72.8346900293723));
#115589=CARTESIAN_POINT('Ctrl Pts',(14.9317024110222,-25.5620228609035,
72.8718191787439));
#115590=CARTESIAN_POINT('Ctrl Pts',(14.9321338882588,-25.5675548798091,
72.9089557860247));
#115591=CARTESIAN_POINT('Ctrl Pts',(14.9323223207997,-25.5732944842521,
72.946096887067));
#115592=CARTESIAN_POINT('Ctrl Pts',(14.9323694289349,-25.5747293853629,
72.9553821623276));
#115593=CARTESIAN_POINT('Ctrl Pts',(14.9323992627362,-25.5761790818121,
72.9646677473044));
#115594=CARTESIAN_POINT('Ctrl Pts',(14.9324139020858,-25.5772981979159,
72.9717911886955));
#115595=CARTESIAN_POINT('Ctrl Pts',(14.9324212217606,-25.5778577559678,
72.975352909391));
#115596=CARTESIAN_POINT('Ctrl Pts',(14.9324226631454,-25.5780789378129,
72.976752333311));
#115597=CARTESIAN_POINT('Ctrl Pts',(14.9324232811651,-25.5781482284294,
72.9771871753668));
#115598=CARTESIAN_POINT('Ctrl Pts',(14.9324238991848,-25.5782175190459,
72.9776220174227));
#115599=CARTESIAN_POINT('Ctrl Pts',(14.9324245829475,-25.5782981840234,
72.9781259632307));
#115600=CARTESIAN_POINT('Ctrl Pts',(14.9324252956337,-25.578390236186,72.9786990130744));
#115601=CARTESIAN_POINT('Ctrl Pts',(14.9324281463782,-25.5787584448367,
72.9809912124489));
#115602=CARTESIAN_POINT('Ctrl Pts',(14.9324316612965,-25.5793088484383,
72.9843890844908));
#115603=CARTESIAN_POINT('Ctrl Pts',(14.9324318700046,-25.5800517252917,
72.988891520403));
#115604=CARTESIAN_POINT('',(14.2241252549691,-25.68032884552,69.591853101251));
#115605=CARTESIAN_POINT('Origin',(-15.5675364832709,-75.,72.98888938658));
#115606=CARTESIAN_POINT('',(-18.5675364832709,-75.,62.73888938658));
#115607=CARTESIAN_POINT('Origin',(-18.5675364832709,-75.,72.98888938658));
#115608=CARTESIAN_POINT('',(-15.5675364833309,-75.,62.73888938658));
#115609=CARTESIAN_POINT('',(-15.5675364832709,-75.,62.73888938658));
#115610=CARTESIAN_POINT('Origin',(-15.5675364833309,-75.,72.98888938658));
#115611=CARTESIAN_POINT('Origin',(-18.5675364832709,-75.,72.98888938658));
#115612=CARTESIAN_POINT('',(-20.0675364832709,-75.,84.7388893856825));
#115613=CARTESIAN_POINT('',(-20.0675364832709,-75.,61.23888938658));
#115614=CARTESIAN_POINT('Origin',(-20.0675364832709,-75.,72.98888938658));
#115615=CARTESIAN_POINT('',(-18.5675364832709,-75.,61.23888938658));
#115616=CARTESIAN_POINT('',(-18.5675364832709,-75.,61.23888938658));
#115617=CARTESIAN_POINT('Origin',(-18.5675364832709,-75.,72.98888938658));
#115618=CARTESIAN_POINT('Origin',(-20.0675364832709,-75.,72.98888938658));
#115619=CARTESIAN_POINT('Origin',(-20.5675364832709,-75.,72.98888938658));
#115620=CARTESIAN_POINT('',(-20.5675364832709,-75.,84.23888938658));
#115621=CARTESIAN_POINT('',(-20.5675364832709,-75.,84.23888938658));
#115622=CARTESIAN_POINT('Origin',(-20.5675364832709,-75.,72.98888938658));
#115623=CARTESIAN_POINT('Origin',(-20.5675364832709,-75.,72.98888938658));
#115624=CARTESIAN_POINT('',(-20.3675364832709,-75.,65.23888938658));
#115625=CARTESIAN_POINT('',(-20.3675364832709,-75.,80.73888938658));
#115626=CARTESIAN_POINT('Origin',(-20.3675364832709,-75.,72.98888938658));
#115627=CARTESIAN_POINT('',(-18.0675364832709,-75.,80.73888938658));
#115628=CARTESIAN_POINT('',(-20.5675364832709,-75.,80.73888938658));
#115629=CARTESIAN_POINT('',(-18.0675364832709,-75.,65.23888938658));
#115630=CARTESIAN_POINT('Origin',(-18.0675364832709,-75.,72.98888938658));
#115631=CARTESIAN_POINT('Origin',(-18.0675364832709,-75.,72.98888938658));
#115632=CARTESIAN_POINT('Origin',(-20.3675364832709,-75.,72.98888938658));
#115633=CARTESIAN_POINT('Origin',(-18.0675364832709,-75.,72.98888938658));
#115634=CARTESIAN_POINT('',(-17.0930718951698,-78.0310889133651,78.2388893867872));
#115635=CARTESIAN_POINT('',(-17.0930718951698,-71.9689110866348,78.2388893867871));
#115636=CARTESIAN_POINT('Ctrl Pts',(-17.0930718944527,-78.0310889135721,
78.23888938658));
#115637=CARTESIAN_POINT('Ctrl Pts',(-16.2180718918697,-75.,78.23888938658));
#115638=CARTESIAN_POINT('Ctrl Pts',(-17.0930718944527,-71.9689110864278,
78.23888938658));
#115639=CARTESIAN_POINT('',(-17.0930718951697,-81.0621778267302,72.98888938658));
#115640=CARTESIAN_POINT('Ctrl Pts',(-17.0930718945656,-81.0621778268498,
72.9888893859586));
#115641=CARTESIAN_POINT('Ctrl Pts',(-16.2180718917851,-79.5466333698683,
75.61388938658));
#115642=CARTESIAN_POINT('Ctrl Pts',(-17.0930718945656,-78.0310889128867,
78.2388893872014));
#115643=CARTESIAN_POINT('',(-17.0930718951697,-78.0310889133651,67.7388893863729));
#115644=CARTESIAN_POINT('Ctrl Pts',(-17.0930718945656,-78.0310889128867,
67.7388893859586));
#115645=CARTESIAN_POINT('Ctrl Pts',(-16.2180718917851,-79.5466333698682,
70.36388938658));
#115646=CARTESIAN_POINT('Ctrl Pts',(-17.0930718945656,-81.0621778268498,
72.9888893872014));
#115647=CARTESIAN_POINT('',(-16.6241608063082,-75.,67.73888938658));
#115648=CARTESIAN_POINT('Ctrl Pts',(-17.0930718944527,-78.0310889135721,
67.73888938658));
#115649=CARTESIAN_POINT('Ctrl Pts',(-16.6241608063082,-76.4067332603947,
67.73888938658));
#115650=CARTESIAN_POINT('Ctrl Pts',(-16.6241608063082,-75.,67.73888938658));
#115651=CARTESIAN_POINT('',(-18.0675364832709,-75.,65.23888938658));
#115652=CARTESIAN_POINT('',(-17.0930718951697,-71.9689110866349,67.7388893863728));
#115653=CARTESIAN_POINT('Ctrl Pts',(-16.6241608063082,-75.,67.73888938658));
#115654=CARTESIAN_POINT('Ctrl Pts',(-16.6241608063082,-73.5932667396054,
67.73888938658));
#115655=CARTESIAN_POINT('Ctrl Pts',(-17.0930718944527,-71.968911086428,
67.73888938658));
#115656=CARTESIAN_POINT('',(-17.0930718951698,-68.9378221732697,72.98888938658));
#115657=CARTESIAN_POINT('Ctrl Pts',(-17.0930718945656,-68.9378221731502,
72.9888893872015));
#115658=CARTESIAN_POINT('Ctrl Pts',(-16.2180718917851,-70.4533666301317,
70.36388938658));
#115659=CARTESIAN_POINT('Ctrl Pts',(-17.0930718945656,-71.9689110871133,
67.7388893859586));
#115660=CARTESIAN_POINT('Ctrl Pts',(-17.0930718945656,-71.9689110871132,
78.2388893872014));
#115661=CARTESIAN_POINT('Ctrl Pts',(-16.2180718917851,-70.4533666301317,
75.61388938658));
#115662=CARTESIAN_POINT('Ctrl Pts',(-17.0930718945656,-68.9378221731501,
72.9888893859586));
#115663=CARTESIAN_POINT('Origin',(-20.5675364832709,-75.,72.98888938658));
#115664=CARTESIAN_POINT('',(-20.5675364832709,-75.,65.03888938658));
#115665=CARTESIAN_POINT('',(-20.5675364832709,-75.,65.03888938658));
#115666=CARTESIAN_POINT('Origin',(-20.5675364832709,-75.,72.98888938658));
#115667=CARTESIAN_POINT('Origin',(-15.0675364833309,75.,72.98888938658));
#115668=CARTESIAN_POINT('',(-15.0675364833309,84.4840963577871,72.4394203008163));
#115669=CARTESIAN_POINT('',(-15.0675364833309,65.5,72.98888938658));
#115670=CARTESIAN_POINT('Origin',(-15.0675364833309,75.,72.98888938658));
#115671=CARTESIAN_POINT('Origin',(-15.0675364833309,75.,72.98888938658));
#115672=CARTESIAN_POINT('',(-15.5675364832709,84.9832593239864,72.4105008752498));
#115673=CARTESIAN_POINT('Origin',(-15.0675364833309,84.9832593239864,72.4105008752498));
#115674=CARTESIAN_POINT('Origin',(-15.5675364832709,75.,72.98888938658));
#115675=CARTESIAN_POINT('Origin',(-15.9175364833309,75.,72.98888938658));
#115676=CARTESIAN_POINT('',(-13.5675364833309,65.5,72.98888938658));
#115677=CARTESIAN_POINT('Origin',(-13.5675364833309,75.,72.98888938658));
#115678=CARTESIAN_POINT('',(-15.9175364833309,65.5,72.98888938658));
#115679=CARTESIAN_POINT('Origin',(-13.2677182305225,75.,72.98888938658));
#115680=CARTESIAN_POINT('',(-13.22669566117,66.3412155148882,72.9888893865797));
#115681=CARTESIAN_POINT('Ctrl Pts',(-13.22669566117,66.3412155148882,72.9888893865797));
#115682=CARTESIAN_POINT('Ctrl Pts',(-13.2104605534334,66.357449920082,73.9348371888089));
#115683=CARTESIAN_POINT('Ctrl Pts',(-13.1935918113208,66.5285128660429,
74.8664087689662));
#115684=CARTESIAN_POINT('Ctrl Pts',(-13.1607289900761,67.1584349638421,
76.6215069908932));
#115685=CARTESIAN_POINT('Ctrl Pts',(-13.1451833963657,67.6075512811205,
77.4360748130446));
#115686=CARTESIAN_POINT('Ctrl Pts',(-13.1183032532819,68.5324033671701,
78.610611579631));
#115687=CARTESIAN_POINT('Ctrl Pts',(-13.1080428039918,68.928953991022,79.0221823155135));
#115688=CARTESIAN_POINT('Ctrl Pts',(-13.0883350900634,69.7818215132367,
79.7468724686923));
#115689=CARTESIAN_POINT('Ctrl Pts',(-13.0788920662947,70.2343312777093,
80.0618859789133));
#115690=CARTESIAN_POINT('Ctrl Pts',(-13.0522833578858,71.5410395253665,
80.7939570097886));
#115691=CARTESIAN_POINT('Ctrl Pts',(-13.03483318715,72.4423882065013,81.1156940890532));
#115692=CARTESIAN_POINT('Ctrl Pts',(-13.0100115445559,73.8291489133028,
81.3621080239062));
#115693=CARTESIAN_POINT('Ctrl Pts',(-13.0019625279167,74.2894034272058,
81.4056373417021));
#115694=CARTESIAN_POINT('Ctrl Pts',(-12.9849785040465,75.227891744384,81.4163718781257));
#115695=CARTESIAN_POINT('Ctrl Pts',(-12.9761722647469,75.7045067720495,
81.3811420042793));
#115696=CARTESIAN_POINT('Ctrl Pts',(-12.9675119086199,76.1752581060379,
81.3058749742284));
#115697=CARTESIAN_POINT('',(-13.5675364833309,80.654580018939,66.0024639308014));
#115698=CARTESIAN_POINT('Ctrl Pts',(-13.5590247159961,80.6563382683147,
65.9999193993703));
#115699=CARTESIAN_POINT('Ctrl Pts',(-13.5400068999588,79.7853367243258,
65.319462092606));
#115700=CARTESIAN_POINT('Ctrl Pts',(-13.5251921994605,78.7953578411616,
64.8005562641523));
#115701=CARTESIAN_POINT('Ctrl Pts',(-13.492890683205,76.5983471916873,64.1275891133102));
#115702=CARTESIAN_POINT('Ctrl Pts',(-13.4743351779794,75.5313749841502,
64.0511778965532));
#115703=CARTESIAN_POINT('Ctrl Pts',(-13.4484851075557,74.0420263880311,
64.1414492774393));
#115704=CARTESIAN_POINT('Ctrl Pts',(-13.4386640566306,73.4721998577258,
64.2318124979119));
#115705=CARTESIAN_POINT('Ctrl Pts',(-13.4186751669976,72.3508272271238,
64.5237563092107));
#115706=CARTESIAN_POINT('Ctrl Pts',(-13.4083630346961,71.8020941955304,
64.7265441047799));
#115707=CARTESIAN_POINT('Ctrl Pts',(-13.378889434965,70.2710191495859,65.4707072119258));
#115708=CARTESIAN_POINT('Ctrl Pts',(-13.3606766606445,69.3623365579809,
66.1482847756555));
#115709=CARTESIAN_POINT('Ctrl Pts',(-13.3311112102964,68.2320374767698,
67.3943249844395));
#115710=CARTESIAN_POINT('Ctrl Pts',(-13.3213178770165,67.897308892087,67.8425591305012));
#115711=CARTESIAN_POINT('Ctrl Pts',(-13.2977592138052,67.184560519637,69.0149548811999));
#115712=CARTESIAN_POINT('Ctrl Pts',(-13.2841131442571,66.86000923957,69.7671246312326));
#115713=CARTESIAN_POINT('Ctrl Pts',(-13.2551217230953,66.4298369296489,
71.3475877782227));
#115714=CARTESIAN_POINT('Ctrl Pts',(-13.2407852022714,66.3271265834845,
72.1679542467925));
#115715=CARTESIAN_POINT('Ctrl Pts',(-13.22669566117,66.3412155148882,72.9888893865797));
#115716=CARTESIAN_POINT('',(-13.5677219667119,82.8053136859618,77.4672764703467));
#115717=CARTESIAN_POINT('Origin',(-13.5675364833309,75.,72.98888938658));
#115718=CARTESIAN_POINT('',(-13.2736619003203,83.7052176583754,72.9888947630299));
#115719=CARTESIAN_POINT('Ctrl Pts',(-13.2736619003203,83.7052176583754,
72.9888947630299));
#115720=CARTESIAN_POINT('Ctrl Pts',(-13.3229312239107,83.753373874782,73.7448830644767));
#115721=CARTESIAN_POINT('Ctrl Pts',(-13.371980109432,83.7042558727909,74.5139171860313));
#115722=CARTESIAN_POINT('Ctrl Pts',(-13.470077354358,83.4046953760079,76.0245633284111));
#115723=CARTESIAN_POINT('Ctrl Pts',(-13.5191257137627,83.1524546020321,
76.7655416665762));
#115724=CARTESIAN_POINT('Ctrl Pts',(-13.5676947124535,82.8052754641751,
77.4672501945017));
#115725=CARTESIAN_POINT('Ctrl Pts',(-12.9679003706342,82.2015397612608,
68.6647904662762));
#115726=CARTESIAN_POINT('Ctrl Pts',(-13.0193150349774,82.6340458634664,
69.2881849289807));
#115727=CARTESIAN_POINT('Ctrl Pts',(-13.0702284178419,82.9868581475013,
69.9759204830991));
#115728=CARTESIAN_POINT('Ctrl Pts',(-13.1720553132675,83.4982142737106,
71.4337103090243));
#115729=CARTESIAN_POINT('Ctrl Pts',(-13.2229688258284,83.6545977325296,
72.2041789688228));
#115730=CARTESIAN_POINT('Ctrl Pts',(-13.2736619003203,83.7052176583754,
72.9888947630299));
#115731=CARTESIAN_POINT('Origin',(-15.9175364833309,75.,72.98888938658));
#115732=CARTESIAN_POINT('',(-8.59968985140647,83.3999999997258,72.98882151283));
#115733=CARTESIAN_POINT('Ctrl Pts',(-9.34771011126149,66.6,72.98888938658));
#115734=CARTESIAN_POINT('Ctrl Pts',(-9.34482801228272,66.6,73.0851880451777));
#115735=CARTESIAN_POINT('Ctrl Pts',(-9.34195702478471,66.6016559635923,
73.1815258398187));
#115736=CARTESIAN_POINT('Ctrl Pts',(-9.30786458115699,66.6413112039165,
74.3335679385027));
#115737=CARTESIAN_POINT('Ctrl Pts',(-9.28193074981338,66.8764288734639,
75.3728643345099));
#115738=CARTESIAN_POINT('Ctrl Pts',(-9.22587128847865,67.679423604765,77.2176616875703));
#115739=CARTESIAN_POINT('Ctrl Pts',(-9.19621563570561,68.2075392243034,
78.0223270669282));
#115740=CARTESIAN_POINT('Ctrl Pts',(-9.13661313794164,69.5837355649427,
79.4966046033503));
#115741=CARTESIAN_POINT('Ctrl Pts',(-9.11063836871128,70.4483040656611,
80.1280967594261));
#115742=CARTESIAN_POINT('Ctrl Pts',(-9.06544015277399,71.9032877835412,
80.816474494744));
#115743=CARTESIAN_POINT('Ctrl Pts',(-9.0492530382319,72.4207379848354,81.0018836652407));
#115744=CARTESIAN_POINT('Ctrl Pts',(-9.01641236916751,73.4770724783752,
81.2673682415297));
#115745=CARTESIAN_POINT('Ctrl Pts',(-8.99989317304966,74.0131508282444,
81.3482387615376));
#115746=CARTESIAN_POINT('Ctrl Pts',(-8.96482585598902,75.2614006272828,
81.414712312213));
#115747=CARTESIAN_POINT('Ctrl Pts',(-8.94677685625615,75.9714458658481,
81.3626105564356));
#115748=CARTESIAN_POINT('Ctrl Pts',(-8.89744367046157,77.738984272286,81.0048289169403));
#115749=CARTESIAN_POINT('Ctrl Pts',(-8.8636309510077,78.7585842810629,80.5803202299836));
#115750=CARTESIAN_POINT('Ctrl Pts',(-8.80454412642285,80.4315045504105,
79.4620643314559));
#115751=CARTESIAN_POINT('Ctrl Pts',(-8.78167961117171,81.1060256594941,
78.8300902543004));
#115752=CARTESIAN_POINT('Ctrl Pts',(-8.73113802125434,82.2232693318652,
77.3736308124975));
#115753=CARTESIAN_POINT('Ctrl Pts',(-8.70335941293635,82.6586024229665,
76.5591999956128));
#115754=CARTESIAN_POINT('Ctrl Pts',(-8.64831230121883,83.2492253893665,
74.8205244935375));
#115755=CARTESIAN_POINT('Ctrl Pts',(-8.62456332243574,83.400007425365,73.9078125751677));
#115756=CARTESIAN_POINT('Ctrl Pts',(-8.59968985140647,83.3999999997258,
72.9888215128297));
#115757=CARTESIAN_POINT('',(-8.57006447465355,83.3346137605936,71.9543844308784));
#115758=CARTESIAN_POINT('Ctrl Pts',(-8.57089042794284,83.336032673353,71.9542110458426));
#115759=CARTESIAN_POINT('Ctrl Pts',(-8.57495963766164,83.3535848314682,
72.0956224949622));
#115760=CARTESIAN_POINT('Ctrl Pts',(-8.57897898148748,83.3675359712116,
72.2374588562827));
#115761=CARTESIAN_POINT('Ctrl Pts',(-8.58861924885021,83.3926174828801,
72.5823258349277));
#115762=CARTESIAN_POINT('Ctrl Pts',(-8.5941877887613,83.3999983571592,72.7855388109754));
#115763=CARTESIAN_POINT('Ctrl Pts',(-8.59968985140647,83.3999999997258,
72.98882151283));
#115764=CARTESIAN_POINT('',(-8.56753648333115,72.6784966214631,81.0617217311459));
#115765=CARTESIAN_POINT('Origin',(-8.56753648333091,75.,72.98888938658));
#115766=CARTESIAN_POINT('Ctrl Pts',(-8.56753648333163,72.6784966214636,
81.0617217311443));
#115767=CARTESIAN_POINT('Ctrl Pts',(-8.59656065877325,71.6765852906451,
80.7736022161819));
#115768=CARTESIAN_POINT('Ctrl Pts',(-8.62742781849965,70.7370700765324,
80.3014901279046));
#115769=CARTESIAN_POINT('Ctrl Pts',(-8.66662311789324,69.6339116236681,
79.4606631122048));
#115770=CARTESIAN_POINT('Ctrl Pts',(-8.67610817330382,69.3729450473901,
79.2350896258631));
#115771=CARTESIAN_POINT('Ctrl Pts',(-8.71654432300731,68.3297664008052,
78.2148070440606));
#115772=CARTESIAN_POINT('Ctrl Pts',(-8.74937209339453,67.6960196716305,
77.2846877425061));
#115773=CARTESIAN_POINT('Ctrl Pts',(-8.79628814797203,67.0522382181187,
75.7609558810951));
#115774=CARTESIAN_POINT('Ctrl Pts',(-8.81096863053585,66.8905908306959,
75.2447202116387));
#115775=CARTESIAN_POINT('Ctrl Pts',(-8.84234325928866,66.6600179277575,
74.1476246372836));
#115776=CARTESIAN_POINT('Ctrl Pts',(-8.85902939320876,66.6,73.5686245783471));
#115777=CARTESIAN_POINT('Ctrl Pts',(-8.87591635085981,66.6,72.98888938658));
#115778=CARTESIAN_POINT('Origin',(-15.5675364833309,75.,72.98888938658));
#115779=CARTESIAN_POINT('',(-8.69331175948402,75.0000000064252,84.9888491626591));
#115780=CARTESIAN_POINT('',(-10.0948603023692,68.5588728119111,83.113703237526));
#115781=CARTESIAN_POINT('Ctrl Pts',(-8.69331176731091,75.00000000541,84.98885921934));
#115782=CARTESIAN_POINT('Ctrl Pts',(-8.69350218314475,74.6600650057603,
84.98888938658));
#115783=CARTESIAN_POINT('Ctrl Pts',(-8.70999108976109,74.3134431213811,
84.9744403493725));
#115784=CARTESIAN_POINT('Ctrl Pts',(-8.75917218585936,73.7855419536267,
84.9285832566471));
#115785=CARTESIAN_POINT('Ctrl Pts',(-8.77964050725442,73.6082514723118,
84.909267817465));
#115786=CARTESIAN_POINT('Ctrl Pts',(-8.81645492339044,73.3406310239618,
84.8739468570477));
#115787=CARTESIAN_POINT('Ctrl Pts',(-8.83639011496931,73.2064000704339,
84.8546995602693));
#115788=CARTESIAN_POINT('Ctrl Pts',(-8.862321809622,73.0491315493374,84.829402717515));
#115789=CARTESIAN_POINT('Ctrl Pts',(-8.87693003117094,72.9647120676162,
84.815081151703));
#115790=CARTESIAN_POINT('Ctrl Pts',(-8.8839421782897,72.9252717938844,84.8081870735222));
#115791=CARTESIAN_POINT('Ctrl Pts',(-8.88799686898513,72.9027238430882,
84.8041957936489));
#115792=CARTESIAN_POINT('Ctrl Pts',(-8.88930163845279,72.8955012600355,
84.8029108023554));
#115793=CARTESIAN_POINT('Ctrl Pts',(-8.93704499978251,72.6319881317605,
84.7558764051637));
#115794=CARTESIAN_POINT('Ctrl Pts',(-8.99631542872801,72.3531384263844,
84.6973357387733));
#115795=CARTESIAN_POINT('Ctrl Pts',(-9.10361344344678,71.9082647950302,
84.5847753581377));
#115796=CARTESIAN_POINT('Ctrl Pts',(-9.14244484356978,71.7555519361259,
84.5431226993059));
#115797=CARTESIAN_POINT('Ctrl Pts',(-9.20529003657942,71.5202786694363,
84.4735847300639));
#115798=CARTESIAN_POINT('Ctrl Pts',(-9.23786215629052,71.4010923796508,
84.4370504540915));
#115799=CARTESIAN_POINT('Ctrl Pts',(-9.27787462823113,71.2594384594255,
84.3911445732516));
#115800=CARTESIAN_POINT('Ctrl Pts',(-9.2983837806042,71.1879754503105,84.3673465065967));
#115801=CARTESIAN_POINT('Ctrl Pts',(-9.30950553626907,71.149523341116,84.3543678833721));
#115802=CARTESIAN_POINT('Ctrl Pts',(-9.31473235990037,71.1315334729288,
84.3482482258899));
#115803=CARTESIAN_POINT('Ctrl Pts',(-9.31772809691117,71.1212424447593,
84.3447357758996));
#115804=CARTESIAN_POINT('Ctrl Pts',(-9.31880084972148,71.1175603615012,
84.3434772194659));
#115805=CARTESIAN_POINT('Ctrl Pts',(-9.34657930546541,71.0222570215131,
84.3108766922396));
#115806=CARTESIAN_POINT('Ctrl Pts',(-9.37891704962667,70.913135968742,84.2722861271594));
#115807=CARTESIAN_POINT('Ctrl Pts',(-9.43490363978099,70.7273239494605,
84.2026583458093));
#115808=CARTESIAN_POINT('Ctrl Pts',(-9.45481249881782,70.6617014838166,
84.1774864582193));
#115809=CARTESIAN_POINT('Ctrl Pts',(-9.48654578085119,70.55787279937,84.1364851159369));
#115810=CARTESIAN_POINT('Ctrl Pts',(-9.49743520710866,70.5223643250653,
84.1222770859608));
#115811=CARTESIAN_POINT('Ctrl Pts',(-9.51983739078298,70.449574862264,84.0927253889727));
#115812=CARTESIAN_POINT('Ctrl Pts',(-9.53095785234192,70.4135596763115,
84.0779105446965));
#115813=CARTESIAN_POINT('Ctrl Pts',(-9.59204144661402,70.2164634050565,
83.9955682249674));
#115814=CARTESIAN_POINT('Ctrl Pts',(-9.63385426088831,70.0825860012239,
83.9357611550359));
#115815=CARTESIAN_POINT('Ctrl Pts',(-9.68599239058464,69.9159933359892,
83.8588763565762));
#115816=CARTESIAN_POINT('Ctrl Pts',(-9.70160825186424,69.8661689165978,
83.8353718207634));
#115817=CARTESIAN_POINT('Ctrl Pts',(-9.72238677085485,69.7998390819442,
83.8036444519207));
#115818=CARTESIAN_POINT('Ctrl Pts',(-9.73211471211796,69.7687762601497,
83.7886618832566));
#115819=CARTESIAN_POINT('Ctrl Pts',(-9.74230667001859,69.7361860747107,
83.7727864150422));
#115820=CARTESIAN_POINT('Ctrl Pts',(-9.74711332224232,69.7208001835745,
83.7652565559044));
#115821=CARTESIAN_POINT('Ctrl Pts',(-9.74911131746822,69.7144007217004,
83.7621175843978));
#115822=CARTESIAN_POINT('Ctrl Pts',(-9.75042953682232,69.7101775976573,
83.7600445931811));
#115823=CARTESIAN_POINT('Ctrl Pts',(-9.7506298848693,69.7095359546722,83.7597299081517));
#115824=CARTESIAN_POINT('Ctrl Pts',(-9.89216934436306,69.2558786469672,
83.536716801684));
#115825=CARTESIAN_POINT('Ctrl Pts',(-10.0065470818248,68.8761013310119,
83.3155165038809));
#115826=CARTESIAN_POINT('Ctrl Pts',(-10.0948603023669,68.55887270828,83.11370340042));
#115827=CARTESIAN_POINT('',(-11.4810890049562,63.0000050909298,72.9889042778823));
#115828=CARTESIAN_POINT('Ctrl Pts',(-10.0948603023724,68.558873019173,83.1137029117378));
#115829=CARTESIAN_POINT('Ctrl Pts',(-10.133102456483,68.4213962033965,83.026242433531));
#115830=CARTESIAN_POINT('Ctrl Pts',(-10.1701648695647,68.2886100604876,
82.9378350766575));
#115831=CARTESIAN_POINT('Ctrl Pts',(-10.2059877970713,68.1603864864389,
82.8488901634555));
#115832=CARTESIAN_POINT('Ctrl Pts',(-10.2427052753644,68.0289609825926,
82.7577241659478));
#115833=CARTESIAN_POINT('Ctrl Pts',(-10.2781207464655,67.9023287183454,
82.6659935513413));
#115834=CARTESIAN_POINT('Ctrl Pts',(-10.3122145517979,67.7803371412517,
82.5741097836734));
#115835=CARTESIAN_POINT('Ctrl Pts',(-10.3353371804666,67.6976017026478,
82.5117936467752));
#115836=CARTESIAN_POINT('Ctrl Pts',(-10.3578528237975,67.6170005007825,
82.4494064462423));
#115837=CARTESIAN_POINT('Ctrl Pts',(-10.3797659715751,67.5384825179955,
82.3870688292528));
#115838=CARTESIAN_POINT('Ctrl Pts',(-10.4068308106687,67.441505278958,82.3100758937589));
#115839=CARTESIAN_POINT('Ctrl Pts',(-10.4329770164788,67.347706085323,82.2331590847956));
#115840=CARTESIAN_POINT('Ctrl Pts',(-10.4582672655742,67.2569866678418,
82.1565373005544));
#115841=CARTESIAN_POINT('Ctrl Pts',(-10.4929960292256,67.132410069311,82.0513196799045));
#115842=CARTESIAN_POINT('Ctrl Pts',(-10.5260204794163,67.0136339528322,
81.9466545403682));
#115843=CARTESIAN_POINT('Ctrl Pts',(-10.5573359267471,66.9003753871923,
81.8430489324138));
#115844=CARTESIAN_POINT('Ctrl Pts',(-10.5735475602532,66.8417427788768,
81.7894135451373));
#115845=CARTESIAN_POINT('Ctrl Pts',(-10.5893015019345,66.7845887376899,
81.7360612971428));
#115846=CARTESIAN_POINT('Ctrl Pts',(-10.6045989629336,66.7288733548622,
81.6830574812477));
#115847=CARTESIAN_POINT('Ctrl Pts',(-10.6270224795161,66.6472039320208,
81.605362761534));
#115848=CARTESIAN_POINT('Ctrl Pts',(-10.6484634459094,66.5686253077469,
81.5284170018002));
#115849=CARTESIAN_POINT('Ctrl Pts',(-10.6689218629804,66.4930090465584,
81.4524110711747));
#115850=CARTESIAN_POINT('Ctrl Pts',(-10.679151071516,66.4552009159641,81.4144081058619));
#115851=CARTESIAN_POINT('Ctrl Pts',(-10.6891346427481,66.4181333499334,
81.3766398443326));
#115852=CARTESIAN_POINT('Ctrl Pts',(-10.6988725767297,66.381790184475,81.3391286570921));
#115853=CARTESIAN_POINT('Ctrl Pts',(-10.7024765937321,66.3683395504414,
81.325245737281));
#115854=CARTESIAN_POINT('Ctrl Pts',(-10.706046974037,66.3549881473234,81.3113980276785));
#115855=CARTESIAN_POINT('Ctrl Pts',(-10.709583694381,66.3417351446778,81.297586618752));
#115856=CARTESIAN_POINT('Ctrl Pts',(-10.7108250243624,66.3370835613104,
81.2927390440732));
#115857=CARTESIAN_POINT('Ctrl Pts',(-10.7120622078409,66.3324440998453,
81.287895941108));
#115858=CARTESIAN_POINT('Ctrl Pts',(-10.7132952497367,66.3278167251015,
81.2830573588835));
#115859=CARTESIAN_POINT('Ctrl Pts',(-10.715668323907,66.3189110232607,81.2737451736792));
#115860=CARTESIAN_POINT('Ctrl Pts',(-10.7180260457432,66.3100500875175,
81.2644497305875));
#115861=CARTESIAN_POINT('Ctrl Pts',(-10.7203684152401,66.3012336595681,
81.2551713679032));
#115862=CARTESIAN_POINT('Ctrl Pts',(-10.7221251923627,66.2946213386061,
81.2482125958899));
#115863=CARTESIAN_POINT('Ctrl Pts',(-10.7238733337944,66.2880340533221,
81.2412634315616));
#115864=CARTESIAN_POINT('Ctrl Pts',(-10.7256128395322,66.2814716949002,
81.2343240161859));
#115865=CARTESIAN_POINT('Ctrl Pts',(-10.7261926747782,66.2792842420929,
81.2320108777274));
#115866=CARTESIAN_POINT('Ctrl Pts',(-10.7265389790354,66.2779776304599,
81.2306288274579));
#115867=CARTESIAN_POINT('Ctrl Pts',(-10.7273494667053,66.27491764138,81.2273878556018));
#115868=CARTESIAN_POINT('Ctrl Pts',(-10.7793655551984,66.0785313560826,
81.0193863212973));
#115869=CARTESIAN_POINT('Ctrl Pts',(-10.8286358129281,65.8881034723919,
80.8027848089594));
#115870=CARTESIAN_POINT('Ctrl Pts',(-10.8751613041746,65.7044664115946,
80.5778594555792));
#115871=CARTESIAN_POINT('Ctrl Pts',(-10.9198306168304,65.5281557254704,
80.3619077124559));
#115872=CARTESIAN_POINT('Ctrl Pts',(-10.9619698078079,65.3581048515807,
80.1382831909005));
#115873=CARTESIAN_POINT('Ctrl Pts',(-11.0015776921892,65.1950899867055,
79.9072521474355));
#115874=CARTESIAN_POINT('Ctrl Pts',(-11.0029937456614,65.1892619105779,
79.8989923699595));
#115875=CARTESIAN_POINT('Ctrl Pts',(-11.0044065633973,65.1834428321696,
79.890723127841));
#115876=CARTESIAN_POINT('Ctrl Pts',(-11.0058161517136,65.1776327838717,
79.8824444393747));
#115877=CARTESIAN_POINT('Ctrl Pts',(-11.0435518881779,65.0220934332085,
79.6608177398417));
#115878=CARTESIAN_POINT('Ctrl Pts',(-11.0789695059325,64.873026151247,79.4324241836466));
#115879=CARTESIAN_POINT('Ctrl Pts',(-11.1120688318277,64.7310579934169,
79.1976100654547));
#115880=CARTESIAN_POINT('Ctrl Pts',(-11.1148890648589,64.7189615752194,
79.1776026932682));
#115881=CARTESIAN_POINT('Ctrl Pts',(-11.117692469965,64.7069167213773,79.1575487267407));
#115882=CARTESIAN_POINT('Ctrl Pts',(-11.1204790485698,64.6949238339657,
79.1374483905087));
#115883=CARTESIAN_POINT('Ctrl Pts',(-11.1382245102557,64.6185508496559,
79.0094456326251));
#115884=CARTESIAN_POINT('Ctrl Pts',(-11.1552874613776,64.5442849053233,
78.8795620147912));
#115885=CARTESIAN_POINT('Ctrl Pts',(-11.1716678992142,64.4722319657888,
78.7478570972825));
#115886=CARTESIAN_POINT('Ctrl Pts',(-11.1798581181324,64.4362054960215,
78.6820046385282));
#115887=CARTESIAN_POINT('Ctrl Pts',(-11.1878777087469,64.4007323054803,
78.6156968418008));
#115888=CARTESIAN_POINT('Ctrl Pts',(-11.1957266710059,64.3658260660908,
78.5489415654864));
#115889=CARTESIAN_POINT('Ctrl Pts',(-11.1996511521354,64.3483729463961,
78.5155639273292));
#115890=CARTESIAN_POINT('Ctrl Pts',(-11.2035329761818,64.3310615664533,
78.4820744193169));
#115891=CARTESIAN_POINT('Ctrl Pts',(-11.2073721431682,64.3138936541916,
78.4484740371538));
#115892=CARTESIAN_POINT('Ctrl Pts',(-11.2092917266615,64.3053096980607,
78.4316738460722));
#115893=CARTESIAN_POINT('Ctrl Pts',(-11.21120064589,64.2967616089859,78.4148459364674));
#115894=CARTESIAN_POINT('Ctrl Pts',(-11.2130989008581,64.2882496045795,
78.3979904344908));
#115895=CARTESIAN_POINT('Ctrl Pts',(-11.2145225920841,64.2818656012747,
78.3853488080083));
#115896=CARTESIAN_POINT('Ctrl Pts',(-11.2159402846636,64.2755018956071,
78.3726916608183));
#115897=CARTESIAN_POINT('Ctrl Pts',(-11.2173519785987,64.2691585797592,
78.3600190465254));
#115898=CARTESIAN_POINT('Ctrl Pts',(-11.2178225432437,64.2670441411433,
78.3557948417611));
#115899=CARTESIAN_POINT('Ctrl Pts',(-11.2184210608201,64.2643536295815,
78.3504100947542));
#115900=CARTESIAN_POINT('Ctrl Pts',(-11.2187616729857,64.2628220639561,
78.3473412785494));
#115901=CARTESIAN_POINT('Ctrl Pts',(-11.2191016706038,64.2612932616486,
78.3442779992375));
#115902=CARTESIAN_POINT('Ctrl Pts',(-11.2194413371642,64.2597656118155,
78.3412137409868));
#115903=CARTESIAN_POINT('Ctrl Pts',(-11.2197806726984,64.2582391159477,
78.3381485044332));
#115904=CARTESIAN_POINT('Ctrl Pts',(-11.2452797298039,64.143531985737,78.1078141184037));
#115905=CARTESIAN_POINT('Ctrl Pts',(-11.2689091762991,64.0353380185579,
77.8719524167333));
#115906=CARTESIAN_POINT('Ctrl Pts',(-11.2906711856469,63.9342181600986,
77.6308953725145));
#115907=CARTESIAN_POINT('Ctrl Pts',(-11.3121098637698,63.8346007000241,
77.3934198573781));
#115908=CARTESIAN_POINT('Ctrl Pts',(-11.331736163075,63.7418486954108,77.1509021497749));
#115909=CARTESIAN_POINT('Ctrl Pts',(-11.349557324713,63.6565317893308,76.9036976654529));
#115910=CARTESIAN_POINT('Ctrl Pts',(-11.3522702568957,63.6435439165455,
76.8660654945054));
#115911=CARTESIAN_POINT('Ctrl Pts',(-11.3549413665753,63.630728410555,76.82832478512));
#115912=CARTESIAN_POINT('Ctrl Pts',(-11.357570690475,63.6180873502402,76.7904768718687));
#115913=CARTESIAN_POINT('Ctrl Pts',(-11.3745287988962,63.5365574666819,
76.5463726683083));
#115914=CARTESIAN_POINT('Ctrl Pts',(-11.3897484533509,63.4622819653971,
76.2978054605891));
#115915=CARTESIAN_POINT('Ctrl Pts',(-11.4032166767484,63.3957559838242,
76.0452199248016));
#115916=CARTESIAN_POINT('Ctrl Pts',(-11.4073561755882,63.3753090239386,
75.9675870031096));
#115917=CARTESIAN_POINT('Ctrl Pts',(-11.4113302485379,63.3555943162169,
75.8895748038605));
#115918=CARTESIAN_POINT('Ctrl Pts',(-11.4151385858384,63.3366267390366,
75.8111970970855));
#115919=CARTESIAN_POINT('Ctrl Pts',(-11.4225524542904,63.2997016688621,
75.6586155472498));
#115920=CARTESIAN_POINT('Ctrl Pts',(-11.4293373885995,63.2656083264762,
75.5046503952037));
#115921=CARTESIAN_POINT('Ctrl Pts',(-11.4354993489759,63.2344585032999,
75.34940560247));
#115922=CARTESIAN_POINT('Ctrl Pts',(-11.4459029018496,63.1818666635891,
75.0872978784816));
#115923=CARTESIAN_POINT('Ctrl Pts',(-11.4545307022797,63.1376642995191,
74.8215401834039));
#115924=CARTESIAN_POINT('Ctrl Pts',(-11.4613769255451,63.1023184811442,
74.5526099866829));
#115925=CARTESIAN_POINT('Ctrl Pts',(-11.4656979782655,63.0800096637533,
74.3828723790852));
#115926=CARTESIAN_POINT('Ctrl Pts',(-11.4693093299393,63.0612294271659,
74.2118718404528));
#115927=CARTESIAN_POINT('Ctrl Pts',(-11.4722096451391,63.046100307838,74.0397378739752));
#115928=CARTESIAN_POINT('Ctrl Pts',(-11.4764452699417,63.0240057185764,
73.7883531631491));
#115929=CARTESIAN_POINT('Ctrl Pts',(-11.4791643413329,63.0096976470856,
73.5345483639279));
#115930=CARTESIAN_POINT('Ctrl Pts',(-11.4803701594022,63.0035133775259,
73.2789208597845));
#115931=CARTESIAN_POINT('Ctrl Pts',(-11.4808250032522,63.0011806234832,
73.1824961991291));
#115932=CARTESIAN_POINT('Ctrl Pts',(-11.4810645445765,63.0000039177617,
73.0858126969849));
#115933=CARTESIAN_POINT('Ctrl Pts',(-11.4810890049761,63.000001907456,72.9889042779483));
#115934=CARTESIAN_POINT('',(-10.0948866959807,68.5588359045711,62.8641001495972));
#115935=CARTESIAN_POINT('Ctrl Pts',(-11.4810890049462,63.0000066826667,
72.9889042778822));
#115936=CARTESIAN_POINT('Ctrl Pts',(-11.4810244535258,63.0000209039102,
72.7386008713444));
#115937=CARTESIAN_POINT('Ctrl Pts',(-11.4795275015916,63.0078785296247,
72.4899373152444));
#115938=CARTESIAN_POINT('Ctrl Pts',(-11.47660614196,63.023222893841,72.2434339617198));
#115939=CARTESIAN_POINT('Ctrl Pts',(-11.4736219335098,63.0388973698158,
71.9916274457857));
#115940=CARTESIAN_POINT('Ctrl Pts',(-11.4691513830198,63.0623841707853,
71.7420749690625));
#115941=CARTESIAN_POINT('Ctrl Pts',(-11.4632023050969,63.0933255526803,
71.4952817751537));
#115942=CARTESIAN_POINT('Ctrl Pts',(-11.4617464824254,63.1008973420957,
71.4348880248103));
#115943=CARTESIAN_POINT('Ctrl Pts',(-11.4602021144584,63.1089156523144,
71.3746592912387));
#115944=CARTESIAN_POINT('Ctrl Pts',(-11.4585693081243,63.1173754402577,
71.3146025538948));
#115945=CARTESIAN_POINT('Ctrl Pts',(-11.4515256738386,63.1538694513121,
71.0555285379512));
#115946=CARTESIAN_POINT('Ctrl Pts',(-11.4428362393565,63.1985761183067,
70.7996584347455));
#115947=CARTESIAN_POINT('Ctrl Pts',(-11.4324898914039,63.2510013435756,
70.5473945000403));
#115948=CARTESIAN_POINT('Ctrl Pts',(-11.4234647054344,63.2967322052971,
70.3273430447311));
#115949=CARTESIAN_POINT('Ctrl Pts',(-11.4131787609363,63.3483368706343,
70.1100348172557));
#115950=CARTESIAN_POINT('Ctrl Pts',(-11.4016248773891,63.4055085587195,
69.8957124157511));
#115951=CARTESIAN_POINT('Ctrl Pts',(-11.3908685226147,63.4587338623659,
69.6961840253826));
#115952=CARTESIAN_POINT('Ctrl Pts',(-11.3790120736584,63.5167729773594,
69.4992875261014));
#115953=CARTESIAN_POINT('Ctrl Pts',(-11.3660704530696,63.579377814658,69.3052223934151));
#115954=CARTESIAN_POINT('Ctrl Pts',(-11.3498974798454,63.6576142573346,
69.0627017467036));
#115955=CARTESIAN_POINT('Ctrl Pts',(-11.3320293496765,63.7429795757764,
68.8246039756175));
#115956=CARTESIAN_POINT('Ctrl Pts',(-11.3124495579103,63.8348996525675,
68.5912730209228));
#115957=CARTESIAN_POINT('Ctrl Pts',(-11.3093161883228,63.8496096952754,
68.5539328833982));
#115958=CARTESIAN_POINT('Ctrl Pts',(-11.3061389972225,63.8644876721369,
68.516714739936));
#115959=CARTESIAN_POINT('Ctrl Pts',(-11.3029179326569,63.8795313071419,
68.4796199057335));
#115960=CARTESIAN_POINT('Ctrl Pts',(-11.2831903810548,63.9716667113824,
68.2524309621477));
#115961=CARTESIAN_POINT('Ctrl Pts',(-11.2618246134247,64.0700160665622,
68.0298633002975));
#115962=CARTESIAN_POINT('Ctrl Pts',(-11.2388206575932,64.1740820572025,
67.8121857422244));
#115963=CARTESIAN_POINT('Ctrl Pts',(-11.2273186796775,64.2261150525226,
67.7033469631879));
#115964=CARTESIAN_POINT('Ctrl Pts',(-11.2154071551784,64.2795777051529,
67.5957302111428));
#115965=CARTESIAN_POINT('Ctrl Pts',(-11.2030860857381,64.3344106010308,
67.4893664567818));
#115966=CARTESIAN_POINT('Ctrl Pts',(-11.1969255510179,64.3618270489698,
67.4361845796012));
#115967=CARTESIAN_POINT('Ctrl Pts',(-11.1906626300008,64.3895860653485,
67.3833159637608));
#115968=CARTESIAN_POINT('Ctrl Pts',(-11.1842973224823,64.4176803955192,
67.3307643015798));
#115969=CARTESIAN_POINT('Ctrl Pts',(-11.1811146687231,64.4317275606045,
67.3044884704894));
#115970=CARTESIAN_POINT('Ctrl Pts',(-11.1779064183332,64.4458585544738,
67.2782918787736));
#115971=CARTESIAN_POINT('Ctrl Pts',(-11.174672571257,64.4600724756541,67.2521749866161));
#115972=CARTESIAN_POINT('Ctrl Pts',(-11.1730556477189,64.4671794362442,
67.2391165405373));
#115973=CARTESIAN_POINT('Ctrl Pts',(-11.1714323250089,64.4743071286741,
67.2260780194078));
#115974=CARTESIAN_POINT('Ctrl Pts',(-11.1698026031183,64.4814554407902,
67.213059480252));
#115975=CARTESIAN_POINT('Ctrl Pts',(-11.168987742173,64.4850295968483,67.2065502106741));
#115976=CARTESIAN_POINT('Ctrl Pts',(-11.1681712814325,64.4886089078284,
67.2000459365936));
#115977=CARTESIAN_POINT('Ctrl Pts',(-11.1673532208957,64.4921933597455,
67.1935466651054));
#115978=CARTESIAN_POINT('Ctrl Pts',(-11.1665624051131,64.4956584347858,
67.1872638458808));
#115979=CARTESIAN_POINT('Ctrl Pts',(-11.1659133956055,64.4985010255737,
67.1821184487777));
#115980=CARTESIAN_POINT('Ctrl Pts',(-11.1649906082438,64.5025403038718,
67.174825409623));
#115981=CARTESIAN_POINT('Ctrl Pts',(-11.1649588168765,64.5026794628862,
67.1745741538129));
#115982=CARTESIAN_POINT('Ctrl Pts',(-11.164926699816,64.5028200447192,67.1743203504369));
#115983=CARTESIAN_POINT('Ctrl Pts',(-11.1648942398947,64.502962124333,67.1740638655116));
#115984=CARTESIAN_POINT('Ctrl Pts',(-11.133705344973,64.6394783563636,66.9276220667889));
#115985=CARTESIAN_POINT('Ctrl Pts',(-11.1001630834324,64.7836965504124,
66.6878447959721));
#115986=CARTESIAN_POINT('Ctrl Pts',(-11.0642655908435,64.9348380776373,
66.455054390543));
#115987=CARTESIAN_POINT('Ctrl Pts',(-11.0283680982545,65.0859796048621,
66.222263985114));
#115988=CARTESIAN_POINT('Ctrl Pts',(-10.9901154073647,65.2440446410345,
65.9964602437078));
#115989=CARTESIAN_POINT('Ctrl Pts',(-10.9495093621566,65.4083044678963,
65.7779331134484));
#115990=CARTESIAN_POINT('Ctrl Pts',(-10.9164961960038,65.5418495331351,
65.600268127283));
#115991=CARTESIAN_POINT('Ctrl Pts',(-10.8819326095739,65.6794935075489,
65.4274080152561));
#115992=CARTESIAN_POINT('Ctrl Pts',(-10.8458035256173,65.8208659609748,
65.2594975392633));
#115993=CARTESIAN_POINT('Ctrl Pts',(-10.8374939995453,65.8533809865151,
65.2208788884364));
#115994=CARTESIAN_POINT('Ctrl Pts',(-10.8291016705225,65.8860933193816,
65.1825220121138));
#115995=CARTESIAN_POINT('Ctrl Pts',(-10.8206283362097,65.9189985771524,
65.1444274192187));
#115996=CARTESIAN_POINT('Ctrl Pts',(-10.7979710152082,66.0069857803518,
65.0425641635285));
#115997=CARTESIAN_POINT('Ctrl Pts',(-10.7747251214092,66.0963494876869,
64.942579704158));
#115998=CARTESIAN_POINT('Ctrl Pts',(-10.7508906568507,66.1869974467674,
64.8444930011935));
#115999=CARTESIAN_POINT('Ctrl Pts',(-10.7389734245714,66.2323214263077,
64.7954496497112));
#116000=CARTESIAN_POINT('Ctrl Pts',(-10.7269090494873,66.2779664681663,
64.7468807246663));
#116001=CARTESIAN_POINT('Ctrl Pts',(-10.7146975314213,66.3239213020834,
64.6987882485336));
#116002=CARTESIAN_POINT('Ctrl Pts',(-10.7085917723883,66.346898719042,64.6747420104673));
#116003=CARTESIAN_POINT('Ctrl Pts',(-10.7024492276056,66.3699535839574,
64.6508148841806));
#116004=CARTESIAN_POINT('Ctrl Pts',(-10.6962698970365,66.3930844949761,
64.6270071118253));
#116005=CARTESIAN_POINT('Ctrl Pts',(-10.693180231752,66.4046499504855,64.6151032256477));
#116006=CARTESIAN_POINT('Ctrl Pts',(-10.6900813700207,66.4162344175122,
64.6032291779221));
#116007=CARTESIAN_POINT('Ctrl Pts',(-10.6869733118381,66.4278377216821,
64.5913849977991));
#116008=CARTESIAN_POINT('Ctrl Pts',(-10.6846422682011,66.4365401998095,
64.5825018627067));
#116009=CARTESIAN_POINT('Ctrl Pts',(-10.6823060515603,66.4452532738292,
64.5736355281385));
#116010=CARTESIAN_POINT('Ctrl Pts',(-10.6799646619137,66.4539768703599,
64.564786006148));
#116011=CARTESIAN_POINT('Ctrl Pts',(-10.6791841986982,66.4568847358701,
64.5618361654845));
#116012=CARTESIAN_POINT('Ctrl Pts',(-10.678163888481,66.4606846596497,64.5579863129423));
#116013=CARTESIAN_POINT('Ctrl Pts',(-10.6776215479318,66.4627039716936,
64.5559420887767));
#116014=CARTESIAN_POINT('Ctrl Pts',(-10.652920616734,66.5546736537245,64.4628377827436));
#116015=CARTESIAN_POINT('Ctrl Pts',(-10.6266237018721,66.6518339313718,
64.3675198611269));
#116016=CARTESIAN_POINT('Ctrl Pts',(-10.5986163301073,66.7544884150816,
64.2704343258768));
#116017=CARTESIAN_POINT('Ctrl Pts',(-10.5712573585473,66.8547663391904,
64.1755964231955));
#116018=CARTESIAN_POINT('Ctrl Pts',(-10.542266066329,66.9602873558472,64.0790717461688));
#116019=CARTESIAN_POINT('Ctrl Pts',(-10.5115377512955,67.0713326407731,
63.9813254725246));
#116020=CARTESIAN_POINT('Ctrl Pts',(-10.4965124517656,67.1256307259617,
63.9335302374838));
#116021=CARTESIAN_POINT('Ctrl Pts',(-10.4810718844178,67.1812495720263,
63.8854436899028));
#116022=CARTESIAN_POINT('Ctrl Pts',(-10.4652041499233,67.2382215142498,
63.8371247472103));
#116023=CARTESIAN_POINT('Ctrl Pts',(-10.4356119623104,67.3444701033932,
63.7470133820432));
#116024=CARTESIAN_POINT('Ctrl Pts',(-10.4045313128674,67.4554250840708,
63.656091786564));
#116025=CARTESIAN_POINT('Ctrl Pts',(-10.3719812538623,67.5712962804336,
63.5647574873318));
#116026=CARTESIAN_POINT('Ctrl Pts',(-10.3401570523442,67.6845835805459,
63.4754599181993));
#116027=CARTESIAN_POINT('Ctrl Pts',(-10.3069279981041,67.8025704642133,
63.385767843356));
#116028=CARTESIAN_POINT('Ctrl Pts',(-10.2723471316926,67.9254453728009,
63.2960856483857));
#116029=CARTESIAN_POINT('Ctrl Pts',(-10.2388925685195,68.0443182299126,
63.2093244139668));
#116030=CARTESIAN_POINT('Ctrl Pts',(-10.2041726718904,68.1677660318666,
63.1225724811793));
#116031=CARTESIAN_POINT('Ctrl Pts',(-10.1682715444886,68.2959498272669,
63.0362266371425));
#116032=CARTESIAN_POINT('Ctrl Pts',(-10.1443231826302,68.381456666154,62.9786284036718));
#116033=CARTESIAN_POINT('Ctrl Pts',(-10.1198499387848,68.4690707061841,
62.9212114915483));
#116034=CARTESIAN_POINT('Ctrl Pts',(-10.0948866960176,68.5588367757668,
62.8641015189355));
#116035=CARTESIAN_POINT('',(-8.69365830054191,74.99999996484,60.98889557741));
#116036=CARTESIAN_POINT('Ctrl Pts',(-10.0948866959449,68.55883546897,62.86409946493));
#116037=CARTESIAN_POINT('Ctrl Pts',(-10.0517874763325,68.713679379568,62.7655898290921));
#116038=CARTESIAN_POINT('Ctrl Pts',(-10.0025194376179,68.8832413055288,
62.6626774372055));
#116039=CARTESIAN_POINT('Ctrl Pts',(-9.91936415089262,69.161045298009,62.5047129513255));
#116040=CARTESIAN_POINT('Ctrl Pts',(-9.89010351720865,69.2575565756358,
62.4514647396401));
#116041=CARTESIAN_POINT('Ctrl Pts',(-9.84389925951936,69.4083541324548,
62.3711334956229));
#116042=CARTESIAN_POINT('Ctrl Pts',(-9.82021880388388,69.4852604507093,
62.3308537265188));
#116043=CARTESIAN_POINT('Ctrl Pts',(-9.79157953375854,69.5776573407017,
62.2837614623395));
#116044=CARTESIAN_POINT('Ctrl Pts',(-9.77700688072487,69.6245281826994,
62.2602035713135));
#116045=CARTESIAN_POINT('Ctrl Pts',(-9.76965729971529,69.6481322203813,
62.2484233295547));
#116046=CARTESIAN_POINT('Ctrl Pts',(-9.76649392474845,69.6582844236361,
62.2433745542121));
#116047=CARTESIAN_POINT('Ctrl Pts',(-9.76438199598519,69.6650606067955,
62.2400087014928));
#116048=CARTESIAN_POINT('Ctrl Pts',(-9.76289125250944,69.6698422307222,
62.237637219044));
#116049=CARTESIAN_POINT('Ctrl Pts',(-9.74224303814605,69.736061144494,62.2048232038921));
#116050=CARTESIAN_POINT('Ctrl Pts',(-9.7152274917603,69.822130672148,62.1628079730791));
#116051=CARTESIAN_POINT('Ctrl Pts',(-9.66421461894981,69.9851088712327,
62.0868501574437));
#116052=CARTESIAN_POINT('Ctrl Pts',(-9.645462069141,70.0450855257516,62.0593877994143));
#116053=CARTESIAN_POINT('Ctrl Pts',(-9.61471085611982,70.1436997066793,
62.0153920835851));
#116054=CARTESIAN_POINT('Ctrl Pts',(-9.60402338706143,70.1780128534713,
62.0002606485247));
#116055=CARTESIAN_POINT('Ctrl Pts',(-9.58177431950867,70.2495538013399,
61.9691442671256));
#116056=CARTESIAN_POINT('Ctrl Pts',(-9.57054973139168,70.2856945972867,
61.9536190736345));
#116057=CARTESIAN_POINT('Ctrl Pts',(-9.50887136344287,70.4846360990521,
61.869476191664));
#116058=CARTESIAN_POINT('Ctrl Pts',(-9.4658047898713,70.6256256598509,61.8138358171528));
#116059=CARTESIAN_POINT('Ctrl Pts',(-9.41061911069516,70.8083647148666,
61.7445825194025));
#116060=CARTESIAN_POINT('Ctrl Pts',(-9.39379291449998,70.8644935704817,
61.7238746103894));
#116061=CARTESIAN_POINT('Ctrl Pts',(-9.37090716550251,70.9413769302308,
61.6960455635373));
#116062=CARTESIAN_POINT('Ctrl Pts',(-9.36005267732761,70.9779916361502,
61.6829401129446));
#116063=CARTESIAN_POINT('Ctrl Pts',(-9.34841878385691,71.0174873934192,
61.6690029851454));
#116064=CARTESIAN_POINT('Ctrl Pts',(-9.34285925613824,71.0364272480192,
61.6623653530905));
#116065=CARTESIAN_POINT('Ctrl Pts',(-9.34014384703307,71.0456948436297,
61.6591283889064));
#116066=CARTESIAN_POINT('Ctrl Pts',(-9.33899389057818,71.0496232796143,
61.6577585658768));
#116067=CARTESIAN_POINT('Ctrl Pts',(-9.33823031745369,71.0522325908458,
61.6568492175692));
#116068=CARTESIAN_POINT('Ctrl Pts',(-9.33816064917692,71.0524704010327,
61.6567661833087));
#116069=CARTESIAN_POINT('Ctrl Pts',(-9.29335562400464,71.2056773548895,
61.6034324787957));
#116070=CARTESIAN_POINT('Ctrl Pts',(-9.25256208948599,71.3495159998227,
61.5567275679463));
#116071=CARTESIAN_POINT('Ctrl Pts',(-9.19635506156912,71.5541522804732,
61.4940547720857));
#116072=CARTESIAN_POINT('Ctrl Pts',(-9.16949736607596,71.6536924314009,
61.4645663009794));
#116073=CARTESIAN_POINT('Ctrl Pts',(-9.14034357031482,71.7648525579011,
61.4331264352157));
#116074=CARTESIAN_POINT('Ctrl Pts',(-9.12631171801281,71.8191781361214,
61.4181151035729));
#116075=CARTESIAN_POINT('Ctrl Pts',(-9.11943205325644,71.846025843946,61.4107826062409));
#116076=CARTESIAN_POINT('Ctrl Pts',(-9.116512824374,71.8574643349694,61.4076767929975));
#116077=CARTESIAN_POINT('Ctrl Pts',(-9.11457316042354,71.8650749413428,
61.4056143565919));
#116078=CARTESIAN_POINT('Ctrl Pts',(-9.11392168583116,71.8676329160552,
61.4049218626105));
#116079=CARTESIAN_POINT('Ctrl Pts',(-9.07173262458759,72.0336242990951,
61.3601142300229));
#116080=CARTESIAN_POINT('Ctrl Pts',(-9.03417637446264,72.1909616694013,
61.3212391441379));
#116081=CARTESIAN_POINT('Ctrl Pts',(-8.98287353135119,72.421132329324,61.2690075114148));
#116082=CARTESIAN_POINT('Ctrl Pts',(-8.95847999281444,72.5347600286294,
61.244412301046));
#116083=CARTESIAN_POINT('Ctrl Pts',(-8.93222215980482,72.6646996977874,
61.2182123336129));
#116084=CARTESIAN_POINT('Ctrl Pts',(-8.91964356712081,72.7290045056888,
61.2057154921927));
#116085=CARTESIAN_POINT('Ctrl Pts',(-8.91349185173401,72.7609896077938,
61.1996153101984));
#116086=CARTESIAN_POINT('Ctrl Pts',(-8.91088488391578,72.7746615487225,
61.1970324401455));
#116087=CARTESIAN_POINT('Ctrl Pts',(-8.90915345684435,72.7837681728654,
61.1953174952357));
#116088=CARTESIAN_POINT('Ctrl Pts',(-8.90853914396999,72.787004805579,61.1947091358399));
#116089=CARTESIAN_POINT('Ctrl Pts',(-8.76569912277902,73.5426843179641,
61.0533060591291));
#116090=CARTESIAN_POINT('Ctrl Pts',(-8.69444127063165,74.2829857452934,
60.9888893886809));
#116091=CARTESIAN_POINT('Ctrl Pts',(-8.69365830054191,74.99999996484,60.98889557741));
#116092=CARTESIAN_POINT('',(-8.56753648333091,75.,60.98888938658));
#116093=CARTESIAN_POINT('',(-15.5675364833309,75.,60.98888938658));
#116094=CARTESIAN_POINT('Origin',(-8.56753648333091,75.,72.98888938658));
#116095=CARTESIAN_POINT('',(-10.0948723726626,81.4411120680386,62.8640650186986));
#116096=CARTESIAN_POINT('Ctrl Pts',(-8.69365830112979,74.9999999638356,
60.9889038049687));
#116097=CARTESIAN_POINT('Ctrl Pts',(-8.69384525819957,75.1754233378247,
60.9889252073905));
#116098=CARTESIAN_POINT('Ctrl Pts',(-8.6982707338728,75.3522672414099,60.9928047886458));
#116099=CARTESIAN_POINT('Ctrl Pts',(-8.70692055121058,75.5303670372353,
61.0006933469007));
#116100=CARTESIAN_POINT('Ctrl Pts',(-8.71504876408759,75.6977269937859,
61.0081062064195));
#116101=CARTESIAN_POINT('Ctrl Pts',(-8.72690760340725,75.8661963210868,
61.0190593542814));
#116102=CARTESIAN_POINT('Ctrl Pts',(-8.74250791810455,76.0356077139438,
61.0337104975575));
#116103=CARTESIAN_POINT('Ctrl Pts',(-8.74350902300405,76.046479198187,61.034650692137));
#116104=CARTESIAN_POINT('Ctrl Pts',(-8.74452554254038,76.0573545496545,
61.0356061263879));
#116105=CARTESIAN_POINT('Ctrl Pts',(-8.74555748243123,76.0682337189115,
61.0365768465842));
#116106=CARTESIAN_POINT('Ctrl Pts',(-8.75602273934144,76.1785631114021,
61.0464212535427));
#116107=CARTESIAN_POINT('Ctrl Pts',(-8.76806128130061,76.2892941174044,
61.0578380775563));
#116108=CARTESIAN_POINT('Ctrl Pts',(-8.7816935935759,76.4003647326638,61.0708786774501));
#116109=CARTESIAN_POINT('Ctrl Pts',(-8.7903528007498,76.4709164812624,61.0791620305506));
#116110=CARTESIAN_POINT('Ctrl Pts',(-8.79965517985068,76.5416050269056,
61.0881006652942));
#116111=CARTESIAN_POINT('Ctrl Pts',(-8.80959012670336,76.6124245282971,
61.0977035097661));
#116112=CARTESIAN_POINT('Ctrl Pts',(-8.82237796377352,76.7035803501261,
61.1100638789093));
#116113=CARTESIAN_POINT('Ctrl Pts',(-8.83622366435869,76.794946917876,61.1235238847051));
#116114=CARTESIAN_POINT('Ctrl Pts',(-8.85112722717444,76.8864966022424,
61.1381012094152));
#116115=CARTESIAN_POINT('Ctrl Pts',(-8.85857900858232,76.9322714444256,
61.1453898717702));
#116116=CARTESIAN_POINT('Ctrl Pts',(-8.86629525561024,76.9780920688098,
61.1529578765693));
#116117=CARTESIAN_POINT('Ctrl Pts',(-8.87427596840209,77.023954905813,61.160807494838));
#116118=CARTESIAN_POINT('Ctrl Pts',(-8.87826632479801,77.0468863243146,
61.1647323039724));
#116119=CARTESIAN_POINT('Ctrl Pts',(-8.88232279763742,77.0698282960359,
61.1687275173494));
#116120=CARTESIAN_POINT('Ctrl Pts',(-8.88644538694687,77.0927803713609,
61.1727934236992));
#116121=CARTESIAN_POINT('Ctrl Pts',(-8.88953732892895,77.1099944278547,
61.1758428534616));
#116122=CARTESIAN_POINT('Ctrl Pts',(-8.89266646142556,77.1272141676282,
61.1789320480973));
#116123=CARTESIAN_POINT('Ctrl Pts',(-8.89583278444763,77.1444393994645,
61.1820611305557));
#116124=CARTESIAN_POINT('Ctrl Pts',(-8.89688822545498,77.1501811434099,
61.1831041580418));
#116125=CARTESIAN_POINT('Ctrl Pts',(-8.89817253250436,77.1571368374197,
61.1843738562206));
#116126=CARTESIAN_POINT('Ctrl Pts',(-8.89901150431184,77.1616664547679,
61.1852035135444));
#116127=CARTESIAN_POINT('Ctrl Pts',(-8.92259264299848,77.2889812631243,
61.208522848285));
#116128=CARTESIAN_POINT('Ctrl Pts',(-8.94869408539285,77.4192468165972,
61.2345070151699));
#116129=CARTESIAN_POINT('Ctrl Pts',(-8.97731850656541,77.5523261726857,
61.2634710633927));
#116130=CARTESIAN_POINT('Ctrl Pts',(-8.98128295423502,77.5707575023513,
61.2674825489975));
#116131=CARTESIAN_POINT('Ctrl Pts',(-8.98529573764546,77.5892427551795,
61.2715512181843));
#116132=CARTESIAN_POINT('Ctrl Pts',(-8.98935680388911,77.6077815160241,
61.2756779307514));
#116133=CARTESIAN_POINT('Ctrl Pts',(-9.00017439012048,77.6571637797025,
61.2866703811001));
#116134=CARTESIAN_POINT('Ctrl Pts',(-9.01133389180735,77.7069265004623,
61.2980748268113));
#116135=CARTESIAN_POINT('Ctrl Pts',(-9.02283815665349,77.7570601265521,
61.309907433083));
#116136=CARTESIAN_POINT('Ctrl Pts',(-9.02908498811848,77.7842827537343,
61.3163325543888));
#116137=CARTESIAN_POINT('Ctrl Pts',(-9.03543346584944,77.8116147226887,
61.3228839209108));
#116138=CARTESIAN_POINT('Ctrl Pts',(-9.04188245493954,77.8390552997318,
61.3295643639931));
#116139=CARTESIAN_POINT('Ctrl Pts',(-9.05104523026728,77.878043091275,61.3390559910058));
#116140=CARTESIAN_POINT('Ctrl Pts',(-9.06041225574227,77.9172494421727,
61.3488080181036));
#116141=CARTESIAN_POINT('Ctrl Pts',(-9.06998353136695,77.9566702598686,
61.3588281350206));
#116142=CARTESIAN_POINT('Ctrl Pts',(-9.07476916917929,77.9763806687166,
61.3638381934791));
#116143=CARTESIAN_POINT('Ctrl Pts',(-9.07960586952718,77.9961446939862,
61.3689152751757));
#116144=CARTESIAN_POINT('Ctrl Pts',(-9.08449363240003,78.0159618136268,
61.3740603435686));
#116145=CARTESIAN_POINT('Ctrl Pts',(-9.08693751383645,78.0258703734471,
61.376632877765));
#116146=CARTESIAN_POINT('Ctrl Pts',(-9.08939416090401,78.0357922068428,
61.3792224086809));
#116147=CARTESIAN_POINT('Ctrl Pts',(-9.09186357360078,78.0457272474666,
61.3818290567522));
#116148=CARTESIAN_POINT('Ctrl Pts',(-9.09309827994918,78.0506947677785,
61.3831323807878));
#116149=CARTESIAN_POINT('Ctrl Pts',(-9.09433617770486,78.0556655898965,
61.3844399841149));
#116150=CARTESIAN_POINT('Ctrl Pts',(-9.09557726686759,78.060639705455,61.3857518817859));
#116151=CARTESIAN_POINT('Ctrl Pts',(-9.09681835603032,78.0656138210136,
61.387063779457));
#116152=CARTESIAN_POINT('Ctrl Pts',(-9.09837266160549,78.0718290451585,
61.3887081459466));
#116153=CARTESIAN_POINT('Ctrl Pts',(-9.09931010857661,78.0755719240635,
61.3897004728883));
#116154=CARTESIAN_POINT('Ctrl Pts',(-9.11922887776139,78.1551001995736,
61.4107853255961));
#116155=CARTESIAN_POINT('Ctrl Pts',(-9.1407460830329,78.2384488549837,61.4337575836913));
#116156=CARTESIAN_POINT('Ctrl Pts',(-9.16387330016365,78.3255241006586,
61.4588727406335));
#116157=CARTESIAN_POINT('Ctrl Pts',(-9.17557641127034,78.3695869582439,
61.4715818128273));
#116158=CARTESIAN_POINT('Ctrl Pts',(-9.18769115678514,78.4146039068995,
61.4848399730603));
#116159=CARTESIAN_POINT('Ctrl Pts',(-9.20021442302084,78.4605617067419,
61.4986824948998));
#116160=CARTESIAN_POINT('Ctrl Pts',(-9.21885004348183,78.5289505838102,
61.5192812730754));
#116161=CARTESIAN_POINT('Ctrl Pts',(-9.2383947815182,78.5994224592807,61.541173598283));
#116162=CARTESIAN_POINT('Ctrl Pts',(-9.25884863686747,78.6719265687999,
61.5644800667747));
#116163=CARTESIAN_POINT('Ctrl Pts',(-9.2690755645421,78.7081786235595,61.5761333010206));
#116164=CARTESIAN_POINT('Ctrl Pts',(-9.27952977153974,78.7449387014591,
61.5881401814723));
#116165=CARTESIAN_POINT('Ctrl Pts',(-9.29021125784852,78.7821997258525,
61.6005162513103));
#116166=CARTESIAN_POINT('Ctrl Pts',(-9.29555200100291,78.8008302380492,
61.6067042862293));
#116167=CARTESIAN_POINT('Ctrl Pts',(-9.30094956398611,78.8195859849683,
61.6129846249781));
#116168=CARTESIAN_POINT('Ctrl Pts',(-9.30640394680137,78.8384660515663,
61.6193592424304));
#116169=CARTESIAN_POINT('Ctrl Pts',(-9.309131138209,78.8479060848653,61.6225465511565));
#116170=CARTESIAN_POINT('Ctrl Pts',(-9.31187253457468,78.8573771979606,
61.625757429952));
#116171=CARTESIAN_POINT('Ctrl Pts',(-9.31462813589891,78.8668792738138,
61.6289921273608));
#116172=CARTESIAN_POINT('Ctrl Pts',(-9.31600593656103,78.8716303117403,
61.6306094760651));
#116173=CARTESIAN_POINT('Ctrl Pts',(-9.31738728846278,78.8763890903488,
61.632232779447));
#116174=CARTESIAN_POINT('Ctrl Pts',(-9.31877219160423,78.8811555948331,
61.6338620686736));
#116175=CARTESIAN_POINT('Ctrl Pts',(-9.32015709474568,78.8859220993175,
61.6354913579001));
#116176=CARTESIAN_POINT('Ctrl Pts',(-9.32207911460549,78.8925292812147,
61.6377557517266));
#116177=CARTESIAN_POINT('Ctrl Pts',(-9.32293755474769,78.8954782710375,
61.6387679251359));
#116178=CARTESIAN_POINT('Ctrl Pts',(-9.32540791029129,78.9039646558167,
61.6416806829042));
#116179=CARTESIAN_POINT('Ctrl Pts',(-9.32791655809782,78.9125679742487,
61.6446441886323));
#116180=CARTESIAN_POINT('Ctrl Pts',(-9.33046352415257,78.9212879068898,
61.6476592438058));
#116181=CARTESIAN_POINT('Ctrl Pts',(-9.34717122788578,78.9784893175131,
61.667437539823));
#116182=CARTESIAN_POINT('Ctrl Pts',(-9.3655294968389,79.0407103562356,61.6894307270498));
#116183=CARTESIAN_POINT('Ctrl Pts',(-9.38554373915658,79.1078507385285,
61.7138910349835));
#116184=CARTESIAN_POINT('Ctrl Pts',(-9.39640552175165,79.1442880027646,
61.7271657092263));
#116185=CARTESIAN_POINT('Ctrl Pts',(-9.40775469220893,79.1821738158082,
61.7411677299387));
#116186=CARTESIAN_POINT('Ctrl Pts',(-9.41958877910638,79.2214898186444,
61.7559424868357));
#116187=CARTESIAN_POINT('Ctrl Pts',(-9.43807081163282,79.2828920754915,
61.7790171473404));
#116188=CARTESIAN_POINT('Ctrl Pts',(-9.45773959183724,79.3477825665806,
61.8039753638204));
#116189=CARTESIAN_POINT('Ctrl Pts',(-9.47859511967813,79.4160775816128,
61.8310049113892));
#116190=CARTESIAN_POINT('Ctrl Pts',(-9.48902288359857,79.4502250891288,
61.8445196851735));
#116191=CARTESIAN_POINT('Ctrl Pts',(-9.49974733441796,79.4852234981225,
61.8585525848617));
#116192=CARTESIAN_POINT('Ctrl Pts',(-9.51076847209598,79.5210608981225,
61.8731287732406));
#116193=CARTESIAN_POINT('Ctrl Pts',(-9.51627904093499,79.5389795981225,
61.8804168674301));
#116194=CARTESIAN_POINT('Ctrl Pts',(-9.52186378148761,79.5571080376222,
61.8878408038733));
#116195=CARTESIAN_POINT('Ctrl Pts',(-9.52752269375218,79.5754446213074,
61.8954038234184));
#116196=CARTESIAN_POINT('Ctrl Pts',(-9.53250202705314,79.591579164043,61.9020585996927));
#116197=CARTESIAN_POINT('Ctrl Pts',(-9.53722776857092,79.6068699851859,
61.9084020592662));
#116198=CARTESIAN_POINT('Ctrl Pts',(-9.54252091927987,79.6239686624488,
61.915542315475));
#116199=CARTESIAN_POINT('Ctrl Pts',(-9.54324332801525,79.6263022883924,
61.9165168170038));
#116200=CARTESIAN_POINT('Ctrl Pts',(-9.543976307386,79.6286695552575,61.9175062316699));
#116201=CARTESIAN_POINT('Ctrl Pts',(-9.54472194568067,79.631077170464,61.9185134474129));
#116202=CARTESIAN_POINT('Ctrl Pts',(-9.5668688246071,79.7025879322633,61.9484296752574));
#116203=CARTESIAN_POINT('Ctrl Pts',(-9.58752489475418,79.7690234373903,
61.9770336810328));
#116204=CARTESIAN_POINT('Ctrl Pts',(-9.60667184392161,79.8304899452595,
62.0040640470899));
#116205=CARTESIAN_POINT('Ctrl Pts',(-9.61673055756171,79.8627809382373,
62.0182642577541));
#116206=CARTESIAN_POINT('Ctrl Pts',(-9.62637339967271,79.8937002699575,
62.0320307794531));
#116207=CARTESIAN_POINT('Ctrl Pts',(-9.63560119149857,79.9232614284828,
62.0453297721826));
#116208=CARTESIAN_POINT('Ctrl Pts',(-9.64820426117206,79.963635263042,62.0634931784579));
#116209=CARTESIAN_POINT('Ctrl Pts',(-9.66003293470919,80.0014757893863,
62.0807841343321));
#116210=CARTESIAN_POINT('Ctrl Pts',(-9.67109405079398,80.0368130179988,
62.0971251414243));
#116211=CARTESIAN_POINT('Ctrl Pts',(-9.68740373782591,80.0889179895793,
62.1212200618118));
#116212=CARTESIAN_POINT('Ctrl Pts',(-9.70203412279025,80.1355847671629,
62.1432491475576));
#116213=CARTESIAN_POINT('Ctrl Pts',(-9.71498478797446,80.1769050203069,
62.1630077286355));
#116214=CARTESIAN_POINT('Ctrl Pts',(-9.71576166184407,80.1793837057255,
62.1641929901739));
#116215=CARTESIAN_POINT('Ctrl Pts',(-9.71653249553801,80.1818431456697,
62.1653700949537));
#116216=CARTESIAN_POINT('Ctrl Pts',(-9.71729729042005,80.1842833575417,
62.16653900399));
#116217=CARTESIAN_POINT('Ctrl Pts',(-9.72405434070977,80.2058429086365,
62.1768664490702));
#116218=CARTESIAN_POINT('Ctrl Pts',(-9.73033964617562,80.2259017641078,
62.1865538905201));
#116219=CARTESIAN_POINT('Ctrl Pts',(-9.7361532068364,80.2444714445637,62.1955766594361));
#116220=CARTESIAN_POINT('Ctrl Pts',(-9.73905998716679,80.2537562847916,
62.2000880438941));
#116221=CARTESIAN_POINT('Ctrl Pts',(-9.74184883129493,80.2626688041486,
62.2044333159049));
#116222=CARTESIAN_POINT('Ctrl Pts',(-9.74451973922586,80.2712103088226,
62.2086097405811));
#116223=CARTESIAN_POINT('Ctrl Pts',(-9.74585519319132,80.2754810611597,
62.2106979529192));
#116224=CARTESIAN_POINT('Ctrl Pts',(-9.74716116310733,80.2796590581362,
62.2127439569184));
#116225=CARTESIAN_POINT('Ctrl Pts',(-9.74843764897426,80.283744453113,62.2147474318027));
#116226=CARTESIAN_POINT('Ctrl Pts',(-9.74907589190773,80.2857871506015,
62.2157491692448));
#116227=CARTESIAN_POINT('Ctrl Pts',(-9.74970676382892,80.287806697483,62.2167402746261));
#116228=CARTESIAN_POINT('Ctrl Pts',(-9.75033026473789,80.2898031123722,
62.2177207091992));
#116229=CARTESIAN_POINT('Ctrl Pts',(-9.75095376564686,80.2917995272614,
62.2187011437723));
#116230=CARTESIAN_POINT('Ctrl Pts',(-9.7510833222648,80.2922140646321,62.2189043469225));
#116231=CARTESIAN_POINT('Ctrl Pts',(-9.75217865442817,80.2957229792706,
62.2206299626292));
#116232=CARTESIAN_POINT('Ctrl Pts',(-9.78387650612535,80.3972675696231,
62.270567609481));
#116233=CARTESIAN_POINT('Ctrl Pts',(-9.81432835451053,80.4952254170197,
62.3205249514219));
#116234=CARTESIAN_POINT('Ctrl Pts',(-9.8434407469923,80.5896997430749,62.3702581386498));
#116235=CARTESIAN_POINT('Ctrl Pts',(-9.8650914418614,80.6599596781753,62.407244382986));
#116236=CARTESIAN_POINT('Ctrl Pts',(-9.88600253165974,80.7282928637747,
62.44410692794));
#116237=CARTESIAN_POINT('Ctrl Pts',(-9.90615340852189,80.794740148219,62.4807503211802));
#116238=CARTESIAN_POINT('Ctrl Pts',(-9.93782589210618,80.8991797981746,
62.5383451980092));
#116239=CARTESIAN_POINT('Ctrl Pts',(-9.96761929950232,80.9989601739828,
62.5953972789563));
#116240=CARTESIAN_POINT('Ctrl Pts',(-9.99557073594596,81.0942161190798,
62.6515538909901));
#116241=CARTESIAN_POINT('Ctrl Pts',(-10.0249108575926,81.1942045766444,
62.7105004797159));
#116242=CARTESIAN_POINT('Ctrl Pts',(-10.0522219028098,81.2892080666935,
62.76846016398));
#116243=CARTESIAN_POINT('Ctrl Pts',(-10.0775940451767,81.3793801999264,
62.8250569690241));
#116244=CARTESIAN_POINT('Ctrl Pts',(-10.0834563564733,81.4002147478192,
62.8381338343814));
#116245=CARTESIAN_POINT('Ctrl Pts',(-10.0892153309249,81.4207913544346,
62.8511380792578));
#116246=CARTESIAN_POINT('Ctrl Pts',(-10.0948723726601,81.4411118802155,
62.8640653139415));
#116247=CARTESIAN_POINT('',(-10.7325524156118,83.7450179064977,64.7715505688173));
#116248=CARTESIAN_POINT('Ctrl Pts',(-10.0948723726639,81.4411122211604,
62.8640647780043));
#116249=CARTESIAN_POINT('Ctrl Pts',(-10.1238158396739,81.5451332595941,
62.9302398682223));
#116250=CARTESIAN_POINT('Ctrl Pts',(-10.1526418118159,81.6482221786327,
62.9980739436566));
#116251=CARTESIAN_POINT('Ctrl Pts',(-10.1812698397242,81.7503263490054,
63.0675440049332));
#116252=CARTESIAN_POINT('Ctrl Pts',(-10.2098978676326,81.8524305193781,
63.1370140662099));
#116253=CARTESIAN_POINT('Ctrl Pts',(-10.2383279513072,81.9535503248741,
63.2081195517163));
#116254=CARTESIAN_POINT('Ctrl Pts',(-10.2664843011526,82.0536858471839,
63.2808764091866));
#116255=CARTESIAN_POINT('Ctrl Pts',(-10.2946406509979,82.1538213694936,
63.353633266657));
#116256=CARTESIAN_POINT('Ctrl Pts',(-10.3225232670139,82.252972511183,63.4280416176109));
#116257=CARTESIAN_POINT('Ctrl Pts',(-10.3500718066949,82.3511229877178,
63.5041125932418));
#116258=CARTESIAN_POINT('Ctrl Pts',(-10.3776203463759,82.4492734642527,
63.5801835688728));
#116259=CARTESIAN_POINT('Ctrl Pts',(-10.4048348097219,82.5464232578521,
63.6579171984223));
#116260=CARTESIAN_POINT('Ctrl Pts',(-10.4316631941731,82.6425496669633,
63.7373254870007));
#116261=CARTESIAN_POINT('Ctrl Pts',(-10.4584915786242,82.7386760760745,
63.8167337755791));
#116262=CARTESIAN_POINT('Ctrl Pts',(-10.4849338841806,82.8337791084527,
63.8978167095015));
#116263=CARTESIAN_POINT('Ctrl Pts',(-10.5109460339877,82.9278331310342,
63.9805897775263));
#116264=CARTESIAN_POINT('Ctrl Pts',(-10.5369581837949,83.0218871536157,
64.0633628455512));
#116265=CARTESIAN_POINT('Ctrl Pts',(-10.5625401778529,83.1148920931469,
64.1478261377776));
#116266=CARTESIAN_POINT('Ctrl Pts',(-10.5876554908367,83.2068100073309,
64.2339896439459));
#116267=CARTESIAN_POINT('Ctrl Pts',(-10.6127708038206,83.2987279215148,
64.3201531501143));
#116268=CARTESIAN_POINT('Ctrl Pts',(-10.6374194357302,83.3895589867901,
64.408016670944));
#116269=CARTESIAN_POINT('Ctrl Pts',(-10.6615778397041,83.4792788066254,
64.4976096880002));
#116270=CARTESIAN_POINT('Ctrl Pts',(-10.6857362436779,83.5689986264608,
64.5872027050565));
#116271=CARTESIAN_POINT('Ctrl Pts',(-10.7094044197159,83.6576065909718,
64.678525829176));
#116272=CARTESIAN_POINT('Ctrl Pts',(-10.7325524156119,83.745018045238,64.7715504384495));
#116273=CARTESIAN_POINT('',(-10.7325548086171,83.7450176039532,81.2062285734056));
#116274=CARTESIAN_POINT('Ctrl Pts',(-10.7325524156115,83.7450176952948,
64.7715507672746));
#116275=CARTESIAN_POINT('Ctrl Pts',(-10.7501562547286,83.8114962912959,
64.8422991787488));
#116276=CARTESIAN_POINT('Ctrl Pts',(-10.7667240350834,83.8787704405261,
64.9156125289802));
#116277=CARTESIAN_POINT('Ctrl Pts',(-10.7822782455101,83.9466666344631,
64.9915677571402));
#116278=CARTESIAN_POINT('Ctrl Pts',(-10.7837981649509,83.9533012846502,
64.9989899164616));
#116279=CARTESIAN_POINT('Ctrl Pts',(-10.7853084365357,83.9599418483979,
65.0064372924184));
#116280=CARTESIAN_POINT('Ctrl Pts',(-10.7868091014514,83.9665881465513,
65.013909950191));
#116281=CARTESIAN_POINT('Ctrl Pts',(-10.8032614660996,84.0394540606112,
65.0958355614857));
#116282=CARTESIAN_POINT('Ctrl Pts',(-10.8185561237797,84.1130118947079,
65.1808006373549));
#116283=CARTESIAN_POINT('Ctrl Pts',(-10.832689957148,84.1870643803022,65.2689256223875));
#116284=CARTESIAN_POINT('Ctrl Pts',(-10.8388533377215,84.2193566565192,
65.3073545331184));
#116285=CARTESIAN_POINT('Ctrl Pts',(-10.8447964533634,84.2517425768332,
65.3463842196399));
#116286=CARTESIAN_POINT('Ctrl Pts',(-10.8505214018681,84.2842037635522,
65.3860241055826));
#116287=CARTESIAN_POINT('Ctrl Pts',(-10.8640271490599,84.3607830692007,
65.4795387071206));
#116288=CARTESIAN_POINT('Ctrl Pts',(-10.8763166551811,84.4377836100341,
65.5764500611726));
#116289=CARTESIAN_POINT('Ctrl Pts',(-10.8873758646346,84.5149629273589,
65.6768811296746));
#116290=CARTESIAN_POINT('Ctrl Pts',(-10.8922499094149,84.5489776053826,
65.7211433825304));
#116291=CARTESIAN_POINT('Ctrl Pts',(-10.8968854238649,84.5830265448267,
65.7660891430358));
#116292=CARTESIAN_POINT('Ctrl Pts',(-10.9012834140875,84.617086714057,65.8117281677846));
#116293=CARTESIAN_POINT('Ctrl Pts',(-10.9116143286586,84.6970943268044,
65.9189346057086));
#116294=CARTESIAN_POINT('Ctrl Pts',(-10.920632708015,84.77716637353,66.0299671776509));
#116295=CARTESIAN_POINT('Ctrl Pts',(-10.9283128382425,84.8570095906465,
66.1449612477235));
#116296=CARTESIAN_POINT('Ctrl Pts',(-10.9306986035121,84.8818121875772,
66.1806831496261));
#116297=CARTESIAN_POINT('Ctrl Pts',(-10.9329554612622,84.9065924256239,
66.2167872334362));
#116298=CARTESIAN_POINT('Ctrl Pts',(-10.9350832924956,84.9313407463341,
66.2532772859761));
#116299=CARTESIAN_POINT('Ctrl Pts',(-10.9358584453185,84.9403563723677,
66.2665703360984));
#116300=CARTESIAN_POINT('Ctrl Pts',(-10.9366167445909,84.9493676639085,
66.2799144663096));
#116301=CARTESIAN_POINT('Ctrl Pts',(-10.9373582249864,84.9583741277226,
66.2933098234466));
#116302=CARTESIAN_POINT('Ctrl Pts',(-10.9440570613183,85.0397421954264,
66.4143289435964));
#116303=CARTESIAN_POINT('Ctrl Pts',(-10.9493806507756,85.1207191934572,
66.5395306431455));
#116304=CARTESIAN_POINT('Ctrl Pts',(-10.9533178722974,85.200945015527,66.6690229320925));
#116305=CARTESIAN_POINT('Ctrl Pts',(-10.95495748534,85.2343541857984,66.7229485861856));
#116306=CARTESIAN_POINT('Ctrl Pts',(-10.956357038406,85.2676326509186,66.7776181129226));
#116307=CARTESIAN_POINT('Ctrl Pts',(-10.9575173777474,85.3007524839038,
66.8330383629357));
#116308=CARTESIAN_POINT('Ctrl Pts',(-10.9600931298752,85.3742727699435,
66.9560617077453));
#116309=CARTESIAN_POINT('Ctrl Pts',(-10.9614887331737,85.4470130418676,
67.0827853050045));
#116310=CARTESIAN_POINT('Ctrl Pts',(-10.9617079988126,85.5186654928951,
67.2132797997646));
#116311=CARTESIAN_POINT('Ctrl Pts',(-10.9618285298819,85.5580530895288,
67.2850130684641));
#116312=CARTESIAN_POINT('Ctrl Pts',(-10.9615938364338,85.5971114297609,
67.357885402198));
#116313=CARTESIAN_POINT('Ctrl Pts',(-10.9610019761566,85.6357852055068,
67.4319049822405));
#116314=CARTESIAN_POINT('Ctrl Pts',(-10.960166156352,85.6903999666699,67.5364347729694));
#116315=CARTESIAN_POINT('Ctrl Pts',(-10.9586176011902,85.7442481188906,
67.6432527692208));
#116316=CARTESIAN_POINT('Ctrl Pts',(-10.9563601692076,85.7971735499566,
67.7523800120814));
#116317=CARTESIAN_POINT('Ctrl Pts',(-10.9544321874464,85.8423750295958,
67.8455811962171));
#116318=CARTESIAN_POINT('Ctrl Pts',(-10.9519858673571,85.886903029062,67.9404660981445));
#116319=CARTESIAN_POINT('Ctrl Pts',(-10.9490212087671,85.930654905422,68.0370430779914));
#116320=CARTESIAN_POINT('Ctrl Pts',(-10.9485794522018,85.937174266096,68.0514337788437));
#116321=CARTESIAN_POINT('Ctrl Pts',(-10.9481262039085,85.9436763919122,
68.0658620559854));
#116322=CARTESIAN_POINT('Ctrl Pts',(-10.9476614373451,85.9501609285741,
68.080327917286));
#116323=CARTESIAN_POINT('Ctrl Pts',(-10.9465666637759,85.9654354769264,
68.1144027493692));
#116324=CARTESIAN_POINT('Ctrl Pts',(-10.9454079726398,85.9806124352409,
68.1486861231865));
#116325=CARTESIAN_POINT('Ctrl Pts',(-10.9441854670397,85.9956873076151,
68.1831782342848));
#116326=CARTESIAN_POINT('Ctrl Pts',(-10.9433147177819,86.0064246276983,
68.2077457946603));
#116327=CARTESIAN_POINT('Ctrl Pts',(-10.9424115723738,86.0171101545612,
68.2324192477099));
#116328=CARTESIAN_POINT('Ctrl Pts',(-10.941476030815,86.0277422448405,68.2571986441174));
#116329=CARTESIAN_POINT('Ctrl Pts',(-10.9410082600356,86.0330582899801,
68.2695883423211));
#116330=CARTESIAN_POINT('Ctrl Pts',(-10.9405323902186,86.0383609758636,
68.2820045264164));
#116331=CARTESIAN_POINT('Ctrl Pts',(-10.9400484213637,86.043650095586,68.2944472011266));
#116332=CARTESIAN_POINT('Ctrl Pts',(-10.9396261812646,86.0482646041711,
68.3053028505135));
#116333=CARTESIAN_POINT('Ctrl Pts',(-10.9391360171996,86.053523683442,68.317730587338));
#116334=CARTESIAN_POINT('Ctrl Pts',(-10.9387395065561,86.0577128820342,
68.3276685659382));
#116335=CARTESIAN_POINT('Ctrl Pts',(-10.9386815392793,86.0583253156173,
68.3291214337621));
#116336=CARTESIAN_POINT('Ctrl Pts',(-10.9386255999408,86.0589149648276,
68.3305210536576));
#116337=CARTESIAN_POINT('Ctrl Pts',(-10.9385722176855,86.059476548673,68.3318547014369));
#116338=CARTESIAN_POINT('Ctrl Pts',(-10.9349831434126,86.0972337794337,
68.4215204697137));
#116339=CARTESIAN_POINT('Ctrl Pts',(-10.9308041525169,86.1359710144443,
68.5165530785467));
#116340=CARTESIAN_POINT('Ctrl Pts',(-10.926022556049,86.1752952890009,68.6170738907957));
#116341=CARTESIAN_POINT('Ctrl Pts',(-10.9237789724588,86.1937467199572,
68.6642394862912));
#116342=CARTESIAN_POINT('Ctrl Pts',(-10.9214030150662,86.2123267369797,
68.7126133546548));
#116343=CARTESIAN_POINT('Ctrl Pts',(-10.9188952104483,86.230991194323,68.7622078211464));
#116344=CARTESIAN_POINT('Ctrl Pts',(-10.9167755798745,86.2467666475405,
68.8041257388006));
#116345=CARTESIAN_POINT('Ctrl Pts',(-10.91456175562,86.2626023824771,68.846915631229));
#116346=CARTESIAN_POINT('Ctrl Pts',(-10.9122560350931,86.2784706480888,
68.8905849692834));
#116347=CARTESIAN_POINT('Ctrl Pts',(-10.9068322158739,86.315798070468,68.993309732435));
#116348=CARTESIAN_POINT('Ctrl Pts',(-10.9008895022725,86.3533075084191,
69.100900201655));
#116349=CARTESIAN_POINT('Ctrl Pts',(-10.8944278943129,86.3906100147042,
69.2134425579111));
#116350=CARTESIAN_POINT('Ctrl Pts',(-10.8911970903331,86.4092612678467,
69.2697137360391));
#116351=CARTESIAN_POINT('Ctrl Pts',(-10.8878365627587,86.4278602099881,
69.327222722184));
#116352=CARTESIAN_POINT('Ctrl Pts',(-10.8843463115825,86.446354708905,69.3859790953269));
#116353=CARTESIAN_POINT('Ctrl Pts',(-10.8828959388797,86.4540400917119,
69.410395286432));
#116354=CARTESIAN_POINT('Ctrl Pts',(-10.8814231734589,86.4617074161907,
69.4350268841941));
#116355=CARTESIAN_POINT('Ctrl Pts',(-10.8799279934186,86.4693528151707,
69.4598745093374));
#116356=CARTESIAN_POINT('Ctrl Pts',(-10.8796241345346,86.4709065560845,
69.4649241832518));
#116357=CARTESIAN_POINT('Ctrl Pts',(-10.8793193502041,86.4724593912341,
69.4699827791575));
#116358=CARTESIAN_POINT('Ctrl Pts',(-10.8790136421172,86.4740112879634,
69.4750503022557));
#116359=CARTESIAN_POINT('Ctrl Pts',(-10.8781086484231,86.4786053985345,
69.4900517910762));
#116360=CARTESIAN_POINT('Ctrl Pts',(-10.8771955470043,86.483191286066,69.5051315140166));
#116361=CARTESIAN_POINT('Ctrl Pts',(-10.8762743378606,86.4877680971712,
69.5202896029158));
#116362=CARTESIAN_POINT('Ctrl Pts',(-10.8758137332888,86.4900565027238,
69.5278686473654));
#116363=CARTESIAN_POINT('Ctrl Pts',(-10.8753511017858,86.4923426390575,
69.5354672833387));
#116364=CARTESIAN_POINT('Ctrl Pts',(-10.8748864433516,86.4946263986312,
69.5430855268734));
#116365=CARTESIAN_POINT('Ctrl Pts',(-10.8744217849174,86.4969101582049,
69.550703770408));
#116366=CARTESIAN_POINT('Ctrl Pts',(-10.8738819795741,86.4995470533043,
69.5595362016483));
#116367=CARTESIAN_POINT('Ctrl Pts',(-10.8734863872555,86.5014704390232,
69.5659990961329));
#116368=CARTESIAN_POINT('Ctrl Pts',(-10.861496809166,86.5597642485571,69.7618759483011));
#116369=CARTESIAN_POINT('Ctrl Pts',(-10.8494413886398,86.6130533604805,
69.9592421054953));
#116370=CARTESIAN_POINT('Ctrl Pts',(-10.8373200119521,86.6612678630307,
70.1578404613565));
#116371=CARTESIAN_POINT('Ctrl Pts',(-10.8366432775534,86.663959670507,70.1689281737838));
#116372=CARTESIAN_POINT('Ctrl Pts',(-10.8359663362774,86.6666356621964,
70.1800197255885));
#116373=CARTESIAN_POINT('Ctrl Pts',(-10.8352891930952,86.6692958268583,
70.19111506744));
#116374=CARTESIAN_POINT('Ctrl Pts',(-10.8288862721828,86.6944497741948,
70.2960302437859));
#116375=CARTESIAN_POINT('Ctrl Pts',(-10.8224649904436,86.718188651506,70.4012846876382));
#116376=CARTESIAN_POINT('Ctrl Pts',(-10.8160253477116,86.7405039769241,
70.5068400814735));
#116377=CARTESIAN_POINT('Ctrl Pts',(-10.8126527026787,86.7521912202326,
70.5621227872892));
#116378=CARTESIAN_POINT('Ctrl Pts',(-10.8092384943889,86.7636043511571,
70.6180593279552));
#116379=CARTESIAN_POINT('Ctrl Pts',(-10.8058408027958,86.7745539441851,
70.6737478244563));
#116380=CARTESIAN_POINT('Ctrl Pts',(-10.8027510283912,86.7845112258722,
70.7243895282146));
#116381=CARTESIAN_POINT('Ctrl Pts',(-10.799675022111,86.7940858244824,70.7748258842997));
#116382=CARTESIAN_POINT('Ctrl Pts',(-10.7966513366151,86.8031715694856,
70.8243706394832));
#116383=CARTESIAN_POINT('Ctrl Pts',(-10.795628375841,86.8062454211655,70.8411324161896));
#116384=CARTESIAN_POINT('Ctrl Pts',(-10.7946164566296,86.8092803959527,
70.857883432425));
#116385=CARTESIAN_POINT('Ctrl Pts',(-10.7936156928137,86.8122766857533,
70.8746235236739));
#116386=CARTESIAN_POINT('Ctrl Pts',(-10.7832031496532,86.8434518705211,
71.0487974095269));
#116387=CARTESIAN_POINT('Ctrl Pts',(-10.7740019632466,86.8704392100341,
71.2217865823219));
#116388=CARTESIAN_POINT('Ctrl Pts',(-10.766068932557,86.8934600952167,71.3933899853205));
#116389=CARTESIAN_POINT('Ctrl Pts',(-10.7630545361072,86.9022075811753,
71.4585959209859));
#116390=CARTESIAN_POINT('Ctrl Pts',(-10.7602227798109,86.9103823632979,
71.5236020369678));
#116391=CARTESIAN_POINT('Ctrl Pts',(-10.7575751102966,86.9179965202485,
71.5883983800714));
#116392=CARTESIAN_POINT('Ctrl Pts',(-10.7512353234622,86.9362284527947,
71.7435518086617));
#116393=CARTESIAN_POINT('Ctrl Pts',(-10.7459521425721,86.9512463597118,
71.8975006171607));
#116394=CARTESIAN_POINT('Ctrl Pts',(-10.7416545618065,86.9632218800474,
72.0501051761386));
#116395=CARTESIAN_POINT('Ctrl Pts',(-10.7396275911568,86.9688701806982,
72.1220817087337));
#116396=CARTESIAN_POINT('Ctrl Pts',(-10.7378248801488,86.9738416376222,
72.193759898553));
#116397=CARTESIAN_POINT('Ctrl Pts',(-10.7362536744843,86.9781538748905,
72.2651275589387));
#116398=CARTESIAN_POINT('Ctrl Pts',(-10.7334570248527,86.9858293925143,
72.3921576134045));
#116399=CARTESIAN_POINT('Ctrl Pts',(-10.731393790858,86.9914166271671,72.518203273173));
#116400=CARTESIAN_POINT('Ctrl Pts',(-10.7300469114455,86.9950190418003,
72.643195786795));
#116401=CARTESIAN_POINT('Ctrl Pts',(-10.7290772139338,86.9976126314517,
72.7331852307752));
#116402=CARTESIAN_POINT('Ctrl Pts',(-10.7284825825092,86.9991773308193,
72.822629261593));
#116403=CARTESIAN_POINT('Ctrl Pts',(-10.7282633821769,86.9997504820953,
72.9115048423941));
#116404=CARTESIAN_POINT('Ctrl Pts',(-10.7282448252273,86.999799003643,72.9190288258855));
#116405=CARTESIAN_POINT('Ctrl Pts',(-10.7282289586258,86.9998404182714,
72.9265487366744));
#116406=CARTESIAN_POINT('Ctrl Pts',(-10.7282157704445,86.9998747499382,
72.9340645613803));
#116407=CARTESIAN_POINT('Ctrl Pts',(-10.7281312849499,87.0000946838152,
72.9822120771066));
#116408=CARTESIAN_POINT('Ctrl Pts',(-10.7281571517953,87.0000239499403,
73.0301918431451));
#116409=CARTESIAN_POINT('Ctrl Pts',(-10.728293370978,86.9996687874899,73.0780004629468));
#116410=CARTESIAN_POINT('Ctrl Pts',(-10.7283614805694,86.9994912062647,
73.1019047728476));
#116411=CARTESIAN_POINT('Ctrl Pts',(-10.7284571782452,86.9992425162455,
73.1257662963088));
#116412=CARTESIAN_POINT('Ctrl Pts',(-10.7285804640057,86.9989234877188,
73.1495846162313));
#116413=CARTESIAN_POINT('Ctrl Pts',(-10.728642106886,86.9987639734554,73.1614937761926));
#116414=CARTESIAN_POINT('Ctrl Pts',(-10.7287106467875,86.9985868744688,
73.1733921352721));
#116415=CARTESIAN_POINT('Ctrl Pts',(-10.7287860837103,86.9983922864601,
73.1852796422712));
#116416=CARTESIAN_POINT('Ctrl Pts',(-10.7288545066269,86.9982157909377,
73.1960618676091));
#116417=CARTESIAN_POINT('Ctrl Pts',(-10.7289413385066,86.9979921653486,
73.2085723766105));
#116418=CARTESIAN_POINT('Ctrl Pts',(-10.7290119709596,86.9978104599079,
73.2180840633153));
#116419=CARTESIAN_POINT('Ctrl Pts',(-10.7290192114644,86.997791833355,73.219059102563));
#116420=CARTESIAN_POINT('Ctrl Pts',(-10.7290262654236,86.9977736896406,
73.2200026305993));
#116421=CARTESIAN_POINT('Ctrl Pts',(-10.7290330855424,86.9977561506881,
73.2209095561051));
#116422=CARTESIAN_POINT('Ctrl Pts',(-10.7298120572208,86.9957529088541,
73.3244956231166));
#116423=CARTESIAN_POINT('Ctrl Pts',(-10.7312749998046,86.9923257875855,
73.4324657801859));
#116424=CARTESIAN_POINT('Ctrl Pts',(-10.7334586988057,86.9871180640138,
73.544768708703));
#116425=CARTESIAN_POINT('Ctrl Pts',(-10.7357270800446,86.9817083887606,
73.6614266620112));
#116426=CARTESIAN_POINT('Ctrl Pts',(-10.7387751755121,86.9743773859167,
73.7827603223291));
#116427=CARTESIAN_POINT('Ctrl Pts',(-10.7425955242636,86.9646968342411,
73.9086881881113));
#116428=CARTESIAN_POINT('Ctrl Pts',(-10.7453217724827,86.9577886725832,
73.998551873902));
#116429=CARTESIAN_POINT('Ctrl Pts',(-10.7484409799655,86.9496833232534,
74.0907545682361));
#116430=CARTESIAN_POINT('Ctrl Pts',(-10.7519438181274,86.9402147372432,
74.1852559325971));
#116431=CARTESIAN_POINT('Ctrl Pts',(-10.7530457951687,86.9372359629136,
74.2149856343677));
#116432=CARTESIAN_POINT('Ctrl Pts',(-10.7541856980251,86.9341222035809,
74.2449427618101));
#116433=CARTESIAN_POINT('Ctrl Pts',(-10.7553625082042,86.9308681814672,
74.2751259708024));
#116434=CARTESIAN_POINT('Ctrl Pts',(-10.7600481078438,86.9179119332007,
74.3953037494167));
#116435=CARTESIAN_POINT('Ctrl Pts',(-10.7653388979247,86.902733708385,74.519066681511));
#116436=CARTESIAN_POINT('Ctrl Pts',(-10.7712469033839,86.8849886449845,
74.6463126737205));
#116437=CARTESIAN_POINT('Ctrl Pts',(-10.7743570859573,86.8756470173687,
74.7132994546634));
#116438=CARTESIAN_POINT('Ctrl Pts',(-10.777637739596,86.8655937143387,74.7812510227291));
#116439=CARTESIAN_POINT('Ctrl Pts',(-10.7810863610267,86.8547763442664,
74.850148998758));
#116440=CARTESIAN_POINT('Ctrl Pts',(-10.7817163187627,86.8528003413629,
74.8627345532661));
#116441=CARTESIAN_POINT('Ctrl Pts',(-10.7823518727809,86.8507988391756,
74.8753516807464));
#116442=CARTESIAN_POINT('Ctrl Pts',(-10.7829929716454,86.8487715159117,
74.888000270938));
#116443=CARTESIAN_POINT('Ctrl Pts',(-10.7884017017479,86.831667688448,74.9947120658207));
#116444=CARTESIAN_POINT('Ctrl Pts',(-10.794212258259,86.8127265612355,75.103664440251));
#116445=CARTESIAN_POINT('Ctrl Pts',(-10.8004246409436,86.7917515545281,
75.2147801090942));
#116446=CARTESIAN_POINT('Ctrl Pts',(-10.8035308322859,86.7812640511744,
75.2703379435157));
#116447=CARTESIAN_POINT('Ctrl Pts',(-10.806737480238,86.7702679332875,75.3264365751154));
#116448=CARTESIAN_POINT('Ctrl Pts',(-10.8100445847874,86.7587380138097,
75.3830648877445));
#116449=CARTESIAN_POINT('Ctrl Pts',(-10.8116981370622,86.7529730540708,
75.411379044059));
#116450=CARTESIAN_POINT('Ctrl Pts',(-10.8133768034894,86.747074635108,75.4398256190323));
#116451=CARTESIAN_POINT('Ctrl Pts',(-10.8150805840696,86.7410395639213,
75.4684031694774));
#116452=CARTESIAN_POINT('Ctrl Pts',(-10.8159324743596,86.738022028328,75.4826919447));
#116453=CARTESIAN_POINT('Ctrl Pts',(-10.8167906431878,86.7349703291177,
75.4970134636656));
#116454=CARTESIAN_POINT('Ctrl Pts',(-10.8176550905538,86.7318840647869,
75.5113675406235));
#116455=CARTESIAN_POINT('Ctrl Pts',(-10.8179225350347,86.7309292300633,
75.515808434091));
#116456=CARTESIAN_POINT('Ctrl Pts',(-10.8181905804556,86.7299710868356,
75.5202524439623));
#116457=CARTESIAN_POINT('Ctrl Pts',(-10.8184592268714,86.7290096232093,
75.5246995645498));
#116458=CARTESIAN_POINT('Ctrl Pts',(-10.8186247466155,86.7284172415357,
75.527439546245));
#116459=CARTESIAN_POINT('Ctrl Pts',(-10.8187904945019,86.7278235994056,
75.530180708798));
#116460=CARTESIAN_POINT('Ctrl Pts',(-10.8189564705061,86.7272286940407,
75.5329230509585));
#116461=CARTESIAN_POINT('Ctrl Pts',(-10.8193918334579,86.7256682289784,
75.5401163448538));
#116462=CARTESIAN_POINT('Ctrl Pts',(-10.8196988436352,86.7245665827455,
75.545181674583));
#116463=CARTESIAN_POINT('Ctrl Pts',(-10.8202672682649,86.7225211743997,
75.5545272568814));
#116464=CARTESIAN_POINT('Ctrl Pts',(-10.8275417622956,86.6963447738284,
75.6741286588835));
#116465=CARTESIAN_POINT('Ctrl Pts',(-10.8345942233826,86.6691746593892,
75.7895144494221));
#116466=CARTESIAN_POINT('Ctrl Pts',(-10.8413435140449,86.641359333253,75.9007191351649));
#116467=CARTESIAN_POINT('Ctrl Pts',(-10.8473523085855,86.6165957561314,
75.9997230367618));
#116468=CARTESIAN_POINT('Ctrl Pts',(-10.8531217396086,86.5913204207394,
76.0954131499708));
#116469=CARTESIAN_POINT('Ctrl Pts',(-10.8586241561333,86.5657622751962,
76.1878199247765));
#116470=CARTESIAN_POINT('Ctrl Pts',(-10.8652247671061,86.5351031320437,
76.2986696158165));
#116471=CARTESIAN_POINT('Ctrl Pts',(-10.8714407767674,86.5040378671458,
76.4047944775482));
#116472=CARTESIAN_POINT('Ctrl Pts',(-10.8772777948961,86.4729322436842,
76.5062569106158));
#116473=CARTESIAN_POINT('Ctrl Pts',(-10.8833283429498,86.4406887136234,
76.6114310446336));
#116474=CARTESIAN_POINT('Ctrl Pts',(-10.8889720238455,86.4084019813046,
76.7115955374519));
#116475=CARTESIAN_POINT('Ctrl Pts',(-10.8942558342815,86.376442466493,76.8068279872566));
#116476=CARTESIAN_POINT('Ctrl Pts',(-10.8952324396605,86.3705353972565,
76.824429777455));
#116477=CARTESIAN_POINT('Ctrl Pts',(-10.896196850492,86.3646394044195,76.8418630967093));
#116478=CARTESIAN_POINT('Ctrl Pts',(-10.8971494929465,86.3587566888011,
76.8591284569882));
#116479=CARTESIAN_POINT('Ctrl Pts',(-10.9005529294257,86.3377399381437,
76.920811155172));
#116480=CARTESIAN_POINT('Ctrl Pts',(-10.9038058355024,86.3168931915867,
76.9803500170193));
#116481=CARTESIAN_POINT('Ctrl Pts',(-10.9069337564245,86.2963127364398,
77.0377685506294));
#116482=CARTESIAN_POINT('Ctrl Pts',(-10.9120682687526,86.2625297210428,
77.1320216267242));
#116483=CARTESIAN_POINT('Ctrl Pts',(-10.9167765779744,86.2294653974887,
77.2205664752667));
#116484=CARTESIAN_POINT('Ctrl Pts',(-10.9210486754665,86.197501551463,77.3035187659328));
#116485=CARTESIAN_POINT('Ctrl Pts',(-10.9252227188449,86.1662713466046,
77.3845671175261));
#116486=CARTESIAN_POINT('Ctrl Pts',(-10.9289809732627,86.1360914017084,
77.4602769639134));
#116487=CARTESIAN_POINT('Ctrl Pts',(-10.9323304910036,86.1072728402612,
77.5307522283811));
#116488=CARTESIAN_POINT('Ctrl Pts',(-10.9326964170239,86.1041244880745,
77.53845146602));
#116489=CARTESIAN_POINT('Ctrl Pts',(-10.9330574760382,86.1009923411827,
77.5460882227403));
#116490=CARTESIAN_POINT('Ctrl Pts',(-10.93341369061,86.0978767752278,77.5536626280678));
#116491=CARTESIAN_POINT('Ctrl Pts',(-10.936890719826,86.067465571677,77.6275967978205));
#116492=CARTESIAN_POINT('Ctrl Pts',(-10.9398996029891,86.0386383539991,
77.6955923112921));
#116493=CARTESIAN_POINT('Ctrl Pts',(-10.9424403395056,86.0117111061841,
77.7577689141376));
#116494=CARTESIAN_POINT('Ctrl Pts',(-10.9437107077639,85.9982474822766,
77.7888572155604));
#116495=CARTESIAN_POINT('Ctrl Pts',(-10.9448640393378,85.9852579622718,
77.8184906332928));
#116496=CARTESIAN_POINT('Ctrl Pts',(-10.9459003341546,85.9727768087027,
77.8466830224824));
#116497=CARTESIAN_POINT('Ctrl Pts',(-10.9464184815629,85.9665362319182,
77.8607792170771));
#116498=CARTESIAN_POINT('Ctrl Pts',(-10.9469073697786,85.9604226970262,
77.8745151324323));
#116499=CARTESIAN_POINT('Ctrl Pts',(-10.9473669988077,85.9544401629786,
77.8878924275129));
#116500=CARTESIAN_POINT('Ctrl Pts',(-10.9475968133222,85.9514488959548,
77.8945810750531));
#116501=CARTESIAN_POINT('Ctrl Pts',(-10.9478193130394,85.9484903760411,
77.9011800661612));
#116502=CARTESIAN_POINT('Ctrl Pts',(-10.9480344979591,85.9455650791476,
77.9076896009303));
#116503=CARTESIAN_POINT('Ctrl Pts',(-10.948142090419,85.9441024307008,77.9109443683149));
#116504=CARTESIAN_POINT('Ctrl Pts',(-10.9482478541794,85.9426480878169,
77.9141767715282));
#116505=CARTESIAN_POINT('Ctrl Pts',(-10.9483517892405,85.9412021087518,
77.9173868352419));
#116506=CARTESIAN_POINT('Ctrl Pts',(-10.9484037567711,85.9404791192192,
77.9189918670988));
#116507=CARTESIAN_POINT('Ctrl Pts',(-10.9484552671268,85.9397582206293,
77.9205913140754));
#116508=CARTESIAN_POINT('Ctrl Pts',(-10.9485063203077,85.9390394201873,
77.922185179234));
#116509=CARTESIAN_POINT('Ctrl Pts',(-10.9485573734885,85.9383206197453,
77.9237790443926));
#116510=CARTESIAN_POINT('Ctrl Pts',(-10.948568260266,85.9381698679242,77.9241138486253));
#116511=CARTESIAN_POINT('Ctrl Pts',(-10.9486581083257,85.9368893204608,
77.9269500323));
#116512=CARTESIAN_POINT('Ctrl Pts',(-10.951395910894,85.8978691552357,78.0133727216242));
#116513=CARTESIAN_POINT('Ctrl Pts',(-10.9537314325388,85.8582240439881,
78.0984489820115));
#116514=CARTESIAN_POINT('Ctrl Pts',(-10.9556525073569,85.8180244885345,
78.1821875838237));
#116515=CARTESIAN_POINT('Ctrl Pts',(-10.9591130519213,85.7456106752817,
78.3330308308512));
#116516=CARTESIAN_POINT('Ctrl Pts',(-10.9612268328035,85.6713997206963,
78.4795321797455));
#116517=CARTESIAN_POINT('Ctrl Pts',(-10.9619612599143,85.5957953551927,
78.621749827295));
#116518=CARTESIAN_POINT('Ctrl Pts',(-10.9622618887243,85.5648476272331,
78.679964892498));
#116519=CARTESIAN_POINT('Ctrl Pts',(-10.9623318059689,85.5336660407217,
78.737462455626));
#116520=CARTESIAN_POINT('Ctrl Pts',(-10.9621704102873,85.5022767295138,
78.7942475578633));
#116521=CARTESIAN_POINT('Ctrl Pts',(-10.9617720353596,85.4247981101503,
78.9344109176964));
#116522=CARTESIAN_POINT('Ctrl Pts',(-10.9599623479946,85.3460566132439,
79.0702318537373));
#116523=CARTESIAN_POINT('Ctrl Pts',(-10.9567596072908,85.2664470382299,
79.2017831826618));
#116524=CARTESIAN_POINT('Ctrl Pts',(-10.9555382395348,85.2360878624529,
79.251950388275));
#116525=CARTESIAN_POINT('Ctrl Pts',(-10.9541145859146,85.2056020553527,
79.3014969164829));
#116526=CARTESIAN_POINT('Ctrl Pts',(-10.9524907355255,85.1750101072347,
79.3504276719218));
#116527=CARTESIAN_POINT('Ctrl Pts',(-10.9482417584689,85.0949630249782,
79.4784601917986));
#116528=CARTESIAN_POINT('Ctrl Pts',(-10.942619355958,85.0141917592843,79.6022756610076));
#116529=CARTESIAN_POINT('Ctrl Pts',(-10.9356304201028,84.9330452710067,
79.721987764502));
#116530=CARTESIAN_POINT('Ctrl Pts',(-10.9335818511937,84.9092599371,79.7570772972067));
#116531=CARTESIAN_POINT('Ctrl Pts',(-10.931416110014,84.8854421357569,79.7918143835424));
#116532=CARTESIAN_POINT('Ctrl Pts',(-10.9291339382821,84.8616000941366,
79.8262021308764));
#116533=CARTESIAN_POINT('Ctrl Pts',(-10.9286955685532,84.8570204084039,
79.8328074828154));
#116534=CARTESIAN_POINT('Ctrl Pts',(-10.9282527382848,84.8524398377061,
79.8393999309981));
#116535=CARTESIAN_POINT('Ctrl Pts',(-10.9278054549261,84.8478584363307,
79.8459795023192));
#116536=CARTESIAN_POINT('Ctrl Pts',(-10.9200712462639,84.7686390477297,
79.9597502843571));
#116537=CARTESIAN_POINT('Ctrl Pts',(-10.9110030852049,84.6891747323319,
80.0696694873031));
#116538=CARTESIAN_POINT('Ctrl Pts',(-10.9006326689777,84.6097646350222,
80.175850627459));
#116539=CARTESIAN_POINT('Ctrl Pts',(-10.8970713501343,84.5824943047176,
80.2123144382621));
#116540=CARTESIAN_POINT('Ctrl Pts',(-10.8933567088875,84.5552300138256,
80.2483375603649));
#116541=CARTESIAN_POINT('Ctrl Pts',(-10.8894907894036,84.5279827932135,
80.2839250246018));
#116542=CARTESIAN_POINT('Ctrl Pts',(-10.8786864366559,84.4518330999468,
80.3833837739681));
#116543=CARTESIAN_POINT('Ctrl Pts',(-10.866697330589,84.3758192380347,80.4794390140921));
#116544=CARTESIAN_POINT('Ctrl Pts',(-10.8535044037148,84.3001723967285,
80.5722125416248));
#116545=CARTESIAN_POINT('Ctrl Pts',(-10.8489469098624,84.2740402110887,
80.6042611374695));
#116546=CARTESIAN_POINT('Ctrl Pts',(-10.844246106719,84.2479515284257,80.635918193433));
#116547=CARTESIAN_POINT('Ctrl Pts',(-10.8394022657455,84.2219149668464,
80.6671889838823));
#116548=CARTESIAN_POINT('Ctrl Pts',(-10.8255735235187,84.1475828612858,
80.7564643549623));
#116549=CARTESIAN_POINT('Ctrl Pts',(-10.8105760714285,84.0736782582328,
80.8425905963213));
#116550=CARTESIAN_POINT('Ctrl Pts',(-10.7944085851747,84.0004093351753,
80.9256789089337));
#116551=CARTESIAN_POINT('Ctrl Pts',(-10.7896138356913,83.978680160617,80.9503201943951));
#116552=CARTESIAN_POINT('Ctrl Pts',(-10.7847164308873,83.9570066589367,
80.9746943605333));
#116553=CARTESIAN_POINT('Ctrl Pts',(-10.7797169475032,83.9353936757825,
80.9988044841311));
#116554=CARTESIAN_POINT('Ctrl Pts',(-10.7649032283752,83.8713533265372,
81.0702439853112));
#116555=CARTESIAN_POINT('Ctrl Pts',(-10.7491908635468,83.8078463452034,
81.1393644748102));
#116556=CARTESIAN_POINT('Ctrl Pts',(-10.7325548086161,83.7450174768963,
81.2062284540156));
#116557=CARTESIAN_POINT('',(-10.0948776383655,81.4411710637376,83.1136760388969));
#116558=CARTESIAN_POINT('Ctrl Pts',(-10.7325548086179,83.7450177191935,
81.2062286816919));
#116559=CARTESIAN_POINT('Ctrl Pts',(-10.7094056412749,83.6576110466643,
81.2992481947719));
#116560=CARTESIAN_POINT('Ctrl Pts',(-10.6857306659004,83.5690067944165,
81.3905677640237));
#116561=CARTESIAN_POINT('Ctrl Pts',(-10.6615694462013,83.4792858039514,
81.4801620977175));
#116562=CARTESIAN_POINT('Ctrl Pts',(-10.6374082265022,83.3895648134863,
81.5697564314113));
#116563=CARTESIAN_POINT('Ctrl Pts',(-10.6127607624786,83.2987275812377,
81.657626026861));
#116564=CARTESIAN_POINT('Ctrl Pts',(-10.5876490343607,83.2068057061495,
81.7437931611233));
#116565=CARTESIAN_POINT('Ctrl Pts',(-10.5625373062429,83.1148838310612,
81.8299602953855));
#116566=CARTESIAN_POINT('Ctrl Pts',(-10.5369613140309,83.0218771946117,
81.9144248336993));
#116567=CARTESIAN_POINT('Ctrl Pts',(-10.5109555987824,82.9278254887252,
81.997195721309));
#116568=CARTESIAN_POINT('Ctrl Pts',(-10.4849498835339,82.8337737828386,
82.0799666089187));
#116569=CARTESIAN_POINT('Ctrl Pts',(-10.4585144452489,82.7386771162062,
82.1610439757537));
#116570=CARTESIAN_POINT('Ctrl Pts',(-10.4316882718126,82.6425589685798,
82.2404456022542));
#116571=CARTESIAN_POINT('Ctrl Pts',(-10.4048620983762,82.5464408209533,
82.3198472287548));
#116572=CARTESIAN_POINT('Ctrl Pts',(-10.3776451897886,82.4493012237793,
82.3975731462497));
#116573=CARTESIAN_POINT('Ctrl Pts',(-10.3500918160521,82.351155775502,82.4736407678395));
#116574=CARTESIAN_POINT('Ctrl Pts',(-10.3225384423156,82.2530103272247,
82.5497083894292));
#116575=CARTESIAN_POINT('Ctrl Pts',(-10.2946486034302,82.1538589465135,
82.6241176161567));
#116576=CARTESIAN_POINT('Ctrl Pts',(-10.2664905900852,82.0537231169019,
82.6968752842873));
#116577=CARTESIAN_POINT('Ctrl Pts',(-10.2383325767402,81.9535872872904,
82.7696329524178));
#116578=CARTESIAN_POINT('Ctrl Pts',(-10.2099063889356,81.8524671189661,
82.8407392030616));
#116579=CARTESIAN_POINT('Ctrl Pts',(-10.181277888407,81.7503663349919,82.9102075622766));
#116580=CARTESIAN_POINT('Ctrl Pts',(-10.1526494167491,81.6482656539822,
82.9796758514356));
#116581=CARTESIAN_POINT('Ctrl Pts',(-10.1238186327753,81.5451840202451,
83.0475057597329));
#116582=CARTESIAN_POINT('Ctrl Pts',(-10.0948776413094,81.4411712996156,
83.1136764109577));
#116583=CARTESIAN_POINT('Ctrl Pts',(-10.0948775537519,81.44117080392,83.11367632661));
#116584=CARTESIAN_POINT('Ctrl Pts',(-10.0503152587603,81.2811042916383,
83.2155075847456));
#116585=CARTESIAN_POINT('Ctrl Pts',(-9.99904314712063,81.1049072372153,
83.3223055647842));
#116586=CARTESIAN_POINT('Ctrl Pts',(-9.912070254689,80.8148282663644,83.4865137751945));
#116587=CARTESIAN_POINT('Ctrl Pts',(-9.88140183638311,80.7138382560085,
83.5419112301925));
#116588=CARTESIAN_POINT('Ctrl Pts',(-9.83288302768125,80.5557177866961,
83.625503240927));
#116589=CARTESIAN_POINT('Ctrl Pts',(-9.80799457801955,80.4749988320776,
83.6674224966469));
#116590=CARTESIAN_POINT('Ctrl Pts',(-9.77785722412043,80.377884338857,83.7164278765081));
#116591=CARTESIAN_POINT('Ctrl Pts',(-9.7625133398474,80.3285867257644,83.7409403779417));
#116592=CARTESIAN_POINT('Ctrl Pts',(-9.75477259588003,80.3037522380146,
83.7531971798874));
#116593=CARTESIAN_POINT('Ctrl Pts',(-9.75144039093026,80.2930690347116,
83.7584500077144));
#116594=CARTESIAN_POINT('Ctrl Pts',(-9.74921564468608,80.28593803639,83.7619518506129));
#116595=CARTESIAN_POINT('Ctrl Pts',(-9.74760337617057,80.2807717678712,
83.76448470132));
#116596=CARTESIAN_POINT('Ctrl Pts',(-9.72722943538018,80.2154968625108,
83.7964589701507));
#116597=CARTESIAN_POINT('Ctrl Pts',(-9.69987038258628,80.1283934374761,
83.8385299499183));
#116598=CARTESIAN_POINT('Ctrl Pts',(-9.64742804717243,79.9608419184596,
83.9156376385006));
#116599=CARTESIAN_POINT('Ctrl Pts',(-9.62804664266397,79.8988361406045,
83.9436586549674));
#116600=CARTESIAN_POINT('Ctrl Pts',(-9.59612359684555,79.7964020015627,
83.98870389199));
#116601=CARTESIAN_POINT('Ctrl Pts',(-9.57944933917239,79.7428281743368,
84.0119784579149));
#116602=CARTESIAN_POINT('Ctrl Pts',(-9.56170597935333,79.6856801076756,
84.0362803711258));
#116603=CARTESIAN_POINT('Ctrl Pts',(-9.54963949455265,79.6467826136689,
84.052697816691));
#116604=CARTESIAN_POINT('Ctrl Pts',(-9.54307101057707,79.6255896711592,
84.0615737659991));
#116605=CARTESIAN_POINT('Ctrl Pts',(-9.49038169671332,79.4554449164131,
84.1323106572381));
#116606=CARTESIAN_POINT('Ctrl Pts',(-9.44836711016332,79.3176255198826,
84.1860108422029));
#116607=CARTESIAN_POINT('Ctrl Pts',(-9.39257576899831,79.1321384223008,
84.2552014191141));
#116608=CARTESIAN_POINT('Ctrl Pts',(-9.37518374505331,79.0738455902002,
84.2763669865997));
#116609=CARTESIAN_POINT('Ctrl Pts',(-9.3509033438008,78.9918160771606,84.305525217164));
#116610=CARTESIAN_POINT('Ctrl Pts',(-9.33921505184079,78.9521534352811,
84.3194563301342));
#116611=CARTESIAN_POINT('Ctrl Pts',(-9.32636955138672,78.9082664269095,
84.3346264026876));
#116612=CARTESIAN_POINT('Ctrl Pts',(-9.32014451120116,78.8869217029075,
84.3419467200815));
#116613=CARTESIAN_POINT('Ctrl Pts',(-9.31751900327339,78.8779025117332,
84.3450279074121));
#116614=CARTESIAN_POINT('Ctrl Pts',(-9.31577807941876,78.8719183095939,
84.3470696368959));
#116615=CARTESIAN_POINT('Ctrl Pts',(-9.31544178421389,78.8707627633681,
84.347464173305));
#116616=CARTESIAN_POINT('Ctrl Pts',(-9.26955506958364,78.7128328443911,
84.4012091119334));
#116617=CARTESIAN_POINT('Ctrl Pts',(-9.22873679430673,78.5675302623779,
84.4472128255647));
#116618=CARTESIAN_POINT('Ctrl Pts',(-9.17302628066541,78.3619860064613,
84.5085318351849));
#116619=CARTESIAN_POINT('Ctrl Pts',(-9.14655024866327,78.2623134976708,
84.5372674497077));
#116620=CARTESIAN_POINT('Ctrl Pts',(-9.11807518809318,78.1515678237594,
84.567724741971));
#116621=CARTESIAN_POINT('Ctrl Pts',(-9.10444106866622,78.0975922362132,
84.5822219191351));
#116622=CARTESIAN_POINT('Ctrl Pts',(-9.09777486166728,78.0709552791927,
84.5892920098368));
#116623=CARTESIAN_POINT('Ctrl Pts',(-9.09495024139227,78.0596147781854,
84.5922842614441));
#116624=CARTESIAN_POINT('Ctrl Pts',(-9.09307434467153,78.05207120322,84.5942707496973));
#116625=CARTESIAN_POINT('Ctrl Pts',(-9.09244053606258,78.0495203074527,
84.594941784726));
#116626=CARTESIAN_POINT('Ctrl Pts',(-9.05180720977179,77.885591750876,84.6379394466845));
#116627=CARTESIAN_POINT('Ctrl Pts',(-9.01546474124791,77.7288171154016,
84.6755714490163));
#116628=CARTESIAN_POINT('Ctrl Pts',(-8.96554035573562,77.4972590772881,
84.7264335172893));
#116629=CARTESIAN_POINT('Ctrl Pts',(-8.94172549229785,77.3823802815235,
84.7504680239201));
#116630=CARTESIAN_POINT('Ctrl Pts',(-8.91594931126095,77.2499936291791,
84.7761747632328));
#116631=CARTESIAN_POINT('Ctrl Pts',(-8.90356317731929,77.1842173036598,
84.7884584738757));
#116632=CARTESIAN_POINT('Ctrl Pts',(-8.89836239632504,77.1561175822305,
84.7936023187275));
#116633=CARTESIAN_POINT('Ctrl Pts',(-8.89491911168967,77.1374045486816,
84.7970049108324));
#116634=CARTESIAN_POINT('Ctrl Pts',(-8.89357005880115,77.1300413420178,
84.7983371356429));
#116635=CARTESIAN_POINT('Ctrl Pts',(-8.75977550793369,76.3942664536245,
84.9303191121072));
#116636=CARTESIAN_POINT('Ctrl Pts',(-8.69370887000654,75.6839064820694,
84.98888938658));
#116637=CARTESIAN_POINT('Ctrl Pts',(-8.69331176731091,75.00000000541,84.98885921934));
#116638=CARTESIAN_POINT('Origin',(27.4324635166691,25.,72.98888938658));
#116639=CARTESIAN_POINT('',(-7.08826202869291,64.825987357,58.34040756172));
#116640=CARTESIAN_POINT('',(-10.067463384623,56.310682064485,72.9888891145402));
#116641=CARTESIAN_POINT('Ctrl Pts',(-7.08826202869291,64.825987357,58.34040756172));
#116642=CARTESIAN_POINT('Ctrl Pts',(-7.24267999369472,64.1486336869958,
58.7046006729965));
#116643=CARTESIAN_POINT('Ctrl Pts',(-7.40664860408434,63.505158727736,59.1068827930799));
#116644=CARTESIAN_POINT('Ctrl Pts',(-7.66100278224209,62.5907643549632,
59.7694119675106));
#116645=CARTESIAN_POINT('Ctrl Pts',(-7.74717579931205,62.2944359083917,
60.0001063446241));
#116646=CARTESIAN_POINT('Ctrl Pts',(-7.87768758671566,61.8626477550637,
60.3611577658764));
#116647=CARTESIAN_POINT('Ctrl Pts',(-7.9432553932647,61.649929807532,60.5454358170881));
#116648=CARTESIAN_POINT('Ctrl Pts',(-8.00912491301031,61.4419760536987,
60.7353844945309));
#116649=CARTESIAN_POINT('Ctrl Pts',(-8.05308578013046,61.3043989275207,
60.8632816219083));
#116650=CARTESIAN_POINT('Ctrl Pts',(-8.07558635098398,61.2346134642867,
60.9293321247506));
#116651=CARTESIAN_POINT('Ctrl Pts',(-8.26928846854225,60.6387810788844,
61.5030451637313));
#116652=CARTESIAN_POINT('Ctrl Pts',(-8.43901295569384,60.1518492983687,
62.041887135517));
#116653=CARTESIAN_POINT('Ctrl Pts',(-8.68450790024914,59.4854971373579,
62.8942474257412));
#116654=CARTESIAN_POINT('Ctrl Pts',(-8.76481806882766,59.2740540019814,
63.1857138175993));
#116655=CARTESIAN_POINT('Ctrl Pts',(-8.92142008072934,58.8725162344827,
63.7834240098156));
#116656=CARTESIAN_POINT('Ctrl Pts',(-8.99797239407982,58.6817880507017,
64.0907755449453));
#116657=CARTESIAN_POINT('Ctrl Pts',(-9.2185027435778,58.1454275641928,65.0284224069521));
#116658=CARTESIAN_POINT('Ctrl Pts',(-9.35433664401844,57.830887894101,65.677944992921));
#116659=CARTESIAN_POINT('Ctrl Pts',(-9.53607045987608,57.4236293703346,
66.68852121302));
#116660=CARTESIAN_POINT('Ctrl Pts',(-9.59297517919348,57.2986350259743,
67.0314238232507));
#116661=CARTESIAN_POINT('Ctrl Pts',(-9.6721357626539,57.1272812547768,67.55475293626));
#116662=CARTESIAN_POINT('Ctrl Pts',(-9.71016660933379,57.0456388055137,
67.8186607659407));
#116663=CARTESIAN_POINT('Ctrl Pts',(-9.74574171923844,56.9700480107542,
68.0859115726082));
#116664=CARTESIAN_POINT('Ctrl Pts',(-9.76889793333612,56.9209989596931,
68.2648188670356));
#116665=CARTESIAN_POINT('Ctrl Pts',(-9.78005219265401,56.8974491471374,
68.3534662981843));
#116666=CARTESIAN_POINT('Ctrl Pts',(-9.96966609619479,56.4982548013989,
69.9067322790409));
#116667=CARTESIAN_POINT('Ctrl Pts',(-10.0675364833309,56.3104931139281,
71.424806576562));
#116668=CARTESIAN_POINT('Ctrl Pts',(-10.0674651278229,56.31068206442,72.9888891141279));
#116669=CARTESIAN_POINT('',(-7.0883818064374,64.8259873343748,87.637422020082));
#116670=CARTESIAN_POINT('Ctrl Pts',(-10.0674651278229,56.31068206442,72.9888891141279));
#116671=CARTESIAN_POINT('Ctrl Pts',(-10.0675364833309,56.3105869691024,
73.724381242214));
#116672=CARTESIAN_POINT('Ctrl Pts',(-10.045894923569,56.3529537458112,74.4525676988862));
#116673=CARTESIAN_POINT('Ctrl Pts',(-9.98293498174587,56.4801967189142,
75.5320924062045));
#116674=CARTESIAN_POINT('Ctrl Pts',(-9.94383162901423,56.5597414074757,
76.0686695361057));
#116675=CARTESIAN_POINT('Ctrl Pts',(-9.88530911783133,56.680409147648,76.6887457170077));
#116676=CARTESIAN_POINT('Ctrl Pts',(-9.8528778023235,56.7477094186136,76.997259346543));
#116677=CARTESIAN_POINT('Ctrl Pts',(-9.83587656653315,56.7831011543162,
77.1511298884427));
#116678=CARTESIAN_POINT('Ctrl Pts',(-9.82842272910424,56.798642241093,77.2169910887884));
#116679=CARTESIAN_POINT('Ctrl Pts',(-9.8234163439587,56.8090858989546,77.2608799805709));
#116680=CARTESIAN_POINT('Ctrl Pts',(-9.82103027562739,56.8140658122574,
77.2816438526153));
#116681=CARTESIAN_POINT('Ctrl Pts',(-9.73272175794122,56.9984745832181,
78.0438490465314));
#116682=CARTESIAN_POINT('Ctrl Pts',(-9.62773423677328,57.2214589055245,
78.7577383351392));
#116683=CARTESIAN_POINT('Ctrl Pts',(-9.44733341207722,57.6221809328644,
79.7898119286563));
#116684=CARTESIAN_POINT('Ctrl Pts',(-9.38337611636343,57.7667958659578,
80.1273831484367));
#116685=CARTESIAN_POINT('Ctrl Pts',(-9.28243301353116,58.0002796515679,
80.6239996048413));
#116686=CARTESIAN_POINT('Ctrl Pts',(-9.2307092849391,58.1211618908655,80.8698732871114));
#116687=CARTESIAN_POINT('Ctrl Pts',(-9.17724028826713,58.2482546499019,
81.1120885623046));
#116688=CARTESIAN_POINT('Ctrl Pts',(-9.14122097838372,58.3343632714237,
81.272752011587));
#116689=CARTESIAN_POINT('Ctrl Pts',(-9.12343746339077,58.3771094829852,
81.350890758788));
#116690=CARTESIAN_POINT('Ctrl Pts',(-9.02949491806345,58.6042723990177,
81.7574127347759));
#116691=CARTESIAN_POINT('Ctrl Pts',(-8.95228473824977,58.7944286240105,
82.0717518718014));
#116692=CARTESIAN_POINT('Ctrl Pts',(-8.83457068817163,59.0923017997501,
82.5270655282608));
#116693=CARTESIAN_POINT('Ctrl Pts',(-8.77523768283496,59.2443980971824,
82.7506742777178));
#116694=CARTESIAN_POINT('Ctrl Pts',(-8.71540134802023,59.4012339589587,
82.9682394673107));
#116695=CARTESIAN_POINT('Ctrl Pts',(-8.67542120793468,59.5068444366637,
83.1119434230033));
#116696=CARTESIAN_POINT('Ctrl Pts',(-8.65577194947727,59.5591419591804,
83.181771430353));
#116697=CARTESIAN_POINT('Ctrl Pts',(-8.55350454907456,59.8336060090282,
83.5411136575106));
#116698=CARTESIAN_POINT('Ctrl Pts',(-8.4695959972588,60.0660422041825,83.8228958350763));
#116699=CARTESIAN_POINT('Ctrl Pts',(-8.34112301080695,60.4339939298278,
84.2370625817306));
#116700=CARTESIAN_POINT('Ctrl Pts',(-8.29786343947522,60.559860743862,84.3737006135942));
#116701=CARTESIAN_POINT('Ctrl Pts',(-8.21055983276111,60.8180268495683,
84.6441490396162));
#116702=CARTESIAN_POINT('Ctrl Pts',(-8.16692619209731,60.9490733898373,
84.7767354767832));
#116703=CARTESIAN_POINT('Ctrl Pts',(-7.7636854370743,62.1799879268859,85.9793603608846));
#116704=CARTESIAN_POINT('Ctrl Pts',(-7.40740356864993,63.426703148092,86.8849892493009));
#116705=CARTESIAN_POINT('Ctrl Pts',(-7.08824925985691,64.82598733535,87.63736578702));
#116706=CARTESIAN_POINT('',(-7.08815755253877,22.5,87.6373268799153));
#116707=CARTESIAN_POINT('',(-7.08815755536701,25.,87.6373268732506));
#116708=CARTESIAN_POINT('',(-8.23395173885291,22.5,84.57149802283));
#116709=CARTESIAN_POINT('Origin',(27.4324635166691,22.5,72.98888938658));
#116710=CARTESIAN_POINT('',(-8.23395173818611,10.,84.5714980248862));
#116711=CARTESIAN_POINT('',(-8.23395173885291,22.5,84.57149802283));
#116712=CARTESIAN_POINT('',(-7.08815755056573,10.,58.340451888595));
#116713=CARTESIAN_POINT('Origin',(27.4324635166691,10.,72.98888938658));
#116714=CARTESIAN_POINT('',(-7.08815755142092,25.,58.34045189061));
#116715=CARTESIAN_POINT('Origin',(6.43246351666909,-92.5,72.98888938658));
#116716=CARTESIAN_POINT('',(14.9324629260191,25.5800360490065,72.98888938658));
#116717=CARTESIAN_POINT('',(14.2241913549675,25.6803058095512,69.5919860434059));
#116718=CARTESIAN_POINT('Ctrl Pts',(14.9324629260191,25.5800360490065,72.98888938658));
#116719=CARTESIAN_POINT('Ctrl Pts',(14.9324626931148,25.556144234287,72.8429202738032));
#116720=CARTESIAN_POINT('Ctrl Pts',(14.9228631443724,25.5035388027324,72.4703017419395));
#116721=CARTESIAN_POINT('Ctrl Pts',(14.8679915267049,25.4553343707258,71.8723531717214));
#116722=CARTESIAN_POINT('Ctrl Pts',(14.7503488053081,25.4533873314043,71.1936658431954));
#116723=CARTESIAN_POINT('Ctrl Pts',(14.572743094615,25.5073301307937,70.5070039054373));
#116724=CARTESIAN_POINT('Ctrl Pts',(14.3852859030436,25.5948194038957,69.973693869023));
#116725=CARTESIAN_POINT('Ctrl Pts',(14.2575749161567,25.6622795837767,69.6685609430364));
#116726=CARTESIAN_POINT('Ctrl Pts',(14.2241960818191,25.68030397154,69.591995772582));
#116727=CARTESIAN_POINT('',(14.2241493853463,26.6269447605316,76.3858806723372));
#116728=CARTESIAN_POINT('Ctrl Pts',(14.2241515060895,26.6269447605405,76.3858815969566));
#116729=CARTESIAN_POINT('Ctrl Pts',(14.301420357292,26.5533368797724,76.2086481732271));
#116730=CARTESIAN_POINT('Ctrl Pts',(14.3723588782976,26.4805897804971,76.0294311309084));
#116731=CARTESIAN_POINT('Ctrl Pts',(14.4369615507881,26.4097165788527,75.8486116146905));
#116732=CARTESIAN_POINT('Ctrl Pts',(14.5194755009863,26.3191935771651,75.6176593648704));
#116733=CARTESIAN_POINT('Ctrl Pts',(14.5916532948012,26.2317276051259,75.3840929064488));
#116734=CARTESIAN_POINT('Ctrl Pts',(14.6535466657325,26.149138675707,75.148470794251));
#116735=CARTESIAN_POINT('Ctrl Pts',(14.7063523690853,26.0786760972192,74.9474445587614));
#116736=CARTESIAN_POINT('Ctrl Pts',(14.7516720122209,26.0117635317123,74.7449220071315));
#116737=CARTESIAN_POINT('Ctrl Pts',(14.7894951923039,25.949445299615,74.5413138042756));
#116738=CARTESIAN_POINT('Ctrl Pts',(14.8275519301444,25.8867422530599,74.3364483228102));
#116739=CARTESIAN_POINT('Ctrl Pts',(14.8580193379202,25.8286904550241,74.1304837409515));
#116740=CARTESIAN_POINT('Ctrl Pts',(14.8808863595751,25.7762233263775,73.9238500636511));
#116741=CARTESIAN_POINT('Ctrl Pts',(14.9059012075637,25.7188281278553,73.6978079447862));
#116742=CARTESIAN_POINT('Ctrl Pts',(14.9218208569589,25.6681159683744,73.4709651355588));
#116743=CARTESIAN_POINT('Ctrl Pts',(14.9286358566856,25.6250936747152,73.2439493185516));
#116744=CARTESIAN_POINT('Ctrl Pts',(14.931187773495,25.608983723318,73.1589419080368));
#116745=CARTESIAN_POINT('Ctrl Pts',(14.932463061676,25.593952023497,73.0739102388527));
#116746=CARTESIAN_POINT('Ctrl Pts',(14.9324629260191,25.5800360490065,72.98888938658));
#116747=CARTESIAN_POINT('',(14.2241883540074,89.,76.3858032888143));
#116748=CARTESIAN_POINT('',(14.2241883532291,89.,76.385803290591));
#116749=CARTESIAN_POINT('',(14.2241883539424,89.,69.591975484192));
#116750=CARTESIAN_POINT('Origin',(6.43246351666909,89.,72.98888938658));
#116751=CARTESIAN_POINT('',(14.2241883529691,89.,69.591975481954));
#116752=CARTESIAN_POINT('Origin',(-15.5675364832709,75.,72.98888938658));
#116753=CARTESIAN_POINT('',(-18.5675364832709,75.,62.73888938658));
#116754=CARTESIAN_POINT('Origin',(-18.5675364832709,75.,72.98888938658));
#116755=CARTESIAN_POINT('',(-15.5675364833309,75.,62.73888938658));
#116756=CARTESIAN_POINT('',(-15.5675364832709,75.,62.73888938658));
#116757=CARTESIAN_POINT('Origin',(-15.5675364833309,75.,72.98888938658));
#116758=CARTESIAN_POINT('Origin',(-18.5675364832709,75.,72.98888938658));
#116759=CARTESIAN_POINT('',(-20.0675364832709,75.,84.7388893856825));
#116760=CARTESIAN_POINT('',(-20.0675364832709,75.,61.23888938658));
#116761=CARTESIAN_POINT('Origin',(-20.0675364832709,75.,72.98888938658));
#116762=CARTESIAN_POINT('',(-18.5675364832709,75.,61.23888938658));
#116763=CARTESIAN_POINT('',(-18.5675364832709,75.,61.23888938658));
#116764=CARTESIAN_POINT('Origin',(-18.5675364832709,75.,72.98888938658));
#116765=CARTESIAN_POINT('Origin',(-20.0675364832709,75.,72.98888938658));
#116766=CARTESIAN_POINT('Origin',(-20.5675364832709,75.,72.98888938658));
#116767=CARTESIAN_POINT('',(-20.5675364832709,75.,84.23888938658));
#116768=CARTESIAN_POINT('',(-20.5675364832709,75.,84.23888938658));
#116769=CARTESIAN_POINT('Origin',(-20.5675364832709,75.,72.98888938658));
#116770=CARTESIAN_POINT('Origin',(-20.5675364832709,75.,72.98888938658));
#116771=CARTESIAN_POINT('',(-20.3675364832709,75.,65.23888938658));
#116772=CARTESIAN_POINT('',(-20.3675364832709,75.,80.73888938658));
#116773=CARTESIAN_POINT('Origin',(-20.3675364832709,75.,72.98888938658));
#116774=CARTESIAN_POINT('',(-18.0675364832709,75.,80.73888938658));
#116775=CARTESIAN_POINT('',(-20.5675364832709,75.,80.73888938658));
#116776=CARTESIAN_POINT('',(-18.0675364832709,75.,65.23888938658));
#116777=CARTESIAN_POINT('Origin',(-18.0675364832709,75.,72.98888938658));
#116778=CARTESIAN_POINT('Origin',(-18.0675364832709,75.,72.98888938658));
#116779=CARTESIAN_POINT('Origin',(-20.3675364832709,75.,72.98888938658));
#116780=CARTESIAN_POINT('Origin',(-18.0675364832709,75.,72.98888938658));
#116781=CARTESIAN_POINT('',(-17.0930718951697,71.9689110866349,78.2388893867872));
#116782=CARTESIAN_POINT('',(-17.0930718951698,78.0310889133652,78.2388893867871));
#116783=CARTESIAN_POINT('Ctrl Pts',(-17.0930718944527,71.9689110864279,
78.23888938658));
#116784=CARTESIAN_POINT('Ctrl Pts',(-16.2180718918697,75.,78.23888938658));
#116785=CARTESIAN_POINT('Ctrl Pts',(-17.0930718944527,78.0310889135722,
78.23888938658));
#116786=CARTESIAN_POINT('',(-17.0930718951698,68.9378221732697,72.98888938658));
#116787=CARTESIAN_POINT('Ctrl Pts',(-17.0930718945656,68.9378221731502,
72.9888893859585));
#116788=CARTESIAN_POINT('Ctrl Pts',(-16.2180718917851,70.4533666301317,
75.61388938658));
#116789=CARTESIAN_POINT('Ctrl Pts',(-17.0930718945656,71.9689110871133,
78.2388893872015));
#116790=CARTESIAN_POINT('',(-17.0930718951698,71.9689110866349,67.7388893863728));
#116791=CARTESIAN_POINT('Ctrl Pts',(-17.0930718945656,71.9689110871132,
67.7388893859585));
#116792=CARTESIAN_POINT('Ctrl Pts',(-16.2180718917851,70.4533666301317,
70.36388938658));
#116793=CARTESIAN_POINT('Ctrl Pts',(-17.0930718945656,68.9378221731501,
72.9888893872014));
#116794=CARTESIAN_POINT('',(-16.6241608063082,75.,67.73888938658));
#116795=CARTESIAN_POINT('Ctrl Pts',(-17.0930718944527,71.9689110864279,
67.73888938658));
#116796=CARTESIAN_POINT('Ctrl Pts',(-16.6241608063082,73.5932667396053,
67.73888938658));
#116797=CARTESIAN_POINT('Ctrl Pts',(-16.6241608063082,75.,67.73888938658));
#116798=CARTESIAN_POINT('',(-18.0675364832709,75.,65.23888938658));
#116799=CARTESIAN_POINT('',(-17.0930718951698,78.0310889133651,67.7388893863728));
#116800=CARTESIAN_POINT('Ctrl Pts',(-16.6241608063082,75.,67.73888938658));
#116801=CARTESIAN_POINT('Ctrl Pts',(-16.6241608063082,76.4067332603946,
67.73888938658));
#116802=CARTESIAN_POINT('Ctrl Pts',(-17.0930718944527,78.0310889135721,
67.73888938658));
#116803=CARTESIAN_POINT('',(-17.0930718951697,81.0621778267303,72.98888938658));
#116804=CARTESIAN_POINT('Ctrl Pts',(-17.0930718945656,81.0621778268498,
72.9888893872014));
#116805=CARTESIAN_POINT('Ctrl Pts',(-16.2180718917851,79.5466333698683,
70.36388938658));
#116806=CARTESIAN_POINT('Ctrl Pts',(-17.0930718945656,78.0310889128867,
67.7388893859585));
#116807=CARTESIAN_POINT('Ctrl Pts',(-17.0930718945656,78.0310889128868,
78.2388893872014));
#116808=CARTESIAN_POINT('Ctrl Pts',(-16.2180718917851,79.5466333698683,
75.61388938658));
#116809=CARTESIAN_POINT('Ctrl Pts',(-17.0930718945656,81.0621778268498,
72.9888893859586));
#116810=CARTESIAN_POINT('Origin',(-20.5675364832709,75.,72.98888938658));
#116811=CARTESIAN_POINT('',(-20.5675364832709,75.,65.03888938658));
#116812=CARTESIAN_POINT('',(-20.5675364832709,75.,65.03888938658));
#116813=CARTESIAN_POINT('Origin',(-20.5675364832709,75.,72.98888938658));
#116814=CARTESIAN_POINT('Origin',(-15.5675364832709,75.,72.98888938658));
#116815=CARTESIAN_POINT('',(-15.5675364832709,68.9378221735089,72.98888938658));
#116816=CARTESIAN_POINT('',(-15.5675364832709,71.9689110867545,78.23888938658));
#116817=CARTESIAN_POINT('',(-15.5675364832709,71.9689110867545,78.23888938658));
#116818=CARTESIAN_POINT('',(-15.5675364832709,78.0310889132456,78.23888938658));
#116819=CARTESIAN_POINT('',(-15.5675364832709,78.0310889132456,78.23888938658));
#116820=CARTESIAN_POINT('',(-15.5675364832709,81.0621778264911,72.98888938658));
#116821=CARTESIAN_POINT('',(-15.5675364832709,81.0621778264911,72.98888938658));
#116822=CARTESIAN_POINT('',(-15.5675364832709,78.0310889132455,67.73888938658));
#116823=CARTESIAN_POINT('',(-15.5675364832709,78.0310889132455,67.73888938658));
#116824=CARTESIAN_POINT('',(-15.5675364832709,71.9689110867545,67.73888938658));
#116825=CARTESIAN_POINT('',(-15.5675364832709,71.9689110867545,67.73888938658));
#116826=CARTESIAN_POINT('',(-15.5675364832709,68.9378221735089,72.98888938658));
#116827=CARTESIAN_POINT('Origin',(-25.5675364832709,71.9689110867545,78.23888938658));
#116828=CARTESIAN_POINT('',(-25.5675364832709,68.9378221735089,72.98888938658));
#116829=CARTESIAN_POINT('',(-25.5675364832709,71.9689110867545,78.23888938658));
#116830=CARTESIAN_POINT('Origin',(-25.5675364832709,78.0310889132456,78.23888938658));
#116831=CARTESIAN_POINT('',(-25.5675364832709,78.0310889132456,78.23888938658));
#116832=CARTESIAN_POINT('Origin',(-25.5675364832709,81.0621778264911,72.98888938658));
#116833=CARTESIAN_POINT('',(-25.5675364832709,81.0621778264911,72.98888938658));
#116834=CARTESIAN_POINT('Origin',(-25.5675364832709,78.0310889132455,67.73888938658));
#116835=CARTESIAN_POINT('',(-25.5675364832709,78.0310889132455,67.73888938658));
#116836=CARTESIAN_POINT('Origin',(-25.5675364832709,71.9689110867545,67.73888938658));
#116837=CARTESIAN_POINT('',(-25.5675364832709,71.9689110867545,67.73888938658));
#116838=CARTESIAN_POINT('Origin',(-25.5675364832709,68.9378221735089,72.98888938658));
#116839=CARTESIAN_POINT('Origin',(-18.5675364832709,75.,72.98888938658));
#116840=CARTESIAN_POINT('Origin',(-20.5675364832709,75.,72.98888938658));
#116841=CARTESIAN_POINT('Origin',(22.4176035807091,15.,81.066383761497));
#116842=CARTESIAN_POINT('',(21.1895064189465,15.000000374545,65.4633429305526));
#116843=CARTESIAN_POINT('',(19.9598072485171,15.0000009014414,58.489372381727));
#116844=CARTESIAN_POINT('',(23.5337568174491,15.,78.758247596214));
#116845=CARTESIAN_POINT('',(20.4074539076363,16.323529159868,65.6012398886274));
#116846=CARTESIAN_POINT('Origin',(19.7122947894285,15.,65.7238151970529));
#116847=CARTESIAN_POINT('',(19.1777534373736,16.323529923502,58.6272689137465));
#116848=CARTESIAN_POINT('',(22.7517036150791,16.32352940976,78.896144732003));
#116849=CARTESIAN_POINT('Origin',(18.4825956513191,15.,58.74984483153));
#116850=CARTESIAN_POINT('Ctrl Pts',(12.7032824634691,21.12789835764,82.238037292941));
#116851=CARTESIAN_POINT('Ctrl Pts',(12.7138554120091,21.14828359132,82.237040898622));
#116852=CARTESIAN_POINT('Ctrl Pts',(12.8158373280291,21.35262796258,82.223214955634));
#116853=CARTESIAN_POINT('Ctrl Pts',(12.9542723631091,21.78746324258,82.119828041772));
#116854=CARTESIAN_POINT('Ctrl Pts',(12.9927499413291,22.43374057185,81.82237309057));
#116855=CARTESIAN_POINT('Ctrl Pts',(12.9040637925191,22.89144264331,81.525965837519));
#116856=CARTESIAN_POINT('Ctrl Pts',(12.8188596948191,23.13940046188,81.341229725473));
#116857=CARTESIAN_POINT('Ctrl Pts',(12.8039698070391,23.17979419886,81.3104543621581));
#116858=CARTESIAN_POINT('Ctrl Pts',(12.2574243304591,21.44258358145,82.137599709054));
#116859=CARTESIAN_POINT('Ctrl Pts',(12.2648149716791,21.4590752496,82.1384735189879));
#116860=CARTESIAN_POINT('Ctrl Pts',(12.3361831962091,21.62530550758,82.144718783879));
#116861=CARTESIAN_POINT('Ctrl Pts',(12.4361287210991,21.99868109559,82.108019885141));
#116862=CARTESIAN_POINT('Ctrl Pts',(12.4736490564891,22.61131241278,81.933979041512));
#116863=CARTESIAN_POINT('Ctrl Pts',(12.4198055527491,23.08419677334,81.721137563021));
#116864=CARTESIAN_POINT('Ctrl Pts',(12.3623243256291,23.35151971112,81.5753002657141));
#116865=CARTESIAN_POINT('Ctrl Pts',(12.3521479900591,23.39541857132,81.550693031506));
#116866=CARTESIAN_POINT('Ctrl Pts',(11.8797380580991,21.71775544054,82.436832824221));
#116867=CARTESIAN_POINT('Ctrl Pts',(11.8879752712991,21.73377171117,82.439230205427));
#116868=CARTESIAN_POINT('Ctrl Pts',(11.9685429834291,21.89572596927,82.461081441199));
#116869=CARTESIAN_POINT('Ctrl Pts',(12.1037386879891,22.27116764255,82.462282033507));
#116870=CARTESIAN_POINT('Ctrl Pts',(12.2280447882491,22.92210242598,82.328679396874));
#116871=CARTESIAN_POINT('Ctrl Pts',(12.2548992725691,23.44220679821,82.11473481512));
#116872=CARTESIAN_POINT('Ctrl Pts',(12.2436859938191,23.73958274288,81.954178203878));
#116873=CARTESIAN_POINT('Ctrl Pts',(12.2410687116591,23.78853957945,81.926787648707));
#116874=CARTESIAN_POINT('Ctrl Pts',(11.7737606800391,21.80512243469,82.974478406183));
#116875=CARTESIAN_POINT('Ctrl Pts',(11.7864171226091,21.82433766992,82.977231665452));
#116876=CARTESIAN_POINT('Ctrl Pts',(11.9110398512391,22.01815839942,83.00181349883));
#116877=CARTESIAN_POINT('Ctrl Pts',(12.1362289260491,22.45807851148,82.99170083158));
#116878=CARTESIAN_POINT('Ctrl Pts',(12.3882945132591,23.19862430865,82.793768148027));
#116879=CARTESIAN_POINT('Ctrl Pts',(12.4982137765991,23.77253931309,82.494646053088));
#116880=CARTESIAN_POINT('Ctrl Pts',(12.5268794937091,24.09446043562,82.273684311624));
#116881=CARTESIAN_POINT('Ctrl Pts',(12.5305931541991,24.1473023328,82.236058931096));
#116882=CARTESIAN_POINT('',(12.5172885372655,21.4321684423365,82.2239071870765));
#116883=CARTESIAN_POINT('',(12.6211114714367,23.194984440251,81.5466523813612));
#116884=CARTESIAN_POINT('Ctrl Pts',(12.5172885372655,21.4321684423365,82.2239071870765));
#116885=CARTESIAN_POINT('Ctrl Pts',(12.5342731760867,21.4730660932803,82.2209158140286));
#116886=CARTESIAN_POINT('Ctrl Pts',(12.5505055162535,21.5160946454251,82.216479391709));
#116887=CARTESIAN_POINT('Ctrl Pts',(12.5658342343901,21.5611251493771,82.210418068523));
#116888=CARTESIAN_POINT('Ctrl Pts',(12.5804334410794,21.6040125994993,82.2046452107266));
#116889=CARTESIAN_POINT('Ctrl Pts',(12.5942131719627,21.6487162279354,82.1973985931567));
#116890=CARTESIAN_POINT('Ctrl Pts',(12.6070526543159,21.6950838572293,82.1885421434366));
#116891=CARTESIAN_POINT('Ctrl Pts',(12.6170577467715,21.731215564511,82.181640806152));
#116892=CARTESIAN_POINT('Ctrl Pts',(12.6264921283407,21.7683570037951,82.1737622916675));
#116893=CARTESIAN_POINT('Ctrl Pts',(12.6353019488066,21.8064159145208,82.1648503782335));
#116894=CARTESIAN_POINT('Ctrl Pts',(12.6419587616857,21.8351737136229,82.1581164226036));
#116895=CARTESIAN_POINT('Ctrl Pts',(12.64825458311,21.8644643485648,82.1507925482019));
#116896=CARTESIAN_POINT('Ctrl Pts',(12.6541492093415,21.894240056901,82.1428653077459));
#116897=CARTESIAN_POINT('Ctrl Pts',(12.6624164044795,21.9360003961519,82.1317473774173));
#116898=CARTESIAN_POINT('Ctrl Pts',(12.6698938329058,21.9787150737606,82.1194418905041));
#116899=CARTESIAN_POINT('Ctrl Pts',(12.6764904514613,22.0222859506516,82.1059172229102));
#116900=CARTESIAN_POINT('Ctrl Pts',(12.6821405015729,22.059604712647,82.0943332501509));
#116901=CARTESIAN_POINT('Ctrl Pts',(12.6871406011452,22.0975462801781,82.081857873438));
#116902=CARTESIAN_POINT('Ctrl Pts',(12.6914248518296,22.1360375972392,82.0684949110168));
#116903=CARTESIAN_POINT('Ctrl Pts',(12.6935669771719,22.1552832557698,82.0618134298062));
#116904=CARTESIAN_POINT('Ctrl Pts',(12.6955301256819,22.1746663379845,82.0549103304341));
#116905=CARTESIAN_POINT('Ctrl Pts',(12.697306057862,22.1941777204868,82.0477877712179));
#116906=CARTESIAN_POINT('Ctrl Pts',(12.6981940239521,22.2039334117379,82.0442264916098));
#116907=CARTESIAN_POINT('Ctrl Pts',(12.6990351936357,22.2137211822264,82.0406103594189));
#116908=CARTESIAN_POINT('Ctrl Pts',(12.699828535949,22.2235398957011,82.03693975532));
#116909=CARTESIAN_POINT('Ctrl Pts',(12.7002252071056,22.2284492524385,82.0351044532705));
#116910=CARTESIAN_POINT('Ctrl Pts',(12.7006099219181,22.2333663451915,82.0332555340571));
#116911=CARTESIAN_POINT('Ctrl Pts',(12.7009825534323,22.2382910332833,82.0313930508635));
#116912=CARTESIAN_POINT('Ctrl Pts',(12.7011688691894,22.2407533773292,82.0304618092667));
#116913=CARTESIAN_POINT('Ctrl Pts',(12.7013521641543,22.2432176202277,82.0295271767241));
#116914=CARTESIAN_POINT('Ctrl Pts',(12.701532422489,22.2456837444361,82.0285891603029));
#116915=CARTESIAN_POINT('Ctrl Pts',(12.7017126808237,22.2481498686444,82.0276511438817));
#116916=CARTESIAN_POINT('Ctrl Pts',(12.7019711143474,22.2517695268232,82.0262692122548));
#116917=CARTESIAN_POINT('Ctrl Pts',(12.7020640718486,22.2530877435032,82.0257649667038));
#116918=CARTESIAN_POINT('Ctrl Pts',(12.7037070878608,22.2763871124193,82.0168524690137));
#116919=CARTESIAN_POINT('Ctrl Pts',(12.7051346969877,22.3029829310185,82.0065495121645));
#116920=CARTESIAN_POINT('Ctrl Pts',(12.7061815011432,22.3327077677197,81.9946690642417));
#116921=CARTESIAN_POINT('Ctrl Pts',(12.7072104468936,22.3619255007986,81.9829912959245));
#116922=CARTESIAN_POINT('Ctrl Pts',(12.7078707303876,22.3941672419834,81.9697884885638));
#116923=CARTESIAN_POINT('Ctrl Pts',(12.707973025637,22.4292409366076,81.954868550681));
#116924=CARTESIAN_POINT('Ctrl Pts',(12.7080548403087,22.4572925111177,81.9429357402461));
#116925=CARTESIAN_POINT('Ctrl Pts',(12.7077790066496,22.4871551917192,81.9299040392018));
#116926=CARTESIAN_POINT('Ctrl Pts',(12.7070379455413,22.5187090825413,81.9156747183529));
#116927=CARTESIAN_POINT('Ctrl Pts',(12.7062349330901,22.5529008204859,81.9002558525042));
#116928=CARTESIAN_POINT('Ctrl Pts',(12.7048861036379,22.5890768462464,81.8834317772353));
#116929=CARTESIAN_POINT('Ctrl Pts',(12.702834427738,22.6271006413617,81.8650511210193));
#116930=CARTESIAN_POINT('Ctrl Pts',(12.7006542075314,22.667506753477,81.8455188556689));
#116931=CARTESIAN_POINT('Ctrl Pts',(12.6977134308586,22.7099757493514,81.8242030713352));
#116932=CARTESIAN_POINT('Ctrl Pts',(12.6936892868462,22.7542534992715,81.8011037562274));
#116933=CARTESIAN_POINT('Ctrl Pts',(12.6899832884161,22.7950306859686,81.7798306543551));
#116934=CARTESIAN_POINT('Ctrl Pts',(12.6853581107381,22.8373416451533,81.7570449391417));
#116935=CARTESIAN_POINT('Ctrl Pts',(12.6795926657466,22.8809919056613,81.732779052393));
#116936=CARTESIAN_POINT('Ctrl Pts',(12.673998690671,22.9233439651614,81.7092348566094));
#116937=CARTESIAN_POINT('Ctrl Pts',(12.6673308978515,22.9669565596022,81.6842972397914));
#116938=CARTESIAN_POINT('Ctrl Pts',(12.6594231085505,23.0116601500446,81.6580274464931));
#116939=CARTESIAN_POINT('Ctrl Pts',(12.6517293215199,23.0551539624462,81.6324685719097));
#116940=CARTESIAN_POINT('Ctrl Pts',(12.64286152633,23.0996802668986,81.6056488217044));
#116941=CARTESIAN_POINT('Ctrl Pts',(12.6327052588187,23.145094629419,81.5776535648036));
#116942=CARTESIAN_POINT('Ctrl Pts',(12.6290120242389,23.1616091505153,81.5674733435029));
#116943=CARTESIAN_POINT('Ctrl Pts',(12.6251488006487,23.1782412365338,81.5571379482193));
#116944=CARTESIAN_POINT('Ctrl Pts',(12.6211114714367,23.194984440251,81.5466523813612));
#116945=CARTESIAN_POINT('',(11.9367286423891,21.85927935059,82.709938120253));
#116946=CARTESIAN_POINT('Ctrl Pts',(12.5172885370886,21.4321684424534,82.2239071871077));
#116947=CARTESIAN_POINT('Ctrl Pts',(12.4901986054513,21.4500656883045,82.2286841217066));
#116948=CARTESIAN_POINT('Ctrl Pts',(12.463084003402,21.4681677807312,82.2351093103302));
#116949=CARTESIAN_POINT('Ctrl Pts',(12.436158321932,21.486342887008,82.2432343641709));
#116950=CARTESIAN_POINT('Ctrl Pts',(12.4095744841301,21.5042872453645,82.2512562637717));
#116951=CARTESIAN_POINT('Ctrl Pts',(12.3831754932965,21.5223023630035,82.2609354122807));
#116952=CARTESIAN_POINT('Ctrl Pts',(12.3571761792444,21.5402500104206,82.2722728721136));
#116953=CARTESIAN_POINT('Ctrl Pts',(12.331333296169,21.5580896716037,82.2835421174578));
#116954=CARTESIAN_POINT('Ctrl Pts',(12.3058860226616,21.5758622159077,82.2964498591008));
#116955=CARTESIAN_POINT('Ctrl Pts',(12.2810439524597,21.5934270741106,82.3109460939382));
#116956=CARTESIAN_POINT('Ctrl Pts',(12.2563091655433,21.6109160764899,82.3253797251484));
#116957=CARTESIAN_POINT('Ctrl Pts',(12.2321750779958,21.6281987093121,82.3413879941782));
#116958=CARTESIAN_POINT('Ctrl Pts',(12.2088363986967,21.6451383982326,82.358871396183));
#116959=CARTESIAN_POINT('Ctrl Pts',(12.1976321134016,21.6532706967677,82.3672647170509));
#116960=CARTESIAN_POINT('Ctrl Pts',(12.1866108985648,21.661324033758,82.3759972842875));
#116961=CARTESIAN_POINT('Ctrl Pts',(12.1757925791577,21.6692839648808,82.385054228068));
#116962=CARTESIAN_POINT('Ctrl Pts',(12.1532704744542,21.6858553375157,82.4039094151299));
#116963=CARTESIAN_POINT('Ctrl Pts',(12.1316297125416,21.7020208130826,82.4241729741317));
#116964=CARTESIAN_POINT('Ctrl Pts',(12.1110283811666,21.7176603411047,82.4456798235158));
#116965=CARTESIAN_POINT('Ctrl Pts',(12.0903040996834,21.7333932068644,82.4673150271996));
#116966=CARTESIAN_POINT('Ctrl Pts',(12.0706321574346,21.7485934559033,82.4902077461713));
#116967=CARTESIAN_POINT('Ctrl Pts',(12.0521383030712,21.7631575075447,82.5141551663165));
#116968=CARTESIAN_POINT('Ctrl Pts',(12.0335582924248,21.7777894079174,82.5382141489662));
#116969=CARTESIAN_POINT('Ctrl Pts',(12.016167631061,21.7917789116451,82.5633368727513));
#116970=CARTESIAN_POINT('Ctrl Pts',(12.0000529277821,21.8050445217185,82.5892938730034));
#116971=CARTESIAN_POINT('Ctrl Pts',(11.9837508572241,21.8184643723773,82.6155526779137));
#116972=CARTESIAN_POINT('Ctrl Pts',(11.9687546780973,21.831143241998,82.6426644005985));
#116973=CARTESIAN_POINT('Ctrl Pts',(11.9551095463526,21.8430239972692,82.6703799767414));
#116974=CARTESIAN_POINT('Ctrl Pts',(11.9486802243942,21.8486219791852,82.6834390197483));
#116975=CARTESIAN_POINT('Ctrl Pts',(11.9425502049782,21.8540431752193,82.6966320435008));
#116976=CARTESIAN_POINT('Ctrl Pts',(11.9367208468594,21.8592837631663,82.709932965079));
#116977=CARTESIAN_POINT('Ctrl Pts',(11.9367286423891,21.85927935059,82.709938120253));
#116978=CARTESIAN_POINT('Ctrl Pts',(12.0071900742098,21.9487713614003,82.6799677853506));
#116979=CARTESIAN_POINT('Ctrl Pts',(12.0805141882767,22.0494537651696,82.6349778443183));
#116980=CARTESIAN_POINT('Ctrl Pts',(12.1883057397716,22.213950793166,82.5387148842099));
#116981=CARTESIAN_POINT('Ctrl Pts',(12.2238600590811,22.2709879989896,82.5018176720259));
#116982=CARTESIAN_POINT('Ctrl Pts',(12.2757972429648,22.3591664953451,82.4387235891574));
#116983=CARTESIAN_POINT('Ctrl Pts',(12.3014185157823,22.4039115576769,82.405247458691));
#116984=CARTESIAN_POINT('Ctrl Pts',(12.3305204624122,22.4570972242989,82.3627454175667));
#116985=CARTESIAN_POINT('Ctrl Pts',(12.3428035577651,22.4800826633257,82.3437861552096));
#116986=CARTESIAN_POINT('Ctrl Pts',(12.3509480101634,22.4954467029582,82.3309807498732));
#116987=CARTESIAN_POINT('Ctrl Pts',(12.3542990499949,22.5018085230508,82.325635432429));
#116988=CARTESIAN_POINT('Ctrl Pts',(12.4346388523314,22.6558582457957,82.1945792914));
#116989=CARTESIAN_POINT('Ctrl Pts',(12.4898962985337,22.7845944228403,82.0626293863271));
#116990=CARTESIAN_POINT('Ctrl Pts',(12.5733519052877,23.0108494673222,81.8009014666782));
#116991=CARTESIAN_POINT('Ctrl Pts',(12.6014038389502,23.1090913488287,81.6707965042619));
#116992=CARTESIAN_POINT('Ctrl Pts',(12.6211132020991,23.19498548026,81.546653375664));
#116993=CARTESIAN_POINT('Ctrl Pts',(19.8429432353291,17.66670903096,80.88967894675));
#116994=CARTESIAN_POINT('Ctrl Pts',(20.0692982204291,17.57364273498,80.504253529771));
#116995=CARTESIAN_POINT('Ctrl Pts',(20.5023128070991,17.38259467766,79.684876559745));
#116996=CARTESIAN_POINT('Ctrl Pts',(21.0289682966291,17.11506095695,78.40607475062));
#116997=CARTESIAN_POINT('Ctrl Pts',(21.4337450075691,16.87634404777,77.091691432304));
#116998=CARTESIAN_POINT('Ctrl Pts',(21.7264515133391,16.6689476013,75.737023720658));
#116999=CARTESIAN_POINT('Ctrl Pts',(21.9058894958591,16.49221282193,74.267914636433));
#117000=CARTESIAN_POINT('Ctrl Pts',(21.9436945982691,16.36324862353,72.7108971134944));
#117001=CARTESIAN_POINT('Ctrl Pts',(21.8274598255191,16.29549033631,71.134112925171));
#117002=CARTESIAN_POINT('Ctrl Pts',(21.5557051837891,16.29308032823,69.560465808041));
#117003=CARTESIAN_POINT('Ctrl Pts',(21.1189566322091,16.35954526088,67.982905962895));
#117004=CARTESIAN_POINT('Ctrl Pts',(20.6097838163291,16.47512090179,66.682075896747));
#117005=CARTESIAN_POINT('Ctrl Pts',(20.2389056685491,16.57078829643,65.920640579465));
#117006=CARTESIAN_POINT('Ctrl Pts',(20.1031948314991,16.60676833735,65.660578297905));
#117007=CARTESIAN_POINT('Ctrl Pts',(15.9217651634291,18.86023850409,78.8653534140521));
#117008=CARTESIAN_POINT('Ctrl Pts',(16.0904271054691,18.7673148555,78.591765890084));
#117009=CARTESIAN_POINT('Ctrl Pts',(16.4154187039391,18.57712863705,78.005939013225));
#117010=CARTESIAN_POINT('Ctrl Pts',(16.8157392045791,18.31228006428,77.079624029397));
#117011=CARTESIAN_POINT('Ctrl Pts',(17.1269628424391,18.07701240892,76.117836928949));
#117012=CARTESIAN_POINT('Ctrl Pts',(17.3548149996891,17.87334248467,75.11896421969));
#117013=CARTESIAN_POINT('Ctrl Pts',(17.4975479419891,17.70032472588,74.028850771698));
#117014=CARTESIAN_POINT('Ctrl Pts',(17.5323952584791,17.57438021074,72.868074785256));
#117015=CARTESIAN_POINT('Ctrl Pts',(17.4489288771991,17.50830697097,71.6894403714931));
#117016=CARTESIAN_POINT('Ctrl Pts',(17.2457919781591,17.50595826264,70.512431280761));
#117017=CARTESIAN_POINT('Ctrl Pts',(16.9161419351691,17.57076519201,69.334239814392));
#117018=CARTESIAN_POINT('Ctrl Pts',(16.5309101724491,17.68362893957,68.366455266264));
#117019=CARTESIAN_POINT('Ctrl Pts',(16.2506832159191,17.77725583824,67.8027331628201));
#117020=CARTESIAN_POINT('Ctrl Pts',(16.1482365562791,17.81250084465,67.610590819165));
#117021=CARTESIAN_POINT('Ctrl Pts',(13.7245240389691,22.48149564395,77.145847903068));
#117022=CARTESIAN_POINT('Ctrl Pts',(13.8434718950791,22.38900479815,76.936687900911));
#117023=CARTESIAN_POINT('Ctrl Pts',(14.0698770466191,22.2014334629,76.494081975836));
#117024=CARTESIAN_POINT('Ctrl Pts',(14.3427852808591,21.94473182854,75.809156314966));
#117025=CARTESIAN_POINT('Ctrl Pts',(14.5508108918891,21.71992946569,75.109894854898));
#117026=CARTESIAN_POINT('Ctrl Pts',(14.6998789996491,21.52756608686,74.392905753835));
#117027=CARTESIAN_POINT('Ctrl Pts',(14.7897760814891,21.3658260448,73.6186841310744));
#117028=CARTESIAN_POINT('Ctrl Pts',(14.8063911950091,21.24904347311,72.8007794935411));
#117029=CARTESIAN_POINT('Ctrl Pts',(14.7437806796791,21.18808279255,71.974011411747));
#117030=CARTESIAN_POINT('Ctrl Pts',(14.6012904929691,21.18592007224,71.149238564271));
#117031=CARTESIAN_POINT('Ctrl Pts',(14.3738366030991,21.24569649639,70.321565846831));
#117032=CARTESIAN_POINT('Ctrl Pts',(14.1091114755891,21.35033215796,69.63726307722));
#117033=CARTESIAN_POINT('Ctrl Pts',(13.9161056624891,21.43776804022,69.235362518137));
#117034=CARTESIAN_POINT('Ctrl Pts',(13.8454360114391,21.47078289727,69.0979054154141));
#117035=CARTESIAN_POINT('Ctrl Pts',(14.1931489316191,26.97809399155,76.468292357438));
#117036=CARTESIAN_POINT('Ctrl Pts',(14.2916734495191,26.88614056693,76.248530254187));
#117037=CARTESIAN_POINT('Ctrl Pts',(14.4711914398691,26.70181619234,75.797419155646));
#117038=CARTESIAN_POINT('Ctrl Pts',(14.6702301335491,26.45523079894,75.13930481074));
#117039=CARTESIAN_POINT('Ctrl Pts',(14.8096524336191,26.2434234307,74.49995704091));
#117040=CARTESIAN_POINT('Ctrl Pts',(14.8997805017791,26.06509964957,73.870100268841));
#117041=CARTESIAN_POINT('Ctrl Pts',(14.9433609581991,25.91736340798,73.2132478891327));
#117042=CARTESIAN_POINT('Ctrl Pts',(14.9342853630891,25.81195743237,72.5378598662094));
#117043=CARTESIAN_POINT('Ctrl Pts',(14.8716775461091,25.75734513428,71.865834093289));
#117044=CARTESIAN_POINT('Ctrl Pts',(14.7558645741991,25.75541335958,71.197896549204));
#117045=CARTESIAN_POINT('Ctrl Pts',(14.5818943027391,25.8089432896,70.521630061898));
#117046=CARTESIAN_POINT('Ctrl Pts',(14.3825817446091,25.90336194739,69.949720331184));
#117047=CARTESIAN_POINT('Ctrl Pts',(14.2359764423691,25.98311030206,69.604378827809));
#117048=CARTESIAN_POINT('Ctrl Pts',(14.1819742353591,26.0133559313,69.484929408113));
#117049=CARTESIAN_POINT('',(15.6158099654941,20.1981134279197,68.3761656716912));
#117050=CARTESIAN_POINT('Origin',(22.9325826401891,25.68032358419,65.795421779755));
#117051=CARTESIAN_POINT('',(15.9984184148119,20.3875458432315,78.383019919252));
#117052=CARTESIAN_POINT('Ctrl Pts',(15.6158091070711,20.1981127933161,68.3761659747572));
#117053=CARTESIAN_POINT('Ctrl Pts',(16.2185010787615,20.1430815615197,69.9680357680762));
#117054=CARTESIAN_POINT('Ctrl Pts',(16.560638794584,20.1332273419861,71.64811321169));
#117055=CARTESIAN_POINT('Ctrl Pts',(16.7005936251506,20.218545920064,75.1663223132348));
#117056=CARTESIAN_POINT('Ctrl Pts',(16.4573509577271,20.3124614378109,76.8746944962966));
#117057=CARTESIAN_POINT('Ctrl Pts',(15.9984175514895,20.387544970039,78.3830197000386));
#117058=CARTESIAN_POINT('Origin',(22.9324069483482,26.6270131840282,80.1828101714809));
#117059=CARTESIAN_POINT('Origin',(17.7894674803291,1.4210854715202E-14,
100.88908350184));
#117060=CARTESIAN_POINT('',(18.9921123831974,17.0122606549803,65.8508016863977));
#117061=CARTESIAN_POINT('Origin',(11.8338327653321,1.4210854715202E-14,
67.1130006183879));
#117062=CARTESIAN_POINT('',(15.2821042656531,17.8079467178956,57.8022951133291));
#117063=CARTESIAN_POINT('Ctrl Pts',(18.9921123831974,17.0122606549803,65.8508016863977));
#117064=CARTESIAN_POINT('Ctrl Pts',(18.8584828352797,17.0408671426352,65.4783085652489));
#117065=CARTESIAN_POINT('Ctrl Pts',(18.7209892451032,17.0708101915551,65.1082362936578));
#117066=CARTESIAN_POINT('Ctrl Pts',(18.5796489012198,17.101896657633,64.7405625793287));
#117067=CARTESIAN_POINT('Ctrl Pts',(18.4320707453025,17.1343550712161,64.3566622204565));
#117068=CARTESIAN_POINT('Ctrl Pts',(18.2802986847668,17.1680604374422,63.9753763743597));
#117069=CARTESIAN_POINT('Ctrl Pts',(18.1243308189613,17.2027999736258,63.596735420507));
#117070=CARTESIAN_POINT('Ctrl Pts',(17.9683629531559,17.2375395098094,63.2180944666542));
#117071=CARTESIAN_POINT('Ctrl Pts',(17.8081990244202,17.2733136613848,62.842098371325));
#117072=CARTESIAN_POINT('Ctrl Pts',(17.6438191240194,17.3099101632158,62.4688350059709));
#117073=CARTESIAN_POINT('Ctrl Pts',(17.4791788661025,17.3465646293981,62.09498043742));
#117074=CARTESIAN_POINT('Ctrl Pts',(17.3103091873621,17.3840443729146,61.7238679103735));
#117075=CARTESIAN_POINT('Ctrl Pts',(17.1371257413606,17.422108587588,61.3554290200356));
#117076=CARTESIAN_POINT('Ctrl Pts',(16.9636788689392,17.4602307010967,60.986429703513));
#117077=CARTESIAN_POINT('Ctrl Pts',(16.7859049271392,17.4989395052665,60.620112265243));
#117078=CARTESIAN_POINT('Ctrl Pts',(16.6037058990406,17.5379817897613,60.2564573874014));
#117079=CARTESIAN_POINT('Ctrl Pts',(16.422299248806,17.5768542805842,59.8943840332285));
#117080=CARTESIAN_POINT('Ctrl Pts',(16.2365057539938,17.6160577681685,59.5349502630608));
#117081=CARTESIAN_POINT('Ctrl Pts',(16.0462180137517,17.65532478812,59.1781841243065));
#117082=CARTESIAN_POINT('Ctrl Pts',(15.8632233084799,17.6930868464312,58.8350915302737));
#117083=CARTESIAN_POINT('Ctrl Pts',(15.6760720768127,17.730907883019,58.4944663422677));
#117084=CARTESIAN_POINT('Ctrl Pts',(15.4846614635924,17.7685293574614,58.1563733471083));
#117085=CARTESIAN_POINT('Ctrl Pts',(15.4176654200366,17.7816973312637,58.0380366851618));
#117086=CARTESIAN_POINT('Ctrl Pts',(15.3501475082489,17.7948406501483,57.9200105893426));
#117087=CARTESIAN_POINT('Ctrl Pts',(15.2821042656531,17.8079467178956,57.8022951133291));
#117088=CARTESIAN_POINT('Ctrl Pts',(19.1777532421465,16.3235298342272,58.6272695410447));
#117089=CARTESIAN_POINT('Ctrl Pts',(18.9453611592213,16.4404319258409,58.5715817835269));
#117090=CARTESIAN_POINT('Ctrl Pts',(18.7156139825874,16.5504510635377,58.5177831660704));
#117091=CARTESIAN_POINT('Ctrl Pts',(18.4889489462576,16.6540581469211,58.4658115211243));
#117092=CARTESIAN_POINT('Ctrl Pts',(18.2590018284741,16.7591654479487,58.4130873332418));
#117093=CARTESIAN_POINT('Ctrl Pts',(18.0322266560163,16.8576739887225,58.3622434270875));
#117094=CARTESIAN_POINT('Ctrl Pts',(17.8090267987014,16.9500767735686,58.3132242642099));
#117095=CARTESIAN_POINT('Ctrl Pts',(17.5806932957228,17.0446048427291,58.2630776498368));
#117096=CARTESIAN_POINT('Ctrl Pts',(17.3561014070839,17.1327433971003,58.2148406933092));
#117097=CARTESIAN_POINT('Ctrl Pts',(17.135628872468,17.2150165121611,58.1684634758667));
#117098=CARTESIAN_POINT('Ctrl Pts',(16.9124418330387,17.2983025913412,58.1215152522433));
#117099=CARTESIAN_POINT('Ctrl Pts',(16.6934760271185,17.3755782319407,58.0764728766697));
#117100=CARTESIAN_POINT('Ctrl Pts',(16.4790704722335,17.4473782663621,58.0332938821258));
#117101=CARTESIAN_POINT('Ctrl Pts',(16.2603714273099,17.5206161027693,57.9892502244296));
#117102=CARTESIAN_POINT('Ctrl Pts',(16.0464169541269,17.5881571707185,57.9471453496133));
#117103=CARTESIAN_POINT('Ctrl Pts',(15.8375146169777,17.6505548979763,57.9069433976324));
#117104=CARTESIAN_POINT('Ctrl Pts',(15.6481633096011,17.7071128637455,57.8705039194027));
#117105=CARTESIAN_POINT('Ctrl Pts',(15.4629619198439,17.7594451174825,57.8356279892979));
#117106=CARTESIAN_POINT('Ctrl Pts',(15.2821054022649,17.807950818201,57.8022949128784));
#117107=CARTESIAN_POINT('Origin',(18.4825956495891,15.00000121252,58.74984482171));
#117108=CARTESIAN_POINT('',(18.87832452956,15.0000021622099,57.3029855895947));
#117109=CARTESIAN_POINT('Origin',(18.4825952511691,15.00000123316,58.74984256216));
#117110=CARTESIAN_POINT('Origin',(18.4825924316391,15.00000208393,58.74984406621));
#117111=CARTESIAN_POINT('Origin',(24.2283495281091,17.,82.697478608263));
#117112=CARTESIAN_POINT('',(21.1895064189391,9.5,65.4633429305539));
#117113=CARTESIAN_POINT('',(21.1895064189391,17.,65.4633429305539));
#117114=CARTESIAN_POINT('',(19.9598075156051,9.54868022077971,58.4893745818179));
#117115=CARTESIAN_POINT('',(19.9598072163191,15.00000057102,58.48937219914));
#117116=CARTESIAN_POINT('',(20.0012895471991,9.5,58.72463018868));
#117117=CARTESIAN_POINT('Origin',(19.9938181733183,9.83076353882643,58.6822579212327));
#117118=CARTESIAN_POINT('',(24.2283495281091,9.5,82.697478608263));
#117119=CARTESIAN_POINT('Ctrl Pts',(18.5989684124291,9.99292997789002,57.25761225601));
#117120=CARTESIAN_POINT('Ctrl Pts',(18.6222625186891,9.92394001275902,57.26454489492));
#117121=CARTESIAN_POINT('Ctrl Pts',(18.6746819394891,9.75907899964801,57.29185528042));
#117122=CARTESIAN_POINT('Ctrl Pts',(18.7402509692591,9.51839895443402,57.3713825578401));
#117123=CARTESIAN_POINT('Ctrl Pts',(18.7909229819691,9.28449495434002,57.49585505039));
#117124=CARTESIAN_POINT('Ctrl Pts',(18.8206195909491,9.09361539184202,57.63791449765));
#117125=CARTESIAN_POINT('Ctrl Pts',(18.8336214569991,8.94122220603702,57.78727492797));
#117126=CARTESIAN_POINT('Ctrl Pts',(18.8336610801191,8.82264484939901,57.93631838649));
#117127=CARTESIAN_POINT('Ctrl Pts',(18.8241401371591,8.73276899790502,58.07983530743));
#117128=CARTESIAN_POINT('Ctrl Pts',(18.8079424561291,8.66610608857702,58.21541004732));
#117129=CARTESIAN_POINT('Ctrl Pts',(18.7872031755891,8.61777448570702,58.34273076413));
#117130=CARTESIAN_POINT('Ctrl Pts',(18.7709241463591,8.59460757857502,58.4247208402));
#117131=CARTESIAN_POINT('Ctrl Pts',(18.7624724636291,8.58514829630202,58.46435199577));
#117132=CARTESIAN_POINT('Ctrl Pts',(19.1654129070991,10.56056596522,57.24431313358));
#117133=CARTESIAN_POINT('Ctrl Pts',(19.1935754232291,10.48544979949,57.22567128383));
#117134=CARTESIAN_POINT('Ctrl Pts',(19.2603011303891,10.29996486048,57.19274799569));
#117135=CARTESIAN_POINT('Ctrl Pts',(19.3536368863391,10.00561091375,57.18966955586));
#117136=CARTESIAN_POINT('Ctrl Pts',(19.4379237982291,9.69047600408601,57.24547446787));
#117137=CARTESIAN_POINT('Ctrl Pts',(19.5003292194691,9.40799131016201,57.34649268402));
#117138=CARTESIAN_POINT('Ctrl Pts',(19.5434774508091,9.16014843910101,57.48118063348));
#117139=CARTESIAN_POINT('Ctrl Pts',(19.5697672879791,8.94773680058601,57.63993508744));
#117140=CARTESIAN_POINT('Ctrl Pts',(19.5814446261691,8.77008394202101,57.81469108227));
#117141=CARTESIAN_POINT('Ctrl Pts',(19.5805345073391,8.62473681342901,57.99968336702));
#117142=CARTESIAN_POINT('Ctrl Pts',(19.5684896165591,8.50880607634101,58.1914376917));
#117143=CARTESIAN_POINT('Ctrl Pts',(19.5532261047991,8.44806080916502,58.32574241798));
#117144=CARTESIAN_POINT('Ctrl Pts',(19.5439231135291,8.42241936143501,58.39293424589));
#117145=CARTESIAN_POINT('Ctrl Pts',(19.4392357106891,10.92141167485,57.90603676144));
#117146=CARTESIAN_POINT('Ctrl Pts',(19.4699542803791,10.87379705862,57.87087569833));
#117147=CARTESIAN_POINT('Ctrl Pts',(19.5462693720491,10.75026038072,57.79424981718));
#117148=CARTESIAN_POINT('Ctrl Pts',(19.6642017406291,10.53149760247,57.71309988849));
#117149=CARTESIAN_POINT('Ctrl Pts',(19.7840987440191,10.27151168125,57.6793926310801));
#117150=CARTESIAN_POINT('Ctrl Pts',(19.8855888519391,10.01808188889,57.69883695166));
#117151=CARTESIAN_POINT('Ctrl Pts',(19.9685932208391,9.77937666711901,57.763832807));
#117152=CARTESIAN_POINT('Ctrl Pts',(20.0333327084191,9.56174852794401,57.86707398515));
#117153=CARTESIAN_POINT('Ctrl Pts',(20.0802536347391,9.369648419902,58.00118585982));
#117154=CARTESIAN_POINT('Ctrl Pts',(20.1101332724391,9.2050307565,58.15955190861));
#117155=CARTESIAN_POINT('Ctrl Pts',(20.1236001164291,9.068480502455,58.33700345402));
#117156=CARTESIAN_POINT('Ctrl Pts',(20.1217629015091,8.99459062150501,58.46851211914));
#117157=CARTESIAN_POINT('Ctrl Pts',(20.1180160422391,8.963053782842,58.5356858368));
#117158=CARTESIAN_POINT('Ctrl Pts',(19.1716240193791,10.74757975927,58.64149899143));
#117159=CARTESIAN_POINT('Ctrl Pts',(19.2002636935791,10.73610478672,58.6138843975));
#117160=CARTESIAN_POINT('Ctrl Pts',(19.2727377436391,10.70079842939,58.54979795779));
#117161=CARTESIAN_POINT('Ctrl Pts',(19.3897465656791,10.6182049493,58.46605148569));
#117162=CARTESIAN_POINT('Ctrl Pts',(19.5148912603391,10.4996360383,58.40332391661));
#117163=CARTESIAN_POINT('Ctrl Pts',(19.6263270987591,10.36952005018,58.37478490362));
#117164=CARTESIAN_POINT('Ctrl Pts',(19.7226815576091,10.23623676329,58.37839571799));
#117165=CARTESIAN_POINT('Ctrl Pts',(19.8031323356991,10.10674994874,58.41134223997));
#117166=CARTESIAN_POINT('Ctrl Pts',(19.8673175928291,9.98666003797102,58.46985863138));
#117167=CARTESIAN_POINT('Ctrl Pts',(19.9155116515791,9.87969595699702,58.54974895378));
#117168=CARTESIAN_POINT('Ctrl Pts',(19.9481259915791,9.78824200696503,58.64715774711));
#117169=CARTESIAN_POINT('Ctrl Pts',(19.9599258661791,9.73758529007002,58.72330031862));
#117170=CARTESIAN_POINT('Ctrl Pts',(19.9630939247691,9.71579676191702,58.76289359955));
#117171=CARTESIAN_POINT('',(18.8782362963603,10.0000000055723,57.3029603857805));
#117172=CARTESIAN_POINT('Ctrl Pts',(18.8783268084662,9.99999999999988,57.3029850932652));
#117173=CARTESIAN_POINT('Ctrl Pts',(18.9208387324483,9.98511016261138,57.3146419262317));
#117174=CARTESIAN_POINT('Ctrl Pts',(18.9623037038507,9.97062352280902,57.3279940735751));
#117175=CARTESIAN_POINT('Ctrl Pts',(19.002593961926,9.95647282485062,57.3428781052431));
#117176=CARTESIAN_POINT('Ctrl Pts',(19.0432887126542,9.9421800614493,57.3579115646324));
#117177=CARTESIAN_POINT('Ctrl Pts',(19.082784869332,9.92822962541205,57.3745069335272));
#117178=CARTESIAN_POINT('Ctrl Pts',(19.1209943308262,9.91457522331445,57.3924755789189));
#117179=CARTESIAN_POINT('Ctrl Pts',(19.1317186250454,9.91074282631757,57.3975188596239));
#117180=CARTESIAN_POINT('Ctrl Pts',(19.1423418240855,9.90693390618994,57.4026702453094));
#117181=CARTESIAN_POINT('Ctrl Pts',(19.1528625920286,9.90314781642201,57.4079254265304));
#117182=CARTESIAN_POINT('Ctrl Pts',(19.1910683050448,9.88939879544672,57.4270093894752));
#117183=CARTESIAN_POINT('Ctrl Pts',(19.2279196888839,9.87594969708246,57.4474595822681));
#117184=CARTESIAN_POINT('Ctrl Pts',(19.2633601514774,9.86288426186219,57.4690647053599));
#117185=CARTESIAN_POINT('Ctrl Pts',(19.2879038683567,9.8538360068597,57.4840269825285));
#117186=CARTESIAN_POINT('Ctrl Pts',(19.3117719511216,9.84497216265779,57.4995438337743));
#117187=CARTESIAN_POINT('Ctrl Pts',(19.3349570005266,9.83632379875053,57.5155533891061));
#117188=CARTESIAN_POINT('Ctrl Pts',(19.3504611502475,9.83054052322165,57.5262591908706));
#117189=CARTESIAN_POINT('Ctrl Pts',(19.3656621190298,9.82483923989344,57.5371869700974));
#117190=CARTESIAN_POINT('Ctrl Pts',(19.3805545544829,9.81921869377156,57.5483160349634));
#117191=CARTESIAN_POINT('Ctrl Pts',(19.4145014659596,9.8064068080158,57.5736844430398));
#117192=CARTESIAN_POINT('Ctrl Pts',(19.4468420661731,9.79401353306645,57.6000969576853));
#117193=CARTESIAN_POINT('Ctrl Pts',(19.4775552412542,9.78202389464304,57.6273208358166));
#117194=CARTESIAN_POINT('Ctrl Pts',(19.5077497374716,9.7702367351889,57.6540849617362));
#117195=CARTESIAN_POINT('Ctrl Pts',(19.5363719187633,9.75884011241947,57.6816332563403));
#117196=CARTESIAN_POINT('Ctrl Pts',(19.563444322055,9.74782565388447,57.7097684917865));
#117197=CARTESIAN_POINT('Ctrl Pts',(19.5924501923908,9.73602456062194,57.7399131000219));
#117198=CARTESIAN_POINT('Ctrl Pts',(19.6196776011776,9.72466241231091,57.7707303908133));
#117199=CARTESIAN_POINT('Ctrl Pts',(19.645181703832,9.71377420667168,57.8020131219249));
#117200=CARTESIAN_POINT('Ctrl Pts',(19.6509595334378,9.71130753698532,57.8091000715193));
#117201=CARTESIAN_POINT('Ctrl Pts',(19.6566490582282,9.70886518326726,57.816211069799));
#117202=CARTESIAN_POINT('Ctrl Pts',(19.6622511520499,9.70644752473145,57.823343979969));
#117203=CARTESIAN_POINT('Ctrl Pts',(19.6773116371737,9.69994797089116,57.8425198615096));
#117204=CARTESIAN_POINT('Ctrl Pts',(19.6917339583362,9.69361877354101,57.8618463008517));
#117205=CARTESIAN_POINT('Ctrl Pts',(19.7055337051702,9.68745455567342,57.8812762234864));
#117206=CARTESIAN_POINT('Ctrl Pts',(19.7284229573522,9.67723014076388,57.913504090013));
#117207=CARTESIAN_POINT('Ctrl Pts',(19.7495978658298,9.6674605475487,57.9460143695294));
#117208=CARTESIAN_POINT('Ctrl Pts',(19.7691396514823,9.65815512299354,57.9786127487493));
#117209=CARTESIAN_POINT('Ctrl Pts',(19.7845013999463,9.65084015219668,58.0042382525192));
#117210=CARTESIAN_POINT('Ctrl Pts',(19.7988547861705,9.64381178723341,58.0299190632408));
#117211=CARTESIAN_POINT('Ctrl Pts',(19.8122520110905,9.63706604159557,58.055577334875));
#117212=CARTESIAN_POINT('Ctrl Pts',(19.8293686065232,9.6284475254727,58.0883589189483));
#117213=CARTESIAN_POINT('Ctrl Pts',(19.8449239825892,9.62029165568125,58.1211021915863));
#117214=CARTESIAN_POINT('Ctrl Pts',(19.8590233443336,9.61261841013919,58.1536519928569));
#117215=CARTESIAN_POINT('Ctrl Pts',(19.8695982291186,9.60686327816901,58.1780651829325));
#117216=CARTESIAN_POINT('Ctrl Pts',(19.8793545690103,9.60137903712872,58.202370450052));
#117217=CARTESIAN_POINT('Ctrl Pts',(19.8883433273238,9.59616278333,58.2265163526361));
#117218=CARTESIAN_POINT('Ctrl Pts',(19.9001508647372,9.58931076776362,58.2582341537162));
#117219=CARTESIAN_POINT('Ctrl Pts',(19.9106335214388,9.58292271136002,58.2896751695036));
#117220=CARTESIAN_POINT('Ctrl Pts',(19.9199000760921,9.57700602057025,58.3207104461368));
#117221=CARTESIAN_POINT('Ctrl Pts',(19.9269921362974,9.57247774346322,58.3444629689037));
#117222=CARTESIAN_POINT('Ctrl Pts',(19.9333722047035,9.56822479168832,58.3679787526273));
#117223=CARTESIAN_POINT('Ctrl Pts',(19.9390931750267,9.56423707813824,58.3912149749821));
#117224=CARTESIAN_POINT('Ctrl Pts',(19.9463972232821,9.55914590469158,58.4208810071001));
#117225=CARTESIAN_POINT('Ctrl Pts',(19.9526268159925,9.55448824756716,58.4500894277211));
#117226=CARTESIAN_POINT('Ctrl Pts',(19.9578906509278,9.55024207996741,58.4787308390512));
#117227=CARTESIAN_POINT('Ctrl Pts',(19.9585443021874,9.54971480036342,58.4822874655076));
#117228=CARTESIAN_POINT('Ctrl Pts',(19.9591830680236,9.54919382674418,58.4858354008373));
#117229=CARTESIAN_POINT('Ctrl Pts',(19.9598071616935,9.54867908433721,58.4893744789377));
#117230=CARTESIAN_POINT('',(19.0913779940088,8.6460405135737,58.2486549879977));
#117231=CARTESIAN_POINT('Ctrl Pts',(19.0913780598671,8.64604000277229,58.2486547535097));
#117232=CARTESIAN_POINT('Ctrl Pts',(19.0954302009912,8.66285126361277,58.213171559027));
#117233=CARTESIAN_POINT('Ctrl Pts',(19.0988408317573,8.68159370027269,58.176982504357));
#117234=CARTESIAN_POINT('Ctrl Pts',(19.1015351597539,8.70248101758052,58.1403385759788));
#117235=CARTESIAN_POINT('Ctrl Pts',(19.1041640143191,8.72286076330142,58.1045851122115));
#117236=CARTESIAN_POINT('Ctrl Pts',(19.1061109304425,8.74528295029375,58.0683986435903));
#117237=CARTESIAN_POINT('Ctrl Pts',(19.1072942385465,8.76992764012634,58.0320567084334));
#117238=CARTESIAN_POINT('Ctrl Pts',(19.1084368662561,8.79372508172332,57.9969641556242));
#117239=CARTESIAN_POINT('Ctrl Pts',(19.1088674197003,8.81959529261079,57.9617268250813));
#117240=CARTESIAN_POINT('Ctrl Pts',(19.1085015617408,8.8476758943756,57.9266348400689));
#117241=CARTESIAN_POINT('Ctrl Pts',(19.1081426901077,8.87522027642978,57.8922129622787));
#117242=CARTESIAN_POINT('Ctrl Pts',(19.1070174722854,8.90489192584823,57.8579310879301));
#117243=CARTESIAN_POINT('Ctrl Pts',(19.1050366211492,8.93678978933392,57.8241001163336));
#117244=CARTESIAN_POINT('Ctrl Pts',(19.1031111812215,8.96779536004109,57.7912155131877));
#117245=CARTESIAN_POINT('Ctrl Pts',(19.1003772169515,9.00090472545617,57.7587572142995));
#117246=CARTESIAN_POINT('Ctrl Pts',(19.096744615821,9.03617293713031,57.727042886517));
#117247=CARTESIAN_POINT('Ctrl Pts',(19.0943428289093,9.05949141503571,57.7060741496127));
#117248=CARTESIAN_POINT('Ctrl Pts',(19.0915480345517,9.08375290262299,57.685431298777));
#117249=CARTESIAN_POINT('Ctrl Pts',(19.0883324721565,9.10896303915117,57.665213240763));
#117250=CARTESIAN_POINT('Ctrl Pts',(19.0836454651811,9.14570935946355,57.6357433791046));
#117251=CARTESIAN_POINT('Ctrl Pts',(19.0780646694153,9.18447336932474,57.6071751849723));
#117252=CARTESIAN_POINT('Ctrl Pts',(19.0714997588372,9.2252361160707,57.5798340720463));
#117253=CARTESIAN_POINT('Ctrl Pts',(19.0650441419727,9.26532023788887,57.5529481384756));
#117254=CARTESIAN_POINT('Ctrl Pts',(19.057636789312,9.30733741658159,57.5272491409521));
#117255=CARTESIAN_POINT('Ctrl Pts',(19.0491882101566,9.35122280768896,57.5030640999627));
#117256=CARTESIAN_POINT('Ctrl Pts',(19.0409254270953,9.39414309755229,57.4794109219136));
#117257=CARTESIAN_POINT('Ctrl Pts',(19.0316665837391,9.43885053921676,57.457206268645));
#117258=CARTESIAN_POINT('Ctrl Pts',(19.021326269496,9.48523556076868,57.4367671620351));
#117259=CARTESIAN_POINT('Ctrl Pts',(19.0198671000966,9.49178116493962,57.4338829055015));
#117260=CARTESIAN_POINT('Ctrl Pts',(19.0183863940477,9.4983600912586,57.4310338190697));
#117261=CARTESIAN_POINT('Ctrl Pts',(19.0168839108807,9.50497194766504,57.4282208040115));
#117262=CARTESIAN_POINT('Ctrl Pts',(19.0065288051913,9.5505408255026,57.4088335197662));
#117263=CARTESIAN_POINT('Ctrl Pts',(18.9951392061905,9.59767797885603,57.3911594931486));
#117264=CARTESIAN_POINT('Ctrl Pts',(18.9826423348366,9.64622838184959,57.3754959660479));
#117265=CARTESIAN_POINT('Ctrl Pts',(18.970337340225,9.6940333428125,57.3600729364658));
#117266=CARTESIAN_POINT('Ctrl Pts',(18.9569586843622,9.74320860365135,57.3465995994608));
#117267=CARTESIAN_POINT('Ctrl Pts',(18.9424390835605,9.79355619944309,57.3353571391542));
#117268=CARTESIAN_POINT('Ctrl Pts',(18.9282301475949,9.84282654608677,57.3243552252052));
#117269=CARTESIAN_POINT('Ctrl Pts',(18.9129284431077,9.89321958803115,57.3154902019306));
#117270=CARTESIAN_POINT('Ctrl Pts',(18.8964748979544,9.9445008817099,57.309016397297));
#117271=CARTESIAN_POINT('Ctrl Pts',(18.8905744661776,9.96289094731345,57.3066948160073));
#117272=CARTESIAN_POINT('Ctrl Pts',(18.8845259520051,9.98139478071069,57.3046806302731));
#117273=CARTESIAN_POINT('Ctrl Pts',(18.8783268084,10.,57.3029850935068));
#117274=CARTESIAN_POINT('Origin',(18.9749992656191,9.54868042581501,58.66301925565));
#117275=CARTESIAN_POINT('Ctrl Pts',(18.5706725300191,8.81765680955601,58.08301260777));
#117276=CARTESIAN_POINT('Ctrl Pts',(18.5857598980191,8.75765050426302,58.16857732362));
#117277=CARTESIAN_POINT('Ctrl Pts',(18.6277718770991,8.62602790954801,58.40683909675));
#117278=CARTESIAN_POINT('Ctrl Pts',(18.6885460064291,8.54234388419301,58.75150631155));
#117279=CARTESIAN_POINT('Ctrl Pts',(18.7326364903191,8.543692731993,59.00155587124));
#117280=CARTESIAN_POINT('Ctrl Pts',(18.7479295693691,8.55159287998601,59.0882872324));
#117281=CARTESIAN_POINT('Ctrl Pts',(19.4066515538591,8.59303798548101,57.77801712375));
#117282=CARTESIAN_POINT('Ctrl Pts',(19.4244719901391,8.52216007648402,57.87908184005));
#117283=CARTESIAN_POINT('Ctrl Pts',(19.4740138287791,8.36702838946302,58.16004756881));
#117284=CARTESIAN_POINT('Ctrl Pts',(19.5454018805591,8.26883637037401,58.56490932905));
#117285=CARTESIAN_POINT('Ctrl Pts',(19.5971457817591,8.27039928348501,58.85836357521));
#117286=CARTESIAN_POINT('Ctrl Pts',(19.6150981880091,8.27967362318701,58.96017673036));
#117287=CARTESIAN_POINT('Ctrl Pts',(20.1098257338891,9.12697886077701,58.02863494815));
#117288=CARTESIAN_POINT('Ctrl Pts',(20.1211494000291,9.08194381522401,58.09285465006));
#117289=CARTESIAN_POINT('Ctrl Pts',(20.1527920273191,8.98269553590501,58.27230890692));
#117290=CARTESIAN_POINT('Ctrl Pts',(20.1989497491491,8.91899043439601,58.53408235561));
#117291=CARTESIAN_POINT('Ctrl Pts',(20.2325007301691,8.92004449336401,58.72435942426));
#117292=CARTESIAN_POINT('Ctrl Pts',(20.2441316560191,8.92605224520602,58.79032168259));
#117293=CARTESIAN_POINT('Ctrl Pts',(19.9274540441491,9.84790099344701,58.5665821712));
#117294=CARTESIAN_POINT('Ctrl Pts',(19.9300058300991,9.83775874799601,58.58105406848));
#117295=CARTESIAN_POINT('Ctrl Pts',(19.9374811043791,9.81396373949001,58.62344845562));
#117296=CARTESIAN_POINT('Ctrl Pts',(19.9495730632891,9.79682256166901,58.69202536232));
#117297=CARTESIAN_POINT('Ctrl Pts',(19.9585601282791,9.79718957038302,58.74299354062));
#117298=CARTESIAN_POINT('Ctrl Pts',(19.9616558485791,9.79878680488901,58.76055024285));
#117299=CARTESIAN_POINT('',(19.0165386378691,8.5,58.89829442788));
#117300=CARTESIAN_POINT('Ctrl Pts',(19.0165386378691,8.5,58.89829442788));
#117301=CARTESIAN_POINT('Ctrl Pts',(19.032697313698,8.50000152435189,58.758360191488));
#117302=CARTESIAN_POINT('Ctrl Pts',(19.0473582025624,8.51918644290929,58.632939395879));
#117303=CARTESIAN_POINT('Ctrl Pts',(19.0723610486273,8.5742843133173,58.416069360015));
#117304=CARTESIAN_POINT('Ctrl Pts',(19.0827530892467,8.61013548696591,58.3244461106695));
#117305=CARTESIAN_POINT('Ctrl Pts',(19.0913779610791,8.64604076897401,58.24865510524));
#117306=CARTESIAN_POINT('Ctrl Pts',(19.0165386356542,8.50002857532344,58.8982944240715));
#117307=CARTESIAN_POINT('Ctrl Pts',(19.0471525139605,8.50003022814292,58.8928916452605));
#117308=CARTESIAN_POINT('Ctrl Pts',(19.0783619071455,8.50148345605102,58.8873852580101));
#117309=CARTESIAN_POINT('Ctrl Pts',(19.1099794394775,8.5045453023276,58.8818079404131));
#117310=CARTESIAN_POINT('Ctrl Pts',(19.1410879060831,8.50755785060767,58.8763204217671));
#117311=CARTESIAN_POINT('Ctrl Pts',(19.1725911301666,8.51212836874123,58.8707642981432));
#117312=CARTESIAN_POINT('Ctrl Pts',(19.2042713121879,8.51837713746225,58.8651776049256));
#117313=CARTESIAN_POINT('Ctrl Pts',(19.2352952562048,8.52449646628568,58.859706637066));
#117314=CARTESIAN_POINT('Ctrl Pts',(19.2664883366558,8.53222581446347,58.8542064515618));
#117315=CARTESIAN_POINT('Ctrl Pts',(19.297614759377,8.54164019590478,58.8487182728915));
#117316=CARTESIAN_POINT('Ctrl Pts',(19.3248593796421,8.54988050188843,58.8439145296166));
#117317=CARTESIAN_POINT('Ctrl Pts',(19.3520521700985,8.55941143136103,58.8391201186967));
#117318=CARTESIAN_POINT('Ctrl Pts',(19.3790206125476,8.57025382158666,58.8343652312728));
#117319=CARTESIAN_POINT('Ctrl Pts',(19.409325475612,8.58243758606239,58.8290220894677));
#117320=CARTESIAN_POINT('Ctrl Pts',(19.4393468014256,8.59627864031572,58.8237288999887));
#117321=CARTESIAN_POINT('Ctrl Pts',(19.468829263876,8.61175911113363,58.8185306779929));
#117322=CARTESIAN_POINT('Ctrl Pts',(19.4978600974361,8.62700244341984,58.8134120852762));
#117323=CARTESIAN_POINT('Ctrl Pts',(19.5263676033458,8.643835338317,58.8083857221369));
#117324=CARTESIAN_POINT('Ctrl Pts',(19.5541087839704,8.66218968833763,58.8034944312797));
#117325=CARTESIAN_POINT('Ctrl Pts',(19.5817057332889,8.68044861084528,58.7986285711091));
#117326=CARTESIAN_POINT('Ctrl Pts',(19.6085434726281,8.70021302554924,58.7938965291188));
#117327=CARTESIAN_POINT('Ctrl Pts',(19.6343960913359,8.7213663065163,58.7893381365852));
#117328=CARTESIAN_POINT('Ctrl Pts',(19.6601785398842,8.74246217244482,58.7847921166137));
#117329=CARTESIAN_POINT('Ctrl Pts',(19.6849804499355,8.76493896360552,58.780418938428));
#117330=CARTESIAN_POINT('Ctrl Pts',(19.7086029926765,8.7886360079756,58.7762536596547));
#117331=CARTESIAN_POINT('Ctrl Pts',(19.7331398265837,8.81325022703638,58.7719271671786));
#117332=CARTESIAN_POINT('Ctrl Pts',(19.7564032709207,8.83918055026988,58.7678251484334));
#117333=CARTESIAN_POINT('Ctrl Pts',(19.7782114202349,8.86620434281197,58.763979678758));
#117334=CARTESIAN_POINT('Ctrl Pts',(19.7993118639889,8.89235117472967,58.7602590000601));
#117335=CARTESIAN_POINT('Ctrl Pts',(19.8190497488021,8.91952067586753,58.756778522324));
#117336=CARTESIAN_POINT('Ctrl Pts',(19.8373056309835,8.94748353013081,58.7535593088364));
#117337=CARTESIAN_POINT('Ctrl Pts',(19.8564799622845,8.97685318898586,58.7501781374787));
#117338=CARTESIAN_POINT('Ctrl Pts',(19.8740187726101,9.00709715222103,58.7470852943527));
#117339=CARTESIAN_POINT('Ctrl Pts',(19.8898418485087,9.03793256084594,58.744294927503));
#117340=CARTESIAN_POINT('Ctrl Pts',(19.9056649244073,9.06876796947085,58.7415045606532));
#117341=CARTESIAN_POINT('Ctrl Pts',(19.9197724007878,9.10019375962582,58.739016646318));
#117342=CARTESIAN_POINT('Ctrl Pts',(19.9321441024897,9.13192558069005,58.7368347476417));
#117343=CARTESIAN_POINT('Ctrl Pts',(19.9443565817857,9.16324901679515,58.7346809297554));
#117344=CARTESIAN_POINT('Ctrl Pts',(19.9548782145085,9.19486980610647,58.7328253088665));
#117345=CARTESIAN_POINT('Ctrl Pts',(19.963742894296,9.22652726318772,58.7312616983276));
#117346=CARTESIAN_POINT('Ctrl Pts',(19.9727144348331,9.25856634032482,58.7296792389867));
#117347=CARTESIAN_POINT('Ctrl Pts',(19.9799893524906,9.29064224036267,58.7283957810469));
#117348=CARTESIAN_POINT('Ctrl Pts',(19.9856502178946,9.32251004117483,58.7273966395878));
#117349=CARTESIAN_POINT('Ctrl Pts',(19.9914529813404,9.35517665598586,58.7263724531566));
#117350=CARTESIAN_POINT('Ctrl Pts',(19.9955603937584,9.38762397511958,58.725646904131));
#117351=CARTESIAN_POINT('Ctrl Pts',(19.9981021899527,9.41962530702886,58.725197077525));
#117352=CARTESIAN_POINT('Ctrl Pts',(20.0002586629659,9.44677540222559,58.7248154423103));
#117353=CARTESIAN_POINT('Ctrl Pts',(20.0012891940811,9.47360506846782,58.7246320997432));
#117354=CARTESIAN_POINT('Ctrl Pts',(20.0012895469767,9.5,58.7246301887192));
#117355=CARTESIAN_POINT('Origin',(17.6260947381591,9.5,51.01300153266));
#117356=CARTESIAN_POINT('',(20.2047121520095,8.50000000009378,65.6369887302606));
#117357=CARTESIAN_POINT('',(17.6261082242393,8.50000000009378,51.0129991547002));
#117358=CARTESIAN_POINT('Origin',(20.2046986659293,9.5,65.6369911082204));
#117359=CARTESIAN_POINT('Origin',(11.833832765324,1.4210854715202E-14,67.1130006183894));
#117360=CARTESIAN_POINT('',(-6.53751764820717,8.5,70.352365368344));
#117361=CARTESIAN_POINT('',(14.8833738632635,20.2647763420359,66.5752842440434));
#117362=CARTESIAN_POINT('Origin',(11.833832765324,1.4210854715202E-14,67.1130006183894));
#117363=CARTESIAN_POINT('Ctrl Pts',(14.8833738632635,20.2647763420359,66.5752842440434));
#117364=CARTESIAN_POINT('Ctrl Pts',(15.4158628606723,19.5539773651717,66.4813920668699));
#117365=CARTESIAN_POINT('Ctrl Pts',(16.038207564819,18.9155234339931,66.3716559042235));
#117366=CARTESIAN_POINT('Ctrl Pts',(17.4246863278478,17.8184518326642,66.1271822901222));
#117367=CARTESIAN_POINT('Ctrl Pts',(18.1846649332837,17.362577725361,65.9931775572271));
#117368=CARTESIAN_POINT('Ctrl Pts',(18.9921125713384,17.0122606549179,65.8508027531287));
#117369=CARTESIAN_POINT('',(13.0648424565899,8.5,66.8959403963056));
#117370=CARTESIAN_POINT('Ctrl Pts',(9.05563024203908,19.74193612938,82.8694660886069));
#117371=CARTESIAN_POINT('Ctrl Pts',(9.2912870723891,19.69133710775,82.83982404191));
#117372=CARTESIAN_POINT('Ctrl Pts',(9.83390957824909,19.60771562075,82.7775183021509));
#117373=CARTESIAN_POINT('Ctrl Pts',(10.6924944126191,19.60610480474,82.6968208510499));
#117374=CARTESIAN_POINT('Ctrl Pts',(11.5835752842391,19.781355271,82.6295254022679));
#117375=CARTESIAN_POINT('Ctrl Pts',(12.3817632835191,20.13187242782,82.5800473343639));
#117376=CARTESIAN_POINT('Ctrl Pts',(13.0117456051291,20.6231476854,82.5470281941081));
#117377=CARTESIAN_POINT('Ctrl Pts',(13.3279861775891,21.03846780615,82.531891260602));
#117378=CARTESIAN_POINT('Ctrl Pts',(13.4400188950291,21.23364550312,82.5267141025));
#117379=CARTESIAN_POINT('Ctrl Pts',(9.04014179690909,20.62748100547,82.628890445775));
#117380=CARTESIAN_POINT('Ctrl Pts',(9.23810271641909,20.56703465702,82.565394916618));
#117381=CARTESIAN_POINT('Ctrl Pts',(9.69456866260909,20.45181847571,82.4295851276741));
#117382=CARTESIAN_POINT('Ctrl Pts',(10.4233163549891,20.36853097734,82.247768026541));
#117383=CARTESIAN_POINT('Ctrl Pts',(11.1933906349991,20.42297948124,82.0910063111319));
#117384=CARTESIAN_POINT('Ctrl Pts',(11.8996157831891,20.6330481663,81.9727340922851));
#117385=CARTESIAN_POINT('Ctrl Pts',(12.4721764120891,20.9837092188,81.892563066293));
#117386=CARTESIAN_POINT('Ctrl Pts',(12.7663175887191,21.30635661408,81.856049847967));
#117387=CARTESIAN_POINT('Ctrl Pts',(12.8712405032191,21.46181296005,81.843530263153));
#117388=CARTESIAN_POINT('Ctrl Pts',(9.1754164244991,21.25111488499,83.28851033235));
#117389=CARTESIAN_POINT('Ctrl Pts',(9.34795109475909,21.22160961919,83.2009960512001));
#117390=CARTESIAN_POINT('Ctrl Pts',(9.73650325255911,21.16897699452,83.0088184827001));
#117391=CARTESIAN_POINT('Ctrl Pts',(10.3245724089391,21.14747847135,82.736721724997));
#117392=CARTESIAN_POINT('Ctrl Pts',(10.9117626573691,21.21052731484,82.487715195758));
#117393=CARTESIAN_POINT('Ctrl Pts',(11.4233081317791,21.36219444676,82.2900975756531));
#117394=CARTESIAN_POINT('Ctrl Pts',(11.8193955837191,21.58897637511,82.150986996173));
#117395=CARTESIAN_POINT('Ctrl Pts',(12.0160830794091,21.78731661116,82.086898923722));
#117396=CARTESIAN_POINT('Ctrl Pts',(12.0855867709291,21.88149337789,82.0647837904481));
#117397=CARTESIAN_POINT('Ctrl Pts',(9.31664801360909,20.94526249146,84.14222888187));
#117398=CARTESIAN_POINT('Ctrl Pts',(9.50324388522909,20.95436551881,84.06624169837));
#117399=CARTESIAN_POINT('Ctrl Pts',(9.9148240365791,20.99150149227,83.89517208715));
#117400=CARTESIAN_POINT('Ctrl Pts',(10.5019640432991,21.10911496024,83.6402764497801));
#117401=CARTESIAN_POINT('Ctrl Pts',(11.0401629057291,21.30096012362,83.39499096567));
#117402=CARTESIAN_POINT('Ctrl Pts',(11.4627087352791,21.538789162,83.19241279179));
#117403=CARTESIAN_POINT('Ctrl Pts',(11.7521790465591,21.79103472492,83.04566744004));
#117404=CARTESIAN_POINT('Ctrl Pts',(11.8803788675091,21.9664992403,82.977323729301));
#117405=CARTESIAN_POINT('Ctrl Pts',(11.9240687861891,22.04343555306,82.953631578989));
#117406=CARTESIAN_POINT('',(9.2477991596469,20.0000000010953,82.8003500634525));
#117407=CARTESIAN_POINT('',(9.42147268300909,20.99999557355,83.78518826663));
#117408=CARTESIAN_POINT('Origin',(9.42146753586009,19.9999823863366,83.7851933307501));
#117409=CARTESIAN_POINT('Ctrl Pts',(9.42147268300909,20.99999557355,83.78518826663));
#117410=CARTESIAN_POINT('Ctrl Pts',(9.55304779465049,20.9999809750948,83.7291788487243));
#117411=CARTESIAN_POINT('Ctrl Pts',(9.90914050500111,21.0105650864534,83.5772223250782));
#117412=CARTESIAN_POINT('Ctrl Pts',(10.4545613751438,21.0771645183637,83.343573390357));
#117413=CARTESIAN_POINT('Ctrl Pts',(11.0175584794691,21.2301198695261,83.1023167131314));
#117414=CARTESIAN_POINT('Ctrl Pts',(11.4774912323362,21.4455062539072,82.9056378798363));
#117415=CARTESIAN_POINT('Ctrl Pts',(11.7701254599278,21.6678362651009,82.7808538677759));
#117416=CARTESIAN_POINT('Ctrl Pts',(11.9020761286329,21.8153229542896,82.7246877181993));
#117417=CARTESIAN_POINT('Ctrl Pts',(11.9367286423891,21.85927935059,82.709938120253));
#117418=CARTESIAN_POINT('Ctrl Pts',(9.24780017804999,20.0000000009406,82.8003558393504));
#117419=CARTESIAN_POINT('Ctrl Pts',(9.41381134930932,20.0000101594718,82.7710848429586));
#117420=CARTESIAN_POINT('Ctrl Pts',(9.57682815077475,20.0068943525989,82.7423593667788));
#117421=CARTESIAN_POINT('Ctrl Pts',(9.73685811767206,20.0206313648514,82.714153161567));
#117422=CARTESIAN_POINT('Ctrl Pts',(9.75787737369477,20.0224356630283,82.7104483963892));
#117423=CARTESIAN_POINT('Ctrl Pts',(9.77884511234476,20.0243582057448,82.706752604443));
#117424=CARTESIAN_POINT('Ctrl Pts',(9.79976062639953,20.0264001910967,82.7030658937577));
#117425=CARTESIAN_POINT('Ctrl Pts',(9.90991246820188,20.0371543349761,82.6836497813391));
#117426=CARTESIAN_POINT('Ctrl Pts',(10.0186334701653,20.0511934060788,82.6644820073428));
#117427=CARTESIAN_POINT('Ctrl Pts',(10.1259182750038,20.0685190477532,82.6455641010232));
#117428=CARTESIAN_POINT('Ctrl Pts',(10.1502333775788,20.0724457431983,82.6412765336146));
#117429=CARTESIAN_POINT('Ctrl Pts',(10.1744749114995,20.076541190263,82.6370017847766));
#117430=CARTESIAN_POINT('Ctrl Pts',(10.1986431558949,20.0808053197147,82.6327398452152));
#117431=CARTESIAN_POINT('Ctrl Pts',(10.2225046454665,20.0850153268124,82.6285320002127));
#117432=CARTESIAN_POINT('Ctrl Pts',(10.2467930053505,20.0894810818087,82.6242487629126));
#117433=CARTESIAN_POINT('Ctrl Pts',(10.2706890022724,20.0940576724294,82.6200346565755));
#117434=CARTESIAN_POINT('Ctrl Pts',(10.2904577504564,20.0978438073128,82.6165483987194));
#117435=CARTESIAN_POINT('Ctrl Pts',(10.3099580439718,20.1017048020977,82.613109442041));
#117436=CARTESIAN_POINT('Ctrl Pts',(10.3287297773731,20.1055318013188,82.6097989607847));
#117437=CARTESIAN_POINT('Ctrl Pts',(10.4121350942416,20.1225356696282,82.5950900507299));
#117438=CARTESIAN_POINT('Ctrl Pts',(10.4940463096557,20.1415290275566,82.5806445104727));
#117439=CARTESIAN_POINT('Ctrl Pts',(10.5745125079426,20.1624361396842,82.5664572751468));
#117440=CARTESIAN_POINT('Ctrl Pts',(10.6687093560787,20.1869108148641,82.5498491480088));
#117441=CARTESIAN_POINT('Ctrl Pts',(10.7609229035475,20.2140105162765,82.5335947896854));
#117442=CARTESIAN_POINT('Ctrl Pts',(10.8511148020616,20.2437803092907,82.5176937523984));
#117443=CARTESIAN_POINT('Ctrl Pts',(10.9136822460994,20.2644320517324,82.5066629694014));
#117444=CARTESIAN_POINT('Ctrl Pts',(10.975278171351,20.2863680756695,82.4958022140613));
#117445=CARTESIAN_POINT('Ctrl Pts',(11.0359035648296,20.3095996373692,82.4851115273486));
#117446=CARTESIAN_POINT('Ctrl Pts',(11.0675766555811,20.3217367192056,82.4795262920038));
#117447=CARTESIAN_POINT('Ctrl Pts',(11.0993314772997,20.3343588413361,82.4739263564523));
#117448=CARTESIAN_POINT('Ctrl Pts',(11.1307220159251,20.3473028790355,82.4683906090922));
#117449=CARTESIAN_POINT('Ctrl Pts',(11.1619517472033,20.3601806070615,82.4628832202403));
#117450=CARTESIAN_POINT('Ctrl Pts',(11.1928207334175,20.3733769581208,82.4574394030529));
#117451=CARTESIAN_POINT('Ctrl Pts',(11.2229069821298,20.3866822567242,82.4521339013917));
#117452=CARTESIAN_POINT('Ctrl Pts',(11.2334477503644,20.3913437906434,82.4502751098915));
#117453=CARTESIAN_POINT('Ctrl Pts',(11.2438926075315,20.3960182581678,82.4484332669831));
#117454=CARTESIAN_POINT('Ctrl Pts',(11.2542239598114,20.4006952414998,82.4466114892795));
#117455=CARTESIAN_POINT('Ctrl Pts',(11.2700155143389,20.407844047901,82.4438268875));
#117456=CARTESIAN_POINT('Ctrl Pts',(11.2857053529294,20.4150750395933,82.4410603493937));
#117457=CARTESIAN_POINT('Ctrl Pts',(11.3012948100236,20.4223871806256,82.4383117024514));
#117458=CARTESIAN_POINT('Ctrl Pts',(11.3716798206214,20.4554008462678,82.4259018062634));
#117459=CARTESIAN_POINT('Ctrl Pts',(11.4400135594739,20.4900689328506,82.4138566940165));
#117460=CARTESIAN_POINT('Ctrl Pts',(11.5062760631553,20.5263935357958,82.4021735431031));
#117461=CARTESIAN_POINT('Ctrl Pts',(11.5544472188273,20.5528005987044,82.3936801893944));
#117462=CARTESIAN_POINT('Ctrl Pts',(11.6015252661522,20.5800829070673,82.3853780955072));
#117463=CARTESIAN_POINT('Ctrl Pts',(11.647519334929,20.6082432514823,82.3772659700509));
#117464=CARTESIAN_POINT('Ctrl Pts',(11.6951740296187,20.6374203312917,82.3688609545306));
#117465=CARTESIAN_POINT('Ctrl Pts',(11.741809545569,20.6676409430077,82.3606344338639));
#117466=CARTESIAN_POINT('Ctrl Pts',(11.7872463267942,20.6987950811283,82.3526204474684));
#117467=CARTESIAN_POINT('Ctrl Pts',(11.8263526434061,20.7256086791928,82.3457230070941));
#117468=CARTESIAN_POINT('Ctrl Pts',(11.8645714129522,20.7531131352691,82.338982978887));
#117469=CARTESIAN_POINT('Ctrl Pts',(11.9018088960741,20.7812154666837,82.3324193291663));
#117470=CARTESIAN_POINT('Ctrl Pts',(11.9332265859284,20.8049257246964,82.3268815029238));
#117471=CARTESIAN_POINT('Ctrl Pts',(11.9639454805571,20.8290611782182,82.3214692070529));
#117472=CARTESIAN_POINT('Ctrl Pts',(11.9938802796988,20.8535531845223,82.3161950225982));
#117473=CARTESIAN_POINT('Ctrl Pts',(12.0432245216299,20.8939255778271,82.3075011064474));
#117474=CARTESIAN_POINT('Ctrl Pts',(12.0904669901627,20.935294926462,82.2991770861494));
#117475=CARTESIAN_POINT('Ctrl Pts',(12.1356130952059,20.9776340615505,82.2912177691209));
#117476=CARTESIAN_POINT('Ctrl Pts',(12.1835950663075,21.0226327420422,82.2827584852184));
#117477=CARTESIAN_POINT('Ctrl Pts',(12.2292104629269,21.0687261422084,82.2747110466225));
#117478=CARTESIAN_POINT('Ctrl Pts',(12.2725058106192,21.1159255274227,82.2670693314398));
#117479=CARTESIAN_POINT('Ctrl Pts',(12.3043664816712,21.1506591458444,82.2614458594807));
#117480=CARTESIAN_POINT('Ctrl Pts',(12.3349716875747,21.1859926223862,82.2560420928028));
#117481=CARTESIAN_POINT('Ctrl Pts',(12.3643457345344,21.2219474207367,82.2508562354651));
#117482=CARTESIAN_POINT('Ctrl Pts',(12.4000777563314,21.2656845891333,82.2445479059497));
#117483=CARTESIAN_POINT('Ctrl Pts',(12.4339866756333,21.3103385304835,82.238562052063));
#117484=CARTESIAN_POINT('Ctrl Pts',(12.4659848864984,21.3558676724476,82.232913638037));
#117485=CARTESIAN_POINT('Ctrl Pts',(12.4836712988028,21.3810330537258,82.2297915828773));
#117486=CARTESIAN_POINT('Ctrl Pts',(12.5007742972253,21.4064667735531,82.226772634051));
#117487=CARTESIAN_POINT('Ctrl Pts',(12.5172801388854,21.4321684410533,82.2238595693975));
#117488=CARTESIAN_POINT('Origin',(-7.20566857569291,10.,84.1784376645));
#117489=CARTESIAN_POINT('',(-4.19330934979995,8.50000005802184,83.6470312449829));
#117490=CARTESIAN_POINT('',(-3.1851014235548,10.,84.9926431156514));
#117491=CARTESIAN_POINT('Ctrl Pts',(-4.19330934571277,8.50000001959754,
83.6470312442563));
#117492=CARTESIAN_POINT('Ctrl Pts',(-4.19329531627948,8.50000000653218,
83.6471108434094));
#117493=CARTESIAN_POINT('Ctrl Pts',(-4.19328128427642,8.5,83.6471904399934));
#117494=CARTESIAN_POINT('Ctrl Pts',(-4.15980554940295,8.5,83.8370407665797));
#117495=CARTESIAN_POINT('Ctrl Pts',(-4.10685468483148,8.53950345297412,
84.0345242483906));
#117496=CARTESIAN_POINT('Ctrl Pts',(-3.97184256650876,8.6947907400348,84.3859356237976));
#117497=CARTESIAN_POINT('Ctrl Pts',(-3.88961764476103,8.81043822068695,
84.5398608579619));
#117498=CARTESIAN_POINT('Ctrl Pts',(-3.71525661408043,9.07833587624806,
84.7811467125873));
#117499=CARTESIAN_POINT('Ctrl Pts',(-3.61058564106113,9.25135231079439,
84.879888801679));
#117500=CARTESIAN_POINT('Ctrl Pts',(-3.3954856573262,9.62155435638349,84.9943545575053));
#117501=CARTESIAN_POINT('Ctrl Pts',(-3.2849218663493,9.8186103084606,85.0102441529475));
#117502=CARTESIAN_POINT('Ctrl Pts',(-3.18510142355393,10.,84.9926431156565));
#117503=CARTESIAN_POINT('',(-6.8072945652419,8.50000000000004,84.1081934943927));
#117504=CARTESIAN_POINT('',(-6.80729512863291,8.5,84.10819367738));
#117505=CARTESIAN_POINT('',(-6.54682286425215,10.,85.5854053072757));
#117506=CARTESIAN_POINT('Origin',(-6.80729512863291,10.,84.10819367738));
#117507=CARTESIAN_POINT('',(-6.94519630919256,10.,85.6556492940183));
#117508=CARTESIAN_POINT('Origin',(11.833832765324,1.4210854715202E-14,67.1130006183894));
#117509=CARTESIAN_POINT('',(-6.53751764820717,8.5,70.352365368344));
#117510=CARTESIAN_POINT('',(13.3597592683937,20.4707111483689,82.0753376302183));
#117511=CARTESIAN_POINT('Origin',(14.4385554303262,1.4210854715202E-14,
81.8851169135651));
#117512=CARTESIAN_POINT('',(15.1826200703325,20.4790215093801,80.7654567789229));
#117513=CARTESIAN_POINT('Ctrl Pts',(13.3597592422362,20.4707111483689,82.0753374818706));
#117514=CARTESIAN_POINT('Ctrl Pts',(13.5489200678292,20.4809897643711,82.0419835619616));
#117515=CARTESIAN_POINT('Ctrl Pts',(13.7352332109664,20.4885496274001,81.9876000411839));
#117516=CARTESIAN_POINT('Ctrl Pts',(14.0953296708824,20.4982351765127,81.841707426555));
#117517=CARTESIAN_POINT('Ctrl Pts',(14.2709193683375,20.5002927571102,81.7485872067569));
#117518=CARTESIAN_POINT('Ctrl Pts',(14.6067578621981,20.4996156846239,81.5206315743113));
#117519=CARTESIAN_POINT('Ctrl Pts',(14.7693220761259,20.4964642438232,81.3803787318923));
#117520=CARTESIAN_POINT('Ctrl Pts',(15.0202379695866,20.4881014789292,81.0852130979036));
#117521=CARTESIAN_POINT('Ctrl Pts',(15.1191031310536,20.4831599384662,80.9316197555286));
#117522=CARTESIAN_POINT('Ctrl Pts',(15.1826197616608,20.4790215522793,80.7654566598632));
#117523=CARTESIAN_POINT('Ctrl Pts',(15.9984193009007,20.3875466887266,78.3830201467867));
#117524=CARTESIAN_POINT('Ctrl Pts',(15.8770688204797,20.4073988582131,78.7818268437993));
#117525=CARTESIAN_POINT('Ctrl Pts',(15.7502010071011,20.4250600452808,79.1746414174431));
#117526=CARTESIAN_POINT('Ctrl Pts',(15.6182044599264,20.4401531721352,79.5610824354396));
#117527=CARTESIAN_POINT('Ctrl Pts',(15.549503107267,20.4480088187635,79.7622166410514));
#117528=CARTESIAN_POINT('Ctrl Pts',(15.4794122215352,20.4551693893405,79.9616248643147));
#117529=CARTESIAN_POINT('Ctrl Pts',(15.4079854932393,20.4615855988943,80.1592571638601));
#117530=CARTESIAN_POINT('Ctrl Pts',(15.3342663988258,20.4682077299811,80.3632322652954));
#117531=CARTESIAN_POINT('Ctrl Pts',(15.2591243512077,20.4740369355328,80.5653156100083));
#117532=CARTESIAN_POINT('Ctrl Pts',(15.1826202858407,20.4790215304872,80.7654568607777));
#117533=CARTESIAN_POINT('Ctrl Pts',(14.8833738632635,20.2647763420359,66.5752842440434));
#117534=CARTESIAN_POINT('Ctrl Pts',(15.0733159401335,20.2477695588669,67.0115691027874));
#117535=CARTESIAN_POINT('Ctrl Pts',(15.2555091649434,20.23108766834,67.4513545027359));
#117536=CARTESIAN_POINT('Ctrl Pts',(15.4297724903522,20.2151317187521,67.8942334785676));
#117537=CARTESIAN_POINT('Ctrl Pts',(15.4928256588264,20.2093584260918,68.0544790300126));
#117538=CARTESIAN_POINT('Ctrl Pts',(15.5548406861411,20.2036796842702,68.2151295830088));
#117539=CARTESIAN_POINT('Ctrl Pts',(15.6158090592685,20.1981127976809,68.3761658484978));
#117540=CARTESIAN_POINT('Ctrl Pts',(12.6103939613991,23.39573848791,81.293275948705));
#117541=CARTESIAN_POINT('Ctrl Pts',(12.6301344989091,23.36712060978,81.286688115074));
#117542=CARTESIAN_POINT('Ctrl Pts',(12.8623544188791,23.03339800576,81.2092658486509));
#117543=CARTESIAN_POINT('Ctrl Pts',(13.3195155352191,22.43787252879,81.0584942952861));
#117544=CARTESIAN_POINT('Ctrl Pts',(14.0054384121691,21.66395729877,80.8371498110769));
#117545=CARTESIAN_POINT('Ctrl Pts',(14.6750728316091,20.99216918735,80.625783923235));
#117546=CARTESIAN_POINT('Ctrl Pts',(15.3162005729891,20.41109563502,80.4277322359629));
#117547=CARTESIAN_POINT('Ctrl Pts',(15.9201036787491,19.91127773927,80.245012905101));
#117548=CARTESIAN_POINT('Ctrl Pts',(16.4827047066491,19.4827933493,80.0780860889519));
#117549=CARTESIAN_POINT('Ctrl Pts',(17.0027455733291,19.11617373137,79.926546278835));
#117550=CARTESIAN_POINT('Ctrl Pts',(17.4804240494591,18.80293987069,79.789629873945));
#117551=CARTESIAN_POINT('Ctrl Pts',(17.9170466493591,18.53549113312,79.666341537588));
#117552=CARTESIAN_POINT('Ctrl Pts',(18.2457112148691,18.34670706214,79.574782208674));
#117553=CARTESIAN_POINT('Ctrl Pts',(18.4288583779791,18.24601358153,79.524208507212));
#117554=CARTESIAN_POINT('Ctrl Pts',(18.4788029562491,18.2188868654,79.510449919603));
#117555=CARTESIAN_POINT('Ctrl Pts',(12.4260057050691,23.15454775929,82.3416317744899));
#117556=CARTESIAN_POINT('Ctrl Pts',(12.4484290189691,23.12610953721,82.335556515214));
#117557=CARTESIAN_POINT('Ctrl Pts',(12.7119653073691,22.79485591383,82.264081173276));
#117558=CARTESIAN_POINT('Ctrl Pts',(13.2254892213291,22.21157537144,82.123130223133));
#117559=CARTESIAN_POINT('Ctrl Pts',(13.9832319374791,21.46817083564,81.911502389663));
#117560=CARTESIAN_POINT('Ctrl Pts',(14.7127953478491,20.83289001182,81.705550703378));
#117561=CARTESIAN_POINT('Ctrl Pts',(15.4031177402791,20.29055202507,81.509530462387));
#117562=CARTESIAN_POINT('Ctrl Pts',(16.0467726803191,19.82929174299,81.326377521192));
#117563=CARTESIAN_POINT('Ctrl Pts',(16.6411046175391,19.43781087338,81.1573453210401));
#117564=CARTESIAN_POINT('Ctrl Pts',(17.1862122875291,19.10591070303,81.0026466246689));
#117565=CARTESIAN_POINT('Ctrl Pts',(17.6834900333091,18.82474934939,80.861975064868));
#117566=CARTESIAN_POINT('Ctrl Pts',(18.1352802572891,18.58660771731,80.734659490498));
#117567=CARTESIAN_POINT('Ctrl Pts',(18.4735435632491,18.41979202888,80.639728546379));
#117568=CARTESIAN_POINT('Ctrl Pts',(18.6613901681291,18.33128071504,80.587171652487));
#117569=CARTESIAN_POINT('Ctrl Pts',(18.7125685143091,18.30747099738,80.572865027715));
#117570=CARTESIAN_POINT('Ctrl Pts',(11.5978097779391,22.5674100597,82.742358165064));
#117571=CARTESIAN_POINT('Ctrl Pts',(11.6227733666891,22.53672166376,82.73823514027));
#117572=CARTESIAN_POINT('Ctrl Pts',(11.9160671669291,22.17956444248,82.6896285494211));
#117573=CARTESIAN_POINT('Ctrl Pts',(12.4854557092891,21.55712977634,82.591528127515));
#117574=CARTESIAN_POINT('Ctrl Pts',(13.3211227504391,20.77626353478,82.4380379028789));
#117575=CARTESIAN_POINT('Ctrl Pts',(14.1224813937691,20.11780076625,82.283329059817));
#117576=CARTESIAN_POINT('Ctrl Pts',(14.8783020667991,19.56212479249,82.131672635088));
#117577=CARTESIAN_POINT('Ctrl Pts',(15.5811274847591,19.09431145646,81.9864168604));
#117578=CARTESIAN_POINT('Ctrl Pts',(16.2285628910291,18.7009157217,81.849546008323));
#117579=CARTESIAN_POINT('Ctrl Pts',(16.8211097747291,18.37024197503,81.722081374855));
#117580=CARTESIAN_POINT('Ctrl Pts',(17.3606117917191,18.09238223453,81.6044624197011));
#117581=CARTESIAN_POINT('Ctrl Pts',(17.8498880368591,17.8588580807,81.496683301038));
#117582=CARTESIAN_POINT('Ctrl Pts',(18.2156163347991,17.69650125828,81.415469693152));
#117583=CARTESIAN_POINT('Ctrl Pts',(18.4184926455491,17.61080394924,81.370213465902));
#117584=CARTESIAN_POINT('Ctrl Pts',(18.4737491950091,17.58778530033,81.357872779003));
#117585=CARTESIAN_POINT('Ctrl Pts',(10.7887911682091,22.10433914807,82.174666798942));
#117586=CARTESIAN_POINT('Ctrl Pts',(10.8141189968491,22.07077205096,82.172372871705));
#117587=CARTESIAN_POINT('Ctrl Pts',(11.1117900557491,21.6800749259,82.145250032619));
#117588=CARTESIAN_POINT('Ctrl Pts',(11.6918244678991,20.99843062262,82.088727484073));
#117589=CARTESIAN_POINT('Ctrl Pts',(12.5491405664491,20.14211901076,81.9952556772969));
#117590=CARTESIAN_POINT('Ctrl Pts',(13.3766873742891,19.41934260798,81.896597547713));
#117591=CARTESIAN_POINT('Ctrl Pts',(14.1618774648791,18.80893238109,81.7961233164201));
#117592=CARTESIAN_POINT('Ctrl Pts',(14.8959250259991,18.29470115512,81.696758155871));
#117593=CARTESIAN_POINT('Ctrl Pts',(15.5753262268891,17.86200505198,81.600569675382));
#117594=CARTESIAN_POINT('Ctrl Pts',(16.1997088336891,17.49808293197,81.5089307213659));
#117595=CARTESIAN_POINT('Ctrl Pts',(16.7702588729991,17.19211091299,81.422718126577));
#117596=CARTESIAN_POINT('Ctrl Pts',(17.2893313360391,16.93481823995,81.3423998907959));
#117597=CARTESIAN_POINT('Ctrl Pts',(17.6784046821991,16.75584136857,81.2810116085869));
#117598=CARTESIAN_POINT('Ctrl Pts',(17.8946094266191,16.66133724348,81.2464955986819));
#117599=CARTESIAN_POINT('Ctrl Pts',(17.9535239433391,16.63595046951,81.2370610578369));
#117600=CARTESIAN_POINT('Ctrl Pts',(12.5172852744664,21.43216844352,82.2238886792731));
#117601=CARTESIAN_POINT('Ctrl Pts',(12.7388749288692,21.15829039737,82.184816444556));
#117602=CARTESIAN_POINT('Ctrl Pts',(12.9611536694374,20.90216875751,82.1456227053559));
#117603=CARTESIAN_POINT('Ctrl Pts',(13.181766647766,20.66173879788,82.1067226849821));
#117604=CARTESIAN_POINT('Ctrl Pts',(13.2412317619777,20.5969321164344,82.0962373809357));
#117605=CARTESIAN_POINT('Ctrl Pts',(13.3005758510999,20.5332655058573,82.0857734168779));
#117606=CARTESIAN_POINT('Ctrl Pts',(13.3597592946233,20.4707111483689,82.0753377789735));
#117607=CARTESIAN_POINT('Ctrl Pts',(12.6211132020991,23.19498548026,81.546653375664));
#117608=CARTESIAN_POINT('Ctrl Pts',(12.8357939683531,22.9022256951466,81.4798426388965));
#117609=CARTESIAN_POINT('Ctrl Pts',(13.2793186839497,22.3474956363199,81.342352295626));
#117610=CARTESIAN_POINT('Ctrl Pts',(13.9768208390301,21.5902063508969,81.1283687718575));
#117611=CARTESIAN_POINT('Ctrl Pts',(14.6131840765691,20.9760939162043,80.9356018413964));
#117612=CARTESIAN_POINT('Ctrl Pts',(15.0160011538732,20.6207817077894,80.8150471263846));
#117613=CARTESIAN_POINT('Ctrl Pts',(15.182620190286,20.4790216117855,80.7654568892173));
#117614=CARTESIAN_POINT('Origin',(-6.70435958676991,20.,86.62860989379));
#117615=CARTESIAN_POINT('',(-6.1121826461617,20.00000000008,85.5087648635416));
#117616=CARTESIAN_POINT('',(-5.93853418691238,20.9999970776591,86.4935742132893));
#117617=CARTESIAN_POINT('Origin',(-5.93853418697242,20.,86.4935742132939));
#117618=CARTESIAN_POINT('',(-5.93853418690691,20.99999766213,86.49357421329));
#117619=CARTESIAN_POINT('',(-8.75366715310791,20.00000000008,85.97453149762));
#117620=CARTESIAN_POINT('Ctrl Pts',(0.957715876419088,23.49481230627,90.05041057889));
#117621=CARTESIAN_POINT('Ctrl Pts',(1.41501551649909,23.49481230627,89.9030012875299));
#117622=CARTESIAN_POINT('Ctrl Pts',(2.31555886405909,23.49481230627,89.60436039102));
#117623=CARTESIAN_POINT('Ctrl Pts',(3.60119053426909,23.49481230627,89.1258337619599));
#117624=CARTESIAN_POINT('Ctrl Pts',(4.77329563338909,23.49481230627,88.61996295293));
#117625=CARTESIAN_POINT('Ctrl Pts',(5.85230040977909,23.49481230627,88.07694753354));
#117626=CARTESIAN_POINT('Ctrl Pts',(6.88449642105908,23.49481230627,87.4679726818399));
#117627=CARTESIAN_POINT('Ctrl Pts',(7.88241911249909,23.49481230627,86.77324032414));
#117628=CARTESIAN_POINT('Ctrl Pts',(8.82724414092909,23.49481230627,85.99908763589));
#117629=CARTESIAN_POINT('Ctrl Pts',(9.71652793426909,23.49481230627,85.14645307785));
#117630=CARTESIAN_POINT('Ctrl Pts',(10.5558228444891,23.49481230627,84.20870787798));
#117631=CARTESIAN_POINT('Ctrl Pts',(11.3451188799491,23.49481230627,83.18434038658));
#117632=CARTESIAN_POINT('Ctrl Pts',(11.9952966407791,23.49481230627,82.206938842754));
#117633=CARTESIAN_POINT('Ctrl Pts',(12.3726190997991,23.49481230627,81.5679157537));
#117634=CARTESIAN_POINT('Ctrl Pts',(12.5199395434791,23.49481230627,81.306465323002));
#117635=CARTESIAN_POINT('Ctrl Pts',(1.31223816379909,22.19079499982,91.1502067021801));
#117636=CARTESIAN_POINT('Ctrl Pts',(1.77575274979909,22.19079499982,91.00079655301));
#117637=CARTESIAN_POINT('Ctrl Pts',(2.69548452203909,22.19079499982,90.69589495095));
#117638=CARTESIAN_POINT('Ctrl Pts',(4.02863623059909,22.19079499982,90.1999352359901));
#117639=CARTESIAN_POINT('Ctrl Pts',(5.26015181865909,22.19079499982,89.6686560663001));
#117640=CARTESIAN_POINT('Ctrl Pts',(6.4052033873591,22.19079499982,89.0925893293601));
#117641=CARTESIAN_POINT('Ctrl Pts',(7.50852137763909,22.19079499982,88.44181096938));
#117642=CARTESIAN_POINT('Ctrl Pts',(8.57970895306909,22.19079499982,87.6961548951001));
#117643=CARTESIAN_POINT('Ctrl Pts',(9.5949459237791,22.19079499982,86.86429832097));
#117644=CARTESIAN_POINT('Ctrl Pts',(10.5489790579091,22.19079499982,85.94949099884));
#117645=CARTESIAN_POINT('Ctrl Pts',(11.4462119670491,22.19079499982,84.94685287882));
#117646=CARTESIAN_POINT('Ctrl Pts',(12.2859883987391,22.19079499982,83.85676531586));
#117647=CARTESIAN_POINT('Ctrl Pts',(12.9740777733391,22.19079499982,82.822164502385));
#117648=CARTESIAN_POINT('Ctrl Pts',(13.3716617553591,22.19079499982,82.14877575625));
#117649=CARTESIAN_POINT('Ctrl Pts',(13.5266438736891,22.19079499982,81.8737270015279));
#117650=CARTESIAN_POINT('Ctrl Pts',(1.04499173760909,20.68183692524,90.3211570374501));
#117651=CARTESIAN_POINT('Ctrl Pts',(1.50382136543909,20.68183692524,90.1732551773701));
#117652=CARTESIAN_POINT('Ctrl Pts',(2.40908849580909,20.68183692524,89.87307302805));
#117653=CARTESIAN_POINT('Ctrl Pts',(3.70641859067909,20.68183692524,89.39025474333));
#117654=CARTESIAN_POINT('Ctrl Pts',(4.89314929098909,20.68183692524,88.8781289352801));
#117655=CARTESIAN_POINT('Ctrl Pts',(5.98841338556909,20.68183692524,88.3269769831401));
#117656=CARTESIAN_POINT('Ctrl Pts',(7.03811811826909,20.68183692524,87.7077109951301));
#117657=CARTESIAN_POINT('Ctrl Pts',(8.05407706883909,20.68183692524,87.00044229944));
#117658=CARTESIAN_POINT('Ctrl Pts',(9.01623602272909,20.68183692524,86.21208413945));
#117659=CARTESIAN_POINT('Ctrl Pts',(9.9214597292391,20.68183692524,85.3441439667299));
#117660=CARTESIAN_POINT('Ctrl Pts',(10.7750177448491,20.68183692524,84.39042350749));
#117661=CARTESIAN_POINT('Ctrl Pts',(11.5767409822491,20.68183692524,83.34987712961));
#117662=CARTESIAN_POINT('Ctrl Pts',(12.2362517775791,20.68183692524,82.358394339851));
#117663=CARTESIAN_POINT('Ctrl Pts',(12.6185621934391,20.68183692524,81.710911155554));
#117664=CARTESIAN_POINT('Ctrl Pts',(12.7677687787691,20.68183692524,81.446113106153));
#117665=CARTESIAN_POINT('Ctrl Pts',(0.521235740009087,21.03030703444,88.69636549059));
#117666=CARTESIAN_POINT('Ctrl Pts',(0.970883673709088,21.03030703444,88.55141961189));
#117667=CARTESIAN_POINT('Ctrl Pts',(1.84780264977909,21.03030703444,88.26048675999));
#117668=CARTESIAN_POINT('Ctrl Pts',(3.07492868137909,21.03030703444,87.80342336748));
#117669=CARTESIAN_POINT('Ctrl Pts',(4.17388887751909,21.03030703444,87.3288347799701));
#117670=CARTESIAN_POINT('Ctrl Pts',(5.17157827841909,21.03030703444,86.82651142453));
#117671=CARTESIAN_POINT('Ctrl Pts',(6.11621045464909,21.03030703444,86.2690041438399));
#117672=CARTESIAN_POINT('Ctrl Pts',(7.02393101296908,21.03030703444,85.63696795942));
#117673=CARTESIAN_POINT('Ctrl Pts',(7.8820663881191,21.03030703444,84.93385904153));
#117674=CARTESIAN_POINT('Ctrl Pts',(8.69163220008909,21.03030703444,84.15777023963));
#117675=CARTESIAN_POINT('Ctrl Pts',(9.45959510503909,21.03030703444,83.29991979292));
#117676=CARTESIAN_POINT('Ctrl Pts',(10.1867407736191,21.03030703444,82.356465425506));
#117677=CARTESIAN_POINT('Ctrl Pts',(10.7902425793991,21.03030703444,81.449486379538));
#117678=CARTESIAN_POINT('Ctrl Pts',(11.1426194915691,21.03030703444,80.852773540713));
#117679=CARTESIAN_POINT('Ctrl Pts',(11.2805070479191,21.03030703444,80.6080650710599));
#117680=CARTESIAN_POINT('',(0.756634314019088,21.00000000035,88.9355837865));
#117681=CARTESIAN_POINT('Ctrl Pts',(0.756634314019086,21.000000000506,88.9355837865));
#117682=CARTESIAN_POINT('Ctrl Pts',(0.93994744103186,21.000000000506,88.8761073500416));
#117683=CARTESIAN_POINT('Ctrl Pts',(1.11959860663145,21.0000000005717,88.8170344284642));
#117684=CARTESIAN_POINT('Ctrl Pts',(1.29567538370028,21.0000000005633,88.7581145497408));
#117685=CARTESIAN_POINT('Ctrl Pts',(1.48070951214041,21.0000000005545,88.6961973077917));
#117686=CARTESIAN_POINT('Ctrl Pts',(1.66179643777212,21.0000000004149,88.6344492947818));
#117687=CARTESIAN_POINT('Ctrl Pts',(1.8390552467172,21.0000000002067,88.5726343848086));
#117688=CARTESIAN_POINT('Ctrl Pts',(1.87867901386347,21.0000000001602,88.5588165124359));
#117689=CARTESIAN_POINT('Ctrl Pts',(1.91811155806819,21.0000000001135,88.5449954954783));
#117690=CARTESIAN_POINT('Ctrl Pts',(1.95735431199024,21.0000000000752,88.531169025967));
#117691=CARTESIAN_POINT('Ctrl Pts',(2.00286697124637,21.0000000000307,88.5151334695217));
#117692=CARTESIAN_POINT('Ctrl Pts',(2.04812434624247,20.9999999999972,88.4990905761022));
#117693=CARTESIAN_POINT('Ctrl Pts',(2.09312837856909,20.9999999999972,88.483037093));
#117694=CARTESIAN_POINT('Ctrl Pts',(2.24351527878013,20.9999999999972,88.4293922652698));
#117695=CARTESIAN_POINT('Ctrl Pts',(2.39108406144822,21.0000000003555,88.3756366703905));
#117696=CARTESIAN_POINT('Ctrl Pts',(2.5354704698584,21.0000000005385,88.3218406192587));
#117697=CARTESIAN_POINT('Ctrl Pts',(2.67828857452791,21.0000000007195,88.2686288928506));
#117698=CARTESIAN_POINT('Ctrl Pts',(2.81799304255477,21.000000000706,88.2153775179761));
#117699=CARTESIAN_POINT('Ctrl Pts',(2.95425406246973,21.0000000004912,88.1622002390388));
#117700=CARTESIAN_POINT('Ctrl Pts',(3.04816581560319,21.0000000003433,88.1255502015227));
#117701=CARTESIAN_POINT('Ctrl Pts',(3.14044239566545,21.0000000001096,88.0889363184504));
#117702=CARTESIAN_POINT('Ctrl Pts',(3.23098221778327,21.0000000000248,88.052408776881));
#117703=CARTESIAN_POINT('Ctrl Pts',(3.2494640903951,21.0000000000075,88.0449524184045));
#117704=CARTESIAN_POINT('Ctrl Pts',(3.26787361139831,20.9999999999972,88.0374996931925));
#117705=CARTESIAN_POINT('Ctrl Pts',(3.28620992071076,20.9999999999972,88.03005113008));
#117706=CARTESIAN_POINT('Ctrl Pts',(3.47134091295659,20.9999999999972,87.954847344175));
#117707=CARTESIAN_POINT('Ctrl Pts',(3.64897689064145,20.9999999997563,87.8799868520678));
#117708=CARTESIAN_POINT('Ctrl Pts',(3.82034472080339,21.000000000393,87.8052335230894));
#117709=CARTESIAN_POINT('Ctrl Pts',(3.97819715652474,21.0000000009796,87.7363758206468));
#117710=CARTESIAN_POINT('Ctrl Pts',(4.13073188522359,21.0000000007529,87.6676097819603));
#117711=CARTESIAN_POINT('Ctrl Pts',(4.27889814688429,21.0000000000916,87.5987088186199));
#117712=CARTESIAN_POINT('Ctrl Pts',(4.2915842068743,21.000000000035,87.5928094880671));
#117713=CARTESIAN_POINT('Ctrl Pts',(4.30423823260115,20.9999999999972,87.586909137677));
#117714=CARTESIAN_POINT('Ctrl Pts',(4.31686081404071,20.9999999999972,87.5810076073234));
#117715=CARTESIAN_POINT('Ctrl Pts',(4.31910810196864,20.9999999999972,87.579956915911));
#117716=CARTESIAN_POINT('Ctrl Pts',(4.32135438131283,20.9999999999984,87.5789061686031));
#117717=CARTESIAN_POINT('Ctrl Pts',(4.32359966125888,21.0000000000008,87.5778553613796));
#117718=CARTESIAN_POINT('Ctrl Pts',(4.42088083646353,21.000000000105,87.5323270691057));
#117719=CARTESIAN_POINT('Ctrl Pts',(4.51628790649546,21.0000000025738,87.4866900145638));
#117720=CARTESIAN_POINT('Ctrl Pts',(4.61055451505413,21.0000000047615,87.4406063796447));
#117721=CARTESIAN_POINT('Ctrl Pts',(4.70337776390992,21.0000000069156,87.3952283526033));
#117722=CARTESIAN_POINT('Ctrl Pts',(4.79509535721351,21.0000000085217,87.3494173844181));
#117723=CARTESIAN_POINT('Ctrl Pts',(4.88638328488241,21.0000000077554,87.3028072525664));
#117724=CARTESIAN_POINT('Ctrl Pts',(4.97507500508643,21.000000007011,87.2575227020411));
#117725=CARTESIAN_POINT('Ctrl Pts',(5.06336126825696,21.0000000036719,87.211483844095));
#117726=CARTESIAN_POINT('Ctrl Pts',(5.15183690010692,21.0000000013663,87.1643125760065));
#117727=CARTESIAN_POINT('Ctrl Pts',(5.18170994870006,21.0000000005878,87.1483855964039));
#117728=CARTESIAN_POINT('Ctrl Pts',(5.21160436110771,20.9999999999972,87.1323291520711));
#117729=CARTESIAN_POINT('Ctrl Pts',(5.24154231686215,20.9999999999972,87.1161275298069));
#117730=CARTESIAN_POINT('Ctrl Pts',(5.26025608299938,20.9999999999972,87.1060001392601));
#117731=CARTESIAN_POINT('Ctrl Pts',(5.27898824498872,21.0000000002298,87.0958185962174));
#117732=CARTESIAN_POINT('Ctrl Pts',(5.2977362483153,21.0000000005657,87.0855832092499));
#117733=CARTESIAN_POINT('Ctrl Pts',(5.41724408030014,21.0000000027072,87.0203384530646));
#117734=CARTESIAN_POINT('Ctrl Pts',(5.5373939734491,21.0000000060343,86.9529020405239));
#117735=CARTESIAN_POINT('Ctrl Pts',(5.65753673683337,21.0000000050463,86.8834118691035));
#117736=CARTESIAN_POINT('Ctrl Pts',(5.77345936830357,21.0000000040931,86.8163626078292));
#117737=CARTESIAN_POINT('Ctrl Pts',(5.8893751368828,21.0000000014303,86.7474012834568));
#117738=CARTESIAN_POINT('Ctrl Pts',(6.00472156171291,21.0000000005319,86.676695723562));
#117739=CARTESIAN_POINT('Ctrl Pts',(6.05642031158837,21.0000000001292,86.6450051959952));
#117740=CARTESIAN_POINT('Ctrl Pts',(6.10800499045389,20.9999999999972,86.6129648797915));
#117741=CARTESIAN_POINT('Ctrl Pts',(6.15942655135603,20.9999999999972,86.5805929331082));
#117742=CARTESIAN_POINT('Ctrl Pts',(6.19537674171716,20.9999999999972,86.5579608382202));
#117743=CARTESIAN_POINT('Ctrl Pts',(6.23124719525267,21.0000000000476,86.5351662312197));
#117744=CARTESIAN_POINT('Ctrl Pts',(6.2670292769119,21.0000000000872,86.512212433455));
#117745=CARTESIAN_POINT('Ctrl Pts',(6.40028191327865,21.0000000002348,86.4267323852033));
#117746=CARTESIAN_POINT('Ctrl Pts',(6.53230650202812,21.0000000000892,86.3390413814324));
#117747=CARTESIAN_POINT('Ctrl Pts',(6.66269166437902,21.0000000000251,86.2493922214948));
#117748=CARTESIAN_POINT('Ctrl Pts',(6.79307682672993,20.9999999999609,86.1597430615573));
#117749=CARTESIAN_POINT('Ctrl Pts',(6.92182230893109,20.9999999999972,86.0681357906987));
#117750=CARTESIAN_POINT('Ctrl Pts',(7.0485510816308,20.9999999999972,85.9748650028717));
#117751=CARTESIAN_POINT('Ctrl Pts',(7.09916077095027,20.9999999999972,85.9376169060587));
#117752=CARTESIAN_POINT('Ctrl Pts',(7.14944610400102,21.0000000000191,85.9001003667346));
#117753=CARTESIAN_POINT('Ctrl Pts',(7.1994227681535,21.0000000000378,85.8623048375778));
#117754=CARTESIAN_POINT('Ctrl Pts',(7.32807752282551,21.0000000000858,85.7650079368374));
#117755=CARTESIAN_POINT('Ctrl Pts',(7.45468888847659,21.0000000000897,85.6658652185241));
#117756=CARTESIAN_POINT('Ctrl Pts',(7.57952991246622,21.0000000000568,85.5647153018767));
#117757=CARTESIAN_POINT('Ctrl Pts',(7.68167013643052,21.0000000000299,85.4819582496661));
#117758=CARTESIAN_POINT('Ctrl Pts',(7.78262481832806,20.9999999999972,85.3978567469911));
#117759=CARTESIAN_POINT('Ctrl Pts',(7.88252783227743,20.9999999999972,85.3123017409167));
#117760=CARTESIAN_POINT('Ctrl Pts',(7.94500648545622,20.9999999999972,85.2587962325149));
#117761=CARTESIAN_POINT('Ctrl Pts',(8.00707501935217,21.0000000000007,85.2047245834137));
#117762=CARTESIAN_POINT('Ctrl Pts',(8.06876006198254,20.9999999999989,85.1500566565699));
#117763=CARTESIAN_POINT('Ctrl Pts',(8.19199549949309,20.9999999999952,85.0408401334858));
#117764=CARTESIAN_POINT('Ctrl Pts',(8.31370272600517,21.0000000000204,84.9292458792537));
#117765=CARTESIAN_POINT('Ctrl Pts',(8.4340961907889,21.0000000000293,84.8150402865715));
#117766=CARTESIAN_POINT('Ctrl Pts',(8.51332555497591,21.0000000000352,84.7398830800648));
#117767=CARTESIAN_POINT('Ctrl Pts',(8.59198518630918,20.9999999999972,84.6635942037091));
#117768=CARTESIAN_POINT('Ctrl Pts',(8.67012689091576,20.9999999999972,84.5860990407983));
#117769=CARTESIAN_POINT('Ctrl Pts',(8.74384121285911,20.9999999999972,84.5129946285434));
#117770=CARTESIAN_POINT('Ctrl Pts',(8.8171026280427,21.0000000000352,84.4388238577954));
#117771=CARTESIAN_POINT('Ctrl Pts',(8.88988045449224,21.0000000000318,84.3635930688318));
#117772=CARTESIAN_POINT('Ctrl Pts',(9.0701638994232,21.0000000000234,84.1772332053831));
#117773=CARTESIAN_POINT('Ctrl Pts',(9.24747949353293,21.0000000000373,83.9843643404513));
#117774=CARTESIAN_POINT('Ctrl Pts',(9.42147268297582,21.0000000000345,83.7851882666207));
#117775=CARTESIAN_POINT('',(1.21030572547832,22.7988981836224,90.3337691724699));
#117776=CARTESIAN_POINT('Origin',(0.756612526612343,22.5000005075418,88.9355510391788));
#117777=CARTESIAN_POINT('Ctrl Pts',(12.6211182849899,23.194988543039,81.5466562879185));
#117778=CARTESIAN_POINT('Ctrl Pts',(12.4932187937712,23.2005913915118,81.7639926710847));
#117779=CARTESIAN_POINT('Ctrl Pts',(12.3627405816846,23.2058937154176,81.9773859230737));
#117780=CARTESIAN_POINT('Ctrl Pts',(12.2297445484923,23.2108375253335,82.1867818886298));
#117781=CARTESIAN_POINT('Ctrl Pts',(12.0799119016713,23.2164071961522,82.4226863062268));
#117782=CARTESIAN_POINT('Ctrl Pts',(11.9268841365456,23.2215219023617,82.6535157173191));
#117783=CARTESIAN_POINT('Ctrl Pts',(11.770784498812,23.2261014255578,82.8791446435673));
#117784=CARTESIAN_POINT('Ctrl Pts',(11.6733482848867,23.2289599293204,83.0199805138157));
#117785=CARTESIAN_POINT('Ctrl Pts',(11.5747152411408,23.2316099698021,83.1587912947737));
#117786=CARTESIAN_POINT('Ctrl Pts',(11.4749149002699,23.2340322162995,83.2955566725622));
#117787=CARTESIAN_POINT('Ctrl Pts',(11.3162265942549,23.2378837281286,83.5130215222145));
#117788=CARTESIAN_POINT('Ctrl Pts',(11.1545882040806,23.2411594814845,83.725312223375));
#117789=CARTESIAN_POINT('Ctrl Pts',(10.9901795614978,23.2437806622171,83.9323201856936));
#117790=CARTESIAN_POINT('Ctrl Pts',(10.8850257656668,23.2454571379745,84.0647199954788));
#117791=CARTESIAN_POINT('Ctrl Pts',(10.7787384305381,23.246865819069,84.1949598703842));
#117792=CARTESIAN_POINT('Ctrl Pts',(10.6713609019886,23.2479852956996,84.3230218260961));
#117793=CARTESIAN_POINT('Ctrl Pts',(10.5941883156074,23.248789867272,84.4150603789743));
#117794=CARTESIAN_POINT('Ctrl Pts',(10.5164525980134,23.2494450421076,84.5059741148954));
#117795=CARTESIAN_POINT('Ctrl Pts',(10.4381795739186,23.24994255375,84.5957555369526));
#117796=CARTESIAN_POINT('Ctrl Pts',(10.2676153414658,23.2510266781007,84.7913976437804));
#117797=CARTESIAN_POINT('Ctrl Pts',(10.0944510855359,23.2513968052464,84.9816931937978));
#117798=CARTESIAN_POINT('Ctrl Pts',(9.918759213001,23.2510526136532,85.1666740707244));
#117799=CARTESIAN_POINT('Ctrl Pts',(9.88699239518467,23.2509903804293,85.2001204318568));
#117800=CARTESIAN_POINT('Ctrl Pts',(9.85514281024508,23.2509047730507,85.2333930675873));
#117801=CARTESIAN_POINT('Ctrl Pts',(9.82321071099612,23.2507957610793,85.2664921901425));
#117802=CARTESIAN_POINT('Ctrl Pts',(9.65324116957873,23.2502155075031,85.4426736130474));
#117803=CARTESIAN_POINT('Ctrl Pts',(9.48093802884081,23.2489727089887,85.613939274566));
#117804=CARTESIAN_POINT('Ctrl Pts',(9.30643613027418,23.2470585771029,85.7803407810742));
#117805=CARTESIAN_POINT('Ctrl Pts',(9.27598738730181,23.2467245812536,85.8093760909677));
#117806=CARTESIAN_POINT('Ctrl Pts',(9.24547157334416,23.2463701281518,85.8382632907172));
#117807=CARTESIAN_POINT('Ctrl Pts',(9.2148892476124,23.2459951489363,85.8670026333113));
#117808=CARTESIAN_POINT('Ctrl Pts',(9.12168396549575,23.2448523305685,85.9545910841644));
#117809=CARTESIAN_POINT('Ctrl Pts',(9.02785809547641,23.2435191969874,86.0408090358809));
#117810=CARTESIAN_POINT('Ctrl Pts',(8.93341171656685,23.2419982707098,86.1256702646693));
#117811=CARTESIAN_POINT('Ctrl Pts',(8.81461189297349,23.2400851664112,86.2324133619313));
#117812=CARTESIAN_POINT('Ctrl Pts',(8.6948307292937,23.2378749655979,86.337010199082));
#117813=CARTESIAN_POINT('Ctrl Pts',(8.57409648579421,23.2353716487655,86.4395061305676));
#117814=CARTESIAN_POINT('Ctrl Pts',(8.46573723845031,23.2331249164388,86.5314964530284));
#117815=CARTESIAN_POINT('Ctrl Pts',(8.35660744053645,23.2306439797656,86.6217952727136));
#117816=CARTESIAN_POINT('Ctrl Pts',(8.24671423456762,23.2279295907953,86.7104347179882));
#117817=CARTESIAN_POINT('Ctrl Pts',(8.19176763158321,23.2265723963101,86.7547544406254));
#117818=CARTESIAN_POINT('Ctrl Pts',(8.13663010537614,23.2251567756296,86.7986592337719));
#117819=CARTESIAN_POINT('Ctrl Pts',(8.08130107438259,23.2236822322506,86.8421534874745));
#117820=CARTESIAN_POINT('Ctrl Pts',(8.05363655888582,23.2229449605611,86.8639006143258));
#117821=CARTESIAN_POINT('Ctrl Pts',(8.02592416291969,23.2221929539408,86.8855450991431));
#117822=CARTESIAN_POINT('Ctrl Pts',(7.99816380423124,23.2214261205358,86.9070874391833));
#117823=CARTESIAN_POINT('Ctrl Pts',(7.99636893047286,23.221376540155,86.9084802807264));
#117824=CARTESIAN_POINT('Ctrl Pts',(7.9945738562225,23.2213268977379,86.9098726952744));
#117825=CARTESIAN_POINT('Ctrl Pts',(7.99277858143012,23.2212771933182,86.911264682935));
#117826=CARTESIAN_POINT('Ctrl Pts',(7.9806905755884,23.2209425218144,86.920637262021));
#117827=CARTESIAN_POINT('Ctrl Pts',(7.96859347796431,23.2206050393413,86.9299904876475));
#117828=CARTESIAN_POINT('Ctrl Pts',(7.95648730188297,23.2202647561823,86.9393244303098));
#117829=CARTESIAN_POINT('Ctrl Pts',(7.94953522715104,23.2200693456797,86.9446845263877));
#117830=CARTESIAN_POINT('Ctrl Pts',(7.9425801585374,23.2198730116799,86.9500382634073));
#117831=CARTESIAN_POINT('Ctrl Pts',(7.93562209831243,23.2196757561466,86.9553856546025));
#117832=CARTESIAN_POINT('Ctrl Pts',(7.92866403808747,23.2194785006134,86.9607330457977));
#117833=CARTESIAN_POINT('Ctrl Pts',(7.92337482480999,23.2193281201649,86.9647934011114));
#117834=CARTESIAN_POINT('Ctrl Pts',(7.91473894495999,23.2190812268188,86.9714088038817));
#117835=CARTESIAN_POINT('Ctrl Pts',(7.75412374001771,23.2144893582334,87.0944459801958));
#117836=CARTESIAN_POINT('Ctrl Pts',(7.59313440095865,23.2092503649804,87.213320286633));
#117837=CARTESIAN_POINT('Ctrl Pts',(7.43187198895906,23.2034201191061,87.3282788054784));
#117838=CARTESIAN_POINT('Ctrl Pts',(7.28392337804805,23.1980712174763,87.4337463658644));
#117839=CARTESIAN_POINT('Ctrl Pts',(7.13574410135277,23.1922245520801,87.5359175245917));
#117840=CARTESIAN_POINT('Ctrl Pts',(6.98738482421358,23.1859233657266,87.6349560317578));
#117841=CARTESIAN_POINT('Ctrl Pts',(6.82499126114028,23.1790261084519,87.7433632467989));
#117842=CARTESIAN_POINT('Ctrl Pts',(6.66238224676357,23.1715841250771,87.8480182462217));
#117843=CARTESIAN_POINT('Ctrl Pts',(6.49962387552277,23.1636562178235,87.9492019279517));
#117844=CARTESIAN_POINT('Ctrl Pts',(6.33000192396702,23.1553939878082,88.0546525627166));
#117845=CARTESIAN_POINT('Ctrl Pts',(6.1602174231917,23.1466038280092,88.1563328656577));
#117846=CARTESIAN_POINT('Ctrl Pts',(5.99031550141526,23.1373568935397,88.2545137117141));
#117847=CARTESIAN_POINT('Ctrl Pts',(5.97629193379932,23.1365936590253,88.2626174795754));
#117848=CARTESIAN_POINT('Ctrl Pts',(5.96226755183385,23.1358273159182,88.27069738153));
#117849=CARTESIAN_POINT('Ctrl Pts',(5.94824237341941,23.1350579060704,88.2787535565813));
#117850=CARTESIAN_POINT('Ctrl Pts',(5.77104788922942,23.1253371612015,88.3805354905128));
#117851=CARTESIAN_POINT('Ctrl Pts',(5.59372812088921,23.1151261986145,88.4785346318076));
#117852=CARTESIAN_POINT('Ctrl Pts',(5.41629450000383,23.1045139189269,88.5731175903428));
#117853=CARTESIAN_POINT('Ctrl Pts',(5.24819748102698,23.0944600600745,88.6627235697307));
#117854=CARTESIAN_POINT('Ctrl Pts',(5.07999774069339,23.084046009247,88.7492625038068));
#117855=CARTESIAN_POINT('Ctrl Pts',(4.9116901409163,23.073355125837,88.8330064906868));
#117856=CARTESIAN_POINT('Ctrl Pts',(4.7973680441979,23.0660933966648,88.8898891756063));
#117857=CARTESIAN_POINT('Ctrl Pts',(4.68299588668316,23.0587041056104,88.9454816003795));
#117858=CARTESIAN_POINT('Ctrl Pts',(4.56855907778642,23.0512155486768,88.9998818145646));
#117859=CARTESIAN_POINT('Ctrl Pts',(4.33172366852101,23.0357174282444,89.1124670667651));
#117860=CARTESIAN_POINT('Ctrl Pts',(4.0945289701563,23.0197040987167,89.2200241428719));
#117861=CARTESIAN_POINT('Ctrl Pts',(3.85733585746382,23.0031940856782,89.3232234871173));
#117862=CARTESIAN_POINT('Ctrl Pts',(3.82513871686922,23.0009529784007,89.337232004305));
#117863=CARTESIAN_POINT('Ctrl Pts',(3.79294157723204,22.9987027283982,89.3511601537571));
#117864=CARTESIAN_POINT('Ctrl Pts',(3.76074531545843,22.9964433907818,89.3650095465169));
#117865=CARTESIAN_POINT('Ctrl Pts',(3.50417118157362,22.9784385802809,89.4753762709885));
#117866=CARTESIAN_POINT('Ctrl Pts',(3.24765436648079,22.9598558973906,89.5807460605779));
#117867=CARTESIAN_POINT('Ctrl Pts',(2.99145622685065,22.9407283360055,89.6820323373258));
#117868=CARTESIAN_POINT('Ctrl Pts',(2.80669244682127,22.926934010452,89.7550775022285));
#117869=CARTESIAN_POINT('Ctrl Pts',(2.62209396769549,22.9128564807424,89.8259975035371));
#117870=CARTESIAN_POINT('Ctrl Pts',(2.4377532614348,22.898511215253,89.8951196997858));
#117871=CARTESIAN_POINT('Ctrl Pts',(2.13718806689121,22.8751214409591,90.0078225682093));
#117872=CARTESIAN_POINT('Ctrl Pts',(1.83730931686889,22.851018863972,90.1157480463776));
#117873=CARTESIAN_POINT('Ctrl Pts',(1.53825824495239,22.8262860812645,90.220267935109));
#117874=CARTESIAN_POINT('Ctrl Pts',(1.4288217069242,22.8172352188216,90.2585165683761));
#117875=CARTESIAN_POINT('Ctrl Pts',(1.3194957728693,22.8081001505928,90.2963086713995));
#117876=CARTESIAN_POINT('Ctrl Pts',(1.2102865960548,22.7988855800353,90.3337102128107));
#117877=CARTESIAN_POINT('Ctrl Pts',(-1.18612654204091,23.08684060709,90.8056390119699));
#117878=CARTESIAN_POINT('Ctrl Pts',(-1.02638895989091,23.08684060709,90.77605244985));
#117879=CARTESIAN_POINT('Ctrl Pts',(-0.683862091540912,23.08684060709,90.71121995565));
#117880=CARTESIAN_POINT('Ctrl Pts',(-0.161822890870914,23.08684060709,90.60439269897));
#117881=CARTESIAN_POINT('Ctrl Pts',(0.363860643519087,23.08684060709,90.48319011439));
#117882=CARTESIAN_POINT('Ctrl Pts',(0.845214580869085,23.08684060709,90.3551094761801));
#117883=CARTESIAN_POINT('Ctrl Pts',(1.17290328465909,23.08684060709,90.25335018102));
#117884=CARTESIAN_POINT('Ctrl Pts',(1.33589618381909,23.08684060709,90.19751377573));
#117885=CARTESIAN_POINT('Ctrl Pts',(1.35880646243909,23.08684060709,90.1895581012301));
#117886=CARTESIAN_POINT('Ctrl Pts',(-1.08807919910092,21.82055786604,91.33494523279));
#117887=CARTESIAN_POINT('Ctrl Pts',(-0.926943055190917,21.82055786604,91.30509987628));
#117888=CARTESIAN_POINT('Ctrl Pts',(-0.580391297820914,21.82055786604,91.23951081764));
#117889=CARTESIAN_POINT('Ctrl Pts',(-0.0482616351409153,21.82055786604,
91.13064340811));
#117890=CARTESIAN_POINT('Ctrl Pts',(0.492565115739089,21.82055786604,91.00598854667));
#117891=CARTESIAN_POINT('Ctrl Pts',(0.993006855569089,21.82055786604,90.87289106935));
#117892=CARTESIAN_POINT('Ctrl Pts',(1.33813198802909,21.82055786604,90.76576936584));
#117893=CARTESIAN_POINT('Ctrl Pts',(1.51105882888909,21.82055786604,90.7065309896001));
#117894=CARTESIAN_POINT('Ctrl Pts',(1.53539056153909,21.82055786604,90.69808194737));
#117895=CARTESIAN_POINT('Ctrl Pts',(-1.24665752627091,20.75508697312,90.47886395057));
#117896=CARTESIAN_POINT('Ctrl Pts',(-1.08778336701091,20.75508697312,90.4494371590201));
#117897=CARTESIAN_POINT('Ctrl Pts',(-0.747741323710916,20.75508697312,90.3850717411299));
#117898=CARTESIAN_POINT('Ctrl Pts',(-0.231931619720914,20.75508697312,90.27950400312));
#117899=CARTESIAN_POINT('Ctrl Pts',(0.284403024929085,20.75508697312,90.16043273296));
#117900=CARTESIAN_POINT('Ctrl Pts',(0.753972823749085,20.75508697312,90.03544931493));
#117901=CARTESIAN_POINT('Ctrl Pts',(1.07089688918909,20.75508697312,89.93700058226));
#117902=CARTESIAN_POINT('Ctrl Pts',(1.22775692180909,20.75508697312,89.8832644342999));
#117903=CARTESIAN_POINT('Ctrl Pts',(1.24978964464909,20.75508697312,89.87561334769));
#117904=CARTESIAN_POINT('Ctrl Pts',(-1.49220764661091,21.03031426069,89.1532675363799));
#117905=CARTESIAN_POINT('Ctrl Pts',(-1.33683605048091,21.03031426069,89.1244888704399));
#117906=CARTESIAN_POINT('Ctrl Pts',(-1.00687395381091,21.03031426069,89.06201819526));
#117907=CARTESIAN_POINT('Ctrl Pts',(-0.516334839390912,21.03031426069,88.96155982342));
#117908=CARTESIAN_POINT('Ctrl Pts',(-0.0379249208809143,21.03031426069,
88.85113444793));
#117909=CARTESIAN_POINT('Ctrl Pts',(0.383841316339086,21.03031426069,88.7387152199099));
#117910=CARTESIAN_POINT('Ctrl Pts',(0.657097526779088,21.03031426069,88.65369612211));
#117911=CARTESIAN_POINT('Ctrl Pts',(0.789078959859088,21.03031426069,88.6084798825201));
#117912=CARTESIAN_POINT('Ctrl Pts',(0.807551788049085,21.03031426069,88.60206438782));
#117913=CARTESIAN_POINT('',(-1.28513099060542,21.0000000000039,89.419838384476));
#117914=CARTESIAN_POINT('Ctrl Pts',(-1.28513097334713,21.,89.4198384761759));
#117915=CARTESIAN_POINT('Ctrl Pts',(-1.13188223424533,21.,89.3909954656273));
#117916=CARTESIAN_POINT('Ctrl Pts',(-0.828434316537085,21.,89.3323920366554));
#117917=CARTESIAN_POINT('Ctrl Pts',(-0.374817752490913,20.99999999999,89.23726971619));
#117918=CARTESIAN_POINT('Ctrl Pts',(0.0523864881590876,21.00000000004,89.1373009151));
#117919=CARTESIAN_POINT('Ctrl Pts',(0.441186856229087,20.99999999984,89.03383812529));
#117920=CARTESIAN_POINT('Ctrl Pts',(0.657536503429089,21.00000000035,88.96773970165));
#117921=CARTESIAN_POINT('Ctrl Pts',(0.756634314019088,21.00000000035,88.9355837865));
#117922=CARTESIAN_POINT('',(-1.00773525083376,22.4999925247862,90.8939704740664));
#117923=CARTESIAN_POINT('Origin',(-1.28513134966091,22.5,89.41983613899));
#117924=CARTESIAN_POINT('Ctrl Pts',(-1.00769979882528,22.4999592529598,
90.8939685470445));
#117925=CARTESIAN_POINT('Ctrl Pts',(-0.957084251150433,22.5061488705642,
90.8844393268669));
#117926=CARTESIAN_POINT('Ctrl Pts',(-0.906738505136563,22.5123434672732,
90.8748395747033));
#117927=CARTESIAN_POINT('Ctrl Pts',(-0.856658827927557,22.5185434703929,
90.8651548009734));
#117928=CARTESIAN_POINT('Ctrl Pts',(-0.731233690259289,22.5340714507668,
90.840899171823));
#117929=CARTESIAN_POINT('Ctrl Pts',(-0.607474509670458,22.5496351877152,
90.816110119547));
#117930=CARTESIAN_POINT('Ctrl Pts',(-0.485314354543676,22.565250802786,
90.7905920608092));
#117931=CARTESIAN_POINT('Ctrl Pts',(-0.366271594539289,22.5804679242382,
90.7657251953494));
#117932=CARTESIAN_POINT('Ctrl Pts',(-0.248747016584948,22.5957338562364,
90.7401660636045));
#117933=CARTESIAN_POINT('Ctrl Pts',(-0.132722430427957,22.6110410435462,
90.7137342806339));
#117934=CARTESIAN_POINT('Ctrl Pts',(-0.0187383588171168,22.6260790246524,
90.6877673511863));
#117935=CARTESIAN_POINT('Ctrl Pts',(0.0937983147043079,22.6411564272297,
90.6609582147743));
#117936=CARTESIAN_POINT('Ctrl Pts',(0.204857809483684,22.6562502661615,
90.6331362234104));
#117937=CARTESIAN_POINT('Ctrl Pts',(0.312787937670032,22.6709188001213,
90.6060981831215));
#117938=CARTESIAN_POINT('Ctrl Pts',(0.419323130664292,22.6856024750495,
90.5781035934115));
#117939=CARTESIAN_POINT('Ctrl Pts',(0.52438798738615,22.7002708090524,90.5489958293737));
#117940=CARTESIAN_POINT('Ctrl Pts',(0.577140084527384,22.7076356444918,
90.5343810890694));
#117941=CARTESIAN_POINT('Ctrl Pts',(0.629520735811119,22.7149964976842,
90.5194857203461));
#117942=CARTESIAN_POINT('Ctrl Pts',(0.6815154128319,22.7223490422761,90.504289854534));
#117943=CARTESIAN_POINT('Ctrl Pts',(0.79287133060566,22.7380958340233,90.471745184948));
#117944=CARTESIAN_POINT('Ctrl Pts',(0.902459500416484,22.7538032895651,
90.437822278412));
#117945=CARTESIAN_POINT('Ctrl Pts',(1.01020021045901,22.7694829094358,90.4023270529812));
#117946=CARTESIAN_POINT('Ctrl Pts',(1.07763762528111,22.7792971479819,90.3801097663061));
#117947=CARTESIAN_POINT('Ctrl Pts',(1.14435030260074,22.7891007041396,90.3572764595547));
#117948=CARTESIAN_POINT('Ctrl Pts',(1.21030897714296,22.7989003259575,90.3337791942256));
#117949=CARTESIAN_POINT('Ctrl Pts',(8.45816176827909,16.26511926842,98.7964653589499));
#117950=CARTESIAN_POINT('Ctrl Pts',(8.71225114275908,16.41477280571,98.6494070076199));
#117951=CARTESIAN_POINT('Ctrl Pts',(9.27881268981909,16.73006084598,98.30341626023));
#117952=CARTESIAN_POINT('Ctrl Pts',(10.1626398113191,17.16069654247,97.6962496853799));
#117953=CARTESIAN_POINT('Ctrl Pts',(11.1008309226691,17.54981639277,96.96627400869));
#117954=CARTESIAN_POINT('Ctrl Pts',(12.0284701745891,17.86984908755,96.1523318668001));
#117955=CARTESIAN_POINT('Ctrl Pts',(12.9325147810891,18.12067756051,95.26102236673));
#117956=CARTESIAN_POINT('Ctrl Pts',(13.8034582743191,18.30536666785,94.2997004316301));
#117957=CARTESIAN_POINT('Ctrl Pts',(14.6483615697391,18.43072561429,93.2588424428));
#117958=CARTESIAN_POINT('Ctrl Pts',(15.4901719996691,18.50141397362,92.10037160054));
#117959=CARTESIAN_POINT('Ctrl Pts',(16.3530907398691,18.51438369082,90.76409474325));
#117960=CARTESIAN_POINT('Ctrl Pts',(17.2403956363891,18.45914837749,89.19684938304));
#117961=CARTESIAN_POINT('Ctrl Pts',(18.1343401599191,18.32423291388,87.36260202144));
#117962=CARTESIAN_POINT('Ctrl Pts',(19.0033848293491,18.10320054974,85.24319884147));
#117963=CARTESIAN_POINT('Ctrl Pts',(19.7639909942691,17.81526535809,82.9702592037509));
#117964=CARTESIAN_POINT('Ctrl Pts',(20.1883444225591,17.59455708305,81.382235884647));
#117965=CARTESIAN_POINT('Ctrl Pts',(20.3703684052891,17.48632437673,80.615759308313));
#117966=CARTESIAN_POINT('Ctrl Pts',(6.31418014116909,15.43220418763,92.79563719768));
#117967=CARTESIAN_POINT('Ctrl Pts',(6.49200941171909,15.56346847277,92.67838236751));
#117968=CARTESIAN_POINT('Ctrl Pts',(6.88387432291909,15.84414338516,92.4035075448201));
#117969=CARTESIAN_POINT('Ctrl Pts',(7.48196966441909,16.24577547329,91.9242120499101));
#117970=CARTESIAN_POINT('Ctrl Pts',(8.10612356461909,16.6365848729,91.3501649846601));
#117971=CARTESIAN_POINT('Ctrl Pts',(8.71750994518909,16.99297183984,90.71045662041));
#117972=CARTESIAN_POINT('Ctrl Pts',(9.3124519476191,17.31472032014,90.0082381109));
#117973=CARTESIAN_POINT('Ctrl Pts',(9.88895414563909,17.60257331209,89.2471181028301));
#117974=CARTESIAN_POINT('Ctrl Pts',(10.4549508437891,17.8618188302,88.41744323317));
#117975=CARTESIAN_POINT('Ctrl Pts',(11.0287137839791,18.10025681166,87.4864837035));
#117976=CARTESIAN_POINT('Ctrl Pts',(11.6304101411391,18.32271215478,86.40251363781));
#117977=CARTESIAN_POINT('Ctrl Pts',(12.2670974264291,18.52555248364,85.11784149556));
#117978=CARTESIAN_POINT('Ctrl Pts',(12.9309003101591,18.69913435731,83.5979370835401));
#117979=CARTESIAN_POINT('Ctrl Pts',(13.6016889453491,18.83244677012,81.8239640921051));
#117980=CARTESIAN_POINT('Ctrl Pts',(14.2139669773891,18.91249476228,79.9062655709491));
#117981=CARTESIAN_POINT('Ctrl Pts',(14.5696327416291,18.93553052461,78.560927762134));
#117982=CARTESIAN_POINT('Ctrl Pts',(14.7249351849991,18.94108956235,77.911474252923));
#117983=CARTESIAN_POINT('Ctrl Pts',(2.54935064044909,19.22183178223,89.2228044174901));
#117984=CARTESIAN_POINT('Ctrl Pts',(2.74816966526909,19.38069675838,89.11271227861));
#117985=CARTESIAN_POINT('Ctrl Pts',(3.18450270870909,19.72231812323,88.8567707992701));
#117986=CARTESIAN_POINT('Ctrl Pts',(3.84607183220909,20.21957457743,88.41774917846));
#117987=CARTESIAN_POINT('Ctrl Pts',(4.53420387286909,20.71569136082,87.89920721743));
#117988=CARTESIAN_POINT('Ctrl Pts',(5.20913049307909,21.18237918094,87.3269794904301));
#117989=CARTESIAN_POINT('Ctrl Pts',(5.86983667115909,21.61932357701,86.70255461879));
#117990=CARTESIAN_POINT('Ctrl Pts',(6.5166169471191,22.02651478544,86.02752892074));
#117991=CARTESIAN_POINT('Ctrl Pts',(7.16026643121909,22.41003287152,85.29176070735));
#117992=CARTESIAN_POINT('Ctrl Pts',(7.82357909374909,22.78105285215,84.46472655768));
#117993=CARTESIAN_POINT('Ctrl Pts',(8.5330095959891,23.14891805727,83.49874325701));
#117994=CARTESIAN_POINT('Ctrl Pts',(9.30144695145909,23.51183300341,82.349167312438));
#117995=CARTESIAN_POINT('Ctrl Pts',(10.1247389211891,23.8583235636,80.982966536629));
#117996=CARTESIAN_POINT('Ctrl Pts',(10.9831261496691,24.1725563834,79.382122199941));
#117997=CARTESIAN_POINT('Ctrl Pts',(11.7956651902091,24.42485648488,77.6476829007421));
#117998=CARTESIAN_POINT('Ctrl Pts',(12.2871279910191,24.55396132786,76.431541471836));
#117999=CARTESIAN_POINT('Ctrl Pts',(12.5064116716291,24.60764795684,75.845400513527));
#118000=CARTESIAN_POINT('Ctrl Pts',(-0.111615554140913,24.89134380645,90.66372486418));
#118001=CARTESIAN_POINT('Ctrl Pts',(0.19025221778909,25.10382403371,90.53297074905));
#118002=CARTESIAN_POINT('Ctrl Pts',(0.85803534504909,25.557842799,90.23007744772));
#118003=CARTESIAN_POINT('Ctrl Pts',(1.88634608190909,26.20614559666,89.71458517922));
#118004=CARTESIAN_POINT('Ctrl Pts',(2.97016886586909,26.83497373368,89.11095423698));
#118005=CARTESIAN_POINT('Ctrl Pts',(4.04244300886909,27.40608121153,88.4506164042799));
#118006=CARTESIAN_POINT('Ctrl Pts',(5.09618479047909,27.91912696323,87.73638641167));
#118007=CARTESIAN_POINT('Ctrl Pts',(6.1271003298391,28.37546235392,86.9710385745999));
#118008=CARTESIAN_POINT('Ctrl Pts',(7.14876251537909,28.78369951161,86.14393771161));
#118009=CARTESIAN_POINT('Ctrl Pts',(8.19441250288909,29.15618061071,85.2220293390399));
#118010=CARTESIAN_POINT('Ctrl Pts',(9.30256349945909,29.50014277728,84.1543224935201));
#118011=CARTESIAN_POINT('Ctrl Pts',(10.4897674388291,29.80928089036,82.894592873641));
#118012=CARTESIAN_POINT('Ctrl Pts',(11.7467525600991,30.0679526902,81.410216850361));
#118013=CARTESIAN_POINT('Ctrl Pts',(13.0428227217091,30.25874444737,79.684901641459));
#118014=CARTESIAN_POINT('Ctrl Pts',(14.2592774845091,30.36290197067,77.829109904896));
#118015=CARTESIAN_POINT('Ctrl Pts',(14.9927419533391,30.38363581186,76.53517273404));
#118016=CARTESIAN_POINT('Ctrl Pts',(15.3204046577991,30.3849546111,75.912812767194));
#118017=CARTESIAN_POINT('',(0.214734006960575,24.6920295183809,90.5121348736941));
#118018=CARTESIAN_POINT('Origin',(4.08666499754585,24.6942623759682,99.1828508702515));
#118019=CARTESIAN_POINT('Ctrl Pts',(0.214734710864216,24.6920295184668,
90.5121364516904));
#118020=CARTESIAN_POINT('Ctrl Pts',(0.448085072341334,24.8703386629935,
90.408088292175));
#118021=CARTESIAN_POINT('Ctrl Pts',(0.682365291824861,25.0409638010153,
90.2997216953764));
#118022=CARTESIAN_POINT('Ctrl Pts',(0.916972181677289,25.2039041524456,
90.1870952943443));
#118023=CARTESIAN_POINT('Ctrl Pts',(1.18245519028357,25.3882887404188,90.0596463698336));
#118024=CARTESIAN_POINT('Ctrl Pts',(1.44835601157772,25.5628320122888,89.9267421084685));
#118025=CARTESIAN_POINT('Ctrl Pts',(1.7139478183002,25.7276223328341,89.788483032972));
#118026=CARTESIAN_POINT('Ctrl Pts',(1.80455090592196,25.7838383435456,89.741317801159));
#118027=CARTESIAN_POINT('Ctrl Pts',(1.89511814408961,25.8389196837459,89.6935296954762));
#118028=CARTESIAN_POINT('Ctrl Pts',(1.98562111022021,25.8928708578754,89.645123576841));
#118029=CARTESIAN_POINT('Ctrl Pts',(1.99510975164078,25.8985272840393,89.6400485133162));
#118030=CARTESIAN_POINT('Ctrl Pts',(2.00459768683022,25.9041712877118,89.6349666568877));
#118031=CARTESIAN_POINT('Ctrl Pts',(2.01408488454097,25.9098028720523,89.6298780152039));
#118032=CARTESIAN_POINT('Ctrl Pts',(2.27638611268886,26.0655044326133,89.4891876866217));
#118033=CARTESIAN_POINT('Ctrl Pts',(2.5381215790732,26.2117095514659,89.3433083869172));
#118034=CARTESIAN_POINT('Ctrl Pts',(2.79864368999521,26.3485037793546,89.1924156666076));
#118035=CARTESIAN_POINT('Ctrl Pts',(2.83590914671666,26.3680710220776,89.1708317552905));
#118036=CARTESIAN_POINT('Ctrl Pts',(2.87314982374135,26.3874457695934,89.1491453083512));
#118037=CARTESIAN_POINT('Ctrl Pts',(2.91036387529036,26.4066283314947,89.1273568819364));
#118038=CARTESIAN_POINT('Ctrl Pts',(2.95962816543374,26.4320223763747,89.0985131705966));
#118039=CARTESIAN_POINT('Ctrl Pts',(3.00884579357381,26.4570796201783,89.0694907422277));
#118040=CARTESIAN_POINT('Ctrl Pts',(3.05801251725147,26.4818008189935,89.0402909133547));
#118041=CARTESIAN_POINT('Ctrl Pts',(3.15723971555294,26.5316925976924,88.9813604621628));
#118042=CARTESIAN_POINT('Ctrl Pts',(3.25625952770616,26.5802156066599,88.9217074232645));
#118043=CARTESIAN_POINT('Ctrl Pts',(3.35503904348991,26.6273747875817,88.8613446270082));
#118044=CARTESIAN_POINT('Ctrl Pts',(3.42890125067334,26.6626379812125,88.8162084535023));
#118045=CARTESIAN_POINT('Ctrl Pts',(3.50262907322627,26.6971386911426,88.7706754717244));
#118046=CARTESIAN_POINT('Ctrl Pts',(3.57620910916385,26.7308791747741,88.724751175111));
#118047=CARTESIAN_POINT('Ctrl Pts',(3.61299912713264,26.7477494165898,88.7017890268044));
#118048=CARTESIAN_POINT('Ctrl Pts',(3.64975220037152,26.7644296018314,88.6787290532671));
#118049=CARTESIAN_POINT('Ctrl Pts',(3.68646667213144,26.7809200510704,88.6555719581755));
#118050=CARTESIAN_POINT('Ctrl Pts',(3.71420411411316,26.7933784321145,88.6380769881874));
#118051=CARTESIAN_POINT('Ctrl Pts',(3.74287781855371,26.8061518366951,88.6199185032941));
#118052=CARTESIAN_POINT('Ctrl Pts',(3.77031481493722,26.8182802241769,88.6024743503514));
#118053=CARTESIAN_POINT('Ctrl Pts',(3.77919460759156,26.8222054922552,88.5968286718305));
#118054=CARTESIAN_POINT('Ctrl Pts',(3.78794498704772,26.8260634946765,88.5912580810618));
#118055=CARTESIAN_POINT('Ctrl Pts',(3.79649264115169,26.8298225071378,88.5858100219609));
#118056=CARTESIAN_POINT('Ctrl Pts',(3.90574097342447,26.877866781906,88.516177890892));
#118057=CARTESIAN_POINT('Ctrl Pts',(4.01538651343084,26.924563711977,88.4452071775689));
#118058=CARTESIAN_POINT('Ctrl Pts',(4.12536961495221,26.9698843234981,88.3728825083693));
#118059=CARTESIAN_POINT('Ctrl Pts',(4.38795683492624,27.0780883404992,88.2002056738561));
#118060=CARTESIAN_POINT('Ctrl Pts',(4.65246842891141,27.1784438479384,88.0198092728228));
#118061=CARTESIAN_POINT('Ctrl Pts',(4.91808261803891,27.2705546094886,87.8315435610201));
#118062=CARTESIAN_POINT('Ctrl Pts',(5.00364879866118,27.3002275952803,87.7708947758253));
#118063=CARTESIAN_POINT('Ctrl Pts',(5.08932938844843,27.3290453301415,87.7094295101056));
#118064=CARTESIAN_POINT('Ctrl Pts',(5.17509696863496,27.3569956224824,87.6471432192937));
#118065=CARTESIAN_POINT('Ctrl Pts',(5.44404841356497,27.4446426272707,87.4518248032119));
#118066=CARTESIAN_POINT('Ctrl Pts',(5.71385425895366,27.5237565399761,87.2484310772638));
#118067=CARTESIAN_POINT('Ctrl Pts',(5.98365442899377,27.5939687504165,87.0368916265424));
#118068=CARTESIAN_POINT('Ctrl Pts',(6.05136012798605,27.6115883345144,86.9838063139075));
#118069=CARTESIAN_POINT('Ctrl Pts',(6.11906554879761,27.628647551287,86.9302081419426));
#118070=CARTESIAN_POINT('Ctrl Pts',(6.18675729780204,27.6451410027722,86.8760962144203));
#118071=CARTESIAN_POINT('Ctrl Pts',(6.24335188846402,27.658930573128,86.8308552148436));
#118072=CARTESIAN_POINT('Ctrl Pts',(6.29993692536935,27.672324676065,86.7852550990612));
#118073=CARTESIAN_POINT('Ctrl Pts',(6.35650433239512,27.68532020831,86.7392959497498));
#118074=CARTESIAN_POINT('Ctrl Pts',(6.49958850185862,27.7181916980208,86.6230447893338));
#118075=CARTESIAN_POINT('Ctrl Pts',(6.64255971585015,27.7485128921454,86.5044963583867));
#118076=CARTESIAN_POINT('Ctrl Pts',(6.7852886742244,27.7762356542623,86.3836534502605));
#118077=CARTESIAN_POINT('Ctrl Pts',(6.85665315341153,27.7900970353207,86.3232319961974));
#118078=CARTESIAN_POINT('Ctrl Pts',(6.92795709856489,27.8033088083776,86.2622369578808));
#118079=CARTESIAN_POINT('Ctrl Pts',(6.99918458829304,27.8158652735421,86.2006688566683));
#118080=CARTESIAN_POINT('Ctrl Pts',(7.03479833315711,27.8221435061243,86.169884806062));
#118081=CARTESIAN_POINT('Ctrl Pts',(7.07039296614475,27.8282579117335,86.1389574921));
#118082=CARTESIAN_POINT('Ctrl Pts',(7.1059665142924,27.834207785269,86.1078869900565));
#118083=CARTESIAN_POINT('Ctrl Pts',(7.12375328836623,27.8371827220367,86.0923517390348));
#118084=CARTESIAN_POINT('Ctrl Pts',(7.1415347913618,27.8401165257861,86.0767806911431));
#118085=CARTESIAN_POINT('Ctrl Pts',(7.15931077778746,27.8430091094421,86.0611738564153));
#118086=CARTESIAN_POINT('Ctrl Pts',(7.16020518693599,27.8431546514797,86.0603885894025));
#118087=CARTESIAN_POINT('Ctrl Pts',(7.16110281836779,27.8433006095559,86.0596003904142));
#118088=CARTESIAN_POINT('Ctrl Pts',(7.16200318248296,27.8434469037773,86.0588096872644));
#118089=CARTESIAN_POINT('Ctrl Pts',(7.17899715712277,27.8462081425327,86.0438855148673));
#118090=CARTESIAN_POINT('Ctrl Pts',(7.19696213785824,27.8490860148214,86.0280666995787));
#118091=CARTESIAN_POINT('Ctrl Pts',(7.2126219330494,27.8515631175667,86.014246018903));
#118092=CARTESIAN_POINT('Ctrl Pts',(7.3955209150022,27.8804945029882,85.8528270223818));
#118093=CARTESIAN_POINT('Ctrl Pts',(7.58290941906807,27.9057765944473,85.6831190222835));
#118094=CARTESIAN_POINT('Ctrl Pts',(7.77409387939456,27.9268419894547,85.5047753250708));
#118095=CARTESIAN_POINT('Ctrl Pts',(7.89515415183026,27.9401808479279,85.3918459764464));
#118096=CARTESIAN_POINT('Ctrl Pts',(8.01773533519229,27.9518288665838,85.2754541736625));
#118097=CARTESIAN_POINT('Ctrl Pts',(8.14165068493019,27.9616413427991,85.1555130160333));
#118098=CARTESIAN_POINT('Ctrl Pts',(8.33529254401225,27.9769752472796,84.9680816058579));
#118099=CARTESIAN_POINT('Ctrl Pts',(8.532195054996,27.9878261331155,84.7719813593696));
#118100=CARTESIAN_POINT('Ctrl Pts',(8.73159286517084,27.9936606308062,84.5669176085115));
#118101=CARTESIAN_POINT('Ctrl Pts',(8.87368832939101,27.9978184280114,84.4207844646853));
#118102=CARTESIAN_POINT('Ctrl Pts',(9.01704988471146,27.9994288667593,84.2700997131144));
#118103=CARTESIAN_POINT('Ctrl Pts',(9.16138571517198,27.9983013850854,84.1147624618979));
#118104=CARTESIAN_POINT('Ctrl Pts',(9.35575610573425,27.9967830576361,83.9055769665743));
#118105=CARTESIAN_POINT('Ctrl Pts',(9.55189495406335,27.9902984775844,83.6879527320489));
#118106=CARTESIAN_POINT('Ctrl Pts',(9.74904736009992,27.9784210280426,83.4616906788339));
#118107=CARTESIAN_POINT('Ctrl Pts',(9.75943215812474,27.9777953957359,83.4497725604069));
#118108=CARTESIAN_POINT('Ctrl Pts',(9.76981975905456,27.9771548047027,83.4378304824439));
#118109=CARTESIAN_POINT('Ctrl Pts',(9.78021004950441,27.9764991939486,83.4258644180379));
#118110=CARTESIAN_POINT('Ctrl Pts',(9.93003295121258,27.9670456078297,83.2533196273041));
#118111=CARTESIAN_POINT('Ctrl Pts',(10.0804161000811,27.9544685945203,83.0757866926596));
#118112=CARTESIAN_POINT('Ctrl Pts',(10.2310127297883,27.9385884831185,82.8931903393292));
#118113=CARTESIAN_POINT('Ctrl Pts',(10.2319927570955,27.9384851412121,82.8920020696262));
#118114=CARTESIAN_POINT('Ctrl Pts',(10.2329727934239,27.938381659436,82.8908135854978));
#118115=CARTESIAN_POINT('Ctrl Pts',(10.233952838676,27.9382780377418,82.8896248869249));
#118116=CARTESIAN_POINT('Ctrl Pts',(10.3082724870422,27.930420106831,82.799482457522));
#118117=CARTESIAN_POINT('Ctrl Pts',(10.3826435118955,27.9217575070292,82.7081067746664));
#118118=CARTESIAN_POINT('Ctrl Pts',(10.4570232118485,27.9122715604355,82.615491198011));
#118119=CARTESIAN_POINT('Ctrl Pts',(10.494703480398,27.9074660420573,82.5685727538327));
#118120=CARTESIAN_POINT('Ctrl Pts',(10.5323859748428,27.902449222046,82.5213361058194));
#118121=CARTESIAN_POINT('Ctrl Pts',(10.5700650950581,27.8972187339656,82.4737804394676));
#118122=CARTESIAN_POINT('Ctrl Pts',(10.5889046551658,27.8946034899254,82.4500026062917));
#118123=CARTESIAN_POINT('Ctrl Pts',(10.6077433716528,27.8919348288679,82.4261450184844));
#118124=CARTESIAN_POINT('Ctrl Pts',(10.6265805403487,27.8892124574999,82.4022075787539));
#118125=CARTESIAN_POINT('Ctrl Pts',(10.6359991246967,27.8878512718159,82.3902388588887));
#118126=CARTESIAN_POINT('Ctrl Pts',(10.6454173220933,27.8864766585542,82.3782501760398));
#118127=CARTESIAN_POINT('Ctrl Pts',(10.6548350442347,27.8850885813009,82.3662415183625));
#118128=CARTESIAN_POINT('Ctrl Pts',(10.6595439053054,27.8843945426743,82.3602371895238));
#118129=CARTESIAN_POINT('Ctrl Pts',(10.6642526475621,27.8836971380498,82.3542278669779));
#118130=CARTESIAN_POINT('Ctrl Pts',(10.6689612599484,27.8829963628918,82.348213549265));
#118131=CARTESIAN_POINT('Ctrl Pts',(10.6736698723347,27.8822955877338,82.3421992315521));
#118132=CARTESIAN_POINT('Ctrl Pts',(10.6795441809366,27.8814162537848,82.3346882475515));
#118133=CARTESIAN_POINT('Ctrl Pts',(10.6830866964339,27.8808839212869,82.3301556091715));
#118134=CARTESIAN_POINT('Ctrl Pts',(10.7537849753811,27.8702601169703,82.2396973647956));
#118135=CARTESIAN_POINT('Ctrl Pts',(10.8291598045365,27.8581390422069,82.1420941961379));
#118136=CARTESIAN_POINT('Ctrl Pts',(10.9088955347453,27.8442893594117,82.0371953640855));
#118137=CARTESIAN_POINT('Ctrl Pts',(10.9894121916854,27.8303040336935,81.9312691594636));
#118138=CARTESIAN_POINT('Ctrl Pts',(11.0743757019637,27.8145558305146,81.8179034621183));
#118139=CARTESIAN_POINT('Ctrl Pts',(11.1634132907465,27.7967856191051,81.6969321954422));
#118140=CARTESIAN_POINT('Ctrl Pts',(11.2188687161481,27.7857177695973,81.6215874657993));
#118141=CARTESIAN_POINT('Ctrl Pts',(11.2759036035297,27.7738651429691,81.5432921853156));
#118142=CARTESIAN_POINT('Ctrl Pts',(11.3344183799878,27.7611617527346,81.4620047494625));
#118143=CARTESIAN_POINT('Ctrl Pts',(11.4301282618082,27.7403834117471,81.3290466942514));
#118144=CARTESIAN_POINT('Ctrl Pts',(11.5298000370535,27.7173292049529,81.1880834873095));
#118145=CARTESIAN_POINT('Ctrl Pts',(11.6329585192826,27.6917064185804,81.0389322040532));
#118146=CARTESIAN_POINT('Ctrl Pts',(11.7358149219911,27.6661586635467,80.8902176812761));
#118147=CARTESIAN_POINT('Ctrl Pts',(11.8421376498616,27.6380569513037,80.7333626172256));
#118148=CARTESIAN_POINT('Ctrl Pts',(11.9514044066712,27.6071058859235,80.5681872211007));
#118149=CARTESIAN_POINT('Ctrl Pts',(12.0492938537255,27.579377574365,80.4202105750855));
#118150=CARTESIAN_POINT('Ctrl Pts',(12.1495455023141,27.5493621274191,80.2655559235485));
#118151=CARTESIAN_POINT('Ctrl Pts',(12.2517485599061,27.5168474912581,80.1040985739415));
#118152=CARTESIAN_POINT('Ctrl Pts',(12.296333474959,27.5026633530789,80.0336646516451));
#118153=CARTESIAN_POINT('Ctrl Pts',(12.3412893211916,27.4880036350616,79.9619362240762));
#118154=CARTESIAN_POINT('Ctrl Pts',(12.3865799860944,27.4728509251013,79.888903372782));
#118155=CARTESIAN_POINT('Ctrl Pts',(12.4004630852323,27.4682061141885,79.8665163683735));
#118156=CARTESIAN_POINT('Ctrl Pts',(12.4143776401482,27.4635149835819,79.8440067925359));
#118157=CARTESIAN_POINT('Ctrl Pts',(12.4283225849059,27.4587770342044,79.8213743700025));
#118158=CARTESIAN_POINT('Ctrl Pts',(12.4371238517049,27.4557867063633,79.8070900546119));
#118159=CARTESIAN_POINT('Ctrl Pts',(12.4459372238459,27.4527777286304,79.7927568042114));
#118160=CARTESIAN_POINT('Ctrl Pts',(12.4547624356809,27.4497499808059,79.7783745484681));
#118161=CARTESIAN_POINT('Ctrl Pts',(12.4661664835309,27.4458374876313,79.7597896197714));
#118162=CARTESIAN_POINT('Ctrl Pts',(12.4775903008183,27.4418936486109,79.7411228625664));
#118163=CARTESIAN_POINT('Ctrl Pts',(12.489033314005,27.4379182106952,79.7223741203786));
#118164=CARTESIAN_POINT('Ctrl Pts',(12.4947548205984,27.4359304917374,79.7129997492847));
#118165=CARTESIAN_POINT('Ctrl Pts',(12.500481126124,27.4339348730558,79.70360488192));
#118166=CARTESIAN_POINT('Ctrl Pts',(12.5062121581154,27.4319313223091,79.694189499433));
#118167=CARTESIAN_POINT('Ctrl Pts',(12.5119431901068,27.4299277715624,79.6847741169461));
#118168=CARTESIAN_POINT('Ctrl Pts',(12.5166768585406,27.4282688187441,79.676989005964));
#118169=CARTESIAN_POINT('Ctrl Pts',(12.5234193609175,27.4258968418557,79.6658817875526));
#118170=CARTESIAN_POINT('Ctrl Pts',(12.6277194954064,27.389204602886,79.4940636243047));
#118171=CARTESIAN_POINT('Ctrl Pts',(12.7267772690378,27.3524203174733,79.3266390217625));
#118172=CARTESIAN_POINT('Ctrl Pts',(12.8209630720956,27.3158288233724,79.1637887314953));
#118173=CARTESIAN_POINT('Ctrl Pts',(12.9170176284925,27.2785113124562,78.9977073064514));
#118174=CARTESIAN_POINT('Ctrl Pts',(13.0080050168062,27.2413940893072,78.8363833821447));
#118175=CARTESIAN_POINT('Ctrl Pts',(13.0942922600167,27.2047381959935,78.6799821906079));
#118176=CARTESIAN_POINT('Ctrl Pts',(13.1831069669234,27.1670086046897,78.518999808168));
#118177=CARTESIAN_POINT('Ctrl Pts',(13.2669422569155,27.1297675963549,78.3632326678671));
#118178=CARTESIAN_POINT('Ctrl Pts',(13.3461699531508,27.0932597216902,78.2128348956482));
#118179=CARTESIAN_POINT('Ctrl Pts',(13.391271668521,27.0724769922895,78.1272184024616));
#118180=CARTESIAN_POINT('Ctrl Pts',(13.4348797008029,27.0519311347474,78.043341470321));
#118181=CARTESIAN_POINT('Ctrl Pts',(13.477058519881,27.03166203572,77.9612291258042));
#118182=CARTESIAN_POINT('Ctrl Pts',(13.5102451213573,27.0157141612559,77.8966225362097));
#118183=CARTESIAN_POINT('Ctrl Pts',(13.5425468915552,26.9999375445627,77.8331082976471));
#118184=CARTESIAN_POINT('Ctrl Pts',(13.573994157241,26.984350213617,77.7706978590314));
#118185=CARTESIAN_POINT('Ctrl Pts',(13.647200350837,26.9480644144555,77.6254123929643));
#118186=CARTESIAN_POINT('Ctrl Pts',(13.7157782150303,26.9128067215343,77.4861101507085));
#118187=CARTESIAN_POINT('Ctrl Pts',(13.7800855430065,26.878778616932,77.3529178756503));
#118188=CARTESIAN_POINT('Ctrl Pts',(13.8454410221642,26.8441958850552,77.2175546871853));
#118189=CARTESIAN_POINT('Ctrl Pts',(13.9063856804312,26.8108829197527,77.0885020861424));
#118190=CARTESIAN_POINT('Ctrl Pts',(13.9632588799502,26.7790170672471,76.965870056256));
#118191=CARTESIAN_POINT('Ctrl Pts',(14.021432781162,26.7464224361841,76.840433406791));
#118192=CARTESIAN_POINT('Ctrl Pts',(14.0753469777581,26.7153416801476,76.7217142165492));
#118193=CARTESIAN_POINT('Ctrl Pts',(14.1253256651883,26.685932309831,76.6098087379326));
#118194=CARTESIAN_POINT('Ctrl Pts',(14.1601432684105,26.6654443010547,76.5318498968105));
#118195=CARTESIAN_POINT('Ctrl Pts',(14.1930500706757,26.6457667714177,76.457197435002));
#118196=CARTESIAN_POINT('Ctrl Pts',(14.224144487831,26.6269447605154,76.3858785370778));
#118197=CARTESIAN_POINT('Origin',(-10.9843331791359,89.,65.395787724084));
#118198=CARTESIAN_POINT('',(12.8491777742141,90.5,75.7863477566628));
#118199=CARTESIAN_POINT('Origin',(12.8491780888091,89.,75.786347893815));
#118200=CARTESIAN_POINT('',(0.214666887831327,89.,90.5121648016016));
#118201=CARTESIAN_POINT('Origin',(-10.9843331791359,89.,65.395787724084));
#118202=CARTESIAN_POINT('',(-0.396188735614809,90.4999999999959,89.1421781913432));
#118203=CARTESIAN_POINT('Origin',(-0.396187662550911,89.,89.14218059794));
#118204=CARTESIAN_POINT('Origin',(-10.9843331791359,90.5,65.395787724084));
#118205=CARTESIAN_POINT('Origin',(6.43246351666909,89.,72.98888938658));
#118206=CARTESIAN_POINT('',(12.8491777735034,90.5,70.191431016807));
#118207=CARTESIAN_POINT('Origin',(12.8491780888091,89.,70.191430879345));
#118208=CARTESIAN_POINT('Origin',(6.43246351666909,90.5,72.98888938658));
#118209=CARTESIAN_POINT('Origin',(-10.9843331791359,89.,80.581991049076));
#118210=CARTESIAN_POINT('',(-0.396188735973519,90.4999999999959,56.8356005826213));
#118211=CARTESIAN_POINT('',(0.214666887829776,89.,55.4656139715578));
#118212=CARTESIAN_POINT('Origin',(-0.396187662550911,89.,56.83559817522));
#118213=CARTESIAN_POINT('Origin',(-10.9843331791359,89.,80.581991049076));
#118214=CARTESIAN_POINT('Origin',(-10.9843331791359,90.5,80.581991049076));
#118215=CARTESIAN_POINT('Ctrl Pts',(20.8483779149991,16.41007210111,65.906087946997));
#118216=CARTESIAN_POINT('Ctrl Pts',(20.1925712483991,16.57554287881,64.475654366764));
#118217=CARTESIAN_POINT('Ctrl Pts',(18.6376319248691,16.98964070821,61.61992743409));
#118218=CARTESIAN_POINT('Ctrl Pts',(16.6713472851791,17.48480467007,58.95952934426));
#118219=CARTESIAN_POINT('Ctrl Pts',(15.5130979896291,17.74010536827,57.61807705647));
#118220=CARTESIAN_POINT('Ctrl Pts',(15.3837024999291,17.76815938829,57.47076094755));
#118221=CARTESIAN_POINT('Ctrl Pts',(16.5559173247791,17.39873241323,67.856902903292));
#118222=CARTESIAN_POINT('Ctrl Pts',(15.9859836856991,17.56285104948,66.616102235752));
#118223=CARTESIAN_POINT('Ctrl Pts',(14.6351635728291,17.97417903959,64.140742823463));
#118224=CARTESIAN_POINT('Ctrl Pts',(12.9298166594891,18.46868755045,61.83930771341));
#118225=CARTESIAN_POINT('Ctrl Pts',(11.9267347229591,18.72463122147,60.6803866708301));
#118226=CARTESIAN_POINT('Ctrl Pts',(11.8146919425591,18.75276856151,60.55313564187));
#118227=CARTESIAN_POINT('Ctrl Pts',(13.9709992217891,21.16901952499,69.377261511201));
#118228=CARTESIAN_POINT('Ctrl Pts',(13.4841936868091,21.32798172742,68.290595666228));
#118229=CARTESIAN_POINT('Ctrl Pts',(12.3245021055191,21.72874684849,66.102133407878));
#118230=CARTESIAN_POINT('Ctrl Pts',(10.8279137708991,22.22075577646,64.01412309014));
#118231=CARTESIAN_POINT('Ctrl Pts',(9.93074736335909,22.47915144446,62.94493798825));
#118232=CARTESIAN_POINT('Ctrl Pts',(9.83032735308908,22.50760652801,62.8273104973501));
#118233=CARTESIAN_POINT('Ctrl Pts',(14.3007957475191,25.96018691159,69.757147250502));
#118234=CARTESIAN_POINT('Ctrl Pts',(13.8555520737491,26.11259647311,68.717136258303));
#118235=CARTESIAN_POINT('Ctrl Pts',(12.7847401829791,26.49993861813,66.5881181087229));
#118236=CARTESIAN_POINT('Ctrl Pts',(11.3472397804891,26.98877115137,64.46832374737));
#118237=CARTESIAN_POINT('Ctrl Pts',(10.4572738893891,27.25028274335,63.354172063168));
#118238=CARTESIAN_POINT('Ctrl Pts',(10.3573188072491,27.27914160579,63.2312323188751));
#118239=CARTESIAN_POINT('',(10.4221245511888,26.952572131543,63.31891762201));
#118240=CARTESIAN_POINT('Ctrl Pts',(14.22419092811,25.6803054598776,69.5919861772058));
#118241=CARTESIAN_POINT('Ctrl Pts',(14.1934725897366,25.6908438843884,69.5215276352073));
#118242=CARTESIAN_POINT('Ctrl Pts',(14.1589619430435,25.7027345557711,69.4431671438523));
#118243=CARTESIAN_POINT('Ctrl Pts',(14.1204327313001,25.7160784589078,69.3570002391341));
#118244=CARTESIAN_POINT('Ctrl Pts',(14.0817643578833,25.7294705582002,69.2705221126153));
#118245=CARTESIAN_POINT('Ctrl Pts',(14.039048314131,25.7443267224897,69.176180926378));
#118246=CARTESIAN_POINT('Ctrl Pts',(13.9920105642602,25.760760407159,69.074097146258));
#118247=CARTESIAN_POINT('Ctrl Pts',(13.9678857806148,25.769188937185,69.0217402814876));
#118248=CARTESIAN_POINT('Ctrl Pts',(13.9426234552543,25.7780325843239,68.9673471478871));
#118249=CARTESIAN_POINT('Ctrl Pts',(13.9161820562462,25.7873073621252,68.9109366361141));
#118250=CARTESIAN_POINT('Ctrl Pts',(13.8646942311264,25.8053676068691,68.8010916704903));
#118251=CARTESIAN_POINT('Ctrl Pts',(13.8087383000022,25.8250626495538,68.683595516882));
#118252=CARTESIAN_POINT('Ctrl Pts',(13.7479745393579,25.8465122969549,68.5586086826413));
#118253=CARTESIAN_POINT('Ctrl Pts',(13.7324012602,25.8520096747221,68.5265755293268));
#118254=CARTESIAN_POINT('Ctrl Pts',(13.7165119540592,25.8576223016977,68.4940504934647));
#118255=CARTESIAN_POINT('Ctrl Pts',(13.7003004465873,25.8633521726573,68.4610365899567));
#118256=CARTESIAN_POINT('Ctrl Pts',(13.6605676941403,25.8773955023592,68.3801228774186));
#118257=CARTESIAN_POINT('Ctrl Pts',(13.6188999657739,25.8921431903905,68.2962722386112));
#118258=CARTESIAN_POINT('Ctrl Pts',(13.5752017215861,25.9076239016636,68.2095325118103));
#118259=CARTESIAN_POINT('Ctrl Pts',(13.5533525994922,25.9153642573001,68.1661626484099));
#118260=CARTESIAN_POINT('Ctrl Pts',(13.5309957354795,25.9232878687553,68.1220705701642));
#118261=CARTESIAN_POINT('Ctrl Pts',(13.5081185883337,25.9313981582767,68.0772627600019));
#118262=CARTESIAN_POINT('Ctrl Pts',(13.4966800147608,25.9354533030373,68.0548588549208));
#118263=CARTESIAN_POINT('Ctrl Pts',(13.4851113633025,25.939555117315,68.0322760204064));
#118264=CARTESIAN_POINT('Ctrl Pts',(13.4734110270797,25.9437040194584,68.0095150949663));
#118265=CARTESIAN_POINT('Ctrl Pts',(13.4624685152899,25.9475841994596,67.9882283823253));
#118266=CARTESIAN_POINT('Ctrl Pts',(13.4506285380081,25.9517830008408,67.9652732993136));
#118267=CARTESIAN_POINT('Ctrl Pts',(13.4400845638854,25.9555223814671,67.9448944647072));
#118268=CARTESIAN_POINT('Ctrl Pts',(13.439354340207,25.9557813525385,67.943483127066));
#118269=CARTESIAN_POINT('Ctrl Pts',(13.4386303503209,25.9560381137129,67.9420841374378));
#118270=CARTESIAN_POINT('Ctrl Pts',(13.4379133304858,25.9562924038131,67.9406989021384));
#118271=CARTESIAN_POINT('Ctrl Pts',(13.3607550418609,25.9836564849563,67.7916341485257));
#118272=CARTESIAN_POINT('Ctrl Pts',(13.2857009269469,26.0102700616628,67.6499684523326));
#118273=CARTESIAN_POINT('Ctrl Pts',(13.2131177177402,26.035965285323,67.5155491144957));
#118274=CARTESIAN_POINT('Ctrl Pts',(13.139430690727,26.06205127216,67.3790855785548));
#118275=CARTESIAN_POINT('Ctrl Pts',(13.0682903286398,26.087191078862,67.2500902843998));
#118276=CARTESIAN_POINT('Ctrl Pts',(13.0000406297685,26.1112452964015,67.1284103791098));
#118277=CARTESIAN_POINT('Ctrl Pts',(12.9304855521089,26.135759587258,67.004403161466));
#118278=CARTESIAN_POINT('Ctrl Pts',(12.8639328391001,26.1591466630811,66.8879936409601));
#118279=CARTESIAN_POINT('Ctrl Pts',(12.8007048462081,26.1812916013322,66.7790301998885));
#118280=CARTESIAN_POINT('Ctrl Pts',(12.7825538915208,26.1876487819474,66.7477499015427));
#118281=CARTESIAN_POINT('Ctrl Pts',(12.7646766648217,26.193903784652,66.7170833086437));
#118282=CARTESIAN_POINT('Ctrl Pts',(12.7470801615792,26.2000543217691,66.6870270209143));
#118283=CARTESIAN_POINT('Ctrl Pts',(12.7413586970835,26.202054155444,66.6772542847777));
#118284=CARTESIAN_POINT('Ctrl Pts',(12.7356669087703,26.204042946285,66.6675460714649));
#118285=CARTESIAN_POINT('Ctrl Pts',(12.730005029151,26.2060206160786,66.6579022642968));
#118286=CARTESIAN_POINT('Ctrl Pts',(12.6963581285086,26.2177733313468,66.6005919286103));
#118287=CARTESIAN_POINT('Ctrl Pts',(12.6637677778018,26.2291330895811,66.5455560250034));
#118288=CARTESIAN_POINT('Ctrl Pts',(12.6322805997689,26.2400850348388,66.4927709300283));
#118289=CARTESIAN_POINT('Ctrl Pts',(12.6165370107524,26.2455610074676,66.4663783825407));
#118290=CARTESIAN_POINT('Ctrl Pts',(12.6010691618075,26.2509350268608,66.4405485689667));
#118291=CARTESIAN_POINT('Ctrl Pts',(12.5858825271088,26.2562055126126,66.4152786705119));
#118292=CARTESIAN_POINT('Ctrl Pts',(12.5782892097594,26.2588407554886,66.4026437212844));
#118293=CARTESIAN_POINT('Ctrl Pts',(12.5707661926246,26.2614501149547,66.3901487528226));
#118294=CARTESIAN_POINT('Ctrl Pts',(12.563314139175,26.2640333993445,66.3777934235363));
#118295=CARTESIAN_POINT('Ctrl Pts',(12.5595881124501,26.2653250415394,66.3716157588932));
#118296=CARTESIAN_POINT('Ctrl Pts',(12.555879826438,26.2666101649652,66.3654730041698));
#118297=CARTESIAN_POINT('Ctrl Pts',(12.5521893627096,26.2678887465314,66.35936511724));
#118298=CARTESIAN_POINT('Ctrl Pts',(12.5503441308454,26.2685280373144,66.3563111737751));
#118299=CARTESIAN_POINT('Ctrl Pts',(12.5485033545391,26.2691656926326,66.3532659472665));
#118300=CARTESIAN_POINT('Ctrl Pts',(12.5466670439017,26.2698017096539,66.3502294324841));
#118301=CARTESIAN_POINT('Ctrl Pts',(12.5448307332644,26.2704377266752,66.3471929177017));
#118302=CARTESIAN_POINT('Ctrl Pts',(12.5436494615672,26.2708468404772,66.3452399622795));
#118303=CARTESIAN_POINT('Ctrl Pts',(12.5411715190533,26.2717048430112,66.3411460181136));
#118304=CARTESIAN_POINT('Ctrl Pts',(11.962278170298,26.4721501549424,65.3847246990396));
#118305=CARTESIAN_POINT('Ctrl Pts',(11.3231338036213,26.6855355653743,64.460421737533));
#118306=CARTESIAN_POINT('Ctrl Pts',(10.6245339352504,26.893097015685,63.5729680868371));
#118307=CARTESIAN_POINT('Ctrl Pts',(10.5576059451875,26.9129820332934,63.4879473306014));
#118308=CARTESIAN_POINT('Ctrl Pts',(10.4901322849598,26.9328135924601,63.4032648117697));
#118309=CARTESIAN_POINT('Ctrl Pts',(10.4221147584861,26.9525719251785,63.3189269730742));
#118310=CARTESIAN_POINT('Origin',(17.8170756838691,26.95256493355,57.35532384706));
#118311=CARTESIAN_POINT('Ctrl Pts',(15.6451955709591,17.70734006941,57.66551497159));
#118312=CARTESIAN_POINT('Ctrl Pts',(15.4053160301991,17.76750394009,57.5702232381));
#118313=CARTESIAN_POINT('Ctrl Pts',(14.8524063434191,17.89090859263,57.35645087848));
#118314=CARTESIAN_POINT('Ctrl Pts',(13.9432808889591,18.03861939721,57.02808486809));
#118315=CARTESIAN_POINT('Ctrl Pts',(12.9188376719691,18.13614112929,56.68942936417));
#118316=CARTESIAN_POINT('Ctrl Pts',(11.8651204328191,18.16653625119,56.3745849123));
#118317=CARTESIAN_POINT('Ctrl Pts',(10.8194002598291,18.13134446021,56.09433316092));
#118318=CARTESIAN_POINT('Ctrl Pts',(9.75348782079909,18.03185317263,55.8398643760501));
#118319=CARTESIAN_POINT('Ctrl Pts',(8.60334640165909,17.85384778506,55.5992400384));
#118320=CARTESIAN_POINT('Ctrl Pts',(7.32308763312909,17.56641516118,55.37248137399));
#118321=CARTESIAN_POINT('Ctrl Pts',(6.08206864086909,17.18674270191,55.19570687228));
#118322=CARTESIAN_POINT('Ctrl Pts',(5.28049439426909,16.87792525594,55.10601469316));
#118323=CARTESIAN_POINT('Ctrl Pts',(4.94559772960909,16.736925875,55.07276081499));
#118324=CARTESIAN_POINT('Ctrl Pts',(12.0373027887591,18.6574860008,60.7132364091101));
#118325=CARTESIAN_POINT('Ctrl Pts',(11.8364311238391,18.77666302266,60.6457111203401));
#118326=CARTESIAN_POINT('Ctrl Pts',(11.3704473225491,19.03747034031,60.48554158426));
#118327=CARTESIAN_POINT('Ctrl Pts',(10.5891293699691,19.41263661724,60.205607251));
#118328=CARTESIAN_POINT('Ctrl Pts',(9.68271453490909,19.76202380549,59.87027563324));
#118329=CARTESIAN_POINT('Ctrl Pts',(8.71691702481909,20.03893729113,59.50718051343));
#118330=CARTESIAN_POINT('Ctrl Pts',(7.72171670189909,20.22883548888,59.13283164616));
#118331=CARTESIAN_POINT('Ctrl Pts',(6.66769425441909,20.33228659359,58.7406236989601));
#118332=CARTESIAN_POINT('Ctrl Pts',(5.48364232856909,20.33573846041,58.30895983799));
#118333=CARTESIAN_POINT('Ctrl Pts',(4.10481591372909,20.19187673024,57.82159800215));
#118334=CARTESIAN_POINT('Ctrl Pts',(2.69831955594909,19.86874669915,57.3431750580601));
#118335=CARTESIAN_POINT('Ctrl Pts',(1.74651831724909,19.53037562758,57.0299445529801));
#118336=CARTESIAN_POINT('Ctrl Pts',(1.34062365781909,19.36074341708,56.8973330406101));
#118337=CARTESIAN_POINT('Ctrl Pts',(10.0358374714891,22.38383994892,63.019033831034));
#118338=CARTESIAN_POINT('Ctrl Pts',(9.84598787858909,22.55213797617,62.881678099));
#118339=CARTESIAN_POINT('Ctrl Pts',(9.39884778054908,22.91846423345,62.55638442729));
#118340=CARTESIAN_POINT('Ctrl Pts',(8.62363209760909,23.43709896161,61.99154664531));
#118341=CARTESIAN_POINT('Ctrl Pts',(7.69183910901909,23.90734852226,61.32157759184));
#118342=CARTESIAN_POINT('Ctrl Pts',(6.6663237622691,24.26349060744,60.60358414559));
#118343=CARTESIAN_POINT('Ctrl Pts',(5.58132317884909,24.48664443975,59.87044986124));
#118344=CARTESIAN_POINT('Ctrl Pts',(4.40709163424909,24.57682141001,59.10837536092));
#118345=CARTESIAN_POINT('Ctrl Pts',(3.06417177756909,24.51032471516,58.27536784085));
#118346=CARTESIAN_POINT('Ctrl Pts',(1.47641806860909,24.21374904793,57.34023061635));
#118347=CARTESIAN_POINT('Ctrl Pts',(-0.16335550177091,23.64851785533,56.42568615944));
#118348=CARTESIAN_POINT('Ctrl Pts',(-1.27954381589091,23.08548524468,55.82771633623));
#118349=CARTESIAN_POINT('Ctrl Pts',(-1.75618235438091,22.80589742487,55.57457975359));
#118350=CARTESIAN_POINT('Ctrl Pts',(10.5754944201391,27.14617507505,63.506087747273));
#118351=CARTESIAN_POINT('Ctrl Pts',(10.3635337299691,27.33076219475,63.233915867281));
#118352=CARTESIAN_POINT('Ctrl Pts',(9.85835504468908,27.72144576791,62.60188493816));
#118353=CARTESIAN_POINT('Ctrl Pts',(8.96468660719909,28.23256140694,61.5518599865));
#118354=CARTESIAN_POINT('Ctrl Pts',(7.87596066045909,28.63622689438,60.36556961314));
#118355=CARTESIAN_POINT('Ctrl Pts',(6.67097845427909,28.86730764335,59.15176956186));
#118356=CARTESIAN_POINT('Ctrl Pts',(5.39779469245909,28.91635220029,57.96271623088));
#118357=CARTESIAN_POINT('Ctrl Pts',(4.02739324090909,28.78323759979,56.77137740692));
#118358=CARTESIAN_POINT('Ctrl Pts',(2.47484018625909,28.42805287238,55.51415168585));
#118359=CARTESIAN_POINT('Ctrl Pts',(0.665369677529091,27.75379664694,54.15318031056));
#118360=CARTESIAN_POINT('Ctrl Pts',(-1.16653927068091,26.7608832154,52.87171230437));
#118361=CARTESIAN_POINT('Ctrl Pts',(-2.38450511710091,25.88299926927,52.06077692591));
#118362=CARTESIAN_POINT('Ctrl Pts',(-2.89859565635591,25.46348290666,51.72223367689));
#118363=CARTESIAN_POINT('',(0.214722992422839,21.3110521316348,55.4657680174377));
#118364=CARTESIAN_POINT('Ctrl Pts',(10.4221245511888,26.952572131543,63.31891762201));
#118365=CARTESIAN_POINT('Ctrl Pts',(10.2814066492482,26.993572523789,63.1444235191351));
#118366=CARTESIAN_POINT('Ctrl Pts',(10.1346923009253,27.0285147217768,62.9668635799751));
#118367=CARTESIAN_POINT('Ctrl Pts',(9.98184065432509,27.0565650645596,62.786777213206));
#118368=CARTESIAN_POINT('Ctrl Pts',(9.96268076478778,27.0600811632157,62.7642034629637));
#118369=CARTESIAN_POINT('Ctrl Pts',(9.94342447433925,27.0634889599087,62.7415900735869));
#118370=CARTESIAN_POINT('Ctrl Pts',(9.92407153256859,27.0667868020637,62.7189381553192));
#118371=CARTESIAN_POINT('Ctrl Pts',(9.90528602597828,27.0699879503061,62.6969503994038));
#118372=CARTESIAN_POINT('Ctrl Pts',(9.88640945302957,27.0730854973525,62.6749263412792));
#118373=CARTESIAN_POINT('Ctrl Pts',(9.8674415908049,27.0760779304426,62.6528670059662));
#118374=CARTESIAN_POINT('Ctrl Pts',(9.79869381173847,27.086923808935,62.5729143843959));
#118375=CARTESIAN_POINT('Ctrl Pts',(9.72874671454407,27.0963888624975,62.4924982081541));
#118376=CARTESIAN_POINT('Ctrl Pts',(9.65759474141652,27.1044036647129,62.4116697829035));
#118377=CARTESIAN_POINT('Ctrl Pts',(9.61220315905006,27.109516728187,62.3601050832748));
#118378=CARTESIAN_POINT('Ctrl Pts',(9.56632112929409,27.1140395147692,62.3083725197215));
#118379=CARTESIAN_POINT('Ctrl Pts',(9.5199475857354,27.11795403698,62.2564859095843));
#118380=CARTESIAN_POINT('Ctrl Pts',(9.49676081395605,27.1199112980854,62.2305426045156));
#118381=CARTESIAN_POINT('Ctrl Pts',(9.47345116346099,27.121716493098,62.2045607880786));
#118382=CARTESIAN_POINT('Ctrl Pts',(9.45001849613942,27.1233673617675,62.1785421858642));
#118383=CARTESIAN_POINT('Ctrl Pts',(9.43830216247863,27.1241927961022,62.1655328847569));
#118384=CARTESIAN_POINT('Ctrl Pts',(9.42655507458789,27.1249796488512,62.1525143872246));
#118385=CARTESIAN_POINT('Ctrl Pts',(9.41477721697565,27.1257276380715,62.1394869111806));
#118386=CARTESIAN_POINT('Ctrl Pts',(9.40594382376647,27.1262886299868,62.1297163041475));
#118387=CARTESIAN_POINT('Ctrl Pts',(9.39709312258736,27.1268277611672,62.119940646703));
#118388=CARTESIAN_POINT('Ctrl Pts',(9.38822510715136,27.1273449126714,62.1101600311071));
#118389=CARTESIAN_POINT('Ctrl Pts',(9.38526910200603,27.1275172965062,62.1068998259085));
#118390=CARTESIAN_POINT('Ctrl Pts',(9.38137384331691,27.1277402806879,62.1026062763353));
#118391=CARTESIAN_POINT('Ctrl Pts',(9.37935132008672,27.1278547332123,62.100377766239));
#118392=CARTESIAN_POINT('Ctrl Pts',(9.33983231774599,27.1300910732023,62.0568338927249));
#118393=CARTESIAN_POINT('Ctrl Pts',(9.29613981450071,27.1319600387806,62.0089688918052));
#118394=CARTESIAN_POINT('Ctrl Pts',(9.24818733537905,27.1332027091348,61.956876784848));
#118395=CARTESIAN_POINT('Ctrl Pts',(9.20000809183754,27.1344512560031,61.9045383374173));
#118396=CARTESIAN_POINT('Ctrl Pts',(9.14752838831708,27.1350675138919,61.847932585123));
#118397=CARTESIAN_POINT('Ctrl Pts',(9.09064900126491,27.1347427847506,61.7871776110701));
#118398=CARTESIAN_POINT('Ctrl Pts',(9.06506963794882,27.1345967500425,61.7598553483823));
#118399=CARTESIAN_POINT('Ctrl Pts',(9.03860033203933,27.1342597963946,61.7316942581623));
#118400=CARTESIAN_POINT('Ctrl Pts',(9.01123138962838,27.1337008833808,61.7027066707963));
#118401=CARTESIAN_POINT('Ctrl Pts',(8.98852386077562,27.13323716311,61.67865618077));
#118402=CARTESIAN_POINT('Ctrl Pts',(8.96519703880106,27.1326206187768,61.6540367698852));
#118403=CARTESIAN_POINT('Ctrl Pts',(8.94124519193602,27.1318325819045,61.6288560163335));
#118404=CARTESIAN_POINT('Ctrl Pts',(8.93903805036325,27.1317599650015,61.626535632093));
#118405=CARTESIAN_POINT('Ctrl Pts',(8.93682560129779,27.1316858912838,61.6242104815798));
#118406=CARTESIAN_POINT('Ctrl Pts',(8.93460784034833,27.1316103457679,61.6218805709601));
#118407=CARTESIAN_POINT('Ctrl Pts',(8.91452314150809,27.1309261832415,61.6007802115493));
#118408=CARTESIAN_POINT('Ctrl Pts',(8.89452126022697,27.1301435289572,61.5798314489841));
#118409=CARTESIAN_POINT('Ctrl Pts',(8.87341065881786,27.1292010067377,61.5577961809475));
#118410=CARTESIAN_POINT('Ctrl Pts',(8.86689381231496,27.1289100499567,61.5509938896881));
#118411=CARTESIAN_POINT('Ctrl Pts',(8.86027120104815,27.1286035315052,61.5440881800932));
#118412=CARTESIAN_POINT('Ctrl Pts',(8.8535074709814,27.1282787291607,61.5370429720019));
#118413=CARTESIAN_POINT('Ctrl Pts',(8.76572859058654,27.1240634831555,61.4456111034465));
#118414=CARTESIAN_POINT('Ctrl Pts',(8.68104973639839,27.1180728992385,61.3586725401621));
#118415=CARTESIAN_POINT('Ctrl Pts',(8.59964480291943,27.1107438490325,61.2760963895947));
#118416=CARTESIAN_POINT('Ctrl Pts',(8.57468192486981,27.1084963908172,61.2507743570308));
#118417=CARTESIAN_POINT('Ctrl Pts',(8.55002670460079,27.1061227585507,61.2258625402158));
#118418=CARTESIAN_POINT('Ctrl Pts',(8.52568363313075,27.1036347301996,61.201357175705));
#118419=CARTESIAN_POINT('Ctrl Pts',(8.47382023755181,27.0983339365531,61.1491480115904));
#118420=CARTESIAN_POINT('Ctrl Pts',(8.42337401150025,27.0925143842389,61.0987837393931));
#118421=CARTESIAN_POINT('Ctrl Pts',(8.37438496064367,27.0862842171409,61.0502283048172));
#118422=CARTESIAN_POINT('Ctrl Pts',(8.34989043521538,27.0831691335919,61.0259505875293));
#118423=CARTESIAN_POINT('Ctrl Pts',(8.32576016401583,27.0799513963409,61.0021251196712));
#118424=CARTESIAN_POINT('Ctrl Pts',(8.30199870177388,27.0766436642737,60.9787474266291));
#118425=CARTESIAN_POINT('Ctrl Pts',(8.2901179706529,27.0749897982401,60.9670585801081));
#118426=CARTESIAN_POINT('Ctrl Pts',(8.27832943929354,27.0733134335021,60.9554816797772));
#118427=CARTESIAN_POINT('Ctrl Pts',(8.26663365856629,27.071616129553,60.9440161775303));
#118428=CARTESIAN_POINT('Ctrl Pts',(8.26078576820267,27.0707674775785,60.9382834264068));
#118429=CARTESIAN_POINT('Ctrl Pts',(8.25496106534509,27.0699135908012,60.9325785249595));
#118430=CARTESIAN_POINT('Ctrl Pts',(8.24915961727369,27.0690546611449,60.9269014049513));
#118431=CARTESIAN_POINT('Ctrl Pts',(8.24335816920229,27.0681957314886,60.9212242849432));
#118432=CARTESIAN_POINT('Ctrl Pts',(8.2386130797743,27.0674877290304,60.9165841299647));
#118433=CARTESIAN_POINT('Ctrl Pts',(8.23182510390789,27.0664629345651,60.9099533214476));
#118434=CARTESIAN_POINT('Ctrl Pts',(8.11648638367961,27.0490500143582,60.7972851294147));
#118435=CARTESIAN_POINT('Ctrl Pts',(8.00223494191034,27.0286870805438,60.6876598283109));
#118436=CARTESIAN_POINT('Ctrl Pts',(7.88922788442964,27.0056723798554,60.5810237234782));
#118437=CARTESIAN_POINT('Ctrl Pts',(7.75397942678112,26.9781280579278,60.453400112796));
#118438=CARTESIAN_POINT('Ctrl Pts',(7.62051474582978,26.9467864738024,60.3300581414355));
#118439=CARTESIAN_POINT('Ctrl Pts',(7.48909721297415,26.912148066346,60.2108850727485));
#118440=CARTESIAN_POINT('Ctrl Pts',(7.42012718180227,26.8939692739878,60.148341132959));
#118441=CARTESIAN_POINT('Ctrl Pts',(7.35172031310869,26.8748818989521,60.0869451782984));
#118442=CARTESIAN_POINT('Ctrl Pts',(7.28391041918654,26.8549548660802,60.0266793543247));
#118443=CARTESIAN_POINT('Ctrl Pts',(7.23308109372499,26.84001784759,59.9815049556671));
#118444=CARTESIAN_POINT('Ctrl Pts',(7.18258713569114,26.8246089951325,59.9369655314101));
#118445=CARTESIAN_POINT('Ctrl Pts',(7.13244179464783,26.8087565024949,59.8930532223584));
#118446=CARTESIAN_POINT('Ctrl Pts',(7.10736912412617,26.8008302561761,59.8710970678326));
#118447=CARTESIAN_POINT('Ctrl Pts',(7.08238360440521,26.7927930998124,59.8492976960571));
#118448=CARTESIAN_POINT('Ctrl Pts',(7.05748680242125,26.7846484759186,59.8276540880368));
#118449=CARTESIAN_POINT('Ctrl Pts',(7.03864287135314,26.778483960037,59.811272439588));
#118450=CARTESIAN_POINT('Ctrl Pts',(7.01912796897405,26.7720165488119,59.7943551656028));
#118451=CARTESIAN_POINT('Ctrl Pts',(7.00058154509988,26.7657948074645,59.778321121133));
#118452=CARTESIAN_POINT('Ctrl Pts',(6.99462423665639,26.7637963180245,59.7731708156536));
#118453=CARTESIAN_POINT('Ctrl Pts',(6.98876691844394,26.7618235394718,59.7681114531265));
#118454=CARTESIAN_POINT('Ctrl Pts',(6.98306410141104,26.759895640288,59.7631895502394));
#118455=CARTESIAN_POINT('Ctrl Pts',(6.92582299967832,26.7405446646773,59.713786747685));
#118456=CARTESIAN_POINT('Ctrl Pts',(6.86780102036232,26.7202464698308,59.6641221341678));
#118457=CARTESIAN_POINT('Ctrl Pts',(6.80900131236983,26.6989614566225,59.6142241745268));
#118458=CARTESIAN_POINT('Ctrl Pts',(6.6750357626757,26.6504670237069,59.5005398073734));
#118459=CARTESIAN_POINT('Ctrl Pts',(6.53703097285645,26.5968507260649,59.3856427811481));
#118460=CARTESIAN_POINT('Ctrl Pts',(6.39506530351964,26.5376331238691,59.2698754606097));
#118461=CARTESIAN_POINT('Ctrl Pts',(6.29292692206693,26.49502852749,59.1865856990769));
#118462=CARTESIAN_POINT('Ctrl Pts',(6.18873892527997,26.4495243827305,59.1028459007061));
#118463=CARTESIAN_POINT('Ctrl Pts',(6.08254064887584,26.4009401198577,59.0187902614544));
#118464=CARTESIAN_POINT('Ctrl Pts',(6.02944151067378,26.3766479884214,58.9767624418286));
#118465=CARTESIAN_POINT('Ctrl Pts',(5.97583981231385,26.3515858274571,58.9346556496021));
#118466=CARTESIAN_POINT('Ctrl Pts',(5.92174144205499,26.3257309408639,58.8924872877607));
#118467=CARTESIAN_POINT('Ctrl Pts',(5.89469225692556,26.3128034975672,58.87140310684));
#118468=CARTESIAN_POINT('Ctrl Pts',(5.86751890463645,26.2996778728634,58.8503035324909));
#118469=CARTESIAN_POINT('Ctrl Pts',(5.84022215204843,26.2863512303691,58.829190754269));
#118470=CARTESIAN_POINT('Ctrl Pts',(5.82657377575442,26.2796879091219,58.818634365158));
#118471=CARTESIAN_POINT('Ctrl Pts',(5.81289454943385,26.2729743334271,58.8080746750166));
#118472=CARTESIAN_POINT('Ctrl Pts',(5.79918457251528,26.2662101484786,58.7975119596882));
#118473=CARTESIAN_POINT('Ctrl Pts',(5.78763485513043,26.2605117855304,58.788613594827));
#118474=CARTESIAN_POINT('Ctrl Pts',(5.77492168842818,26.2542098195369,58.7788360061934));
#118475=CARTESIAN_POINT('Ctrl Pts',(5.76393033383615,26.2487384151678,58.7703961828101));
#118476=CARTESIAN_POINT('Ctrl Pts',(5.76187451049826,26.2477150435079,58.7688175979565));
#118477=CARTESIAN_POINT('Ctrl Pts',(5.75987893234084,26.2467208583818,58.7672857384051));
#118478=CARTESIAN_POINT('Ctrl Pts',(5.75796249058962,26.245765411025,58.7658150144878));
#118479=CARTESIAN_POINT('Ctrl Pts',(5.75464223830328,26.2441100900276,58.7632669722914));
#118480=CARTESIAN_POINT('Ctrl Pts',(5.75132049304372,26.2424518611636,58.7607189918301));
#118481=CARTESIAN_POINT('Ctrl Pts',(5.74799725649708,26.2407907204187,58.758171076555));
#118482=CARTESIAN_POINT('Ctrl Pts',(5.58044261383318,26.1570374756447,58.6297074455561));
#118483=CARTESIAN_POINT('Ctrl Pts',(5.40909309321754,26.0658809328938,58.5014082207791));
#118484=CARTESIAN_POINT('Ctrl Pts',(5.23422053837367,25.9668212156878,58.3736999585156));
#118485=CARTESIAN_POINT('Ctrl Pts',(5.05984397712084,25.86804246301,58.2463539170686));
#118486=CARTESIAN_POINT('Ctrl Pts',(4.88196434708753,25.761404800653,58.1195955448284));
#118487=CARTESIAN_POINT('Ctrl Pts',(4.70089759350769,25.6464293458342,57.9938628415067));
#118488=CARTESIAN_POINT('Ctrl Pts',(4.52764611784975,25.5364165090325,57.8735570650002));
#118489=CARTESIAN_POINT('Ctrl Pts',(4.35147646196849,25.4187699381707,57.7541905673983));
#118490=CARTESIAN_POINT('Ctrl Pts',(4.17274238471399,25.2930685727607,57.6361260281792));
#118491=CARTESIAN_POINT('Ctrl Pts',(3.99912209081811,25.1709636650629,57.5214394484695));
#118492=CARTESIAN_POINT('Ctrl Pts',(3.82308218514099,25.0412577714307,57.4079813739881));
#118493=CARTESIAN_POINT('Ctrl Pts',(3.64498832129322,24.9035899436578,57.29609430042));
#118494=CARTESIAN_POINT('Ctrl Pts',(3.61989910262178,24.8841957985682,57.2803320546323));
#118495=CARTESIAN_POINT('Ctrl Pts',(3.59476918753824,24.8646436889377,57.2646010042274));
#118496=CARTESIAN_POINT('Ctrl Pts',(3.56959966427412,24.8449326566351,57.2489021238195));
#118497=CARTESIAN_POINT('Ctrl Pts',(3.5618666053648,24.8388766589763,57.2440788156571));
#118498=CARTESIAN_POINT('Ctrl Pts',(3.55412980772363,24.8328056597867,57.239258544239));
#118499=CARTESIAN_POINT('Ctrl Pts',(3.54638930684746,24.826719625658,57.2344413338674));
#118500=CARTESIAN_POINT('Ctrl Pts',(3.49031332815,24.7826294142349,57.1995431030552));
#118501=CARTESIAN_POINT('Ctrl Pts',(3.4340429523821,24.7377501024215,57.1648055170815));
#118502=CARTESIAN_POINT('Ctrl Pts',(3.37759196808357,24.6920691766732,57.1302378655454));
#118503=CARTESIAN_POINT('Ctrl Pts',(3.34936647593431,24.669228713799,57.1129540397773));
#118504=CARTESIAN_POINT('Ctrl Pts',(3.32109583321996,24.646187847441,57.0957126950519));
#118505=CARTESIAN_POINT('Ctrl Pts',(3.29278181910187,24.6229450529,57.0785150056188));
#118506=CARTESIAN_POINT('Ctrl Pts',(3.27862481204283,24.6113236556295,57.0699161609022));
#118507=CARTESIAN_POINT('Ctrl Pts',(3.26445696223054,24.5996517763133,57.0613282298503));
#118508=CARTESIAN_POINT('Ctrl Pts',(3.25027849397554,24.587929225742,57.0527513591214));
#118509=CARTESIAN_POINT('Ctrl Pts',(3.24318925984804,24.5820679504564,57.0484629237569));
#118510=CARTESIAN_POINT('Ctrl Pts',(3.23609737111571,24.576194007357,57.0441772534636));
#118511=CARTESIAN_POINT('Ctrl Pts',(3.22900285601976,24.5703073729452,57.0398943666173));
#118512=CARTESIAN_POINT('Ctrl Pts',(3.22190834092382,24.5644207385335,57.035611479771));
#118513=CARTESIAN_POINT('Ctrl Pts',(3.21632152231737,24.5597790772393,57.0322412838866));
#118514=CARTESIAN_POINT('Ctrl Pts',(3.20771145995645,24.5526093723229,57.0270540747882));
#118515=CARTESIAN_POINT('Ctrl Pts',(3.01702554634636,24.3938228647475,56.9121736401804));
#118516=CARTESIAN_POINT('Ctrl Pts',(2.82881053842557,24.2294935613802,56.8019286901944));
#118517=CARTESIAN_POINT('Ctrl Pts',(2.64342884833907,24.0599839636375,56.6961523244788));
#118518=CARTESIAN_POINT('Ctrl Pts',(2.53066793462781,23.9568774642017,56.6318124231565));
#118519=CARTESIAN_POINT('Ctrl Pts',(2.41895457083286,23.8518549938012,56.5691261814459));
#118520=CARTESIAN_POINT('Ctrl Pts',(2.30836409397114,23.7450044702533,56.5080591013602));
#118521=CARTESIAN_POINT('Ctrl Pts',(2.14640352322155,23.5885210887742,56.4186259112216));
#118522=CARTESIAN_POINT('Ctrl Pts',(1.98685270757876,23.4281143258072,56.3326643026614));
#118523=CARTESIAN_POINT('Ctrl Pts',(1.82994511721138,23.2639864925265,56.2500260357267));
#118524=CARTESIAN_POINT('Ctrl Pts',(1.67088138732323,23.0976033030393,56.1662521982765));
#118525=CARTESIAN_POINT('Ctrl Pts',(1.51453385646949,22.9273959923632,56.0858937160226));
#118526=CARTESIAN_POINT('Ctrl Pts',(1.36112026579838,22.7536190886725,56.0088149386751));
#118527=CARTESIAN_POINT('Ctrl Pts',(1.23542781254438,22.6112428803573,55.9456639454923));
#118528=CARTESIAN_POINT('Ctrl Pts',(1.11170426995191,22.466471375799,55.8847148596342));
#118529=CARTESIAN_POINT('Ctrl Pts',(0.990058160464487,22.319466349336,55.8259018516421));
#118530=CARTESIAN_POINT('Ctrl Pts',(0.868248809376559,22.1722640511649,
55.767009920209));
#118531=CARTESIAN_POINT('Ctrl Pts',(0.74852275231373,22.0228197708775,55.7102593206989));
#118532=CARTESIAN_POINT('Ctrl Pts',(0.631054499834477,21.8711790855951,
55.6555578594923));
#118533=CARTESIAN_POINT('Ctrl Pts',(0.512649166714672,21.7183287155893,
55.6004200277836));
#118534=CARTESIAN_POINT('Ctrl Pts',(0.396537737896709,21.5632467730203,
55.5473641780413));
#118535=CARTESIAN_POINT('Ctrl Pts',(0.282886631224853,21.4060296276657,
55.4963092820682));
#118536=CARTESIAN_POINT('Ctrl Pts',(0.260062346259937,21.3744560774204,
55.4860560471577));
#118537=CARTESIAN_POINT('Ctrl Pts',(0.237337252860129,21.3427965692195,
55.4758835564763));
#118538=CARTESIAN_POINT('Ctrl Pts',(0.214712643454674,21.3110521213042,
55.465791216911));
#118539=CARTESIAN_POINT('',(4.86118877219909,16.96274263543,55.19970909287));
#118540=CARTESIAN_POINT('Ctrl Pts',(4.86118877219909,16.96274263543,55.19970909287));
#118541=CARTESIAN_POINT('Ctrl Pts',(3.21558079015593,18.2032496927606,55.9931907979944));
#118542=CARTESIAN_POINT('Ctrl Pts',(1.60457389977557,19.7107791425907,56.0853779332709));
#118543=CARTESIAN_POINT('Ctrl Pts',(0.214754169499088,21.31105212978,55.4656980988));
#118544=CARTESIAN_POINT('Ctrl Pts',(15.2821022274612,17.8079499022762,57.8022939269451));
#118545=CARTESIAN_POINT('Ctrl Pts',(15.092084226211,17.8569950920321,57.7280471206653));
#118546=CARTESIAN_POINT('Ctrl Pts',(14.8978323790944,17.9029043539499,57.6536660080466));
#118547=CARTESIAN_POINT('Ctrl Pts',(14.6993937859133,17.9453287930748,57.5793905280265));
#118548=CARTESIAN_POINT('Ctrl Pts',(14.4630225436543,17.9958629014725,57.4909168737826));
#118549=CARTESIAN_POINT('Ctrl Pts',(14.2207098803036,18.0414524117732,57.4025925276253));
#118550=CARTESIAN_POINT('Ctrl Pts',(13.9725790603985,18.0815246521105,57.3148176057679));
#118551=CARTESIAN_POINT('Ctrl Pts',(13.9004739636052,18.0931693674641,57.2893108217296));
#118552=CARTESIAN_POINT('Ctrl Pts',(13.8278777812175,18.1043481499142,57.263850679352));
#118553=CARTESIAN_POINT('Ctrl Pts',(13.7547940963012,18.115046875106,57.2384476074277));
#118554=CARTESIAN_POINT('Ctrl Pts',(13.5410615600471,18.1463351944148,57.1641565669957));
#118555=CARTESIAN_POINT('Ctrl Pts',(13.3231571973339,18.173517895102,57.0903522859025));
#118556=CARTESIAN_POINT('Ctrl Pts',(13.1012753400396,18.1962394952848,57.0172914311508));
#118557=CARTESIAN_POINT('Ctrl Pts',(12.9720833719076,18.2094692756847,56.9747513346604));
#118558=CARTESIAN_POINT('Ctrl Pts',(12.8415273351186,18.2211892081843,56.9324614523191));
#118559=CARTESIAN_POINT('Ctrl Pts',(12.7096497119619,18.231329974947,56.8904801232899));
#118560=CARTESIAN_POINT('Ctrl Pts',(12.4444257808021,18.2517244434051,56.8060499307075));
#118561=CARTESIAN_POINT('Ctrl Pts',(12.1738535015571,18.2657306505299,56.7228668117145));
#118562=CARTESIAN_POINT('Ctrl Pts',(11.8982362092349,18.2728269465582,56.641337813959));
#118563=CARTESIAN_POINT('Ctrl Pts',(11.816782613109,18.2749241256786,56.6172434256868));
#118564=CARTESIAN_POINT('Ctrl Pts',(11.7348914914288,18.2764174198421,56.5932935716011));
#118565=CARTESIAN_POINT('Ctrl Pts',(11.6525706270574,18.2772939817353,56.5694993585778));
#118566=CARTESIAN_POINT('Ctrl Pts',(11.5263631906892,18.2786378528207,56.5330200692871));
#118567=CARTESIAN_POINT('Ctrl Pts',(11.3991455032489,18.2785321023952,56.4969065926259));
#118568=CARTESIAN_POINT('Ctrl Pts',(11.2709602716692,18.276929295604,56.4611958066604));
#118569=CARTESIAN_POINT('Ctrl Pts',(11.1650621990578,18.2756051637375,56.4316939415971));
#118570=CARTESIAN_POINT('Ctrl Pts',(11.0585025136665,18.2732596241015,56.4024671445837));
#118571=CARTESIAN_POINT('Ctrl Pts',(10.9513041961047,18.2698666163817,56.3735365751458));
#118572=CARTESIAN_POINT('Ctrl Pts',(10.8977050373239,18.2681701125217,56.3590712904268));
#118573=CARTESIAN_POINT('Ctrl Pts',(10.8439462208197,18.2662117444404,56.344680060825));
#118574=CARTESIAN_POINT('Ctrl Pts',(10.7900307491872,18.2639882578872,56.3303655288327));
#118575=CARTESIAN_POINT('Ctrl Pts',(10.7630730133709,18.2628765146106,56.3232082628366));
#118576=CARTESIAN_POINT('Ctrl Pts',(10.736076113812,18.2616984918937,56.316070171194));
#118577=CARTESIAN_POINT('Ctrl Pts',(10.7090404294249,18.2604537834562,56.3089515838742));
#118578=CARTESIAN_POINT('Ctrl Pts',(10.6853842055862,18.2593646635733,56.3027228199694));
#118579=CARTESIAN_POINT('Ctrl Pts',(10.6616982871151,18.258224487445,56.2965089890576));
#118580=CARTESIAN_POINT('Ctrl Pts',(10.6379829303447,18.2570329830165,56.2903103121946));
#118581=CARTESIAN_POINT('Ctrl Pts',(10.6345950222346,18.2568627680981,56.2894247869284));
#118582=CARTESIAN_POINT('Ctrl Pts',(10.6299498050268,18.2566276114753,56.288211440762));
#118583=CARTESIAN_POINT('Ctrl Pts',(10.6278174044834,18.2565191949143,56.2876546648398));
#118584=CARTESIAN_POINT('Ctrl Pts',(10.624434478532,18.2563471985231,56.2867713731327));
#118585=CARTESIAN_POINT('Ctrl Pts',(10.6210431006008,18.2561738055463,56.2858864140547));
#118586=CARTESIAN_POINT('Ctrl Pts',(10.6176432727053,18.2559990005717,56.2849997937491));
#118587=CARTESIAN_POINT('Ctrl Pts',(10.5197768751936,18.2509671184732,56.259477815007));
#118588=CARTESIAN_POINT('Ctrl Pts',(10.4149081209611,18.2447691498421,56.2325775734398));
#118589=CARTESIAN_POINT('Ctrl Pts',(10.3030846392931,18.2370134649294,56.204453451112));
#118590=CARTESIAN_POINT('Ctrl Pts',(10.1918637896328,18.2292995764615,56.1764808935188));
#118591=CARTESIAN_POINT('Ctrl Pts',(10.0737626481988,18.2200446326264,56.1472975810232));
#118592=CARTESIAN_POINT('Ctrl Pts',(9.9488378237052,18.2088174848259,56.1170763702377));
#118593=CARTESIAN_POINT('Ctrl Pts',(9.83465594272455,18.198555818587,56.0894540405128));
#118594=CARTESIAN_POINT('Ctrl Pts',(9.71477342786885,18.1866460127634,56.0609648476129));
#118595=CARTESIAN_POINT('Ctrl Pts',(9.58924430789209,18.1727259445411,56.0317566527638));
#118596=CARTESIAN_POINT('Ctrl Pts',(9.45494599459543,18.1578334504045,56.0005080364794));
#118597=CARTESIAN_POINT('Ctrl Pts',(9.31418394076855,18.1406405777714,55.9684363423956));
#118598=CARTESIAN_POINT('Ctrl Pts',(9.1670458181545,18.120660125274,55.9357383746402));
#118599=CARTESIAN_POINT('Ctrl Pts',(9.02222235037387,18.1009939886732,55.9035547841771));
#118600=CARTESIAN_POINT('Ctrl Pts',(8.87122151575632,18.078627145095,55.8707644658192));
#118601=CARTESIAN_POINT('Ctrl Pts',(8.71415143451219,18.0530552455148,55.8375736497027));
#118602=CARTESIAN_POINT('Ctrl Pts',(8.63126405316597,18.0395607099836,55.8200585391809));
#118603=CARTESIAN_POINT('Ctrl Pts',(8.54668696617735,18.0251729808728,55.8024322121376));
#118604=CARTESIAN_POINT('Ctrl Pts',(8.46043936686297,18.0098135712464,55.7847271238998));
#118605=CARTESIAN_POINT('Ctrl Pts',(8.42076900727369,18.002748872544,55.7765835092075));
#118606=CARTESIAN_POINT('Ctrl Pts',(8.38074526108865,17.9954785609053,55.7684232534171));
#118607=CARTESIAN_POINT('Ctrl Pts',(8.3403705785985,17.987994825621,55.7602495303123));
#118608=CARTESIAN_POINT('Ctrl Pts',(8.1788518450135,17.9580561766696,55.7275505882243));
#118609=CARTESIAN_POINT('Ctrl Pts',(8.01173044245365,17.9247086739793,55.6946404784799));
#118610=CARTESIAN_POINT('Ctrl Pts',(7.83920340169692,17.8874645237823,55.6617567079231));
#118611=CARTESIAN_POINT('Ctrl Pts',(7.67027183132816,17.850996543156,55.629558236452));
#118612=CARTESIAN_POINT('Ctrl Pts',(7.49615737387537,17.8107924659674,55.5973851070223));
#118613=CARTESIAN_POINT('Ctrl Pts',(7.31708859833298,17.7663712540038,55.565469020871));
#118614=CARTESIAN_POINT('Ctrl Pts',(7.26721682661411,17.753999669199,55.5565801916607));
#118615=CARTESIAN_POINT('Ctrl Pts',(7.21696104451305,17.7413008471286,55.5477113488666));
#118616=CARTESIAN_POINT('Ctrl Pts',(7.1663268426109,17.7282640937974,55.5388676077781));
#118617=CARTESIAN_POINT('Ctrl Pts',(7.02456228981143,17.6917640713517,55.514107091104));
#118618=CARTESIAN_POINT('Ctrl Pts',(6.87983029660342,17.6526158128162,55.4895432732945));
#118619=CARTESIAN_POINT('Ctrl Pts',(6.73225177878659,17.6105711023872,55.4652840000943));
#118620=CARTESIAN_POINT('Ctrl Pts',(6.53967588068064,17.5557067631104,55.4336279610377));
#118621=CARTESIAN_POINT('Ctrl Pts',(6.34235173618997,17.4959262820899,55.4024975297025));
#118622=CARTESIAN_POINT('Ctrl Pts',(6.14052458838782,17.430705751096,55.3721629295414));
#118623=CARTESIAN_POINT('Ctrl Pts',(6.0112340933984,17.388925471151,55.3527305810549));
#118624=CARTESIAN_POINT('Ctrl Pts',(5.88009655935121,17.344912249901,55.3336246860117));
#118625=CARTESIAN_POINT('Ctrl Pts',(5.74718567469591,17.2985221805562,55.3149141909974));
#118626=CARTESIAN_POINT('Ctrl Pts',(5.57957686810175,17.2400214476715,55.2913191051001));
#118627=CARTESIAN_POINT('Ctrl Pts',(5.40914470359067,17.1777406306088,55.2683529979293));
#118628=CARTESIAN_POINT('Ctrl Pts',(5.23620340618366,17.1114219519761,55.2461528140407));
#118629=CARTESIAN_POINT('Ctrl Pts',(5.11243895042099,17.0639613668473,55.2302653787202));
#118630=CARTESIAN_POINT('Ctrl Pts',(4.98739047852652,17.0144327233601,55.2147701156798));
#118631=CARTESIAN_POINT('Ctrl Pts',(4.86118934214646,16.9627394489676,55.199715256373));
#118632=CARTESIAN_POINT('Ctrl Pts',(29.5338632414891,-0.462029067073086,
63.010868215388));
#118633=CARTESIAN_POINT('Ctrl Pts',(29.5346219246491,-0.433752793220286,
63.011230106753));
#118634=CARTESIAN_POINT('Ctrl Pts',(29.5608039722791,0.641998223276014,
63.023714156154));
#118635=CARTESIAN_POINT('Ctrl Pts',(29.4078372281691,2.83176758612401,62.95026782851));
#118636=CARTESIAN_POINT('Ctrl Pts',(28.5737667388991,6.01426195252202,62.55847749973));
#118637=CARTESIAN_POINT('Ctrl Pts',(27.1713456340891,8.95881369369201,61.93185808602));
#118638=CARTESIAN_POINT('Ctrl Pts',(25.3938118350091,11.44424088043,61.19592371053));
#118639=CARTESIAN_POINT('Ctrl Pts',(23.4862351945491,13.39803722808,60.47438298443));
#118640=CARTESIAN_POINT('Ctrl Pts',(21.5959186421791,14.88576337841,59.82526804813));
#118641=CARTESIAN_POINT('Ctrl Pts',(19.7728932383691,16.01167021338,59.25919610008));
#118642=CARTESIAN_POINT('Ctrl Pts',(17.9890179586191,16.88023517151,58.75958030935));
#118643=CARTESIAN_POINT('Ctrl Pts',(16.1694318501091,17.56205741783,58.30367386163));
#118644=CARTESIAN_POINT('Ctrl Pts',(14.2545233152291,18.07545203247,57.8825033362001));
#118645=CARTESIAN_POINT('Ctrl Pts',(12.2750306503891,18.39974030706,57.50985034058));
#118646=CARTESIAN_POINT('Ctrl Pts',(10.2979506383991,18.52298246441,57.20011317475));
#118647=CARTESIAN_POINT('Ctrl Pts',(8.29553577903909,18.45025449476,56.94745644735));
#118648=CARTESIAN_POINT('Ctrl Pts',(6.18046749893909,18.15452185092,56.74590079812));
#118649=CARTESIAN_POINT('Ctrl Pts',(3.8630583959391,17.55006605826,56.60308243839));
#118650=CARTESIAN_POINT('Ctrl Pts',(1.35289501732909,16.52026706539,56.54071687939));
#118651=CARTESIAN_POINT('Ctrl Pts',(-1.22835397511091,14.96025853102,56.57780430316));
#118652=CARTESIAN_POINT('Ctrl Pts',(-2.82698452737391,13.56768331313,56.66360640014));
#118653=CARTESIAN_POINT('Ctrl Pts',(-3.58348738863291,12.77819820572,56.71617340988));
#118654=CARTESIAN_POINT('Ctrl Pts',(30.0860529662091,-0.465286448929386,
62.05420413572));
#118655=CARTESIAN_POINT('Ctrl Pts',(30.0868281149291,-0.436810905979286,
62.05457485453));
#118656=CARTESIAN_POINT('Ctrl Pts',(30.1135782153191,0.646521910559514,
62.06736342767));
#118657=CARTESIAN_POINT('Ctrl Pts',(29.9572832439191,2.85177150159601,61.99211983581));
#118658=CARTESIAN_POINT('Ctrl Pts',(29.1052651413891,6.05572682568202,61.59085102028));
#118659=CARTESIAN_POINT('Ctrl Pts',(27.6732347629591,9.01845477515302,60.9493802108601));
#118660=CARTESIAN_POINT('Ctrl Pts',(25.8588487868591,11.51786388819,60.196375469));
#118661=CARTESIAN_POINT('Ctrl Pts',(23.9121691835891,13.48193550668,59.45836886149));
#118662=CARTESIAN_POINT('Ctrl Pts',(21.9833029704391,14.97718508481,58.7946079262));
#118663=CARTESIAN_POINT('Ctrl Pts',(20.1231372976191,16.10868985698,58.2158677272001));
#118664=CARTESIAN_POINT('Ctrl Pts',(18.3028628908391,16.98156509667,57.70514405855));
#118665=CARTESIAN_POINT('Ctrl Pts',(16.4460310900391,17.66679861647,57.23916702843));
#118666=CARTESIAN_POINT('Ctrl Pts',(14.4917463634591,18.18280526933,56.80876811987));
#118667=CARTESIAN_POINT('Ctrl Pts',(12.4713202820591,18.50878353077,56.42804576509));
#118668=CARTESIAN_POINT('Ctrl Pts',(10.4531101100391,18.6326885709,56.11172577456));
#118669=CARTESIAN_POINT('Ctrl Pts',(8.40879716453909,18.55957000061,55.85386194703));
#118670=CARTESIAN_POINT('Ctrl Pts',(6.24923249066909,18.26219087574,55.6483878136801));
#118671=CARTESIAN_POINT('Ctrl Pts',(3.88282255928909,17.6542832528,55.50319038629));
#118672=CARTESIAN_POINT('Ctrl Pts',(1.31936572697909,16.61847639235,55.44054243506));
#118673=CARTESIAN_POINT('Ctrl Pts',(-1.31681310253091,15.04922855625,55.47988027154));
#118674=CARTESIAN_POINT('Ctrl Pts',(-2.94946644714391,13.64834848308,55.5686612246301));
#118675=CARTESIAN_POINT('Ctrl Pts',(-3.72205763400691,12.85415388889,55.6229400250801));
#118676=CARTESIAN_POINT('Ctrl Pts',(29.6438402590691,-0.440906405366586,
61.0422837596));
#118677=CARTESIAN_POINT('Ctrl Pts',(29.6445863481391,-0.413922302316986,
61.04263099393));
#118678=CARTESIAN_POINT('Ctrl Pts',(29.6703352983091,0.612664138304914,
61.0546093697601));
#118679=CARTESIAN_POINT('Ctrl Pts',(29.5199825989191,2.70205115803401,60.98418855492));
#118680=CARTESIAN_POINT('Ctrl Pts',(28.6983885856991,5.74538083047302,60.60757066705));
#118681=CARTESIAN_POINT('Ctrl Pts',(27.3118968411491,8.57206800556001,60.00247848032));
#118682=CARTESIAN_POINT('Ctrl Pts',(25.5485386075391,10.96682866558,59.28852217894));
#118683=CARTESIAN_POINT('Ctrl Pts',(23.6522177073491,12.85399448613,58.58612492656));
#118684=CARTESIAN_POINT('Ctrl Pts',(21.7712823376891,14.29293457848,57.95274708762));
#118685=CARTESIAN_POINT('Ctrl Pts',(19.9569744205691,15.3825412991,57.399474373));
#118686=CARTESIAN_POINT('Ctrl Pts',(18.1821311163691,16.22315601275,56.9105053048901));
#118687=CARTESIAN_POINT('Ctrl Pts',(16.3728054944391,16.88285767912,56.46373198555));
#118688=CARTESIAN_POINT('Ctrl Pts',(14.4702883739891,17.37931439633,56.0503330424501));
#118689=CARTESIAN_POINT('Ctrl Pts',(12.5056416128591,17.69264386349,55.6837038022));
#118690=CARTESIAN_POINT('Ctrl Pts',(10.5455810396291,17.81158752306,55.37787002278));
#118691=CARTESIAN_POINT('Ctrl Pts',(8.56254414565909,17.74139242357,55.12695247192));
#118692=CARTESIAN_POINT('Ctrl Pts',(6.4700871073191,17.45633647142,54.9246919594001));
#118693=CARTESIAN_POINT('Ctrl Pts',(4.17965284087909,16.87426425135,54.77784196221));
#118694=CARTESIAN_POINT('Ctrl Pts',(1.70063539712909,15.88342358762,54.70699356138));
#118695=CARTESIAN_POINT('Ctrl Pts',(-0.847455673380912,14.38332778486,54.73062029495));
#118696=CARTESIAN_POINT('Ctrl Pts',(-2.42552047959091,13.04460583201,54.80507482908));
#118697=CARTESIAN_POINT('Ctrl Pts',(-3.17239712901691,12.28565963609,54.85169577897));
#118698=CARTESIAN_POINT('Ctrl Pts',(28.5669936237991,-0.408723671234686,
60.79836945316));
#118699=CARTESIAN_POINT('Ctrl Pts',(28.5676887698891,-0.383708334716086,
60.79867999721));
#118700=CARTESIAN_POINT('Ctrl Pts',(28.5916818669991,0.567970383760914,
60.80939260235));
#118701=CARTESIAN_POINT('Ctrl Pts',(28.4517075181491,2.50441369284601,60.74649096621));
#118702=CARTESIAN_POINT('Ctrl Pts',(27.6841573416491,5.33571041184002,60.40859830391));
#118703=CARTESIAN_POINT('Ctrl Pts',(26.3813035283791,7.98281775714401,59.8615184069));
#118704=CARTESIAN_POINT('Ctrl Pts',(24.7153386034591,10.23943783787,59.21096093285));
#118705=CARTESIAN_POINT('Ctrl Pts',(22.9178680255491,12.02508460897,58.5672777695));
#118706=CARTESIAN_POINT('Ctrl Pts',(21.1323491770191,13.38969369344,57.98459351753));
#118707=CARTESIAN_POINT('Ctrl Pts',(19.4095888040891,14.4239931358,57.47420458465));
#118708=CARTESIAN_POINT('Ctrl Pts',(17.7250457055691,15.22202253043,57.02215382759));
#118709=CARTESIAN_POINT('Ctrl Pts',(16.0093287990591,15.84802102278,56.60823505731));
#118710=CARTESIAN_POINT('Ctrl Pts',(14.2076068025491,16.3186709616,56.22423386201));
#118711=CARTESIAN_POINT('Ctrl Pts',(12.3500720308091,16.61530346173,55.88239455409));
#118712=CARTESIAN_POINT('Ctrl Pts',(10.5001323733591,16.72769787988,55.59558481383));
#118713=CARTESIAN_POINT('Ctrl Pts',(8.63169365612909,16.66136189094,55.35811567321));
#118714=CARTESIAN_POINT('Ctrl Pts',(6.66335190121909,16.39257307097,55.16358639907));
#118715=CARTESIAN_POINT('Ctrl Pts',(4.51205869883909,15.8446047236,55.01715480186));
#118716=CARTESIAN_POINT('Ctrl Pts',(2.18651660771909,14.91312142525,54.93685948768));
#118717=CARTESIAN_POINT('Ctrl Pts',(-0.202134170110909,13.50430936028,54.93959559631));
#118718=CARTESIAN_POINT('Ctrl Pts',(-1.68141039720091,12.24763887117,54.99407390047));
#118719=CARTESIAN_POINT('Ctrl Pts',(-2.38169007766091,11.53522211755,55.02989751292));
#118720=CARTESIAN_POINT('',(-2.29964905112222,12.0405998988806,54.9957533296306));
#118721=CARTESIAN_POINT('Ctrl Pts',(4.86118859572189,16.9627436220233,55.1997071844704));
#118722=CARTESIAN_POINT('Ctrl Pts',(4.68019380908066,16.8884238711505,55.1780230937973));
#118723=CARTESIAN_POINT('Ctrl Pts',(4.49747300369887,16.8105144441383,55.1576454460921));
#118724=CARTESIAN_POINT('Ctrl Pts',(4.31324259250774,16.728823982826,55.1386016985526));
#118725=CARTESIAN_POINT('Ctrl Pts',(4.08125567542773,16.6259575876845,55.1146213998996));
#118726=CARTESIAN_POINT('Ctrl Pts',(3.8468734963356,16.5170959661948,55.0927569037346));
#118727=CARTESIAN_POINT('Ctrl Pts',(3.61057048418905,16.4018815131822,55.0730204256337));
#118728=CARTESIAN_POINT('Ctrl Pts',(3.37819526251966,16.2885821361869,55.0536120040821));
#118729=CARTESIAN_POINT('Ctrl Pts',(3.14396235812309,16.1691393004344,55.036261253206));
#118730=CARTESIAN_POINT('Ctrl Pts',(2.90836790423341,16.0431949807409,55.0209649897225));
#118731=CARTESIAN_POINT('Ctrl Pts',(2.87714666293793,16.0265046982236,55.0189379117279));
#118732=CARTESIAN_POINT('Ctrl Pts',(2.8459015783102,16.0097002122994,55.016946895061));
#118733=CARTESIAN_POINT('Ctrl Pts',(2.81463386825826,15.9927806666211,55.0149919150382));
#118734=CARTESIAN_POINT('Ctrl Pts',(2.58345076949164,15.8676831461077,55.0005374398324));
#118735=CARTESIAN_POINT('Ctrl Pts',(2.35102690793354,15.7362970187507,54.9880538400737));
#118736=CARTESIAN_POINT('Ctrl Pts',(2.11788131495968,15.5982672566783,54.9775249063338));
#118737=CARTESIAN_POINT('Ctrl Pts',(2.07828347526746,15.5748240497037,54.9757366545163));
#118738=CARTESIAN_POINT('Ctrl Pts',(2.03866493000065,15.5511891631188,54.974004762886));
#118739=CARTESIAN_POINT('Ctrl Pts',(1.99902836376755,15.5273608138029,54.9723291226172));
#118740=CARTESIAN_POINT('Ctrl Pts',(1.76453865798392,15.3863924315389,54.9624160440894));
#118741=CARTESIAN_POINT('Ctrl Pts',(1.52941429199146,15.2386535900276,54.9544729303309));
#118742=CARTESIAN_POINT('Ctrl Pts',(1.29420737288338,15.083814302669,54.9484358207017));
#118743=CARTESIAN_POINT('Ctrl Pts',(1.27342059356983,15.0701301384973,54.9479022816969));
#118744=CARTESIAN_POINT('Ctrl Pts',(1.25263320162065,15.056390512645,54.9473836198031));
#118745=CARTESIAN_POINT('Ctrl Pts',(1.23184559706263,15.0425951949651,54.9468797853324));
#118746=CARTESIAN_POINT('Ctrl Pts',(1.14353560697248,14.9839898677281,54.9447393935912));
#118747=CARTESIAN_POINT('Ctrl Pts',(1.05522169704458,14.9243794649775,54.9428666185128));
#118748=CARTESIAN_POINT('Ctrl Pts',(0.966935191652489,14.8637462740514,
54.9412574715373));
#118749=CARTESIAN_POINT('Ctrl Pts',(0.922791938956445,14.8334296785884,
54.9404528980496));
#118750=CARTESIAN_POINT('Ctrl Pts',(0.87865553714637,14.8028573865017,54.9397142291387));
#118751=CARTESIAN_POINT('Ctrl Pts',(0.834530021960648,14.7720271720485,
54.9390409369179));
#118752=CARTESIAN_POINT('Ctrl Pts',(0.812467264367783,14.7566120648218,
54.9387042908075));
#118753=CARTESIAN_POINT('Ctrl Pts',(0.790407228415868,14.7411324770304,
54.9383839887219));
#118754=CARTESIAN_POINT('Ctrl Pts',(0.768350422076952,14.7255881303148,
54.9380799633647));
#118755=CARTESIAN_POINT('Ctrl Pts',(0.75180781732276,14.7139298702781,54.9378519443468));
#118756=CARTESIAN_POINT('Ctrl Pts',(0.735267029224624,14.7022351833486,
54.9376330809763));
#118757=CARTESIAN_POINT('Ctrl Pts',(0.718728273521809,14.6905039519781,
54.9374233444669));
#118758=CARTESIAN_POINT('Ctrl Pts',(0.713215354954205,14.6865935415213,
54.9373534322972));
#118759=CARTESIAN_POINT('Ctrl Pts',(0.706358237698069,14.6817233852973,
54.9372679778407));
#118760=CARTESIAN_POINT('Ctrl Pts',(0.702190203405758,14.6787605347623,
54.9372166491539));
#118761=CARTESIAN_POINT('Ctrl Pts',(0.414311150449465,14.4741214780138,
54.9336714638866));
#118762=CARTESIAN_POINT('Ctrl Pts',(0.130361881835239,14.2607100262735,
54.9329242570408));
#118763=CARTESIAN_POINT('Ctrl Pts',(-0.148954082189152,14.0384416901636,
54.9346480764321));
#118764=CARTESIAN_POINT('Ctrl Pts',(-0.223061625545815,13.9794699073921,
54.9351054366862));
#118765=CARTESIAN_POINT('Ctrl Pts',(-0.296842775194991,13.9198745072161,
54.9357367725867));
#118766=CARTESIAN_POINT('Ctrl Pts',(-0.370283853487526,13.8596536078829,
54.9365360485735));
#118767=CARTESIAN_POINT('Ctrl Pts',(-0.640247022236335,13.6382866946122,
54.9394741192435));
#118768=CARTESIAN_POINT('Ctrl Pts',(-0.905618976193242,13.4084677122387,
54.9446812477808));
#118769=CARTESIAN_POINT('Ctrl Pts',(-1.16567793374027,13.1703272706806,
54.9518066483159));
#118770=CARTESIAN_POINT('Ctrl Pts',(-1.41754491008076,12.9396883666207,
54.9587075953355));
#118771=CARTESIAN_POINT('Ctrl Pts',(-1.66442842803035,12.7012435830281,
54.9674079551425));
#118772=CARTESIAN_POINT('Ctrl Pts',(-1.90562432250537,12.4551152970694,
54.9775911038724));
#118773=CARTESIAN_POINT('Ctrl Pts',(-2.03874091225642,12.3192765086878,
54.9832112079575));
#118774=CARTESIAN_POINT('Ctrl Pts',(-2.17012420063582,12.1810974577443,
54.9892829940561));
#118775=CARTESIAN_POINT('Ctrl Pts',(-2.29964905112222,12.0405998988806,
54.9957533296306));
#118776=CARTESIAN_POINT('Ctrl Pts',(18.8783242222685,15.00000216221,57.3029867131023));
#118777=CARTESIAN_POINT('Ctrl Pts',(18.6127767826748,15.1297977097545,57.2303573983608));
#118778=CARTESIAN_POINT('Ctrl Pts',(18.3456529579163,15.2531803415356,57.1590406458946));
#118779=CARTESIAN_POINT('Ctrl Pts',(18.0769627299134,15.3701589810481,57.0890865260526));
#118780=CARTESIAN_POINT('Ctrl Pts',(17.9957291190046,15.4055253483233,57.0679371683146));
#118781=CARTESIAN_POINT('Ctrl Pts',(17.9143522632205,15.4403060098944,57.0469124191582));
#118782=CARTESIAN_POINT('Ctrl Pts',(17.832832288681,15.4745003070782,57.0260138163773));
#118783=CARTESIAN_POINT('Ctrl Pts',(17.8156701817998,15.4816991094124,57.0216141087397));
#118784=CARTESIAN_POINT('Ctrl Pts',(17.7985017315288,15.488871921816,57.0172199923451));
#118785=CARTESIAN_POINT('Ctrl Pts',(17.7813269427055,15.496018733811,57.0128314769495));
#118786=CARTESIAN_POINT('Ctrl Pts',(17.597031111528,15.5727083321772,56.9657400628558));
#118787=CARTESIAN_POINT('Ctrl Pts',(17.4120056425813,15.6464079374915,56.9192934226056));
#118788=CARTESIAN_POINT('Ctrl Pts',(17.2262544323235,15.7171175514224,56.8735045150547));
#118789=CARTESIAN_POINT('Ctrl Pts',(17.1333788271946,15.7524723583878,56.8506100612793));
#118790=CARTESIAN_POINT('Ctrl Pts',(17.0403217757781,15.7870796675443,56.8278800786812));
#118791=CARTESIAN_POINT('Ctrl Pts',(16.9470837154508,15.8209394790412,56.8053164191352));
#118792=CARTESIAN_POINT('Ctrl Pts',(16.9004646852872,15.8378693847897,56.7940345893622));
#118793=CARTESIAN_POINT('Ctrl Pts',(16.8538004022893,15.8546124161202,56.7827943427494));
#118794=CARTESIAN_POINT('Ctrl Pts',(16.807090919087,15.8711685730292,56.7715959255905));
#118795=CARTESIAN_POINT('Ctrl Pts',(16.7691902434841,15.8846024517454,56.7625093858366));
#118796=CARTESIAN_POINT('Ctrl Pts',(16.7320664876038,15.8976320223834,56.7536425910697));
#118797=CARTESIAN_POINT('Ctrl Pts',(16.6937562393354,15.9109424860321,56.7445276971792));
#118798=CARTESIAN_POINT('Ctrl Pts',(16.6848522395858,15.9140360803144,56.7424092297563));
#118799=CARTESIAN_POINT('Ctrl Pts',(16.6758840662253,15.917144647716,56.7402774022098));
#118800=CARTESIAN_POINT('Ctrl Pts',(16.6668269197058,15.9202764204705,56.7381264185738));
#118801=CARTESIAN_POINT('Ctrl Pts',(16.4836225612769,15.9836246744713,56.6946171768736));
#118802=CARTESIAN_POINT('Ctrl Pts',(16.2992644068695,16.0442560768477,56.6516427589442));
#118803=CARTESIAN_POINT('Ctrl Pts',(16.11368872958,16.1022137938751,56.6092177628598));
#118804=CARTESIAN_POINT('Ctrl Pts',(15.8774529239984,16.1759933331533,56.5552112072963));
#118805=CARTESIAN_POINT('Ctrl Pts',(15.6392447884627,16.2454417113728,56.5020946551783));
#118806=CARTESIAN_POINT('Ctrl Pts',(15.3989232603713,16.3106085166983,56.4498915487045));
#118807=CARTESIAN_POINT('Ctrl Pts',(15.1618975210043,16.3748816192254,56.3984043598226));
#118808=CARTESIAN_POINT('Ctrl Pts',(14.9228156990975,16.4349899187113,56.3478055828261));
#118809=CARTESIAN_POINT('Ctrl Pts',(14.6815204260846,16.4909365220136,56.2981269141177));
#118810=CARTESIAN_POINT('Ctrl Pts',(14.5535595378906,16.5206054706034,56.271781903323));
#118811=CARTESIAN_POINT('Ctrl Pts',(14.4249758180904,16.5491032729303,56.2456958206221));
#118812=CARTESIAN_POINT('Ctrl Pts',(14.2957435954912,16.576424990075,56.2198747060703));
#118813=CARTESIAN_POINT('Ctrl Pts',(14.2878336666268,16.5780972729989,56.2182942706711));
#118814=CARTESIAN_POINT('Ctrl Pts',(14.279922746965,16.5797646169782,56.216715115788));
#118815=CARTESIAN_POINT('Ctrl Pts',(14.2720108369673,16.5814270232247,56.215137242614));
#118816=CARTESIAN_POINT('Ctrl Pts',(13.9886158069621,16.6409724007936,56.1586197372808));
#118817=CARTESIAN_POINT('Ctrl Pts',(13.7039524089762,16.6941863964793,56.1037459715631));
#118818=CARTESIAN_POINT('Ctrl Pts',(13.4180554492033,16.741109133657,56.050550191522));
#118819=CARTESIAN_POINT('Ctrl Pts',(13.1340559574864,16.7877204495626,55.9977074662787));
#118820=CARTESIAN_POINT('Ctrl Pts',(12.8488388845799,16.8281239109499,55.9465203811792));
#118821=CARTESIAN_POINT('Ctrl Pts',(12.5624151426491,16.8623139613762,55.8970317856168));
#118822=CARTESIAN_POINT('Ctrl Pts',(12.4972314222718,16.8700948620504,55.8857692738108));
#118823=CARTESIAN_POINT('Ctrl Pts',(12.4319851226791,16.8775537685843,55.8745947731496));
#118824=CARTESIAN_POINT('Ctrl Pts',(12.3666762308545,16.8846902730156,55.8635088691272));
#118825=CARTESIAN_POINT('Ctrl Pts',(12.1858178738426,16.904453224586,55.8328089394323));
#118826=CARTESIAN_POINT('Ctrl Pts',(12.0044796821691,16.9217442788938,55.8027883025021));
#118827=CARTESIAN_POINT('Ctrl Pts',(11.8226672654872,16.9365537724192,55.7734537879868));
#118828=CARTESIAN_POINT('Ctrl Pts',(11.7183577198391,16.9450502853037,55.7566239699977));
#118829=CARTESIAN_POINT('Ctrl Pts',(11.6138924170508,16.9527331913848,55.7400200906268));
#118830=CARTESIAN_POINT('Ctrl Pts',(11.5092722772993,16.9596024906979,55.7236437786283));
#118831=CARTESIAN_POINT('Ctrl Pts',(11.4536892865923,16.9632520384885,55.7149433085297));
#118832=CARTESIAN_POINT('Ctrl Pts',(11.400122252971,16.9665326225997,55.7066281879219));
#118833=CARTESIAN_POINT('Ctrl Pts',(11.3470814439974,16.9695624093708,55.6984575201622));
#118834=CARTESIAN_POINT('Ctrl Pts',(11.3002870915886,16.9722353872653,55.6912490873732));
#118835=CARTESIAN_POINT('Ctrl Pts',(11.2539021857595,16.9747123402,55.6841533134244));
#118836=CARTESIAN_POINT('Ctrl Pts',(11.2069005490931,16.9770423115579,55.6770138507463));
#118837=CARTESIAN_POINT('Ctrl Pts',(11.0063457496235,16.9869842406395,55.6465499433747));
#118838=CARTESIAN_POINT('Ctrl Pts',(10.8051909091927,16.9937263467392,55.6169182014827));
#118839=CARTESIAN_POINT('Ctrl Pts',(10.6034419396794,16.9972686283256,55.58813544389));
#118840=CARTESIAN_POINT('Ctrl Pts',(10.5630955412427,16.9979770250258,55.5823793767896));
#118841=CARTESIAN_POINT('Ctrl Pts',(10.5227253892399,16.9985574497193,55.576657276456));
#118842=CARTESIAN_POINT('Ctrl Pts',(10.4823315117015,16.9990098854209,55.5709692927393));
#118843=CARTESIAN_POINT('Ctrl Pts',(10.320739004239,17.0008198186072,55.5482149644305));
#118844=CARTESIAN_POINT('Ctrl Pts',(10.1587669981462,17.0005819416682,55.5260065254767));
#118845=CARTESIAN_POINT('Ctrl Pts',(9.99641916947968,16.9982960003329,55.5043489511402));
#118846=CARTESIAN_POINT('Ctrl Pts',(9.89495391115787,16.9968673170544,55.4908132519397));
#118847=CARTESIAN_POINT('Ctrl Pts',(9.7933418469281,16.994638677846,55.4774927539923));
#118848=CARTESIAN_POINT('Ctrl Pts',(9.69158385139753,16.9916100826178,55.4643889746107));
#118849=CARTESIAN_POINT('Ctrl Pts',(9.64070485363225,16.9900957850037,55.45783708492));
#118850=CARTESIAN_POINT('Ctrl Pts',(9.58978937249366,16.9883814983837,55.4513393785284));
#118851=CARTESIAN_POINT('Ctrl Pts',(9.5388375149835,16.986467222751,55.4448960676726));
#118852=CARTESIAN_POINT('Ctrl Pts',(9.50095971915006,16.9850441432966,55.4401060869926));
#118853=CARTESIAN_POINT('Ctrl Pts',(9.46399488492687,16.98354948681,55.4354629744234));
#118854=CARTESIAN_POINT('Ctrl Pts',(9.42586210998851,16.9818974962683,55.430706000245));
#118855=CARTESIAN_POINT('Ctrl Pts',(9.41270003863564,16.981327288162,55.4290640627343));
#118856=CARTESIAN_POINT('Ctrl Pts',(9.39939882519323,16.9807379061749,55.427408684632));
#118857=CARTESIAN_POINT('Ctrl Pts',(9.38587291883542,16.9801244288179,55.4257295494624));
#118858=CARTESIAN_POINT('Ctrl Pts',(9.14440294537702,16.9691723818947,55.395752946482));
#118859=CARTESIAN_POINT('Ctrl Pts',(8.90351586532162,16.9536344281327,55.3671722628587));
#118860=CARTESIAN_POINT('Ctrl Pts',(8.66322315413537,16.9335124031959,55.3399705237772));
#118861=CARTESIAN_POINT('Ctrl Pts',(8.48386964246388,16.9184934048395,55.3196672553021));
#118862=CARTESIAN_POINT('Ctrl Pts',(8.30484714506715,16.9009200618216,55.3001323488735));
#118863=CARTESIAN_POINT('Ctrl Pts',(8.12616603302871,16.8807920330551,55.2813536914305));
#118864=CARTESIAN_POINT('Ctrl Pts',(7.91712955232603,16.8572445397087,55.2593848083213));
#118865=CARTESIAN_POINT('Ctrl Pts',(7.70855805259612,16.8302009995561,55.238450604365));
#118866=CARTESIAN_POINT('Ctrl Pts',(7.50046210261416,16.7996614123033,55.2185354391638));
#118867=CARTESIAN_POINT('Ctrl Pts',(7.39641412762318,16.7843916186769,55.2085778565632));
#118868=CARTESIAN_POINT('Ctrl Pts',(7.29248503207262,16.768247813263,55.1988751062129));
#118869=CARTESIAN_POINT('Ctrl Pts',(7.18867608397116,16.7512299960567,55.1894256651067));
#118870=CARTESIAN_POINT('Ctrl Pts',(7.13677160992043,16.7427210874536,55.1847009445537));
#118871=CARTESIAN_POINT('Ctrl Pts',(7.08489717240314,16.7339936759037,55.1800395558109));
#118872=CARTESIAN_POINT('Ctrl Pts',(7.0330529264252,16.7250477614135,55.1754413353781));
#118873=CARTESIAN_POINT('Ctrl Pts',(6.98768921119449,16.7172200862346,55.1714178924994));
#118874=CARTESIAN_POINT('Ctrl Pts',(6.94234861133948,16.7092251197422,55.1674428131252));
#118875=CARTESIAN_POINT('Ctrl Pts',(6.89703122952768,16.7010628619411,55.1635159990321));
#118876=CARTESIAN_POINT('Ctrl Pts',(6.89055731784029,16.6998968251124,55.1629550255902));
#118877=CARTESIAN_POINT('Ctrl Pts',(6.88523427686265,16.6989358196951,55.1624943851822));
#118878=CARTESIAN_POINT('Ctrl Pts',(6.87761091625737,16.6975545091299,55.1618360335067));
#118879=CARTESIAN_POINT('Ctrl Pts',(6.81796790451055,16.6867475269429,55.1566852766753));
#118880=CARTESIAN_POINT('Ctrl Pts',(6.75841106823449,16.675656026884,55.1516220895054));
#118881=CARTESIAN_POINT('Ctrl Pts',(6.69894050187817,16.6642799974611,55.1466458983541));
#118882=CARTESIAN_POINT('Ctrl Pts',(6.4278669534886,16.612426772392,55.1239638578846));
#118883=CARTESIAN_POINT('Ctrl Pts',(6.15858533275166,16.5546660050314,55.1030880538125));
#118884=CARTESIAN_POINT('Ctrl Pts',(5.89111960752089,16.4910081648164,55.0839395476397));
#118885=CARTESIAN_POINT('Ctrl Pts',(5.73725476114619,16.4543877574847,55.0729239980472));
#118886=CARTESIAN_POINT('Ctrl Pts',(5.58399094712087,16.4158148823987,55.0624803584915));
#118887=CARTESIAN_POINT('Ctrl Pts',(5.43133401166316,16.3752841611111,55.0525958371668));
#118888=CARTESIAN_POINT('Ctrl Pts',(5.1932133509905,16.3120626500699,55.0371775481697));
#118889=CARTESIAN_POINT('Ctrl Pts',(4.95656700803464,16.2440862458202,55.0231190695121));
#118890=CARTESIAN_POINT('Ctrl Pts',(4.72141062423708,16.1713549480517,55.0103787866828));
#118891=CARTESIAN_POINT('Ctrl Pts',(4.65556535494333,16.1509897263626,55.0068114272081));
#118892=CARTESIAN_POINT('Ctrl Pts',(4.58983691459802,16.1302518486424,55.003347472626));
#118893=CARTESIAN_POINT('Ctrl Pts',(4.52422559886721,16.1091410100962,54.9999861303057));
#118894=CARTESIAN_POINT('Ctrl Pts',(4.4726764875169,16.0925547710489,54.9973452107078));
#118895=CARTESIAN_POINT('Ctrl Pts',(4.42119967559925,16.0757383052224,54.994767633101));
#118896=CARTESIAN_POINT('Ctrl Pts',(4.36979535037543,16.0586918314921,54.9922527529268));
#118897=CARTESIAN_POINT('Ctrl Pts',(4.31137967123683,16.0393202837569,54.9893948526881));
#118898=CARTESIAN_POINT('Ctrl Pts',(4.25305758892359,16.0196515551977,54.9866179184494));
#118899=CARTESIAN_POINT('Ctrl Pts',(4.19482934568938,15.9996856457891,54.9839210346576));
#118900=CARTESIAN_POINT('Ctrl Pts',(4.14387963285945,15.9822154750566,54.9815612613397));
#118901=CARTESIAN_POINT('Ctrl Pts',(4.09300176550862,15.9645177752357,54.9792627771575));
#118902=CARTESIAN_POINT('Ctrl Pts',(4.04219590177801,15.9465925463056,54.9770249897373));
#118903=CARTESIAN_POINT('Ctrl Pts',(4.03493792124507,15.9440317993156,54.9767053058201));
#118904=CARTESIAN_POINT('Ctrl Pts',(4.02898435525666,15.9419279656044,54.976443828588));
#118905=CARTESIAN_POINT('Ctrl Pts',(4.02042636895411,15.9388963749819,54.976069652515));
#118906=CARTESIAN_POINT('Ctrl Pts',(3.76622253922922,15.8488469265306,54.9649552399189));
#118907=CARTESIAN_POINT('Ctrl Pts',(3.51477256686552,15.7533796106994,54.9553998714821));
#118908=CARTESIAN_POINT('Ctrl Pts',(3.26608481102119,15.6525216252025,54.947305074222));
#118909=CARTESIAN_POINT('Ctrl Pts',(3.01662939797749,15.5513523080985,54.9391852896866));
#118910=CARTESIAN_POINT('Ctrl Pts',(2.76995287456916,15.4447588538453,54.9325352163513));
#118911=CARTESIAN_POINT('Ctrl Pts',(2.52608079000258,15.3327212238872,54.9272690335963));
#118912=CARTESIAN_POINT('Ctrl Pts',(2.48924126768141,15.3157967252223,54.9264735195977));
#118913=CARTESIAN_POINT('Ctrl Pts',(2.45246577929163,15.2987479080524,54.9257096084919));
#118914=CARTESIAN_POINT('Ctrl Pts',(2.41575445572796,15.2815746123853,54.9249770288859));
#118915=CARTESIAN_POINT('Ctrl Pts',(2.33630193044391,15.2444072870004,54.9233915426102));
#118916=CARTESIAN_POINT('Ctrl Pts',(2.25714875042345,15.2066591154509,54.9219527803405));
#118917=CARTESIAN_POINT('Ctrl Pts',(2.17829605290603,15.168329539463,54.9206580947122));
#118918=CARTESIAN_POINT('Ctrl Pts',(1.99811405393256,15.080744715624,54.9176996791868));
#118919=CARTESIAN_POINT('Ctrl Pts',(1.81950057314376,14.9901250853999,54.9154933218064));
#118920=CARTESIAN_POINT('Ctrl Pts',(1.64246035550463,14.8964714583744,54.9139967485022));
#118921=CARTESIAN_POINT('Ctrl Pts',(1.51520136375156,14.8291519176044,54.912920990619));
#118922=CARTESIAN_POINT('Ctrl Pts',(1.3887556138919,14.7602645360824,54.9122120483486));
#118923=CARTESIAN_POINT('Ctrl Pts',(1.26312512636562,14.6898093136131,54.9118552464249));
#118924=CARTESIAN_POINT('Ctrl Pts',(1.20030988260248,14.6545817023784,54.9116768454631));
#118925=CARTESIAN_POINT('Ctrl Pts',(1.13769845398559,14.6189621309022,54.9115864926887));
#118926=CARTESIAN_POINT('Ctrl Pts',(1.07529108426283,14.5829505991502,54.9115824312511));
#118927=CARTESIAN_POINT('Ctrl Pts',(1.04408739940145,14.5649448332741,54.9115804005323));
#118928=CARTESIAN_POINT('Ctrl Pts',(1.0129347292531,14.5468410773292,54.9115999434474));
#118929=CARTESIAN_POINT('Ctrl Pts',(0.981833103304978,14.5286393313122,
54.9116408451671));
#118930=CARTESIAN_POINT('Ctrl Pts',(0.958506883843886,14.5149880217994,
54.9116715214569));
#118931=CARTESIAN_POINT('Ctrl Pts',(0.935209376744892,14.5012815928711,
54.9117142121395));
#118932=CARTESIAN_POINT('Ctrl Pts',(0.911940594245692,14.4875200445262,
54.9117688277537));
#118933=CARTESIAN_POINT('Ctrl Pts',(0.904184333412627,14.4829328617446,
54.9117870329584));
#118934=CARTESIAN_POINT('Ctrl Pts',(0.897758611058758,14.4791273142993,
54.9118029917875));
#118935=CARTESIAN_POINT('Ctrl Pts',(0.888681387048689,14.4737401230426,
54.911827415081));
#118936=CARTESIAN_POINT('Ctrl Pts',(0.665558682792343,14.3413202686666,
54.9124277518466));
#118937=CARTESIAN_POINT('Ctrl Pts',(0.446148520268852,14.2044010760549,
54.9141197456218));
#118938=CARTESIAN_POINT('Ctrl Pts',(0.230394363731208,14.0630045829432,
54.9167998817626));
#118939=CARTESIAN_POINT('Ctrl Pts',(0.0610584854176204,13.9520287401795,
54.9189034018741));
#118940=CARTESIAN_POINT('Ctrl Pts',(-0.106024987154981,13.8382939133016,
54.9216158988433));
#118941=CARTESIAN_POINT('Ctrl Pts',(-0.270873407103883,13.7217912087955,
54.9248921647364));
#118942=CARTESIAN_POINT('Ctrl Pts',(-0.480997690549446,13.5732908633788,
54.9290682619254));
#118943=CARTESIAN_POINT('Ctrl Pts',(-0.687491725483667,13.4202947474371,
54.9341601219953));
#118944=CARTESIAN_POINT('Ctrl Pts',(-0.890361482265292,13.2628389385424,
54.9400609774921));
#118945=CARTESIAN_POINT('Ctrl Pts',(-1.09332741816922,13.105308480958,54.9459646305429));
#118946=CARTESIAN_POINT('Ctrl Pts',(-1.2926659920302,12.943313812555,54.9526782096502));
#118947=CARTESIAN_POINT('Ctrl Pts',(-1.48835062831574,12.7768509970127,
54.9601021061303));
#118948=CARTESIAN_POINT('Ctrl Pts',(-1.68291599205989,12.6113403117047,
54.9674835395757));
#118949=CARTESIAN_POINT('Ctrl Pts',(-1.87386942063507,12.4414121400208,
54.9755673514226));
#118950=CARTESIAN_POINT('Ctrl Pts',(-2.06114762481944,12.2670275136822,
54.9842604084735));
#118951=CARTESIAN_POINT('Ctrl Pts',(-2.14132463669145,12.1923704636686,
54.9879820553219));
#118952=CARTESIAN_POINT('Ctrl Pts',(-2.22082754382691,12.1168962028275,
54.9918154127102));
#118953=CARTESIAN_POINT('Ctrl Pts',(-2.29964905112222,12.0405998988806,
54.9957533296306));
#118954=CARTESIAN_POINT('Origin',(18.4825952511691,16.31176789041,58.74984256216));
#118955=CARTESIAN_POINT('',(18.8783254659891,15.00000123934,57.30298584572));
#118956=CARTESIAN_POINT('Origin',(1.07038457110909,10.,122.41156512159));
#118957=CARTESIAN_POINT('',(-2.29973550275167,9.99999999999999,54.9957487971692));
#118958=CARTESIAN_POINT('Origin',(1.07038457110909,10.,122.41156512159));
#118959=CARTESIAN_POINT('',(-2.22484390946911,8.5000000000004,56.4938787766214));
#118960=CARTESIAN_POINT('Origin',(-2.22484394585091,10.,56.49387804884));
#118961=CARTESIAN_POINT('Origin',(1.07038457110909,8.5,122.41156512159));
#118962=CARTESIAN_POINT('Origin',(16.1036855657591,8.5,84.13007607401));
#118963=CARTESIAN_POINT('',(-5.70733149090974,8.50000000000053,58.926389902638));
#118964=CARTESIAN_POINT('Origin',(-2.02513312664091,8.50000000000101,60.48888938658));
#118965=CARTESIAN_POINT('Origin',(27.4324635166691,8.5,72.98888938658));
#118966=CARTESIAN_POINT('Origin',(-6.80729512863291,10.,84.10819367738));
#118967=CARTESIAN_POINT('Origin',(-6.80729512863291,10.,84.10819367738));
#118968=CARTESIAN_POINT('Origin',(-6.80729512863291,10.,84.10819367738));
#118969=CARTESIAN_POINT('Origin',(-8.75366715310791,111.0724296188,85.97453149762));
#118970=CARTESIAN_POINT('',(-6.54676185926042,20.0375488868139,85.5853826642543));
#118971=CARTESIAN_POINT('',(-6.54675958911291,20.03754888577,85.5853955666));
#118972=CARTESIAN_POINT('Ctrl Pts',(-6.54675958911291,20.03754888577,85.5853955666));
#118973=CARTESIAN_POINT('Ctrl Pts',(-6.40319215776023,20.012661527608,85.5600793384597));
#118974=CARTESIAN_POINT('Ctrl Pts',(-6.25833300218533,20.000145232378,85.5345367609292));
#118975=CARTESIAN_POINT('Ctrl Pts',(-6.11218320925691,20.00000000008,85.50876167007));
#118976=CARTESIAN_POINT('Ctrl Pts',(-6.75849120365391,19.73404260182,85.68410573154));
#118977=CARTESIAN_POINT('Ctrl Pts',(-6.63053349123792,19.71244938409,85.65842703201));
#118978=CARTESIAN_POINT('Ctrl Pts',(-6.35597941290291,19.68586616255,85.6033939864201));
#118979=CARTESIAN_POINT('Ctrl Pts',(-6.08345357859991,19.70033953338,85.5491449197301));
#118980=CARTESIAN_POINT('Ctrl Pts',(-5.94102950564791,19.71905670448,85.5209003835101));
#118981=CARTESIAN_POINT('Ctrl Pts',(-6.62106101297492,20.57404799423,85.3408528354601));
#118982=CARTESIAN_POINT('Ctrl Pts',(-6.52824231671291,20.56394872862,85.3292460691401));
#118983=CARTESIAN_POINT('Ctrl Pts',(-6.33031752895692,20.55653875518,85.3049678702));
#118984=CARTESIAN_POINT('Ctrl Pts',(-6.13666228963791,20.57814865479,85.28260809697));
#118985=CARTESIAN_POINT('Ctrl Pts',(-6.03628168416291,20.5971517614,85.27142548283));
#118986=CARTESIAN_POINT('Ctrl Pts',(-6.36266993702292,21.23542234314,85.92234121122));
#118987=CARTESIAN_POINT('Ctrl Pts',(-6.29925055569891,21.22679739812,85.92211116805));
#118988=CARTESIAN_POINT('Ctrl Pts',(-6.16331617101391,21.21744860275,85.92215843362));
#118989=CARTESIAN_POINT('Ctrl Pts',(-6.02869814368591,21.22697975827,85.92360048863));
#118990=CARTESIAN_POINT('Ctrl Pts',(-5.95843846253591,21.23704574569,85.92475783753));
#118991=CARTESIAN_POINT('Ctrl Pts',(-6.25992640685391,21.01016240069,86.8060857876899));
#118992=CARTESIAN_POINT('Ctrl Pts',(-6.18869458337992,20.99141388005,86.8023584409401));
#118993=CARTESIAN_POINT('Ctrl Pts',(-6.03375079962092,20.9610897075,86.79426130529));
#118994=CARTESIAN_POINT('Ctrl Pts',(-5.87513708666991,20.95225717825,86.7859377939401));
#118995=CARTESIAN_POINT('Ctrl Pts',(-5.79083124578291,20.95373020502,86.7815031789699));
#118996=CARTESIAN_POINT('',(-6.21291509723754,21.0225564527532,86.5058292049926));
#118997=CARTESIAN_POINT('Origin',(-6.37308545636947,20.0375750950329,86.5701674523326));
#118998=CARTESIAN_POINT('Origin',(-5.93751316552096,22.6785117147427,86.5230655023542));
#118999=CARTESIAN_POINT('Origin',(156.848906078169,21.,64.897742657285));
#119000=CARTESIAN_POINT('',(-5.70733054567061,21.0000000000039,87.0513884694204));
#119001=CARTESIAN_POINT('Origin',(27.4324635166691,21.,72.98888938658));
#119002=CARTESIAN_POINT('Origin',(-2.02513312664091,21.00000000001,85.48888938658));
#119003=CARTESIAN_POINT('Ctrl Pts',(-8.35462806748892,22.42643511175,84.29934907621));
#119004=CARTESIAN_POINT('Ctrl Pts',(-8.35090947121791,22.37969257573,84.32927895922));
#119005=CARTESIAN_POINT('Ctrl Pts',(-8.33351057093391,22.20164105692,84.44276426472));
#119006=CARTESIAN_POINT('Ctrl Pts',(-8.28365361158691,21.90483406201,84.6285915005799));
#119007=CARTESIAN_POINT('Ctrl Pts',(-8.18724379590092,21.54970983089,84.84428475201));
#119008=CARTESIAN_POINT('Ctrl Pts',(-8.07006104322492,21.23582300564,85.0284324468699));
#119009=CARTESIAN_POINT('Ctrl Pts',(-7.93917357924691,20.96122182353,85.18316506841));
#119010=CARTESIAN_POINT('Ctrl Pts',(-7.79858230655091,20.72092123751,85.31219748715));
#119011=CARTESIAN_POINT('Ctrl Pts',(-7.6482694193289,20.5075413273,85.4200547810799));
#119012=CARTESIAN_POINT('Ctrl Pts',(-7.4836205707029,20.31265218618,85.51083397843));
#119013=CARTESIAN_POINT('Ctrl Pts',(-7.29258471097291,20.12666462895,85.58725205448));
#119014=CARTESIAN_POINT('Ctrl Pts',(-7.05745176478091,19.9467868938,85.6450057031999));
#119015=CARTESIAN_POINT('Ctrl Pts',(-6.76628674550091,19.79030673,85.6657564249));
#119016=CARTESIAN_POINT('Ctrl Pts',(-6.54310988125591,19.72773437946,85.6357518205));
#119017=CARTESIAN_POINT('Ctrl Pts',(-6.42976359251691,19.71267560486,85.60686271593));
#119018=CARTESIAN_POINT('Ctrl Pts',(-7.94697006594592,23.04092220471,84.80596115758));
#119019=CARTESIAN_POINT('Ctrl Pts',(-7.93335072749191,22.99384694058,84.82825711759));
#119020=CARTESIAN_POINT('Ctrl Pts',(-7.87927599267992,22.8151897012,84.91112157838));
#119021=CARTESIAN_POINT('Ctrl Pts',(-7.77554997450592,22.52107215757,85.0361032601));
#119022=CARTESIAN_POINT('Ctrl Pts',(-7.63029827947891,22.17542681458,85.16338885188));
#119023=CARTESIAN_POINT('Ctrl Pts',(-7.48571075372192,21.87555618959,85.25742491269));
#119024=CARTESIAN_POINT('Ctrl Pts',(-7.34661185907992,21.61836861234,85.32424726386));
#119025=CARTESIAN_POINT('Ctrl Pts',(-7.21476913077092,21.3981324291,85.36956564192));
#119026=CARTESIAN_POINT('Ctrl Pts',(-7.08904716940091,21.20725692061,85.39810235033));
#119027=CARTESIAN_POINT('Ctrl Pts',(-6.96603251958891,21.03773902674,85.4130071847901));
#119028=CARTESIAN_POINT('Ctrl Pts',(-6.83949966896591,20.88136131406,85.41536453852));
#119029=CARTESIAN_POINT('Ctrl Pts',(-6.70427653768091,20.7367020702,85.40328206329));
#119030=CARTESIAN_POINT('Ctrl Pts',(-6.56371790810491,20.6183554452,85.37415966696));
#119031=CARTESIAN_POINT('Ctrl Pts',(-6.47361817696992,20.57431207621,85.34615928593));
#119032=CARTESIAN_POINT('Ctrl Pts',(-6.42908978116191,20.56370269296,85.33103245456));
#119033=CARTESIAN_POINT('Ctrl Pts',(-8.4348349802069,23.50406104764,85.39579476813));
#119034=CARTESIAN_POINT('Ctrl Pts',(-8.40969820765591,23.45673500638,85.42776643184));
#119035=CARTESIAN_POINT('Ctrl Pts',(-8.31090848053591,23.27762123549,85.54572550045));
#119036=CARTESIAN_POINT('Ctrl Pts',(-8.12775601955191,22.98553073094,85.71799464822));
#119037=CARTESIAN_POINT('Ctrl Pts',(-7.8815186557559,22.64702962472,85.88325981061));
#119038=CARTESIAN_POINT('Ctrl Pts',(-7.64457453124492,22.35772300805,85.9958072564301));
#119039=CARTESIAN_POINT('Ctrl Pts',(-7.42361387635791,22.11366006255,86.06659135295));
#119040=CARTESIAN_POINT('Ctrl Pts',(-7.22054442786891,21.90854641711,86.10532035578));
#119041=CARTESIAN_POINT('Ctrl Pts',(-7.03315811824792,21.73463247331,86.11946431853));
#119042=CARTESIAN_POINT('Ctrl Pts',(-6.85657254671691,21.58423688521,86.11359046581));
#119043=CARTESIAN_POINT('Ctrl Pts',(-6.68328271986891,21.45017610857,86.08876818199));
#119044=CARTESIAN_POINT('Ctrl Pts',(-6.51001739351891,21.33206103707,86.0429626720599));
#119045=CARTESIAN_POINT('Ctrl Pts',(-6.34791600768991,21.24245565535,85.97816203645));
#119046=CARTESIAN_POINT('Ctrl Pts',(-6.25807374458691,21.21237757737,85.93509102818));
#119047=CARTESIAN_POINT('Ctrl Pts',(-6.21484666490891,21.20512169981,85.91670410992));
#119048=CARTESIAN_POINT('Ctrl Pts',(-9.31121502261391,23.33454012732,85.4558723699601));
#119049=CARTESIAN_POINT('Ctrl Pts',(-9.28491347993491,23.28730587704,85.5047740045099));
#119050=CARTESIAN_POINT('Ctrl Pts',(-9.17983912464392,23.10835920862,85.68707148129));
#119051=CARTESIAN_POINT('Ctrl Pts',(-8.97424581930491,22.81552675479,85.96561818075));
#119052=CARTESIAN_POINT('Ctrl Pts',(-8.6798271479399,22.4744106712,86.2557803286799));
#119053=CARTESIAN_POINT('Ctrl Pts',(-8.38155509163591,22.1812373514,86.4762244427199));
#119054=CARTESIAN_POINT('Ctrl Pts',(-8.09015620392992,21.93237044768,86.63872510375));
#119055=CARTESIAN_POINT('Ctrl Pts',(-7.80990628928392,21.72172155819,86.75483732633));
#119056=CARTESIAN_POINT('Ctrl Pts',(-7.53868429503691,21.54159923843,86.83447387236));
#119057=CARTESIAN_POINT('Ctrl Pts',(-7.26899562207991,21.38420438667,86.8845110107599));
#119058=CARTESIAN_POINT('Ctrl Pts',(-6.98628046299991,21.24197502821,86.90763628799));
#119059=CARTESIAN_POINT('Ctrl Pts',(-6.67655582865691,21.11414409591,86.89926709383));
#119060=CARTESIAN_POINT('Ctrl Pts',(-6.34315059286091,21.01401866802,86.85006128191));
#119061=CARTESIAN_POINT('Ctrl Pts',(-6.12047856213391,20.97882892856,86.79050676521));
#119062=CARTESIAN_POINT('Ctrl Pts',(-6.00968384453291,20.97034558027,86.75522540636));
#119063=CARTESIAN_POINT('Ctrl Pts',(-8.23395173885521,22.5,84.5714980228307));
#119064=CARTESIAN_POINT('Ctrl Pts',(-8.22142766674582,22.4758562186449,
84.6100482185526));
#119065=CARTESIAN_POINT('Ctrl Pts',(-8.20731320283664,22.4496738732414,
84.6514255097405));
#119066=CARTESIAN_POINT('Ctrl Pts',(-8.1912618489509,22.4215351161334,84.6955546689892));
#119067=CARTESIAN_POINT('Ctrl Pts',(-8.17628816671385,22.3952855666885,
84.7367210411645));
#119068=CARTESIAN_POINT('Ctrl Pts',(-8.15962851767868,22.3673340632109,
84.7802824882887));
#119069=CARTESIAN_POINT('Ctrl Pts',(-8.14097429954895,22.33774180324,84.8261449122856));
#119070=CARTESIAN_POINT('Ctrl Pts',(-8.12603890112914,22.3140489210331,
84.8628644129437));
#119071=CARTESIAN_POINT('Ctrl Pts',(-8.10982451010508,22.2893043566117,
84.9010584792541));
#119072=CARTESIAN_POINT('Ctrl Pts',(-8.09216019510566,22.2635324072133,
84.9406592830494));
#119073=CARTESIAN_POINT('Ctrl Pts',(-8.07270453650607,22.2351469165246,
84.9842760164997));
#119074=CARTESIAN_POINT('Ctrl Pts',(-8.05149008683296,22.2055140674626,
85.0296011650061));
#119075=CARTESIAN_POINT('Ctrl Pts',(-8.02827282937339,22.1746900474528,
85.0764886326811));
#119076=CARTESIAN_POINT('Ctrl Pts',(-8.00665737524525,22.1459926359809,
85.1201412436097));
#119077=CARTESIAN_POINT('Ctrl Pts',(-7.98330611454984,22.116262884349,85.1651482272115));
#119078=CARTESIAN_POINT('Ctrl Pts',(-7.95800680800294,22.0855457664435,
85.2113489761293));
#119079=CARTESIAN_POINT('Ctrl Pts',(-7.94921119087629,22.0748665801256,
85.2274112384562));
#119080=CARTESIAN_POINT('Ctrl Pts',(-7.94017995739716,22.0640680393239,
85.2436173769373));
#119081=CARTESIAN_POINT('Ctrl Pts',(-7.93090361526843,22.053151982212,85.2599592296446));
#119082=CARTESIAN_POINT('Ctrl Pts',(-7.906206213193,22.0240889908057,85.303467899481));
#119083=CARTESIAN_POINT('Ctrl Pts',(-7.8797728759181,21.9941928412466,85.3479419904631));
#119084=CARTESIAN_POINT('Ctrl Pts',(-7.85140570019092,21.9635035437492,
85.3931920714271));
#119085=CARTESIAN_POINT('Ctrl Pts',(-7.82485750363657,21.9347821260828,
85.4355405961829));
#119086=CARTESIAN_POINT('Ctrl Pts',(-7.7966159059768,21.9053659437477,85.4785689025909));
#119087=CARTESIAN_POINT('Ctrl Pts',(-7.76649755550958,21.8752897319992,
85.5220796372438));
#119088=CARTESIAN_POINT('Ctrl Pts',(-7.76443396327619,21.873229026947,85.525060823554));
#119089=CARTESIAN_POINT('Ctrl Pts',(-7.76236155050475,21.8711652245217,
85.5280442567256));
#119090=CARTESIAN_POINT('Ctrl Pts',(-7.76028025348173,21.869098336431,85.5310298651969));
#119091=CARTESIAN_POINT('Ctrl Pts',(-7.73211084979391,21.841123951054,85.571438710909));
#119092=CARTESIAN_POINT('Ctrl Pts',(-7.70231553838991,21.8125833290727,
85.6122494955127));
#119093=CARTESIAN_POINT('Ctrl Pts',(-7.67073246783274,21.7835331002349,
85.6532530028498));
#119094=CARTESIAN_POINT('Ctrl Pts',(-7.65172373904734,21.7660487989498,
85.6779315580527));
#119095=CARTESIAN_POINT('Ctrl Pts',(-7.63206708837751,21.7483801122145,
85.702679152938));
#119096=CARTESIAN_POINT('Ctrl Pts',(-7.61172320807623,21.7305417927462,
85.7274421778844));
#119097=CARTESIAN_POINT('Ctrl Pts',(-7.60387233078295,21.7236578327941,
85.736998440868));
#119098=CARTESIAN_POINT('Ctrl Pts',(-7.59591906966474,21.7167486318406,
85.7465569330663));
#119099=CARTESIAN_POINT('Ctrl Pts',(-7.58786101727019,21.7098151309467,
85.7561143014515));
#119100=CARTESIAN_POINT('Ctrl Pts',(-7.58287821376429,21.7055277087669,
85.7620242268733));
#119101=CARTESIAN_POINT('Ctrl Pts',(-7.57785533858723,21.7012309955984,
85.7679337194716));
#119102=CARTESIAN_POINT('Ctrl Pts',(-7.57279185930897,21.6969253210417,
85.7738419360785));
#119103=CARTESIAN_POINT('Ctrl Pts',(-7.56616586015563,21.6912909746961,
85.7815733468504));
#119104=CARTESIAN_POINT('Ctrl Pts',(-7.55947028595343,21.6856412267916,
85.7893025976754));
#119105=CARTESIAN_POINT('Ctrl Pts',(-7.55270397316235,21.6799769114545,
85.7970277121451));
#119106=CARTESIAN_POINT('Ctrl Pts',(-7.5493208167668,21.677144753786,85.80089026938));
#119107=CARTESIAN_POINT('Ctrl Pts',(-7.54591997503914,21.6743089546902,
85.8047517922779));
#119108=CARTESIAN_POINT('Ctrl Pts',(-7.54250128881515,21.6714696081392,
85.8086120319138));
#119109=CARTESIAN_POINT('Ctrl Pts',(-7.54079194570317,21.6700499348637,
85.8105421517318));
#119110=CARTESIAN_POINT('Ctrl Pts',(-7.53907814141567,21.6686293747617,
85.8124719507154));
#119111=CARTESIAN_POINT('Ctrl Pts',(-7.53735985637281,21.6672079404422,
85.8144013971823));
#119112=CARTESIAN_POINT('Ctrl Pts',(-7.53564157132995,21.6657865061226,
85.8163308436492));
#119113=CARTESIAN_POINT('Ctrl Pts',(-7.53325512565926,21.6638173628125,
85.8190010194744));
#119114=CARTESIAN_POINT('Ctrl Pts',(-7.53219153923514,21.662941027586,85.8201886471735));
#119115=CARTESIAN_POINT('Ctrl Pts',(-7.5082070923888,21.6431791961245,85.8469702915965));
#119116=CARTESIAN_POINT('Ctrl Pts',(-7.48262569868808,21.6226690970833,
85.8745392519396));
#119117=CARTESIAN_POINT('Ctrl Pts',(-7.45529229994458,21.6014761715685,
85.9027111175446));
#119118=CARTESIAN_POINT('Ctrl Pts',(-7.44255729541833,21.5916020975505,
85.9158367752558));
#119119=CARTESIAN_POINT('Ctrl Pts',(-7.42944167748955,21.5815800239868,
85.9290927323526));
#119120=CARTESIAN_POINT('Ctrl Pts',(-7.41592801790452,21.5714178742797,
85.9424570368911));
#119121=CARTESIAN_POINT('Ctrl Pts',(-7.38929896106609,21.5513930645344,
85.968791785293));
#119122=CARTESIAN_POINT('Ctrl Pts',(-7.36112512444487,21.530822813742,85.9955496136367));
#119123=CARTESIAN_POINT('Ctrl Pts',(-7.33127204040911,21.5097958253814,
86.0225360407876));
#119124=CARTESIAN_POINT('Ctrl Pts',(-7.30339328044189,21.4901594501031,
86.047737729297));
#119125=CARTESIAN_POINT('Ctrl Pts',(-7.27405020128941,21.4701247211595,
86.0731388693538));
#119126=CARTESIAN_POINT('Ctrl Pts',(-7.24311923952744,21.4497833014211,
86.0985477000223));
#119127=CARTESIAN_POINT('Ctrl Pts',(-7.21216793008562,21.4294285002463,
86.1239732456819));
#119128=CARTESIAN_POINT('Ctrl Pts',(-7.17962619705669,21.4087658566656,
86.1494066116004));
#119129=CARTESIAN_POINT('Ctrl Pts',(-7.14537550743067,21.3879312712363,
86.174626888892));
#119130=CARTESIAN_POINT('Ctrl Pts',(-7.13907688309786,21.3840998381124,
86.179264840827));
#119131=CARTESIAN_POINT('Ctrl Pts',(-7.13272043120045,21.3802626745631,
86.1838954779573));
#119132=CARTESIAN_POINT('Ctrl Pts',(-7.12630536519258,21.3764207432868,
86.1885172729001));
#119133=CARTESIAN_POINT('Ctrl Pts',(-7.10844112800482,21.3657219957613,
86.2013877314412));
#119134=CARTESIAN_POINT('Ctrl Pts',(-7.0912092503863,21.3556240801419,86.2133797962381));
#119135=CARTESIAN_POINT('Ctrl Pts',(-7.07430698339713,21.3459028412265,
86.2247499007996));
#119136=CARTESIAN_POINT('Ctrl Pts',(-7.07122130368359,21.3441281307849,
86.2268256283342));
#119137=CARTESIAN_POINT('Ctrl Pts',(-7.06814652587917,21.342366022409,86.2288805256242));
#119138=CARTESIAN_POINT('Ctrl Pts',(-7.06508069946555,21.3406152175656,
86.2309160183396));
#119139=CARTESIAN_POINT('Ctrl Pts',(-7.04789054710154,21.3307984184523,
86.2423290682622));
#119140=CARTESIAN_POINT('Ctrl Pts',(-7.03098420424403,21.3213352771548,
86.2531353338268));
#119141=CARTESIAN_POINT('Ctrl Pts',(-7.01400310668316,21.312011519002,86.2635653853502));
#119142=CARTESIAN_POINT('Ctrl Pts',(-6.9970220091223,21.3026877608493,86.2739954368736));
#119143=CARTESIAN_POINT('Ctrl Pts',(-6.97996598709154,21.2935030330653,
86.2840493949244));
#119144=CARTESIAN_POINT('Ctrl Pts',(-6.96244875624373,21.2842670815851,
86.2939168179826));
#119145=CARTESIAN_POINT('Ctrl Pts',(-6.93266456847538,21.26856338301,86.31069419471));
#119146=CARTESIAN_POINT('Ctrl Pts',(-6.90228320749175,21.2531257985842,
86.3265648508905));
#119147=CARTESIAN_POINT('Ctrl Pts',(-6.87132227451052,21.2380561271013,
86.3414757926713));
#119148=CARTESIAN_POINT('Ctrl Pts',(-6.82196897998102,21.2140343078747,
86.365244588717));
#119149=CARTESIAN_POINT('Ctrl Pts',(-6.77114060472277,21.1909468139287,
86.3865756596193));
#119150=CARTESIAN_POINT('Ctrl Pts',(-6.7189898404278,21.169247598944,86.4053578137257));
#119151=CARTESIAN_POINT('Ctrl Pts',(-6.69360340937748,21.1586846545173,
86.4145007642968));
#119152=CARTESIAN_POINT('Ctrl Pts',(-6.66790423558804,21.1484509219892,
86.4230393996217));
#119153=CARTESIAN_POINT('Ctrl Pts',(-6.64191335523892,21.1386003907898,
86.43095830036));
#119154=CARTESIAN_POINT('Ctrl Pts',(-6.59340489783472,21.1202157086753,
86.4457378558807));
#119155=CARTESIAN_POINT('Ctrl Pts',(-6.54387772623071,21.1031655777177,
86.4583594906108));
#119156=CARTESIAN_POINT('Ctrl Pts',(-6.49343465793604,21.0877698814451,
86.4688980397014));
#119157=CARTESIAN_POINT('Ctrl Pts',(-6.45258501756962,21.0753021891103,
86.4774323330125));
#119158=CARTESIAN_POINT('Ctrl Pts',(-6.41113526624891,21.0639193972677,
86.484600503558));
#119159=CARTESIAN_POINT('Ctrl Pts',(-6.36916128441197,21.0537978031306,
86.4904298740942));
#119160=CARTESIAN_POINT('Ctrl Pts',(-6.32275972737502,21.0426085447591,
86.4968741487993));
#119161=CARTESIAN_POINT('Ctrl Pts',(-6.27571569550032,21.0329606922833,
86.5016818168602));
#119162=CARTESIAN_POINT('Ctrl Pts',(-6.22791363557178,21.024996082316,86.5048800287462));
#119163=CARTESIAN_POINT('Ctrl Pts',(-6.22292237448476,21.0241644560668,
86.5052139706424));
#119164=CARTESIAN_POINT('Ctrl Pts',(-6.21792289450644,21.023351190184,86.505530354876));
#119165=CARTESIAN_POINT('Ctrl Pts',(-6.21291509723754,21.0225564527532,
86.5058292049926));
#119166=CARTESIAN_POINT('Ctrl Pts',(-8.23395173885521,22.5,84.5714980228307));
#119167=CARTESIAN_POINT('Ctrl Pts',(-8.21760659462262,22.4147034792435,
84.621797380569));
#119168=CARTESIAN_POINT('Ctrl Pts',(-8.19943848710039,22.3338593791439,
84.6687450527327));
#119169=CARTESIAN_POINT('Ctrl Pts',(-8.18020402924739,22.2574714230342,
84.7124495350668));
#119170=CARTESIAN_POINT('Ctrl Pts',(-8.16709282862747,22.2054014439813,
84.7422407691245));
#119171=CARTESIAN_POINT('Ctrl Pts',(-8.15348570968668,22.155401258526,84.7705256576035));
#119172=CARTESIAN_POINT('Ctrl Pts',(-8.1396129664063,22.1074638808062,84.7973449949855));
#119173=CARTESIAN_POINT('Ctrl Pts',(-8.12311399437653,22.0504515481914,
84.8292414619193));
#119174=CARTESIAN_POINT('Ctrl Pts',(-8.1062398891631,21.9963593206321,84.8590634254539));
#119175=CARTESIAN_POINT('Ctrl Pts',(-8.08935621921663,21.9452011132389,
84.8868623392333));
#119176=CARTESIAN_POINT('Ctrl Pts',(-8.07167595547547,21.8916291942128,
84.9159728423939));
#119177=CARTESIAN_POINT('Ctrl Pts',(-8.05396691424662,21.841263506198,84.9428994902048));
#119178=CARTESIAN_POINT('Ctrl Pts',(-8.03656426649347,21.7941099687286,
84.9677854423284));
#119179=CARTESIAN_POINT('Ctrl Pts',(-8.03184007172358,21.7813094743294,
84.974541085868));
#119180=CARTESIAN_POINT('Ctrl Pts',(-8.02713820360347,21.7687455339146,
84.9811463777592));
#119181=CARTESIAN_POINT('Ctrl Pts',(-8.02246480578853,21.7564179432622,
84.9876042296749));
#119182=CARTESIAN_POINT('Ctrl Pts',(-8.0190828900531,21.7474970521979,84.9922774699757));
#119183=CARTESIAN_POINT('Ctrl Pts',(-8.01571587757638,21.7386999287141,
84.9968734997127));
#119184=CARTESIAN_POINT('Ctrl Pts',(-8.01236595424368,21.7300264779375,
85.001393387132));
#119185=CARTESIAN_POINT('Ctrl Pts',(-7.99985006379615,21.6976209722166,
85.0182804648816));
#119186=CARTESIAN_POINT('Ctrl Pts',(-7.98757294713772,21.6669439334479,
85.034105627324));
#119187=CARTESIAN_POINT('Ctrl Pts',(-7.97563821227694,21.6379953616346,
85.0489286136373));
#119188=CARTESIAN_POINT('Ctrl Pts',(-7.96967084484655,21.623521075728,85.0563401067939));
#119189=CARTESIAN_POINT('Ctrl Pts',(-7.9637888644607,21.6094789065459,85.063501084823));
#119190=CARTESIAN_POINT('Ctrl Pts',(-7.95800396907429,21.5958688540644,
85.0704190837983));
#119191=CARTESIAN_POINT('Ctrl Pts',(-7.95511152138109,21.5890638278237,
85.0738780832859));
#119192=CARTESIAN_POINT('Ctrl Pts',(-7.95224333724095,21.5823668307585,
85.0772763315146));
#119193=CARTESIAN_POINT('Ctrl Pts',(-7.94940079325356,21.5757778628675,
85.0806147757484));
#119194=CARTESIAN_POINT('Ctrl Pts',(-7.94715518130021,21.5705725731264,
85.0832521492807));
#119195=CARTESIAN_POINT('Ctrl Pts',(-7.94539568124722,21.5665142395513,
85.0853058853073));
#119196=CARTESIAN_POINT('Ctrl Pts',(-7.94300939935868,21.5610441974117,
85.0880715302674));
#119197=CARTESIAN_POINT('Ctrl Pts',(-7.94237507422545,21.5595901423709,
85.0888066982776));
#119198=CARTESIAN_POINT('Ctrl Pts',(-7.94169623917092,21.5580363940842,
85.0895920510289));
#119199=CARTESIAN_POINT('Ctrl Pts',(-7.94095142577195,21.5563350467186,
85.0904516160242));
#119200=CARTESIAN_POINT('Ctrl Pts',(-7.92481966153642,21.5194859048771,
85.109068762102));
#119201=CARTESIAN_POINT('Ctrl Pts',(-7.90841653112025,21.4834288245106,
85.1270711143947));
#119202=CARTESIAN_POINT('Ctrl Pts',(-7.89179152635374,21.4481629112508,
85.144469492258));
#119203=CARTESIAN_POINT('Ctrl Pts',(-7.86346596351681,21.3880771033924,
85.1741127225818));
#119204=CARTESIAN_POINT('Ctrl Pts',(-7.83449617097394,21.3302906458657,
85.2020005238258));
#119205=CARTESIAN_POINT('Ctrl Pts',(-7.80511118203973,21.2748094023012,
85.2281791540894));
#119206=CARTESIAN_POINT('Ctrl Pts',(-7.79107260695249,21.2483034333707,
85.2406859026016));
#119207=CARTESIAN_POINT('Ctrl Pts',(-7.77693928027529,21.2223229817798,
85.2528030566652));
#119208=CARTESIAN_POINT('Ctrl Pts',(-7.76273610728766,21.1968654811886,
85.2645382455123));
#119209=CARTESIAN_POINT('Ctrl Pts',(-7.76002406525863,21.1920044679757,
85.2667790353273));
#119210=CARTESIAN_POINT('Ctrl Pts',(-7.75730945440262,21.1871625853629,
85.2690059210676));
#119211=CARTESIAN_POINT('Ctrl Pts',(-7.75459243225009,21.1823398204644,
85.2712189735255));
#119212=CARTESIAN_POINT('Ctrl Pts',(-7.72656223953097,21.1325857066023,
85.2940499566427));
#119213=CARTESIAN_POINT('Ctrl Pts',(-7.69827563591021,21.0848691356955,
85.3154067867001));
#119214=CARTESIAN_POINT('Ctrl Pts',(-7.66989477041555,21.03918914901,85.3353556251637));
#119215=CARTESIAN_POINT('Ctrl Pts',(-7.65432883088826,21.0141352298303,
85.3462968846268));
#119216=CARTESIAN_POINT('Ctrl Pts',(-7.63873440030209,20.9896940454143,
85.3568150785505));
#119217=CARTESIAN_POINT('Ctrl Pts',(-7.62313693229151,20.9658655957017,
85.3669241648387));
#119218=CARTESIAN_POINT('Ctrl Pts',(-7.62011930331171,20.9612555256347,
85.368879961236));
#119219=CARTESIAN_POINT('Ctrl Pts',(-7.61710156474831,20.9566684038422,
85.370820445469));
#119220=CARTESIAN_POINT('Ctrl Pts',(-7.61408388714227,20.9521042062413,
85.3727457322644));
#119221=CARTESIAN_POINT('Ctrl Pts',(-7.60930270507376,20.944872731387,85.3757961398642));
#119222=CARTESIAN_POINT('Ctrl Pts',(-7.60452167614984,20.9376988048727,
85.3788083963661));
#119223=CARTESIAN_POINT('Ctrl Pts',(-7.59974145817027,20.9305824721789,
85.381782858467));
#119224=CARTESIAN_POINT('Ctrl Pts',(-7.59584281462332,20.9247785434349,
85.38420876614));
#119225=CARTESIAN_POINT('Ctrl Pts',(-7.5919447078127,20.919012910613,85.3866095361309));
#119226=CARTESIAN_POINT('Ctrl Pts',(-7.58804748868746,20.9132855737127,
85.3889853720183));
#119227=CARTESIAN_POINT('Ctrl Pts',(-7.58609887912484,20.9104219052625,
85.390173289962));
#119228=CARTESIAN_POINT('Ctrl Pts',(-7.58415049153295,20.9075678107926,
85.3913549744375));
#119229=CARTESIAN_POINT('Ctrl Pts',(-7.5822023694505,20.904723290303,85.3925304516039));
#119230=CARTESIAN_POINT('Ctrl Pts',(-7.58025424736805,20.9018787698134,
85.3937059287704));
#119231=CARTESIAN_POINT('Ctrl Pts',(-7.57893328365522,20.8999532776846,
85.3945008138175));
#119232=CARTESIAN_POINT('Ctrl Pts',(-7.57635884326463,20.8962184507747,
85.396038287666));
#119233=CARTESIAN_POINT('Ctrl Pts',(-7.54126018515817,20.8452996517695,
85.4169994523349));
#119234=CARTESIAN_POINT('Ctrl Pts',(-7.50558531703489,20.7965597621204,
85.436354179377));
#119235=CARTESIAN_POINT('Ctrl Pts',(-7.46947393676564,20.7499909550496,
85.4541206031617));
#119236=CARTESIAN_POINT('Ctrl Pts',(-7.43569965747034,20.7064360456351,
85.4707371975569));
#119237=CARTESIAN_POINT('Ctrl Pts',(-7.40154379163175,20.6647807397546,
85.4859642826928));
#119238=CARTESIAN_POINT('Ctrl Pts',(-7.36712038208436,20.6250355889639,
85.499811424579));
#119239=CARTESIAN_POINT('Ctrl Pts',(-7.35051750899141,20.6058659685424,
85.5064900872233));
#119240=CARTESIAN_POINT('Ctrl Pts',(-7.33385233478653,20.5871400356242,
85.5128482195878));
#119241=CARTESIAN_POINT('Ctrl Pts',(-7.31713719799185,20.5688555431679,
85.5188893576003));
#119242=CARTESIAN_POINT('Ctrl Pts',(-7.28333834177506,20.5318833700342,
85.5311048457282));
#119243=CARTESIAN_POINT('Ctrl Pts',(-7.24933600575288,20.4967193018425,
85.5420222251503));
#119244=CARTESIAN_POINT('Ctrl Pts',(-7.21523874947433,20.4633745956437,
85.5516581337858));
#119245=CARTESIAN_POINT('Ctrl Pts',(-7.19291786555609,20.4415463491046,
85.5579660312993));
#119246=CARTESIAN_POINT('Ctrl Pts',(-7.17055608797526,20.4204967554895,
85.5637254316562));
#119247=CARTESIAN_POINT('Ctrl Pts',(-7.14818109510134,20.4002191741198,
85.5689472100749));
#119248=CARTESIAN_POINT('Ctrl Pts',(-7.11825287463554,20.3730963978505,
85.5759317278631));
#119249=CARTESIAN_POINT('Ctrl Pts',(-7.08830176189899,20.3473563759075,
85.5819536290381));
#119250=CARTESIAN_POINT('Ctrl Pts',(-7.05840633710034,20.3230076680704,
85.5870306408997));
#119251=CARTESIAN_POINT('Ctrl Pts',(-7.01998447469757,20.2917144950011,
85.5935556611153));
#119252=CARTESIAN_POINT('Ctrl Pts',(-6.98168418706005,20.2627155071484,
85.5985165424507));
#119253=CARTESIAN_POINT('Ctrl Pts',(-6.94356148768183,20.2359899576851,
85.6019927183458));
#119254=CARTESIAN_POINT('Ctrl Pts',(-6.90863319582898,20.2115038167033,
85.6051776157476));
#119255=CARTESIAN_POINT('Ctrl Pts',(-6.87385512777084,20.1889265390783,
85.6071162886427));
#119256=CARTESIAN_POINT('Ctrl Pts',(-6.83932345299749,20.1682889367351,
85.6078564420343));
#119257=CARTESIAN_POINT('Ctrl Pts',(-6.80072505024667,20.1452208842216,
85.6086837618471));
#119258=CARTESIAN_POINT('Ctrl Pts',(-6.76243438098927,20.124575521933,85.6080140932172));
#119259=CARTESIAN_POINT('Ctrl Pts',(-6.72453642013718,20.1063527673125,
85.6059151707774));
#119260=CARTESIAN_POINT('Ctrl Pts',(-6.71391650835035,20.1012463171967,
85.6053270026898));
#119261=CARTESIAN_POINT('Ctrl Pts',(-6.70332717263078,20.0963299095061,
85.6046265848816));
#119262=CARTESIAN_POINT('Ctrl Pts',(-6.69276971843498,20.0916031601899,
85.6038153499371));
#119263=CARTESIAN_POINT('Ctrl Pts',(-6.65757504863047,20.0758459162232,
85.6011109909621));
#119264=CARTESIAN_POINT('Ctrl Pts',(-6.62273893243763,20.0621968271072,
85.5971767052845));
#119265=CARTESIAN_POINT('Ctrl Pts',(-6.58841052103251,20.0506322793736,
85.5921113489862));
#119266=CARTESIAN_POINT('Ctrl Pts',(-6.57444222050592,20.0459266413441,
85.5900502451904));
#119267=CARTESIAN_POINT('Ctrl Pts',(-6.56055738483732,20.0415660736729,
85.5878016471825));
#119268=CARTESIAN_POINT('Ctrl Pts',(-6.54676386035728,20.0375488864052,
85.5853713237095));
#119269=CARTESIAN_POINT('Origin',(-2.02513312664091,22.5,85.48888938658));
#119270=CARTESIAN_POINT('Origin',(-5.70733270705591,22.5,87.05138938658));
#119271=CARTESIAN_POINT('Origin',(-2.02513312664091,22.5,85.48888938658));
#119272=CARTESIAN_POINT('Ctrl Pts',(-1.86852584115091,-0.200657301970986,
95.96514097396));
#119273=CARTESIAN_POINT('Ctrl Pts',(-1.87679361636091,0.397260618019714,
95.95539499753));
#119274=CARTESIAN_POINT('Ctrl Pts',(-1.81764502158091,1.61545674784001,
96.02675082903));
#119275=CARTESIAN_POINT('Ctrl Pts',(-1.51056034305091,3.37210791261202,
96.3812545342701));
#119276=CARTESIAN_POINT('Ctrl Pts',(-1.03549752546091,4.99180633572701,
96.87949059878));
#119277=CARTESIAN_POINT('Ctrl Pts',(-0.47565565201091,6.40141962980201,
97.39996719591));
#119278=CARTESIAN_POINT('Ctrl Pts',(0.128959222729088,7.63825880799903,
97.89143667163));
#119279=CARTESIAN_POINT('Ctrl Pts',(0.78047764573909,8.77397550221601,98.34798763131));
#119280=CARTESIAN_POINT('Ctrl Pts',(1.50402784399909,9.87146117248002,98.77288024243));
#119281=CARTESIAN_POINT('Ctrl Pts',(2.31936621098909,10.95615772036,99.1532466824299));
#119282=CARTESIAN_POINT('Ctrl Pts',(3.21879357943909,12.01000937004,99.45696306809));
#119283=CARTESIAN_POINT('Ctrl Pts',(4.1912683517691,13.0170795927,99.65335362598));
#119284=CARTESIAN_POINT('Ctrl Pts',(5.2757469215191,14.01086777604,99.7165874722901));
#119285=CARTESIAN_POINT('Ctrl Pts',(6.5351502248891,15.02007613619,99.5796055175001));
#119286=CARTESIAN_POINT('Ctrl Pts',(7.73731890968909,15.84006914657,99.1892695249101));
#119287=CARTESIAN_POINT('Ctrl Pts',(8.5044225018091,16.29480837482,98.77493643233));
#119288=CARTESIAN_POINT('Ctrl Pts',(8.76798669870909,16.44357118509,98.6108142135001));
#119289=CARTESIAN_POINT('Ctrl Pts',(-2.76633335145391,-0.277061106735686,
89.62464525754));
#119290=CARTESIAN_POINT('Ctrl Pts',(-2.78010061236391,0.548141406161314,
89.61313564381));
#119291=CARTESIAN_POINT('Ctrl Pts',(-2.67974655644691,2.23539163023501,
89.69951614818));
#119292=CARTESIAN_POINT('Ctrl Pts',(-2.18690829439091,4.52753916756702,
90.11267233159));
#119293=CARTESIAN_POINT('Ctrl Pts',(-1.49193309304091,6.44657897676101,
90.65739218289));
#119294=CARTESIAN_POINT('Ctrl Pts',(-0.744560214060911,7.96637647141302,
91.1950322953901));
#119295=CARTESIAN_POINT('Ctrl Pts',(-0.000714101840911076,9.19387013708703,
91.67997579193));
#119296=CARTESIAN_POINT('Ctrl Pts',(0.743218764159092,10.2409288401,92.11363373692));
#119297=CARTESIAN_POINT('Ctrl Pts',(1.51015059767909,11.1834522333,92.50353807267));
#119298=CARTESIAN_POINT('Ctrl Pts',(2.30766423261909,12.04981733614,92.84138179648));
#119299=CARTESIAN_POINT('Ctrl Pts',(3.11198293474909,12.83069438562,93.10362209738));
#119300=CARTESIAN_POINT('Ctrl Pts',(3.89792431306909,13.52231896489,93.27156799052));
#119301=CARTESIAN_POINT('Ctrl Pts',(4.67814510883909,14.15587807635,93.33468615681));
#119302=CARTESIAN_POINT('Ctrl Pts',(5.4599957395091,14.75400852768,93.25754212455));
#119303=CARTESIAN_POINT('Ctrl Pts',(6.06740744298909,15.2155704877,93.02226348412));
#119304=CARTESIAN_POINT('Ctrl Pts',(6.38629556221909,15.47756556229,92.7840149103));
#119305=CARTESIAN_POINT('Ctrl Pts',(6.48862860801909,15.56565674012,92.69092482342));
#119306=CARTESIAN_POINT('Ctrl Pts',(-8.21314323670391,-0.382376649944286,
86.25787732271));
#119307=CARTESIAN_POINT('Ctrl Pts',(-8.23233050746892,0.756384491850314,
86.2455034223201));
#119308=CARTESIAN_POINT('Ctrl Pts',(-8.09201734092391,3.08654305365901,
86.33967991873));
#119309=CARTESIAN_POINT('Ctrl Pts',(-7.41007493507491,6.21008628532401,
86.78035394901));
#119310=CARTESIAN_POINT('Ctrl Pts',(-6.46595117430891,8.76366891642203,
87.33791220527));
#119311=CARTESIAN_POINT('Ctrl Pts',(-5.47046355413091,10.73360469488,87.86524851897));
#119312=CARTESIAN_POINT('Ctrl Pts',(-4.49835120662891,12.28405501304,88.3219438496));
#119313=CARTESIAN_POINT('Ctrl Pts',(-3.54419140703191,13.57328011442,88.71413997378));
#119314=CARTESIAN_POINT('Ctrl Pts',(-2.58024571757991,14.70275906295,89.05110200106));
#119315=CARTESIAN_POINT('Ctrl Pts',(-1.60151740187091,15.70963613843,89.32658646923));
#119316=CARTESIAN_POINT('Ctrl Pts',(-0.643241151590912,16.5857007526,89.52289696124));
#119317=CARTESIAN_POINT('Ctrl Pts',(0.258320540729089,17.33121239699,89.6296159923701));
#119318=CARTESIAN_POINT('Ctrl Pts',(1.10917349098909,17.98470665617,89.644481026));
#119319=CARTESIAN_POINT('Ctrl Pts',(1.89817703664909,18.57234274478,89.5498507959201));
#119320=CARTESIAN_POINT('Ctrl Pts',(2.42972632590909,19.00878869518,89.36136454575));
#119321=CARTESIAN_POINT('Ctrl Pts',(2.66092298708909,19.26095009207,89.20319983242));
#119322=CARTESIAN_POINT('Ctrl Pts',(2.72918498241909,19.3474423808,89.14448415142));
#119323=CARTESIAN_POINT('Ctrl Pts',(-14.2862958551049,-0.440758245828086,
88.2895013269199));
#119324=CARTESIAN_POINT('Ctrl Pts',(-14.3069203009679,0.872018283434913,
88.2777849287));
#119325=CARTESIAN_POINT('Ctrl Pts',(-14.1566719512549,3.55593252096201,
88.36691425296));
#119326=CARTESIAN_POINT('Ctrl Pts',(-13.4184630337948,7.20801986586801,
88.78415381662));
#119327=CARTESIAN_POINT('Ctrl Pts',(-12.3753852541951,10.27436448968,89.3116591898701));
#119328=CARTESIAN_POINT('Ctrl Pts',(-11.2498853426949,12.71021402121,89.8086449352));
#119329=CARTESIAN_POINT('Ctrl Pts',(-10.1248635377679,14.68333765206,90.23571355337));
#119330=CARTESIAN_POINT('Ctrl Pts',(-8.99406462449291,16.37115120725,90.59773884278));
#119331=CARTESIAN_POINT('Ctrl Pts',(-7.82135743268891,17.89486271208,90.90193228787));
#119332=CARTESIAN_POINT('Ctrl Pts',(-6.59288141698792,19.29990188201,91.1401305760401));
#119333=CARTESIAN_POINT('Ctrl Pts',(-5.34245787553691,20.5707644631,91.2935385755));
#119334=CARTESIAN_POINT('Ctrl Pts',(-4.10638909157991,21.70068773103,91.3503426401699));
#119335=CARTESIAN_POINT('Ctrl Pts',(-2.86088161342491,22.73992455031,91.30356781784));
#119336=CARTESIAN_POINT('Ctrl Pts',(-1.58517092003091,23.72520760639,91.1267204027899));
#119337=CARTESIAN_POINT('Ctrl Pts',(-0.555955217310912,24.48794052554,90.8430628426899));
#119338=CARTESIAN_POINT('Ctrl Pts',(0.0112272501190876,24.92026069551,90.6113068883499));
#119339=CARTESIAN_POINT('Ctrl Pts',(0.19711543522909,25.06537831943,90.52555227838));
#119340=CARTESIAN_POINT('Ctrl Pts',(-1.00773525083376,22.4999925247862,
90.8939704740664));
#119341=CARTESIAN_POINT('Ctrl Pts',(-0.913881385337355,22.6929489369076,
90.8763043702935));
#119342=CARTESIAN_POINT('Ctrl Pts',(-0.821284198747461,22.877174794995,
90.856339427234));
#119343=CARTESIAN_POINT('Ctrl Pts',(-0.730256985160353,23.0529605945689,
90.8342888831775));
#119344=CARTESIAN_POINT('Ctrl Pts',(-0.637872403585209,23.2313676543977,
90.8119095286318));
#119345=CARTESIAN_POINT('Ctrl Pts',(-0.547105332201889,23.4010810682236,
90.7873821522087));
#119346=CARTESIAN_POINT('Ctrl Pts',(-0.458254687202534,23.5624045216343,
90.7609754970322));
#119347=CARTESIAN_POINT('Ctrl Pts',(-0.36847061103016,23.7254227780524,
90.7342914235531));
#119348=CARTESIAN_POINT('Ctrl Pts',(-0.280643724697561,23.8798738645884,
90.7056887345579));
#119349=CARTESIAN_POINT('Ctrl Pts',(-0.195048516452712,24.0260711389505,
90.6754865677338));
#119350=CARTESIAN_POINT('Ctrl Pts',(-0.107589728737015,24.1754514213897,
90.6446268391229));
#119351=CARTESIAN_POINT('Ctrl Pts',(-0.0224611347238633,24.3162145750682,
90.6120976040466));
#119352=CARTESIAN_POINT('Ctrl Pts',(0.0600841858518275,24.4486948738206,
90.5782772436489));
#119353=CARTESIAN_POINT('Ctrl Pts',(0.112701886340464,24.5331431336587,
90.5567187884704));
#119354=CARTESIAN_POINT('Ctrl Pts',(0.164270749100463,24.6142258216448,
90.5346364601734));
#119355=CARTESIAN_POINT('Ctrl Pts',(0.214734006960575,24.6920295183809,
90.5121348736941));
#119356=CARTESIAN_POINT('Origin',(-10.9843331791359,-92.5,65.395787724084));
#119357=CARTESIAN_POINT('',(0.214666888280743,89.,90.5121648014016));
#119358=CARTESIAN_POINT('Origin',(-2.02513312664091,89.,85.48888938658));
#119359=CARTESIAN_POINT('',(-7.08815755064843,89.,87.6373268843701));
#119360=CARTESIAN_POINT('Origin',(-2.02513312664091,89.,85.48888938658));
#119361=CARTESIAN_POINT('',(-5.70733025617244,90.4999999999959,87.051388346575));
#119362=CARTESIAN_POINT('Origin',(-5.70733270705591,89.,87.05138938658));
#119363=CARTESIAN_POINT('Origin',(-2.02513312664091,90.49999999999,85.48888938658));
#119364=CARTESIAN_POINT('Origin',(-2.27593483123091,90.5,69.192338555332));
#119365=CARTESIAN_POINT('',(-5.7073302546465,90.4999999999959,58.9263904272322));
#119366=CARTESIAN_POINT('Origin',(27.4324635166691,90.5,72.98888938658));
#119367=CARTESIAN_POINT('Origin',(-2.02513312664091,90.49999999999,60.48888938658));
#119368=CARTESIAN_POINT('Origin',(-2.02513312664091,89.,60.48888938658));
#119369=CARTESIAN_POINT('',(-7.08815755380101,89.,58.3404518962193));
#119370=CARTESIAN_POINT('Origin',(-5.70733270705591,89.,58.92638938658));
#119371=CARTESIAN_POINT('Origin',(-2.02513312664091,89.,60.48888938658));
#119372=CARTESIAN_POINT('Origin',(-10.9843331791359,-92.5,80.581991049076));
#119373=CARTESIAN_POINT('',(0.214770984780106,21.31105212978,55.4656603870195));
#119374=CARTESIAN_POINT('Ctrl Pts',(5.21275554925909,16.84790218393,55.1007357528));
#119375=CARTESIAN_POINT('Ctrl Pts',(5.08987221057909,16.79738018542,55.08711855268));
#119376=CARTESIAN_POINT('Ctrl Pts',(4.53992236271909,16.56567500218,55.02943324933));
#119377=CARTESIAN_POINT('Ctrl Pts',(3.59664713182909,16.12384541239,54.9543844059));
#119378=CARTESIAN_POINT('Ctrl Pts',(2.42419774846909,15.48152670993,54.8998706626));
#119379=CARTESIAN_POINT('Ctrl Pts',(1.37116655289909,14.81743214788,54.87937490558));
#119380=CARTESIAN_POINT('Ctrl Pts',(0.421859436239088,14.13775868448,54.88216912445));
#119381=CARTESIAN_POINT('Ctrl Pts',(-0.446505860180913,13.43742265295,54.90142155045));
#119382=CARTESIAN_POINT('Ctrl Pts',(-1.26178821829091,12.69950859659,54.93347110475));
#119383=CARTESIAN_POINT('Ctrl Pts',(-1.81779397457091,12.13439310831,54.96399549816));
#119384=CARTESIAN_POINT('Ctrl Pts',(-2.10763051195091,11.81847011659,54.9822761899501));
#119385=CARTESIAN_POINT('Ctrl Pts',(-2.14449596917091,11.77792717693,54.9846401213));
#119386=CARTESIAN_POINT('Ctrl Pts',(3.41542118564909,18.16535552692,56.05233703107));
#119387=CARTESIAN_POINT('Ctrl Pts',(3.29153510574909,18.12260617231,56.02604874878));
#119388=CARTESIAN_POINT('Ctrl Pts',(2.73528597745909,17.92273095754,55.9107434192));
#119389=CARTESIAN_POINT('Ctrl Pts',(1.76818306694909,17.51347174676,55.73169222743));
#119390=CARTESIAN_POINT('Ctrl Pts',(0.548997708799087,16.87566838021,55.5460284887601));
#119391=CARTESIAN_POINT('Ctrl Pts',(-0.557108605230912,16.18769292699,55.40933909873));
#119392=CARTESIAN_POINT('Ctrl Pts',(-1.55941549777091,15.46717855553,55.3104586032101));
#119393=CARTESIAN_POINT('Ctrl Pts',(-2.48080341267091,14.7114503467,55.23984281602));
#119394=CARTESIAN_POINT('Ctrl Pts',(-3.34714675340591,13.90828499752,55.1905881852));
#119395=CARTESIAN_POINT('Ctrl Pts',(-3.93855870358191,13.28946121546,55.16788012438));
#119396=CARTESIAN_POINT('Ctrl Pts',(-4.24409608839291,12.94795249993,55.15906941751));
#119397=CARTESIAN_POINT('Ctrl Pts',(-4.28290610423791,12.90420804222,55.1579968414401));
#119398=CARTESIAN_POINT('Ctrl Pts',(1.65053628828909,19.82150258154,56.17061479967));
#119399=CARTESIAN_POINT('Ctrl Pts',(1.52396188714909,19.77706403619,56.12774489951));
#119400=CARTESIAN_POINT('Ctrl Pts',(0.954443363319088,19.56713881503,55.93839722755));
#119401=CARTESIAN_POINT('Ctrl Pts',(-0.0439950975309107,19.12236569434,
55.63472119012));
#119402=CARTESIAN_POINT('Ctrl Pts',(-1.31089293764091,18.41257410019,55.30270839141));
#119403=CARTESIAN_POINT('Ctrl Pts',(-2.46454089411091,17.63895669212,55.04252121858));
#119404=CARTESIAN_POINT('Ctrl Pts',(-3.50973548507091,16.82817478502,54.83934772625));
#119405=CARTESIAN_POINT('Ctrl Pts',(-4.47093084477291,15.97725182874,54.67900864002));
#119406=CARTESIAN_POINT('Ctrl Pts',(-5.37247266060192,15.07666324399,54.55030739518));
#119407=CARTESIAN_POINT('Ctrl Pts',(-5.98639287753791,14.38579398253,54.47647799956));
#119408=CARTESIAN_POINT('Ctrl Pts',(-6.30055887152191,14.01004943148,54.4418538746401));
#119409=CARTESIAN_POINT('Ctrl Pts',(-6.34040880614791,13.96201778839,54.43751017046));
#119410=CARTESIAN_POINT('Ctrl Pts',(0.161630205399088,21.58781829589,55.43924838639));
#119411=CARTESIAN_POINT('Ctrl Pts',(0.0310528536290871,21.53246180977,55.37817436325));
#119412=CARTESIAN_POINT('Ctrl Pts',(-0.556874190470912,21.27199336722,55.1085788369));
#119413=CARTESIAN_POINT('Ctrl Pts',(-1.58983220620091,20.72852246885,54.67685193629));
#119414=CARTESIAN_POINT('Ctrl Pts',(-2.89883538253791,19.88017244876,54.20348512935));
#119415=CARTESIAN_POINT('Ctrl Pts',(-4.08793142591791,18.97096941006,53.82953698486));
#119416=CARTESIAN_POINT('Ctrl Pts',(-5.15998373732991,18.03294899289,53.53384318326));
#119417=CARTESIAN_POINT('Ctrl Pts',(-6.14227849942291,17.06016425825,53.29630626823));
#119418=CARTESIAN_POINT('Ctrl Pts',(-7.05829938720391,16.04342353451,53.1009784983001));
#119419=CARTESIAN_POINT('Ctrl Pts',(-7.67872411882791,15.27211287311,52.98519291411));
#119420=CARTESIAN_POINT('Ctrl Pts',(-7.99325585674391,14.85820643969,52.92959524119));
#119421=CARTESIAN_POINT('Ctrl Pts',(-8.03309757611691,14.80539351529,52.92259715796));
#119422=CARTESIAN_POINT('Ctrl Pts',(0.214764603391513,21.3110521291418,
55.4656747003203));
#119423=CARTESIAN_POINT('Ctrl Pts',(0.180854938597129,21.2147111573871,
55.4505468232702));
#119424=CARTESIAN_POINT('Ctrl Pts',(0.147018940254829,21.1178106894989,
55.4358631290332));
#119425=CARTESIAN_POINT('Ctrl Pts',(0.113269006376136,21.0203699849487,
55.4216182940488));
#119426=CARTESIAN_POINT('Ctrl Pts',(0.0414294124360488,20.8129591890258,
55.3912969557997));
#119427=CARTESIAN_POINT('Ctrl Pts',(-0.0300191465661176,20.6031023493503,
55.3629607110215));
#119428=CARTESIAN_POINT('Ctrl Pts',(-0.10098994563944,20.3909832464082,
55.3364624582132));
#119429=CARTESIAN_POINT('Ctrl Pts',(-0.175487023028061,20.1683247243989,
55.3086476045564));
#119430=CARTESIAN_POINT('Ctrl Pts',(-0.249457389675094,19.9431739149331,
55.2828585215437));
#119431=CARTESIAN_POINT('Ctrl Pts',(-0.322817933803376,19.7157137436041,
55.2589715907221));
#119432=CARTESIAN_POINT('Ctrl Pts',(-0.350917171761308,19.6285898331142,
55.2498221963001));
#119433=CARTESIAN_POINT('Ctrl Pts',(-0.378927138419568,19.5411267856233,
55.240952285874));
#119434=CARTESIAN_POINT('Ctrl Pts',(-0.406843922230958,19.4533336453778,
55.2323562594312));
#119435=CARTESIAN_POINT('Ctrl Pts',(-0.473595533320854,19.2434121302915,
55.2118023654759));
#119436=CARTESIAN_POINT('Ctrl Pts',(-0.539816199718292,19.0316029376036,
55.1928122593711));
#119437=CARTESIAN_POINT('Ctrl Pts',(-0.605437038356976,18.8179768810558,
55.1752806605715));
#119438=CARTESIAN_POINT('Ctrl Pts',(-0.689037512667965,18.5458188284756,
55.1529455303677));
#119439=CARTESIAN_POINT('Ctrl Pts',(-0.77166554544613,18.2707117621105,
55.1329772781823));
#119440=CARTESIAN_POINT('Ctrl Pts',(-0.853135974721628,17.9928053600222,
55.115210672658));
#119441=CARTESIAN_POINT('Ctrl Pts',(-0.917278510361073,17.7740066933293,
55.1012228351301));
#119442=CARTESIAN_POINT('Ctrl Pts',(-0.980699436725039,17.5534772495342,
55.0886003290476));
#119443=CARTESIAN_POINT('Ctrl Pts',(-1.04330728897502,17.331346469236,55.0772416027675));
#119444=CARTESIAN_POINT('Ctrl Pts',(-1.10591514122499,17.1092156889378,
55.0658828764875));
#119445=CARTESIAN_POINT('Ctrl Pts',(-1.16770970176269,16.8854836897017,
55.0557884827401));
#119446=CARTESIAN_POINT('Ctrl Pts',(-1.22862268601253,16.6602282693306,
55.0468703568845));
#119447=CARTESIAN_POINT('Ctrl Pts',(-1.24405012706333,16.603177793772,55.0446116617538));
#119448=CARTESIAN_POINT('Ctrl Pts',(-1.25942117156684,16.5460293014174,
55.0424284610014));
#119449=CARTESIAN_POINT('Ctrl Pts',(-1.27473433959933,16.4887822934079,
55.0403191528466));
#119450=CARTESIAN_POINT('Ctrl Pts',(-1.28995091842717,16.4318963761251,
55.0382231493454));
#119451=CARTESIAN_POINT('Ctrl Pts',(-1.30511034814177,16.3749131821594,
55.0362001097604));
#119452=CARTESIAN_POINT('Ctrl Pts',(-1.32021095540953,16.317832398685,55.0342485000666));
#119453=CARTESIAN_POINT('Ctrl Pts',(-1.32776125904341,16.2892920069477,
55.0332726952197));
#119454=CARTESIAN_POINT('Ctrl Pts',(-1.3352968570784,16.2607272178333,55.0323147479457));
#119455=CARTESIAN_POINT('Ctrl Pts',(-1.34281751604111,16.2321380119861,
55.0313744699216));
#119456=CARTESIAN_POINT('Ctrl Pts',(-1.34657784552247,16.2178434090626,
55.0309043309095));
#119457=CARTESIAN_POINT('Ctrl Pts',(-1.35033444023579,16.2035427019558,
55.0304386092098));
#119458=CARTESIAN_POINT('Ctrl Pts',(-1.35408727034747,16.1892358887999,
55.0299772813598));
#119459=CARTESIAN_POINT('Ctrl Pts',(-1.35596368540331,16.1820824822219,
55.0297466174348));
#119460=CARTESIAN_POINT('Ctrl Pts',(-1.35783915930872,16.1749275491317,
55.0295170519722));
#119461=CARTESIAN_POINT('Ctrl Pts',(-1.35971368824907,16.1677710893663,
55.0292885820492));
#119462=CARTESIAN_POINT('Ctrl Pts',(-1.36158821718942,16.1606146296009,
55.0290601121261));
#119463=CARTESIAN_POINT('Ctrl Pts',(-1.36390932142334,16.1517456707088,
55.0287786611796));
#119464=CARTESIAN_POINT('Ctrl Pts',(-1.36533443633472,16.146297129903,55.0286064559783));
#119465=CARTESIAN_POINT('Ctrl Pts',(-1.42768981805868,15.9078982197032,
55.0210716803769));
#119466=CARTESIAN_POINT('Ctrl Pts',(-1.4884755321976,15.6700343355104,55.0148090280403));
#119467=CARTESIAN_POINT('Ctrl Pts',(-1.54768204110244,15.4328191754794,
55.0096521710442));
#119468=CARTESIAN_POINT('Ctrl Pts',(-1.59598853326158,15.2392757208825,
55.0054446999966));
#119469=CARTESIAN_POINT('Ctrl Pts',(-1.64323935791373,15.0461703467149,
55.0019734168841));
#119470=CARTESIAN_POINT('Ctrl Pts',(-1.68944051522512,14.8535968995406,
54.9991481034072));
#119471=CARTESIAN_POINT('Ctrl Pts',(-1.7356416725365,14.6610234523662,54.9963227899303));
#119472=CARTESIAN_POINT('Ctrl Pts',(-1.78079333866968,14.4689815333594,
54.9941437027382));
#119473=CARTESIAN_POINT('Ctrl Pts',(-1.82492463553365,14.2775166933926,
54.9925345386017));
#119474=CARTESIAN_POINT('Ctrl Pts',(-1.84080564612811,14.2086164940318,
54.9919554676358));
#119475=CARTESIAN_POINT('Ctrl Pts',(-1.85655476412944,14.1397905502665,
54.9914503172646));
#119476=CARTESIAN_POINT('Ctrl Pts',(-1.87217181097862,14.0710412448739,
54.9910155527655));
#119477=CARTESIAN_POINT('Ctrl Pts',(-1.94160339402295,13.7653897889553,
54.9890826401148));
#119478=CARTESIAN_POINT('Ctrl Pts',(-2.00842718663851,13.4612560904928,
54.9885384899925));
#119479=CARTESIAN_POINT('Ctrl Pts',(-2.07260302534106,13.1588273555174,
54.9890942440626));
#119480=CARTESIAN_POINT('Ctrl Pts',(-2.09829868771968,13.0377365084847,
54.9893167650181));
#119481=CARTESIAN_POINT('Ctrl Pts',(-2.12356740923878,12.9169225119993,
54.9897158412855));
#119482=CARTESIAN_POINT('Ctrl Pts',(-2.14841466004433,12.7963954402831,
54.9902741273346));
#119483=CARTESIAN_POINT('Ctrl Pts',(-2.17450028860511,12.6698613440601,
54.9908602381531));
#119484=CARTESIAN_POINT('Ctrl Pts',(-2.2001213545838,12.5436435262945,54.9916218281353));
#119485=CARTESIAN_POINT('Ctrl Pts',(-2.2253115642739,12.417699967537,54.9925407754541));
#119486=CARTESIAN_POINT('Ctrl Pts',(-2.25050177396401,12.2917564087794,
54.9934597227729));
#119487=CARTESIAN_POINT('Ctrl Pts',(-2.27526132344878,12.1660867047988,
54.9945360459858));
#119488=CARTESIAN_POINT('Ctrl Pts',(-2.29964905129997,12.0405998990293,
54.995753327958));
#119489=CARTESIAN_POINT('Origin',(1.07038457110909,25.,122.41156512159));
#119490=CARTESIAN_POINT('',(-2.29973550185091,10.,54.99574879712));
#119491=CARTESIAN_POINT('Origin',(-2.02513312664091,10.,60.48888938658));
#119492=CARTESIAN_POINT('Origin',(-5.70733270705591,10.,58.92638938658));
#119493=CARTESIAN_POINT('Origin',(-2.02513312664091,10.,60.48888938658));
#119494=CARTESIAN_POINT('Origin',(27.4324635166691,10.,72.98888938658));
#119495=CARTESIAN_POINT('Origin',(-6.80729512863291,91.08441266238,84.10819367738));
#119496=CARTESIAN_POINT('Origin',(27.4324635166691,22.5,72.98888938658));
#119497=CARTESIAN_POINT('Origin',(-2.02513312664091,-92.5,85.48888938658));
#119498=CARTESIAN_POINT('',(-7.08838232372406,85.1740126527982,87.6374222456928));
#119499=CARTESIAN_POINT('Ctrl Pts',(-7.0883818064374,64.8259873343748,87.637422020082));
#119500=CARTESIAN_POINT('Ctrl Pts',(-7.06379466657136,65.03820054502,87.6953798859809));
#119501=CARTESIAN_POINT('Ctrl Pts',(-7.03897737033209,65.2515735354143,
87.7510159589579));
#119502=CARTESIAN_POINT('Ctrl Pts',(-7.01415562444538,65.4660641629207,
87.8044130368114));
#119503=CARTESIAN_POINT('Ctrl Pts',(-6.98858405264758,65.6870342149981,
87.8594231564201));
#119504=CARTESIAN_POINT('Ctrl Pts',(-6.96300721566767,65.9091904325734,
87.9120570715152));
#119505=CARTESIAN_POINT('Ctrl Pts',(-6.93763343777821,66.1325240456197,
87.9623874104707));
#119506=CARTESIAN_POINT('Ctrl Pts',(-6.91119723122836,66.3652088885995,
88.0148251374087));
#119507=CARTESIAN_POINT('Ctrl Pts',(-6.88498087704221,66.5991717001637,
88.064762513918));
#119508=CARTESIAN_POINT('Ctrl Pts',(-6.85918743756997,66.8344433770868,
88.1122603178858));
#119509=CARTESIAN_POINT('Ctrl Pts',(-6.85102495572795,66.9088964484926,
88.1272912703434));
#119510=CARTESIAN_POINT('Ctrl Pts',(-6.84290462584899,66.9834808964798,
88.1420777481535));
#119511=CARTESIAN_POINT('Ctrl Pts',(-6.83483238691541,67.0581985226156,
88.1566212148313));
#119512=CARTESIAN_POINT('Ctrl Pts',(-6.82950733941523,67.107487810451,88.1662151641078));
#119513=CARTESIAN_POINT('Ctrl Pts',(-6.82420321472302,67.1568350591063,
88.175703359103));
#119514=CARTESIAN_POINT('Ctrl Pts',(-6.81892161009561,67.2062392427801,
88.1850867777694));
#119515=CARTESIAN_POINT('Ctrl Pts',(-6.79460045638261,67.4337395632247,
88.2282962915135));
#119516=CARTESIAN_POINT('Ctrl Pts',(-6.77075805880709,67.6624482893294,
88.2692850297369));
#119517=CARTESIAN_POINT('Ctrl Pts',(-6.74754274177323,67.8923491571023,
88.3081363926079));
#119518=CARTESIAN_POINT('Ctrl Pts',(-6.72950180658429,68.0710082143671,
88.3383283093729));
#119519=CARTESIAN_POINT('Ctrl Pts',(-6.7118393390258,68.2503882255433,88.3672287815631));
#119520=CARTESIAN_POINT('Ctrl Pts',(-6.6946249460294,68.4304987288456,88.3948638281204));
#119521=CARTESIAN_POINT('Ctrl Pts',(-6.67494189379613,68.6364382844837,
88.4264619254201));
#119522=CARTESIAN_POINT('Ctrl Pts',(-6.65584162687453,68.8433259942116,
88.4564106873118));
#119523=CARTESIAN_POINT('Ctrl Pts',(-6.63741314843917,69.0511618587221,
88.4847590086765));
#119524=CARTESIAN_POINT('Ctrl Pts',(-6.62819890922149,69.1550797909774,
88.4989331693589));
#119525=CARTESIAN_POINT('Ctrl Pts',(-6.61915252166941,69.25923476194,88.5127071591024));
#119526=CARTESIAN_POINT('Ctrl Pts',(-6.61028438410816,69.3636267717451,
88.5260871339677));
#119527=CARTESIAN_POINT('Ctrl Pts',(-6.60585031532754,69.4158227766476,
88.5327771214003));
#119528=CARTESIAN_POINT('Ctrl Pts',(-6.60146080436318,69.4680780412606,
88.53936860247));
#119529=CARTESIAN_POINT('Ctrl Pts',(-6.59711712217367,69.5203925655962,
88.5458623381286));
#119530=CARTESIAN_POINT('Ctrl Pts',(-6.59494528107892,69.546549827764,88.5491092059579));
#119531=CARTESIAN_POINT('Ctrl Pts',(-6.5927848969414,69.5727219048623,88.5523316373004));
#119532=CARTESIAN_POINT('Ctrl Pts',(-6.5906361265566,69.5989087968919,88.555529727633));
#119533=CARTESIAN_POINT('Ctrl Pts',(-6.58848735617179,69.6250956889215,
88.5587278179656));
#119534=CARTESIAN_POINT('Ctrl Pts',(-6.58644313922851,69.6501509912735,
88.5617638446549));
#119535=CARTESIAN_POINT('Ctrl Pts',(-6.58422481242837,69.6775139177743,
88.5650510709359));
#119536=CARTESIAN_POINT('Ctrl Pts',(-6.56410003276806,69.9257518539767,
88.5948729639929));
#119537=CARTESIAN_POINT('Ctrl Pts',(-6.54513276355699,70.1744087231534,
88.6223706242821));
#119538=CARTESIAN_POINT('Ctrl Pts',(-6.52746288468714,70.4235233797567,
88.6476244002884));
#119539=CARTESIAN_POINT('Ctrl Pts',(-6.51570354940074,70.5893096193416,
88.6644308323808));
#119540=CARTESIAN_POINT('Ctrl Pts',(-6.50451897291542,70.7552995617695,
88.6802428581044));
#119541=CARTESIAN_POINT('Ctrl Pts',(-6.49395412391555,70.9215145754299,
88.6950770967392));
#119542=CARTESIAN_POINT('Ctrl Pts',(-6.47849417436243,71.1647433926325,
88.7167846082195));
#119543=CARTESIAN_POINT('Ctrl Pts',(-6.46435935369875,71.4084526956892,
88.7363996338555));
#119544=CARTESIAN_POINT('Ctrl Pts',(-6.45152719394054,71.6525968740843,
88.7540050221084));
#119545=CARTESIAN_POINT('Ctrl Pts',(-6.43849859227522,71.9004785486544,
88.7718799235304));
#119546=CARTESIAN_POINT('Ctrl Pts',(-6.42681257394867,72.1488090208903,
88.7876831470584));
#119547=CARTESIAN_POINT('Ctrl Pts',(-6.41648044535944,72.397570219193,88.801473345101));
#119548=CARTESIAN_POINT('Ctrl Pts',(-6.40604941678005,72.6487125802786,
88.8153955440609));
#119549=CARTESIAN_POINT('Ctrl Pts',(-6.39699804956997,72.9002945114833,
88.8272659517491));
#119550=CARTESIAN_POINT('Ctrl Pts',(-6.38937723579345,73.1523192932256,
88.8371172189261));
#119551=CARTESIAN_POINT('Ctrl Pts',(-6.38177776433586,73.4036382719624,
88.8469408973322));
#119552=CARTESIAN_POINT('Ctrl Pts',(-6.37560062815082,73.6553982145796,
88.8547566569079));
#119553=CARTESIAN_POINT('Ctrl Pts',(-6.37093868730099,73.9076153300843,
88.8605704111973));
#119554=CARTESIAN_POINT('Ctrl Pts',(-6.36634677417501,74.1560438538663,
88.8662968361977));
#119555=CARTESIAN_POINT('Ctrl Pts',(-6.36322473582904,74.4049164792301,
88.8700808561546));
#119556=CARTESIAN_POINT('Ctrl Pts',(-6.36170502115568,74.6542527439161,
88.8719037070657));
#119557=CARTESIAN_POINT('Ctrl Pts',(-6.36100385159357,74.7692921013646,
88.8727447383446));
#119558=CARTESIAN_POINT('Ctrl Pts',(-6.36064440344129,74.8844301613427,
88.8731679528114));
#119559=CARTESIAN_POINT('Ctrl Pts',(-6.36064303502608,74.9996686417215,
88.8731697877771));
#119560=CARTESIAN_POINT('Ctrl Pts',(-6.36064303474299,74.9996924816059,
88.8731697881567));
#119561=CARTESIAN_POINT('Ctrl Pts',(-6.3606430344747,74.9997163214862,88.8731697885189));
#119562=CARTESIAN_POINT('Ctrl Pts',(-6.36064303422121,74.9997401613624,
88.8731697888638));
#119563=CARTESIAN_POINT('Ctrl Pts',(-6.36064037275879,75.2500455466579,
88.8731734100344));
#119564=CARTESIAN_POINT('Ctrl Pts',(-6.36226542360875,75.4998974699238,
88.8712654838432));
#119565=CARTESIAN_POINT('Ctrl Pts',(-6.3654009159308,75.7493144063505,88.86742892387));
#119566=CARTESIAN_POINT('Ctrl Pts',(-6.36856862205069,76.0012938324725,
88.8635529473859));
#119567=CARTESIAN_POINT('Ctrl Pts',(-6.37327830216265,76.2528298495998,
88.8577085595702));
#119568=CARTESIAN_POINT('Ctrl Pts',(-6.37945537706228,76.503929709642,88.8498538555591));
#119569=CARTESIAN_POINT('Ctrl Pts',(-6.38565350919478,76.7558855522182,
88.8419723753902));
#119570=CARTESIAN_POINT('Ctrl Pts',(-6.39332941744835,77.0074028106557,
88.8320668995079));
#119571=CARTESIAN_POINT('Ctrl Pts',(-6.40244884291788,77.258468608758,88.8200700124218));
#119572=CARTESIAN_POINT('Ctrl Pts',(-6.40753815588165,77.3985818675713,
88.8133748633496));
#119573=CARTESIAN_POINT('Ctrl Pts',(-6.41307774881445,77.5385541127024,
88.8060279003157));
#119574=CARTESIAN_POINT('Ctrl Pts',(-6.41906658906012,77.6783794171587,
88.7980139264912));
#119575=CARTESIAN_POINT('Ctrl Pts',(-6.42961407071633,77.9246382541503,
88.7838998011448));
#119576=CARTESIAN_POINT('Ctrl Pts',(-6.44153211992909,78.170458717253,88.7677456921256));
#119577=CARTESIAN_POINT('Ctrl Pts',(-6.45477301806723,78.4158477603694,
88.7495427829172));
#119578=CARTESIAN_POINT('Ctrl Pts',(-6.46538522170445,78.6125201060613,
88.7349536683953));
#119579=CARTESIAN_POINT('Ctrl Pts',(-6.47684792880327,78.8089152817468,
88.7190479852231));
#119580=CARTESIAN_POINT('Ctrl Pts',(-6.48915462984713,79.0050284462474,
88.7018073908017));
#119581=CARTESIAN_POINT('Ctrl Pts',(-6.49071151880142,79.0298382160235,
88.6996263277431));
#119582=CARTESIAN_POINT('Ctrl Pts',(-6.49228179757586,79.0546436053862,
88.6974240762827));
#119583=CARTESIAN_POINT('Ctrl Pts',(-6.49386552851074,79.0794444862278,
88.6952005063406));
#119584=CARTESIAN_POINT('Ctrl Pts',(-6.50635116928276,79.2749668961259,
88.6776705743827));
#119585=CARTESIAN_POINT('Ctrl Pts',(-6.51967251742695,79.4702103739657,
88.658816297229));
#119586=CARTESIAN_POINT('Ctrl Pts',(-6.53376695262603,79.6651764666531,
88.6385971265922));
#119587=CARTESIAN_POINT('Ctrl Pts',(-6.54170806880242,79.7750246706158,
88.6272051991578));
#119588=CARTESIAN_POINT('Ctrl Pts',(-6.54989472187858,79.8847846386297,
88.6153797943906));
#119589=CARTESIAN_POINT('Ctrl Pts',(-6.55831553553021,79.9944563692783,
88.6031135000803));
#119590=CARTESIAN_POINT('Ctrl Pts',(-6.56252594235602,80.0492922346025,
88.5969803529252));
#119591=CARTESIAN_POINT('Ctrl Pts',(-6.56679488603044,80.1041060406106,
88.5907369818051));
#119592=CARTESIAN_POINT('Ctrl Pts',(-6.57112091400058,80.1588977872398,
88.584382459583));
#119593=CARTESIAN_POINT('Ctrl Pts',(-6.57328392798565,80.1862936605544,
88.5812051984719));
#119594=CARTESIAN_POINT('Ctrl Pts',(-6.57546121277668,80.2136840190252,
88.5780001494511));
#119595=CARTESIAN_POINT('Ctrl Pts',(-6.57765258443277,80.2410688626487,
88.5747671967393));
#119596=CARTESIAN_POINT('Ctrl Pts',(-6.57984395608886,80.2684537062723,
88.5715342440275));
#119597=CARTESIAN_POINT('Ctrl Pts',(-6.58214377145534,80.2969968411338,
88.5681335599459));
#119598=CARTESIAN_POINT('Ctrl Pts',(-6.584268774623,80.3232068489765,88.5649845114387));
#119599=CARTESIAN_POINT('Ctrl Pts',(-6.60448466570381,80.5725517308274,
88.5350265223882));
#119600=CARTESIAN_POINT('Ctrl Pts',(-6.62580884323505,80.8205332639971,
88.5028111501408));
#119601=CARTESIAN_POINT('Ctrl Pts',(-6.64805940844237,81.0671975548834,
88.4683166923041));
#119602=CARTESIAN_POINT('Ctrl Pts',(-6.66995048632655,81.3098766577614,
88.4343795380772));
#119603=CARTESIAN_POINT('Ctrl Pts',(-6.69273887743609,81.5512810694582,
88.3982363328307));
#119604=CARTESIAN_POINT('Ctrl Pts',(-6.7162618961127,81.7914169235885,88.3598360359073));
#119605=CARTESIAN_POINT('Ctrl Pts',(-6.73899066478621,82.023444638814,88.3227323173004));
#119606=CARTESIAN_POINT('Ctrl Pts',(-6.76240583176186,82.2542881886803,
88.2835212815749));
#119607=CARTESIAN_POINT('Ctrl Pts',(-6.78636214031899,82.4839140899401,
88.2421290564647));
#119608=CARTESIAN_POINT('Ctrl Pts',(-6.80235074803454,82.6371680208544,
88.2145035962156));
#119609=CARTESIAN_POINT('Ctrl Pts',(-6.81858041995665,82.7898787767762,
88.1859060023952));
#119610=CARTESIAN_POINT('Ctrl Pts',(-6.83500657856313,82.9420255751848,
88.1563072065959));
#119611=CARTESIAN_POINT('Ctrl Pts',(-6.85992974853696,83.1728756849734,
88.1113973870575));
#119612=CARTESIAN_POINT('Ctrl Pts',(-6.88530658635467,83.4024289215281,
88.0641834221432));
#119613=CARTESIAN_POINT('Ctrl Pts',(-6.91096134814823,83.6307464515349,
88.014605662357));
#119614=CARTESIAN_POINT('Ctrl Pts',(-6.93592464561993,83.8529102145597,
87.9663641555568));
#119615=CARTESIAN_POINT('Ctrl Pts',(-6.96115166965242,84.0739039790992,
87.9158844277155));
#119616=CARTESIAN_POINT('Ctrl Pts',(-6.98645600059154,84.2937475202454,
87.8630911193911));
#119617=CARTESIAN_POINT('Ctrl Pts',(-7.01070139620015,84.5043910515804,
87.8125071047854));
#119618=CARTESIAN_POINT('Ctrl Pts',(-7.03501818894437,84.713978522577,87.7597989460343));
#119619=CARTESIAN_POINT('Ctrl Pts',(-7.05921250535445,84.9224941290667,
87.7048834370974));
#119620=CARTESIAN_POINT('Ctrl Pts',(-7.06896083979781,85.0065088965959,
87.6827569699482));
#119621=CARTESIAN_POINT('Ctrl Pts',(-7.07868890741303,85.0903492738633,
87.6602719689559));
#119622=CARTESIAN_POINT('Ctrl Pts',(-7.08838232372406,85.1740126527982,
87.6374222456928));
#119623=CARTESIAN_POINT('',(-7.08815755158633,25.,87.6373268821602));
#119624=CARTESIAN_POINT('Origin',(27.4324635166691,25.,72.98888938658));
#119625=CARTESIAN_POINT('',(-8.15022843086022,88.9999999999406,84.8262046973771));
#119626=CARTESIAN_POINT('Ctrl Pts',(-7.08815755274652,85.1740126534065,
87.6373268794261));
#119627=CARTESIAN_POINT('Ctrl Pts',(-7.17036726380078,85.5345012501752,
87.4435908386425));
#119628=CARTESIAN_POINT('Ctrl Pts',(-7.25522061315342,85.8855446623315,
87.2391013265329));
#119629=CARTESIAN_POINT('Ctrl Pts',(-7.34216730501181,86.2271428898753,
87.0236694424198));
#119630=CARTESIAN_POINT('Ctrl Pts',(-7.38564065101201,86.3979420039261,
86.9159535001874));
#119631=CARTESIAN_POINT('Ctrl Pts',(-7.42963643207846,86.5663798218163,
86.8055018223152));
#119632=CARTESIAN_POINT('Ctrl Pts',(-7.47408022130472,86.7324563435456,
86.69229058004));
#119633=CARTESIAN_POINT('Ctrl Pts',(-7.49630211591786,86.8154946044102,
86.6356849589023));
#119634=CARTESIAN_POINT('Ctrl Pts',(-7.51863596096647,86.8979425412346,
86.5783894265339));
#119635=CARTESIAN_POINT('Ctrl Pts',(-7.54107208032303,86.9798001540188,
86.5204010481027));
#119636=CARTESIAN_POINT('Ctrl Pts',(-7.56219127703993,87.0568530079322,
86.4658163870069));
#119637=CARTESIAN_POINT('Ctrl Pts',(-7.58374961926499,87.1346233889664,
86.409704963375));
#119638=CARTESIAN_POINT('Ctrl Pts',(-7.60475461115699,87.2096079961757,
86.3546421099823));
#119639=CARTESIAN_POINT('Ctrl Pts',(-7.60606441236483,87.214283786083,86.3512085741708));
#119640=CARTESIAN_POINT('Ctrl Pts',(-7.60737207769441,87.2189487439171,
86.3477791216078));
#119641=CARTESIAN_POINT('Ctrl Pts',(-7.60867737276574,87.2236020202508,
86.3443543791131));
#119642=CARTESIAN_POINT('Ctrl Pts',(-7.69897653199269,87.5455115637841,
86.1074337206083));
#119643=CARTESIAN_POINT('Ctrl Pts',(-7.79034517661201,87.8565795431264,
85.8604972245752));
#119644=CARTESIAN_POINT('Ctrl Pts',(-7.88218584960569,88.1568059583733,
85.6033866075186));
#119645=CARTESIAN_POINT('Ctrl Pts',(-7.97128639647277,88.448074923533,85.3539470527077));
#119646=CARTESIAN_POINT('Ctrl Pts',(-8.06083103308143,88.7291396040179,
85.0949311765289));
#119647=CARTESIAN_POINT('Ctrl Pts',(-8.15022843086787,88.9999999999152,
84.8262046973541));
#119648=CARTESIAN_POINT('Origin',(27.4324635166691,89.,72.98888938658));
#119649=CARTESIAN_POINT('Origin',(27.4324635166691,89.,72.98888938658));
#119650=CARTESIAN_POINT('',(-8.15023280835573,89.,61.1515872344397));
#119651=CARTESIAN_POINT('Ctrl Pts',(-8.15022843089586,89.,84.82620469727));
#119652=CARTESIAN_POINT('Ctrl Pts',(-8.23099022828455,89.040788968413,84.5834366301713));
#119653=CARTESIAN_POINT('Ctrl Pts',(-8.3072115088959,89.0804132599216,84.3407528351496));
#119654=CARTESIAN_POINT('Ctrl Pts',(-8.37920382923813,89.1187594637775,
84.0984057817494));
#119655=CARTESIAN_POINT('Ctrl Pts',(-8.4538662110039,89.1585278570998,83.8470705263394));
#119656=CARTESIAN_POINT('Ctrl Pts',(-8.52398061097728,89.1969217770695,
83.5960976664654));
#119657=CARTESIAN_POINT('Ctrl Pts',(-8.58989600097626,89.2338606648925,
83.3457359072875));
#119658=CARTESIAN_POINT('Ctrl Pts',(-8.65741525486121,89.2716983556834,
83.0892823054612));
#119659=CARTESIAN_POINT('Ctrl Pts',(-8.7205291465347,89.3080096915148,82.8334699848971));
#119660=CARTESIAN_POINT('Ctrl Pts',(-8.77960675471714,89.3427512305223,
82.5785301532357));
#119661=CARTESIAN_POINT('Ctrl Pts',(-8.84016030158506,89.3783607190456,
82.3172211476758));
#119662=CARTESIAN_POINT('Ctrl Pts',(-8.89647381090144,89.4123214017868,
82.0568287849466));
#119663=CARTESIAN_POINT('Ctrl Pts',(-8.94893137920165,89.4446254527761,
81.7975638237655));
#119664=CARTESIAN_POINT('Ctrl Pts',(-9.00272174432682,89.4777502573381,
81.5317116812056));
#119665=CARTESIAN_POINT('Ctrl Pts',(-9.05245813981911,89.5091336420425,
81.2670449049156));
#119666=CARTESIAN_POINT('Ctrl Pts',(-9.09853431394997,89.5388008973398,
81.0037513160143));
#119667=CARTESIAN_POINT('Ctrl Pts',(-9.14578370419498,89.5692235561105,
80.7337536053606));
#119668=CARTESIAN_POINT('Ctrl Pts',(-9.18918444346121,89.5978420867409,
80.4651997864143));
#119669=CARTESIAN_POINT('Ctrl Pts',(-9.22913424351228,89.6247112734543,
80.1982527545268));
#119670=CARTESIAN_POINT('Ctrl Pts',(-9.27008186582461,89.6522515692249,
79.9246382126481));
#119671=CARTESIAN_POINT('Ctrl Pts',(-9.30740428114443,89.6779545858764,
79.6527115481155));
#119672=CARTESIAN_POINT('Ctrl Pts',(-9.34149710551561,89.7018997176548,
79.382609315175));
#119673=CARTESIAN_POINT('Ctrl Pts',(-9.37682272870595,89.7267107070066,
79.1027401673497));
#119674=CARTESIAN_POINT('Ctrl Pts',(-9.40868125352791,89.7496349422738,
78.8248296112862));
#119675=CARTESIAN_POINT('Ctrl Pts',(-9.43747375244598,89.7707738252341,
78.548990948235));
#119676=CARTESIAN_POINT('Ctrl Pts',(-9.46681260492824,89.79231383017,78.2679180942535));
#119677=CARTESIAN_POINT('Ctrl Pts',(-9.49296806742673,89.8120006729132,
77.9889961971702));
#119678=CARTESIAN_POINT('Ctrl Pts',(-9.51632189397733,89.8299460219586,
77.7123096368855));
#119679=CARTESIAN_POINT('Ctrl Pts',(-9.54005451876946,89.8481824439315,
77.4311352303687));
#119680=CARTESIAN_POINT('Ctrl Pts',(-9.56089390164509,89.864620967278,77.1522689208994));
#119681=CARTESIAN_POINT('Ctrl Pts',(-9.57919626952247,89.8793745450462,
76.8757679999358));
#119682=CARTESIAN_POINT('Ctrl Pts',(-9.59773862113798,89.8943215742174,
76.5956415522067));
#119683=CARTESIAN_POINT('Ctrl Pts',(-9.61367694107309,89.9075396619312,
76.3179425767034));
#119684=CARTESIAN_POINT('Ctrl Pts',(-9.62733674672953,89.9191340964769,
76.042704161449));
#119685=CARTESIAN_POINT('Ctrl Pts',(-9.64118935864556,89.9308921848559,
75.763580794192));
#119686=CARTESIAN_POINT('Ctrl Pts',(-9.65269862180367,89.9409808739967,
75.4869875985512));
#119687=CARTESIAN_POINT('Ctrl Pts',(-9.66215898432848,89.9494907165252,
75.2129373093804));
#119688=CARTESIAN_POINT('Ctrl Pts',(-9.67166871289319,89.9580449650925,
74.9374569716806));
#119689=CARTESIAN_POINT('Ctrl Pts',(-9.6791079897816,89.9650041387877,74.6645458048206));
#119690=CARTESIAN_POINT('Ctrl Pts',(-9.68473211235737,89.9704355901593,
74.394200121574));
#119691=CARTESIAN_POINT('Ctrl Pts',(-9.69038567099905,89.9758954691761,
74.122439477461));
#119692=CARTESIAN_POINT('Ctrl Pts',(-9.69420494935699,89.9798117901643,
73.853270926103));
#119693=CARTESIAN_POINT('Ctrl Pts',(-9.69640658254741,89.9822244493205,
73.5866789427521));
#119694=CARTESIAN_POINT('Ctrl Pts',(-9.69765753916908,89.9835953098073,
73.4352027530279));
#119695=CARTESIAN_POINT('Ctrl Pts',(-9.69838547816114,89.9844801812682,
73.2845582091729));
#119696=CARTESIAN_POINT('Ctrl Pts',(-9.69862415412181,89.9848820179164,
73.1347413557224));
#119697=CARTESIAN_POINT('Ctrl Pts',(-9.69880899985258,89.9851932255835,
73.0187137269644));
#119698=CARTESIAN_POINT('Ctrl Pts',(-9.69870030258848,89.9852146484256,
72.9031825241757));
#119699=CARTESIAN_POINT('Ctrl Pts',(-9.69831197418757,89.9849463301446,
72.7881457028777));
#119700=CARTESIAN_POINT('Ctrl Pts',(-9.69811780998711,89.9848121710041,
72.7306272922287));
#119701=CARTESIAN_POINT('Ctrl Pts',(-9.69785371532275,89.9846055568432,
72.6732324771218));
#119702=CARTESIAN_POINT('Ctrl Pts',(-9.69752128278207,89.9843263864972,
72.6159609876627));
#119703=CARTESIAN_POINT('Ctrl Pts',(-9.69723837411871,89.9840888053348,
72.5672214734792));
#119704=CARTESIAN_POINT('Ctrl Pts',(-9.6968968822444,89.9837889265374,72.5172614285427));
#119705=CARTESIAN_POINT('Ctrl Pts',(-9.69652059962177,89.98345152985,72.4694248344562));
#119706=CARTESIAN_POINT('Ctrl Pts',(-9.69645473039663,89.9833924677062,
72.4610509176282));
#119707=CARTESIAN_POINT('Ctrl Pts',(-9.69638792490953,89.9833322559799,
72.4527420703728));
#119708=CARTESIAN_POINT('Ctrl Pts',(-9.6963204727055,89.9832710277394,72.4445162301548));
#119709=CARTESIAN_POINT('Ctrl Pts',(-9.69415092230604,89.9813016665379,
72.1799381457496));
#119710=CARTESIAN_POINT('Ctrl Pts',(-9.69042915325381,89.9778218956941,
71.9131805112186));
#119711=CARTESIAN_POINT('Ctrl Pts',(-9.68497059678481,89.9727958742029,
71.6442252251322));
#119712=CARTESIAN_POINT('Ctrl Pts',(-9.67950014414439,89.9677588991906,
71.3746837880731));
#119713=CARTESIAN_POINT('Ctrl Pts',(-9.67228544970801,89.9611687731311,
71.1029347875081));
#119714=CARTESIAN_POINT('Ctrl Pts',(-9.66309824485758,89.9529598432053,
70.8289704889018));
#119715=CARTESIAN_POINT('Ctrl Pts',(-9.65404878935528,89.9448739947568,
70.5591139035943));
#119716=CARTESIAN_POINT('Ctrl Pts',(-9.64308557086269,89.9352172001176,
70.2871076504854));
#119717=CARTESIAN_POINT('Ctrl Pts',(-9.62994819833856,89.9239017139816,
70.0129590830614));
#119718=CARTESIAN_POINT('Ctrl Pts',(-9.61651086337457,89.9123278640956,
69.7325509479028));
#119719=CARTESIAN_POINT('Ctrl Pts',(-9.60079931872581,89.8990184010136,
69.4499010640564));
#119720=CARTESIAN_POINT('Ctrl Pts',(-9.58248695867312,89.8838576197446,
69.1650389459225));
#119721=CARTESIAN_POINT('Ctrl Pts',(-9.56417459862044,89.8686968384756,
68.8801768277886));
#119722=CARTESIAN_POINT('Ctrl Pts',(-9.54326161077761,89.8516841940021,
68.5931019996591));
#119723=CARTESIAN_POINT('Ctrl Pts',(-9.51937003839826,89.8326890010658,
68.3038725446563));
#119724=CARTESIAN_POINT('Ctrl Pts',(-9.51325248701204,89.8278251910564,
68.2298139592566));
#119725=CARTESIAN_POINT('Ctrl Pts',(-9.50688313067602,89.82278018902,68.1549359143919));
#119726=CARTESIAN_POINT('Ctrl Pts',(-9.50041457050318,89.8176926172772,
68.0811433185792));
#119727=CARTESIAN_POINT('Ctrl Pts',(-9.49643999587079,89.8145665841186,
68.035801825026));
#119728=CARTESIAN_POINT('Ctrl Pts',(-9.49242901214205,89.8114245665556,
67.9908700903788));
#119729=CARTESIAN_POINT('Ctrl Pts',(-9.48842673027931,89.8082995552444,
67.946789497296));
#119730=CARTESIAN_POINT('Ctrl Pts',(-9.47791079514489,89.8000886352317,
67.8309684048684));
#119731=CARTESIAN_POINT('Ctrl Pts',(-9.46686551069631,89.7915572195587,
67.7146039273164));
#119732=CARTESIAN_POINT('Ctrl Pts',(-9.45525766962326,89.7826964392123,
67.5977024306567));
#119733=CARTESIAN_POINT('Ctrl Pts',(-9.43204198747717,89.7649748785196,
67.3638994373374));
#119734=CARTESIAN_POINT('Ctrl Pts',(-9.40657713178295,89.7459365233459,
67.1279482182838));
#119735=CARTESIAN_POINT('Ctrl Pts',(-9.37857876259766,89.7255146874016,
66.8899176101877));
#119736=CARTESIAN_POINT('Ctrl Pts',(-9.34777506896367,89.7030466652926,
66.6280372885596));
#119737=CARTESIAN_POINT('Ctrl Pts',(-9.31390519847322,89.6789034791376,
66.3636392431617));
#119738=CARTESIAN_POINT('Ctrl Pts',(-9.27655786722363,89.6530046963734,
66.09684619365));
#119739=CARTESIAN_POINT('Ctrl Pts',(-9.23993781998643,89.6276102540804,
65.8352485439977));
#119740=CARTESIAN_POINT('Ctrl Pts',(-9.19997422560453,89.6005274408591,
65.5713480466599));
#119741=CARTESIAN_POINT('Ctrl Pts',(-9.1562484296008,89.5716957264074,65.3052953170558));
#119742=CARTESIAN_POINT('Ctrl Pts',(-9.11386252192325,89.5437475013635,
65.0473952336954));
#119743=CARTESIAN_POINT('Ctrl Pts',(-9.06794113880673,89.5141554994056,
64.7874727033319));
#119744=CARTESIAN_POINT('Ctrl Pts',(-9.01807743618613,89.4828855884678,
64.5257001931378));
#119745=CARTESIAN_POINT('Ctrl Pts',(-8.98110727649462,89.4597013173416,
64.3316156988844));
#119746=CARTESIAN_POINT('Ctrl Pts',(-8.94196943300685,89.4355950611352,
64.136514953116));
#119747=CARTESIAN_POINT('Ctrl Pts',(-8.90049023128382,89.4105628602268,
63.9404818633314));
#119748=CARTESIAN_POINT('Ctrl Pts',(-8.87374043729102,89.3944196802795,
63.8140608004931));
#119749=CARTESIAN_POINT('Ctrl Pts',(-8.84601675892349,89.3778915875108,
63.6872522230383));
#119750=CARTESIAN_POINT('Ctrl Pts',(-8.81727136207657,89.3609798242451,
63.5600813823535));
#119751=CARTESIAN_POINT('Ctrl Pts',(-8.80289866365312,89.3525239426123,
63.4964959620111));
#119752=CARTESIAN_POINT('Ctrl Pts',(-8.78827052166063,89.3439721398952,
63.4328199795232));
#119753=CARTESIAN_POINT('Ctrl Pts',(-8.77338087736314,89.3353248110982,
63.3690568457531));
#119754=CARTESIAN_POINT('Ctrl Pts',(-8.76139824326063,89.3283657612467,
63.317742637977));
#119755=CARTESIAN_POINT('Ctrl Pts',(-8.7498000098866,89.3216673898715,63.2687267767439));
#119756=CARTESIAN_POINT('Ctrl Pts',(-8.73810400382164,89.3149473055847,
63.219886471355));
#119757=CARTESIAN_POINT('Ctrl Pts',(-8.7352665301426,89.3133170001472,63.2080377188622));
#119758=CARTESIAN_POINT('Ctrl Pts',(-8.73242306773881,89.3116853999522,
63.19619935055));
#119759=CARTESIAN_POINT('Ctrl Pts',(-8.72956628736566,89.3100484417968,
63.1843411558216));
#119760=CARTESIAN_POINT('Ctrl Pts',(-8.67103681448578,89.2765105825837,
62.9413914725765));
#119761=CARTESIAN_POINT('Ctrl Pts',(-8.61029041858642,89.2425921176504,
62.7040929500362));
#119762=CARTESIAN_POINT('Ctrl Pts',(-8.54759953967446,89.2083683446713,
62.4724949310574));
#119763=CARTESIAN_POINT('Ctrl Pts',(-8.46136277254382,89.1612905625131,
62.1539116733774));
#119764=CARTESIAN_POINT('Ctrl Pts',(-8.37144770856337,89.1136344577483,
61.8461167293845));
#119765=CARTESIAN_POINT('Ctrl Pts',(-8.27854025383427,89.0656082931277,
61.5491975618905));
#119766=CARTESIAN_POINT('Ctrl Pts',(-8.23636727388946,89.0438080351906,
61.4144186452527));
#119767=CARTESIAN_POINT('Ctrl Pts',(-8.19357735405081,89.0219317507927,
61.2818800821673));
#119768=CARTESIAN_POINT('Ctrl Pts',(-8.15023280835573,89.,61.1515872344397));
#119769=CARTESIAN_POINT('Origin',(27.4324635166691,89.,72.98888938658));
#119770=CARTESIAN_POINT('Origin',(27.4324635166691,25.,72.98888938658));
#119771=CARTESIAN_POINT('',(-7.08823084473591,85.17401267208,58.34042080741));
#119772=CARTESIAN_POINT('Ctrl Pts',(-8.15023171813679,88.9999966970448,
61.1515839572636));
#119773=CARTESIAN_POINT('Ctrl Pts',(-8.06825403899497,88.7516349867913,
60.9051607496867));
#119774=CARTESIAN_POINT('Ctrl Pts',(-7.98615707526439,88.4947314647135,
60.6669181708804));
#119775=CARTESIAN_POINT('Ctrl Pts',(-7.90440000894433,88.2292835455461,
60.4367550592167));
#119776=CARTESIAN_POINT('Ctrl Pts',(-7.86352129457012,88.0965589975983,
60.3216729932293));
#119777=CARTESIAN_POINT('Ctrl Pts',(-7.82272705501043,87.9616983314395,
60.2086106683171));
#119778=CARTESIAN_POINT('Ctrl Pts',(-7.78207158303099,87.8247015470696,
60.0975544009398));
#119779=CARTESIAN_POINT('Ctrl Pts',(-7.76174384704127,87.7562031548847,
60.0420262672512));
#119780=CARTESIAN_POINT('Ctrl Pts',(-7.74145077759651,87.687170733147,59.9869996572717));
#119781=CARTESIAN_POINT('Ctrl Pts',(-7.72119896745376,87.6176042818565,
59.9324728049764));
#119782=CARTESIAN_POINT('Ctrl Pts',(-7.71107306238239,87.5828210562113,
59.9052093788288));
#119783=CARTESIAN_POINT('Ctrl Pts',(-7.7009574705316,87.5479043231778,59.8780708926836));
#119784=CARTESIAN_POINT('Ctrl Pts',(-7.69085300541049,87.5128540827562,
59.8510571266594));
#119785=CARTESIAN_POINT('Ctrl Pts',(-7.68580077284993,87.4953289625454,
59.8375502436472));
#119786=CARTESIAN_POINT('Ctrl Pts',(-7.68075132187224,87.4777704654875,
59.8240745407027));
#119787=CARTESIAN_POINT('Ctrl Pts',(-7.67570475343219,87.4601785915826,
59.8106299902009));
#119788=CARTESIAN_POINT('Ctrl Pts',(-7.67191982710215,87.4469846861539,
59.8005465773246));
#119789=CARTESIAN_POINT('Ctrl Pts',(-7.66813652219137,87.4337720062488,
59.7904806877004));
#119790=CARTESIAN_POINT('Ctrl Pts',(-7.66435488111403,87.4205405518672,
59.7804323096526));
#119791=CARTESIAN_POINT('Ctrl Pts',(-7.66309433408825,87.4161300670734,
59.7770828503034));
#119792=CARTESIAN_POINT('Ctrl Pts',(-7.66213046872563,87.4127561859883,
59.774522489036));
#119793=CARTESIAN_POINT('Ctrl Pts',(-7.66057379620993,87.4073028393268,
59.7703897683601));
#119794=CARTESIAN_POINT('Ctrl Pts',(-7.57292901815406,87.1002650051115,
59.5377066685055));
#119795=CARTESIAN_POINT('Ctrl Pts',(-7.48650824070021,86.7842493410492,
59.3152773725034));
#119796=CARTESIAN_POINT('Ctrl Pts',(-7.4018625872353,86.45925584714,59.1029351562491));
#119797=CARTESIAN_POINT('Ctrl Pts',(-7.31672440178161,86.1323712969823,
58.8893573734914));
#119798=CARTESIAN_POINT('Ctrl Pts',(-7.23338203755186,85.7964041334929,
58.6859841080592));
#119799=CARTESIAN_POINT('Ctrl Pts',(-7.15234364504138,85.451354356672,58.4926445767232));
#119800=CARTESIAN_POINT('Ctrl Pts',(-7.13078249036753,85.3595500725821,
58.4412044702432));
#119801=CARTESIAN_POINT('Ctrl Pts',(-7.10938414421814,85.2671028443848,
58.3904746433863));
#119802=CARTESIAN_POINT('Ctrl Pts',(-7.08815755789147,85.17401267208,58.3404519058586));
#119803=CARTESIAN_POINT('',(-7.08815755789148,25.,58.3404519058586));
#119804=CARTESIAN_POINT('Origin',(-2.02513312664091,25.,60.48888938658));
#119805=CARTESIAN_POINT('',(-6.3608745026988,75.000000198958,57.1044283173089));
#119806=CARTESIAN_POINT('Ctrl Pts',(-7.08823084473591,85.17401267208,58.34042080741));
#119807=CARTESIAN_POINT('Ctrl Pts',(-6.99794733253354,84.395480762676,58.1278617890738));
#119808=CARTESIAN_POINT('Ctrl Pts',(-6.90526175250424,83.6014255566489,
57.9461672025321));
#119809=CARTESIAN_POINT('Ctrl Pts',(-6.77559318043826,82.3870578026733,
57.7156418039018));
#119810=CARTESIAN_POINT('Ctrl Pts',(-6.73388351299471,81.9783877271923,
57.6457886604248));
#119811=CARTESIAN_POINT('Ctrl Pts',(-6.67482258874527,81.3595613777372,
57.5509009776497));
#119812=CARTESIAN_POINT('Ctrl Pts',(-6.64616402539984,81.0486928939511,
57.5059302335453));
#119813=CARTESIAN_POINT('Ctrl Pts',(-6.61448392509546,80.6834662053486,
57.4576672877489));
#119814=CARTESIAN_POINT('Ctrl Pts',(-6.60130482845044,80.5263947407648,
57.4378709142691));
#119815=CARTESIAN_POINT('Ctrl Pts',(-6.59260961427136,80.4215591552874,
57.4248692009795));
#119816=CARTESIAN_POINT('Ctrl Pts',(-6.58847590583747,80.3711606040599,
57.4187159022452));
#119817=CARTESIAN_POINT('Ctrl Pts',(-6.44248206665566,78.5687353454011,
57.2023906778076));
#119818=CARTESIAN_POINT('Ctrl Pts',(-6.36088860509349,76.7965548568022,
57.1049235783142));
#119819=CARTESIAN_POINT('Ctrl Pts',(-6.36082055131841,75.0000001903814,
57.1044704220667));
#119820=CARTESIAN_POINT('Ctrl Pts',(-6.36082055131591,75.00000012423,57.10447042205));
#119821=CARTESIAN_POINT('Ctrl Pts',(-6.36078005892346,74.1015163751048,
57.1047845229305));
#119822=CARTESIAN_POINT('Ctrl Pts',(-6.38054795665555,73.2093627488455,
57.1296675067439));
#119823=CARTESIAN_POINT('Ctrl Pts',(-6.43768908071951,71.8806274937553,
57.2055446823194));
#119824=CARTESIAN_POINT('Ctrl Pts',(-6.46127736870379,71.4392982727752,
57.2372936872005));
#119825=CARTESIAN_POINT('Ctrl Pts',(-6.50284689574204,70.7796782373796,
57.2950449971091));
#119826=CARTESIAN_POINT('Ctrl Pts',(-6.52517432368794,70.4504616687004,
57.3264550703474));
#119827=CARTESIAN_POINT('Ctrl Pts',(-6.55374105031257,70.0674142076908,
57.3676560019655));
#119828=CARTESIAN_POINT('Ctrl Pts',(-6.56650106834364,69.9034735534973,
57.386304042184));
#119829=CARTESIAN_POINT('Ctrl Pts',(-6.57512008494194,69.7942292381198,
57.3989577885545));
#119830=CARTESIAN_POINT('Ctrl Pts',(-6.57964842000668,69.7376238449638,
57.4056364990831));
#119831=CARTESIAN_POINT('Ctrl Pts',(-6.72015827311288,68.0029873888583,
57.6138146305435));
#119832=CARTESIAN_POINT('Ctrl Pts',(-6.90771375469196,66.3832968065684,
57.9152166422413));
#119833=CARTESIAN_POINT('Ctrl Pts',(-7.08826202869291,64.825987357,58.34040756172));
#119834=CARTESIAN_POINT('Ctrl Pts',(-7.03188519117291,64.48864439232,87.78728731875));
#119835=CARTESIAN_POINT('Ctrl Pts',(-6.88609751213191,65.18356633688,88.1317453461401));
#119836=CARTESIAN_POINT('Ctrl Pts',(-6.48107502800391,67.06022719065,88.90591654349));
#119837=CARTESIAN_POINT('Ctrl Pts',(-5.85681573002291,70.58880890762,89.73590455514));
#119838=CARTESIAN_POINT('Ctrl Pts',(-5.56514360048791,75.000227314,90.0489960419));
#119839=CARTESIAN_POINT('Ctrl Pts',(-5.85684197554291,79.41149656929,89.73588726852));
#119840=CARTESIAN_POINT('Ctrl Pts',(-6.48119721579791,82.94037009471,88.9057205787));
#119841=CARTESIAN_POINT('Ctrl Pts',(-6.88619858540991,84.81690451187,88.13154376415));
#119842=CARTESIAN_POINT('Ctrl Pts',(-7.03199311061991,85.51186803899,87.78703386752));
#119843=CARTESIAN_POINT('Ctrl Pts',(-7.61748537101091,65.71636999684,86.17253031082));
#119844=CARTESIAN_POINT('Ctrl Pts',(-7.51830008809391,66.33734423762,86.47777868194));
#119845=CARTESIAN_POINT('Ctrl Pts',(-7.23957881195592,68.00723840045,87.16157842494));
#119846=CARTESIAN_POINT('Ctrl Pts',(-6.79943501286791,71.12056079708,87.89696611428));
#119847=CARTESIAN_POINT('Ctrl Pts',(-6.59060414049291,75.00020008,88.17713487981));
#119848=CARTESIAN_POINT('Ctrl Pts',(-6.79945418426991,78.87970714104,87.89695030624));
#119849=CARTESIAN_POINT('Ctrl Pts',(-7.23966394454191,81.99329091746,87.16140528946));
#119850=CARTESIAN_POINT('Ctrl Pts',(-7.51836939848791,83.66307480429,86.4776005098));
#119851=CARTESIAN_POINT('Ctrl Pts',(-7.61755877579091,84.28408768177,86.17230574268));
#119852=CARTESIAN_POINT('Ctrl Pts',(-8.94180860021491,66.85942373552,84.99045086646));
#119853=CARTESIAN_POINT('Ctrl Pts',(-8.87784689601391,67.42208270543,85.27891160191));
#119854=CARTESIAN_POINT('Ctrl Pts',(-8.69724452663791,68.91837287318,85.9195538233101));
#119855=CARTESIAN_POINT('Ctrl Pts',(-8.40920338350691,71.64461634376,86.6015220059799));
#119856=CARTESIAN_POINT('Ctrl Pts',(-8.27170246170191,75.00017346889,86.8622727040301));
#119857=CARTESIAN_POINT('Ctrl Pts',(-8.40921610499591,78.3556137306,86.60150734616));
#119858=CARTESIAN_POINT('Ctrl Pts',(-8.69729997195491,81.08209623368,85.91939262999));
#119859=CARTESIAN_POINT('Ctrl Pts',(-8.87789174106491,82.57829325392,85.27874430401));
#119860=CARTESIAN_POINT('Ctrl Pts',(-8.94185593213491,83.1409906991,84.99023863948));
#119861=CARTESIAN_POINT('Ctrl Pts',(-10.7849842451049,67.728030224,84.437303609));
#119862=CARTESIAN_POINT('Ctrl Pts',(-10.7390193110219,68.25768814305,84.73418589492));
#119863=CARTESIAN_POINT('Ctrl Pts',(-10.6120633653509,69.64235959775,85.38604975076));
#119864=CARTESIAN_POINT('Ctrl Pts',(-10.4188592067689,72.07396927714,86.06464821073));
#119865=CARTESIAN_POINT('Ctrl Pts',(-10.3293343809289,75.00015189878,86.32270937777));
#119866=CARTESIAN_POINT('Ctrl Pts',(-10.4188671733959,77.92622889483,86.06463417814));
#119867=CARTESIAN_POINT('Ctrl Pts',(-10.6121014201629,80.35806705098,85.38588762974));
#119868=CARTESIAN_POINT('Ctrl Pts',(-10.7390510501279,81.74266061082,84.73401513024));
#119869=CARTESIAN_POINT('Ctrl Pts',(-10.7850182747159,82.27235965491,84.43708513232));
#119870=CARTESIAN_POINT('',(-10.5124658720316,82.2724294924703,84.5902497248058));
#119871=CARTESIAN_POINT('Origin',(-13.9921841235194,85.1739455889546,90.5667900805245));
#119872=CARTESIAN_POINT('',(-10.5124533228377,67.7276214880894,84.5902767292648));
#119873=CARTESIAN_POINT('Ctrl Pts',(-7.0883818064374,64.8259873343747,87.637422020082));
#119874=CARTESIAN_POINT('Ctrl Pts',(-7.1363573875817,64.9120414131586,87.5243405857398));
#119875=CARTESIAN_POINT('Ctrl Pts',(-7.18874895534319,64.9985784645067,
87.4123798504516));
#119876=CARTESIAN_POINT('Ctrl Pts',(-7.24554630246499,65.0853673865831,
87.3018945690997));
#119877=CARTESIAN_POINT('Ctrl Pts',(-7.30203975256059,65.1716919402222,
87.1920004447321));
#119878=CARTESIAN_POINT('Ctrl Pts',(-7.36289203093885,65.258265410166,87.0835664700366));
#119879=CARTESIAN_POINT('Ctrl Pts',(-7.42804307835773,65.3448487590915,
86.97693850846));
#119880=CARTESIAN_POINT('Ctrl Pts',(-7.4929119982875,65.4310571709469,86.8707722843422));
#119881=CARTESIAN_POINT('Ctrl Pts',(-7.56204252324817,65.5172750897001,
86.7663969043445));
#119882=CARTESIAN_POINT('Ctrl Pts',(-7.63532522931996,65.6032591451936,
86.6641439642266));
#119883=CARTESIAN_POINT('Ctrl Pts',(-7.70836562802005,65.6889588966322,
86.5622291208097));
#119884=CARTESIAN_POINT('Ctrl Pts',(-7.78553069649791,65.7744260296269,
86.4624231268371));
#119885=CARTESIAN_POINT('Ctrl Pts',(-7.86666300528646,65.8594165712825,
86.3650381068938));
#119886=CARTESIAN_POINT('Ctrl Pts',(-7.94972480666814,65.9464283622167,
86.2653370715743));
#119887=CARTESIAN_POINT('Ctrl Pts',(-8.03694480940951,66.0329402845693,
86.1681740647751));
#119888=CARTESIAN_POINT('Ctrl Pts',(-8.12810281466341,66.1186922363791,
86.0738596015708));
#119889=CARTESIAN_POINT('Ctrl Pts',(-8.21684696864524,66.2021734884584,
85.9820425722051));
#119890=CARTESIAN_POINT('Ctrl Pts',(-8.3093228698759,66.2849342013616,85.8929254695088));
#119891=CARTESIAN_POINT('Ctrl Pts',(-8.40528331540584,66.3667405844881,
85.8067664771821));
#119892=CARTESIAN_POINT('Ctrl Pts',(-8.50125644712467,66.4485577826043,
85.7205960944409));
#119893=CARTESIAN_POINT('Ctrl Pts',(-8.60071471462732,66.5294201127503,
85.6373849072769));
#119894=CARTESIAN_POINT('Ctrl Pts',(-8.70337175913268,66.6091042380695,
85.5573582535216));
#119895=CARTESIAN_POINT('Ctrl Pts',(-8.80613614014928,66.6888716797949,
85.4772479252181));
#119896=CARTESIAN_POINT('Ctrl Pts',(-8.91210559832289,66.7674581872891,
85.4003290361888));
#119897=CARTESIAN_POINT('Ctrl Pts',(-9.02095916621875,66.8446544329877,
85.3267904997943));
#119898=CARTESIAN_POINT('Ctrl Pts',(-9.13482440844064,66.9254048335946,
85.2498662113115));
#119899=CARTESIAN_POINT('Ctrl Pts',(-9.25184515284972,67.0046335847733,
85.1766412400787));
#119900=CARTESIAN_POINT('Ctrl Pts',(-9.37162211306383,67.0821226882352,
85.1072847713051));
#119901=CARTESIAN_POINT('Ctrl Pts',(-9.48691984041536,67.1567139744701,
85.0405219881085));
#119902=CARTESIAN_POINT('Ctrl Pts',(-9.60477082817847,67.2296932391917,
84.9773435825922));
#119903=CARTESIAN_POINT('Ctrl Pts',(-9.72479786071144,67.3008886557696,
84.9178564386286));
#119904=CARTESIAN_POINT('Ctrl Pts',(-9.84523065795204,67.3723247563566,
84.8581681917711));
#119905=CARTESIAN_POINT('Ctrl Pts',(-9.96785372820824,67.4419647734391,
84.8021962284059));
#119906=CARTESIAN_POINT('Ctrl Pts',(-10.0922728788578,67.5096601064754,
84.7500042148469));
#119907=CARTESIAN_POINT('Ctrl Pts',(-10.2174394678376,67.5777621139378,
84.6974986618427));
#119908=CARTESIAN_POINT('Ctrl Pts',(-10.3444232654319,67.6438958867125,
84.6488185701164));
#119909=CARTESIAN_POINT('Ctrl Pts',(-10.4728174088399,67.7079374181744,
84.6039841038095));
#119910=CARTESIAN_POINT('Ctrl Pts',(-10.4860152695413,67.714520360269,84.5993754898554));
#119911=CARTESIAN_POINT('Ctrl Pts',(-10.4992280313844,67.7210812198742,
84.5948074711202));
#119912=CARTESIAN_POINT('Ctrl Pts',(-10.5124552525542,67.7276198791653,
84.5902800433982));
#119913=CARTESIAN_POINT('',(-9.07682641225642,74.9999993273739,86.7031084130398));
#119914=CARTESIAN_POINT('Ctrl Pts',(-9.07682655323991,74.99999932735,86.70310871249));
#119915=CARTESIAN_POINT('Ctrl Pts',(-9.07712526169529,74.2289612612945,
86.7030795502179));
#119916=CARTESIAN_POINT('Ctrl Pts',(-9.14270438815803,73.4895290149526,
86.6375361780761));
#119917=CARTESIAN_POINT('Ctrl Pts',(-9.3533357059732,72.1026301973661,86.4100844515529));
#119918=CARTESIAN_POINT('Ctrl Pts',(-9.49858983167106,71.4552329230801,
86.2491187506501));
#119919=CARTESIAN_POINT('Ctrl Pts',(-9.80521029864172,70.2481781832132,
85.8621722888973));
#119920=CARTESIAN_POINT('Ctrl Pts',(-9.96584170202329,69.6878707034077,
85.6360582877567));
#119921=CARTESIAN_POINT('Ctrl Pts',(-10.2616407451189,68.6483272973767,
85.140895052477));
#119922=CARTESIAN_POINT('Ctrl Pts',(-10.397197373174,68.1684971409187,84.8713728384291));
#119923=CARTESIAN_POINT('Ctrl Pts',(-10.5124537296469,67.72762114885,84.59027742783));
#119924=CARTESIAN_POINT('Ctrl Pts',(-10.5124660110345,82.2724296180547,
84.590249978775));
#119925=CARTESIAN_POINT('Ctrl Pts',(-10.4327317076632,81.9674479999995,
84.7846994560194));
#119926=CARTESIAN_POINT('Ctrl Pts',(-10.3563178345119,81.6928249029256,
84.9429181111852));
#119927=CARTESIAN_POINT('Ctrl Pts',(-10.2548252957151,81.3329087641512,
85.1382332495564));
#119928=CARTESIAN_POINT('Ctrl Pts',(-10.2231180616871,81.2215555837217,
85.1963100913213));
#119929=CARTESIAN_POINT('Ctrl Pts',(-10.1646866545284,81.0167060472492,
85.3001066634692));
#119930=CARTESIAN_POINT('Ctrl Pts',(-10.137530445106,80.9217074846821,85.3465427226686));
#119931=CARTESIAN_POINT('Ctrl Pts',(-10.0667221831868,80.6732715679706,
85.4650986193299));
#119932=CARTESIAN_POINT('Ctrl Pts',(-10.006574102531,80.4619738935322,85.5619003025072));
#119933=CARTESIAN_POINT('Ctrl Pts',(-9.89784633786381,80.0728164008409,
85.7232268450414));
#119934=CARTESIAN_POINT('Ctrl Pts',(-9.85855483704574,79.9310487048605,
85.7796419776147));
#119935=CARTESIAN_POINT('Ctrl Pts',(-9.79567450569929,79.699751948937,85.8664855704092));
#119936=CARTESIAN_POINT('Ctrl Pts',(-9.77406187507859,79.6195447847065,
85.8958006922035));
#119937=CARTESIAN_POINT('Ctrl Pts',(-9.7407926882298,79.4944941612481,85.9400809236713));
#119938=CARTESIAN_POINT('Ctrl Pts',(-9.72394611655148,79.4307838217257,
85.962297655564));
#119939=CARTESIAN_POINT('Ctrl Pts',(-9.70395555604986,79.3543637447838,
85.9882951610611));
#119940=CARTESIAN_POINT('Ctrl Pts',(-9.69388109680604,79.3156286336885,
86.0013061847912));
#119941=CARTESIAN_POINT('Ctrl Pts',(-9.68954704161508,79.2989151157696,
86.0068841881018));
#119942=CARTESIAN_POINT('Ctrl Pts',(-9.68665408161935,79.2877476867685,
86.0106031809924));
#119943=CARTESIAN_POINT('Ctrl Pts',(-9.68488954554205,79.2809281193058,
86.0128684664986));
#119944=CARTESIAN_POINT('Ctrl Pts',(-9.5386321981269,78.715198548132,86.2004537835104));
#119945=CARTESIAN_POINT('Ctrl Pts',(-9.38875542898227,78.0813549654087,
86.3702394608437));
#119946=CARTESIAN_POINT('Ctrl Pts',(-9.15798583588213,76.6544047057943,
86.6219716832798));
#119947=CARTESIAN_POINT('Ctrl Pts',(-9.07716136819869,75.8598507335324,
86.7030186537697));
#119948=CARTESIAN_POINT('Ctrl Pts',(-9.07682655323991,74.99999932735,86.70310871249));
#119949=CARTESIAN_POINT('Ctrl Pts',(-6.95501669863192,85.15292062438,87.96390315669));
#119950=CARTESIAN_POINT('Ctrl Pts',(-7.05577166295491,85.6220618517,87.73413944146));
#119951=CARTESIAN_POINT('Ctrl Pts',(-7.30568233571291,86.70369358379,87.14935422758));
#119952=CARTESIAN_POINT('Ctrl Pts',(-7.70041279880391,88.17329653931,86.15516126834));
#119953=CARTESIAN_POINT('Ctrl Pts',(-7.99020466768391,89.12453288443,85.35040692656));
#119954=CARTESIAN_POINT('Ctrl Pts',(-8.11816676495491,89.52580380127,84.97601340087));
#119955=CARTESIAN_POINT('Ctrl Pts',(-7.61083224231891,83.87335575514,86.20258040905));
#119956=CARTESIAN_POINT('Ctrl Pts',(-7.67997552099091,84.2850156158801,
86.00281171969));
#119957=CARTESIAN_POINT('Ctrl Pts',(-7.85160010872291,85.2354085891601,
85.49468691626));
#119958=CARTESIAN_POINT('Ctrl Pts',(-8.12329981631592,86.53242756658,84.63146474731));
#119959=CARTESIAN_POINT('Ctrl Pts',(-8.32333534303391,87.37732082528,83.93205479338));
#119960=CARTESIAN_POINT('Ctrl Pts',(-8.41178168001291,87.73490557796,83.60629776158));
#119961=CARTESIAN_POINT('Ctrl Pts',(-9.10619845304691,82.6941092224099,
84.9604499123));
#119962=CARTESIAN_POINT('Ctrl Pts',(-9.14942950263491,83.05174595081,84.78078660695));
#119963=CARTESIAN_POINT('Ctrl Pts',(-9.25676191996691,83.87817202196,84.32433369085));
#119964=CARTESIAN_POINT('Ctrl Pts',(-9.42681211112791,85.00969446553,83.55043534523));
#119965=CARTESIAN_POINT('Ctrl Pts',(-9.55212940395591,85.75040379967,82.923637684635));
#119966=CARTESIAN_POINT('Ctrl Pts',(-9.6075636437929,86.06468918842,82.6315536));
#119967=CARTESIAN_POINT('Ctrl Pts',(-11.1563479441029,81.83974872807,84.47405456341));
#119968=CARTESIAN_POINT('Ctrl Pts',(-11.1843007701189,82.15710835684,84.30077826739));
#119969=CARTESIAN_POINT('Ctrl Pts',(-11.2535782960269,82.89044679757,83.86116867218));
#119970=CARTESIAN_POINT('Ctrl Pts',(-11.3627176534689,83.89507618764,83.11793696059));
#119971=CARTESIAN_POINT('Ctrl Pts',(-11.4425836537559,84.5536008381701,
82.517191706728));
#119972=CARTESIAN_POINT('Ctrl Pts',(-11.4777960592089,84.8332193001001,
82.237404575152));
#119973=CARTESIAN_POINT('',(-11.2183641640957,84.8936549215229,82.398008587887));
#119974=CARTESIAN_POINT('Origin',(-15.2667795907663,89.0000989196622,87.1935200637487));
#119975=CARTESIAN_POINT('Ctrl Pts',(-11.2183640786879,84.89365483489,82.398008486721));
#119976=CARTESIAN_POINT('Ctrl Pts',(-11.1916877670009,84.79458413089,82.505356281463));
#119977=CARTESIAN_POINT('Ctrl Pts',(-11.1374110586199,84.59363295486,82.71600930826));
#119978=CARTESIAN_POINT('Ctrl Pts',(-11.0534777220769,84.28413888454,83.01989100238));
#119979=CARTESIAN_POINT('Ctrl Pts',(-10.9672488249899,83.96689130624,83.31172338868));
#119980=CARTESIAN_POINT('Ctrl Pts',(-10.8789840138769,83.64218959052,83.59155535029));
#119981=CARTESIAN_POINT('Ctrl Pts',(-10.7889745724689,83.31029580231,83.85945164347));
#119982=CARTESIAN_POINT('Ctrl Pts',(-10.6976034072729,82.97143399976,84.11547480699));
#119983=CARTESIAN_POINT('Ctrl Pts',(-10.6052905178419,82.6257943239,84.35970336408));
#119984=CARTESIAN_POINT('Ctrl Pts',(-10.5434121371829,82.39092339779,84.51470624232));
#119985=CARTESIAN_POINT('Ctrl Pts',(-10.5124662721409,82.27243061678,84.59024934201));
#119986=CARTESIAN_POINT('Ctrl Pts',(-8.05759391320591,89.09479728929,85.11444853606));
#119987=CARTESIAN_POINT('Ctrl Pts',(-8.14537547024391,89.40820525939,84.88191214513));
#119988=CARTESIAN_POINT('Ctrl Pts',(-8.30485040107691,90.04383584284,84.32400074789));
#119989=CARTESIAN_POINT('Ctrl Pts',(-8.44711181861191,90.8927881628099,
83.3107809761201));
#119990=CARTESIAN_POINT('Ctrl Pts',(-8.49152901544292,91.61200955648,82.169824637043));
#119991=CARTESIAN_POINT('Ctrl Pts',(-8.46019247365591,92.1812155164301,
81.000788275304));
#119992=CARTESIAN_POINT('Ctrl Pts',(-8.38144499566592,92.62910837717,79.824303302778));
#119993=CARTESIAN_POINT('Ctrl Pts',(-8.28032368080192,92.9778795319,78.655233108223));
#119994=CARTESIAN_POINT('Ctrl Pts',(-8.17567642246891,93.24688018349,77.491375495357));
#119995=CARTESIAN_POINT('Ctrl Pts',(-8.0792216397619,93.45170953512,76.301792744643));
#119996=CARTESIAN_POINT('Ctrl Pts',(-8.00171757232991,93.59651183087,75.055323443605));
#119997=CARTESIAN_POINT('Ctrl Pts',(-7.95626984505191,93.67512561334,73.7508838101839));
#119998=CARTESIAN_POINT('Ctrl Pts',(-7.95303968845091,93.68056164489,72.4254389675695));
#119999=CARTESIAN_POINT('Ctrl Pts',(-7.9922643335139,93.61318488753,71.123698735184));
#120000=CARTESIAN_POINT('Ctrl Pts',(-8.06589394090391,93.47774173659,69.859266094178));
#120001=CARTESIAN_POINT('Ctrl Pts',(-8.16449146505991,93.27322272629,68.611528925018));
#120002=CARTESIAN_POINT('Ctrl Pts',(-8.27702127703391,92.99001093203,67.360147933957));
#120003=CARTESIAN_POINT('Ctrl Pts',(-8.38089851070491,92.63191641036,66.161932842428));
#120004=CARTESIAN_POINT('Ctrl Pts',(-8.45501279011491,92.20760376093,65.048518071429));
#120005=CARTESIAN_POINT('Ctrl Pts',(-8.48706795306991,91.72614549686,64.034326581107));
#120006=CARTESIAN_POINT('Ctrl Pts',(-8.46914099990891,91.1781515568,63.102992965472));
#120007=CARTESIAN_POINT('Ctrl Pts',(-8.39597121741591,90.56662317277,62.26482137247));
#120008=CARTESIAN_POINT('Ctrl Pts',(-8.26891544260791,89.90502511908,61.53563424739));
#120009=CARTESIAN_POINT('Ctrl Pts',(-8.14307662048791,89.402762062,61.0959841259));
#120010=CARTESIAN_POINT('Ctrl Pts',(-8.06733038719591,89.1295723537,60.8891544567201));
#120011=CARTESIAN_POINT('Ctrl Pts',(-8.05741235095491,89.09421528998,60.8629107499701));
#120012=CARTESIAN_POINT('Ctrl Pts',(-8.43449075962691,87.3255218789,83.72838173066));
#120013=CARTESIAN_POINT('Ctrl Pts',(-8.48604994062191,87.6134946867,83.5184247158101));
#120014=CARTESIAN_POINT('Ctrl Pts',(-8.58295769954691,88.1972243351,83.01531841742));
#120015=CARTESIAN_POINT('Ctrl Pts',(-8.67270363534791,88.97328181171,82.100770985326));
#120016=CARTESIAN_POINT('Ctrl Pts',(-8.70161580970891,89.62442872423,81.072223265241));
#120017=CARTESIAN_POINT('Ctrl Pts',(-8.68122039286491,90.13306172578,80.022995701701));
#120018=CARTESIAN_POINT('Ctrl Pts',(-8.62854234137091,90.52766929495,78.973848658753));
#120019=CARTESIAN_POINT('Ctrl Pts',(-8.55957570510291,90.83104487852,77.938493180666));
#120020=CARTESIAN_POINT('Ctrl Pts',(-8.48707215371791,91.06266767612,76.914171416008));
#120021=CARTESIAN_POINT('Ctrl Pts',(-8.4193990100769,91.23770308926,75.872605345747));
#120022=CARTESIAN_POINT('Ctrl Pts',(-8.36449198774192,91.36077676341,74.785590258427));
#120023=CARTESIAN_POINT('Ctrl Pts',(-8.33208811649991,91.42737337254,73.651011260914));
#120024=CARTESIAN_POINT('Ctrl Pts',(-8.32977951489891,91.43197300079,72.4993099454986));
#120025=CARTESIAN_POINT('Ctrl Pts',(-8.35776326441891,91.3749128398,71.367369082459));
#120026=CARTESIAN_POINT('Ctrl Pts',(-8.40999132472892,91.25987022267,70.2652675785361));
#120027=CARTESIAN_POINT('Ctrl Pts',(-8.47928365007991,91.08527122531,69.173517146296));
#120028=CARTESIAN_POINT('Ctrl Pts',(-8.55733844158391,90.84161384012,68.0726655952461));
#120029=CARTESIAN_POINT('Ctrl Pts',(-8.62816744586991,90.53014063058,67.011431700305));
#120030=CARTESIAN_POINT('Ctrl Pts',(-8.67775615445391,90.1562527277,66.018533444014));
#120031=CARTESIAN_POINT('Ctrl Pts',(-8.69874863300591,89.72661187799,65.108917233721));
#120032=CARTESIAN_POINT('Ctrl Pts',(-8.68698486500291,89.23205723218,64.270218074132));
#120033=CARTESIAN_POINT('Ctrl Pts',(-8.64030304788692,88.67534874195,63.513957909542));
#120034=CARTESIAN_POINT('Ctrl Pts',(-8.56108579733091,88.06966366952,62.85595626257));
#120035=CARTESIAN_POINT('Ctrl Pts',(-8.48488213662791,87.60848496498,62.4594052903301));
#120036=CARTESIAN_POINT('Ctrl Pts',(-8.44021087804591,87.35747749659,62.27270988017));
#120037=CARTESIAN_POINT('Ctrl Pts',(-8.43438199135791,87.32498891706,62.2490170251));
#120038=CARTESIAN_POINT('Ctrl Pts',(-9.6999844477539,85.6881588875,82.7738570047421));
#120039=CARTESIAN_POINT('Ctrl Pts',(-9.73052844606491,85.96801129276,82.5499001395251));
#120040=CARTESIAN_POINT('Ctrl Pts',(-9.78855454575391,86.53325677765,82.029291495388));
#120041=CARTESIAN_POINT('Ctrl Pts',(-9.84289992097791,87.28164187496,81.119418867505));
#120042=CARTESIAN_POINT('Ctrl Pts',(-9.86056579303691,87.90561991059,80.125117128897));
#120043=CARTESIAN_POINT('Ctrl Pts',(-9.84810420539291,88.38735477522,79.136154702713));
#120044=CARTESIAN_POINT('Ctrl Pts',(-9.8156728194649,88.7546501532,78.171273522151));
#120045=CARTESIAN_POINT('Ctrl Pts',(-9.77299215563892,89.03126880255,77.240847039094));
#120046=CARTESIAN_POINT('Ctrl Pts',(-9.72793680936391,89.23817877156,76.338821849754));
#120047=CARTESIAN_POINT('Ctrl Pts',(-9.68574655309991,89.39169056754,75.436996451304));
#120048=CARTESIAN_POINT('Ctrl Pts',(-9.65143069752991,89.4980030391201,
74.5083096496581));
#120049=CARTESIAN_POINT('Ctrl Pts',(-9.63114620088991,89.55493349031,73.5476360749947));
#120050=CARTESIAN_POINT('Ctrl Pts',(-9.62970017204091,89.55884994206,72.5758080726426));
#120051=CARTESIAN_POINT('Ctrl Pts',(-9.64722036840191,89.51012034927,71.618213001195));
#120052=CARTESIAN_POINT('Ctrl Pts',(-9.67987233041491,89.41094576649,70.6783078920771));
#120053=CARTESIAN_POINT('Ctrl Pts',(-9.72309053227491,89.2582139250901,
69.735130882087));
#120054=CARTESIAN_POINT('Ctrl Pts',(-9.77161007194191,89.0409437393701,
68.767148960646));
#120055=CARTESIAN_POINT('Ctrl Pts',(-9.81544045356291,88.75693664562,67.8132966510681));
#120056=CARTESIAN_POINT('Ctrl Pts',(-9.84597155572592,88.40888022177,66.900108010975));
#120057=CARTESIAN_POINT('Ctrl Pts',(-9.85882019495192,88.00260462959,66.045056833334));
#120058=CARTESIAN_POINT('Ctrl Pts',(-9.85161602892291,87.52992169388,65.23989706833));
#120059=CARTESIAN_POINT('Ctrl Pts',(-9.8232552816659,86.99445632834,64.498394809129));
#120060=CARTESIAN_POINT('Ctrl Pts',(-9.77545164269291,86.4097184428599,
63.837833742151));
#120061=CARTESIAN_POINT('Ctrl Pts',(-9.72987140316592,85.96304250074,63.427133769246));
#120062=CARTESIAN_POINT('Ctrl Pts',(-9.70337333602791,85.7192096835,63.228777314971));
#120063=CARTESIAN_POINT('Ctrl Pts',(-9.69991960746991,85.68763621062,63.203508570277));
#120064=CARTESIAN_POINT('Ctrl Pts',(-11.6120575244425,84.49584335857,82.433421016034));
#120065=CARTESIAN_POINT('Ctrl Pts',(-11.6408125507013,84.78644309534,82.161562454506));
#120066=CARTESIAN_POINT('Ctrl Pts',(-11.6910783687624,85.37015616451,81.554491230016));
#120067=CARTESIAN_POINT('Ctrl Pts',(-11.733908231978,86.14138350952,80.554401844931));
#120068=CARTESIAN_POINT('Ctrl Pts',(-11.746737304217,86.78429414385,79.509634128628));
#120069=CARTESIAN_POINT('Ctrl Pts',(-11.737684956696,87.27794978712,78.509867862637));
#120070=CARTESIAN_POINT('Ctrl Pts',(-11.7158054320425,87.64912935359,77.570065178083));
#120071=CARTESIAN_POINT('Ctrl Pts',(-11.6885150129063,87.92274679561,76.695714979443));
#120072=CARTESIAN_POINT('Ctrl Pts',(-11.6609630788506,88.12233512948,75.8753586663711));
#120073=CARTESIAN_POINT('Ctrl Pts',(-11.6360835214809,88.26670988172,75.078273434703));
#120074=CARTESIAN_POINT('Ctrl Pts',(-11.6164150273645,88.36443404092,74.276509733812));
#120075=CARTESIAN_POINT('Ctrl Pts',(-11.6050076721688,88.41589793954,73.460528085693));
#120076=CARTESIAN_POINT('Ctrl Pts',(-11.6042002723842,88.41941509469,72.6403035787583));
#120077=CARTESIAN_POINT('Ctrl Pts',(-11.6140353445887,88.3754368748,71.828258220239));
#120078=CARTESIAN_POINT('Ctrl Pts',(-11.632680458814,88.28456316836,71.0193957560081));
#120079=CARTESIAN_POINT('Ctrl Pts',(-11.6580421193584,88.1414636743,70.18896515103));
#120080=CARTESIAN_POINT('Ctrl Pts',(-11.6876146010148,87.93236709785,69.310782594631));
#120081=CARTESIAN_POINT('Ctrl Pts',(-11.7156592780194,87.65141820721,68.414176228036));
#120082=CARTESIAN_POINT('Ctrl Pts',(-11.7362453816865,87.29965989215,67.524646358954));
#120083=CARTESIAN_POINT('Ctrl Pts',(-11.7454264830685,86.88382894687,66.6637147582931));
#120084=CARTESIAN_POINT('Ctrl Pts',(-11.7403063415502,86.3972673145,65.8265851349111));
#120085=CARTESIAN_POINT('Ctrl Pts',(-11.7185959829517,85.84540569484,65.0298649044641));
#120086=CARTESIAN_POINT('Ctrl Pts',(-11.6797733935927,85.24264318848,64.2934889918351));
#120087=CARTESIAN_POINT('Ctrl Pts',(-11.6399483044843,84.78111485949,63.814097772889));
#120088=CARTESIAN_POINT('Ctrl Pts',(-11.6152461406276,84.5280769991699,
63.574515070347));
#120089=CARTESIAN_POINT('Ctrl Pts',(-11.6119993452045,84.49529024722,63.543845073383));
#120090=CARTESIAN_POINT('',(-11.2183629396496,84.893660453341,63.5797762185932));
#120091=CARTESIAN_POINT('Origin',(-15.2667666827029,88.99999891808,58.78411221242));
#120092=CARTESIAN_POINT('Ctrl Pts',(-11.2183626065601,84.8936601154805,
63.5797766131558));
#120093=CARTESIAN_POINT('Ctrl Pts',(-11.2440643838473,84.9878772718897,
63.6821529156428));
#120094=CARTESIAN_POINT('Ctrl Pts',(-11.2676805974612,85.0819208490858,
63.7873536467638));
#120095=CARTESIAN_POINT('Ctrl Pts',(-11.2893281573193,85.1755780930456,
63.8952945730814));
#120096=CARTESIAN_POINT('Ctrl Pts',(-11.3101899025391,85.265835543506,63.9993172028093));
#120097=CARTESIAN_POINT('Ctrl Pts',(-11.3292235684967,85.3557347030482,
64.1058853743975));
#120098=CARTESIAN_POINT('Ctrl Pts',(-11.3465346355939,85.4450809939655,
64.2149692606675));
#120099=CARTESIAN_POINT('Ctrl Pts',(-11.3652626521845,85.541740478283,64.3329819065866));
#120100=CARTESIAN_POINT('Ctrl Pts',(-11.3819749095474,85.6377537022209,
64.4539388724611));
#120101=CARTESIAN_POINT('Ctrl Pts',(-11.3968262427568,85.7329138232058,
64.5778551626002));
#120102=CARTESIAN_POINT('Ctrl Pts',(-11.4114570696226,85.8266610467739,
64.6999315958282));
#120103=CARTESIAN_POINT('Ctrl Pts',(-11.4242819467732,85.9195807517229,
64.8248806703207));
#120104=CARTESIAN_POINT('Ctrl Pts',(-11.4354420007458,86.0114518154075,
64.9527597856336));
#120105=CARTESIAN_POINT('Ctrl Pts',(-11.4469451661489,86.1061474184867,
65.0845704935991));
#120106=CARTESIAN_POINT('Ctrl Pts',(-11.4566796664678,86.1997293488902,
65.2194944701745));
#120107=CARTESIAN_POINT('Ctrl Pts',(-11.4648120393461,86.2919781405238,
65.3576488543686));
#120108=CARTESIAN_POINT('Ctrl Pts',(-11.466005961,86.3055212762758,65.3779314352756));
#120109=CARTESIAN_POINT('Ctrl Pts',(-11.4671653338274,86.3190356153124,
65.3982837068906));
#120110=CARTESIAN_POINT('Ctrl Pts',(-11.4682906666504,86.3325203963996,
65.418706104327));
#120111=CARTESIAN_POINT('Ctrl Pts',(-11.4743280332397,86.4048657196134,
65.5282714679603));
#120112=CARTESIAN_POINT('Ctrl Pts',(-11.4793359570297,86.476365120929,65.639798478805));
#120113=CARTESIAN_POINT('Ctrl Pts',(-11.4833397084349,86.546884348317,65.7532644534786));
#120114=CARTESIAN_POINT('Ctrl Pts',(-11.489870811182,86.6619185432754,65.938355350461));
#120115=CARTESIAN_POINT('Ctrl Pts',(-11.4937301361174,86.7743463826138,
66.1286040586217));
#120116=CARTESIAN_POINT('Ctrl Pts',(-11.4950660406149,86.8836703778639,
66.3240036328811));
#120117=CARTESIAN_POINT('Ctrl Pts',(-11.4954880319227,86.9182041157297,
66.3857272980393));
#120118=CARTESIAN_POINT('Ctrl Pts',(-11.4956581731352,86.9524278291927,
66.4479651528052));
#120119=CARTESIAN_POINT('Ctrl Pts',(-11.4955809788701,86.986324955698,66.5107175960102));
#120120=CARTESIAN_POINT('Ctrl Pts',(-11.4955462526203,87.0015737579076,
66.5389471155376));
#120121=CARTESIAN_POINT('Ctrl Pts',(-11.4954613695831,87.0167564257236,
66.567280552291));
#120122=CARTESIAN_POINT('Ctrl Pts',(-11.4953266861444,87.0318711487173,
66.5957173402037));
#120123=CARTESIAN_POINT('Ctrl Pts',(-11.4945472651005,87.1193409467324,
66.7602827176819));
#120124=CARTESIAN_POINT('Ctrl Pts',(-11.4920997209308,87.2045347935397,
66.9283086756899));
#120125=CARTESIAN_POINT('Ctrl Pts',(-11.4880865957529,87.2871590215378,
67.0997481823419));
#120126=CARTESIAN_POINT('Ctrl Pts',(-11.4857333004814,87.3356098413936,
67.2002802521017));
#120127=CARTESIAN_POINT('Ctrl Pts',(-11.4828419519049,87.3831763334808,
67.3019850253048));
#120128=CARTESIAN_POINT('Ctrl Pts',(-11.4794366396737,87.4297960762833,
67.4048490959103));
#120129=CARTESIAN_POINT('Ctrl Pts',(-11.478966455102,87.4362330436778,67.4190519342089));
#120130=CARTESIAN_POINT('Ctrl Pts',(-11.4784864812005,87.4426519655538,
67.4332768940122));
#120131=CARTESIAN_POINT('Ctrl Pts',(-11.4779967813246,87.4490526655553,
67.4475239062325));
#120132=CARTESIAN_POINT('Ctrl Pts',(-11.4767131552796,87.4658305036402,
67.4848688941509));
#120133=CARTESIAN_POINT('Ctrl Pts',(-11.4753627008147,87.4824831362804,
67.5223654019056));
#120134=CARTESIAN_POINT('Ctrl Pts',(-11.4739470005395,87.4990076744605,
67.5600128068845));
#120135=CARTESIAN_POINT('Ctrl Pts',(-11.4729691074825,87.5104219769358,
67.5860177011308));
#120136=CARTESIAN_POINT('Ctrl Pts',(-11.4719600740534,87.5217751589472,
67.6120945670384));
#120137=CARTESIAN_POINT('Ctrl Pts',(-11.4709204375023,87.533066255857,67.6382431522244));
#120138=CARTESIAN_POINT('Ctrl Pts',(-11.4704006192268,87.5387118043119,
67.6513174448174));
#120139=CARTESIAN_POINT('Ctrl Pts',(-11.4698731502832,87.5443418316278,
67.6644096671619));
#120140=CARTESIAN_POINT('Ctrl Pts',(-11.4693380985937,87.5499562175845,
67.6775197862553));
#120141=CARTESIAN_POINT('Ctrl Pts',(-11.4688030469042,87.5555706035413,
67.6906299053486));
#120142=CARTESIAN_POINT('Ctrl Pts',(-11.4683098506388,87.5606676415093,
67.7025765857496));
#120143=CARTESIAN_POINT('Ctrl Pts',(-11.4677102641549,87.5667523313235,
67.7169038004129));
#120144=CARTESIAN_POINT('Ctrl Pts',(-11.4593814924172,87.6512739039688,
67.915921129471));
#120145=CARTESIAN_POINT('Ctrl Pts',(-11.4496490888984,87.7310058292564,
68.116671032636));
#120146=CARTESIAN_POINT('Ctrl Pts',(-11.4388614406095,87.805888027071,68.3188814889115));
#120147=CARTESIAN_POINT('Ctrl Pts',(-11.4271990263813,87.8868423913448,
68.5374891074784));
#120148=CARTESIAN_POINT('Ctrl Pts',(-11.4143038178399,87.962128492374,68.7578051176865));
#120149=CARTESIAN_POINT('Ctrl Pts',(-11.4007134055397,88.0316981308213,
68.9795300453518));
#120150=CARTESIAN_POINT('Ctrl Pts',(-11.3979153008475,88.0460216941891,
69.0251805780055));
#120151=CARTESIAN_POINT('Ctrl Pts',(-11.3950876782912,88.0601031022114,
69.0708907961833));
#120152=CARTESIAN_POINT('Ctrl Pts',(-11.3922351522357,88.0739421860231,
69.1166580085631));
#120153=CARTESIAN_POINT('Ctrl Pts',(-11.3893241231477,88.0880650983972,
69.1633638699369));
#120154=CARTESIAN_POINT('Ctrl Pts',(-11.3863878696309,88.1019350238038,
69.2101286604569));
#120155=CARTESIAN_POINT('Ctrl Pts',(-11.3834311287561,88.1155522298085,
69.2569504871902));
#120156=CARTESIAN_POINT('Ctrl Pts',(-11.3713946747561,88.170985857788,69.447555206216));
#120157=CARTESIAN_POINT('Ctrl Pts',(-11.359019694,88.2222305320539,69.6391061576776));
#120158=CARTESIAN_POINT('Ctrl Pts',(-11.3466852494264,88.2692734167392,
69.8314251207791));
#120159=CARTESIAN_POINT('Ctrl Pts',(-11.3401069893598,88.294362534283,69.933993513501));
#120160=CARTESIAN_POINT('Ctrl Pts',(-11.3335399652676,88.3182570085292,
70.0367810142898));
#120161=CARTESIAN_POINT('Ctrl Pts',(-11.3270416342221,88.3409564268637,
70.1397668321956));
#120162=CARTESIAN_POINT('Ctrl Pts',(-11.3259511143649,88.3447657382495,
70.1570494357827));
#120163=CARTESIAN_POINT('Ctrl Pts',(-11.3248625266058,88.3485413950261,
70.1743376210178));
#120164=CARTESIAN_POINT('Ctrl Pts',(-11.3237761609902,88.3522833731834,
70.1916311965887));
#120165=CARTESIAN_POINT('Ctrl Pts',(-11.3199961900763,88.3653034544452,
70.2518035839664));
#120166=CARTESIAN_POINT('Ctrl Pts',(-11.316243007293,88.3779160421096,70.3120420658397));
#120167=CARTESIAN_POINT('Ctrl Pts',(-11.3125281520359,88.390121082633,70.3723422790808));
#120168=CARTESIAN_POINT('Ctrl Pts',(-11.3106707244074,88.3962236028947,
70.4024923857013));
#120169=CARTESIAN_POINT('Ctrl Pts',(-11.3088228770383,88.4022242340392,
70.4326579255869));
#120170=CARTESIAN_POINT('Ctrl Pts',(-11.3069860431439,88.4081229551823,
70.4628383562181));
#120171=CARTESIAN_POINT('Ctrl Pts',(-11.305608417723,88.4125469960397,70.4854736791915));
#120172=CARTESIAN_POINT('Ctrl Pts',(-11.3042369872504,88.4169137123298,
70.5081173782386));
#120173=CARTESIAN_POINT('Ctrl Pts',(-11.3028723541656,88.4212230917365,
70.5307692252172));
#120174=CARTESIAN_POINT('Ctrl Pts',(-11.3024174764707,88.4226595515387,
70.5383198408768));
#120175=CARTESIAN_POINT('Ctrl Pts',(-11.3018522650191,88.4244385126321,
70.5477220291572));
#120176=CARTESIAN_POINT('Ctrl Pts',(-11.3015100091043,88.4255133582408,
70.5534237797669));
#120177=CARTESIAN_POINT('Ctrl Pts',(-11.2940999934808,88.4487843154625,
70.6768695969599));
#120178=CARTESIAN_POINT('Ctrl Pts',(-11.2868138826341,88.4710863076103,
70.8051376168955));
#120179=CARTESIAN_POINT('Ctrl Pts',(-11.2798279157889,88.4920244103432,
70.9382902197918));
#120180=CARTESIAN_POINT('Ctrl Pts',(-11.2792804769337,88.4936651755006,
70.9487244102354));
#120181=CARTESIAN_POINT('Ctrl Pts',(-11.2787348981785,88.4952975498514,
70.9591885819396));
#120182=CARTESIAN_POINT('Ctrl Pts',(-11.2781912731431,88.4969213353755,
70.9696827577816));
#120183=CARTESIAN_POINT('Ctrl Pts',(-11.2716782339142,88.5163755145074,
71.0954109242402));
#120184=CARTESIAN_POINT('Ctrl Pts',(-11.2654434724911,88.5345988950427,
71.2254493003095));
#120185=CARTESIAN_POINT('Ctrl Pts',(-11.2596545734534,88.5512377649264,
71.3597739094034));
#120186=CARTESIAN_POINT('Ctrl Pts',(-11.2538656744158,88.5678766348101,
71.4940985184973));
#120187=CARTESIAN_POINT('Ctrl Pts',(-11.2485224827647,88.5829310285231,
71.6327098498418));
#120188=CARTESIAN_POINT('Ctrl Pts',(-11.2438200976684,88.5960223610397,
71.7755378131299));
#120189=CARTESIAN_POINT('Ctrl Pts',(-11.2436977938004,88.5963628522098,
71.7792526114736));
#120190=CARTESIAN_POINT('Ctrl Pts',(-11.2435759269761,88.5967020137289,
71.7829702735955));
#120191=CARTESIAN_POINT('Ctrl Pts',(-11.24345450108,88.5970398387411,71.7866908005161));
#120192=CARTESIAN_POINT('Ctrl Pts',(-11.2393869943549,88.6083562510806,
71.9113204615367));
#120193=CARTESIAN_POINT('Ctrl Pts',(-11.2358131384022,88.618174848028,72.0391681835653));
#120194=CARTESIAN_POINT('Ctrl Pts',(-11.2328618753785,88.6262364573018,
72.1702168260346));
#120195=CARTESIAN_POINT('Ctrl Pts',(-11.230568415286,88.6325012256408,72.2720562179402));
#120196=CARTESIAN_POINT('Ctrl Pts',(-11.2286511898399,88.6377045122625,
72.3758279368693));
#120197=CARTESIAN_POINT('Ctrl Pts',(-11.2271765482226,88.6417149897169,
72.4815052446917));
#120198=CARTESIAN_POINT('Ctrl Pts',(-11.2265151028858,88.6435138753438,
72.5289064312825));
#120199=CARTESIAN_POINT('Ctrl Pts',(-11.2259411261284,88.6450737693633,
72.5766912940998));
#120200=CARTESIAN_POINT('Ctrl Pts',(-11.2254612012353,88.6463821040866,
72.6248588574509));
#120201=CARTESIAN_POINT('Ctrl Pts',(-11.2246971786375,88.6484649243536,
72.7015398285955));
#120202=CARTESIAN_POINT('Ctrl Pts',(-11.2241715349995,88.6499103101457,
72.7791910010726));
#120203=CARTESIAN_POINT('Ctrl Pts',(-11.2239031859301,88.6506695009302,
72.8578011864478));
#120204=CARTESIAN_POINT('Ctrl Pts',(-11.2236847289416,88.6512875412042,
72.9217959839446));
#120205=CARTESIAN_POINT('Ctrl Pts',(-11.2236380328797,88.6514499822571,
72.9864269822321));
#120206=CARTESIAN_POINT('Ctrl Pts',(-11.2237716537321,88.6511304616044,
73.0516886702974));
#120207=CARTESIAN_POINT('Ctrl Pts',(-11.2238384641583,88.650970701278,73.08431951433));
#120208=CARTESIAN_POINT('Ctrl Pts',(-11.2239503458186,88.6506904384363,
73.1171080311107));
#120209=CARTESIAN_POINT('Ctrl Pts',(-11.2241082420675,88.6502863510213,
73.1500534666971));
#120210=CARTESIAN_POINT('Ctrl Pts',(-11.224187190192,88.6500843073138,73.1665261844903));
#120211=CARTESIAN_POINT('Ctrl Pts',(-11.2242776414149,88.6498513066299,
73.1830381320236));
#120212=CARTESIAN_POINT('Ctrl Pts',(-11.2243797195615,88.6495869224374,
73.199589213211));
#120213=CARTESIAN_POINT('Ctrl Pts',(-11.2244562781714,88.6493886342931,
73.2120025241015));
#120214=CARTESIAN_POINT('Ctrl Pts',(-11.2245393768795,88.6491726928545,
73.2244378476724));
#120215=CARTESIAN_POINT('Ctrl Pts',(-11.2246290659167,88.6489389176174,
73.2368951425909));
#120216=CARTESIAN_POINT('Ctrl Pts',(-11.2246589622624,88.6488609925384,
73.2410475742304));
#120217=CARTESIAN_POINT('Ctrl Pts',(-11.2246989706019,88.648756593375,73.2464457864442));
#120218=CARTESIAN_POINT('Ctrl Pts',(-11.2247209535766,88.6486991910242,
73.249359759689));
#120219=CARTESIAN_POINT('Ctrl Pts',(-11.225283848485,88.647229349411,73.3239748072662));
#120220=CARTESIAN_POINT('Ctrl Pts',(-11.2261056322508,88.6450963337197,
73.3999366369867));
#120221=CARTESIAN_POINT('Ctrl Pts',(-11.2272066924712,88.6422313440667,
73.477242239284));
#120222=CARTESIAN_POINT('Ctrl Pts',(-11.2289107443734,88.6377973531025,
73.5968839775064));
#120223=CARTESIAN_POINT('Ctrl Pts',(-11.2312844404146,88.6316110674878,
73.7197465262424));
#120224=CARTESIAN_POINT('Ctrl Pts',(-11.2343707142876,88.6234126405493,
73.8457961686285));
#120225=CARTESIAN_POINT('Ctrl Pts',(-11.2373579946079,88.6154771816569,
73.9678027148938));
#120226=CARTESIAN_POINT('Ctrl Pts',(-11.2410129804589,88.6056565218842,
74.0927953458536));
#120227=CARTESIAN_POINT('Ctrl Pts',(-11.2453674480413,88.593694657795,74.2206993317718));
#120228=CARTESIAN_POINT('Ctrl Pts',(-11.2465166159642,88.590537856131,74.2544538964924));
#120229=CARTESIAN_POINT('Ctrl Pts',(-11.2477144554566,88.5872318178545,
74.2884109730504));
#120230=CARTESIAN_POINT('Ctrl Pts',(-11.2489614488936,88.583771599319,74.3225686294004));
#120231=CARTESIAN_POINT('Ctrl Pts',(-11.2507210899968,88.5788888609015,
74.3707687356094));
#120232=CARTESIAN_POINT('Ctrl Pts',(-11.2525786286889,88.5736991271919,
74.4193682627737));
#120233=CARTESIAN_POINT('Ctrl Pts',(-11.2545339242869,88.5681887007774,
74.4683632121842));
#120234=CARTESIAN_POINT('Ctrl Pts',(-11.2597788893554,88.5534073070655,
74.5997892730114));
#120235=CARTESIAN_POINT('Ctrl Pts',(-11.2657233837533,88.5363226200422,
74.7340741379433));
#120236=CARTESIAN_POINT('Ctrl Pts',(-11.2723313215113,88.5166659063121,
74.8711490314704));
#120237=CARTESIAN_POINT('Ctrl Pts',(-11.2766411116037,88.5038455207116,
74.960551208014));
#120238=CARTESIAN_POINT('Ctrl Pts',(-11.2812327478108,88.4899305955625,
75.0511394324114));
#120239=CARTESIAN_POINT('Ctrl Pts',(-11.2860912678808,88.4748414623636,
75.1428849073909));
#120240=CARTESIAN_POINT('Ctrl Pts',(-11.2862257893454,88.4744236782919,
75.1454251327036));
#120241=CARTESIAN_POINT('Ctrl Pts',(-11.2863605151317,88.4740049937973,
75.1479662446589));
#120242=CARTESIAN_POINT('Ctrl Pts',(-11.2864954448362,88.473585407131,75.1505082428964));
#120243=CARTESIAN_POINT('Ctrl Pts',(-11.2927354812477,88.4541809617887,
75.2680669496431));
#120244=CARTESIAN_POINT('Ctrl Pts',(-11.2994101983583,88.4328491779489,
75.3875253915086));
#120245=CARTESIAN_POINT('Ctrl Pts',(-11.3064600273543,88.4094230288148,
75.5088220006582));
#120246=CARTESIAN_POINT('Ctrl Pts',(-11.3099849418523,88.3977099542478,
75.569470305233));
#120247=CARTESIAN_POINT('Ctrl Pts',(-11.3136033503414,88.3854731719582,
75.6305780279337));
#120248=CARTESIAN_POINT('Ctrl Pts',(-11.3173060099884,88.3726910795556,
75.6921366923697));
#120249=CARTESIAN_POINT('Ctrl Pts',(-11.3191573398119,88.3663000333544,
75.7229160245877));
#120250=CARTESIAN_POINT('Ctrl Pts',(-11.3210297220361,88.3597726445926,
75.7538080897276));
#120251=CARTESIAN_POINT('Ctrl Pts',(-11.3229218713195,88.3531061736548,
75.7848117696022));
#120252=CARTESIAN_POINT('Ctrl Pts',(-11.3238679459612,88.349772938186,75.8003136095394));
#120253=CARTESIAN_POINT('Ctrl Pts',(-11.3248189616925,88.3464049311971,
75.8158433529954));
#120254=CARTESIAN_POINT('Ctrl Pts',(-11.3257747517608,88.343001805872,75.8314008579735));
#120255=CARTESIAN_POINT('Ctrl Pts',(-11.3262526467949,88.3413002432095,
75.8391796104625));
#120256=CARTESIAN_POINT('Ctrl Pts',(-11.3267317353696,88.3395899009004,
75.8469653033204));
#120257=CARTESIAN_POINT('Ctrl Pts',(-11.3272119959038,88.3378707356376,
75.8547579182132));
#120258=CARTESIAN_POINT('Ctrl Pts',(-11.3275721913045,88.3365813616905,
75.8606023793827));
#120259=CARTESIAN_POINT('Ctrl Pts',(-11.3279330459287,88.3352870248267,
75.8664507341958));
#120260=CARTESIAN_POINT('Ctrl Pts',(-11.3282945501904,88.333987707079,75.8723029743145));
#120261=CARTESIAN_POINT('Ctrl Pts',(-11.328415051611,88.3335546011631,75.8742537210207));
#120262=CARTESIAN_POINT('Ctrl Pts',(-11.328446700373,88.3334409900833,75.8747664148878));
#120263=CARTESIAN_POINT('Ctrl Pts',(-11.3286562706676,88.3326867283402,
75.8781565092706));
#120264=CARTESIAN_POINT('Ctrl Pts',(-11.3299318021828,88.3280959793215,
75.8987900262188));
#120265=CARTESIAN_POINT('Ctrl Pts',(-11.3312032512804,88.3234824888511,
75.919300324912));
#120266=CARTESIAN_POINT('Ctrl Pts',(-11.3324701252167,88.3188478348224,
75.9396874271587));
#120267=CARTESIAN_POINT('Ctrl Pts',(-11.3417138987592,88.2850309797587,
76.0884423671338));
#120268=CARTESIAN_POINT('Ctrl Pts',(-11.3507102095,88.2500896582609,76.2306380982602));
#120269=CARTESIAN_POINT('Ctrl Pts',(-11.3593111082457,88.2146061164511,
76.3663372416437));
#120270=CARTESIAN_POINT('Ctrl Pts',(-11.3678698694557,88.1792964156612,
76.5013715675851));
#120271=CARTESIAN_POINT('Ctrl Pts',(-11.3760375905093,88.1434498786598,
76.6299731632938));
#120272=CARTESIAN_POINT('Ctrl Pts',(-11.3837111937169,88.1076119442604,
76.752204866115));
#120273=CARTESIAN_POINT('Ctrl Pts',(-11.3894955324291,88.0805974185279,
76.844342751195));
#120274=CARTESIAN_POINT('Ctrl Pts',(-11.3950002586896,88.0535870781357,
76.9328614131808));
#120275=CARTESIAN_POINT('Ctrl Pts',(-11.4002002457319,88.0268001149174,
77.0177900264554));
#120276=CARTESIAN_POINT('Ctrl Pts',(-11.4074220590762,87.9895980129032,
77.1357400497272));
#120277=CARTESIAN_POINT('Ctrl Pts',(-11.4140599832157,87.9528283661577,
77.246756436065));
#120278=CARTESIAN_POINT('Ctrl Pts',(-11.4201245213447,87.9169885962003,
77.3509667338731));
#120279=CARTESIAN_POINT('Ctrl Pts',(-11.4256842951077,87.8841318462804,
77.4465033876583));
#120280=CARTESIAN_POINT('Ctrl Pts',(-11.4307626968668,87.8520562688905,
77.536319548865));
#120281=CARTESIAN_POINT('Ctrl Pts',(-11.4353816424501,87.8211137905606,
77.620495962014));
#120282=CARTESIAN_POINT('Ctrl Pts',(-11.4396640130432,87.7924260398857,
77.6985385779736));
#120283=CARTESIAN_POINT('Ctrl Pts',(-11.4435520003413,87.7647119833415,
77.7717331729491));
#120284=CARTESIAN_POINT('Ctrl Pts',(-11.4470732780468,87.7382271402767,
77.8401291250943));
#120285=CARTESIAN_POINT('Ctrl Pts',(-11.4510911140927,87.7080074967171,
77.9181700366335));
#120286=CARTESIAN_POINT('Ctrl Pts',(-11.454635220842,87.6793846231229,77.9899704189875));
#120287=CARTESIAN_POINT('Ctrl Pts',(-11.4577639818982,87.6526652121703,
78.0556405133578));
#120288=CARTESIAN_POINT('Ctrl Pts',(-11.4608616360046,87.6262114524958,
78.1206576987048));
#120289=CARTESIAN_POINT('Ctrl Pts',(-11.4635523479143,87.6016234909309,
78.1796659293152));
#120290=CARTESIAN_POINT('Ctrl Pts',(-11.4658912623909,87.5791543275422,
78.2327480152614));
#120291=CARTESIAN_POINT('Ctrl Pts',(-11.4679294546614,87.5595741010736,
78.2790051564945));
#120292=CARTESIAN_POINT('Ctrl Pts',(-11.469700537194,87.5416022097708,78.3207617484193));
#120293=CARTESIAN_POINT('Ctrl Pts',(-11.4712385085672,87.5253779368081,
78.3580569175926));
#120294=CARTESIAN_POINT('Ctrl Pts',(-11.4729736282064,87.50707391949,78.4001328506095));
#120295=CARTESIAN_POINT('Ctrl Pts',(-11.4744132374809,87.4909913920126,
78.4365382864589));
#120296=CARTESIAN_POINT('Ctrl Pts',(-11.4755981275821,87.4772798964043,
78.4673325524168));
#120297=CARTESIAN_POINT('Ctrl Pts',(-11.4761496383669,87.4708978381051,
78.4816658393345));
#120298=CARTESIAN_POINT('Ctrl Pts',(-11.4766458711987,87.4650288268202,
78.4947831205361));
#120299=CARTESIAN_POINT('Ctrl Pts',(-11.4770904055706,87.4596846443869,
78.5066884459327));
#120300=CARTESIAN_POINT('Ctrl Pts',(-11.4777902013847,87.4512717145153,
78.5254300717866));
#120301=CARTESIAN_POINT('Ctrl Pts',(-11.4783617801018,87.444159905083,78.5411694292968));
#120302=CARTESIAN_POINT('Ctrl Pts',(-11.4788156162087,87.4383839488606,
78.5539203953817));
#120303=CARTESIAN_POINT('Ctrl Pts',(-11.478862614163,87.437785807545,78.5552408485389));
#120304=CARTESIAN_POINT('Ctrl Pts',(-11.4789083435246,87.4372019824694,
78.5565292493966));
#120305=CARTESIAN_POINT('Ctrl Pts',(-11.4789528140825,87.436632503541,78.5577856107489));
#120306=CARTESIAN_POINT('Ctrl Pts',(-11.4791230586672,87.4344523936397,
78.5625952809352));
#120307=CARTESIAN_POINT('Ctrl Pts',(-11.4792748598656,87.4324825592293,
78.5669354103097));
#120308=CARTESIAN_POINT('Ctrl Pts',(-11.4794087272775,87.4307244748754,
78.5708065929922));
#120309=CARTESIAN_POINT('Ctrl Pts',(-11.4794931451181,87.429615813083,78.5732477911756));
#120310=CARTESIAN_POINT('Ctrl Pts',(-11.479570424627,87.4285913534853,78.5755025046763));
#120311=CARTESIAN_POINT('Ctrl Pts',(-11.4796406605466,87.427651407994,78.5775708598944));
#120312=CARTESIAN_POINT('Ctrl Pts',(-11.4796757785065,87.4271814352483,
78.5786050375034));
#120313=CARTESIAN_POINT('Ctrl Pts',(-11.4797091350718,87.4267325904039,
78.5795926252744));
#120314=CARTESIAN_POINT('Ctrl Pts',(-11.4797407407133,87.4263049075492,
78.5805336370791));
#120315=CARTESIAN_POINT('Ctrl Pts',(-11.4797644449444,87.4259841454082,
78.5812393959326));
#120316=CARTESIAN_POINT('Ctrl Pts',(-11.4797871642159,87.4256752867183,
78.581918955712));
#120317=CARTESIAN_POINT('Ctrl Pts',(-11.4798088218001,87.4253793424745,
78.5825701418522));
#120318=CARTESIAN_POINT('Ctrl Pts',(-11.4798160409948,87.4252806943932,
78.582787203899));
#120319=CARTESIAN_POINT('Ctrl Pts',(-11.4798231963261,87.4251831259764,
78.5830021359438));
#120320=CARTESIAN_POINT('Ctrl Pts',(-11.479872260988,87.42451004271,78.584482751014));
#120321=CARTESIAN_POINT('Ctrl Pts',(-11.4874249839525,87.3208995980584,
78.8123998504856));
#120322=CARTESIAN_POINT('Ctrl Pts',(-11.4924355150551,87.2125152025755,
79.0349269405381));
#120323=CARTESIAN_POINT('Ctrl Pts',(-11.4946370187129,87.0998930412592,
79.2520671402321));
#120324=CARTESIAN_POINT('Ctrl Pts',(-11.495653919499,87.0478715222575,79.3523667872323));
#120325=CARTESIAN_POINT('Ctrl Pts',(-11.4960714579233,86.9949456985302,
79.4515163260804));
#120326=CARTESIAN_POINT('Ctrl Pts',(-11.4958632283546,86.9411677295198,
79.5495124210284));
#120327=CARTESIAN_POINT('Ctrl Pts',(-11.4953780111862,86.8158541440381,
79.7778632168492));
#120328=CARTESIAN_POINT('Ctrl Pts',(-11.4914957997757,86.685916172962,79.9999533966771));
#120329=CARTESIAN_POINT('Ctrl Pts',(-11.4839750065312,86.5521807765044,
80.2155247870291));
#120330=CARTESIAN_POINT('Ctrl Pts',(-11.4796020617359,86.4744206936407,
80.3408681861652));
#120331=CARTESIAN_POINT('Ctrl Pts',(-11.4739987782135,86.3953761413322,
80.4640069290554));
#120332=CARTESIAN_POINT('Ctrl Pts',(-11.4671164242811,86.3152043383839,
80.5848843774298));
#120333=CARTESIAN_POINT('Ctrl Pts',(-11.4653349240774,86.2944518335455,
80.6161735556695));
#120334=CARTESIAN_POINT('Ctrl Pts',(-11.4634677184249,86.2736237791093,
80.647311198389));
#120335=CARTESIAN_POINT('Ctrl Pts',(-11.4615142713744,86.2527237865284,
80.6782958810632));
#120336=CARTESIAN_POINT('Ctrl Pts',(-11.4531193396924,86.1629061434915,
80.8114524435487));
#120337=CARTESIAN_POINT('Ctrl Pts',(-11.4432055498831,86.0717204867096,
80.9417551760528));
#120338=CARTESIAN_POINT('Ctrl Pts',(-11.4316032617844,85.9793810212328,
81.069299429788));
#120339=CARTESIAN_POINT('Ctrl Pts',(-11.4201568371083,85.8882820304799,
81.1951302728799));
#120340=CARTESIAN_POINT('Ctrl Pts',(-11.4070668735547,85.7960595052786,
81.3182766347454));
#120341=CARTESIAN_POINT('Ctrl Pts',(-11.3921616073703,85.7028924985339,
81.4387882806349));
#120342=CARTESIAN_POINT('Ctrl Pts',(-11.383513739806,85.6488380505474,81.5087077802744));
#120343=CARTESIAN_POINT('Ctrl Pts',(-11.374254648862,85.5944652161075,81.5777395744793));
#120344=CARTESIAN_POINT('Ctrl Pts',(-11.3643496044752,85.5398057770639,
81.6458860450783));
#120345=CARTESIAN_POINT('Ctrl Pts',(-11.3478951255173,85.4490043071802,
81.7590924702823));
#120346=CARTESIAN_POINT('Ctrl Pts',(-11.3296580331722,85.3574121697646,
81.869858575104));
#120347=CARTESIAN_POINT('Ctrl Pts',(-11.3095049384425,85.265214975612,81.9781604293505));
#120348=CARTESIAN_POINT('Ctrl Pts',(-11.2900334836182,85.1761361753112,
82.0827991804025));
#120349=CARTESIAN_POINT('Ctrl Pts',(-11.2687732012478,85.0864920261908,
82.1851377113581));
#120350=CARTESIAN_POINT('Ctrl Pts',(-11.2456039676521,84.9964467274536,
82.2851060442717));
#120351=CARTESIAN_POINT('Ctrl Pts',(-11.2368017735046,84.9622377322241,
82.3230848868289));
#120352=CARTESIAN_POINT('Ctrl Pts',(-11.2277240798479,84.9279708452815,
82.3607211144414));
#120353=CARTESIAN_POINT('Ctrl Pts',(-11.2183644203191,84.8936551814217,
82.3980088913849));
#120354=CARTESIAN_POINT('Ctrl Pts',(-8.11806431796091,89.5255017784999,
61.00149777281));
#120355=CARTESIAN_POINT('Ctrl Pts',(-8.07086318655591,89.37752140552,60.86342605855));
#120356=CARTESIAN_POINT('Ctrl Pts',(-7.93861582162591,88.95570109335,60.48379909532));
#120357=CARTESIAN_POINT('Ctrl Pts',(-7.71230074227791,88.19557981969,59.86550662082));
#120358=CARTESIAN_POINT('Ctrl Pts',(-7.43411667443291,87.18478569849,59.14981124117));
#120359=CARTESIAN_POINT('Ctrl Pts',(-7.17722923208391,86.15427442674,58.52679204685));
#120360=CARTESIAN_POINT('Ctrl Pts',(-7.01884060245691,85.45023623237,58.15949863958));
#120361=CARTESIAN_POINT('Ctrl Pts',(-6.9550272838599,85.15303793274,58.01394630623));
#120362=CARTESIAN_POINT('Ctrl Pts',(-8.41171488046691,87.73463689348,62.37124535609));
#120363=CARTESIAN_POINT('Ctrl Pts',(-8.37908848527591,87.6027656137199,
62.25111048357));
#120364=CARTESIAN_POINT('Ctrl Pts',(-8.28772302885891,87.22733283713,61.92093632006));
#120365=CARTESIAN_POINT('Ctrl Pts',(-8.13158722580592,86.55302576817,61.38366585189));
#120366=CARTESIAN_POINT('Ctrl Pts',(-7.93999671396091,85.65985867277,60.76212250409));
#120367=CARTESIAN_POINT('Ctrl Pts',(-7.76337792118091,84.7525457800201,
60.22102525981));
#120368=CARTESIAN_POINT('Ctrl Pts',(-7.65463361368691,84.13424336598,59.90180878916));
#120369=CARTESIAN_POINT('Ctrl Pts',(-7.61084293435091,83.8734594803,59.77525700745));
#120370=CARTESIAN_POINT('Ctrl Pts',(-9.60752426142491,86.06445447859,63.346010094274));
#120371=CARTESIAN_POINT('Ctrl Pts',(-9.58707518654291,85.94854941245,63.238292826413));
#120372=CARTESIAN_POINT('Ctrl Pts',(-9.52982036816891,85.61888897018,62.94230156249));
#120373=CARTESIAN_POINT('Ctrl Pts',(-9.43202271378591,85.02829664499,62.46078605318));
#120374=CARTESIAN_POINT('Ctrl Pts',(-9.31208721147991,84.24836667598,61.90361036938));
#120375=CARTESIAN_POINT('Ctrl Pts',(-9.2015883596909,83.45823035843,61.41806587424));
#120376=CARTESIAN_POINT('Ctrl Pts',(-9.13358660596391,82.92076056578,61.13119207966));
#120377=CARTESIAN_POINT('Ctrl Pts',(-9.10620724839091,82.69420059489,61.01737706409));
#120378=CARTESIAN_POINT('Ctrl Pts',(-11.4777715891229,84.83301140937,63.740165181442));
#120379=CARTESIAN_POINT('Ctrl Pts',(-11.4647834620949,84.72988919255,63.636981566655));
#120380=CARTESIAN_POINT('Ctrl Pts',(-11.4283722400189,84.43666934708,63.353393769986));
#120381=CARTESIAN_POINT('Ctrl Pts',(-11.3659621319769,83.91175030367,62.89174862045));
#120382=CARTESIAN_POINT('Ctrl Pts',(-11.2890976560299,83.21910354186,62.35689854292));
#120383=CARTESIAN_POINT('Ctrl Pts',(-11.2179786564239,82.51780777718,61.88995855165));
#120384=CARTESIAN_POINT('Ctrl Pts',(-11.1740589850739,82.04087429545,61.61353407859));
#120385=CARTESIAN_POINT('Ctrl Pts',(-11.1563543840809,81.83983039734,61.50376655049));
#120386=CARTESIAN_POINT('',(-10.512461378761,82.2723685552168,61.3874899937114));
#120387=CARTESIAN_POINT('Ctrl Pts',(-7.08823084473591,85.17401267208,58.34042080741));
#120388=CARTESIAN_POINT('Ctrl Pts',(-7.69416668359522,84.0874238004884,
59.7681360479894));
#120389=CARTESIAN_POINT('Ctrl Pts',(-8.88950038744297,83.0746581634291,
60.8319656797966));
#120390=CARTESIAN_POINT('Ctrl Pts',(-10.5124612559679,82.2723684529,61.38749020456));
#120391=CARTESIAN_POINT('Ctrl Pts',(-10.5124593301194,82.2723668470766,
61.3874935123221));
#120392=CARTESIAN_POINT('Ctrl Pts',(-10.543406490679,82.3908668412531,61.463039940396));
#120393=CARTESIAN_POINT('Ctrl Pts',(-10.5743387198586,82.5083084983807,
61.5405397185248));
#120394=CARTESIAN_POINT('Ctrl Pts',(-10.6051932668095,82.6246361406724,
61.6199953153426));
#120395=CARTESIAN_POINT('Ctrl Pts',(-10.6136794284811,82.656630620479,61.6418485949057));
#120396=CARTESIAN_POINT('Ctrl Pts',(-10.6221596942608,82.6885410365736,
61.6638499155315));
#120397=CARTESIAN_POINT('Ctrl Pts',(-10.630632339241,82.7203668208188,61.6859993897178));
#120398=CARTESIAN_POINT('Ctrl Pts',(-10.6529650963324,82.8042553244039,
61.744382436318));
#120399=CARTESIAN_POINT('Ctrl Pts',(-10.6752448489044,82.8875557846347,
61.8037947274344));
#120400=CARTESIAN_POINT('Ctrl Pts',(-10.6974393984954,82.9702651978949,
61.864241507277));
#120401=CARTESIAN_POINT('Ctrl Pts',(-10.7280541596352,83.0843530698112,
61.9476207044518));
#120402=CARTESIAN_POINT('Ctrl Pts',(-10.7585068118979,83.1973152513338,
62.0329678195663));
#120403=CARTESIAN_POINT('Ctrl Pts',(-10.7887320955408,83.3091128864989,
62.120290979857));
#120404=CARTESIAN_POINT('Ctrl Pts',(-10.805119581979,83.3697271143666,62.1676356837782));
#120405=CARTESIAN_POINT('Ctrl Pts',(-10.821440176059,83.4299988418,62.2155610749663));
#120406=CARTESIAN_POINT('Ctrl Pts',(-10.8376847347992,83.4899230304163,
62.2640698043313));
#120407=CARTESIAN_POINT('Ctrl Pts',(-10.8514018420793,83.5405237599943,
62.3050311782514));
#120408=CARTESIAN_POINT('Ctrl Pts',(-10.8650647364673,83.5908766852467,
62.3464084936124));
#120409=CARTESIAN_POINT('Ctrl Pts',(-10.8786677705792,83.6409782943706,
62.388202788185));
#120410=CARTESIAN_POINT('Ctrl Pts',(-10.9083802716627,83.7504130060041,
62.4794922029256));
#120411=CARTESIAN_POINT('Ctrl Pts',(-10.9378074291972,83.8586494099304,
62.5727717257789));
#120412=CARTESIAN_POINT('Ctrl Pts',(-10.9668956205255,83.9656424031755,
62.668049909996));
#120413=CARTESIAN_POINT('Ctrl Pts',(-10.9832012273164,84.0256181389489,
62.7214588205074));
#120414=CARTESIAN_POINT('Ctrl Pts',(-10.9994002846426,84.0852032442459,
62.7754957722232));
#120415=CARTESIAN_POINT('Ctrl Pts',(-11.0154847086497,84.1443887642205,
62.8301624013932));
#120416=CARTESIAN_POINT('Ctrl Pts',(-11.0280938996011,84.1907865415108,
62.8730176485303));
#120417=CARTESIAN_POINT('Ctrl Pts',(-11.0406326443985,84.2369387500661,
62.9162598687448));
#120418=CARTESIAN_POINT('Ctrl Pts',(-11.053097041941,84.28284136205,62.9598897456861));
#120419=CARTESIAN_POINT('Ctrl Pts',(-11.0814611634103,84.3872978556447,
63.0591743781783));
#120420=CARTESIAN_POINT('Ctrl Pts',(-11.1094404699311,84.4904615396237,
63.1604663878809));
#120421=CARTESIAN_POINT('Ctrl Pts',(-11.1369965900705,84.5922821735986,
63.2637770344675));
#120422=CARTESIAN_POINT('Ctrl Pts',(-11.1465313985047,84.6275135572145,
63.2995239835819));
#120423=CARTESIAN_POINT('Ctrl Pts',(-11.1560154863109,84.6625839225875,
63.3355123900509));
#120424=CARTESIAN_POINT('Ctrl Pts',(-11.1654475910058,84.6974913707312,
63.3717431191836));
#120425=CARTESIAN_POINT('Ctrl Pts',(-11.1832747870022,84.7634683652532,
63.440221187465));
#120426=CARTESIAN_POINT('Ctrl Pts',(-11.2009162748768,84.8288634066181,
63.5095649076378));
#120427=CARTESIAN_POINT('Ctrl Pts',(-11.2183629288857,84.8936604424237,
63.579776231348));
#120428=CARTESIAN_POINT('Ctrl Pts',(-7.03190132372392,85.51125736721,58.19041163275));
#120429=CARTESIAN_POINT('Ctrl Pts',(-6.87538499773691,84.764785848,57.82043934909));
#120430=CARTESIAN_POINT('Ctrl Pts',(-6.44219525692591,82.7628240863,57.00605633808));
#120431=CARTESIAN_POINT('Ctrl Pts',(-5.81802729707191,79.11947090448,56.20016572671));
#120432=CARTESIAN_POINT('Ctrl Pts',(-5.65466277323091,76.16634624041,56.0230347830401));
#120433=CARTESIAN_POINT('Ctrl Pts',(-5.66377280626991,74.75743685423,56.03448007748));
#120434=CARTESIAN_POINT('Ctrl Pts',(-7.61749008897591,84.28355049495,59.80517876415));
#120435=CARTESIAN_POINT('Ctrl Pts',(-7.51101338340191,83.61653066378,59.4773129480801));
#120436=CARTESIAN_POINT('Ctrl Pts',(-7.21262854088391,81.83570965308,58.75816327819));
#120437=CARTESIAN_POINT('Ctrl Pts',(-6.77170475316191,78.62276514827,58.0435574767001));
#120438=CARTESIAN_POINT('Ctrl Pts',(-6.65471902994991,76.02576985881,57.88508025476));
#120439=CARTESIAN_POINT('Ctrl Pts',(-6.66121106065891,74.78666667996,57.89523984334));
#120440=CARTESIAN_POINT('Ctrl Pts',(-8.94180740140891,83.14051916281,60.98727660285));
#120441=CARTESIAN_POINT('Ctrl Pts',(-8.87314584653491,82.53616876214,60.67745020954));
#120442=CARTESIAN_POINT('Ctrl Pts',(-8.67972691500492,80.94176301112,60.00417372484));
#120443=CARTESIAN_POINT('Ctrl Pts',(-8.39095356268692,78.1327640109401,
59.34163189448));
#120444=CARTESIAN_POINT('Ctrl Pts',(-8.31392121950591,75.88722716423,59.1942394639501));
#120445=CARTESIAN_POINT('Ctrl Pts',(-8.31818786704791,74.81548246347,59.20357187645));
#120446=CARTESIAN_POINT('Ctrl Pts',(-10.7849819612819,82.27193645786,61.5404460002401));
#120447=CARTESIAN_POINT('Ctrl Pts',(-10.7356327836559,81.7030684661301,
61.22159696902));
#120448=CARTESIAN_POINT('Ctrl Pts',(-10.5999136901219,80.22940267629,60.53721736543));
#120449=CARTESIAN_POINT('Ctrl Pts',(-10.4069360860469,77.73082049296,59.87887468695));
#120450=CARTESIAN_POINT('Ctrl Pts',(-10.3567983965849,75.77371986632,59.73315775232));
#120451=CARTESIAN_POINT('Ctrl Pts',(-10.3596017519129,74.83910003127,59.74225885137));
#120452=CARTESIAN_POINT('',(-9.07718749310076,74.9999295892969,59.2746757754477));
#120453=CARTESIAN_POINT('Origin',(-12.2732112378425,74.9974087405852,52.48990049032));
#120454=CARTESIAN_POINT('Ctrl Pts',(-9.07715892555296,74.9999296085943,
59.2747363757378));
#120455=CARTESIAN_POINT('Ctrl Pts',(-9.0773126974457,75.1671390338749,59.2747599925217));
#120456=CARTESIAN_POINT('Ctrl Pts',(-9.08051136250148,75.3329507230294,
59.2778799903799));
#120457=CARTESIAN_POINT('Ctrl Pts',(-9.08649604199268,75.4971005092912,
59.2839019342157));
#120458=CARTESIAN_POINT('Ctrl Pts',(-9.09252940111275,75.6625854966585,
59.28997286079));
#120459=CARTESIAN_POINT('Ctrl Pts',(-9.10139410251057,75.8263814458647,
59.2989929030652));
#120460=CARTESIAN_POINT('Ctrl Pts',(-9.11282405185339,75.988270808707,59.3107655533047));
#120461=CARTESIAN_POINT('Ctrl Pts',(-9.12433014853199,76.1512386928359,
59.3226166339837));
#120462=CARTESIAN_POINT('Ctrl Pts',(-9.13843563623841,76.3122745930102,
59.3372568966318));
#120463=CARTESIAN_POINT('Ctrl Pts',(-9.15487070829253,76.4712093978363,
59.3544920669801));
#120464=CARTESIAN_POINT('Ctrl Pts',(-9.17152592658787,76.6322731193941,
59.3719581008109));
#120465=CARTESIAN_POINT('Ctrl Pts',(-9.19057342413913,76.7911791731002,
59.3920887946037));
#120466=CARTESIAN_POINT('Ctrl Pts',(-9.21173623755204,76.9478043091153,
59.4146917667016));
#120467=CARTESIAN_POINT('Ctrl Pts',(-9.22410595925357,77.0393521249075,
59.4279032650512));
#120468=CARTESIAN_POINT('Ctrl Pts',(-9.23719844767898,77.1301216611817,
59.441959603078));
#120469=CARTESIAN_POINT('Ctrl Pts',(-9.25095924211316,77.220096231446,59.4568243459834));
#120470=CARTESIAN_POINT('Ctrl Pts',(-9.27408310622116,77.371290971395,59.4818033031643));
#120471=CARTESIAN_POINT('Ctrl Pts',(-9.29906497055013,77.5203598017278,
59.5090624155835));
#120472=CARTESIAN_POINT('Ctrl Pts',(-9.32559640764624,77.667196408224,59.5384134796225));
#120473=CARTESIAN_POINT('Ctrl Pts',(-9.3361603318799,77.7256617970431,59.5501000842931));
#120474=CARTESIAN_POINT('Ctrl Pts',(-9.34696997058316,77.7837738708436,
59.5621184464069));
#120475=CARTESIAN_POINT('Ctrl Pts',(-9.35800608221007,77.8415281464316,
59.5744571510943));
#120476=CARTESIAN_POINT('Ctrl Pts',(-9.38679503195127,77.9921867292233,
59.6066440626737));
#120477=CARTESIAN_POINT('Ctrl Pts',(-9.4171239637515,78.1404072099406,59.6410096038375));
#120478=CARTESIAN_POINT('Ctrl Pts',(-9.44860318915678,78.2862101560236,
59.6773564370463));
#120479=CARTESIAN_POINT('Ctrl Pts',(-9.48147161938259,78.4384475093367,
59.7153072867217));
#120480=CARTESIAN_POINT('Ctrl Pts',(-9.5155938823567,78.5880492817324,59.7554178387944));
#120481=CARTESIAN_POINT('Ctrl Pts',(-9.55054446592392,78.7350915048918,
59.7974850672691));
#120482=CARTESIAN_POINT('Ctrl Pts',(-9.58549504949114,78.8821337280512,
59.8395522957438));
#120483=CARTESIAN_POINT('Ctrl Pts',(-9.62127390794191,79.0266168736045,
59.8835761093334));
#120484=CARTESIAN_POINT('Ctrl Pts',(-9.65747512115821,79.1686640000084,
59.9293775568926));
#120485=CARTESIAN_POINT('Ctrl Pts',(-9.69746684112778,79.3255844012029,
59.9799747193148));
#120486=CARTESIAN_POINT('Ctrl Pts',(-9.73789118088399,79.4795137713661,
60.0327000453531));
#120487=CARTESIAN_POINT('Ctrl Pts',(-9.77838369612151,79.6304418625122,
60.0873581744602));
#120488=CARTESIAN_POINT('Ctrl Pts',(-9.81982019060805,79.7848884554185,
60.1432905178108));
#120489=CARTESIAN_POINT('Ctrl Pts',(-9.86132792820858,79.9361925289671,
60.2012468526367));
#120490=CARTESIAN_POINT('Ctrl Pts',(-9.90254234074071,80.0843919819349,
60.261023922613));
#120491=CARTESIAN_POINT('Ctrl Pts',(-9.94567186427043,80.2394778220858,
60.3235786549914));
#120492=CARTESIAN_POINT('Ctrl Pts',(-9.98847998753714,80.3911641286306,
60.3881273608188));
#120493=CARTESIAN_POINT('Ctrl Pts',(-10.0305797986512,80.5395425243068,
60.4544428473998));
#120494=CARTESIAN_POINT('Ctrl Pts',(-10.0464894045399,80.5956150276066,
60.4795036072442));
#120495=CARTESIAN_POINT('Ctrl Pts',(-10.0622981738445,80.6512155761922,
60.5048167286596));
#120496=CARTESIAN_POINT('Ctrl Pts',(-10.0779863609401,80.7063506214463,
60.530370087055));
#120497=CARTESIAN_POINT('Ctrl Pts',(-10.0913829565748,80.7534320274796,
60.5521908371166));
#120498=CARTESIAN_POINT('Ctrl Pts',(-10.1046916356889,80.8001740172076,
60.5741867658278));
#120499=CARTESIAN_POINT('Ctrl Pts',(-10.1179001771309,80.8465822591748,
60.596350058545));
#120500=CARTESIAN_POINT('Ctrl Pts',(-10.1645207022042,81.0103835855924,
60.6745770413171));
#120501=CARTESIAN_POINT('Ctrl Pts',(-10.2098646468677,81.170020639701,60.7548765032126));
#120502=CARTESIAN_POINT('Ctrl Pts',(-10.253655887701,81.3255210281248,60.8369308421171));
#120503=CARTESIAN_POINT('Ctrl Pts',(-10.297629569873,81.4816692561275,60.9193270325686));
#120504=CARTESIAN_POINT('Ctrl Pts',(-10.3400377339496,81.633646677204,61.0034930253945));
#120505=CARTESIAN_POINT('Ctrl Pts',(-10.3806383769278,81.781496485306,61.0890737373057));
#120506=CARTESIAN_POINT('Ctrl Pts',(-10.4213964104706,81.9299194410991,
61.1749862074252));
#120507=CARTESIAN_POINT('Ctrl Pts',(-10.460333076907,82.0741830516942,61.2623246295904));
#120508=CARTESIAN_POINT('Ctrl Pts',(-10.4972387190891,82.2143408245832,
61.3506921725723));
#120509=CARTESIAN_POINT('Ctrl Pts',(-10.5023528212912,82.2337628189614,
61.3629374721917));
#120510=CARTESIAN_POINT('Ctrl Pts',(-10.5074279753542,82.2531059827642,
61.3752024712711));
#120511=CARTESIAN_POINT('Ctrl Pts',(-10.5124636729889,82.2723704679908,
61.3874860534033));
#120512=CARTESIAN_POINT('Ctrl Pts',(-5.66390800190791,75.24262194042,56.03434062129));
#120513=CARTESIAN_POINT('Ctrl Pts',(-5.65535143044491,73.89532137167,56.02321678452));
#120514=CARTESIAN_POINT('Ctrl Pts',(-5.80770736214291,70.97306194622,56.19025779444));
#120515=CARTESIAN_POINT('Ctrl Pts',(-6.42570231125791,67.31182980722,56.97863787701));
#120516=CARTESIAN_POINT('Ctrl Pts',(-6.87092179892391,65.25676291415,57.80972125753));
#120517=CARTESIAN_POINT('Ctrl Pts',(-7.03202707322891,64.48823711687,58.19064865432));
#120518=CARTESIAN_POINT('Ctrl Pts',(-6.66130720700991,75.21338769677,57.89513939594));
#120519=CARTESIAN_POINT('Ctrl Pts',(-6.65520853313191,74.02846944445,57.88529563077));
#120520=CARTESIAN_POINT('Ctrl Pts',(-6.76428610217291,71.45857655335,58.0346520151801));
#120521=CARTESIAN_POINT('Ctrl Pts',(-7.20118402052992,68.23053169304,58.7339902498301));
#120522=CARTESIAN_POINT('Ctrl Pts',(-7.50797933384991,66.4027178495701,
59.46781536177));
#120523=CARTESIAN_POINT('Ctrl Pts',(-7.61757435664191,65.71599759142,59.8053935093701));
#120524=CARTESIAN_POINT('Ctrl Pts',(-8.31825584846591,75.18456566475,59.2035141051799));
#120525=CARTESIAN_POINT('Ctrl Pts',(-8.31424745200392,74.15969362865,59.19451697865));
#120526=CARTESIAN_POINT('Ctrl Pts',(-8.38606591942392,71.93755190537,59.33332163781));
#120527=CARTESIAN_POINT('Ctrl Pts',(-8.67229006571891,69.11718615321,59.98168191414));
#120528=CARTESIAN_POINT('Ctrl Pts',(-8.87119397702391,67.48125880356,60.6684860693));
#120529=CARTESIAN_POINT('Ctrl Pts',(-8.94186531869191,66.85906807835,60.98748833076));
#120530=CARTESIAN_POINT('Ctrl Pts',(-10.3596548680249,75.16094109459,59.74223855301));
#120531=CARTESIAN_POINT('Ctrl Pts',(-10.3570220852529,74.26720709964,59.73351406686));
#120532=CARTESIAN_POINT('Ctrl Pts',(-10.4037867479779,72.3304649169,59.8706517777));
#120533=CARTESIAN_POINT('Ctrl Pts',(-10.5947763722079,69.82458415487,60.51456172883));
#120534=CARTESIAN_POINT('Ctrl Pts',(-10.7342345947289,68.31331830637,61.21238901141));
#120535=CARTESIAN_POINT('Ctrl Pts',(-10.7850312275449,67.72766743019,61.54067285792));
#120536=CARTESIAN_POINT('',(-10.5124868003233,67.7275732983192,61.3875216938171));
#120537=CARTESIAN_POINT('Origin',(-13.9923414084008,64.825873417259,55.411082747836));
#120538=CARTESIAN_POINT('Ctrl Pts',(-10.5124868003233,67.7275732983192,
61.3875216938171));
#120539=CARTESIAN_POINT('Ctrl Pts',(-10.4762701075093,67.8661449558079,
61.2991658162155));
#120540=CARTESIAN_POINT('Ctrl Pts',(-10.4380003201166,68.0087788126902,
61.211774700065));
#120541=CARTESIAN_POINT('Ctrl Pts',(-10.3978879892869,68.1555292889392,
61.1257495553478));
#120542=CARTESIAN_POINT('Ctrl Pts',(-10.3579054434168,68.3018049484868,
61.0400027482313));
#120543=CARTESIAN_POINT('Ctrl Pts',(-10.3160920568659,68.4521709674743,
60.9556128504399));
#120544=CARTESIAN_POINT('Ctrl Pts',(-10.2726907444907,68.6066715326339,
60.8729398329561));
#120545=CARTESIAN_POINT('Ctrl Pts',(-10.2295860562707,68.7601161712075,
60.7908318401829));
#120546=CARTESIAN_POINT('Ctrl Pts',(-10.1849149375519,68.9176394274009,
60.7104170559603));
#120547=CARTESIAN_POINT('Ctrl Pts',(-10.1389518423473,69.0792695620243,
60.632015160386));
#120548=CARTESIAN_POINT('Ctrl Pts',(-10.1318974355681,69.1040765231818,
60.6199820529292));
#120549=CARTESIAN_POINT('Ctrl Pts',(-10.1248126674201,69.1289801903125,
60.6079963024182));
#120550=CARTESIAN_POINT('Ctrl Pts',(-10.1176986096817,69.1539806243396,
60.5960590019341));
#120551=CARTESIAN_POINT('Ctrl Pts',(-10.0996746444948,69.2173209807338,
60.5658150123203));
#120552=CARTESIAN_POINT('Ctrl Pts',(-10.0814630365437,69.2812783888663,
60.5358835999103));
#120553=CARTESIAN_POINT('Ctrl Pts',(-10.0630957245031,69.3458681631611,
60.5062844575174));
#120554=CARTESIAN_POINT('Ctrl Pts',(-10.0218973231987,69.4907448569128,
60.4398927425039));
#120555=CARTESIAN_POINT('Ctrl Pts',(-9.97991359072972,69.6388059609115,
60.3751724378893));
#120556=CARTESIAN_POINT('Ctrl Pts',(-9.93751542809077,69.7901601866326,
60.312340052335));
#120557=CARTESIAN_POINT('Ctrl Pts',(-9.89646721486002,69.9366953226874,
60.2515082379473));
#120558=CARTESIAN_POINT('Ctrl Pts',(-9.85503061526349,70.0863176266317,
60.1924459147403));
#120559=CARTESIAN_POINT('Ctrl Pts',(-9.81356881089885,70.2390859076572,
60.1353552330375));
#120560=CARTESIAN_POINT('Ctrl Pts',(-9.77350524883942,70.3867022885978,
60.0801898560245));
#120561=CARTESIAN_POINT('Ctrl Pts',(-9.73341830512795,70.5372562897347,
60.0268653562765));
#120562=CARTESIAN_POINT('Ctrl Pts',(-9.69365921584859,70.6907584294202,
59.9755704936241));
#120563=CARTESIAN_POINT('Ctrl Pts',(-9.6815232341654,70.7376131031394,59.9599133564795));
#120564=CARTESIAN_POINT('Ctrl Pts',(-9.66941796029569,70.7847421335854,
59.9444453679735));
#120565=CARTESIAN_POINT('Ctrl Pts',(-9.65735380374282,70.832144941498,59.9291720205939));
#120566=CARTESIAN_POINT('Ctrl Pts',(-9.62200662870135,70.9710320109257,
59.8844221302116));
#120567=CARTESIAN_POINT('Ctrl Pts',(-9.58703153567298,71.1122271274692,
59.8413601076449));
#120568=CARTESIAN_POINT('Ctrl Pts',(-9.55281926379787,71.2558507181445,
59.8001562974858));
#120569=CARTESIAN_POINT('Ctrl Pts',(-9.51916731788748,71.3971220526677,
59.7596273201692));
#120570=CARTESIAN_POINT('Ctrl Pts',(-9.48625349670778,71.54074326782,59.7208963190959));
#120571=CARTESIAN_POINT('Ctrl Pts',(-9.45446673383467,71.6867871682261,
59.6841468622814));
#120572=CARTESIAN_POINT('Ctrl Pts',(-9.42326249685992,71.8301546603858,
59.648070877957));
#120573=CARTESIAN_POINT('Ctrl Pts',(-9.3931445162145,71.9758570705251,59.6139046705913));
#120574=CARTESIAN_POINT('Ctrl Pts',(-9.3644957399514,72.1239188889196,59.5818403151953));
#120575=CARTESIAN_POINT('Ctrl Pts',(-9.35416809263895,72.1772939520209,
59.5702813798051));
#120576=CARTESIAN_POINT('Ctrl Pts',(-9.34403150850522,72.2309751908338,
59.5589957504543));
#120577=CARTESIAN_POINT('Ctrl Pts',(-9.33410436362879,72.2849622223357,
59.5479929451075));
#120578=CARTESIAN_POINT('Ctrl Pts',(-9.3074741014996,72.4297862194032,59.5184771483512));
#120579=CARTESIAN_POINT('Ctrl Pts',(-9.28235075410872,72.5768144578516,
59.4909958965004));
#120580=CARTESIAN_POINT('Ctrl Pts',(-9.25904207989478,72.7259503851478,
59.4657366079965));
#120581=CARTESIAN_POINT('Ctrl Pts',(-9.25620454146715,72.7441058117825,
59.4626616067705));
#120582=CARTESIAN_POINT('Ctrl Pts',(-9.25339390160451,72.7622924121674,
59.4596195469236));
#120583=CARTESIAN_POINT('Ctrl Pts',(-9.25061071951314,72.7805099599108,
59.4566107760049));
#120584=CARTESIAN_POINT('Ctrl Pts',(-9.22695251543498,72.9353666843967,
59.4310349731716));
#120585=CARTESIAN_POINT('Ctrl Pts',(-9.2052828960784,73.0925588459421,59.407856783846));
#120586=CARTESIAN_POINT('Ctrl Pts',(-9.18587503647428,73.2520001394406,
59.3872619276458));
#120587=CARTESIAN_POINT('Ctrl Pts',(-9.16679028054398,73.4087870409176,
59.3670099363382));
#120588=CARTESIAN_POINT('Ctrl Pts',(-9.14989271692039,73.5677489173827,
59.349256203791));
#120589=CARTESIAN_POINT('Ctrl Pts',(-9.13544671220291,73.7287551183742,
59.3341896287712));
#120590=CARTESIAN_POINT('Ctrl Pts',(-9.1211136461013,73.8885025756618,59.3192408439752));
#120591=CARTESIAN_POINT('Ctrl Pts',(-9.10919408187488,74.050262646377,59.3069375774147));
#120592=CARTESIAN_POINT('Ctrl Pts',(-9.0999490525663,74.2138576301041,59.2974733318929));
#120593=CARTESIAN_POINT('Ctrl Pts',(-9.09078225483746,74.3760682705711,
59.2880891729618));
#120594=CARTESIAN_POINT('Ctrl Pts',(-9.08424506901794,74.5400829676146,
59.28149640993));
#120595=CARTESIAN_POINT('Ctrl Pts',(-9.08059270014877,74.7056776060466,
59.2778893465346));
#120596=CARTESIAN_POINT('Ctrl Pts',(-9.07844102510663,74.8032323337834,
59.2757643617476));
#120597=CARTESIAN_POINT('Ctrl Pts',(-9.07729055840808,74.9013344250172,
59.2746756845705));
#120598=CARTESIAN_POINT('Ctrl Pts',(-9.07719325348408,74.9999295853934,
59.2746634979996));
#120599=CARTESIAN_POINT('Ctrl Pts',(-6.95350273443992,64.85427978905,58.01030135259));
#120600=CARTESIAN_POINT('Ctrl Pts',(-7.13804274350491,63.99524524915,58.4306382535));
#120601=CARTESIAN_POINT('Ctrl Pts',(-7.57336514742491,62.21958654223,59.46854577467));
#120602=CARTESIAN_POINT('Ctrl Pts',(-8.29958740449491,59.85356795294,61.46379788794));
#120603=CARTESIAN_POINT('Ctrl Pts',(-9.03398262523491,57.8394554497201,
63.966105684766));
#120604=CARTESIAN_POINT('Ctrl Pts',(-9.65355624003791,56.34001186882,66.835457200394));
#120605=CARTESIAN_POINT('Ctrl Pts',(-10.0603100074489,55.43622922579,69.955066301403));
#120606=CARTESIAN_POINT('Ctrl Pts',(-10.1459643513009,55.25249740592,72.1222089702131));
#120607=CARTESIAN_POINT('Ctrl Pts',(-10.1403726637939,55.26506242224,73.1850262950981));
#120608=CARTESIAN_POINT('Ctrl Pts',(-7.65862076439791,66.22813057212,59.90322577706));
#120609=CARTESIAN_POINT('Ctrl Pts',(-7.78097032738291,65.48218511246,60.2645947192301));
#120610=CARTESIAN_POINT('Ctrl Pts',(-8.06993590988691,63.93605519502,61.15578231356));
#120611=CARTESIAN_POINT('Ctrl Pts',(-8.55437878141292,61.85463455847,62.86927844546));
#120612=CARTESIAN_POINT('Ctrl Pts',(-9.04755438821391,60.05347845777,65.030787886569));
#120613=CARTESIAN_POINT('Ctrl Pts',(-9.46704764745591,58.68556152658,67.535143565041));
#120614=CARTESIAN_POINT('Ctrl Pts',(-9.74468998856591,57.84498149326,70.289989823668));
#120615=CARTESIAN_POINT('Ctrl Pts',(-9.80338789027092,57.6722837132601,
72.2180181904323));
#120616=CARTESIAN_POINT('Ctrl Pts',(-9.79958208940392,57.68401165871,73.1633534773191));
#120617=CARTESIAN_POINT('Ctrl Pts',(-9.31846800108191,67.47735678569,61.18858040015));
#120618=CARTESIAN_POINT('Ctrl Pts',(-9.39099275510391,66.8364283808701,
61.51211508092));
#120619=CARTESIAN_POINT('Ctrl Pts',(-9.56233860701091,65.50564909822,62.30810424059));
#120620=CARTESIAN_POINT('Ctrl Pts',(-9.84998217425491,63.7004966011401,
63.835139422207));
#120621=CARTESIAN_POINT('Ctrl Pts',(-10.1433419235899,62.1191058317,65.7671445554511));
#120622=CARTESIAN_POINT('Ctrl Pts',(-10.3934232529189,60.90047284578,68.021797610286));
#120623=CARTESIAN_POINT('Ctrl Pts',(-10.5592976252989,60.14127553959,70.5237615137681));
#120624=CARTESIAN_POINT('Ctrl Pts',(-10.5944027227179,59.98414788629,72.2848823047987));
#120625=CARTESIAN_POINT('Ctrl Pts',(-10.5921307252349,59.9947625292,73.1482290672144));
#120626=CARTESIAN_POINT('Ctrl Pts',(-11.5725330395007,68.33063207667,61.58719193961));
#120627=CARTESIAN_POINT('Ctrl Pts',(-11.618420347605,67.76383946612,61.90224348891));
#120628=CARTESIAN_POINT('Ctrl Pts',(-11.7264300397956,66.58745946769,62.67523238084));
#120629=CARTESIAN_POINT('Ctrl Pts',(-11.9049983137748,64.99024109106,64.151600128689));
#120630=CARTESIAN_POINT('Ctrl Pts',(-12.0833450737449,63.5876925334,66.015242312359));
#120631=CARTESIAN_POINT('Ctrl Pts',(-12.2314784131961,62.50367698227,68.189720251468));
#120632=CARTESIAN_POINT('Ctrl Pts',(-12.3272037779371,61.82636655584,70.605607204909));
#120633=CARTESIAN_POINT('Ctrl Pts',(-12.3472039606322,61.68596335411,72.308278726365));
#120634=CARTESIAN_POINT('Ctrl Pts',(-12.3458805480338,61.69543026713,73.1429380190955));
#120635=CARTESIAN_POINT('',(-12.1331989796159,61.4797180052465,72.9888456300652));
#120636=CARTESIAN_POINT('Origin',(-17.5675192547456,56.310652416732,72.9886930857116));
#120637=CARTESIAN_POINT('Ctrl Pts',(-12.1332079421933,61.4797094802272,
72.9888456275718));
#120638=CARTESIAN_POINT('Ctrl Pts',(-12.1331653467128,61.4797185453445,
72.8047456110304));
#120639=CARTESIAN_POINT('Ctrl Pts',(-12.1322831197896,61.4832907140384,
72.6175747076454));
#120640=CARTESIAN_POINT('Ctrl Pts',(-12.130481030127,61.4907627280311,72.4274543646988));
#120641=CARTESIAN_POINT('Ctrl Pts',(-12.1287809460169,61.4978117958562,
72.2480956009586));
#120642=CARTESIAN_POINT('Ctrl Pts',(-12.1262621768532,61.5083318721226,
72.066111858343));
#120643=CARTESIAN_POINT('Ctrl Pts',(-12.1228518473085,61.5226310275087,
71.881646620849));
#120644=CARTESIAN_POINT('Ctrl Pts',(-12.1195127607835,61.5366314683583,
71.7010349289953));
#120645=CARTESIAN_POINT('Ctrl Pts',(-12.1153189970978,61.5542547474794,
71.5180441111482));
#120646=CARTESIAN_POINT('Ctrl Pts',(-12.1101965797031,61.5758140946132,
71.3328517672573));
#120647=CARTESIAN_POINT('Ctrl Pts',(-12.1052203638473,61.5967581053765,
71.1529450929197));
#120648=CARTESIAN_POINT('Ctrl Pts',(-12.0993677620032,61.6214167411873,
70.9709606179531));
#120649=CARTESIAN_POINT('Ctrl Pts',(-12.0925653862056,61.6500998120332,
70.7871047536805));
#120650=CARTESIAN_POINT('Ctrl Pts',(-12.0907794318631,61.6576305125496,
70.7388336512086));
#120651=CARTESIAN_POINT('Ctrl Pts',(-12.0889279767352,61.6654387473065,
70.6904337965565));
#120652=CARTESIAN_POINT('Ctrl Pts',(-12.0870096244634,61.6735303884131,
70.641909464666));
#120653=CARTESIAN_POINT('Ctrl Pts',(-12.079323095454,61.7059522928846,70.4474802713318));
#120654=CARTESIAN_POINT('Ctrl Pts',(-12.070562765951,61.742923132194,70.2510489263372));
#120655=CARTESIAN_POINT('Ctrl Pts',(-12.060658636014,61.7847569874742,70.0528399176));
#120656=CARTESIAN_POINT('Ctrl Pts',(-12.0567749820864,61.8011610752028,
69.9751172705682));
#120657=CARTESIAN_POINT('Ctrl Pts',(-12.05271542204,61.8183130693951,69.8971218150545));
#120658=CARTESIAN_POINT('Ctrl Pts',(-12.0484756078765,61.8362325226126,
69.8188692114161));
#120659=CARTESIAN_POINT('Ctrl Pts',(-12.0380219491557,61.8804146120088,
69.6259300917068));
#120660=CARTESIAN_POINT('Ctrl Pts',(-12.0264752882927,61.9292585199403,
69.4314424213465));
#120661=CARTESIAN_POINT('Ctrl Pts',(-12.0137349078255,61.9830342790126,
69.2356607295991));
#120662=CARTESIAN_POINT('Ctrl Pts',(-12.0013924645638,62.0351303884588,
69.0459941471689));
#120663=CARTESIAN_POINT('Ctrl Pts',(-11.9879297021071,62.0918551359694,
68.8551130122815));
#120664=CARTESIAN_POINT('Ctrl Pts',(-11.9732513573392,62.1534679657069,
68.663294660096));
#120665=CARTESIAN_POINT('Ctrl Pts',(-11.9607095382935,62.2061126592121,
68.499396679716));
#120666=CARTESIAN_POINT('Ctrl Pts',(-11.9472801962284,62.2623262340416,
68.3348150750062));
#120667=CARTESIAN_POINT('Ctrl Pts',(-11.9329017126591,62.3222785805898,
68.1697519096999));
#120668=CARTESIAN_POINT('Ctrl Pts',(-11.9309069607861,62.3305958732299,
68.1468524115318));
#120669=CARTESIAN_POINT('Ctrl Pts',(-11.9288939379843,62.3389851359816,
68.1239436899144));
#120670=CARTESIAN_POINT('Ctrl Pts',(-11.9268625115437,62.3474467822139,
68.1010261931419));
#120671=CARTESIAN_POINT('Ctrl Pts',(-11.9083411270276,62.4245952333618,
67.8920775640391));
#120672=CARTESIAN_POINT('Ctrl Pts',(-11.888269059637,62.5077412898931,67.6823915702289));
#120673=CARTESIAN_POINT('Ctrl Pts',(-11.8665135228292,62.5971460438744,
67.4723866003536));
#120674=CARTESIAN_POINT('Ctrl Pts',(-11.8580218723687,62.6320426279955,
67.3904171773559));
#120675=CARTESIAN_POINT('Ctrl Pts',(-11.8492737462824,62.6678927592649,
67.3083997082421));
#120676=CARTESIAN_POINT('Ctrl Pts',(-11.8402612660364,62.704712083059,67.2263612479458));
#120677=CARTESIAN_POINT('Ctrl Pts',(-11.8242100767523,62.7702871433535,
67.0802510963719));
#120678=CARTESIAN_POINT('Ctrl Pts',(-11.8073196299173,62.8389358061581,
66.9340732660924));
#120679=CARTESIAN_POINT('Ctrl Pts',(-11.7895406122778,62.9107434320246,
66.7879889495863));
#120680=CARTESIAN_POINT('Ctrl Pts',(-11.780651103458,62.9466472449579,66.7149467913332));
#120681=CARTESIAN_POINT('Ctrl Pts',(-11.7715393875097,62.9833408625202,
66.641928037025));
#120682=CARTESIAN_POINT('Ctrl Pts',(-11.7621989800699,63.0208346945652,
66.5689541969016));
#120683=CARTESIAN_POINT('Ctrl Pts',(-11.75752877635,63.0395816105878,66.5324672768399));
#120684=CARTESIAN_POINT('Ctrl Pts',(-11.7528013955934,63.058528584409,66.495991587103));
#120685=CARTESIAN_POINT('Ctrl Pts',(-11.7480160038192,63.0776769209298,
66.459529867771));
#120686=CARTESIAN_POINT('Ctrl Pts',(-11.7447595858139,63.0907071994858,
66.4347179808998));
#120687=CARTESIAN_POINT('Ctrl Pts',(-11.7413647584787,63.104273765333,66.4090764859645));
#120688=CARTESIAN_POINT('Ctrl Pts',(-11.738058747514,63.117474192884,66.3843141959879));
#120689=CARTESIAN_POINT('Ctrl Pts',(-11.7365064885483,63.1236721402702,
66.3726876505715));
#120690=CARTESIAN_POINT('Ctrl Pts',(-11.7349738984648,63.129788732834,66.3612544971653));
#120691=CARTESIAN_POINT('Ctrl Pts',(-11.7334849449445,63.1357273297451,
66.3501893914605));
#120692=CARTESIAN_POINT('Ctrl Pts',(-11.7170783789754,63.2011638800877,
66.228264573638));
#120693=CARTESIAN_POINT('Ctrl Pts',(-11.7001633859446,63.2684475221823,
66.1073814441102));
#120694=CARTESIAN_POINT('Ctrl Pts',(-11.6827276781987,63.3375315176884,
65.9876235892416));
#120695=CARTESIAN_POINT('Ctrl Pts',(-11.6455787104538,63.484723656841,65.7324644209088));
#120696=CARTESIAN_POINT('Ctrl Pts',(-11.6060658609039,63.6400899127347,
65.4824168542107));
#120697=CARTESIAN_POINT('Ctrl Pts',(-11.5641140464249,63.8031665788657,
65.2380129164019));
#120698=CARTESIAN_POINT('Ctrl Pts',(-11.5362719517495,63.9113954131643,
65.0758097397329));
#120699=CARTESIAN_POINT('Ctrl Pts',(-11.5073555995864,64.0230198042498,
64.9160914069143));
#120700=CARTESIAN_POINT('Ctrl Pts',(-11.4773432659756,64.1379005967349,
64.7590012547552));
#120701=CARTESIAN_POINT('Ctrl Pts',(-11.4344204221028,64.3022000605408,
64.5343350837563));
#120702=CARTESIAN_POINT('Ctrl Pts',(-11.3892616495029,64.4731513924225,
64.3150645575879));
#120703=CARTESIAN_POINT('Ctrl Pts',(-11.3418451116646,64.6503209328055,
64.1016187216834));
#120704=CARTESIAN_POINT('Ctrl Pts',(-11.3359829404079,64.672224644771,64.075230121816));
#120705=CARTESIAN_POINT('Ctrl Pts',(-11.330086268261,64.6942233854544,64.0489304810118));
#120706=CARTESIAN_POINT('Ctrl Pts',(-11.3241550735596,64.7163164325531,
64.0227202842263));
#120707=CARTESIAN_POINT('Ctrl Pts',(-11.297202057071,64.8167134508116,63.903613780109));
#120708=CARTESIAN_POINT('Ctrl Pts',(-11.269540961379,64.9190583895597,63.7863595421992));
#120709=CARTESIAN_POINT('Ctrl Pts',(-11.2411950260713,65.0232761843867,
63.6710239744486));
#120710=CARTESIAN_POINT('Ctrl Pts',(-11.2270220584174,65.0753850818002,
63.6133561905732));
#120711=CARTESIAN_POINT('Ctrl Pts',(-11.2126779701479,65.1279620983969,
63.5561680134618));
#120712=CARTESIAN_POINT('Ctrl Pts',(-11.1981661560224,65.180997423307,63.4994671916645));
#120713=CARTESIAN_POINT('Ctrl Pts',(-11.1909102489597,65.2075150857621,
63.4711167807659));
#120714=CARTESIAN_POINT('Ctrl Pts',(-11.1836124156156,65.2341473198062,
63.4428882037445));
#120715=CARTESIAN_POINT('Ctrl Pts',(-11.1762731100198,65.260892870629,63.4147823938254));
#120716=CARTESIAN_POINT('Ctrl Pts',(-11.1726034572219,65.2742656460403,
63.4007294888658));
#120717=CARTESIAN_POINT('Ctrl Pts',(-11.1689234366739,65.2876667503186,
63.386707275337));
#120718=CARTESIAN_POINT('Ctrl Pts',(-11.1652331068892,65.3010960251005,
63.372715867342));
#120719=CARTESIAN_POINT('Ctrl Pts',(-11.1624653595506,65.3111679811869,
63.3622223113457));
#120720=CARTESIAN_POINT('Ctrl Pts',(-11.1596918132918,65.3212557831551,
63.3517460834332));
#120721=CARTESIAN_POINT('Ctrl Pts',(-11.1569124932258,65.3313593638241,
63.3412872311077));
#120722=CARTESIAN_POINT('Ctrl Pts',(-11.1559860532039,65.3347272240471,
63.3378009469992));
#120723=CARTESIAN_POINT('Ctrl Pts',(-11.1547187447784,65.3393332299145,
63.3330394727056));
#120724=CARTESIAN_POINT('Ctrl Pts',(-11.1541312495045,65.3414682015608,
63.3308341723723));
#120725=CARTESIAN_POINT('Ctrl Pts',(-11.1294971591335,65.4309890654857,
63.2383643770943));
#120726=CARTESIAN_POINT('Ctrl Pts',(-11.1033515358283,65.5265230289392,
63.1425216544724));
#120727=CARTESIAN_POINT('Ctrl Pts',(-11.07557230204,65.6283774805403,63.0438117051595));
#120728=CARTESIAN_POINT('Ctrl Pts',(-11.0477429559631,65.7304156722586,
62.9449236882476));
#120729=CARTESIAN_POINT('Ctrl Pts',(-11.0182738064181,65.8387973476537,
62.8431580967832));
#120730=CARTESIAN_POINT('Ctrl Pts',(-10.9870532157423,65.9538609854524,
62.7390650122299));
#120731=CARTESIAN_POINT('Ctrl Pts',(-10.9608634381172,66.050383537443,62.6517452441618));
#120732=CARTESIAN_POINT('Ctrl Pts',(-10.9334412612304,66.1516086733662,
62.5627883573703));
#120733=CARTESIAN_POINT('Ctrl Pts',(-10.9047293596841,66.2577508851825,
62.4725416655751));
#120734=CARTESIAN_POINT('Ctrl Pts',(-10.8975383262697,66.2843347110785,
62.4499389488866));
#120735=CARTESIAN_POINT('Ctrl Pts',(-10.8902664379593,66.3112270383585,
62.4272554276655));
#120736=CARTESIAN_POINT('Ctrl Pts',(-10.8829128118355,66.3384311136375,
62.4044967295375));
#120737=CARTESIAN_POINT('Ctrl Pts',(-10.8469819514119,66.4713540846117,
62.2932945019423));
#120738=CARTESIAN_POINT('Ctrl Pts',(-10.80907714389,66.6117098375458,62.1802881568853));
#120739=CARTESIAN_POINT('Ctrl Pts',(-10.7692527638807,66.7598505141739,
62.066267766513));
#120740=CARTESIAN_POINT('Ctrl Pts',(-10.7300594413498,66.9056437523284,
61.9540541442562));
#120741=CARTESIAN_POINT('Ctrl Pts',(-10.6890064797408,67.0589777669139,
61.8408584917643));
#120742=CARTESIAN_POINT('Ctrl Pts',(-10.646176795151,67.2201664659931,61.7274685250017));
#120743=CARTESIAN_POINT('Ctrl Pts',(-10.6058295911207,67.3720123969497,
61.6206508314378));
#120744=CARTESIAN_POINT('Ctrl Pts',(-10.5639055145783,67.530829139225,61.5136609766));
#120745=CARTESIAN_POINT('Ctrl Pts',(-10.5205053048556,67.6968536294708,
61.4071851455753));
#120746=CARTESIAN_POINT('Ctrl Pts',(-10.517834979129,67.7070687752127,61.4006339064762));
#120747=CARTESIAN_POINT('Ctrl Pts',(-10.5151590760853,67.7173111980251,
61.3940846217744));
#120748=CARTESIAN_POINT('Ctrl Pts',(-10.5124776235678,67.7275809493603,
61.3875374546355));
#120749=CARTESIAN_POINT('Ctrl Pts',(-10.1403245269799,55.26504566043,72.7925531866283));
#120750=CARTESIAN_POINT('Ctrl Pts',(-10.1450666807169,55.25428818104,73.6993150005103));
#120751=CARTESIAN_POINT('Ctrl Pts',(-10.0787320679299,55.39759073255,75.731249626262));
#120752=CARTESIAN_POINT('Ctrl Pts',(-9.7171468928169,56.19403365364,78.782525259709));
#120753=CARTESIAN_POINT('Ctrl Pts',(-9.09680907897791,57.67747381634,81.773917000605));
#120754=CARTESIAN_POINT('Ctrl Pts',(-8.34088152741291,59.72748177467,84.39459302725));
#120755=CARTESIAN_POINT('Ctrl Pts',(-7.59054532717091,62.15234847022,86.46774807429));
#120756=CARTESIAN_POINT('Ctrl Pts',(-7.14211997123491,63.97655318543,87.53799401565));
#120757=CARTESIAN_POINT('Ctrl Pts',(-6.95354550483591,64.85417809566,87.96744232501));
#120758=CARTESIAN_POINT('Ctrl Pts',(-9.79955613262591,57.68387140554,72.8142459416047));
#120759=CARTESIAN_POINT('Ctrl Pts',(-9.80277833012592,57.6738396029,73.6207885064451));
#120760=CARTESIAN_POINT('Ctrl Pts',(-9.75736005205691,57.8083505427,75.42855130615));
#120761=CARTESIAN_POINT('Ctrl Pts',(-9.51030405160591,58.55075850748,78.126834664904));
#120762=CARTESIAN_POINT('Ctrl Pts',(-9.08987811173791,59.90727613614,80.7409654777591));
#120763=CARTESIAN_POINT('Ctrl Pts',(-8.58195139340691,61.74310086763,83.00598344105));
#120764=CARTESIAN_POINT('Ctrl Pts',(-8.08130749399791,63.87735771982,84.78648432159));
#120765=CARTESIAN_POINT('Ctrl Pts',(-7.78363606475891,65.46586756939,85.70542531448));
#120766=CARTESIAN_POINT('Ctrl Pts',(-7.65860430020592,66.22796383846,86.07462806762));
#120767=CARTESIAN_POINT('Ctrl Pts',(-10.5920145387619,59.99452354804,72.8293845444182));
#120768=CARTESIAN_POINT('Ctrl Pts',(-10.5939373540449,59.98545191324,73.5659849178225));
#120769=CARTESIAN_POINT('Ctrl Pts',(-10.5667795569519,60.1077131188501,
75.2172706809381));
#120770=CARTESIAN_POINT('Ctrl Pts',(-10.4191341151519,60.77930377661,77.670484391766));
#120771=CARTESIAN_POINT('Ctrl Pts',(-10.1684208232389,61.98983684518,80.026094579785));
#120772=CARTESIAN_POINT('Ctrl Pts',(-9.86622817732191,63.60334211099,82.0513183903311));
#120773=CARTESIAN_POINT('Ctrl Pts',(-9.5689352031129,65.4550150481601,83.63801640698));
#120774=CARTESIAN_POINT('Ctrl Pts',(-9.39241919703993,66.8223326583,84.45875352908));
#120775=CARTESIAN_POINT('Ctrl Pts',(-9.31830056473391,67.47714606609,84.7893033349101));
#120776=CARTESIAN_POINT('Ctrl Pts',(-12.3455984679183,61.69518876569,72.8346812857541));
#120777=CARTESIAN_POINT('Ctrl Pts',(-12.3467246669001,61.68710326644,73.5468061433598));
#120778=CARTESIAN_POINT('Ctrl Pts',(-12.3312057972915,61.79631693786,75.143292386617));
#120779=CARTESIAN_POINT('Ctrl Pts',(-12.2462629200551,62.3956876081601,
77.512581805897));
#120780=CARTESIAN_POINT('Ctrl Pts',(-12.0982058935566,63.4728781259,79.784555602918));
#120781=CARTESIAN_POINT('Ctrl Pts',(-11.9148004897113,64.90420967114,81.737926201103));
#120782=CARTESIAN_POINT('Ctrl Pts',(-11.7303545528999,66.5426944707001,
83.27176157901));
#120783=CARTESIAN_POINT('Ctrl Pts',(-11.6190836714997,67.75135964745,84.06872322495));
#120784=CARTESIAN_POINT('Ctrl Pts',(-11.5721915986834,68.3304350105,84.39060710346));
#120785=CARTESIAN_POINT('Ctrl Pts',(-10.5124509203882,67.7276234911821,
84.5902726033587));
#120786=CARTESIAN_POINT('Ctrl Pts',(-10.5571607538673,67.5564137297223,
84.4811141924303));
#120787=CARTESIAN_POINT('Ctrl Pts',(-10.6024067360406,67.3854035451806,
84.3665684200013));
#120788=CARTESIAN_POINT('Ctrl Pts',(-10.647902702036,67.2149593627826,84.2464239157399));
#120789=CARTESIAN_POINT('Ctrl Pts',(-10.6923121599897,67.0485856286275,
84.1291486322367));
#120790=CARTESIAN_POINT('Ctrl Pts',(-10.7369598391845,66.8827510813303,
84.006538784529));
#120791=CARTESIAN_POINT('Ctrl Pts',(-10.7815416096712,66.7178284965059,
83.8784014638752));
#120792=CARTESIAN_POINT('Ctrl Pts',(-10.7952986086174,66.6669368472762,
83.8388609753309));
#120793=CARTESIAN_POINT('Ctrl Pts',(-10.8090490512996,66.6161322765244,
83.7987941851335));
#120794=CARTESIAN_POINT('Ctrl Pts',(-10.8227832369869,66.5654263988847,
83.7581955099901));
#120795=CARTESIAN_POINT('Ctrl Pts',(-10.8374969257521,66.5111042483657,
83.7147013936337));
#120796=CARTESIAN_POINT('Ctrl Pts',(-10.8521919416177,66.4568953654081,
83.6705968123089));
#120797=CARTESIAN_POINT('Ctrl Pts',(-10.866861219374,66.40281454008,83.6258763513473));
#120798=CARTESIAN_POINT('Ctrl Pts',(-10.912283231951,66.2353584478959,83.4874037302678));
#120799=CARTESIAN_POINT('Ctrl Pts',(-10.9574603156574,66.0691269645397,
83.3430250688872));
#120800=CARTESIAN_POINT('Ctrl Pts',(-11.0021668171137,65.904586381939,83.1925892385079));
#120801=CARTESIAN_POINT('Ctrl Pts',(-11.0156267029942,65.855047782577,83.1472971882851));
#120802=CARTESIAN_POINT('Ctrl Pts',(-11.0290437632254,65.8056627461838,
83.101456195675));
#120803=CARTESIAN_POINT('Ctrl Pts',(-11.0424113914877,65.7564447705378,
83.0550624239674));
#120804=CARTESIAN_POINT('Ctrl Pts',(-11.0712952412536,65.6500979611824,
82.9548179598197));
#120805=CARTESIAN_POINT('Ctrl Pts',(-11.0999486221246,65.5445305662594,
82.8519924828178));
#120806=CARTESIAN_POINT('Ctrl Pts',(-11.1283013959138,65.439884830871,82.7465497055479));
#120807=CARTESIAN_POINT('Ctrl Pts',(-11.1424777828084,65.3875619631768,
82.6938283169129));
#120808=CARTESIAN_POINT('Ctrl Pts',(-11.1565789783029,65.3354695501648,
82.6404525535991));
#120809=CARTESIAN_POINT('Ctrl Pts',(-11.1705957096327,65.283626287648,82.5864183268548));
#120810=CARTESIAN_POINT('Ctrl Pts',(-11.1776040752976,65.2577046563896,
82.5594012134826));
#120811=CARTESIAN_POINT('Ctrl Pts',(-11.184591322483,65.2318453151878,82.5322194811105));
#120812=CARTESIAN_POINT('Ctrl Pts',(-11.191556267829,65.2060506367561,82.5048726231623));
#120813=CARTESIAN_POINT('Ctrl Pts',(-11.1916810581474,65.2055884757517,
82.5043826518928));
#120814=CARTESIAN_POINT('Ctrl Pts',(-11.1918058413085,65.205126335507,82.5038926276147));
#120815=CARTESIAN_POINT('Ctrl Pts',(-11.1919306173052,65.2046642160358,
82.5034025503252));
#120816=CARTESIAN_POINT('Ctrl Pts',(-11.1952879143089,65.1922301553399,
82.4902162399814));
#120817=CARTESIAN_POINT('Ctrl Pts',(-11.1986400245594,65.1798111337265,
82.4769915511165));
#120818=CARTESIAN_POINT('Ctrl Pts',(-11.2019868941466,65.1674074115863,
82.4637284635117));
#120819=CARTESIAN_POINT('Ctrl Pts',(-11.2048825157721,65.156676044519,82.4522535965384));
#120820=CARTESIAN_POINT('Ctrl Pts',(-11.2075163566646,65.146911979336,82.4417781471476));
#120821=CARTESIAN_POINT('Ctrl Pts',(-11.2105337830348,65.1357230733704,
82.4297294168383));
#120822=CARTESIAN_POINT('Ctrl Pts',(-11.2111336336814,65.133498769724,82.4273341840208));
#120823=CARTESIAN_POINT('Ctrl Pts',(-11.2117486041085,65.131218265178,82.4248766638023));
#120824=CARTESIAN_POINT('Ctrl Pts',(-11.2123837019444,65.128862938698,82.4223364667047));
#120825=CARTESIAN_POINT('Ctrl Pts',(-11.2942472546863,64.8252634259213,
82.0949072938397));
#120826=CARTESIAN_POINT('Ctrl Pts',(-11.3705951712443,64.5372340599892,
81.7515706634562));
#120827=CARTESIAN_POINT('Ctrl Pts',(-11.4414053735863,64.2666193828729,
81.3941165105011));
#120828=CARTESIAN_POINT('Ctrl Pts',(-11.4735077597793,64.1439339987481,
81.2320617375315));
#120829=CARTESIAN_POINT('Ctrl Pts',(-11.5044718368254,64.0248281634478,
81.0671060031894));
#120830=CARTESIAN_POINT('Ctrl Pts',(-11.5342949433969,63.9094748506058,
80.899419378088));
#120831=CARTESIAN_POINT('Ctrl Pts',(-11.5371696397123,63.8983557627067,
80.8832557996171));
#120832=CARTESIAN_POINT('Ctrl Pts',(-11.5400337345991,63.8872715412271,
80.8670668490848));
#120833=CARTESIAN_POINT('Ctrl Pts',(-11.542887259983,63.876222305584,80.8508527026476));
#120834=CARTESIAN_POINT('Ctrl Pts',(-11.5917648555483,63.6869616548419,
80.5731230926512));
#120835=CARTESIAN_POINT('Ctrl Pts',(-11.6375414127317,63.5079663264096,
80.2880005124143));
#120836=CARTESIAN_POINT('Ctrl Pts',(-11.6803771649707,63.3398328677561,
79.9963738633194));
#120837=CARTESIAN_POINT('Ctrl Pts',(-11.7017950410903,63.2557661384293,
79.8505605387719));
#120838=CARTESIAN_POINT('Ctrl Pts',(-11.722477786309,63.1744148043336,79.7031212474435));
#120839=CARTESIAN_POINT('Ctrl Pts',(-11.7424453129458,63.0958527030976,
79.5541677673539));
#120840=CARTESIAN_POINT('Ctrl Pts',(-11.7524290762642,63.0565716524796,
79.479691027309));
#120841=CARTESIAN_POINT('Ctrl Pts',(-11.7622340395622,63.0179879053016,
79.4048357436953));
#120842=CARTESIAN_POINT('Ctrl Pts',(-11.7718627033941,62.9801106499541,
79.329615914249));
#120843=CARTESIAN_POINT('Ctrl Pts',(-11.77667703531,62.9611720222803,79.2920059995258));
#120844=CARTESIAN_POINT('Ctrl Pts',(-11.7814472926542,62.9424100172644,
79.2543049485313));
#120845=CARTESIAN_POINT('Ctrl Pts',(-11.7861737878643,62.9238257804744,
79.2165145132332));
#120846=CARTESIAN_POINT('Ctrl Pts',(-11.7903094711731,62.9075645732832,
79.1834478823473));
#120847=CARTESIAN_POINT('Ctrl Pts',(-11.7944116491156,62.8914394698721,
79.1503128166153));
#120848=CARTESIAN_POINT('Ctrl Pts',(-11.7984805310734,62.8754512364734,
79.1171104905557));
#120849=CARTESIAN_POINT('Ctrl Pts',(-11.7990617999246,62.8731672031307,
79.1123673011186));
#120850=CARTESIAN_POINT('Ctrl Pts',(-11.799770087722,62.8703842409647,79.1065776670679));
#120851=CARTESIAN_POINT('Ctrl Pts',(-11.8002222996932,62.8686075184584,
79.1028768077023));
#120852=CARTESIAN_POINT('Ctrl Pts',(-11.8006505385931,62.866924985178,79.0993721416518));
#120853=CARTESIAN_POINT('Ctrl Pts',(-11.8010783203329,62.8652438987129,
79.0958667426276));
#120854=CARTESIAN_POINT('Ctrl Pts',(-11.8015056452176,62.8635642598512,
79.0923606119149));
#120855=CARTESIAN_POINT('Ctrl Pts',(-11.8460771862884,62.6883718121375,
78.7266584151115));
#120856=CARTESIAN_POINT('Ctrl Pts',(-11.8856781389952,62.5289278991055,
78.3530004020439));
#120857=CARTESIAN_POINT('Ctrl Pts',(-11.9206224684312,62.3858328118145,
77.972949274693));
#120858=CARTESIAN_POINT('Ctrl Pts',(-11.9405131754483,62.3043814718452,
77.756619880263));
#120859=CARTESIAN_POINT('Ctrl Pts',(-11.9588952170532,62.2282272177574,
77.5382181271681));
#120860=CARTESIAN_POINT('Ctrl Pts',(-11.9758265504949,62.1574824052876,
77.3180248654247));
#120861=CARTESIAN_POINT('Ctrl Pts',(-12.0039576391837,62.0399412440611,
76.9521779463928));
#120862=CARTESIAN_POINT('Ctrl Pts',(-12.0280844055031,61.9373317689448,
76.5813885434241));
#120863=CARTESIAN_POINT('Ctrl Pts',(-12.0484148829352,61.8499598392947,
76.2068848559227));
#120864=CARTESIAN_POINT('Ctrl Pts',(-12.0498602892,61.8437480848044,76.180259314152));
#120865=CARTESIAN_POINT('Ctrl Pts',(-12.0512865041583,61.8376133587138,
76.1536149789424));
#120866=CARTESIAN_POINT('Ctrl Pts',(-12.0526936012417,61.8315557753413,
76.1269522832721));
#120867=CARTESIAN_POINT('Ctrl Pts',(-12.0606350094199,61.7973678414036,
75.9764727236643));
#120868=CARTESIAN_POINT('Ctrl Pts',(-12.0679674798593,61.7656370535321,
75.8254083877693));
#120869=CARTESIAN_POINT('Ctrl Pts',(-12.0747040815038,61.7363843803514,
75.6738365926947));
#120870=CARTESIAN_POINT('Ctrl Pts',(-12.0928359949156,61.6576492902919,
75.265873229416));
#120871=CARTESIAN_POINT('Ctrl Pts',(-12.1066523254737,61.5968632578809,
74.854233901312));
#120872=CARTESIAN_POINT('Ctrl Pts',(-12.1162912295882,61.554270718676,74.4406782018442));
#120873=CARTESIAN_POINT('Ctrl Pts',(-12.1182894866595,61.5454407892938,
74.354943289344));
#120874=CARTESIAN_POINT('Ctrl Pts',(-12.120108150671,61.5373929478406,74.2691259786376));
#120875=CARTESIAN_POINT('Ctrl Pts',(-12.121748363988,61.5301296357777,74.1832418854536));
#120876=CARTESIAN_POINT('Ctrl Pts',(-12.1293332128959,61.496541855458,73.7860875253132));
#120877=CARTESIAN_POINT('Ctrl Pts',(-12.1331032131001,61.4797272509038,
73.3875061697423));
#120878=CARTESIAN_POINT('Ctrl Pts',(-12.1331903843725,61.479726180876,72.9888456300909));
#120879=CARTESIAN_POINT('Ctrl Pts',(-8.78823419891791,75.1738592483,86.78284890083));
#120880=CARTESIAN_POINT('Ctrl Pts',(-8.78306415477291,74.72662405869,86.7884138386));
#120881=CARTESIAN_POINT('Ctrl Pts',(-8.81909035422792,73.69777888124,86.7513931292899));
#120882=CARTESIAN_POINT('Ctrl Pts',(-9.02657683818592,72.18719744924,86.52606621289));
#120883=CARTESIAN_POINT('Ctrl Pts',(-9.35664843890192,70.73345419047,86.13264231638));
#120884=CARTESIAN_POINT('Ctrl Pts',(-9.6889294640759,69.49596570738,85.65887409272));
#120885=CARTESIAN_POINT('Ctrl Pts',(-9.98045484259091,68.43292028954,85.1378870539701));
#120886=CARTESIAN_POINT('Ctrl Pts',(-10.1467259739209,67.78111503905,84.74996216346));
#120887=CARTESIAN_POINT('Ctrl Pts',(-10.2190769752779,67.475529743,84.5512406152801));
#120888=CARTESIAN_POINT('Ctrl Pts',(-10.2208450793799,67.46804721363,84.5463644091599));
#120889=CARTESIAN_POINT('Ctrl Pts',(-9.36200580714891,75.1655542348801,
86.72290591126));
#120890=CARTESIAN_POINT('Ctrl Pts',(-9.35704322401691,74.73927457895,86.72795887135));
#120891=CARTESIAN_POINT('Ctrl Pts',(-9.39143229199792,73.75929218439,86.69443228328));
#120892=CARTESIAN_POINT('Ctrl Pts',(-9.59050034197691,72.30758761571,86.4878381917));
#120893=CARTESIAN_POINT('Ctrl Pts',(-9.91209801261292,70.8899328487,86.11982386996));
#120894=CARTESIAN_POINT('Ctrl Pts',(-10.2428814797899,69.6573777794501,
85.6638478182801));
#120895=CARTESIAN_POINT('Ctrl Pts',(-10.5367862749579,68.58546080019,85.1527501978));
#120896=CARTESIAN_POINT('Ctrl Pts',(-10.7064479646429,67.92049428063,84.76549219756));
#120897=CARTESIAN_POINT('Ctrl Pts',(-10.7804323422959,67.60807376471,84.56605837982));
#120898=CARTESIAN_POINT('Ctrl Pts',(-10.7822404632969,67.60042346136,84.5611641469));
#120899=CARTESIAN_POINT('Ctrl Pts',(-9.69871563896591,75.1551813275201,
86.2544898819));
#120900=CARTESIAN_POINT('Ctrl Pts',(-9.69387480142491,74.75534324128,86.25906511331));
#120901=CARTESIAN_POINT('Ctrl Pts',(-9.72730314172991,73.8365765524401,
86.2287688187401));
#120902=CARTESIAN_POINT('Ctrl Pts',(-9.92143095164091,72.46713521092,86.04033581194));
#120903=CARTESIAN_POINT('Ctrl Pts',(-10.2380558150979,71.11646999816,85.69971076544));
#120904=CARTESIAN_POINT('Ctrl Pts',(-10.5679604613399,69.92567467496,85.2691364608701));
#120905=CARTESIAN_POINT('Ctrl Pts',(-10.8632615838429,68.88187046176,84.78024447802));
#120906=CARTESIAN_POINT('Ctrl Pts',(-11.0349129752099,68.22957034288,84.40555652065));
#120907=CARTESIAN_POINT('Ctrl Pts',(-11.1098558768639,67.9226946509401,
84.21193807214));
#120908=CARTESIAN_POINT('Ctrl Pts',(-11.1116874812229,67.91517987633,84.20718621096));
#120909=CARTESIAN_POINT('Ctrl Pts',(-9.5727563377929,75.14969073673,85.69145592532));
#120910=CARTESIAN_POINT('Ctrl Pts',(-9.56786995661691,74.76406348025,85.69590777195));
#120911=CARTESIAN_POINT('Ctrl Pts',(-9.60165769416891,73.87784875743,85.6664135335801));
#120912=CARTESIAN_POINT('Ctrl Pts',(-9.79763359144691,72.55893776929,85.48340130992));
#120913=CARTESIAN_POINT('Ctrl Pts',(-10.1161187252549,71.26127783041,85.1537934673599));
#120914=CARTESIAN_POINT('Ctrl Pts',(-10.4463521283689,70.12108809596,84.73921042658));
#120915=CARTESIAN_POINT('Ctrl Pts',(-10.7411309007689,69.12354444036,84.26996174735));
#120916=CARTESIAN_POINT('Ctrl Pts',(-10.9120379674689,68.50125146073,83.91132461735));
#120917=CARTESIAN_POINT('Ctrl Pts',(-10.9866222962459,68.20858541074,83.7261526762101));
#120918=CARTESIAN_POINT('Ctrl Pts',(-10.9884451157479,68.20141865861,83.7216081912601));
#120919=CARTESIAN_POINT('Ctrl Pts',(-9.44679703661891,75.14420014595,85.12842196873));
#120920=CARTESIAN_POINT('Ctrl Pts',(-9.44186511180891,74.7727837192299,
85.1327504306));
#120921=CARTESIAN_POINT('Ctrl Pts',(-9.47601224660891,73.91912096243,85.1040582484099));
#120922=CARTESIAN_POINT('Ctrl Pts',(-9.67383623125391,72.65074032767,84.9264668079));
#120923=CARTESIAN_POINT('Ctrl Pts',(-9.99418163541291,71.40608566265,84.6078761692801));
#120924=CARTESIAN_POINT('Ctrl Pts',(-10.3247437953979,70.31650151696,84.2092843923));
#120925=CARTESIAN_POINT('Ctrl Pts',(-10.6190002176949,69.36521841896,83.75967901667));
#120926=CARTESIAN_POINT('Ctrl Pts',(-10.7891629597279,68.77293257858,83.41709271406));
#120927=CARTESIAN_POINT('Ctrl Pts',(-10.8633887156269,68.49447617054,83.24036728027));
#120928=CARTESIAN_POINT('Ctrl Pts',(-10.8652027502739,68.4876574409,83.23603017156));
#120929=CARTESIAN_POINT('Ctrl Pts',(-8.94256573698691,75.14727075947,84.84802251596));
#120930=CARTESIAN_POINT('Ctrl Pts',(-8.93745149514391,74.76831266994,84.8526646090801));
#120931=CARTESIAN_POINT('Ctrl Pts',(-8.97303734339591,73.89672718439,84.8218088401));
#120932=CARTESIAN_POINT('Ctrl Pts',(-9.17825945971091,72.6132869262601,
84.63326576691));
#120933=CARTESIAN_POINT('Ctrl Pts',(-9.50605176559191,71.3721378685,84.3019383492));
#120934=CARTESIAN_POINT('Ctrl Pts',(-9.83792998165891,70.30809764094,83.89921264699));
#120935=CARTESIAN_POINT('Ctrl Pts',(-10.1300953692419,69.39022670154,83.45352654093));
#120936=CARTESIAN_POINT('Ctrl Pts',(-10.2972784838039,68.8251829068101,
83.11971723483));
#120937=CARTESIAN_POINT('Ctrl Pts',(-10.3700688263069,68.56008000191,82.948409991363));
#120938=CARTESIAN_POINT('Ctrl Pts',(-10.3718476940469,68.55358860125,82.944206314064));
#120939=CARTESIAN_POINT('Ctrl Pts',(-8.39791503440691,75.15684515891,85.03813500136));
#120940=CARTESIAN_POINT('Ctrl Pts',(-8.3926038609189,74.75364609168,85.0433175978499));
#120941=CARTESIAN_POINT('Ctrl Pts',(-8.4297437505259,73.82567203736,85.00878227787));
#120942=CARTESIAN_POINT('Ctrl Pts',(-8.6429570360019,72.47167265314,84.80025313287));
#120943=CARTESIAN_POINT('Ctrl Pts',(-8.9787931905259,71.18218065664,84.44096904022));
#120944=CARTESIAN_POINT('Ctrl Pts',(-9.31209295830991,70.1015073586001,
84.01675409817));
#120945=CARTESIAN_POINT('Ctrl Pts',(-9.60199969291491,69.18181286463,83.5566371800399));
#120946=CARTESIAN_POINT('Ctrl Pts',(-9.76596433175591,68.62299289916,83.21845014512));
#120947=CARTESIAN_POINT('Ctrl Pts',(-9.83720419749391,68.36144004473,83.04590239804));
#120948=CARTESIAN_POINT('Ctrl Pts',(-9.83894507933091,68.3550359577,83.04166880362));
#120949=CARTESIAN_POINT('Origin',(-10.0948681361921,68.0757882531393,83.873061985328));
#120950=CARTESIAN_POINT('Ctrl Pts',(-9.07682613028944,74.9999993274218,
86.7031078141393));
#120951=CARTESIAN_POINT('Ctrl Pts',(-9.1039999950439,75.0000092485729,86.6903141483864));
#120952=CARTESIAN_POINT('Ctrl Pts',(-9.13088724151182,75.0000188963107,
86.6759898162085));
#120953=CARTESIAN_POINT('Ctrl Pts',(-9.15724126370756,75.0000282223508,
86.660143135858));
#120954=CARTESIAN_POINT('Ctrl Pts',(-9.1832912253031,75.0000374407914,86.6444792872249));
#120955=CARTESIAN_POINT('Ctrl Pts',(-9.20881934010755,75.000046344709,86.6273278788693));
#120956=CARTESIAN_POINT('Ctrl Pts',(-9.23358406665593,75.0000548869962,
86.6087473498606));
#120957=CARTESIAN_POINT('Ctrl Pts',(-9.25813552876578,75.0000633557204,
86.5903268293252));
#120958=CARTESIAN_POINT('Ctrl Pts',(-9.28193582083955,75.0000714688075,
86.5705018011063));
#120959=CARTESIAN_POINT('Ctrl Pts',(-9.30475915361152,75.0000791829749,
86.5493793145271));
#120960=CARTESIAN_POINT('Ctrl Pts',(-9.3274531992086,75.0000868534439,86.5283764803511));
#120961=CARTESIAN_POINT('Ctrl Pts',(-9.3491805030452,75.000094129306,86.5060911919904));
#120962=CARTESIAN_POINT('Ctrl Pts',(-9.36974127645128,75.0001009736224,
86.4826751026743));
#120963=CARTESIAN_POINT('Ctrl Pts',(-9.39024645363451,75.0001077994319,
86.4593223303403));
#120964=CARTESIAN_POINT('Ctrl Pts',(-9.40959070386905,75.0001141958634,
86.4348454293696));
#120965=CARTESIAN_POINT('Ctrl Pts',(-9.42760939948391,75.0001201345612,
86.4094343008029));
#120966=CARTESIAN_POINT('Ctrl Pts',(-9.44563283269775,75.0001260748204,
86.384016490968));
#120967=CARTESIAN_POINT('Ctrl Pts',(-9.46232950021035,75.0001315569872,
86.3576647027745));
#120968=CARTESIAN_POINT('Ctrl Pts',(-9.47757741530337,75.0001365631105,
86.3305987120963));
#120969=CARTESIAN_POINT('Ctrl Pts',(-9.49293759605771,75.0001416060924,
86.3033334429381));
#120970=CARTESIAN_POINT('Ctrl Pts',(-9.50682728712193,75.0001461659229,
86.2753442715377));
#120971=CARTESIAN_POINT('Ctrl Pts',(-9.51917165228589,75.0001502362991,
86.2468739512454));
#120972=CARTESIAN_POINT('Ctrl Pts',(-9.53159872212886,75.000154333946,86.2182128857289));
#120973=CARTESIAN_POINT('Ctrl Pts',(-9.54245964807323,75.0001579355543,
86.1890651223823));
#120974=CARTESIAN_POINT('Ctrl Pts',(-9.55173123092228,75.0001610474391,
86.1596830567647));
#120975=CARTESIAN_POINT('Ctrl Pts',(-9.56108916788585,75.0001641883075,
86.1300273310505));
#120976=CARTESIAN_POINT('Ctrl Pts',(-9.56882823591791,75.0001668303455,
86.1001338087849));
#120977=CARTESIAN_POINT('Ctrl Pts',(-9.57497724561461,75.0001689925852,
86.0702529880198));
#120978=CARTESIAN_POINT('Ctrl Pts',(-9.58119948158406,75.0001711805742,
86.0400163276578));
#120979=CARTESIAN_POINT('Ctrl Pts',(-9.58579401693955,75.0001728773831,
86.0097934597345));
#120980=CARTESIAN_POINT('Ctrl Pts',(-9.5888392751087,75.0001741142058,85.9798218969514));
#120981=CARTESIAN_POINT('Ctrl Pts',(-9.59195555286792,75.000175379873,85.9491513562872));
#120982=CARTESIAN_POINT('Ctrl Pts',(-9.59345005338468,75.0001761639981,
85.9187446672596));
#120983=CARTESIAN_POINT('Ctrl Pts',(-9.59344934447128,75.0001765099556,
85.8888219184229));
#120984=CARTESIAN_POINT('Ctrl Pts',(-9.59344862496941,75.0001768610804,
85.8584522371007));
#120985=CARTESIAN_POINT('Ctrl Pts',(-9.59190851333747,75.0001767610487,
85.8285814699798));
#120986=CARTESIAN_POINT('Ctrl Pts',(-9.5889935805498,75.0001762626353,85.7993962358321));
#120987=CARTESIAN_POINT('Ctrl Pts',(-9.58600511872059,75.0001757516495,
85.769474805535));
#120988=CARTESIAN_POINT('Ctrl Pts',(-9.58157246622322,75.0001748221386,
85.7402741621901));
#120989=CARTESIAN_POINT('Ctrl Pts',(-9.57589365398664,75.0001735355896,
85.7119449365612));
#120990=CARTESIAN_POINT('Ctrl Pts',(-9.57457467685929,75.0001732367721,
85.7053651098151));
#120991=CARTESIAN_POINT('Ctrl Pts',(-9.57318852872199,75.0001729187054,
85.69883207632));
#120992=CARTESIAN_POINT('Ctrl Pts',(-9.57173776914894,75.000172582176,85.6923473348265));
#120993=CARTESIAN_POINT('Ctrl Pts',(-9.56551370280152,75.0001711383933,
85.6645264180797));
#120994=CARTESIAN_POINT('Ctrl Pts',(-9.55783270404159,75.000169375034,85.636404976219));
#120995=CARTESIAN_POINT('Ctrl Pts',(-9.54857347396362,75.0001672728027,
85.6081918997157));
#120996=CARTESIAN_POINT('Ctrl Pts',(-9.53951690601546,75.0001652165842,
85.5805963391533));
#120997=CARTESIAN_POINT('Ctrl Pts',(-9.52894976121176,75.0001628359852,
85.5529135806624));
#120998=CARTESIAN_POINT('Ctrl Pts',(-9.51679285414588,75.0001601213691,
85.525374443193));
#120999=CARTESIAN_POINT('Ctrl Pts',(-9.5048679062755,75.000157458549,85.4983607647188));
#121000=CARTESIAN_POINT('Ctrl Pts',(-9.49141274535669,75.0001544741896,
85.4714859248144));
#121001=CARTESIAN_POINT('Ctrl Pts',(-9.47639499416025,75.0001511698034,
85.4449939781286));
#121002=CARTESIAN_POINT('Ctrl Pts',(-9.46162100403104,75.0001479190524,
85.4189320362492));
#121003=CARTESIAN_POINT('Ctrl Pts',(-9.44533438718474,75.0001443584789,
85.3932414401996));
#121004=CARTESIAN_POINT('Ctrl Pts',(-9.42755231432626,75.0001405017234,
85.3681696172939));
#121005=CARTESIAN_POINT('Ctrl Pts',(-9.41000756113383,75.0001366964402,
85.3434324031083));
#121006=CARTESIAN_POINT('Ctrl Pts',(-9.39100687524647,75.0001326027845,
85.3192984171788));
#121007=CARTESIAN_POINT('Ctrl Pts',(-9.37061743520198,75.0001282469069,
85.2960079213212));
#121008=CARTESIAN_POINT('Ctrl Pts',(-9.34984201493385,75.0001238085708,
85.2722765270976));
#121009=CARTESIAN_POINT('Ctrl Pts',(-9.32762462572574,75.0001190979427,
85.2494218850684));
#121010=CARTESIAN_POINT('Ctrl Pts',(-9.30409180453489,75.0001141571469,
85.2276865690307));
#121011=CARTESIAN_POINT('Ctrl Pts',(-9.28144013241794,75.0001094013514,
85.2067650973444));
#121012=CARTESIAN_POINT('Ctrl Pts',(-9.25757030985385,75.0001044324524,
85.1868814238287));
#121013=CARTESIAN_POINT('Ctrl Pts',(-9.23264164306911,75.0000993002975,
85.1682285148038));
#121014=CARTESIAN_POINT('Ctrl Pts',(-9.20779321329462,75.0000941846614,
85.1496356432316));
#121015=CARTESIAN_POINT('Ctrl Pts',(-9.18189331394217,75.0000889069572,
85.1322663161795));
#121016=CARTESIAN_POINT('Ctrl Pts',(-9.15513836009448,75.0000835269521,
85.116277304706));
#121017=CARTESIAN_POINT('Ctrl Pts',(-9.12839924598676,75.0000781501322,
85.1002977592098));
#121018=CARTESIAN_POINT('Ctrl Pts',(-9.10080683593434,75.0000726713189,
85.0856974009567));
#121019=CARTESIAN_POINT('Ctrl Pts',(-9.07258596059583,75.0000671581359,
85.072589329158));
#121020=CARTESIAN_POINT('Ctrl Pts',(-9.04430746240215,75.0000616336957,
85.0594544926146));
#121021=CARTESIAN_POINT('Ctrl Pts',(-9.01539879073464,75.000056074964,85.0478183180827));
#121022=CARTESIAN_POINT('Ctrl Pts',(-8.98610290733461,75.0000505549175,
85.0377450762615));
#121023=CARTESIAN_POINT('Ctrl Pts',(-8.95654791083624,75.0000449860479,
85.0275827397076));
#121024=CARTESIAN_POINT('Ctrl Pts',(-8.92659973489031,75.0000394567854,
85.0190111633951));
#121025=CARTESIAN_POINT('Ctrl Pts',(-8.89651140594933,75.000034043637,85.012043351497));
#121026=CARTESIAN_POINT('Ctrl Pts',(-8.86622517470581,75.0000285948843,
85.0050297096686));
#121027=CARTESIAN_POINT('Ctrl Pts',(-8.83579781987906,75.0000232640081,
84.9996407568054));
#121028=CARTESIAN_POINT('Ctrl Pts',(-8.80547732474202,75.0000181270819,
84.9958377323157));
#121029=CARTESIAN_POINT('Ctrl Pts',(-8.77474583349593,75.0000129205244,
84.9919831576037));
#121030=CARTESIAN_POINT('Ctrl Pts',(-8.74412491066269,75.0000079134206,
84.9897573534682));
#121031=CARTESIAN_POINT('Ctrl Pts',(-8.71384962962853,75.000003179607,84.9890718459353));
#121032=CARTESIAN_POINT('Ctrl Pts',(-8.70698518555844,75.0000021062891,
84.9889164178779));
#121033=CARTESIAN_POINT('Ctrl Pts',(-8.70013839104306,75.0000010469921,
84.9888399980095));
#121034=CARTESIAN_POINT('Ctrl Pts',(-8.69331176399212,75.0000000025229,
84.9888412596806));
#121035=CARTESIAN_POINT('Ctrl Pts',(-10.2209988615099,82.53201492112,84.5463071490699));
#121036=CARTESIAN_POINT('Ctrl Pts',(-10.2196138809369,82.52615454987,84.5501263019201));
#121037=CARTESIAN_POINT('Ctrl Pts',(-10.1480248596239,82.22369804759,84.7469073932701));
#121038=CARTESIAN_POINT('Ctrl Pts',(-9.98388528962092,81.57953238398,85.13082175917));
#121039=CARTESIAN_POINT('Ctrl Pts',(-9.69703742856391,80.53299869942,85.6454591886499));
#121040=CARTESIAN_POINT('Ctrl Pts',(-9.37340190588592,79.32933774873,86.1104956637399));
#121041=CARTESIAN_POINT('Ctrl Pts',(-9.0509892783709,77.93165755883,86.49818447736));
#121042=CARTESIAN_POINT('Ctrl Pts',(-8.8275504427949,76.40669320108,86.74311300067));
#121043=CARTESIAN_POINT('Ctrl Pts',(-8.78224841483291,75.3376955241,86.7892411675));
#121044=CARTESIAN_POINT('Ctrl Pts',(-8.78824703447191,74.82597871997,86.7828639942501));
#121045=CARTESIAN_POINT('Ctrl Pts',(-10.7823191176949,82.39961247361,84.56103171051));
#121046=CARTESIAN_POINT('Ctrl Pts',(-10.7809027858309,82.39362068301,84.56486500648));
#121047=CARTESIAN_POINT('Ctrl Pts',(-10.7076964146739,82.08439452547,84.76235742167));
#121048=CARTESIAN_POINT('Ctrl Pts',(-10.5401996687189,81.42719321186,85.1456491656101));
#121049=CARTESIAN_POINT('Ctrl Pts',(-10.2509568608329,80.37172515551,85.6506696895));
#121050=CARTESIAN_POINT('Ctrl Pts',(-9.92861983620391,79.1723369897,86.09858813837));
#121051=CARTESIAN_POINT('Ctrl Pts',(-9.61403567648691,77.80751099573,86.46193062935));
#121052=CARTESIAN_POINT('Ctrl Pts',(-9.39940208414091,76.34053759145,86.68685818504));
#121053=CARTESIAN_POINT('Ctrl Pts',(-9.35621111575492,75.32201118481,86.7286338586));
#121054=CARTESIAN_POINT('Ctrl Pts',(-9.36195895042991,74.83428008366,86.72284269431));
#121055=CARTESIAN_POINT('Ctrl Pts',(-11.1116947646629,82.08488536259,84.20707377878));
#121056=CARTESIAN_POINT('Ctrl Pts',(-11.1102600362549,82.07899968205,84.21079560067));
#121057=CARTESIAN_POINT('Ctrl Pts',(-11.0361046246079,81.77525758485,84.40253403785));
#121058=CARTESIAN_POINT('Ctrl Pts',(-10.8666379301449,81.13055427193,84.77340994602));
#121059=CARTESIAN_POINT('Ctrl Pts',(-10.5759897976639,80.10263820646,85.2565886538999));
#121060=CARTESIAN_POINT('Ctrl Pts',(-10.2544147153149,78.94355025105,85.67978173207));
#121061=CARTESIAN_POINT('Ctrl Pts',(-9.94442420176891,77.64203064539,86.01654748314));
#121062=CARTESIAN_POINT('Ctrl Pts',(-9.7349574150989,76.25723670102,86.22195022949));
#121063=CARTESIAN_POINT('Ctrl Pts',(-9.69300518984691,75.30213041752,86.25970207899));
#121064=CARTESIAN_POINT('Ctrl Pts',(-9.69860586706891,74.84465461789,86.25445790009));
#121065=CARTESIAN_POINT('Ctrl Pts',(-10.9884710263669,81.7986750417,83.7215562525299));
#121066=CARTESIAN_POINT('Ctrl Pts',(-10.9870431803459,81.79306191555,83.72511566167));
#121067=CARTESIAN_POINT('Ctrl Pts',(-10.9132428171619,81.50338372185,83.90848951421));
#121068=CARTESIAN_POINT('Ctrl Pts',(-10.7445131062059,80.88833942085,84.2634739684799));
#121069=CARTESIAN_POINT('Ctrl Pts',(-10.4543907240389,79.90600412583,84.7272181823501));
#121070=CARTESIAN_POINT('Ctrl Pts',(-10.1325305891159,78.79624595759,85.13464252384));
#121071=CARTESIAN_POINT('Ctrl Pts',(-9.82082153244591,77.54607482409,85.46040536236));
#121072=CARTESIAN_POINT('Ctrl Pts',(-9.60942177618192,76.21259532136,85.65983948489));
#121073=CARTESIAN_POINT('Ctrl Pts',(-9.56700612091791,75.29137171221,85.69659181294));
#121074=CARTESIAN_POINT('Ctrl Pts',(-9.5726618516689,74.85015223226,85.69148916033));
#121075=CARTESIAN_POINT('Ctrl Pts',(-10.8652472880709,81.5124647208,83.2360387262901));
#121076=CARTESIAN_POINT('Ctrl Pts',(-10.8638263244369,81.50712414905,83.23943572267));
#121077=CARTESIAN_POINT('Ctrl Pts',(-10.7903810097159,81.23150985885,83.41444499058));
#121078=CARTESIAN_POINT('Ctrl Pts',(-10.6223882822669,80.64612456977,83.75353799095));
#121079=CARTESIAN_POINT('Ctrl Pts',(-10.3327916504149,79.7093700452,84.1978477107901));
#121080=CARTESIAN_POINT('Ctrl Pts',(-10.0106464629179,78.64894166412,84.58950331562));
#121081=CARTESIAN_POINT('Ctrl Pts',(-9.69721886312191,77.45011900279,84.90426324159));
#121082=CARTESIAN_POINT('Ctrl Pts',(-9.48388613726391,76.16795394169,85.0977287403));
#121083=CARTESIAN_POINT('Ctrl Pts',(-9.44100705198991,75.2806130069,85.1334815468801));
#121084=CARTESIAN_POINT('Ctrl Pts',(-9.4467178362679,74.85564984662,85.12852042057));
#121085=CARTESIAN_POINT('Ctrl Pts',(-10.3719740027499,81.44650872388,82.9442186851291));
#121086=CARTESIAN_POINT('Ctrl Pts',(-10.3705805897979,81.4414245616901,
82.947511133341));
#121087=CARTESIAN_POINT('Ctrl Pts',(-10.2985565590249,81.17903235171,83.11714879837));
#121088=CARTESIAN_POINT('Ctrl Pts',(-10.1335140283549,80.6205979707,83.4475207026201));
#121089=CARTESIAN_POINT('Ctrl Pts',(-9.84602201196492,79.71691760354,83.88782277379));
#121090=CARTESIAN_POINT('Ctrl Pts',(-9.5227357389799,78.68180165885,84.28323004135));
#121091=CARTESIAN_POINT('Ctrl Pts',(-9.20242869026491,77.4879702719599,
84.60993193468));
#121092=CARTESIAN_POINT('Ctrl Pts',(-8.98135815126292,76.19187815032,84.81498348546));
#121093=CARTESIAN_POINT('Ctrl Pts',(-8.93662392308091,75.28618381722,84.85343067092));
#121094=CARTESIAN_POINT('Ctrl Pts',(-8.94255509050291,74.8525875886,84.84811080075));
#121095=CARTESIAN_POINT('Ctrl Pts',(-9.83910397498791,81.64499218078,83.0415917172));
#121096=CARTESIAN_POINT('Ctrl Pts',(-9.8377403243039,81.63997650984,83.04490752058));
#121097=CARTESIAN_POINT('Ctrl Pts',(-9.76725166882992,81.38110684321,83.2157650996));
#121098=CARTESIAN_POINT('Ctrl Pts',(-9.60539615737491,80.82886035969,83.55042868746));
#121099=CARTESIAN_POINT('Ctrl Pts',(-9.32017770116691,79.92359055334,84.0048347525));
#121100=CARTESIAN_POINT('Ctrl Pts',(-8.9956587438369,78.87281242971,84.42100077467));
#121101=CARTESIAN_POINT('Ctrl Pts',(-8.6679200091869,77.63427137341,84.7745893727101));
#121102=CARTESIAN_POINT('Ctrl Pts',(-8.43849051617991,76.26834068187,85.00101994304));
#121103=CARTESIAN_POINT('Ctrl Pts',(-8.39175222638992,75.30435215535,85.0440503939699));
#121104=CARTESIAN_POINT('Ctrl Pts',(-8.39792146786892,74.84301692091,85.03811183887));
#121105=CARTESIAN_POINT('Origin',(-10.0948766030609,81.92425938485,83.87303403236));
#121106=CARTESIAN_POINT('Ctrl Pts',(-10.9000842015569,85.1489979884701,
82.322918391228));
#121107=CARTESIAN_POINT('Ctrl Pts',(-10.9000339342259,85.1487780176699,
82.323157570113));
#121108=CARTESIAN_POINT('Ctrl Pts',(-10.8749983963149,85.03922423422,82.442269255368));
#121109=CARTESIAN_POINT('Ctrl Pts',(-10.8237045453949,84.8169570122299,
82.675542262189));
#121110=CARTESIAN_POINT('Ctrl Pts',(-10.7429847377379,84.47338318276,83.01175597191));
#121111=CARTESIAN_POINT('Ctrl Pts',(-10.6588700927759,84.1207479250599,
83.33364079941));
#121112=CARTESIAN_POINT('Ctrl Pts',(-10.5716199860159,83.75941600244,83.64129586374));
#121113=CARTESIAN_POINT('Ctrl Pts',(-10.4815593551129,83.38967102889,83.93484316048));
#121114=CARTESIAN_POINT('Ctrl Pts',(-10.3891461035709,83.01172959405,84.2144031959899));
#121115=CARTESIAN_POINT('Ctrl Pts',(-10.2950438513529,82.62625525885,84.47973595617));
#121116=CARTESIAN_POINT('Ctrl Pts',(-10.2314871820529,82.36404301501,84.6474306810499));
#121117=CARTESIAN_POINT('Ctrl Pts',(-10.1996872471569,82.23194589096,84.72880451956));
#121118=CARTESIAN_POINT('Ctrl Pts',(-11.4502964565729,85.02149802074,82.3294407801081));
#121119=CARTESIAN_POINT('Ctrl Pts',(-11.4502456178769,85.0212755613401,
82.329679510253));
#121120=CARTESIAN_POINT('Ctrl Pts',(-11.4249255198359,84.91048240158,82.4485675977571));
#121121=CARTESIAN_POINT('Ctrl Pts',(-11.3730558256989,84.68574072168,82.681278953403));
#121122=CARTESIAN_POINT('Ctrl Pts',(-11.2914660795799,84.3385299168701,
83.01625977792));
#121123=CARTESIAN_POINT('Ctrl Pts',(-11.2065003700329,83.98243486936,83.33647585558));
#121124=CARTESIAN_POINT('Ctrl Pts',(-11.1184361131769,83.61789200861,83.64201291631));
#121125=CARTESIAN_POINT('Ctrl Pts',(-11.0276387921209,83.24534162635,83.93292036531));
#121126=CARTESIAN_POINT('Ctrl Pts',(-10.9346178603449,82.86519761575,84.20924596527));
#121127=CARTESIAN_POINT('Ctrl Pts',(-10.8400534714679,82.4781915141401,
84.4707996776401));
#121128=CARTESIAN_POINT('Ctrl Pts',(-10.7763071557859,82.21549634624,84.6356097280201));
#121129=CARTESIAN_POINT('Ctrl Pts',(-10.7444477634099,82.08331859002,84.71545483133));
#121130=CARTESIAN_POINT('Ctrl Pts',(-11.7566426228269,84.63945625565,82.047965337043));
#121131=CARTESIAN_POINT('Ctrl Pts',(-11.7565914660076,84.63923911138,82.048196506829));
#121132=CARTESIAN_POINT('Ctrl Pts',(-11.7311129311008,84.5310931103201,
82.163319446383));
#121133=CARTESIAN_POINT('Ctrl Pts',(-11.6789226200385,84.3117447011801,
82.388587120115));
#121134=CARTESIAN_POINT('Ctrl Pts',(-11.596848511184,83.97297677322,82.712600409691));
#121135=CARTESIAN_POINT('Ctrl Pts',(-11.5114089474649,83.62570147102,83.02204061675));
#121136=CARTESIAN_POINT('Ctrl Pts',(-11.4228913896159,83.27038454296,83.31698288365));
#121137=CARTESIAN_POINT('Ctrl Pts',(-11.3316838955729,82.90754607615,83.59743190417));
#121138=CARTESIAN_POINT('Ctrl Pts',(-11.2383246207169,82.5377047440001,
83.86339068861));
#121139=CARTESIAN_POINT('Ctrl Pts',(-11.1435029242409,82.16161019115,84.11470474701));
#121140=CARTESIAN_POINT('Ctrl Pts',(-11.0796510175969,81.9066530444801,
84.27276298195));
#121141=CARTESIAN_POINT('Ctrl Pts',(-11.0477585205939,81.7784653785301,
84.3492589645101));
#121142=CARTESIAN_POINT('Ctrl Pts',(-11.6201571429516,84.25100099088,81.661304594338));
#121143=CARTESIAN_POINT('Ctrl Pts',(-11.620106127865,84.2507935134,81.661526002444));
#121144=CARTESIAN_POINT('Ctrl Pts',(-11.594698180855,84.1474619307,81.771787630287));
#121145=CARTESIAN_POINT('Ctrl Pts',(-11.5426507132809,83.9378717021601,
81.9875641102349));
#121146=CARTESIAN_POINT('Ctrl Pts',(-11.4607924010889,83.61414302773,82.297998404337));
#121147=CARTESIAN_POINT('Ctrl Pts',(-11.3755639521849,83.28223876212,82.594554327183));
#121148=CARTESIAN_POINT('Ctrl Pts',(-11.2872483521549,82.9425925833399,
82.877306111483));
#121149=CARTESIAN_POINT('Ctrl Pts',(-11.1962236012409,82.59567566606,83.14627065778));
#121150=CARTESIAN_POINT('Ctrl Pts',(-11.1030150673529,82.24195088805,83.40146328096));
#121151=CARTESIAN_POINT('Ctrl Pts',(-11.0083080083519,81.88212437179,83.64272752465));
#121152=CARTESIAN_POINT('Ctrl Pts',(-10.9445031453299,81.63810050545,83.794551969));
#121153=CARTESIAN_POINT('Ctrl Pts',(-10.9126253973309,81.51538217035,83.8680536305499));
#121154=CARTESIAN_POINT('Ctrl Pts',(-11.4836716630759,83.86254572611,81.274643851633));
#121155=CARTESIAN_POINT('Ctrl Pts',(-11.4836207897219,83.8623479154201,
81.274855498059));
#121156=CARTESIAN_POINT('Ctrl Pts',(-11.4582834306089,83.76383075108,81.380255814191));
#121157=CARTESIAN_POINT('Ctrl Pts',(-11.4063788065229,83.5639987031501,
81.586541100355));
#121158=CARTESIAN_POINT('Ctrl Pts',(-11.3247362909949,83.25530928223,81.8833963989819));
#121159=CARTESIAN_POINT('Ctrl Pts',(-11.2397189569049,82.93877605322,82.1670680376131));
#121160=CARTESIAN_POINT('Ctrl Pts',(-11.1516053146929,82.61480062371,82.437629339314));
#121161=CARTESIAN_POINT('Ctrl Pts',(-11.0607633069079,82.28380525598,82.6951094113881));
#121162=CARTESIAN_POINT('Ctrl Pts',(-10.9677055139879,81.9461970320901,
82.939535873321));
#121163=CARTESIAN_POINT('Ctrl Pts',(-10.8731130924629,81.60263855244,83.17075030229));
#121164=CARTESIAN_POINT('Ctrl Pts',(-10.8093552730629,81.36954796641,83.3163409560501));
#121165=CARTESIAN_POINT('Ctrl Pts',(-10.7774922740679,81.25229896216,83.3868482966));
#121166=CARTESIAN_POINT('Ctrl Pts',(-10.9929990594039,83.71997069593,81.033926038262));
#121167=CARTESIAN_POINT('Ctrl Pts',(-10.9929486955869,83.7197806253201,
81.034132061698));
#121168=CARTESIAN_POINT('Ctrl Pts',(-10.9678651037399,83.62511827294,81.136732224696));
#121169=CARTESIAN_POINT('Ctrl Pts',(-10.9164740096379,83.4330715771,81.337643141076));
#121170=CARTESIAN_POINT('Ctrl Pts',(-10.8356072946589,83.13625009941,81.627127262995));
#121171=CARTESIAN_POINT('Ctrl Pts',(-10.7513489296249,82.83165602498,81.904174282366));
#121172=CARTESIAN_POINT('Ctrl Pts',(-10.6639613365779,82.51961833081,82.1688668813501));
#121173=CARTESIAN_POINT('Ctrl Pts',(-10.5737763001199,82.20041342654,82.421295364125));
#121174=CARTESIAN_POINT('Ctrl Pts',(-10.4812604290489,81.8742682608201,
82.661548720194));
#121175=CARTESIAN_POINT('Ctrl Pts',(-10.3870801353809,81.5417685492,82.889430322419));
#121176=CARTESIAN_POINT('Ctrl Pts',(-10.3234914403189,81.3157055610401,
83.03335392967));
#121177=CARTESIAN_POINT('Ctrl Pts',(-10.2916814647829,81.20185290992,83.1031664991001));
#121178=CARTESIAN_POINT('Ctrl Pts',(-10.4668211332059,83.9158754608199,
81.0954924412439));
#121179=CARTESIAN_POINT('Ctrl Pts',(-10.4667713157959,83.91568617653,81.095700632396));
#121180=CARTESIAN_POINT('Ctrl Pts',(-10.4419598539459,83.8214154083399,
81.19938044292));
#121181=CARTESIAN_POINT('Ctrl Pts',(-10.3911194491209,83.63012480945,81.402524356558));
#121182=CARTESIAN_POINT('Ctrl Pts',(-10.3110846720209,83.33429197876,81.695632548757));
#121183=CARTESIAN_POINT('Ctrl Pts',(-10.2276401954349,83.03045094066,81.976617168283));
#121184=CARTESIAN_POINT('Ctrl Pts',(-10.1410311888439,82.71886465341,82.245574446584));
#121185=CARTESIAN_POINT('Ctrl Pts',(-10.0515506624969,82.39966146212,82.502665128717));
#121186=CARTESIAN_POINT('Ctrl Pts',(-9.95961592701791,82.07288083721,82.748048781055));
#121187=CARTESIAN_POINT('Ctrl Pts',(-9.86587758299191,81.73904818185,82.981479147184));
#121188=CARTESIAN_POINT('Ctrl Pts',(-9.80247025019291,81.5115428283,83.12938516456));
#121189=CARTESIAN_POINT('Ctrl Pts',(-9.7707171349199,81.39680769081,83.20125375235));
#121190=CARTESIAN_POINT('Origin',(-10.7325649783137,84.400884996501,81.8225337390639));
#121191=CARTESIAN_POINT('Ctrl Pts',(-10.9119544098049,84.86842874797,63.380422745097));
#121192=CARTESIAN_POINT('Ctrl Pts',(-10.9167381083619,84.8874759227999,
63.39998682244));
#121193=CARTESIAN_POINT('Ctrl Pts',(-10.9504786885429,85.0241366108199,
63.541195794788));
#121194=CARTESIAN_POINT('Ctrl Pts',(-11.0074315439549,85.2867981542799,
63.824462601624));
#121195=CARTESIAN_POINT('Ctrl Pts',(-11.0713860526219,85.65704572501,64.256521960082));
#121196=CARTESIAN_POINT('Ctrl Pts',(-11.1222079779469,86.0440636034599,
64.750002833932));
#121197=CARTESIAN_POINT('Ctrl Pts',(-11.1583315157829,86.4400410225399,
65.3076455886));
#121198=CARTESIAN_POINT('Ctrl Pts',(-11.1784124764709,86.8363310607599,
65.93168374147));
#121199=CARTESIAN_POINT('Ctrl Pts',(-11.1813287703659,87.2214023399299,
66.619865386485));
#121200=CARTESIAN_POINT('Ctrl Pts',(-11.1670632946759,87.58130362105,67.362729524661));
#121201=CARTESIAN_POINT('Ctrl Pts',(-11.1377395816439,87.90221268558,68.143219650457));
#121202=CARTESIAN_POINT('Ctrl Pts',(-11.0978808367489,88.1743502388799,
68.941806401532));
#121203=CARTESIAN_POINT('Ctrl Pts',(-11.0531195238519,88.3963865257801,
69.752103612324));
#121204=CARTESIAN_POINT('Ctrl Pts',(-11.0097139579119,88.5673268808599,
70.566915779017));
#121205=CARTESIAN_POINT('Ctrl Pts',(-10.9743067365659,88.68604747705,71.372377743079));
#121206=CARTESIAN_POINT('Ctrl Pts',(-10.9517101510869,88.75478071011,72.1496973709892));
#121207=CARTESIAN_POINT('Ctrl Pts',(-10.9431768096399,88.7795591710799,
72.8954247448889));
#121208=CARTESIAN_POINT('Ctrl Pts',(-10.9481909246279,88.76504282562,73.6271941059289));
#121209=CARTESIAN_POINT('Ctrl Pts',(-10.9661875364359,88.7111874448201,
74.366562872615));
#121210=CARTESIAN_POINT('Ctrl Pts',(-10.9960850511939,88.6145104410999,
75.122691718376));
#121211=CARTESIAN_POINT('Ctrl Pts',(-11.0346951715699,88.4723543121901,
75.888569658041));
#121212=CARTESIAN_POINT('Ctrl Pts',(-11.0771783094979,88.2835627033099,
76.658382386414));
#121213=CARTESIAN_POINT('Ctrl Pts',(-11.1183051004929,88.0466951245799,
77.428862016883));
#121214=CARTESIAN_POINT('Ctrl Pts',(-11.1527080864609,87.7600489942401,
78.196068193518));
#121215=CARTESIAN_POINT('Ctrl Pts',(-11.1750828468669,87.42966285556,78.941086404059));
#121216=CARTESIAN_POINT('Ctrl Pts',(-11.1820923536469,87.0683400052,79.641730697645));
#121217=CARTESIAN_POINT('Ctrl Pts',(-11.1727457911329,86.69122473511,80.282286917317));
#121218=CARTESIAN_POINT('Ctrl Pts',(-11.1481220746969,86.31198160359,80.855947397552));
#121219=CARTESIAN_POINT('Ctrl Pts',(-11.1097562815799,85.9405639758301,
81.363318728113));
#121220=CARTESIAN_POINT('Ctrl Pts',(-11.0596843146889,85.58438097307,81.807939054316));
#121221=CARTESIAN_POINT('Ctrl Pts',(-10.9997169907709,85.2500946837,82.193255543295));
#121222=CARTESIAN_POINT('Ctrl Pts',(-10.9476481892759,85.0127333998599,
82.448325023705));
#121223=CARTESIAN_POINT('Ctrl Pts',(-10.9170561372289,84.88870678709,82.576527099225));
#121224=CARTESIAN_POINT('Ctrl Pts',(-10.9119974436429,84.86856730116,82.597213818352));
#121225=CARTESIAN_POINT('Ctrl Pts',(-11.4334076262239,84.7058852730001,
63.4021229260991));
#121226=CARTESIAN_POINT('Ctrl Pts',(-11.4384281336359,84.72577353141,63.422283368637));
#121227=CARTESIAN_POINT('Ctrl Pts',(-11.4738076598529,84.86833137268,63.5676916393111));
#121228=CARTESIAN_POINT('Ctrl Pts',(-11.5331240407119,85.14051214413,63.857962637228));
#121229=CARTESIAN_POINT('Ctrl Pts',(-11.5992378217001,85.5210751481201,
64.298195710351));
#121230=CARTESIAN_POINT('Ctrl Pts',(-11.6514593274787,85.91618297563,64.798734693346));
#121231=CARTESIAN_POINT('Ctrl Pts',(-11.6884177467697,86.31832604546,65.362584895379));
#121232=CARTESIAN_POINT('Ctrl Pts',(-11.7088853971653,86.7189526464401,
65.991987132611));
#121233=CARTESIAN_POINT('Ctrl Pts',(-11.7118379510303,87.10657313034,66.684546553909));
#121234=CARTESIAN_POINT('Ctrl Pts',(-11.6973592798139,87.46724901606,67.430425724164));
#121235=CARTESIAN_POINT('Ctrl Pts',(-11.6677063303148,87.7872078148999,
68.21187499679));
#121236=CARTESIAN_POINT('Ctrl Pts',(-11.6275693811737,88.0568714128401,
69.008438916133));
#121237=CARTESIAN_POINT('Ctrl Pts',(-11.582721209285,88.2753365204001,69.812913501992));
#121238=CARTESIAN_POINT('Ctrl Pts',(-11.5394764818229,88.44224391384,70.617568177949));
#121239=CARTESIAN_POINT('Ctrl Pts',(-11.5043921904999,88.55733668999,71.4088842175801));
#121240=CARTESIAN_POINT('Ctrl Pts',(-11.4820942729849,88.62361512615,72.1695141058363));
#121241=CARTESIAN_POINT('Ctrl Pts',(-11.4736921131039,88.64744151544,72.8976469313896));
#121242=CARTESIAN_POINT('Ctrl Pts',(-11.4786272848249,88.63348875016,73.612004070298));
#121243=CARTESIAN_POINT('Ctrl Pts',(-11.4963735631779,88.58160440959,74.334975761448));
#121244=CARTESIAN_POINT('Ctrl Pts',(-11.5259553584829,88.48805634354,75.076751346021));
#121245=CARTESIAN_POINT('Ctrl Pts',(-11.5643401913829,88.34964052366,75.83152869767));
#121246=CARTESIAN_POINT('Ctrl Pts',(-11.6067999626929,88.16450527128,76.594015687991));
#121247=CARTESIAN_POINT('Ctrl Pts',(-11.6481137161238,87.93058808465,77.360828340916));
#121248=CARTESIAN_POINT('Ctrl Pts',(-11.6828288814868,87.64568228453,78.127539128295));
#121249=CARTESIAN_POINT('Ctrl Pts',(-11.7054934028938,87.3154663606801,
78.874524071436));
#121250=CARTESIAN_POINT('Ctrl Pts',(-11.7126190573528,86.95265177104,79.578735256338));
#121251=CARTESIAN_POINT('Ctrl Pts',(-11.7031198632119,86.57247347689,80.2238099822379));
#121252=CARTESIAN_POINT('Ctrl Pts',(-11.6779789498894,86.1883870293801,
80.8030245735091));
#121253=CARTESIAN_POINT('Ctrl Pts',(-11.6386935480217,85.81075877209,81.316300792395));
#121254=CARTESIAN_POINT('Ctrl Pts',(-11.5871609929257,85.44651420014,81.767814318776));
#121255=CARTESIAN_POINT('Ctrl Pts',(-11.5251031442909,85.10253986725,82.16069340561));
#121256=CARTESIAN_POINT('Ctrl Pts',(-11.4708398731529,84.85643753722,82.422175114672));
#121257=CARTESIAN_POINT('Ctrl Pts',(-11.4387608790089,84.7270567674,82.554194043774));
#121258=CARTESIAN_POINT('Ctrl Pts',(-11.4334511980329,84.70602607796,82.575513314783));
#121259=CARTESIAN_POINT('Ctrl Pts',(-11.6998099956741,84.3301713905001,
63.6965256689001));
#121260=CARTESIAN_POINT('Ctrl Pts',(-11.7049514850605,84.34993837856,63.71642164007));
#121261=CARTESIAN_POINT('Ctrl Pts',(-11.7411683234158,84.49155421921,63.859866042207));
#121262=CARTESIAN_POINT('Ctrl Pts',(-11.8016921928089,84.76097528105,64.14545510258));
#121263=CARTESIAN_POINT('Ctrl Pts',(-11.8689091125722,85.1360255796801,
64.5772345678011));
#121264=CARTESIAN_POINT('Ctrl Pts',(-11.921845642321,85.52396286686,65.066927135476));
#121265=CARTESIAN_POINT('Ctrl Pts',(-11.9592305896123,85.91766516084,65.617595936977));
#121266=CARTESIAN_POINT('Ctrl Pts',(-11.9798957937884,86.30888526874,66.2314198083571));
#121267=CARTESIAN_POINT('Ctrl Pts',(-11.9828668723107,86.6864950662899,
66.905995485085));
#121268=CARTESIAN_POINT('Ctrl Pts',(-11.9682792828025,87.0369737321501,
67.63156738817));
#121269=CARTESIAN_POINT('Ctrl Pts',(-11.9384581314933,87.3469819707,68.3905258639001));
#121270=CARTESIAN_POINT('Ctrl Pts',(-11.898179052113,87.6073349610399,69.1625064764761));
#121271=CARTESIAN_POINT('Ctrl Pts',(-11.8532865053112,87.81739160382,69.940065705042));
#121272=CARTESIAN_POINT('Ctrl Pts',(-11.8101239477353,87.9771542765201,
70.715405132558));
#121273=CARTESIAN_POINT('Ctrl Pts',(-11.7752046363583,88.08685253399,71.475595648902));
#121274=CARTESIAN_POINT('Ctrl Pts',(-11.7530593036793,88.14982244754,72.204598786874));
#121275=CARTESIAN_POINT('Ctrl Pts',(-11.7447241624273,88.17242101204,72.9015623720751));
#121276=CARTESIAN_POINT('Ctrl Pts',(-11.749619003257,88.1591906022601,73.585256804372));
#121277=CARTESIAN_POINT('Ctrl Pts',(-11.7672373901261,88.10992352232,74.277872782123));
#121278=CARTESIAN_POINT('Ctrl Pts',(-11.7966578892543,88.0208597083,74.989867717288));
#121279=CARTESIAN_POINT('Ctrl Pts',(-11.8349276262727,87.88858761723,75.716278183036));
#121280=CARTESIAN_POINT('Ctrl Pts',(-11.8773754599393,87.71092602096,76.452256402395));
#121281=CARTESIAN_POINT('Ctrl Pts',(-11.9187847295823,87.48552957653,77.194453959513));
#121282=CARTESIAN_POINT('Ctrl Pts',(-11.9536593825615,87.20997814688,77.938304641709));
#121283=CARTESIAN_POINT('Ctrl Pts',(-11.9764719383746,86.88958404568,78.664370660746));
#121284=CARTESIAN_POINT('Ctrl Pts',(-11.9836569308835,86.5366335335601,
79.349806919033));
#121285=CARTESIAN_POINT('Ctrl Pts',(-11.9740797596092,86.16596285257,79.978374486369));
#121286=CARTESIAN_POINT('Ctrl Pts',(-11.9486746184099,85.79051571235,80.543594155305));
#121287=CARTESIAN_POINT('Ctrl Pts',(-11.9089194026789,85.42058120531,81.045011693211));
#121288=CARTESIAN_POINT('Ctrl Pts',(-11.8566406556977,85.06261365341,81.487031944037));
#121289=CARTESIAN_POINT('Ctrl Pts',(-11.7935147903732,84.72342073508,81.872514837236));
#121290=CARTESIAN_POINT('Ctrl Pts',(-11.7381303986936,84.47973974133,82.129835708481));
#121291=CARTESIAN_POINT('Ctrl Pts',(-11.7052917488689,84.35121274205,82.260073941226));
#121292=CARTESIAN_POINT('Ctrl Pts',(-11.6998538423245,84.33030929138,82.281114592639));
#121293=CARTESIAN_POINT('Ctrl Pts',(-11.5463481159819,83.97372753764,64.081494764462));
#121294=CARTESIAN_POINT('Ctrl Pts',(-11.5514199133399,83.99248592696,64.100429046463));
#121295=CARTESIAN_POINT('Ctrl Pts',(-11.5871544155405,84.12690339444,64.236961386833));
#121296=CARTESIAN_POINT('Ctrl Pts',(-11.6469827075615,84.38299314048,64.509078924552));
#121297=CARTESIAN_POINT('Ctrl Pts',(-11.7135641609422,84.74011310431,64.921007397318));
#121298=CARTESIAN_POINT('Ctrl Pts',(-11.7660887989998,85.1100555127999,
65.388659305653));
#121299=CARTESIAN_POINT('Ctrl Pts',(-11.803228043564,85.48593260363,65.914912709119));
#121300=CARTESIAN_POINT('Ctrl Pts',(-11.8237794462954,85.8598226158,66.501853529596));
#121301=CARTESIAN_POINT('Ctrl Pts',(-11.8267398536336,86.2210550814401,
67.147209825903));
#121302=CARTESIAN_POINT('Ctrl Pts',(-11.8122150068324,86.5566733499299,
67.84171552602));
#121303=CARTESIAN_POINT('Ctrl Pts',(-11.7824907486777,86.8538867813,68.568647494553));
#121304=CARTESIAN_POINT('Ctrl Pts',(-11.7422935438457,87.10385264418,69.308693118078));
#121305=CARTESIAN_POINT('Ctrl Pts',(-11.697426559345,87.30586554635,70.054895804105));
#121306=CARTESIAN_POINT('Ctrl Pts',(-11.6542166675608,87.4597919165999,
70.799898497466));
#121307=CARTESIAN_POINT('Ctrl Pts',(-11.6192023189939,87.56566634817,71.531240114491));
#121308=CARTESIAN_POINT('Ctrl Pts',(-11.596969089365,87.62652087531,72.2332458051846));
#121309=CARTESIAN_POINT('Ctrl Pts',(-11.5885953418317,87.6483754722201,
72.9047487270023));
#121310=CARTESIAN_POINT('Ctrl Pts',(-11.5935134153919,87.63557929833,73.5634998632841));
#121311=CARTESIAN_POINT('Ctrl Pts',(-11.6112054745317,87.5879564959899,
74.230581459377));
#121312=CARTESIAN_POINT('Ctrl Pts',(-11.640718888804,87.50195800566,74.91579255546));
#121313=CARTESIAN_POINT('Ctrl Pts',(-11.6790549271481,87.37443216287,75.614119392195));
#121314=CARTESIAN_POINT('Ctrl Pts',(-11.7215096375298,87.2034378446199,
76.320805814706));
#121315=CARTESIAN_POINT('Ctrl Pts',(-11.7628638847739,86.98686102094,77.03266861722));
#121316=CARTESIAN_POINT('Ctrl Pts',(-11.7976466644359,86.72249079514,77.7454371892611));
#121317=CARTESIAN_POINT('Ctrl Pts',(-11.8203739445878,86.4154937219899,
78.4406404007131));
#121318=CARTESIAN_POINT('Ctrl Pts',(-11.827524755236,86.0776605602099,79.096575274848));
#121319=CARTESIAN_POINT('Ctrl Pts',(-11.817992502922,85.72318611707,79.697822394072));
#121320=CARTESIAN_POINT('Ctrl Pts',(-11.7927395709794,85.36451608399,80.23815625388));
#121321=CARTESIAN_POINT('Ctrl Pts',(-11.753254992926,85.0114198651101,80.717288073687));
#121322=CARTESIAN_POINT('Ctrl Pts',(-11.7014060920064,84.67018455978,81.139301715589));
#121323=CARTESIAN_POINT('Ctrl Pts',(-11.6388954608823,84.34728442778,81.507005378146));
#121324=CARTESIAN_POINT('Ctrl Pts',(-11.5841568940353,84.11568916058,81.752166503278));
#121325=CARTESIAN_POINT('Ctrl Pts',(-11.5517558461319,83.99369566282,81.876128141433));
#121326=CARTESIAN_POINT('Ctrl Pts',(-11.5463918043089,83.97385917525,81.896151373524));
#121327=CARTESIAN_POINT('Ctrl Pts',(-11.3928862362889,83.6172836847901,
64.466463860024));
#121328=CARTESIAN_POINT('Ctrl Pts',(-11.3978883416199,83.63503347536,64.4844364528561));
#121329=CARTESIAN_POINT('Ctrl Pts',(-11.4331405076649,83.76225256968,64.61405673146));
#121330=CARTESIAN_POINT('Ctrl Pts',(-11.4922732223139,84.00501099991,64.8727027465231));
#121331=CARTESIAN_POINT('Ctrl Pts',(-11.5582192093119,84.34420062893,65.2647802268361));
#121332=CARTESIAN_POINT('Ctrl Pts',(-11.6103319556786,84.69614815874,65.710391475831));
#121333=CARTESIAN_POINT('Ctrl Pts',(-11.6472254975157,85.05420004642,66.21222948126));
#121334=CARTESIAN_POINT('Ctrl Pts',(-11.6676630988025,85.41075996287,66.7722872508351));
#121335=CARTESIAN_POINT('Ctrl Pts',(-11.6706128349566,85.75561509659,67.388424166722));
#121336=CARTESIAN_POINT('Ctrl Pts',(-11.6561507308623,86.0763729677001,
68.05186366387));
#121337=CARTESIAN_POINT('Ctrl Pts',(-11.6265233658621,86.3607915919,68.746769125207));
#121338=CARTESIAN_POINT('Ctrl Pts',(-11.5864080355784,86.6003703273101,
69.45487975968));
#121339=CARTESIAN_POINT('Ctrl Pts',(-11.5415666133789,86.79433948889,70.169725903168));
#121340=CARTESIAN_POINT('Ctrl Pts',(-11.4983093873859,86.94242955668,70.884391862373));
#121341=CARTESIAN_POINT('Ctrl Pts',(-11.4632000016299,87.04448016234,71.58688458008));
#121342=CARTESIAN_POINT('Ctrl Pts',(-11.4408788750509,87.1032193030901,
72.2618928234953));
#121343=CARTESIAN_POINT('Ctrl Pts',(-11.4324665212359,87.12432993239,72.9079350819296));
#121344=CARTESIAN_POINT('Ctrl Pts',(-11.4374078275269,87.1119679944,73.5417429221963));
#121345=CARTESIAN_POINT('Ctrl Pts',(-11.4551735589369,87.06598946966,74.183290136631));
#121346=CARTESIAN_POINT('Ctrl Pts',(-11.4847798883539,86.98305630301,74.841717393632));
#121347=CARTESIAN_POINT('Ctrl Pts',(-11.5231822280239,86.8602767085,75.5119606013541));
#121348=CARTESIAN_POINT('Ctrl Pts',(-11.5656438151199,86.69594966828,76.189355227018));
#121349=CARTESIAN_POINT('Ctrl Pts',(-11.6069430399654,86.48819246535,76.870883274928));
#121350=CARTESIAN_POINT('Ctrl Pts',(-11.6416339463103,86.2350034433901,
77.552569736814));
#121351=CARTESIAN_POINT('Ctrl Pts',(-11.6642759508009,85.9414033983,78.216910140681));
#121352=CARTESIAN_POINT('Ctrl Pts',(-11.6713925795885,85.61868758687,78.843343630664));
#121353=CARTESIAN_POINT('Ctrl Pts',(-11.6619052462348,85.28040938158,79.417270301776));
#121354=CARTESIAN_POINT('Ctrl Pts',(-11.6368045235489,84.9385164556401,
79.9327183524551));
#121355=CARTESIAN_POINT('Ctrl Pts',(-11.5975905831731,84.60225852491,80.3895644541621));
#121356=CARTESIAN_POINT('Ctrl Pts',(-11.5461715283149,84.27775546615,80.791571487141));
#121357=CARTESIAN_POINT('Ctrl Pts',(-11.4842761313909,83.97114812048,81.1414959190551));
#121358=CARTESIAN_POINT('Ctrl Pts',(-11.4301833893769,83.7516385798401,
81.374497298075));
#121359=CARTESIAN_POINT('Ctrl Pts',(-11.3982199433949,83.63617858359,81.49218234164));
#121360=CARTESIAN_POINT('Ctrl Pts',(-11.3929297662929,83.61740905912,81.511188154409));
#121361=CARTESIAN_POINT('Ctrl Pts',(-10.9145013594719,83.50062863623,64.703833009367));
#121362=CARTESIAN_POINT('Ctrl Pts',(-10.9192862146809,83.51710648279,64.720741657142));
#121363=CARTESIAN_POINT('Ctrl Pts',(-10.9530348000159,83.6353242016,64.842777920554));
#121364=CARTESIAN_POINT('Ctrl Pts',(-11.0099991996659,83.86242730732,65.087497166191));
#121365=CARTESIAN_POINT('Ctrl Pts',(-11.0739642549319,84.18236181444,65.460607352468));
#121366=CARTESIAN_POINT('Ctrl Pts',(-11.1247930162699,84.51662290047,65.886619447888));
#121367=CARTESIAN_POINT('Ctrl Pts',(-11.1609206319429,84.85849295892,66.367912971536));
#121368=CARTESIAN_POINT('Ctrl Pts',(-11.1810034813509,85.20052067337,66.906414565492));
#121369=CARTESIAN_POINT('Ctrl Pts',(-11.1839199523509,85.53276388586,67.500173427059));
#121370=CARTESIAN_POINT('Ctrl Pts',(-11.1696534353449,85.84319176642,68.1410073089521));
#121371=CARTESIAN_POINT('Ctrl Pts',(-11.1403281142129,86.1198870157801,
68.81416418141));
#121372=CARTESIAN_POINT('Ctrl Pts',(-11.1004680104759,86.3544282397101,
69.502745154234));
#121373=CARTESIAN_POINT('Ctrl Pts',(-11.0557062733309,86.54569475296,70.2011927159229));
#121374=CARTESIAN_POINT('Ctrl Pts',(-11.0123014929789,86.6928676434501,
70.9032686830991));
#121375=CARTESIAN_POINT('Ctrl Pts',(-10.9768958489299,86.7950307772,71.597036884302));
#121376=CARTESIAN_POINT('Ctrl Pts',(-10.9543007222439,86.85415637997,72.2663793166297));
#121377=CARTESIAN_POINT('Ctrl Pts',(-10.9457680215319,86.87546716438,72.9084210698479));
#121378=CARTESIAN_POINT('Ctrl Pts',(-10.9507817509339,86.86298269682,73.5384365296263));
#121379=CARTESIAN_POINT('Ctrl Pts',(-10.9687771400309,86.81665821225,74.175067882143));
#121380=CARTESIAN_POINT('Ctrl Pts',(-10.9986731127109,86.73347503727,74.826278291994));
#121381=CARTESIAN_POINT('Ctrl Pts',(-11.0372821327079,86.61110788032,75.4860954416901));
#121382=CARTESIAN_POINT('Ctrl Pts',(-11.0797651565069,86.44851693899,76.149537007965));
#121383=CARTESIAN_POINT('Ctrl Pts',(-11.1208928606869,86.24442185857,76.813777645638));
#121384=CARTESIAN_POINT('Ctrl Pts',(-11.1552973714429,85.99732347199,77.475389357107));
#121385=CARTESIAN_POINT('Ctrl Pts',(-11.1776735471369,85.71240740907,78.118016760138));
#121386=CARTESIAN_POINT('Ctrl Pts',(-11.1846836212209,85.4007096691001,
78.722473835778));
#121387=CARTESIAN_POINT('Ctrl Pts',(-11.1753363132029,85.07529630638,79.275168931218));
#121388=CARTESIAN_POINT('Ctrl Pts',(-11.1507100706079,84.7479389048601,
79.770236225873));
#121389=CARTESIAN_POINT('Ctrl Pts',(-11.1123397858179,84.4272465671801,
80.208156931037));
#121390=CARTESIAN_POINT('Ctrl Pts',(-11.0622606849319,84.11957935255,80.5920213789121));
#121391=CARTESIAN_POINT('Ctrl Pts',(-11.0022831502009,83.830696414,80.9247829028901));
#121392=CARTESIAN_POINT('Ctrl Pts',(-10.9502036301909,83.6254599932199,
81.145148417673));
#121393=CARTESIAN_POINT('Ctrl Pts',(-10.9196043154289,83.51817119103,81.255944067916));
#121394=CARTESIAN_POINT('Ctrl Pts',(-10.9145443959369,83.50074826293,81.2738231017611));
#121395=CARTESIAN_POINT('Ctrl Pts',(-10.4071527116419,83.69593260378,64.646750601693));
#121396=CARTESIAN_POINT('Ctrl Pts',(-10.4117071633399,83.71166206633,64.663151272416));
#121397=CARTESIAN_POINT('Ctrl Pts',(-10.4438611337989,83.82464422908,64.78162352002));
#121398=CARTESIAN_POINT('Ctrl Pts',(-10.4985259380069,84.04345337825,65.020576732323));
#121399=CARTESIAN_POINT('Ctrl Pts',(-10.5603901261999,84.35472041601,65.387337694065));
#121400=CARTESIAN_POINT('Ctrl Pts',(-10.6098571637469,84.6825454490501,
65.808317421142));
#121401=CARTESIAN_POINT('Ctrl Pts',(-10.6451724803229,85.0198881580799,
66.285647498717));
#121402=CARTESIAN_POINT('Ctrl Pts',(-10.6648790994309,85.3591721061099,
66.821255809763));
#121403=CARTESIAN_POINT('Ctrl Pts',(-10.6677602912409,85.6903713424199,
67.41332242683));
#121404=CARTESIAN_POINT('Ctrl Pts',(-10.6537012031249,86.00139042658,68.05399654853));
#121405=CARTESIAN_POINT('Ctrl Pts',(-10.6246962130819,86.28021190296,68.729137806898));
#121406=CARTESIAN_POINT('Ctrl Pts',(-10.5851067885619,86.5181817555,69.42267673283));
#121407=CARTESIAN_POINT('Ctrl Pts',(-10.5404295609959,86.71375874238,70.129828876235));
#121408=CARTESIAN_POINT('Ctrl Pts',(-10.4968682926189,86.86550100478,70.84485056109));
#121409=CARTESIAN_POINT('Ctrl Pts',(-10.4611484533439,86.97164340359,71.555416167859));
#121410=CARTESIAN_POINT('Ctrl Pts',(-10.4382627372379,87.0334182268699,
72.2439296553813));
#121411=CARTESIAN_POINT('Ctrl Pts',(-10.4296024032359,87.0557494604799,
72.9059060278074));
#121412=CARTESIAN_POINT('Ctrl Pts',(-10.4346929406019,87.0426615024399,
73.5556262297241));
#121413=CARTESIAN_POINT('Ctrl Pts',(-10.4529318919879,86.9942148532899,
74.211001504031));
#121414=CARTESIAN_POINT('Ctrl Pts',(-10.4831350443589,86.907621009,74.879026858038));
#121415=CARTESIAN_POINT('Ctrl Pts',(-10.5219632581269,86.7810773188199,
75.552525741454));
#121416=CARTESIAN_POINT('Ctrl Pts',(-10.5644690165089,86.61421723637,76.225985233305));
#121417=CARTESIAN_POINT('Ctrl Pts',(-10.6054148153219,86.40636115899,76.896680893526));
#121418=CARTESIAN_POINT('Ctrl Pts',(-10.6395155906909,86.1564947859499,
77.561644728154));
#121419=CARTESIAN_POINT('Ctrl Pts',(-10.6616098430089,85.87017719721,78.205141976549));
#121420=CARTESIAN_POINT('Ctrl Pts',(-10.6685069110429,85.55858177196,78.808743611411));
#121421=CARTESIAN_POINT('Ctrl Pts',(-10.6593081061829,85.2347428489799,
79.359431202932));
#121422=CARTESIAN_POINT('Ctrl Pts',(-10.6351850710339,84.9106867918599,
79.85123162298));
#121423=CARTESIAN_POINT('Ctrl Pts',(-10.5977095208839,84.59465748902,80.285295703793));
#121424=CARTESIAN_POINT('Ctrl Pts',(-10.5490515013679,84.29351399509,80.664105744214));
#121425=CARTESIAN_POINT('Ctrl Pts',(-10.4911079456309,84.01282164204,80.99093874636));
#121426=CARTESIAN_POINT('Ctrl Pts',(-10.4411635379779,83.81521547721,81.206009625821));
#121427=CARTESIAN_POINT('Ctrl Pts',(-10.4120109456419,83.71268034274,81.313565299678));
#121428=CARTESIAN_POINT('Ctrl Pts',(-10.4071952246869,83.69605055436,81.330905291903));
#121429=CARTESIAN_POINT('Origin',(-10.7325537287249,84.40089372352,64.155250052704));
#121430=CARTESIAN_POINT('Ctrl Pts',(-10.1996916360579,82.23193715457,61.24897010379));
#121431=CARTESIAN_POINT('Ctrl Pts',(-10.2310626160719,82.36225161932,61.32924567366));
#121432=CARTESIAN_POINT('Ctrl Pts',(-10.2941931732499,82.6227313586901,
61.49574862112));
#121433=CARTESIAN_POINT('Ctrl Pts',(-10.3879051058939,83.00658407806,61.75970657116));
#121434=CARTESIAN_POINT('Ctrl Pts',(-10.4803285035579,83.38463777582,62.03908119861));
#121435=CARTESIAN_POINT('Ctrl Pts',(-10.5704060709779,83.7545051675001,
62.33244822809));
#121436=CARTESIAN_POINT('Ctrl Pts',(-10.6577144882509,84.1159531733799,
62.6399145318601));
#121437=CARTESIAN_POINT('Ctrl Pts',(-10.7418927390509,84.46869818965,62.96159914678));
#121438=CARTESIAN_POINT('Ctrl Pts',(-10.8226586546719,84.81239048239,63.297613065143));
#121439=CARTESIAN_POINT('Ctrl Pts',(-10.8743262685519,85.03625004551,63.532334707995));
#121440=CARTESIAN_POINT('Ctrl Pts',(-10.8997056579209,85.14730307016,63.6530190115981));
#121441=CARTESIAN_POINT('Ctrl Pts',(-10.9000935484179,85.14900063192,63.654864808037));
#121442=CARTESIAN_POINT('Ctrl Pts',(-10.7444499634089,82.08330821913,61.26232339111));
#121443=CARTESIAN_POINT('Ctrl Pts',(-10.7758793664039,82.21370125987,61.34109026097));
#121444=CARTESIAN_POINT('Ctrl Pts',(-10.8391966950829,82.47465383373,61.5047240749901));
#121445=CARTESIAN_POINT('Ctrl Pts',(-10.9333652704749,82.86001665981,61.76490805656));
#121446=CARTESIAN_POINT('Ctrl Pts',(-11.0264060300299,83.24030836404,62.04107449498));
#121447=CARTESIAN_POINT('Ctrl Pts',(-11.1172082967379,83.61293379475,62.3317633769501));
#121448=CARTESIAN_POINT('Ctrl Pts',(-11.2053255419869,83.97757037,62.63708798503));
#121449=CARTESIAN_POINT('Ctrl Pts',(-11.2903576554999,84.33378428946,62.9571076));
#121450=CARTESIAN_POINT('Ctrl Pts',(-11.3719979235199,84.6811296404201,
63.291900810757));
#121451=CARTESIAN_POINT('Ctrl Pts',(-11.4242452127629,84.9074793665401,
63.526053666644));
#121452=CARTESIAN_POINT('Ctrl Pts',(-11.4499125748089,85.01978652385,63.646508605745));
#121453=CARTESIAN_POINT('Ctrl Pts',(-11.4503048673419,85.0215032608,63.648350908626));
#121454=CARTESIAN_POINT('Ctrl Pts',(-11.0477573137059,81.77845564567,61.6285201490101));
#121455=CARTESIAN_POINT('Ctrl Pts',(-11.0792192451059,81.9049119093501,
61.70398277631));
#121456=CARTESIAN_POINT('Ctrl Pts',(-11.1426405633259,82.15817371936,61.86090998634));
#121457=CARTESIAN_POINT('Ctrl Pts',(-11.2370633855929,82.53266234296,62.11089922386));
#121458=CARTESIAN_POINT('Ctrl Pts',(-11.3304478762849,82.90266797425,62.3767193705));
#121459=CARTESIAN_POINT('Ctrl Pts',(-11.4216536368169,83.2655510331,62.65693374751));
#121460=CARTESIAN_POINT('Ctrl Pts',(-11.5102212165679,83.62094552581,62.9516559917));
#121461=CARTESIAN_POINT('Ctrl Pts',(-11.5957287387605,83.9683415161201,
63.2609080093));
#121462=CARTESIAN_POINT('Ctrl Pts',(-11.6778558235873,84.3072494738502,
63.584746703615));
#121463=CARTESIAN_POINT('Ctrl Pts',(-11.730425861083,84.52816616381,63.81140761883));
#121464=CARTESIAN_POINT('Ctrl Pts',(-11.7562535588696,84.6377886984001,
63.9280461233941));
#121465=CARTESIAN_POINT('Ctrl Pts',(-11.7566483023413,84.63946440061,63.929830064275));
#121466=CARTESIAN_POINT('Ctrl Pts',(-10.9126225976289,81.5153741101001,
62.10972407656));
#121467=CARTESIAN_POINT('Ctrl Pts',(-10.9440700364139,81.63643508906,62.18223294764));
#121468=CARTESIAN_POINT('Ctrl Pts',(-11.0074450234219,81.8788375096601,
62.33297186689));
#121469=CARTESIAN_POINT('Ctrl Pts',(-11.1017545692409,82.23713016388,62.57296683459));
#121470=CARTESIAN_POINT('Ctrl Pts',(-11.1949859149149,82.5910062086201,
62.82802226324));
#121471=CARTESIAN_POINT('Ctrl Pts',(-11.2860119039269,82.93797392928,63.096768725873));
#121472=CARTESIAN_POINT('Ctrl Pts',(-11.3743788428919,83.2776982057901,
63.379313927409));
#121473=CARTESIAN_POINT('Ctrl Pts',(-11.4596745528199,83.6097164751,63.675689054981));
#121474=CARTESIAN_POINT('Ctrl Pts',(-11.5415847426359,83.93357647935,63.9859541283691));
#121475=CARTESIAN_POINT('Ctrl Pts',(-11.5940109837696,84.14466556495,64.203065790909));
#121476=CARTESIAN_POINT('Ctrl Pts',(-11.619767246015,84.2494083216699,64.314779476617));
#121477=CARTESIAN_POINT('Ctrl Pts',(-11.620160897502,84.2510094303001,64.31648809182));
#121478=CARTESIAN_POINT('Ctrl Pts',(-10.7774878815529,81.25229257453,62.59092800412));
#121479=CARTESIAN_POINT('Ctrl Pts',(-10.8089208277219,81.3679582687801,
62.6604831189601));
#121480=CARTESIAN_POINT('Ctrl Pts',(-10.8722494835169,81.59950129996,62.80503374744));
#121481=CARTESIAN_POINT('Ctrl Pts',(-10.9664457528889,81.9415979848,63.035034445325));
#121482=CARTESIAN_POINT('Ctrl Pts',(-11.0595239535449,82.27934444298,63.279325155982));
#121483=CARTESIAN_POINT('Ctrl Pts',(-11.1503701710379,82.6103968254701,
63.536603704234));
#121484=CARTESIAN_POINT('Ctrl Pts',(-11.2385364692169,82.9344508857701,
63.8069718631161));
#121485=CARTESIAN_POINT('Ctrl Pts',(-11.3236203668789,83.2510914340801,
64.090470100661));
#121486=CARTESIAN_POINT('Ctrl Pts',(-11.4053136616849,83.55990348484,64.387161553123));
#121487=CARTESIAN_POINT('Ctrl Pts',(-11.4575961064559,83.7611649660901,
64.5947239629891));
#121488=CARTESIAN_POINT('Ctrl Pts',(-11.4832809331599,83.8610279449301,
64.701512829841));
#121489=CARTESIAN_POINT('Ctrl Pts',(-11.4836734926629,83.86255445999,64.703146119366));
#121490=CARTESIAN_POINT('Ctrl Pts',(-10.2916779629739,81.20184743248,62.87460831108));
#121491=CARTESIAN_POINT('Ctrl Pts',(-10.3230588081249,81.3141634466501,
62.9434785522));
#121492=CARTESIAN_POINT('Ctrl Pts',(-10.3862209030019,81.53873138438,63.086378354437));
#121493=CARTESIAN_POINT('Ctrl Pts',(-10.4800099430289,81.86982923944,63.313076303186));
#121494=CARTESIAN_POINT('Ctrl Pts',(-10.5725375866489,82.19607838981,63.5531753043091));
#121495=CARTESIAN_POINT('Ctrl Pts',(-10.6627375247109,82.51537911082,63.805440673177));
#121496=CARTESIAN_POINT('Ctrl Pts',(-10.7501825183529,82.82751226324,64.069965817418));
#121497=CARTESIAN_POINT('Ctrl Pts',(-10.8345049499589,83.13220277182,64.3468411136921));
#121498=CARTESIAN_POINT('Ctrl Pts',(-10.9154185062159,83.42912960561,64.636155592722));
#121499=CARTESIAN_POINT('Ctrl Pts',(-10.9671840024129,83.6225517154301,
64.838313456043));
#121500=CARTESIAN_POINT('Ctrl Pts',(-10.9926120180209,83.7185090637701,
64.942267675345));
#121501=CARTESIAN_POINT('Ctrl Pts',(-10.9930006518329,83.7199758732201,
64.943857597795));
#121502=CARTESIAN_POINT('Ctrl Pts',(-9.77071511647392,81.39680163372,62.77652121756));
#121503=CARTESIAN_POINT('Ctrl Pts',(-9.80204009060491,81.50998911196,62.84742027707));
#121504=CARTESIAN_POINT('Ctrl Pts',(-9.86502357231191,81.73599641365,62.994278890954));
#121505=CARTESIAN_POINT('Ctrl Pts',(-9.95837591611191,82.06843606335,63.226510670207));
#121506=CARTESIAN_POINT('Ctrl Pts',(-10.0503131647039,82.39528741943,63.471713388376));
#121507=CARTESIAN_POINT('Ctrl Pts',(-10.1398200589239,82.71463258723,63.728676256591));
#121508=CARTESIAN_POINT('Ctrl Pts',(-10.2264915548459,83.02633649328,63.997487316694));
#121509=CARTESIAN_POINT('Ctrl Pts',(-10.3099974211469,83.33026591704,64.278295067199));
#121510=CARTESIAN_POINT('Ctrl Pts',(-10.3900748174189,83.62618944315,64.57122039344));
#121511=CARTESIAN_POINT('Ctrl Pts',(-10.4412859589379,83.8188519043601,
64.775628543979));
#121512=CARTESIAN_POINT('Ctrl Pts',(-10.4664385807459,83.91441438601,64.880679324874));
#121513=CARTESIAN_POINT('Ctrl Pts',(-10.4668230048079,83.91587515524,64.882286004762));
#121514=CARTESIAN_POINT('Origin',(-10.0948816704592,81.9241950980305,62.1047057712127));
#121515=CARTESIAN_POINT('Ctrl Pts',(-8.7885046972379,74.82640395806,59.1949076002999));
#121516=CARTESIAN_POINT('Ctrl Pts',(-8.78188852469191,75.41917609617,59.18747495118));
#121517=CARTESIAN_POINT('Ctrl Pts',(-8.83939730075691,76.54805897963,59.2464797348));
#121518=CARTESIAN_POINT('Ctrl Pts',(-9.08760907888691,78.10809237206,59.52130962476));
#121519=CARTESIAN_POINT('Ctrl Pts',(-9.4057436642799,79.44978989415,59.90923180518));
#121520=CARTESIAN_POINT('Ctrl Pts',(-9.71792425590291,80.60886585816,60.36713913228));
#121521=CARTESIAN_POINT('Ctrl Pts',(-9.9935632318369,81.61530137155,60.86767974539));
#121522=CARTESIAN_POINT('Ctrl Pts',(-10.1509566002329,82.23504579931,61.23828496981));
#121523=CARTESIAN_POINT('Ctrl Pts',(-10.2198405635139,82.52601067952,61.42758786454));
#121524=CARTESIAN_POINT('Ctrl Pts',(-10.2212128295729,82.53181579063,61.43137091566));
#121525=CARTESIAN_POINT('Ctrl Pts',(-9.36212373100291,74.83407745381,59.25507590285));
#121526=CARTESIAN_POINT('Ctrl Pts',(-9.35580368689491,75.39892771435,59.2482959049099));
#121527=CARTESIAN_POINT('Ctrl Pts',(-9.41070341492091,76.47682878814,59.30190722458));
#121528=CARTESIAN_POINT('Ctrl Pts',(-9.6491407943599,77.97728162386,59.55440424595));
#121529=CARTESIAN_POINT('Ctrl Pts',(-9.96067084052391,79.29224334994,59.91952962683));
#121530=CARTESIAN_POINT('Ctrl Pts',(-10.2718202607539,80.4478475221001,
60.36120446053));
#121531=CARTESIAN_POINT('Ctrl Pts',(-10.5499421585019,81.46357762313,60.85287618631));
#121532=CARTESIAN_POINT('Ctrl Pts',(-10.7105860042159,82.09595442055,61.22299843353));
#121533=CARTESIAN_POINT('Ctrl Pts',(-10.7810231783999,82.39342460616,61.41298176732));
#121534=CARTESIAN_POINT('Ctrl Pts',(-10.7824264415109,82.39935974081,61.41677874076));
#121535=CARTESIAN_POINT('Ctrl Pts',(-9.69865424998491,74.84406498959,59.72344078078));
#121536=CARTESIAN_POINT('Ctrl Pts',(-9.69250793835691,75.3737935536399,
59.71728021895));
#121537=CARTESIAN_POINT('Ctrl Pts',(-9.74587699142391,76.38610626559,59.76584842462));
#121538=CARTESIAN_POINT('Ctrl Pts',(-9.97857993167891,77.8023554124599,
59.99650618733));
#121539=CARTESIAN_POINT('Ctrl Pts',(-10.2862352301719,79.05940149627,60.33596972221));
#121540=CARTESIAN_POINT('Ctrl Pts',(-10.5967796833019,80.17658751631,60.75367197684));
#121541=CARTESIAN_POINT('Ctrl Pts',(-10.8763582603389,81.16624364348,61.22439153817));
#121542=CARTESIAN_POINT('Ctrl Pts',(-11.0389090944099,81.78665342459,61.58260102151));
#121543=CARTESIAN_POINT('Ctrl Pts',(-11.1102575055659,82.07884520387,61.76704808987));
#121544=CARTESIAN_POINT('Ctrl Pts',(-11.1116789540119,82.0846751666,61.7707346179));
#121545=CARTESIAN_POINT('Ctrl Pts',(-9.57270218658391,74.84967733165,60.28631102629));
#121546=CARTESIAN_POINT('Ctrl Pts',(-9.5664908527279,75.36060742374,60.28032181312));
#121547=CARTESIAN_POINT('Ctrl Pts',(-9.6204327859899,76.33665356348,60.32757492156));
#121548=CARTESIAN_POINT('Ctrl Pts',(-9.85528193411291,77.70047199869,60.55151405767));
#121549=CARTESIAN_POINT('Ctrl Pts',(-10.1643874204399,78.90721206905,60.87963793133));
#121550=CARTESIAN_POINT('Ctrl Pts',(-10.4751582924239,79.97676444833,61.28168335215));
#121551=CARTESIAN_POINT('Ctrl Pts',(-10.7541916833579,80.9224412974,61.73340035542));
#121552=CARTESIAN_POINT('Ctrl Pts',(-10.9160287957759,81.51429968327,62.07624595922));
#121553=CARTESIAN_POINT('Ctrl Pts',(-10.9870361615569,81.7929646003,62.25264801673));
#121554=CARTESIAN_POINT('Ctrl Pts',(-10.9884508038439,81.7985246354,62.25617370333));
#121555=CARTESIAN_POINT('Ctrl Pts',(-9.44675012318391,74.8552896737,60.8491812718));
#121556=CARTESIAN_POINT('Ctrl Pts',(-9.44047376709891,75.34742129385,60.84336340728));
#121557=CARTESIAN_POINT('Ctrl Pts',(-9.49498858055591,76.28720086137,60.8893014185));
#121558=CARTESIAN_POINT('Ctrl Pts',(-9.73198393654791,77.59858858492,61.1065219280101));
#121559=CARTESIAN_POINT('Ctrl Pts',(-10.0425396107069,78.75502264184,61.42330614045));
#121560=CARTESIAN_POINT('Ctrl Pts',(-10.3535369015469,79.77694138035,61.80969472745));
#121561=CARTESIAN_POINT('Ctrl Pts',(-10.6320251063769,80.67863895132,62.24240917267));
#121562=CARTESIAN_POINT('Ctrl Pts',(-10.7931484971409,81.24194594195,62.56989089692));
#121563=CARTESIAN_POINT('Ctrl Pts',(-10.8638148175489,81.50708399673,62.73824794359));
#121564=CARTESIAN_POINT('Ctrl Pts',(-10.8652226536749,81.5123741042,62.7416127887499));
#121565=CARTESIAN_POINT('Ctrl Pts',(-8.94267290203492,74.85276791002,61.1295699342099));
#121566=CARTESIAN_POINT('Ctrl Pts',(-8.93613631818291,75.35501471312,61.1233605687));
#121567=CARTESIAN_POINT('Ctrl Pts',(-8.99294387579391,76.31213933141,61.17259229662));
#121568=CARTESIAN_POINT('Ctrl Pts',(-9.23852864643191,77.63798521846,61.4027146666999));
#121569=CARTESIAN_POINT('Ctrl Pts',(-9.55488816876592,78.7854157547301,
61.73007623355));
#121570=CARTESIAN_POINT('Ctrl Pts',(-9.86679161853491,79.78238838433,62.11961002449));
#121571=CARTESIAN_POINT('Ctrl Pts',(-10.1430979147219,80.6516568541701,
62.54799863672));
#121572=CARTESIAN_POINT('Ctrl Pts',(-10.3013648947369,81.18895060113,62.86695544977));
#121573=CARTESIAN_POINT('Ctrl Pts',(-10.3706663053529,81.44137306437,63.030146951985));
#121574=CARTESIAN_POINT('Ctrl Pts',(-10.3720469023069,81.44640927474,63.033408284556));
#121575=CARTESIAN_POINT('Ctrl Pts',(-8.39808036489391,74.84380101246,60.93968441354));
#121576=CARTESIAN_POINT('Ctrl Pts',(-8.39126263741091,75.37830192689,60.9327829084));
#121577=CARTESIAN_POINT('Ctrl Pts',(-8.4505472189839,76.39476622932,60.98771117323));
#121578=CARTESIAN_POINT('Ctrl Pts',(-8.70541178033391,77.79227568178,61.2417147644));
#121579=CARTESIAN_POINT('Ctrl Pts',(-9.0280416363969,78.97803537179,61.59448643167));
#121580=CARTESIAN_POINT('Ctrl Pts',(-9.3409240778179,79.9894572848,62.00386093824));
#121581=CARTESIAN_POINT('Ctrl Pts',(-9.61487309398091,80.85956648621,62.44549770459));
#121582=CARTESIAN_POINT('Ctrl Pts',(-9.7700540786129,81.39080772377,62.76847820377));
#121583=CARTESIAN_POINT('Ctrl Pts',(-9.83788087451691,81.63984223761,62.93284329357));
#121584=CARTESIAN_POINT('Ctrl Pts',(-9.8392320429429,81.64481063107,62.9361277708));
#121585=CARTESIAN_POINT('Ctrl Pts',(-9.07717754188791,74.99992957401,59.27469685199));
#121586=CARTESIAN_POINT('Ctrl Pts',(-9.16720240147935,74.999881575874,59.3170480141486));
#121587=CARTESIAN_POINT('Ctrl Pts',(-9.2540427904884,74.9999918735864,59.3767114129878));
#121588=CARTESIAN_POINT('Ctrl Pts',(-9.40351821239664,75.0001891988783,
59.5255401835567));
#121589=CARTESIAN_POINT('Ctrl Pts',(-9.46580962876118,75.000275896729,59.6145335066942));
#121590=CARTESIAN_POINT('Ctrl Pts',(-9.5544246386494,75.0004147462713,59.8054548367023));
#121591=CARTESIAN_POINT('Ctrl Pts',(-9.58072200049164,75.0004668731721,
59.9070017703396));
#121592=CARTESIAN_POINT('Ctrl Pts',(-9.59905684910332,75.0005382403778,
60.1039339215822));
#121593=CARTESIAN_POINT('Ctrl Pts',(-9.59135343873588,75.000557729544,60.199126681737));
#121594=CARTESIAN_POINT('Ctrl Pts',(-9.55275050059052,75.0005744561138,
60.3716696675297));
#121595=CARTESIAN_POINT('Ctrl Pts',(-9.51915258821925,75.0005694408721,
60.4610758883646));
#121596=CARTESIAN_POINT('Ctrl Pts',(-9.418642837365,75.000528745341,60.6314235011406));
#121597=CARTESIAN_POINT('Ctrl Pts',(-9.35157790424357,75.0004929319658,
60.7120836753024));
#121598=CARTESIAN_POINT('Ctrl Pts',(-9.190050282834,75.0003967133209,60.8470403630041));
#121599=CARTESIAN_POINT('Ctrl Pts',(-9.09577378900069,75.0003364917561,
60.9010033430406));
#121600=CARTESIAN_POINT('Ctrl Pts',(-8.89712916494734,75.0002078724708,
60.9719435463236));
#121601=CARTESIAN_POINT('Ctrl Pts',(-8.79314519935575,75.0001398318208,
60.9889116321));
#121602=CARTESIAN_POINT('Ctrl Pts',(-8.69365830054191,74.99999996484,60.98889557741));
#121603=CARTESIAN_POINT('Ctrl Pts',(-10.2211075019859,67.46805497937,61.43143799722));
#121604=CARTESIAN_POINT('Ctrl Pts',(-10.2201352975039,67.47216669351,61.42875836433));
#121605=CARTESIAN_POINT('Ctrl Pts',(-10.1636464373649,67.71082606018,61.27340384402));
#121606=CARTESIAN_POINT('Ctrl Pts',(-10.0368070785259,68.21698868467,60.96586480023));
#121607=CARTESIAN_POINT('Ctrl Pts',(-9.8163009649119,69.03334101746,60.53842192908));
#121608=CARTESIAN_POINT('Ctrl Pts',(-9.5624403228119,69.96232137517,60.13185886181));
#121609=CARTESIAN_POINT('Ctrl Pts',(-9.2889829848119,71.02203085471,59.76217395547));
#121610=CARTESIAN_POINT('Ctrl Pts',(-9.02433492377792,72.23936277407,59.45104885171));
#121611=CARTESIAN_POINT('Ctrl Pts',(-8.8268115228959,73.64000933415,59.23360212871));
#121612=CARTESIAN_POINT('Ctrl Pts',(-8.78269423684091,74.64578270171,59.1882690656));
#121613=CARTESIAN_POINT('Ctrl Pts',(-8.78852660744491,75.17354115938,59.19489180673));
#121614=CARTESIAN_POINT('Ctrl Pts',(-10.7823632829819,67.60046014905,61.41677523848));
#121615=CARTESIAN_POINT('Ctrl Pts',(-10.7813689778119,67.60466446032,61.41408541359));
#121616=CARTESIAN_POINT('Ctrl Pts',(-10.7235979843399,67.84869045929,61.25815041502));
#121617=CARTESIAN_POINT('Ctrl Pts',(-10.5941274714749,68.3652544873801,
60.95074940909));
#121618=CARTESIAN_POINT('Ctrl Pts',(-10.3707860974499,69.19221319007,60.52861635201));
#121619=CARTESIAN_POINT('Ctrl Pts',(-10.1166516420119,70.12249423931,60.13360637521));
#121620=CARTESIAN_POINT('Ctrl Pts',(-9.8458315563439,71.1722927941801,59.7802070981001));
#121621=CARTESIAN_POINT('Ctrl Pts',(-9.58828414872691,72.3577590955501,
59.48963830056));
#121622=CARTESIAN_POINT('Ctrl Pts',(-9.39873529479691,73.70268390503,59.2901244165301));
#121623=CARTESIAN_POINT('Ctrl Pts',(-9.3566156200659,74.66287447499,59.24892709458));
#121624=CARTESIAN_POINT('Ctrl Pts',(-9.36218740473191,75.16597612265,59.25497557749));
#121625=CARTESIAN_POINT('Ctrl Pts',(-11.1116903071099,67.9151459000001,
61.77071136858));
#121626=CARTESIAN_POINT('Ctrl Pts',(-11.1106830339599,67.9192760147101,
61.76809958451));
#121627=CARTESIAN_POINT('Ctrl Pts',(-11.0521597254649,68.1589905993,61.61669524768));
#121628=CARTESIAN_POINT('Ctrl Pts',(-10.9211453351839,68.6658303921001,
61.31902498468));
#121629=CARTESIAN_POINT('Ctrl Pts',(-10.6961403206129,69.47345397702,60.91344584111));
#121630=CARTESIAN_POINT('Ctrl Pts',(-10.4418452002249,70.37535814882,60.53803008547));
#121631=CARTESIAN_POINT('Ctrl Pts',(-10.1725725702669,71.38604201504,60.20586917915));
#121632=CARTESIAN_POINT('Ctrl Pts',(-9.91919160001691,72.51445318339,59.93722926335));
#121633=CARTESIAN_POINT('Ctrl Pts',(-9.73432195636091,73.7824508557801,
59.75515226462));
#121634=CARTESIAN_POINT('Ctrl Pts',(-9.69337441635991,74.68410470834,59.71782522354));
#121635=CARTESIAN_POINT('Ctrl Pts',(-9.69879329749291,75.15605350359,59.723326013));
#121636=CARTESIAN_POINT('Ctrl Pts',(-10.9885018319529,68.2013323702401,
62.25617620429));
#121637=CARTESIAN_POINT('Ctrl Pts',(-10.9874994096209,68.20527119236,62.25367842127));
#121638=CARTESIAN_POINT('Ctrl Pts',(-10.9292575130169,68.43388414708,62.10888120075));
#121639=CARTESIAN_POINT('Ctrl Pts',(-10.7988206274369,68.91738746191,61.82401663069));
#121640=CARTESIAN_POINT('Ctrl Pts',(-10.5744379163129,69.68868530886,61.43514751277));
#121641=CARTESIAN_POINT('Ctrl Pts',(-10.3202028944559,70.55154216846,61.0742426913));
#121642=CARTESIAN_POINT('Ctrl Pts',(-10.0503514212949,71.52010701642,60.75404721078));
#121643=CARTESIAN_POINT('Ctrl Pts',(-9.7954119483149,72.60448967147,60.49402055406));
#121644=CARTESIAN_POINT('Ctrl Pts',(-9.60879199345991,73.82588143466,60.31720507579));
#121645=CARTESIAN_POINT('Ctrl Pts',(-9.56740600328791,74.6952531657101,
60.28089050002));
#121646=CARTESIAN_POINT('Ctrl Pts',(-9.57288207970592,75.15041957795,60.28623701169));
#121647=CARTESIAN_POINT('Ctrl Pts',(-10.8653133567959,68.4875188404901,
62.74164103999));
#121648=CARTESIAN_POINT('Ctrl Pts',(-10.8643157852829,68.49126637,62.73925725804));
#121649=CARTESIAN_POINT('Ctrl Pts',(-10.8063553005689,68.7087776948599,
62.60106715382));
#121650=CARTESIAN_POINT('Ctrl Pts',(-10.6764959196909,69.16894453172,62.32900827669));
#121651=CARTESIAN_POINT('Ctrl Pts',(-10.4527355120119,69.9039166407,61.95684918442));
#121652=CARTESIAN_POINT('Ctrl Pts',(-10.1985605886859,70.7277261881,61.6104552971401));
#121653=CARTESIAN_POINT('Ctrl Pts',(-9.92813027232292,71.65417201779,61.30222524241));
#121654=CARTESIAN_POINT('Ctrl Pts',(-9.67163229661291,72.69452615956,61.05081184478));
#121655=CARTESIAN_POINT('Ctrl Pts',(-9.48326203055891,73.86931201353,60.87925788696));
#121656=CARTESIAN_POINT('Ctrl Pts',(-9.44143759021592,74.7064016230801,
60.84395577649));
#121657=CARTESIAN_POINT('Ctrl Pts',(-9.44697086191892,75.14478565231,60.84914801039));
#121658=CARTESIAN_POINT('Ctrl Pts',(-10.3721223328469,68.5535152893101,
63.0334650724921));
#121659=CARTESIAN_POINT('Ctrl Pts',(-10.3711441818219,68.55708256,63.031154892722));
#121660=CARTESIAN_POINT('Ctrl Pts',(-10.3143103432349,68.76413802923,62.89722284264));
#121661=CARTESIAN_POINT('Ctrl Pts',(-10.1867630303869,69.20298716651,62.63246721916));
#121662=CARTESIAN_POINT('Ctrl Pts',(-9.96549404468091,69.90897428286,62.26598171184));
#121663=CARTESIAN_POINT('Ctrl Pts',(-9.71155972872991,70.7092203882,61.9192958937501));
#121664=CARTESIAN_POINT('Ctrl Pts',(-9.43881198558591,71.61875463628,61.60574375038));
#121665=CARTESIAN_POINT('Ctrl Pts',(-9.17607446874791,72.6575976508201,
61.34385873668));
#121666=CARTESIAN_POINT('Ctrl Pts',(-8.98069674707291,73.847315957,61.16186671212));
#121667=CARTESIAN_POINT('Ctrl Pts',(-8.93711695024591,74.70000094919,61.12404109137));
#121668=CARTESIAN_POINT('Ctrl Pts',(-8.94287920604192,75.1472140833999,
61.12957580005));
#121669=CARTESIAN_POINT('Ctrl Pts',(-9.83927335193191,68.35511659356,62.93618146194));
#121670=CARTESIAN_POINT('Ctrl Pts',(-9.83831618301491,68.35863537848,62.93385518594));
#121671=CARTESIAN_POINT('Ctrl Pts',(-9.78269958523491,68.56288420959,62.7989800378801));
#121672=CARTESIAN_POINT('Ctrl Pts',(-9.65765025599492,68.99671324753,62.53113343182));
#121673=CARTESIAN_POINT('Ctrl Pts',(-9.43907302986091,69.70047057283,62.15548484121));
#121674=CARTESIAN_POINT('Ctrl Pts',(-9.18539866875291,70.5084201503,61.79389976569));
#121675=CARTESIAN_POINT('Ctrl Pts',(-8.91014715234592,71.4375778106,61.4613028108201));
#121676=CARTESIAN_POINT('Ctrl Pts',(-8.64066836697291,72.5184392530701,
61.17687530567));
#121677=CARTESIAN_POINT('Ctrl Pts',(-8.4377197135399,73.77462645762,60.97573715526));
#121678=CARTESIAN_POINT('Ctrl Pts',(-8.39224341035191,74.68033838347,60.93354232265));
#121679=CARTESIAN_POINT('Ctrl Pts',(-8.39825306306791,75.15607828224,60.93968686544));
#121680=CARTESIAN_POINT('Origin',(-10.0948464627305,68.0757372670146,62.1047362602089));
#121681=CARTESIAN_POINT('Ctrl Pts',(-11.6237407641905,61.21249245617,73.1626298883762));
#121682=CARTESIAN_POINT('Ctrl Pts',(-11.6250359865815,61.20366449265,72.4606436349265));
#121683=CARTESIAN_POINT('Ctrl Pts',(-11.6091550238638,61.29933896423,70.962670779947));
#121684=CARTESIAN_POINT('Ctrl Pts',(-11.5165282050679,61.83819205569,68.625444675657));
#121685=CARTESIAN_POINT('Ctrl Pts',(-11.3260709964139,62.87321223361,66.244698162091));
#121686=CARTESIAN_POINT('Ctrl Pts',(-11.0228468995629,64.33705500443,64.127545184309));
#121687=CARTESIAN_POINT('Ctrl Pts',(-10.6320772268289,66.0053612858,62.46170707634));
#121688=CARTESIAN_POINT('Ctrl Pts',(-10.3400165566969,67.18512894546,61.6081075162));
#121689=CARTESIAN_POINT('Ctrl Pts',(-10.1997669692099,67.76783374115,61.24911703265));
#121690=CARTESIAN_POINT('Ctrl Pts',(-12.1814102453093,61.3021055231,73.1626457611423));
#121691=CARTESIAN_POINT('Ctrl Pts',(-12.1827146639685,61.29320969844,72.4598923200226));
#121692=CARTESIAN_POINT('Ctrl Pts',(-12.1667224102372,61.38959736518,70.961546111832));
#121693=CARTESIAN_POINT('Ctrl Pts',(-12.0733368718683,61.93301542577,68.621592685892));
#121694=CARTESIAN_POINT('Ctrl Pts',(-11.8811272628205,62.9779150684401,
66.2383521195351));
#121695=CARTESIAN_POINT('Ctrl Pts',(-11.574501834705,64.45859748606,64.119339944351));
#121696=CARTESIAN_POINT('Ctrl Pts',(-11.1791162023439,66.1463437687401,
62.45789631767));
#121697=CARTESIAN_POINT('Ctrl Pts',(-10.8850195894329,67.33344051896,61.61471183482));
#121698=CARTESIAN_POINT('Ctrl Pts',(-10.7445184442879,67.91647053246,61.26248407009));
#121699=CARTESIAN_POINT('Ctrl Pts',(-12.4918941626243,61.7739078301301,
73.1573469410713));
#121700=CARTESIAN_POINT('Ctrl Pts',(-12.4932037013295,61.76524338757,72.4756060823452));
#121701=CARTESIAN_POINT('Ctrl Pts',(-12.4771494860403,61.85911084582,71.022812237691));
#121702=CARTESIAN_POINT('Ctrl Pts',(-12.3833415285984,62.38864418025,68.752721416032));
#121703=CARTESIAN_POINT('Ctrl Pts',(-12.1901562661264,63.40750159366,66.4408047023301));
#121704=CARTESIAN_POINT('Ctrl Pts',(-11.8816371380848,64.85297076891,64.3854220064841));
#121705=CARTESIAN_POINT('Ctrl Pts',(-11.4836815583349,66.50072553144,62.77735083217));
#121706=CARTESIAN_POINT('Ctrl Pts',(-11.1884514290469,67.65591813368,61.96612394498));
#121707=CARTESIAN_POINT('Ctrl Pts',(-11.0478102285289,68.2213300947501,
61.6286814152101));
#121708=CARTESIAN_POINT('Ctrl Pts',(-12.3535426183118,62.32147807264,73.1501748512657));
#121709=CARTESIAN_POINT('Ctrl Pts',(-12.354849875526,62.31319397975,72.4975793093326));
#121710=CARTESIAN_POINT('Ctrl Pts',(-12.3388232702892,62.40294462491,71.106678664906));
#121711=CARTESIAN_POINT('Ctrl Pts',(-12.2452035426648,62.9091612469,68.933666728549));
#121712=CARTESIAN_POINT('Ctrl Pts',(-12.0524530310782,63.8829683759799,
66.720569091486));
#121713=CARTESIAN_POINT('Ctrl Pts',(-11.7447777351794,65.26404135376,64.752979132619));
#121714=CARTESIAN_POINT('Ctrl Pts',(-11.3479673232469,66.83834635544,63.212594590931));
#121715=CARTESIAN_POINT('Ctrl Pts',(-11.0532422885309,67.94312234868,62.43411232759));
#121716=CARTESIAN_POINT('Ctrl Pts',(-10.9126634966469,68.48441537841,62.10987498673));
#121717=CARTESIAN_POINT('Ctrl Pts',(-12.2151910739994,62.86904831516,73.1430027614602));
#121718=CARTESIAN_POINT('Ctrl Pts',(-12.2164960497225,62.86114457193,72.5195525363199));
#121719=CARTESIAN_POINT('Ctrl Pts',(-12.2004970545381,62.94677840401,71.190545092121));
#121720=CARTESIAN_POINT('Ctrl Pts',(-12.1070655567313,63.42967831355,69.114612041066));
#121721=CARTESIAN_POINT('Ctrl Pts',(-11.91474979603,64.35843515829,67.000333480642));
#121722=CARTESIAN_POINT('Ctrl Pts',(-11.607918332274,65.67511193861,65.120536258753));
#121723=CARTESIAN_POINT('Ctrl Pts',(-11.2122530881599,67.17596717943,63.647838349687));
#121724=CARTESIAN_POINT('Ctrl Pts',(-10.9180331480149,68.23032656369,62.90210071019));
#121725=CARTESIAN_POINT('Ctrl Pts',(-10.7775167647649,68.74750066206,62.59106855825));
#121726=CARTESIAN_POINT('Ctrl Pts',(-11.7178592045691,63.13675620992,73.1386154569617));
#121727=CARTESIAN_POINT('Ctrl Pts',(-11.7191559790235,63.12913475835,72.5335142827482));
#121728=CARTESIAN_POINT('Ctrl Pts',(-11.7032562336092,63.21172891812,71.242543117047));
#121729=CARTESIAN_POINT('Ctrl Pts',(-11.6105013649466,63.67702362726,69.227855437429));
#121730=CARTESIAN_POINT('Ctrl Pts',(-11.4197484019109,64.5709809274,67.175711181192));
#121731=CARTESIAN_POINT('Ctrl Pts',(-11.1159502589549,65.83590193446,65.350851231036));
#121732=CARTESIAN_POINT('Ctrl Pts',(-10.7244015460629,67.27755256816,63.9161937176));
#121733=CARTESIAN_POINT('Ctrl Pts',(-10.4319972678159,68.29572694252,63.182721088991));
#121734=CARTESIAN_POINT('Ctrl Pts',(-10.2917052246899,68.79794574581,62.87473770978));
#121735=CARTESIAN_POINT('Ctrl Pts',(-11.1845489919669,62.95073358981,73.1398623591238));
#121736=CARTESIAN_POINT('Ctrl Pts',(-11.1858369718499,62.94311303201,72.5303968172997));
#121737=CARTESIAN_POINT('Ctrl Pts',(-11.1700436562049,63.02571883533,71.228901597836));
#121738=CARTESIAN_POINT('Ctrl Pts',(-11.0780143658839,63.49055390038,69.199848762541));
#121739=CARTESIAN_POINT('Ctrl Pts',(-10.8889372575579,64.3825636456,67.1327996899));
#121740=CARTESIAN_POINT('Ctrl Pts',(-10.5883918740969,65.64198311034,65.294341452631));
#121741=CARTESIAN_POINT('Ctrl Pts',(-10.2012574935159,67.07712588928,63.843372013349));
#121742=CARTESIAN_POINT('Ctrl Pts',(-9.91080022709891,68.09684792052,63.093719029673));
#121743=CARTESIAN_POINT('Ctrl Pts',(-9.77074875347191,68.60298807605,62.77664792151));
#121744=CARTESIAN_POINT('Ctrl Pts',(-12.1332042595665,61.479712982889,72.9888456302782));
#121745=CARTESIAN_POINT('Ctrl Pts',(-12.154541208045,61.5021440298757,72.9888417288154));
#121746=CARTESIAN_POINT('Ctrl Pts',(-12.1748167181765,61.5257830744051,
72.9888400206132));
#121747=CARTESIAN_POINT('Ctrl Pts',(-12.1938447273005,61.5504617721141,
72.9888400652945));
#121748=CARTESIAN_POINT('Ctrl Pts',(-12.2128355979227,61.5750923024161,
72.9888401098885));
#121749=CARTESIAN_POINT('Ctrl Pts',(-12.2305831957688,61.60075779768,72.9888419004666));
#121750=CARTESIAN_POINT('Ctrl Pts',(-12.2469398266819,61.6272548217178,
72.9888449935941));
#121751=CARTESIAN_POINT('Ctrl Pts',(-12.2633575502906,61.6538508132404,
72.9888480982745));
#121752=CARTESIAN_POINT('Ctrl Pts',(-12.2783734354803,61.6812837707993,
72.9888525151648));
#121753=CARTESIAN_POINT('Ctrl Pts',(-12.2918840994421,61.7093222793794,
72.9888577913022));
#121754=CARTESIAN_POINT('Ctrl Pts',(-12.3054384234256,61.7374513950457,
72.9888630844895));
#121755=CARTESIAN_POINT('Ctrl Pts',(-12.3174775876023,61.7661890889953,
72.9888692423773));
#121756=CARTESIAN_POINT('Ctrl Pts',(-12.3279483638797,61.7952886248432,
72.9888758045281));
#121757=CARTESIAN_POINT('Ctrl Pts',(-12.3385368919628,61.8247154070003,
72.9888824404753));
#121758=CARTESIAN_POINT('Ctrl Pts',(-12.3475215770959,61.8545112926814,
72.9888894897106));
#121759=CARTESIAN_POINT('Ctrl Pts',(-12.3549010685653,61.8844216123198,
72.9888964746818));
#121760=CARTESIAN_POINT('Ctrl Pts',(-12.3610944269458,61.9095243351247,
72.9889023369326));
#121761=CARTESIAN_POINT('Ctrl Pts',(-12.366158217251,61.9347074358474,72.9889081538596));
#121762=CARTESIAN_POINT('Ctrl Pts',(-12.3701190895151,61.959827502654,72.9889136433191));
#121763=CARTESIAN_POINT('Ctrl Pts',(-12.3749397042919,61.9904001031244,
72.9889203243145));
#121764=CARTESIAN_POINT('Ctrl Pts',(-12.3781258301378,62.0208781607225,
72.9889265531504));
#121765=CARTESIAN_POINT('Ctrl Pts',(-12.3797689676216,62.0510265774712,
72.988932368569));
#121766=CARTESIAN_POINT('Ctrl Pts',(-12.3814487003365,62.0818464464216,
72.9889383135061));
#121767=CARTESIAN_POINT('Ctrl Pts',(-12.3815166075881,62.1123211758842,
72.9889438263104));
#121768=CARTESIAN_POINT('Ctrl Pts',(-12.3801113156889,62.1422366139128,
72.98894893607));
#121769=CARTESIAN_POINT('Ctrl Pts',(-12.3790019726615,62.1658519799483,
72.9889529697345));
#121770=CARTESIAN_POINT('Ctrl Pts',(-12.3769755570522,62.1891195437263,
72.9889567519603));
#121771=CARTESIAN_POINT('Ctrl Pts',(-12.374113173743,62.2119528798782,72.9889602925763));
#121772=CARTESIAN_POINT('Ctrl Pts',(-12.370364760107,62.241854112293,72.9889649291648));
#121773=CARTESIAN_POINT('Ctrl Pts',(-12.3651827094674,62.2710089869103,
72.9889692499398));
#121774=CARTESIAN_POINT('Ctrl Pts',(-12.358766718633,62.2992685082974,72.988973146793));
#121775=CARTESIAN_POINT('Ctrl Pts',(-12.3571501629764,62.3063887006933,
72.9889741286335));
#121776=CARTESIAN_POINT('Ctrl Pts',(-12.355455337204,62.3134523062013,72.9889750835445));
#121777=CARTESIAN_POINT('Ctrl Pts',(-12.3536855356837,62.3204574463092,
72.9889760097662));
#121778=CARTESIAN_POINT('Ctrl Pts',(-12.3466752021777,62.3482053987486,
72.9889796786091));
#121779=CARTESIAN_POINT('Ctrl Pts',(-12.338191440408,62.3762050445819,72.9889829510826));
#121780=CARTESIAN_POINT('Ctrl Pts',(-12.3281211515463,62.4042415517801,
72.9889858111758));
#121781=CARTESIAN_POINT('Ctrl Pts',(-12.3238100314073,62.416244062579,72.9889870355901));
#121782=CARTESIAN_POINT('Ctrl Pts',(-12.319208549409,62.4282528358705,72.9889881843647));
#121783=CARTESIAN_POINT('Ctrl Pts',(-12.314309904899,62.4402489088726,72.9889892558765));
#121784=CARTESIAN_POINT('Ctrl Pts',(-12.3032198131789,62.4674069419982,
72.9889916816831));
#121785=CARTESIAN_POINT('Ctrl Pts',(-12.2906036714925,62.4945015538455,
72.9889936107424));
#121786=CARTESIAN_POINT('Ctrl Pts',(-12.276412224394,62.521292316785,72.9889951016));
#121787=CARTESIAN_POINT('Ctrl Pts',(-12.2624553258617,62.5476402964769,
72.9889965678174));
#121788=CARTESIAN_POINT('Ctrl Pts',(-12.246974328998,62.5736936514737,72.9889976104105));
#121789=CARTESIAN_POINT('Ctrl Pts',(-12.2299687881257,62.5992042926995,
72.9889982713549));
#121790=CARTESIAN_POINT('Ctrl Pts',(-12.213285338897,62.6242317523302,72.9889989197807));
#121791=CARTESIAN_POINT('Ctrl Pts',(-12.1951343757566,62.6487360266731,
72.9889992010127));
#121792=CARTESIAN_POINT('Ctrl Pts',(-12.1755649618719,62.6724756656738,
72.9889991388274));
#121793=CARTESIAN_POINT('Ctrl Pts',(-12.1561793061432,62.6959923878149,
72.988999077226));
#121794=CARTESIAN_POINT('Ctrl Pts',(-12.1354017183969,62.7187578959313,
72.9889986787046));
#121795=CARTESIAN_POINT('Ctrl Pts',(-12.1133302921518,62.7405430183668,
72.9889979490452));
#121796=CARTESIAN_POINT('Ctrl Pts',(-12.0914627435291,62.7621269078182,
72.9889972261258));
#121797=CARTESIAN_POINT('Ctrl Pts',(-12.0683254188729,62.7827476021891,
72.9889961781443));
#121798=CARTESIAN_POINT('Ctrl Pts',(-12.0440613696876,62.8022004457818,
72.9889947931482));
#121799=CARTESIAN_POINT('Ctrl Pts',(-12.0265199799282,62.8162636348557,
72.9889937918826));
#121800=CARTESIAN_POINT('Ctrl Pts',(-12.0083907632135,62.8297168099659,
72.9889926141001));
#121801=CARTESIAN_POINT('Ctrl Pts',(-11.9897418060247,62.8424922777627,
72.9889912497166));
#121802=CARTESIAN_POINT('Ctrl Pts',(-11.9641069654802,62.8600534248304,
72.9889893742362));
#121803=CARTESIAN_POINT('Ctrl Pts',(-11.9374890967615,62.8763321193198,
72.9889872025664));
#121804=CARTESIAN_POINT('Ctrl Pts',(-11.9100952215728,62.8911856415241,
72.9889846305083));
#121805=CARTESIAN_POINT('Ctrl Pts',(-11.8826990290741,62.9060404202215,
72.9889820582326));
#121806=CARTESIAN_POINT('Ctrl Pts',(-11.8545274891427,62.9194693501063,
72.9889790853045));
#121807=CARTESIAN_POINT('Ctrl Pts',(-11.8258127212586,62.9313753840749,
72.9889755961807));
#121808=CARTESIAN_POINT('Ctrl Pts',(-11.7969005111399,62.943363283722,72.9889720830658));
#121809=CARTESIAN_POINT('Ctrl Pts',(-11.7674384630735,62.9538070397002,
72.9889680463902));
#121810=CARTESIAN_POINT('Ctrl Pts',(-11.7376762200055,62.9626590950443,
72.9889633600468));
#121811=CARTESIAN_POINT('Ctrl Pts',(-11.7077660056033,62.9715551608629,
72.988958650404));
#121812=CARTESIAN_POINT('Ctrl Pts',(-11.6775535187158,62.978843725931,72.9889532843411));
#121813=CARTESIAN_POINT('Ctrl Pts',(-11.6472912201003,62.9845296107777,
72.9889471295904));
#121814=CARTESIAN_POINT('Ctrl Pts',(-11.6166074832013,62.9902946782926,
72.9889408891275));
#121815=CARTESIAN_POINT('Ctrl Pts',(-11.5858734214282,62.9944123876513,
72.9889338375723));
#121816=CARTESIAN_POINT('Ctrl Pts',(-11.5553374658601,62.9969397578481,
72.9889258369577));
#121817=CARTESIAN_POINT('Ctrl Pts',(-11.5304153894896,62.9990024839651,
72.9889193072152));
#121818=CARTESIAN_POINT('Ctrl Pts',(-11.5056251349898,63.00000700811,72.988912145239));
#121819=CARTESIAN_POINT('Ctrl Pts',(-11.4810890049462,63.0000066826667,
72.9889042778822));
#121820=CARTESIAN_POINT('Ctrl Pts',(-10.1997576867849,67.76779559893,84.72864147799));
#121821=CARTESIAN_POINT('Ctrl Pts',(-10.3096071503739,67.31146422345,84.44751423884));
#121822=CARTESIAN_POINT('Ctrl Pts',(-10.5431181289799,66.36314644642,83.7842726899399));
#121823=CARTESIAN_POINT('Ctrl Pts',(-10.8727722357109,64.9897459741,82.539892806721));
#121824=CARTESIAN_POINT('Ctrl Pts',(-11.1574332348069,63.69898082881,80.98142837168));
#121825=CARTESIAN_POINT('Ctrl Pts',(-11.3672962669879,62.64696648581,79.225467208697));
#121826=CARTESIAN_POINT('Ctrl Pts',(-11.5032040207249,61.90938280311,77.447206492296));
#121827=CARTESIAN_POINT('Ctrl Pts',(-11.5810454885597,61.46365902169,75.7768267823979));
#121828=CARTESIAN_POINT('Ctrl Pts',(-11.6184127295029,61.24328748873,74.247983007362));
#121829=CARTESIAN_POINT('Ctrl Pts',(-11.6245351204064,61.20669260332,73.2770976585449));
#121830=CARTESIAN_POINT('Ctrl Pts',(-11.6236939394218,61.2124848047,72.8155267773184));
#121831=CARTESIAN_POINT('Ctrl Pts',(-11.6236928456892,61.21249233149,72.8149300730504));
#121832=CARTESIAN_POINT('Ctrl Pts',(-10.7445114810569,67.9164295402001,
84.71528553673));
#121833=CARTESIAN_POINT('Ctrl Pts',(-10.8545618554429,67.45983386763,84.43944843073));
#121834=CARTESIAN_POINT('Ctrl Pts',(-11.0894328441589,66.5068038019001,
83.78520548561));
#121835=CARTESIAN_POINT('Ctrl Pts',(-11.4226175304349,65.11912432056,82.54699405835));
#121836=CARTESIAN_POINT('Ctrl Pts',(-11.7106257883405,63.81306197145,80.989105717709));
#121837=CARTESIAN_POINT('Ctrl Pts',(-11.9227252329622,62.74954121041,79.231327320835));
#121838=CARTESIAN_POINT('Ctrl Pts',(-12.0598976401354,62.00485586623,77.450888058051));
#121839=CARTESIAN_POINT('Ctrl Pts',(-12.1383713127295,61.55537167225,75.779454975613));
#121840=CARTESIAN_POINT('Ctrl Pts',(-12.1760508898936,61.33310788978,74.248646493056));
#121841=CARTESIAN_POINT('Ctrl Pts',(-12.1822137575716,61.2962518831,73.2775160011898));
#121842=CARTESIAN_POINT('Ctrl Pts',(-12.1813663982192,61.30208713828,72.8155200043769));
#121843=CARTESIAN_POINT('Ctrl Pts',(-12.1813652964467,61.30209472109,72.8149227500128));
#121844=CARTESIAN_POINT('Ctrl Pts',(-11.0478118783009,68.22129063266,84.34909471137));
#121845=CARTESIAN_POINT('Ctrl Pts',(-11.1579741129899,67.77848669656,84.08483280083));
#121846=CARTESIAN_POINT('Ctrl Pts',(-11.3936023091109,66.8517673089299,
83.45593242299));
#121847=CARTESIAN_POINT('Ctrl Pts',(-11.7287527020768,65.49798356831,82.2592195154991));
#121848=CARTESIAN_POINT('Ctrl Pts',(-12.0186245999192,64.22271758572,80.749267626391));
#121849=CARTESIAN_POINT('Ctrl Pts',(-12.2319692029754,63.18483956493,79.044107978404));
#121850=CARTESIAN_POINT('Ctrl Pts',(-12.3698457261984,62.4586779496,77.316764725178));
#121851=CARTESIAN_POINT('Ctrl Pts',(-12.4486713889145,62.0206875690101,
75.6957671382841));
#121852=CARTESIAN_POINT('Ctrl Pts',(-12.4865248642707,61.80408781319,74.210555691052));
#121853=CARTESIAN_POINT('Ctrl Pts',(-12.4927102680409,61.76820235719,73.2689474092427));
#121854=CARTESIAN_POINT('Ctrl Pts',(-12.4918594687833,61.7738849678301,
72.8208124201688));
#121855=CARTESIAN_POINT('Ctrl Pts',(-12.4918583625345,61.77389235232,72.8202330845845));
#121856=CARTESIAN_POINT('Ctrl Pts',(-10.9126738311849,68.48438020148,83.8678996071999));
#121857=CARTESIAN_POINT('Ctrl Pts',(-11.0227862255739,68.06046669184,83.61398019171));
#121858=CARTESIAN_POINT('Ctrl Pts',(-11.2580770415569,67.17399290633,83.0103070625101));
#121859=CARTESIAN_POINT('Ctrl Pts',(-11.592351597347,65.88026532928,81.863470621288));
#121860=CARTESIAN_POINT('Ctrl Pts',(-11.8813931347155,64.66188791271,80.4176821685851));
#121861=CARTESIAN_POINT('Ctrl Pts',(-12.0941829469415,63.67014755444,78.785402860033));
#121862=CARTESIAN_POINT('Ctrl Pts',(-12.2317457453268,62.97610441922,77.131945812737));
#121863=CARTESIAN_POINT('Ctrl Pts',(-12.3104145758787,62.55739717061,75.58011615866));
#121864=CARTESIAN_POINT('Ctrl Pts',(-12.3481905694304,62.35033909216,74.158449502137));
#121865=CARTESIAN_POINT('Ctrl Pts',(-12.3543659320548,62.31602551352,73.2569569413241));
#121866=CARTESIAN_POINT('Ctrl Pts',(-12.353516665476,62.32145891959,72.8279667500161));
#121867=CARTESIAN_POINT('Ctrl Pts',(-12.3535155612216,62.32146598023,72.8274121643456));
#121868=CARTESIAN_POINT('Ctrl Pts',(-10.7775357840699,68.74746977031,83.38670450304));
#121869=CARTESIAN_POINT('Ctrl Pts',(-10.8875983381589,68.34244668712,83.14312758258));
#121870=CARTESIAN_POINT('Ctrl Pts',(-11.1225517740029,67.49621850373,82.564681702032));
#121871=CARTESIAN_POINT('Ctrl Pts',(-11.4559504926169,66.26254709025,81.467721727077));
#121872=CARTESIAN_POINT('Ctrl Pts',(-11.7441616695118,65.1010582397,80.086096710779));
#121873=CARTESIAN_POINT('Ctrl Pts',(-11.9563966909076,64.15545554395,78.526697741661));
#121874=CARTESIAN_POINT('Ctrl Pts',(-12.0936457644551,63.49353088885,76.9471269002951));
#121875=CARTESIAN_POINT('Ctrl Pts',(-12.1721577628428,63.09410677221,75.464465179036));
#121876=CARTESIAN_POINT('Ctrl Pts',(-12.2098562745902,62.89659037114,74.106343313221));
#121877=CARTESIAN_POINT('Ctrl Pts',(-12.2160215960688,62.8638486698501,
73.2449664734054));
#121878=CARTESIAN_POINT('Ctrl Pts',(-12.2151738621687,62.86903287134,72.8351210798634));
#121879=CARTESIAN_POINT('Ctrl Pts',(-12.2151727599088,62.86903960813,72.8345912441068));
#121880=CARTESIAN_POINT('Ctrl Pts',(-10.2917276399139,68.79791856628,83.10302775846));
#121881=CARTESIAN_POINT('Ctrl Pts',(-10.4016110229669,68.40461580073,82.861843474006));
#121882=CARTESIAN_POINT('Ctrl Pts',(-10.6353516100079,67.58642976082,82.292125137501));
#121883=CARTESIAN_POINT('Ctrl Pts',(-10.9656017791049,66.39997015062,81.2210262182501));
#121884=CARTESIAN_POINT('Ctrl Pts',(-11.2508278908059,65.28451454765,79.878119282303));
#121885=CARTESIAN_POINT('Ctrl Pts',(-11.4610684930919,64.37557932713,78.364528519757));
#121886=CARTESIAN_POINT('Ctrl Pts',(-11.5971897563413,63.73850785712,76.831647075385));
#121887=CARTESIAN_POINT('Ctrl Pts',(-11.6751379583426,63.35363234109,75.391963104124));
#121888=CARTESIAN_POINT('Ctrl Pts',(-11.7125579305342,63.16333821796,74.074063236392));
#121889=CARTESIAN_POINT('Ctrl Pts',(-11.7186871550696,63.13174883075,73.2373415999963));
#121890=CARTESIAN_POINT('Ctrl Pts',(-11.7178449310008,63.13674911897,72.8394907884618));
#121891=CARTESIAN_POINT('Ctrl Pts',(-11.7178438359108,63.1367556167101,
72.8389764593828));
#121892=CARTESIAN_POINT('Ctrl Pts',(-9.77076807637092,68.60296152033,83.20110941226));
#121893=CARTESIAN_POINT('Ctrl Pts',(-9.88045932418391,68.20659694811,82.952813955229));
#121894=CARTESIAN_POINT('Ctrl Pts',(-10.1128993048199,67.38603701235,82.369655164651));
#121895=CARTESIAN_POINT('Ctrl Pts',(-10.4397731061019,66.20328211146,81.283605864789));
#121896=CARTESIAN_POINT('Ctrl Pts',(-10.7217981634799,65.09310714263,79.928825352772));
#121897=CARTESIAN_POINT('Ctrl Pts',(-10.9299000372949,64.18755471981,78.404219526706));
#121898=CARTESIAN_POINT('Ctrl Pts',(-11.0648118857419,63.55192969764,76.860507224859));
#121899=CARTESIAN_POINT('Ctrl Pts',(-11.1421554969749,63.16741934538,75.409697985201));
#121900=CARTESIAN_POINT('Ctrl Pts',(-11.1792767754389,62.97733743511,74.082574270443));
#121901=CARTESIAN_POINT('Ctrl Pts',(-11.1853672911799,62.9457324032,73.2390344611633));
#121902=CARTESIAN_POINT('Ctrl Pts',(-11.1845309756149,62.95073351593,72.8382378734121));
#121903=CARTESIAN_POINT('Ctrl Pts',(-11.1845298882129,62.95074001469,72.8377197366249));
#121904=CARTESIAN_POINT('Origin',(-8.56753648333091,1.4210854715202E-14,
72.98888938658));
#121905=CARTESIAN_POINT('',(-8.56285234933876,73.333293028708,64.0807251311373));
#121906=CARTESIAN_POINT('',(-8.56795784296129,66.4424972638774,69.9758907965238));
#121907=CARTESIAN_POINT('Ctrl Pts',(-8.56753648333091,73.3335502589656,
64.0821442489851));
#121908=CARTESIAN_POINT('Ctrl Pts',(-8.56753648333091,72.5539028998352,
64.2258274700778));
#121909=CARTESIAN_POINT('Ctrl Pts',(-8.56753648333092,71.7917993992724,
64.4685834837518));
#121910=CARTESIAN_POINT('Ctrl Pts',(-8.56753648333092,70.5771863640527,
65.0448111485544));
#121911=CARTESIAN_POINT('Ctrl Pts',(-8.56753648333091,69.8608492258319,
65.440988650358));
#121912=CARTESIAN_POINT('Ctrl Pts',(-8.56753648333091,68.4965495909561,
66.6238377720524));
#121913=CARTESIAN_POINT('Ctrl Pts',(-8.56753648333093,67.9668494703072,
67.2198258127435));
#121914=CARTESIAN_POINT('Ctrl Pts',(-8.56753648333093,67.0735256632114,
68.5233977289405));
#121915=CARTESIAN_POINT('Ctrl Pts',(-8.56753648333091,66.7090578372287,
69.23213924102));
#121916=CARTESIAN_POINT('Ctrl Pts',(-8.56753648333091,66.4431946200656,
69.976105782015));
#121917=CARTESIAN_POINT('Ctrl Pts',(-8.56753648333091,66.4418053341428,
69.9756606261135));
#121918=CARTESIAN_POINT('Ctrl Pts',(-8.56753648333091,66.2607314661459,
70.5747391016418));
#121919=CARTESIAN_POINT('Ctrl Pts',(-8.56753648333067,66.1409893830732,
71.1924170733865));
#121920=CARTESIAN_POINT('Ctrl Pts',(-8.56753648333067,66.0348383656674,
72.4359711725211));
#121921=CARTESIAN_POINT('Ctrl Pts',(-8.5675364833307,66.0481767601204,73.060065741546));
#121922=CARTESIAN_POINT('Ctrl Pts',(-8.5675364833307,66.2227996979891,74.4574116220633));
#121923=CARTESIAN_POINT('Ctrl Pts',(-8.56753648333093,66.468768244879,75.6274791834595));
#121924=CARTESIAN_POINT('Ctrl Pts',(-8.56753648333093,67.7151076066531,
77.8553329362392));
#121925=CARTESIAN_POINT('Ctrl Pts',(-8.56753648333122,68.4456337803905,
78.7215971823619));
#121926=CARTESIAN_POINT('Ctrl Pts',(-8.56753648333122,69.8118531742968,
79.8204638981078));
#121927=CARTESIAN_POINT('Ctrl Pts',(-8.56753648333126,70.3493421759933,
80.1599025125624));
#121928=CARTESIAN_POINT('Ctrl Pts',(-8.56753648333126,71.4836677103505,
80.7090839391736));
#121929=CARTESIAN_POINT('Ctrl Pts',(-8.56753648333091,72.0732569766187,
80.9188351508686));
#121930=CARTESIAN_POINT('Ctrl Pts',(-8.56753648333091,72.6784966214632,
81.0617217311455));
#121931=CARTESIAN_POINT('Ctrl Pts',(-8.57006447465355,83.3346137605936,
71.9543844308784));
#121932=CARTESIAN_POINT('Ctrl Pts',(-8.56941033891195,83.3220909976787,
71.8009596765008));
#121933=CARTESIAN_POINT('Ctrl Pts',(-8.56886746936034,83.305681306695,71.6484246702876));
#121934=CARTESIAN_POINT('Ctrl Pts',(-8.5683903518647,83.2853788427609,71.4967593339514));
#121935=CARTESIAN_POINT('Ctrl Pts',(-8.56791227764618,83.2650356680335,
71.3447898760967));
#121936=CARTESIAN_POINT('Ctrl Pts',(-8.56750021944195,83.2407839104731,
71.1936931337831));
#121937=CARTESIAN_POINT('Ctrl Pts',(-8.56710838877179,83.2125673414922,
71.0434635951297));
#121938=CARTESIAN_POINT('Ctrl Pts',(-8.56671842313737,83.1844850777445,
70.8939491190778));
#121939=CARTESIAN_POINT('Ctrl Pts',(-8.56634849293726,83.1524754527888,
70.745293194284));
#121940=CARTESIAN_POINT('Ctrl Pts',(-8.56595346041612,83.1164361810017,
70.5975113327712));
#121941=CARTESIAN_POINT('Ctrl Pts',(-8.56561023543377,83.0851233706345,
70.469110697137));
#121942=CARTESIAN_POINT('Ctrl Pts',(-8.56524806059338,83.0507677873467,
70.3413700448385));
#121943=CARTESIAN_POINT('Ctrl Pts',(-8.56483733000771,83.0132750464447,
70.2143161908913));
#121944=CARTESIAN_POINT('Ctrl Pts',(-8.56435630198732,82.9693653412412,
70.0655167929924));
#121945=CARTESIAN_POINT('Ctrl Pts',(-8.56383104291083,82.9211785522005,
69.9176068560262));
#121946=CARTESIAN_POINT('Ctrl Pts',(-8.56332873364437,82.8687104849843,
69.7706206743157));
#121947=CARTESIAN_POINT('Ctrl Pts',(-8.56283735805838,82.8173844812751,
69.6268339158561));
#121948=CARTESIAN_POINT('Ctrl Pts',(-8.56236794406668,82.7619616214511,
69.4839306438142));
#121949=CARTESIAN_POINT('Ctrl Pts',(-8.56198338038889,82.702388237078,69.3419433580854));
#121950=CARTESIAN_POINT('Ctrl Pts',(-8.56184284085215,82.6806170290173,
69.2900538310404));
#121951=CARTESIAN_POINT('Ctrl Pts',(-8.56171363350844,82.6582910038869,
69.2382866788046));
#121952=CARTESIAN_POINT('Ctrl Pts',(-8.56159882782864,82.6354057978218,
69.1866437008642));
#121953=CARTESIAN_POINT('Ctrl Pts',(-8.56127799107733,82.5714506417676,
69.0423218754944));
#121954=CARTESIAN_POINT('Ctrl Pts',(-8.56106962884463,82.5031319272677,
68.8989691362582));
#121955=CARTESIAN_POINT('Ctrl Pts',(-8.56104073355965,82.4304725808081,
68.7565547922964));
#121956=CARTESIAN_POINT('Ctrl Pts',(-8.56103230042259,82.4092668295218,
68.7149909288044));
#121957=CARTESIAN_POINT('Ctrl Pts',(-8.56103815082216,82.3874931148553,
68.6731323533542));
#121958=CARTESIAN_POINT('Ctrl Pts',(-8.56105882880582,82.3655094434444,
68.6316745428395));
#121959=CARTESIAN_POINT('Ctrl Pts',(-8.56107193580283,82.351574820021,68.6053959942441));
#121960=CARTESIAN_POINT('Ctrl Pts',(-8.56109100025004,82.3375568159525,
68.5792780371855));
#121961=CARTESIAN_POINT('Ctrl Pts',(-8.56111616070234,82.323556420184,68.5534931793396));
#121962=CARTESIAN_POINT('Ctrl Pts',(-8.5612477274945,82.2503467998598,68.4186613014251));
#121963=CARTESIAN_POINT('Ctrl Pts',(-8.56147132827033,82.174042389154,68.2865956486264));
#121964=CARTESIAN_POINT('Ctrl Pts',(-8.56175811113411,82.0947707474585,
68.1572071661102));
#121965=CARTESIAN_POINT('Ctrl Pts',(-8.56204998515142,82.0140918246817,
68.0255216961757));
#121966=CARTESIAN_POINT('Ctrl Pts',(-8.56240730446691,81.9303390791557,
67.896609002754));
#121967=CARTESIAN_POINT('Ctrl Pts',(-8.56279965315277,81.8435974231482,
67.7703984890432));
#121968=CARTESIAN_POINT('Ctrl Pts',(-8.56319761464984,81.7556148695475,
67.6423824492459));
#121969=CARTESIAN_POINT('Ctrl Pts',(-8.5636316149234,81.6645569462095,67.5171461454029));
#121970=CARTESIAN_POINT('Ctrl Pts',(-8.56406991392175,81.5704666099132,
67.3946442191827));
#121971=CARTESIAN_POINT('Ctrl Pts',(-8.56451394760364,81.4751452000696,
67.2705394835052));
#121972=CARTESIAN_POINT('Ctrl Pts',(-8.56496239323484,81.3767111650124,
67.1492408053214));
#121973=CARTESIAN_POINT('Ctrl Pts',(-8.5653822485358,81.2751677791634,67.0307348194276));
#121974=CARTESIAN_POINT('Ctrl Pts',(-8.56580299955837,81.1734077600962,
66.9119760122114));
#121975=CARTESIAN_POINT('Ctrl Pts',(-8.56619503813103,81.0685247080004,
66.7960215218833));
#121976=CARTESIAN_POINT('Ctrl Pts',(-8.56652515030154,80.9604863334545,
66.6828963954045));
#121977=CARTESIAN_POINT('Ctrl Pts',(-8.56685368594238,80.8529639220205,
66.5703115250387));
#121978=CARTESIAN_POINT('Ctrl Pts',(-8.56712088525739,80.7423158404718,
66.4605287861003));
#121979=CARTESIAN_POINT('Ctrl Pts',(-8.56729400788887,80.6284811960154,
66.3536151977035));
#121980=CARTESIAN_POINT('Ctrl Pts',(-8.567412542533,80.5505402072772,66.2804129592374));
#121981=CARTESIAN_POINT('Ctrl Pts',(-8.56748697450439,80.4711047740473,
66.2085566378043));
#121982=CARTESIAN_POINT('Ctrl Pts',(-8.5675067948903,80.3901489224879,66.1380803177677));
#121983=CARTESIAN_POINT('Ctrl Pts',(-8.56752047565147,80.3342702087702,
66.0894349631041));
#121984=CARTESIAN_POINT('Ctrl Pts',(-8.56752614823847,80.2773606447956,
66.0411465497854));
#121985=CARTESIAN_POINT('Ctrl Pts',(-8.56752927539675,80.2199013837073,
65.9936363050754));
#121986=CARTESIAN_POINT('Ctrl Pts',(-8.56753240255504,80.162442122619,65.9461260603653));
#121987=CARTESIAN_POINT('Ctrl Pts',(-8.56753298428461,80.104433364226,65.8993941752881));
#121988=CARTESIAN_POINT('Ctrl Pts',(-8.56753648333091,80.04639670726,65.8538149462682));
#121989=CARTESIAN_POINT('Ctrl Pts',(-8.56754409353963,79.9201705773867,
65.7546829496551));
#121990=CARTESIAN_POINT('Ctrl Pts',(-8.56747490722444,79.7915654578427,
65.6594020033908));
#121991=CARTESIAN_POINT('Ctrl Pts',(-8.56735121852545,79.660643441596,65.5679332348105));
#121992=CARTESIAN_POINT('Ctrl Pts',(-8.56722776761322,79.5299731178824,
65.4766403114145));
#121993=CARTESIAN_POINT('Ctrl Pts',(-8.56705002367323,79.3969944738259,
65.389144513119));
#121994=CARTESIAN_POINT('Ctrl Pts',(-8.56684015251371,79.2617278672298,
65.3054383083156));
#121995=CARTESIAN_POINT('Ctrl Pts',(-8.56663265773141,79.127992888336,65.2226799112923));
#121996=CARTESIAN_POINT('Ctrl Pts',(-8.56639375916541,78.9920211157852,
65.1436254255641));
#121997=CARTESIAN_POINT('Ctrl Pts',(-8.56614487816521,78.8537968393649,
65.0683035613709));
#121998=CARTESIAN_POINT('Ctrl Pts',(-8.56593648593594,78.7380593379894,
65.0052353031283));
#121999=CARTESIAN_POINT('Ctrl Pts',(-8.56572109502871,78.6207419150425,
64.9447844778263));
#122000=CARTESIAN_POINT('Ctrl Pts',(-8.56551128067993,78.5018184917218,
64.8869904906993));
#122001=CARTESIAN_POINT('Ctrl Pts',(-8.5652590707752,78.358865135855,64.8175185214435));
#122002=CARTESIAN_POINT('Ctrl Pts',(-8.56501491873875,78.2135914960043,
64.7518844114023));
#122003=CARTESIAN_POINT('Ctrl Pts',(-8.56480066680265,78.0659885596718,
64.6900507575985));
#122004=CARTESIAN_POINT('Ctrl Pts',(-8.56464683650043,77.9600114342514,
64.6456549410436));
#122005=CARTESIAN_POINT('Ctrl Pts',(-8.56450841989892,77.8528329663568,
64.6032192090122));
#122006=CARTESIAN_POINT('Ctrl Pts',(-8.56439350140998,77.7444430632104,
64.5627448543925));
#122007=CARTESIAN_POINT('Ctrl Pts',(-8.56426217032434,77.6205729724613,
64.5164899742403));
#122008=CARTESIAN_POINT('Ctrl Pts',(-8.56415731154464,77.4948545122233,
64.4727108661274));
#122009=CARTESIAN_POINT('Ctrl Pts',(-8.56410423122616,77.3676660355867,
64.4315565945173));
#122010=CARTESIAN_POINT('Ctrl Pts',(-8.56405092899636,77.2399458258337,
64.3902302704566));
#122011=CARTESIAN_POINT('Ctrl Pts',(-8.56404983907014,77.1107436360798,
64.351550878493));
#122012=CARTESIAN_POINT('Ctrl Pts',(-8.56412658632163,76.9804597267701,
64.3156197196934));
#122013=CARTESIAN_POINT('Ctrl Pts',(-8.56414588941054,76.9476913626139,
64.3065824924385));
#122014=CARTESIAN_POINT('Ctrl Pts',(-8.56417011646539,76.9148546383835,
64.2977188696857));
#122015=CARTESIAN_POINT('Ctrl Pts',(-8.56419967519835,76.8819560504712,
64.2890299614086));
#122016=CARTESIAN_POINT('Ctrl Pts',(-8.56433878773446,76.7271251243546,
64.2481372726687));
#122017=CARTESIAN_POINT('Ctrl Pts',(-8.56449961980914,76.5721315732247,
64.2115987798294));
#122018=CARTESIAN_POINT('Ctrl Pts',(-8.56466401278212,76.4170095331184,
64.179271595885));
#122019=CARTESIAN_POINT('Ctrl Pts',(-8.56483069887061,76.2597236976112,
64.1464934804553));
#122020=CARTESIAN_POINT('Ctrl Pts',(-8.56500104589211,76.1023053158395,
64.1180449315697));
#122021=CARTESIAN_POINT('Ctrl Pts',(-8.56515612467349,75.9447685236109,
64.0938270945347));
#122022=CARTESIAN_POINT('Ctrl Pts',(-8.56531272843634,75.7856825788478,
64.0693711091719));
#122023=CARTESIAN_POINT('Ctrl Pts',(-8.56545376219935,75.6264754095279,
64.0492294120697));
#122024=CARTESIAN_POINT('Ctrl Pts',(-8.56555973285479,75.4671468724349,
64.0333515489916));
#122025=CARTESIAN_POINT('Ctrl Pts',(-8.56566623305092,75.3070221626365,
64.0173943434339));
#122026=CARTESIAN_POINT('Ctrl Pts',(-8.56573731883972,75.1467743786349,
64.0057436685047));
#122027=CARTESIAN_POINT('Ctrl Pts',(-8.56575320342664,74.9863959007504,
63.9984003217801));
#122028=CARTESIAN_POINT('Ctrl Pts',(-8.5657690510057,74.8263910722562,63.991074083567));
#122029=CARTESIAN_POINT('Ctrl Pts',(-8.5657299542985,74.6662556684931,63.9880351413726));
#122030=CARTESIAN_POINT('Ctrl Pts',(-8.56561626448623,74.5059820589448,
63.9893358949042));
#122031=CARTESIAN_POINT('Ctrl Pts',(-8.56550328681298,74.3467123835981,
63.9906285006754));
#122032=CARTESIAN_POINT('Ctrl Pts',(-8.56531664759201,74.1873057550039,
63.9962066299903));
#122033=CARTESIAN_POINT('Ctrl Pts',(-8.56503706492985,74.027761791215,64.0061723870185));
#122034=CARTESIAN_POINT('Ctrl Pts',(-8.56476171519069,73.8706333467147,
64.0159872610063));
#122035=CARTESIAN_POINT('Ctrl Pts',(-8.56439621506046,73.713371264694,64.0300579850534));
#122036=CARTESIAN_POINT('Ctrl Pts',(-8.56392214524518,73.5559887369095,
64.04853056409));
#122037=CARTESIAN_POINT('Ctrl Pts',(-8.56369817955241,73.4816362138653,
64.0572575992815));
#122038=CARTESIAN_POINT('Ctrl Pts',(-8.56344998198766,73.4072570453578,
64.066967792157));
#122039=CARTESIAN_POINT('Ctrl Pts',(-8.56317561036611,73.3328541209004,
64.077680326643));
#122040=CARTESIAN_POINT('Ctrl Pts',(-9.33949250599091,68.28843467669,68.385749441946));
#122041=CARTESIAN_POINT('Ctrl Pts',(-9.28372478921891,67.21314456544,69.953566173561));
#122042=CARTESIAN_POINT('Ctrl Pts',(-9.17218935567391,66.21224057553,73.8663634510705));
#122043=CARTESIAN_POINT('Ctrl Pts',(-9.00488620535791,68.84902572167,79.327681027565));
#122044=CARTESIAN_POINT('Ctrl Pts',(-8.83758305504191,74.3860768082,81.799718607153));
#122045=CARTESIAN_POINT('Ctrl Pts',(-8.67027990472591,80.21224973459,80.119224478064));
#122046=CARTESIAN_POINT('Ctrl Pts',(-8.50297675440891,83.58160767004,75.077818068246));
#122047=CARTESIAN_POINT('Ctrl Pts',(-8.33567360409291,82.90653225676,69.051693466476));
#122048=CARTESIAN_POINT('Ctrl Pts',(-8.16837045377691,78.50298784705,64.8818706633));
#122049=CARTESIAN_POINT('Ctrl Pts',(-8.05683502023291,74.47097197897,64.648120002453));
#122050=CARTESIAN_POINT('Ctrl Pts',(-8.00106730345991,72.65076867909,65.196898714115));
#122051=CARTESIAN_POINT('Ctrl Pts',(-9.57007551786691,67.95907438126,68.159857051868));
#122052=CARTESIAN_POINT('Ctrl Pts',(-9.51430780109491,66.83101597355,69.804612106664));
#122053=CARTESIAN_POINT('Ctrl Pts',(-9.40277236755091,65.78099407777,73.9094242130813));
#122054=CARTESIAN_POINT('Ctrl Pts',(-9.23546921723391,68.54717561549,79.638747997329));
#122055=CARTESIAN_POINT('Ctrl Pts',(-9.06816606691691,74.3559494215,82.232097221564));
#122056=CARTESIAN_POINT('Ctrl Pts',(-8.90086291659891,80.46803330067,80.469135290092));
#122057=CARTESIAN_POINT('Ctrl Pts',(-8.73355976628091,84.00273757062,75.180329201596));
#122058=CARTESIAN_POINT('Ctrl Pts',(-8.56625661596291,83.29453381444,68.858481309736));
#122059=CARTESIAN_POINT('Ctrl Pts',(-8.39895346564491,78.67489187492,64.484030524229));
#122060=CARTESIAN_POINT('Ctrl Pts',(-8.28741803209991,74.4450106992,64.238808890051));
#122061=CARTESIAN_POINT('Ctrl Pts',(-8.23165031532691,72.5354835728,64.814518117892));
#122062=CARTESIAN_POINT('Ctrl Pts',(-9.80065852974291,67.62971408584,67.93396466179));
#122063=CARTESIAN_POINT('Ctrl Pts',(-9.74489081297091,66.44888738166,69.655658039767));
#122064=CARTESIAN_POINT('Ctrl Pts',(-9.63335537942691,65.34974758001,73.9524849750929));
#122065=CARTESIAN_POINT('Ctrl Pts',(-9.46605222911191,68.24532550932,79.949814967102));
#122066=CARTESIAN_POINT('Ctrl Pts',(-9.29874907879591,74.32582203482,82.66447583598));
#122067=CARTESIAN_POINT('Ctrl Pts',(-9.13144592848091,80.72381686678,80.8190461021));
#122068=CARTESIAN_POINT('Ctrl Pts',(-8.96414277816591,84.42386747123,75.282840334888));
#122069=CARTESIAN_POINT('Ctrl Pts',(-8.79683962785091,83.68253537209,68.665269152917));
#122070=CARTESIAN_POINT('Ctrl Pts',(-8.62953647753691,78.84679590269,64.086190385108));
#122071=CARTESIAN_POINT('Ctrl Pts',(-8.51800104399391,74.41904941931,63.829497777655));
#122072=CARTESIAN_POINT('Ctrl Pts',(-8.46223332722191,72.4201984664,64.432137521706));
#122073=CARTESIAN_POINT('Ctrl Pts',(-10.0312415416199,67.30035379041,67.708072271712));
#122074=CARTESIAN_POINT('Ctrl Pts',(-9.97547382484791,66.06675878978,69.50670397287));
#122075=CARTESIAN_POINT('Ctrl Pts',(-9.86393839130291,64.91850108225,73.995545737104));
#122076=CARTESIAN_POINT('Ctrl Pts',(-9.69663524098691,67.94347540314,80.260881936865));
#122077=CARTESIAN_POINT('Ctrl Pts',(-9.52933209067091,74.29569464812,83.09685445039));
#122078=CARTESIAN_POINT('Ctrl Pts',(-9.36202894035391,80.97960043285,81.168956914128));
#122079=CARTESIAN_POINT('Ctrl Pts',(-9.19472579003791,84.84499737182,75.38535146824));
#122080=CARTESIAN_POINT('Ctrl Pts',(-9.02742263972191,84.07053692978,68.47205699618));
#122081=CARTESIAN_POINT('Ctrl Pts',(-8.86011948940491,79.01869993056,63.68835024604));
#122082=CARTESIAN_POINT('Ctrl Pts',(-8.74858405586091,74.39308813955,63.420186665253));
#122083=CARTESIAN_POINT('Ctrl Pts',(-8.69281633908891,72.30491336013,64.049756925482));
#122084=CARTESIAN_POINT('',(-9.85448379345391,67.0101053268475,68.6926900228996));
#122085=CARTESIAN_POINT('Ctrl Pts',(-9.85448379345391,67.0101053268475,
68.6926900228996));
#122086=CARTESIAN_POINT('Ctrl Pts',(-9.83968424671194,66.7566723975021,
69.1693478230976));
#122087=CARTESIAN_POINT('Ctrl Pts',(-9.82516107127357,66.5463438560124,
69.6690843869866));
#122088=CARTESIAN_POINT('Ctrl Pts',(-9.81076777080292,66.3808021984325,
70.1832779640609));
#122089=CARTESIAN_POINT('Ctrl Pts',(-9.79800752377682,66.2340427773993,
70.6391315103747));
#122090=CARTESIAN_POINT('Ctrl Pts',(-9.78534935256035,66.1224832757427,
71.1063467143764));
#122091=CARTESIAN_POINT('Ctrl Pts',(-9.77269118134386,66.0472619576907,
71.5789206748202));
#122092=CARTESIAN_POINT('Ctrl Pts',(-9.7641119086294,65.9962795376812,71.8992150376523));
#122093=CARTESIAN_POINT('Ctrl Pts',(-9.75553263591493,65.961974408791,72.2220322993447));
#122094=CARTESIAN_POINT('Ctrl Pts',(-9.74695336320047,65.9447185888639,
72.5456455219375));
#122095=CARTESIAN_POINT('Ctrl Pts',(-9.73851905287355,65.9277543373412,
72.8637907116387));
#122096=CARTESIAN_POINT('Ctrl Pts',(-9.73008474254663,65.9272680677149,
73.1827060455231));
#122097=CARTESIAN_POINT('Ctrl Pts',(-9.72165043221971,65.9436628520002,
73.500745147291));
#122098=CARTESIAN_POINT('Ctrl Pts',(-9.71348628550153,65.9595324867575,
73.8085969796649));
#122099=CARTESIAN_POINT('Ctrl Pts',(-9.70532213878336,65.991219138219,74.1156284875255));
#122100=CARTESIAN_POINT('Ctrl Pts',(-9.69715799206519,66.0391346213581,
74.4203302806321));
#122101=CARTESIAN_POINT('Ctrl Pts',(-9.69539938958562,66.0494558821544,
74.4859647366732));
#122102=CARTESIAN_POINT('Ctrl Pts',(-9.69364078710605,66.0605303262043,
74.551491012646));
#122103=CARTESIAN_POINT('Ctrl Pts',(-9.69188218462648,66.0723623568164,
74.6168938744211));
#122104=CARTESIAN_POINT('Ctrl Pts',(-9.68912429718818,66.0909176636431,
74.719460391308));
#122105=CARTESIAN_POINT('Ctrl Pts',(-9.68636640974989,66.1113251604818,
74.8216626934074));
#122106=CARTESIAN_POINT('Ctrl Pts',(-9.68360852231159,66.1335950524943,
74.9234405765911));
#122107=CARTESIAN_POINT('Ctrl Pts',(-9.6733601644373,66.2163503600525,75.3016489675757));
#122108=CARTESIAN_POINT('Ctrl Pts',(-9.66311180656301,66.3248188849568,
75.673995727457));
#122109=CARTESIAN_POINT('Ctrl Pts',(-9.65286344868873,66.456981133905,76.0379113155534));
#122110=CARTESIAN_POINT('Ctrl Pts',(-9.6420032438932,66.5970337264689,76.4235533728952));
#122111=CARTESIAN_POINT('Ctrl Pts',(-9.63114303909766,66.7636936492638,
76.7997282070751));
#122112=CARTESIAN_POINT('Ctrl Pts',(-9.62028283430213,66.9546167830891,
77.1633862403935));
#122113=CARTESIAN_POINT('Ctrl Pts',(-9.60912582522197,67.1507577562851,
77.5369828765709));
#122114=CARTESIAN_POINT('Ctrl Pts',(-9.5979688161418,67.3725067113742,77.8973701715073));
#122115=CARTESIAN_POINT('Ctrl Pts',(-9.58681180706164,67.6173784973787,
78.2412368390855));
#122116=CARTESIAN_POINT('Ctrl Pts',(-9.57549059509304,67.8658541752745,
78.5901643522403));
#122117=CARTESIAN_POINT('Ctrl Pts',(-9.56416938312445,68.1381389483182,
78.9220824577887));
#122118=CARTESIAN_POINT('Ctrl Pts',(-9.55284817115585,68.4316852140694,
79.2335109677848));
#122119=CARTESIAN_POINT('Ctrl Pts',(-9.54532017783458,68.626877595785,79.4405940742406));
#122120=CARTESIAN_POINT('Ctrl Pts',(-9.53779218451331,68.8314718067912,
79.6386171967666));
#122121=CARTESIAN_POINT('Ctrl Pts',(-9.53026419119205,69.0447283571958,
79.8265486021723));
#122122=CARTESIAN_POINT('Ctrl Pts',(-9.52194613970065,69.2803660486017,
80.0342032905206));
#122123=CARTESIAN_POINT('Ctrl Pts',(-9.51362808820925,69.5268279476083,
80.2297487085396));
#122124=CARTESIAN_POINT('Ctrl Pts',(-9.50531003671786,69.783037643129,80.4116123859453));
#122125=CARTESIAN_POINT('Ctrl Pts',(-9.49781673259709,70.0138437603079,
80.5754440050126));
#122126=CARTESIAN_POINT('Ctrl Pts',(-9.49032342847633,70.2525595800675,
80.7281723744406));
#122127=CARTESIAN_POINT('Ctrl Pts',(-9.48283012435557,70.4983698898005,
80.8686705606302));
#122128=CARTESIAN_POINT('Ctrl Pts',(-9.47469694729936,70.7651705880079,
81.021166256246));
#122129=CARTESIAN_POINT('Ctrl Pts',(-9.46656377024315,71.0403291308939,
81.1592526198816));
#122130=CARTESIAN_POINT('Ctrl Pts',(-9.45843059318694,71.3221041991271,
81.2826982415201));
#122131=CARTESIAN_POINT('Ctrl Pts',(-9.45012412633853,71.6098829166948,
81.4087740611703));
#122132=CARTESIAN_POINT('Ctrl Pts',(-9.44181765949011,71.9045622622991,
81.5195783413505));
#122133=CARTESIAN_POINT('Ctrl Pts',(-9.4335111926417,72.2042657814675,81.6149141880342));
#122134=CARTESIAN_POINT('Ctrl Pts',(-9.42521438877695,72.5036206529783,
81.7101391297152));
#122135=CARTESIAN_POINT('Ctrl Pts',(-9.4169175849122,72.8079870625739,81.7899315289484));
#122136=CARTESIAN_POINT('Ctrl Pts',(-9.40862078104745,73.1154877013141,
81.854146473293));
#122137=CARTESIAN_POINT('Ctrl Pts',(-9.40048676107778,73.4169551551642,
81.9171015157606));
#122138=CARTESIAN_POINT('Ctrl Pts',(-9.3923527411081,73.7214341968443,81.965084457809));
#122139=CARTESIAN_POINT('Ctrl Pts',(-9.38421872113843,74.0271621528231,
81.9980077408963));
#122140=CARTESIAN_POINT('Ctrl Pts',(-9.37902788001143,74.2222668185954,
82.0190182046673));
#122141=CARTESIAN_POINT('Ctrl Pts',(-9.37383703888443,74.4178802756318,
82.0338965468219));
#122142=CARTESIAN_POINT('Ctrl Pts',(-9.36864619775743,74.6135481804256,
82.0426305340964));
#122143=CARTESIAN_POINT('Ctrl Pts',(-9.36110373378891,74.8978601224783,
82.0553213066914));
#122144=CARTESIAN_POINT('Ctrl Pts',(-9.35356126982038,75.1831895074007,
82.0550770709536));
#122145=CARTESIAN_POINT('Ctrl Pts',(-9.34601880585185,75.4681029630233,
82.0416491691116));
#122146=CARTESIAN_POINT('Ctrl Pts',(-9.33843160312578,75.754706406701,82.0281416185437));
#122147=CARTESIAN_POINT('Ctrl Pts',(-9.33084440039971,76.0408881332488,
82.0012933809063));
#122148=CARTESIAN_POINT('Ctrl Pts',(-9.32325719767364,76.3251718586273,
81.9609015624754));
#122149=CARTESIAN_POINT('Ctrl Pts',(-9.31572904715047,76.6072429661492,
81.9208241189129));
#122150=CARTESIAN_POINT('Ctrl Pts',(-9.3082008966273,76.8874446469196,81.867413064794));
#122151=CARTESIAN_POINT('Ctrl Pts',(-9.30067274610414,77.1643306109711,
81.8005207374888));
#122152=CARTESIAN_POINT('Ctrl Pts',(-9.29451315298162,77.3908809269679,
81.7457888989115));
#122153=CARTESIAN_POINT('Ctrl Pts',(-9.28835355985909,77.6152112078615,
81.6820327358978));
#122154=CARTESIAN_POINT('Ctrl Pts',(-9.28219396673657,77.8365331068418,
81.6091970918653));
#122155=CARTESIAN_POINT('Ctrl Pts',(-9.27464830785804,78.1076580852023,
81.5199715678518));
#122156=CARTESIAN_POINT('Ctrl Pts',(-9.26710264897951,78.374267377385,81.4171194611954));
#122157=CARTESIAN_POINT('Ctrl Pts',(-9.25955699010099,78.6352651857245,
81.3016023574398));
#122158=CARTESIAN_POINT('Ctrl Pts',(-9.25196749606842,78.8977792140945,
81.1854141777557));
#122159=CARTESIAN_POINT('Ctrl Pts',(-9.24437800203584,79.1546157026713,
81.0564139756897));
#122160=CARTESIAN_POINT('Ctrl Pts',(-9.23678850800327,79.4046883212804,
80.9156244836224));
#122161=CARTESIAN_POINT('Ctrl Pts',(-9.22924654220847,79.6531948920309,
80.7757166677809));
#122162=CARTESIAN_POINT('Ctrl Pts',(-9.22170457641367,79.8950214601759,
80.6241673829361));
#122163=CARTESIAN_POINT('Ctrl Pts',(-9.21416261061888,80.1291394950741,
80.4620149282776));
#122164=CARTESIAN_POINT('Ctrl Pts',(-9.21178447518684,80.2029616800612,
80.4108849565559));
#122165=CARTESIAN_POINT('Ctrl Pts',(-9.20940633975481,80.2760177457059,
80.3587009664616));
#122166=CARTESIAN_POINT('Ctrl Pts',(-9.20702820432278,80.3482763680922,
80.3054960787968));
#122167=CARTESIAN_POINT('Ctrl Pts',(-9.19830930076526,80.6131965031266,
80.1104322157008));
#122168=CARTESIAN_POINT('Ctrl Pts',(-9.18959039720775,80.8682552155851,
79.9010102664133));
#122169=CARTESIAN_POINT('Ctrl Pts',(-9.18087149365024,81.111814081159,79.6785563218492));
#122170=CARTESIAN_POINT('Ctrl Pts',(-9.17186595779949,81.3633798980331,
79.4487892462418));
#122171=CARTESIAN_POINT('Ctrl Pts',(-9.16286042194875,81.6026765258506,
79.205119591945));
#122172=CARTESIAN_POINT('Ctrl Pts',(-9.15385488609801,81.8279139681047,
78.94906204399));
#122173=CARTESIAN_POINT('Ctrl Pts',(-9.14480155182367,82.0543468966522,
78.6916454267532));
#122174=CARTESIAN_POINT('Ctrl Pts',(-9.13574821754934,82.2665702022945,
78.4217097128373));
#122175=CARTESIAN_POINT('Ctrl Pts',(-9.12669488327501,82.4627926640579,
78.1408390221426));
#122176=CARTESIAN_POINT('Ctrl Pts',(-9.11777922382609,82.6560311541323,
77.8642395559641));
#122177=CARTESIAN_POINT('Ctrl Pts',(-9.10886356437717,82.8337511090989,
77.5770359114317));
#122178=CARTESIAN_POINT('Ctrl Pts',(-9.09994790492826,82.994278877925,77.2807741296127));
#122179=CARTESIAN_POINT('Ctrl Pts',(-9.09380383002873,83.1049038564554,
77.0766103672134));
#122180=CARTESIAN_POINT('Ctrl Pts',(-9.08765975512921,83.2073649566054,
76.8681455411797));
#122181=CARTESIAN_POINT('Ctrl Pts',(-9.08151568022969,83.3011273339562,
76.6558922479745));
#122182=CARTESIAN_POINT('Ctrl Pts',(-9.07246710832417,83.4392141293431,
76.3433001625654));
#122183=CARTESIAN_POINT('Ctrl Pts',(-9.06341853641865,83.5584317260117,
76.0224912178744));
#122184=CARTESIAN_POINT('Ctrl Pts',(-9.05436996451312,83.6587995041413,
75.6958576243948));
#122185=CARTESIAN_POINT('Ctrl Pts',(-9.05138337997155,83.6919270360617,
75.5880484749256));
#122186=CARTESIAN_POINT('Ctrl Pts',(-9.04839679542997,83.7230014791061,
75.479604834333));
#122187=CARTESIAN_POINT('Ctrl Pts',(-9.04541021088839,83.7520247722967,
75.3706127663605));
#122188=CARTESIAN_POINT('Ctrl Pts',(-9.03539106069585,83.8493897487475,
75.0049750676414));
#122189=CARTESIAN_POINT('Ctrl Pts',(-9.02537191050332,83.9237100286563,
74.6330371582655));
#122190=CARTESIAN_POINT('Ctrl Pts',(-9.01535276031078,83.9750640216069,
74.2577698789031));
#122191=CARTESIAN_POINT('Ctrl Pts',(-9.00513012247064,84.027461007528,73.874880969519));
#122192=CARTESIAN_POINT('Ctrl Pts',(-8.9949074846305,84.055949510843,73.4885250035023));
#122193=CARTESIAN_POINT('Ctrl Pts',(-8.98468484679035,84.0605617694674,
73.1018404298762));
#122194=CARTESIAN_POINT('Ctrl Pts',(-8.97452712867039,84.0651447375559,
72.7176115291115));
#122195=CARTESIAN_POINT('Ctrl Pts',(-8.96436941055043,84.0461536980524,
72.3330570424656));
#122196=CARTESIAN_POINT('Ctrl Pts',(-8.95421169243046,84.0035699263375,
71.951256065974));
#122197=CARTESIAN_POINT('Ctrl Pts',(-8.94427537112854,83.9619143071316,
71.5777767932672));
#122198=CARTESIAN_POINT('Ctrl Pts',(-8.93433904982663,83.8976830275582,
71.2069313198722));
#122199=CARTESIAN_POINT('Ctrl Pts',(-8.92440272852471,83.8108120961398,
70.8416174230802));
#122200=CARTESIAN_POINT('Ctrl Pts',(-8.91488179465382,83.7275727998039,
70.4915754560591));
#122201=CARTESIAN_POINT('Ctrl Pts',(-8.90536086078292,83.6235469010876,
70.14661155296));
#122202=CARTESIAN_POINT('Ctrl Pts',(-8.89583992691202,83.4986384743573,
69.8093014238666));
#122203=CARTESIAN_POINT('Ctrl Pts',(-8.89182402375937,83.4459524509587,
69.6670249592661));
#122204=CARTESIAN_POINT('Ctrl Pts',(-8.88780812060673,83.3895506839613,
69.526110587854));
#122205=CARTESIAN_POINT('Ctrl Pts',(-8.88379221745408,83.3294239020245,
69.3867535301559));
#122206=CARTESIAN_POINT('Ctrl Pts',(-8.88276827073607,83.3140931983973,
69.3512212485154));
#122207=CARTESIAN_POINT('Ctrl Pts',(-8.88174432401806,83.2985229335303,
69.3157962727063));
#122208=CARTESIAN_POINT('Ctrl Pts',(-8.88072037730005,83.2827131953649,
69.28048176021));
#122209=CARTESIAN_POINT('Ctrl Pts',(-8.87076384242528,83.1289842887371,
68.9370945809048));
#122210=CARTESIAN_POINT('Ctrl Pts',(-8.8608073075505,82.9526176762723,68.6041515378788));
#122211=CARTESIAN_POINT('Ctrl Pts',(-8.85085077267572,82.7559042186426,
68.2835569890274));
#122212=CARTESIAN_POINT('Ctrl Pts',(-8.84012772695439,82.5440466369946,
67.93828124314));
#122213=CARTESIAN_POINT('Ctrl Pts',(-8.82940468123306,82.3085887208393,
67.6073276606856));
#122214=CARTESIAN_POINT('Ctrl Pts',(-8.81868163551173,82.0523291916876,
67.2930844645106));
#122215=CARTESIAN_POINT('Ctrl Pts',(-8.80794383623225,81.7957170817522,
66.9784089093411));
#122216=CARTESIAN_POINT('Ctrl Pts',(-8.79720603695278,81.5182451844684,
66.6804889429592));
#122217=CARTESIAN_POINT('Ctrl Pts',(-8.7864682376733,81.2226714956049,66.4017442245413));
#122218=CARTESIAN_POINT('Ctrl Pts',(-8.77574164723827,80.9274063466398,
66.1232904787991));
#122219=CARTESIAN_POINT('Ctrl Pts',(-8.76501505680324,80.6140762722008,
65.8639711687019));
#122220=CARTESIAN_POINT('Ctrl Pts',(-8.75428846636821,80.285392018042,65.626231962766));
#122221=CARTESIAN_POINT('Ctrl Pts',(-8.74358371891872,79.9573770767891,
65.3889768746933));
#122222=CARTESIAN_POINT('Ctrl Pts',(-8.73287897146925,79.6140695273579,
65.1732133043622));
#122223=CARTESIAN_POINT('Ctrl Pts',(-8.72217422401977,79.2581386075932,
64.9814173392414));
#122224=CARTESIAN_POINT('Ctrl Pts',(-8.71420778820075,78.993256055091,64.8386834490966));
#122225=CARTESIAN_POINT('Ctrl Pts',(-8.70624135238174,78.7211837617792,
64.7091241008327));
#122226=CARTESIAN_POINT('Ctrl Pts',(-8.69827491656272,78.4431588341649,
64.5938933849846));
#122227=CARTESIAN_POINT('Ctrl Pts',(-8.69216431948956,78.2299018209231,
64.505506496419));
#122228=CARTESIAN_POINT('Ctrl Pts',(-8.6860537224164,78.01314340794,64.4255493009773));
#122229=CARTESIAN_POINT('Ctrl Pts',(-8.67994312534324,77.7934534819807,
64.354525331016));
#122230=CARTESIAN_POINT('Ctrl Pts',(-8.67205571477406,77.5098830512668,
64.2628493123501));
#122231=CARTESIAN_POINT('Ctrl Pts',(-8.66416830420487,77.221428261215,64.1860589478401));
#122232=CARTESIAN_POINT('Ctrl Pts',(-8.65628089363569,76.9297092055054,
64.1240228313856));
#122233=CARTESIAN_POINT('Ctrl Pts',(-8.65130900485802,76.7458218971689,
64.0849178971991));
#122234=CARTESIAN_POINT('Ctrl Pts',(-8.64633711608036,76.5606379014098,
64.0516745335715));
#122235=CARTESIAN_POINT('Ctrl Pts',(-8.6413652273027,76.374564889621,64.0242494098714));
#122236=CARTESIAN_POINT('Ctrl Pts',(-8.63215604425852,76.0299110765988,
63.9734512131585));
#122237=CARTESIAN_POINT('Ctrl Pts',(-8.62294686121434,75.6823641851788,
63.9426311069089));
#122238=CARTESIAN_POINT('Ctrl Pts',(-8.61394688716208,75.3342120447879,
63.9314140909321));
#122239=CARTESIAN_POINT('Ctrl Pts',(-8.60457468117178,74.9716606022213,
63.9197331478848));
#122240=CARTESIAN_POINT('Ctrl Pts',(-8.59542934748614,74.6084520064369,
63.929310146414));
#122241=CARTESIAN_POINT('Ctrl Pts',(-8.58674714167216,74.2471433794914,
63.9597728002335));
#122242=CARTESIAN_POINT('Ctrl Pts',(-8.57938389032876,73.9407228350195,
63.9856077299122));
#122243=CARTESIAN_POINT('Ctrl Pts',(-8.57235374311391,73.6356680467237,
64.0264655590552));
#122244=CARTESIAN_POINT('Ctrl Pts',(-8.56580081221051,73.3335318456389,
64.0821476424436));
#122245=CARTESIAN_POINT('',(-9.46541110279056,67.6020149116865,69.0109979579471));
#122246=CARTESIAN_POINT('Ctrl Pts',(-9.87756472937818,67.62520219141,67.700413019766));
#122247=CARTESIAN_POINT('Ctrl Pts',(-9.81096367927215,66.1498345501,69.757818081886));
#122248=CARTESIAN_POINT('Ctrl Pts',(-9.67776157906115,65.03881684527,75.159924360853));
#122249=CARTESIAN_POINT('Ctrl Pts',(-9.47795842874515,69.94095953137,81.84418107373));
#122250=CARTESIAN_POINT('Ctrl Pts',(-9.27815527842915,78.18756436805,82.675374708005));
#122251=CARTESIAN_POINT('Ctrl Pts',(-9.07835212811315,84.3279816375,77.109502645435));
#122252=CARTESIAN_POINT('Ctrl Pts',(-8.87854897779715,84.30727308569,68.821968198105));
#122253=CARTESIAN_POINT('Ctrl Pts',(-8.67874582748115,78.13920519194,63.285515123434));
#122254=CARTESIAN_POINT('Ctrl Pts',(-8.47894267716618,69.89662703841,64.163123294247));
#122255=CARTESIAN_POINT('Ctrl Pts',(-8.34574057695515,66.65138462743,68.622440986855));
#122256=CARTESIAN_POINT('Ctrl Pts',(-8.27913952685018,66.12404568677,71.098635427588));
#122257=CARTESIAN_POINT('Ctrl Pts',(-9.87845073280442,67.62520219141,67.700413019766));
#122258=CARTESIAN_POINT('Ctrl Pts',(-9.8118496826984,66.1498345501,69.757818081886));
#122259=CARTESIAN_POINT('Ctrl Pts',(-9.6786475824874,65.03881684527,75.159924360853));
#122260=CARTESIAN_POINT('Ctrl Pts',(-9.4788444321714,69.94095953137,81.84418107373));
#122261=CARTESIAN_POINT('Ctrl Pts',(-9.2790412818554,78.18756436805,82.675374708005));
#122262=CARTESIAN_POINT('Ctrl Pts',(-9.0792381315394,84.3279816375,77.109502645435));
#122263=CARTESIAN_POINT('Ctrl Pts',(-8.8794349812234,84.30727308569,68.821968198105));
#122264=CARTESIAN_POINT('Ctrl Pts',(-8.6796318309074,78.13920519194,63.285515123434));
#122265=CARTESIAN_POINT('Ctrl Pts',(-8.47982868059242,69.89662703841,64.163123294247));
#122266=CARTESIAN_POINT('Ctrl Pts',(-8.3466265803814,66.65138462743,68.622440986855));
#122267=CARTESIAN_POINT('Ctrl Pts',(-8.28002553027642,66.12404568677,71.098635427588));
#122268=CARTESIAN_POINT('Ctrl Pts',(-9.87933673623067,67.62520219141,67.700413019766));
#122269=CARTESIAN_POINT('Ctrl Pts',(-9.81273568612466,66.1498345501,69.757818081886));
#122270=CARTESIAN_POINT('Ctrl Pts',(-9.67953358591366,65.03881684527,75.159924360853));
#122271=CARTESIAN_POINT('Ctrl Pts',(-9.47973043559766,69.94095953137,81.84418107373));
#122272=CARTESIAN_POINT('Ctrl Pts',(-9.27992728528165,78.18756436805,82.675374708005));
#122273=CARTESIAN_POINT('Ctrl Pts',(-9.08012413496566,84.3279816375,77.109502645435));
#122274=CARTESIAN_POINT('Ctrl Pts',(-8.88032098464966,84.30727308569,68.821968198105));
#122275=CARTESIAN_POINT('Ctrl Pts',(-8.68051783433366,78.13920519194,63.285515123434));
#122276=CARTESIAN_POINT('Ctrl Pts',(-8.48071468401867,69.89662703841,64.163123294247));
#122277=CARTESIAN_POINT('Ctrl Pts',(-8.34751258380766,66.65138462743,68.622440986855));
#122278=CARTESIAN_POINT('Ctrl Pts',(-8.28091153370267,66.12404568677,71.098635427588));
#122279=CARTESIAN_POINT('Ctrl Pts',(-9.88022273965691,67.62520219141,67.700413019766));
#122280=CARTESIAN_POINT('Ctrl Pts',(-9.81362168955091,66.1498345501,69.757818081886));
#122281=CARTESIAN_POINT('Ctrl Pts',(-9.68041958933991,65.03881684527,75.159924360853));
#122282=CARTESIAN_POINT('Ctrl Pts',(-9.48061643902391,69.94095953137,81.84418107373));
#122283=CARTESIAN_POINT('Ctrl Pts',(-9.28081328870791,78.18756436805,82.675374708005));
#122284=CARTESIAN_POINT('Ctrl Pts',(-9.08101013839191,84.3279816375,77.109502645435));
#122285=CARTESIAN_POINT('Ctrl Pts',(-8.88120698807591,84.30727308569,68.821968198105));
#122286=CARTESIAN_POINT('Ctrl Pts',(-8.68140383775991,78.13920519194,63.285515123434));
#122287=CARTESIAN_POINT('Ctrl Pts',(-8.48160068744491,69.89662703841,64.163123294247));
#122288=CARTESIAN_POINT('Ctrl Pts',(-8.34839858723391,66.65138462743,68.622440986855));
#122289=CARTESIAN_POINT('Ctrl Pts',(-8.28179753712891,66.12404568677,71.098635427588));
#122290=CARTESIAN_POINT('Ctrl Pts',(-9.96688940632291,67.62520219141,67.700413019766));
#122291=CARTESIAN_POINT('Ctrl Pts',(-9.90028835621791,66.1498345501,69.757818081886));
#122292=CARTESIAN_POINT('Ctrl Pts',(-9.76708625600691,65.03881684527,75.159924360853));
#122293=CARTESIAN_POINT('Ctrl Pts',(-9.56728310569091,69.94095953137,81.84418107373));
#122294=CARTESIAN_POINT('Ctrl Pts',(-9.36747995537491,78.18756436805,82.675374708005));
#122295=CARTESIAN_POINT('Ctrl Pts',(-9.16767680505891,84.3279816375,77.109502645435));
#122296=CARTESIAN_POINT('Ctrl Pts',(-8.96787365474291,84.30727308569,68.821968198105));
#122297=CARTESIAN_POINT('Ctrl Pts',(-8.76807050442691,78.13920519194,63.285515123434));
#122298=CARTESIAN_POINT('Ctrl Pts',(-8.56826735411091,69.89662703841,64.163123294247));
#122299=CARTESIAN_POINT('Ctrl Pts',(-8.43506525390091,66.65138462743,68.622440986855));
#122300=CARTESIAN_POINT('Ctrl Pts',(-8.36846420379491,66.12404568677,71.098635427588));
#122301=CARTESIAN_POINT('Ctrl Pts',(-10.0535560729899,67.62520219141,67.700413019766));
#122302=CARTESIAN_POINT('Ctrl Pts',(-9.98695502288491,66.1498345501,69.757818081886));
#122303=CARTESIAN_POINT('Ctrl Pts',(-9.85375292267391,65.03881684527,75.159924360853));
#122304=CARTESIAN_POINT('Ctrl Pts',(-9.65394977235791,69.94095953137,81.84418107373));
#122305=CARTESIAN_POINT('Ctrl Pts',(-9.45414662204191,78.18756436805,82.675374708005));
#122306=CARTESIAN_POINT('Ctrl Pts',(-9.25434347172591,84.3279816375,77.109502645435));
#122307=CARTESIAN_POINT('Ctrl Pts',(-9.05454032140991,84.30727308569,68.821968198105));
#122308=CARTESIAN_POINT('Ctrl Pts',(-8.85473717109391,78.13920519194,63.285515123434));
#122309=CARTESIAN_POINT('Ctrl Pts',(-8.65493402077791,69.89662703841,64.163123294247));
#122310=CARTESIAN_POINT('Ctrl Pts',(-8.52173192056691,66.65138462743,68.622440986855));
#122311=CARTESIAN_POINT('Ctrl Pts',(-8.45513087046191,66.12404568677,71.098635427588));
#122312=CARTESIAN_POINT('Ctrl Pts',(-10.1402227396569,67.62520219141,67.700413019766));
#122313=CARTESIAN_POINT('Ctrl Pts',(-10.0736216895509,66.1498345501,69.757818081886));
#122314=CARTESIAN_POINT('Ctrl Pts',(-9.94041958933991,65.03881684527,75.159924360853));
#122315=CARTESIAN_POINT('Ctrl Pts',(-9.74061643902391,69.94095953137,81.84418107373));
#122316=CARTESIAN_POINT('Ctrl Pts',(-9.54081328870791,78.18756436805,82.675374708005));
#122317=CARTESIAN_POINT('Ctrl Pts',(-9.34101013839191,84.3279816375,77.109502645435));
#122318=CARTESIAN_POINT('Ctrl Pts',(-9.14120698807591,84.30727308569,68.821968198105));
#122319=CARTESIAN_POINT('Ctrl Pts',(-8.94140383775991,78.13920519194,63.285515123434));
#122320=CARTESIAN_POINT('Ctrl Pts',(-8.74160068744491,69.89662703841,64.163123294247));
#122321=CARTESIAN_POINT('Ctrl Pts',(-8.60839858723391,66.65138462743,68.622440986855));
#122322=CARTESIAN_POINT('Ctrl Pts',(-8.54179753712891,66.12404568677,71.098635427588));
#122323=CARTESIAN_POINT('Ctrl Pts',(-10.1421564156154,67.62520219141,67.700413019766));
#122324=CARTESIAN_POINT('Ctrl Pts',(-10.0755553655094,66.1498345501,69.757818081886));
#122325=CARTESIAN_POINT('Ctrl Pts',(-9.94235326529838,65.03881684527,75.159924360853));
#122326=CARTESIAN_POINT('Ctrl Pts',(-9.74255011498238,69.94095953137,81.84418107373));
#122327=CARTESIAN_POINT('Ctrl Pts',(-9.54274696466638,78.18756436805,82.675374708005));
#122328=CARTESIAN_POINT('Ctrl Pts',(-9.34294381435038,84.3279816375,77.109502645435));
#122329=CARTESIAN_POINT('Ctrl Pts',(-9.14314066403438,84.30727308569,68.821968198105));
#122330=CARTESIAN_POINT('Ctrl Pts',(-8.94333751371838,78.13920519194,63.285515123434));
#122331=CARTESIAN_POINT('Ctrl Pts',(-8.7435343634034,69.89662703841,64.163123294247));
#122332=CARTESIAN_POINT('Ctrl Pts',(-8.6103322631924,66.65138462743,68.622440986855));
#122333=CARTESIAN_POINT('Ctrl Pts',(-8.5437312130874,66.12404568677,71.098635427588));
#122334=CARTESIAN_POINT('Ctrl Pts',(-10.1440900915739,67.62520219141,67.700413019766));
#122335=CARTESIAN_POINT('Ctrl Pts',(-10.0774890414678,66.1498345501,69.757818081886));
#122336=CARTESIAN_POINT('Ctrl Pts',(-9.94428694125685,65.03881684527,75.159924360853));
#122337=CARTESIAN_POINT('Ctrl Pts',(-9.74448379094085,69.94095953137,81.84418107373));
#122338=CARTESIAN_POINT('Ctrl Pts',(-9.54468064062485,78.18756436805,82.675374708005));
#122339=CARTESIAN_POINT('Ctrl Pts',(-9.34487749030885,84.3279816375,77.109502645435));
#122340=CARTESIAN_POINT('Ctrl Pts',(-9.14507433999285,84.30727308569,68.821968198105));
#122341=CARTESIAN_POINT('Ctrl Pts',(-8.94527118967685,78.13920519194,63.285515123434));
#122342=CARTESIAN_POINT('Ctrl Pts',(-8.74546803936189,69.89662703841,64.163123294247));
#122343=CARTESIAN_POINT('Ctrl Pts',(-8.61226593915089,66.65138462743,68.622440986855));
#122344=CARTESIAN_POINT('Ctrl Pts',(-8.54566488904589,66.12404568677,71.098635427588));
#122345=CARTESIAN_POINT('Ctrl Pts',(-10.1460237675324,67.62520219141,67.700413019766));
#122346=CARTESIAN_POINT('Ctrl Pts',(-10.0794227174263,66.1498345501,69.757818081886));
#122347=CARTESIAN_POINT('Ctrl Pts',(-9.94622061721532,65.03881684527,75.159924360853));
#122348=CARTESIAN_POINT('Ctrl Pts',(-9.74641746689932,69.94095953137,81.84418107373));
#122349=CARTESIAN_POINT('Ctrl Pts',(-9.54661431658332,78.18756436805,82.675374708005));
#122350=CARTESIAN_POINT('Ctrl Pts',(-9.34681116626732,84.3279816375,77.109502645435));
#122351=CARTESIAN_POINT('Ctrl Pts',(-9.14700801595132,84.30727308569,68.821968198105));
#122352=CARTESIAN_POINT('Ctrl Pts',(-8.94720486563532,78.13920519194,63.285515123434));
#122353=CARTESIAN_POINT('Ctrl Pts',(-8.74740171532038,69.89662703841,64.163123294247));
#122354=CARTESIAN_POINT('Ctrl Pts',(-8.61419961510938,66.65138462743,68.622440986855));
#122355=CARTESIAN_POINT('Ctrl Pts',(-8.54759856500438,66.12404568677,71.098635427588));
#122356=CARTESIAN_POINT('',(-10.0985254849308,67.012152548955,68.6936268712446));
#122357=CARTESIAN_POINT('',(-9.85448379345391,67.0101053268475,68.6926900228996));
#122358=CARTESIAN_POINT('Ctrl Pts',(-10.1056201537506,67.0100609947306,
68.6927734040079));
#122359=CARTESIAN_POINT('Ctrl Pts',(-10.0858657783411,66.6267587441179,
69.4137083799558));
#122360=CARTESIAN_POINT('Ctrl Pts',(-10.0674517206336,66.3421922385653,
70.187160389714));
#122361=CARTESIAN_POINT('Ctrl Pts',(-10.0354771245178,66.0641744360156,
71.41530529054));
#122362=CARTESIAN_POINT('Ctrl Pts',(-10.0234229206655,65.9970171979819,
71.8541444907421));
#122363=CARTESIAN_POINT('Ctrl Pts',(-10.0022989220673,65.9387470053738,
72.5774629218321));
#122364=CARTESIAN_POINT('Ctrl Pts',(-9.99380990519663,65.9289357827518,
72.8605855183034));
#122365=CARTESIAN_POINT('Ctrl Pts',(-9.97011755037087,65.9384360540978,
73.6524999818985));
#122366=CARTESIAN_POINT('Ctrl Pts',(-9.95498934267005,65.9872704953509,
74.1608327726866));
#122367=CARTESIAN_POINT('Ctrl Pts',(-9.93289270928219,66.1395396585373,
74.9780926170575));
#122368=CARTESIAN_POINT('Ctrl Pts',(-9.92514464639115,66.2160738287241,
75.2894488228344));
#122369=CARTESIAN_POINT('Ctrl Pts',(-9.90675928447394,66.4481877519415,
76.0511949084095));
#122370=CARTESIAN_POINT('Ctrl Pts',(-9.89630776232476,66.6238583447981,
76.4950140682969));
#122371=CARTESIAN_POINT('Ctrl Pts',(-9.87665530166429,66.9867250370315,
77.2381296826608));
#122372=CARTESIAN_POINT('Ctrl Pts',(-9.86799181905648,67.1588289504397,
77.5448386454165));
#122373=CARTESIAN_POINT('Ctrl Pts',(-9.83474755552943,67.8577859554754,
78.6415461446342));
#122374=CARTESIAN_POINT('Ctrl Pts',(-9.80803618459269,68.4906818730782,
79.3663681222012));
#122375=CARTESIAN_POINT('Ctrl Pts',(-9.76845513375547,69.5268040522261,
80.2340080815034));
#122376=CARTESIAN_POINT('Ctrl Pts',(-9.75634104363941,69.8522607993321,
80.471575968419));
#122377=CARTESIAN_POINT('Ctrl Pts',(-9.73562568268234,70.4685501783667,
80.8586624789983));
#122378=CARTESIAN_POINT('Ctrl Pts',(-9.72704885670965,70.7519521275781,
81.0148065063888));
#122379=CARTESIAN_POINT('Ctrl Pts',(-9.70232993771758,71.6516208700326,
81.4468481791628));
#122380=CARTESIAN_POINT('Ctrl Pts',(-9.68780978107427,72.2924085246533,
81.6680928606966));
#122381=CARTESIAN_POINT('Ctrl Pts',(-9.66477679705922,73.2570983554498,
81.8880275039081));
#122382=CARTESIAN_POINT('Ctrl Pts',(-9.65716697850892,73.5685498652193,
81.9425296255044));
#122383=CARTESIAN_POINT('Ctrl Pts',(-9.63079350027746,74.5787643785797,
82.0672627216527));
#122384=CARTESIAN_POINT('Ctrl Pts',(-9.60979911610278,75.2860288566837,
82.0752133493487));
#122385=CARTESIAN_POINT('Ctrl Pts',(-9.57636424384008,76.408719975205,81.9587410683443));
#122386=CARTESIAN_POINT('Ctrl Pts',(-9.5638092569189,76.8300110796484,81.8849983390011));
#122387=CARTESIAN_POINT('Ctrl Pts',(-9.53999615768963,77.6650508781469,
81.6749819617454));
#122388=CARTESIAN_POINT('Ctrl Pts',(-9.52918351341566,78.0735305819472,
81.5388149512676));
#122389=CARTESIAN_POINT('Ctrl Pts',(-9.49784468673609,79.2748170163315,
81.0356105848816));
#122390=CARTESIAN_POINT('Ctrl Pts',(-9.47764772497503,80.0258135580735,
80.5810569454226));
#122391=CARTESIAN_POINT('Ctrl Pts',(-9.43962677527073,81.2030303086033,
79.6247405516389));
#122392=CARTESIAN_POINT('Ctrl Pts',(-9.42246712903821,81.6641786070497,
79.1635366659919));
#122393=CARTESIAN_POINT('Ctrl Pts',(-9.39387315677519,82.2894133043008,
78.3914213853036));
#122394=CARTESIAN_POINT('Ctrl Pts',(-9.38341740832812,82.4917721834501,
78.1107530810851));
#122395=CARTESIAN_POINT('Ctrl Pts',(-9.35973644735305,82.9139163017574,
77.4477969979189));
#122396=CARTESIAN_POINT('Ctrl Pts',(-9.34660691469877,83.1230928738138,
77.0589116166437));
#122397=CARTESIAN_POINT('Ctrl Pts',(-9.32459867969423,83.4586217794764,
76.2993696292396));
#122398=CARTESIAN_POINT('Ctrl Pts',(-9.31541138867127,83.5915616317143,
75.932183219999));
#122399=CARTESIAN_POINT('Ctrl Pts',(-9.28836179847158,83.9228722685685,
74.7883461178696));
#122400=CARTESIAN_POINT('Ctrl Pts',(-9.27067528707267,84.0422668468796,
73.9887398515901));
#122401=CARTESIAN_POINT('Ctrl Pts',(-9.23609197264821,84.0696989172094,
72.6868145105387));
#122402=CARTESIAN_POINT('Ctrl Pts',(-9.2218955699631,84.0401778552934,72.1848321359113));
#122403=CARTESIAN_POINT('Ctrl Pts',(-9.18306129567446,83.8528090878916,
70.8507049131391));
#122404=CARTESIAN_POINT('Ctrl Pts',(-9.15351833944773,83.6043238906748,
69.8915616477434));
#122405=CARTESIAN_POINT('Ctrl Pts',(-9.11312336352832,82.8859730463364,
68.4763625114011));
#122406=CARTESIAN_POINT('Ctrl Pts',(-9.1018164298601,82.6346820516927,68.0685004412505));
#122407=CARTESIAN_POINT('Ctrl Pts',(-9.07160828662411,81.8749572103008,
67.0276762953672));
#122408=CARTESIAN_POINT('Ctrl Pts',(-9.05281212830922,81.3090550776609,
66.4356804440943));
#122409=CARTESIAN_POINT('Ctrl Pts',(-9.02087352722843,80.3919244403997,
65.6954459142547));
#122410=CARTESIAN_POINT('Ctrl Pts',(-9.01014874711913,80.0922263287438,
65.4813487697423));
#122411=CARTESIAN_POINT('Ctrl Pts',(-8.97802486309619,79.1834863086863,
64.9109673589789));
#122412=CARTESIAN_POINT('Ctrl Pts',(-8.95607643694238,78.5430298334253,
64.604680300816));
#122413=CARTESIAN_POINT('Ctrl Pts',(-8.93114078948074,77.6373105266441,
64.3018784374812));
#122414=CARTESIAN_POINT('Ctrl Pts',(-8.92511398649856,77.3977461094428,
64.2333870070539));
#122415=CARTESIAN_POINT('Ctrl Pts',(-8.90618495150541,76.6077965411486,
64.0434804307023));
#122416=CARTESIAN_POINT('Ctrl Pts',(-8.89392940839807,76.0470459905734,
63.9647069748064));
#122417=CARTESIAN_POINT('Ctrl Pts',(-8.8621805569852,74.7288603894014,63.9009008652572));
#122418=CARTESIAN_POINT('Ctrl Pts',(-8.8423851688574,73.9685550763677,63.9568528698512));
#122419=CARTESIAN_POINT('Ctrl Pts',(-8.79712880032208,72.3679595129946,
64.2710478711938));
#122420=CARTESIAN_POINT('Ctrl Pts',(-8.77056908072397,71.5320945510507,
64.5602948838878));
#122421=CARTESIAN_POINT('Ctrl Pts',(-8.7356019826268,70.44819469651,65.1297891983091));
#122422=CARTESIAN_POINT('Ctrl Pts',(-8.72638528489723,70.1513073666477,
65.3098447556629));
#122423=CARTESIAN_POINT('Ctrl Pts',(-8.70755440340243,69.5281095573045,
65.7405384651327));
#122424=CARTESIAN_POINT('Ctrl Pts',(-8.69809474021031,69.2072887729914,
65.9972096785191));
#122425=CARTESIAN_POINT('Ctrl Pts',(-8.67461105541209,68.4536022927773,
66.6882193607657));
#122426=CARTESIAN_POINT('Ctrl Pts',(-8.66059211699792,68.0436150970389,
67.14774252102));
#122427=CARTESIAN_POINT('Ctrl Pts',(-8.62796634820956,67.3144144402831,
68.146245304326));
#122428=CARTESIAN_POINT('Ctrl Pts',(-8.60948912160607,66.9966010470373,
68.6871096557166));
#122429=CARTESIAN_POINT('Ctrl Pts',(-8.58347171193975,66.6287424326869,
69.4905465658079));
#122430=CARTESIAN_POINT('Ctrl Pts',(-8.57584088745256,66.530635313355,69.7314186039164));
#122431=CARTESIAN_POINT('Ctrl Pts',(-8.56837920259168,66.4431891936119,
69.9761209669341));
#122432=CARTESIAN_POINT('Ctrl Pts',(-9.99199816632791,67.59428425961,67.303209521688));
#122433=CARTESIAN_POINT('Ctrl Pts',(-9.95025389358791,66.60009764549,68.598158170228));
#122434=CARTESIAN_POINT('Ctrl Pts',(-9.86676534810891,65.30823381695,71.71969580549));
#122435=CARTESIAN_POINT('Ctrl Pts',(-9.74153252989091,65.975649193,76.744817636531));
#122436=CARTESIAN_POINT('Ctrl Pts',(-9.61629971167191,69.0702482942,80.759474381881));
#122437=CARTESIAN_POINT('Ctrl Pts',(-9.49106689345391,73.75942478415,82.684532165368));
#122438=CARTESIAN_POINT('Ctrl Pts',(-9.36583407523591,78.78224537899,82.00215805984));
#122439=CARTESIAN_POINT('Ctrl Pts',(-9.24060125701691,82.78791878897,78.895896207008));
#122440=CARTESIAN_POINT('Ctrl Pts',(-9.11536843879891,84.6992258503,74.201089045577));
#122441=CARTESIAN_POINT('Ctrl Pts',(-8.99013562057991,84.00216577159,69.180291345096));
#122442=CARTESIAN_POINT('Ctrl Pts',(-8.86490280236191,80.88419637879,65.183721669986));
#122443=CARTESIAN_POINT('Ctrl Pts',(-8.73966998414291,76.18381732287,63.28615857581));
#122444=CARTESIAN_POINT('Ctrl Pts',(-8.61443716592491,71.16508250412,63.997905008714));
#122445=CARTESIAN_POINT('Ctrl Pts',(-8.48920434770591,67.17764413613,67.127552977624));
#122446=CARTESIAN_POINT('Ctrl Pts',(-8.36397152948791,65.29387078721,71.833466448308));
#122447=CARTESIAN_POINT('Ctrl Pts',(-8.23873871126891,66.02018597587,76.850086687758));
#122448=CARTESIAN_POINT('Ctrl Pts',(-8.11350589305091,69.16190222137,80.828391821067));
#122449=CARTESIAN_POINT('Ctrl Pts',(-8.03001734757191,72.30180432462,82.07495675794));
#122450=CARTESIAN_POINT('Ctrl Pts',(-7.98827307483191,73.92349052215,82.263193053033));
#122451=CARTESIAN_POINT('Ctrl Pts',(-10.2225811782039,67.91107137654,67.546420332812));
#122452=CARTESIAN_POINT('Ctrl Pts',(-10.1808369054639,66.95941211861,68.78597621942));
#122453=CARTESIAN_POINT('Ctrl Pts',(-10.0973483599859,65.72280909565,71.77398686789));
#122454=CARTESIAN_POINT('Ctrl Pts',(-9.97211554176791,66.36167509171,76.584153937925));
#122455=CARTESIAN_POINT('Ctrl Pts',(-9.84688272354991,69.32389952966,80.42707960685));
#122456=CARTESIAN_POINT('Ctrl Pts',(-9.72164990533191,73.81249166652,82.269791061293));
#122457=CARTESIAN_POINT('Ctrl Pts',(-9.59641708711391,78.6204559381,81.616606210807));
#122458=CARTESIAN_POINT('Ctrl Pts',(-9.47118426889691,82.45478254308,78.643217907434));
#122459=CARTESIAN_POINT('Ctrl Pts',(-9.34595145067991,84.28433147665,74.149235956863));
#122460=CARTESIAN_POINT('Ctrl Pts',(-9.22071863246191,83.61708886061,69.343208048245));
#122461=CARTESIAN_POINT('Ctrl Pts',(-9.09548581424491,80.63249381933,65.517595756513));
#122462=CARTESIAN_POINT('Ctrl Pts',(-8.97025299602791,76.13317831779,63.701202877746));
#122463=CARTESIAN_POINT('Ctrl Pts',(-8.84502017781091,71.32912504901,64.382503624079));
#122464=CARTESIAN_POINT('Ctrl Pts',(-8.71978735959391,67.51225346334,67.37827767835));
#122465=CARTESIAN_POINT('Ctrl Pts',(-8.59455454137691,65.70906045929,71.88289085437));
#122466=CARTESIAN_POINT('Ctrl Pts',(-8.46932172315991,66.40430676786,76.684919997149));
#122467=CARTESIAN_POINT('Ctrl Pts',(-8.34408890494191,69.41163286577,80.493049031652));
#122468=CARTESIAN_POINT('Ctrl Pts',(-8.26060035946391,72.41722242321,81.686290869658));
#122469=CARTESIAN_POINT('Ctrl Pts',(-8.21885608672491,73.96953932369,81.866475163376));
#122470=CARTESIAN_POINT('Ctrl Pts',(-10.4531641900799,68.22785849346,67.789631143935));
#122471=CARTESIAN_POINT('Ctrl Pts',(-10.4114199173409,67.31872659173,68.973794268612));
#122472=CARTESIAN_POINT('Ctrl Pts',(-10.3279313718619,66.13738437435,71.82827793029));
#122473=CARTESIAN_POINT('Ctrl Pts',(-10.2026985536429,66.74770099042,76.423490239315));
#122474=CARTESIAN_POINT('Ctrl Pts',(-10.0774657354239,69.57755076511,80.09468483181));
#122475=CARTESIAN_POINT('Ctrl Pts',(-9.95223291720491,73.86555854886,81.855049957214));
#122476=CARTESIAN_POINT('Ctrl Pts',(-9.82700009898591,78.45866649718,81.231054361786));
#122477=CARTESIAN_POINT('Ctrl Pts',(-9.70176728076691,82.12164629715,78.390539607897));
#122478=CARTESIAN_POINT('Ctrl Pts',(-9.57653446254691,83.86943710299,74.097382868212));
#122479=CARTESIAN_POINT('Ctrl Pts',(-9.45130164432791,83.23201194965,69.506124751474));
#122480=CARTESIAN_POINT('Ctrl Pts',(-9.32606882610791,80.38079125995,65.851469843104));
#122481=CARTESIAN_POINT('Ctrl Pts',(-9.20083600788791,76.08253931283,64.116247179702));
#122482=CARTESIAN_POINT('Ctrl Pts',(-9.07560318966791,71.49316759404,64.76710223939));
#122483=CARTESIAN_POINT('Ctrl Pts',(-8.95037037144891,67.84686279065,67.629002378947));
#122484=CARTESIAN_POINT('Ctrl Pts',(-8.82513755322891,66.1242501314,71.932315260248));
#122485=CARTESIAN_POINT('Ctrl Pts',(-8.69990473500891,66.78842755977,76.519753306352));
#122486=CARTESIAN_POINT('Ctrl Pts',(-8.57467191678891,69.66136350999,80.1577062421));
#122487=CARTESIAN_POINT('Ctrl Pts',(-8.49118337130991,72.53264052159,81.29762498131));
#122488=CARTESIAN_POINT('Ctrl Pts',(-8.44943909856991,74.01558812501,81.469757273692));
#122489=CARTESIAN_POINT('Ctrl Pts',(-10.6837472019569,68.54464561039,68.032841955058));
#122490=CARTESIAN_POINT('Ctrl Pts',(-10.6420029292169,67.67804106486,69.161612317803));
#122491=CARTESIAN_POINT('Ctrl Pts',(-10.5585143837379,66.55195965305,71.882568992689));
#122492=CARTESIAN_POINT('Ctrl Pts',(-10.4332815655199,67.13372688913,76.262826540709));
#122493=CARTESIAN_POINT('Ctrl Pts',(-10.3080487473019,69.83120200056,79.762290056778));
#122494=CARTESIAN_POINT('Ctrl Pts',(-10.1828159290829,73.91862543122,81.440308853139));
#122495=CARTESIAN_POINT('Ctrl Pts',(-10.0575831108649,78.29687705629,80.845502512754));
#122496=CARTESIAN_POINT('Ctrl Pts',(-9.93235029264591,81.78851005125,78.137861308325));
#122497=CARTESIAN_POINT('Ctrl Pts',(-9.80711747442791,83.45454272935,74.0455297795));
#122498=CARTESIAN_POINT('Ctrl Pts',(-9.68188465620991,82.84693503866,69.669041454627));
#122499=CARTESIAN_POINT('Ctrl Pts',(-9.55665183799091,80.1290887005,66.185343929634));
#122500=CARTESIAN_POINT('Ctrl Pts',(-9.43141901977291,76.03190030776,64.531291481639));
#122501=CARTESIAN_POINT('Ctrl Pts',(-9.30618620155491,71.65721013894,65.151700854752));
#122502=CARTESIAN_POINT('Ctrl Pts',(-9.18095338333591,68.18147211787,67.879727079667));
#122503=CARTESIAN_POINT('Ctrl Pts',(-9.05572056511791,66.53943980348,71.981739666301));
#122504=CARTESIAN_POINT('Ctrl Pts',(-8.93048774689891,67.17254835176,76.354586615735));
#122505=CARTESIAN_POINT('Ctrl Pts',(-8.80525492868091,69.91109415439,79.822363452678));
#122506=CARTESIAN_POINT('Ctrl Pts',(-8.72176638320191,72.64805862017,80.908959093025));
#122507=CARTESIAN_POINT('Ctrl Pts',(-8.68002211046191,74.06163692655,81.073039384034));
#122508=CARTESIAN_POINT('',(-10.0976119119436,67.0107639369115,68.6928899475042));
#122509=CARTESIAN_POINT('Ctrl Pts',(-13.1454639400434,80.45858984268,79.025262748814));
#122510=CARTESIAN_POINT('Ctrl Pts',(-13.1047676696649,81.48759917444,78.094747098224));
#122511=CARTESIAN_POINT('Ctrl Pts',(-13.023375128908,83.05789139581,75.697173136178));
#122512=CARTESIAN_POINT('Ctrl Pts',(-12.9012863177725,83.35252030674,71.406833513058));
#122513=CARTESIAN_POINT('Ctrl Pts',(-12.779197506637,81.50958548889,67.521577101676));
#122514=CARTESIAN_POINT('Ctrl Pts',(-12.6571086955016,78.00102966728,65.03524813757));
#122515=CARTESIAN_POINT('Ctrl Pts',(-12.535019884366,73.72453794147,64.584146732116));
#122516=CARTESIAN_POINT('Ctrl Pts',(-12.4129310732305,69.77442198226,66.283678758148));
#122517=CARTESIAN_POINT('Ctrl Pts',(-12.2908422620949,67.16144589233,69.698967665193));
#122518=CARTESIAN_POINT('Ctrl Pts',(-12.1687534509593,66.5542301033,73.956094258219));
#122519=CARTESIAN_POINT('Ctrl Pts',(-12.0466646398237,68.10815086311,77.965728779761));
#122520=CARTESIAN_POINT('Ctrl Pts',(-11.9245758286881,71.42558498136,80.70187013362));
#122521=CARTESIAN_POINT('Ctrl Pts',(-11.8024870175525,75.65765439615,81.464383794463));
#122522=CARTESIAN_POINT('Ctrl Pts',(-11.6803982064169,79.72144063224,80.058154773716));
#122523=CARTESIAN_POINT('Ctrl Pts',(-11.5583093952809,82.57708616044,76.843014459137));
#122524=CARTESIAN_POINT('Ctrl Pts',(-11.4362205841459,83.49387722752,72.6416655369233));
#122525=CARTESIAN_POINT('Ctrl Pts',(-11.3141317730099,82.23722174699,68.52916561233));
#122526=CARTESIAN_POINT('Ctrl Pts',(-11.1920429618739,79.12867764146,65.557837261156));
#122527=CARTESIAN_POINT('Ctrl Pts',(-11.0699541507389,74.96367134257,64.48799561084));
#122528=CARTESIAN_POINT('Ctrl Pts',(-10.9478653396029,70.80796096272,65.593395929895));
#122529=CARTESIAN_POINT('Ctrl Pts',(-10.8257765284669,67.72492593816,68.59118405853));
#122530=CARTESIAN_POINT('Ctrl Pts',(-10.7036877173319,66.50346533712,72.714274237664));
#122531=CARTESIAN_POINT('Ctrl Pts',(-10.5815989061959,67.45613127848,76.907634016596));
#122532=CARTESIAN_POINT('Ctrl Pts',(-10.4595100950609,70.33915187332,80.09825008004));
#122533=CARTESIAN_POINT('Ctrl Pts',(-10.3374212839249,74.4148085262,81.46969511541));
#122534=CARTESIAN_POINT('Ctrl Pts',(-10.2153324727889,78.64020627051,80.671038351543));
#122535=CARTESIAN_POINT('Ctrl Pts',(-10.0932436616539,81.93413376206,77.906643386292));
#122536=CARTESIAN_POINT('Ctrl Pts',(-9.97115485051791,83.45372806371,73.8838737528785));
#122537=CARTESIAN_POINT('Ctrl Pts',(-9.84906603938191,82.81014898713,69.632093987784));
#122538=CARTESIAN_POINT('Ctrl Pts',(-9.72697722824691,80.16807974905,66.239256812192));
#122539=CARTESIAN_POINT('Ctrl Pts',(-9.60488841711091,76.20357708221,64.573569483865));
#122540=CARTESIAN_POINT('Ctrl Pts',(-9.48279960597591,71.93111689791,65.061124710008));
#122541=CARTESIAN_POINT('Ctrl Pts',(-9.36071079483991,68.44386550154,67.577649690078));
#122542=CARTESIAN_POINT('Ctrl Pts',(-9.27931825408291,67.23760922485,70.177481292106));
#122543=CARTESIAN_POINT('Ctrl Pts',(-9.23862198370491,66.9910877936,71.542745649207));
#122544=CARTESIAN_POINT('Ctrl Pts',(-13.3760469519197,80.72646219088,79.321488981906));
#122545=CARTESIAN_POINT('Ctrl Pts',(-13.3353506815413,81.80596865723,78.345309630701));
#122546=CARTESIAN_POINT('Ctrl Pts',(-13.2539581407843,83.45332068284,75.83007821761));
#122547=CARTESIAN_POINT('Ctrl Pts',(-13.1318693296489,83.76240807855,71.329196424715));
#122548=CARTESIAN_POINT('Ctrl Pts',(-13.0097805185134,81.82903391805,67.253276712327));
#122549=CARTESIAN_POINT('Ctrl Pts',(-12.8876917073779,78.14830082834,64.644934774693));
#122550=CARTESIAN_POINT('Ctrl Pts',(-12.7656028962424,73.66194649816,64.171696224628));
#122551=CARTESIAN_POINT('Ctrl Pts',(-12.6435140851068,69.51798435007,65.954630310129));
#122552=CARTESIAN_POINT('Ctrl Pts',(-12.5214252739713,66.77678026333,69.537519547239));
#122553=CARTESIAN_POINT('Ctrl Pts',(-12.3993364628357,66.13976624364,74.003558428952));
#122554=CARTESIAN_POINT('Ctrl Pts',(-12.2772476517001,67.76994340206,78.209959926145));
#122555=CARTESIAN_POINT('Ctrl Pts',(-12.1551588405645,71.2501757691,81.080373432798));
#122556=CARTESIAN_POINT('Ctrl Pts',(-12.0330700294289,75.68992782805,81.880306341227));
#122557=CARTESIAN_POINT('Ctrl Pts',(-11.9109812182932,79.95313845632,80.405068678906));
#122558=CARTESIAN_POINT('Ctrl Pts',(-11.7888924071576,82.94892063066,77.032150034994));
#122559=CARTESIAN_POINT('Ctrl Pts',(-11.666803596022,83.91070188439,72.624626032068));
#122560=CARTESIAN_POINT('Ctrl Pts',(-11.5447147848859,82.59237786598,68.310311161955));
#122561=CARTESIAN_POINT('Ctrl Pts',(-11.4226259737509,79.33128648485,65.193169198556));
#122562=CARTESIAN_POINT('Ctrl Pts',(-11.3005371626149,74.96188856657,64.070826627081));
#122563=CARTESIAN_POINT('Ctrl Pts',(-11.1784483514789,70.60224275103,65.23047285722));
#122564=CARTESIAN_POINT('Ctrl Pts',(-11.0563595403439,67.36791227191,68.375373073155));
#122565=CARTESIAN_POINT('Ctrl Pts',(-10.9342707292079,66.08651027048,72.7007978991383));
#122566=CARTESIAN_POINT('Ctrl Pts',(-10.8121819180729,67.08592690573,77.0999407032));
#122567=CARTESIAN_POINT('Ctrl Pts',(-10.6900931069369,70.11042753827,80.447131604038));
#122568=CARTESIAN_POINT('Ctrl Pts',(-10.5680042958009,74.38609110676,81.885878307519));
#122569=CARTESIAN_POINT('Ctrl Pts',(-10.4459154846659,78.8188440927,81.048028625887));
#122570=CARTESIAN_POINT('Ctrl Pts',(-10.3238266735299,82.27441627954,78.147975002984));
#122571=CARTESIAN_POINT('Ctrl Pts',(-10.2017378623939,83.86858245883,73.9277938074277));
#122572=CARTESIAN_POINT('Ctrl Pts',(-10.0796490512589,83.19342067618,69.46736414145));
#122573=CARTESIAN_POINT('Ctrl Pts',(-9.95756024012291,80.4216957374,65.908028421839));
#122574=CARTESIAN_POINT('Ctrl Pts',(-9.83547142898791,76.26264087496,64.160599913318));
#122575=CARTESIAN_POINT('Ctrl Pts',(-9.71338261785191,71.78051592832,64.672081202253));
#122576=CARTESIAN_POINT('Ctrl Pts',(-9.59129380671691,68.12213274751,67.312100981366));
#122577=CARTESIAN_POINT('Ctrl Pts',(-9.50990126595991,66.8566812005,70.039515533604));
#122578=CARTESIAN_POINT('Ctrl Pts',(-9.46920499558091,66.59806208898,71.471778251044));
#122579=CARTESIAN_POINT('Ctrl Pts',(-13.6066299637959,80.99433453906,79.617715215002));
#122580=CARTESIAN_POINT('Ctrl Pts',(-13.5659336934176,82.12433814002,78.595872163185));
#122581=CARTESIAN_POINT('Ctrl Pts',(-13.4845411526607,83.84874996986,75.962983299055));
#122582=CARTESIAN_POINT('Ctrl Pts',(-13.3624523415252,84.17229585037,71.251559336391));
#122583=CARTESIAN_POINT('Ctrl Pts',(-13.2403635303897,82.14848234721,66.984976322999));
#122584=CARTESIAN_POINT('Ctrl Pts',(-13.1182747192542,78.29557198944,64.254621411829));
#122585=CARTESIAN_POINT('Ctrl Pts',(-12.9961859081187,73.59935505488,63.759245717135));
#122586=CARTESIAN_POINT('Ctrl Pts',(-12.8740970969832,69.26154671793,65.625581862084));
#122587=CARTESIAN_POINT('Ctrl Pts',(-12.7520082858476,66.39211463435,69.376071429236));
#122588=CARTESIAN_POINT('Ctrl Pts',(-12.629919474712,65.72530238397,74.051022599625));
#122589=CARTESIAN_POINT('Ctrl Pts',(-12.5078306635765,67.43173594097,78.454191072474));
#122590=CARTESIAN_POINT('Ctrl Pts',(-12.3857418524408,71.07476655678,81.458876731945));
#122591=CARTESIAN_POINT('Ctrl Pts',(-12.2636530413052,75.72220125986,82.296228887996));
#122592=CARTESIAN_POINT('Ctrl Pts',(-12.1415642301696,80.18483628034,80.751982584142));
#122593=CARTESIAN_POINT('Ctrl Pts',(-12.0194754190339,83.32075510084,77.221285610932));
#122594=CARTESIAN_POINT('Ctrl Pts',(-11.8973866078983,84.32752654126,72.6075865273095));
#122595=CARTESIAN_POINT('Ctrl Pts',(-11.7752977967627,82.94753398501,68.091456711666));
#122596=CARTESIAN_POINT('Ctrl Pts',(-11.653208985627,79.53389532833,64.828501136008));
#122597=CARTESIAN_POINT('Ctrl Pts',(-11.5311201744909,74.96010579067,63.653657643322));
#122598=CARTESIAN_POINT('Ctrl Pts',(-11.4090313633559,70.39652453943,64.867549784492));
#122599=CARTESIAN_POINT('Ctrl Pts',(-11.2869425522199,67.01089860571,68.159562087686));
#122600=CARTESIAN_POINT('Ctrl Pts',(-11.1648537410839,65.66955520384,72.6873215605024));
#122601=CARTESIAN_POINT('Ctrl Pts',(-11.0427649299489,66.71572253294,77.292247389707));
#122602=CARTESIAN_POINT('Ctrl Pts',(-10.9206761188129,69.88170320312,80.796013127978));
#122603=CARTESIAN_POINT('Ctrl Pts',(-10.7985873076779,74.35737368722,82.302061499622));
#122604=CARTESIAN_POINT('Ctrl Pts',(-10.6764984965419,78.99748191481,81.425018900273));
#122605=CARTESIAN_POINT('Ctrl Pts',(-10.5544096854059,82.61469879698,78.389306619751));
#122606=CARTESIAN_POINT('Ctrl Pts',(-10.4323208742709,84.28343685395,73.9717138620569));
#122607=CARTESIAN_POINT('Ctrl Pts',(-10.3102320631349,83.57669236526,69.30263429518));
#122608=CARTESIAN_POINT('Ctrl Pts',(-10.1881432519999,80.67531172579,65.57680003152));
#122609=CARTESIAN_POINT('Ctrl Pts',(-10.0660544408639,76.32170466775,63.747630342775));
#122610=CARTESIAN_POINT('Ctrl Pts',(-9.94396562972891,71.62991495875,64.283037694485));
#122611=CARTESIAN_POINT('Ctrl Pts',(-9.82187681859291,67.80039999349,67.046552272646));
#122612=CARTESIAN_POINT('Ctrl Pts',(-9.74048427783591,66.47575317615,69.901549775107));
#122613=CARTESIAN_POINT('Ctrl Pts',(-9.69978800745791,66.20503638435,71.400810852893));
#122614=CARTESIAN_POINT('Ctrl Pts',(-13.8372129756729,81.26220688726,79.913941448094));
#122615=CARTESIAN_POINT('Ctrl Pts',(-13.7965167052939,82.44270762281,78.846434695661));
#122616=CARTESIAN_POINT('Ctrl Pts',(-13.7151241645369,84.24417925689,76.095888380488));
#122617=CARTESIAN_POINT('Ctrl Pts',(-13.5930353534019,84.58218362219,71.173922248048));
#122618=CARTESIAN_POINT('Ctrl Pts',(-13.4709465422661,82.46793077636,66.716675933649));
#122619=CARTESIAN_POINT('Ctrl Pts',(-13.3488577311306,78.4428431505,63.864308048952));
#122620=CARTESIAN_POINT('Ctrl Pts',(-13.2267689199951,73.53676361156,63.346795209648));
#122621=CARTESIAN_POINT('Ctrl Pts',(-13.1046801088595,69.00510908574,65.296533414067));
#122622=CARTESIAN_POINT('Ctrl Pts',(-12.982591297724,66.00744900535,69.214623311284));
#122623=CARTESIAN_POINT('Ctrl Pts',(-12.8605024865884,65.31083852431,74.098486770361));
#122624=CARTESIAN_POINT('Ctrl Pts',(-12.7384136754528,67.09352847992,78.698422218861));
#122625=CARTESIAN_POINT('Ctrl Pts',(-12.6163248643172,70.89935734453,81.837380031125));
#122626=CARTESIAN_POINT('Ctrl Pts',(-12.4942360531816,75.75447469176,82.71215143476));
#122627=CARTESIAN_POINT('Ctrl Pts',(-12.3721472420459,80.41653410443,81.098896489329));
#122628=CARTESIAN_POINT('Ctrl Pts',(-12.2500584309103,83.69258957107,77.410421186785));
#122629=CARTESIAN_POINT('Ctrl Pts',(-12.1279696197746,84.74435119813,72.5905470224495));
#122630=CARTESIAN_POINT('Ctrl Pts',(-12.005880808639,83.302690104,67.872602261286));
#122631=CARTESIAN_POINT('Ctrl Pts',(-11.8837919975033,79.73650417172,64.463833073406));
#122632=CARTESIAN_POINT('Ctrl Pts',(-11.7617031863677,74.95832301467,63.236488659563));
#122633=CARTESIAN_POINT('Ctrl Pts',(-11.639614375232,70.19080632774,64.50462671182));
#122634=CARTESIAN_POINT('Ctrl Pts',(-11.5175255640959,66.65388493945,67.943751102315));
#122635=CARTESIAN_POINT('Ctrl Pts',(-11.3954367529609,65.25260013719,72.6738452219821));
#122636=CARTESIAN_POINT('Ctrl Pts',(-11.2733479418249,66.34551816019,77.484554076315));
#122637=CARTESIAN_POINT('Ctrl Pts',(-11.1512591306899,69.65297886808,81.144894651979));
#122638=CARTESIAN_POINT('Ctrl Pts',(-11.0291703195539,74.32865626779,82.718244691732));
#122639=CARTESIAN_POINT('Ctrl Pts',(-10.9070815084179,79.176119737,81.802009174614));
#122640=CARTESIAN_POINT('Ctrl Pts',(-10.7849926972829,82.95498131447,78.63063823644));
#122641=CARTESIAN_POINT('Ctrl Pts',(-10.6629038861469,84.69829124907,74.015633916602));
#122642=CARTESIAN_POINT('Ctrl Pts',(-10.5408150750119,83.95996405431,69.137904448843));
#122643=CARTESIAN_POINT('Ctrl Pts',(-10.4187262638759,80.92892771414,65.245571641166));
#122644=CARTESIAN_POINT('Ctrl Pts',(-10.2966374527399,76.3807684605,63.334660772228));
#122645=CARTESIAN_POINT('Ctrl Pts',(-10.1745486416049,71.47931398915,63.89399418673));
#122646=CARTESIAN_POINT('Ctrl Pts',(-10.0524598304689,67.47866723947,66.781003563935));
#122647=CARTESIAN_POINT('Ctrl Pts',(-9.97106728971191,66.0948251518,69.763584016604));
#122648=CARTESIAN_POINT('Ctrl Pts',(-9.93037101933391,65.81201067972,71.32984345473));
#122649=CARTESIAN_POINT('',(-13.5671411043958,83.559062666398,76.0030398856965));
#122650=CARTESIAN_POINT('Ctrl Pts',(-13.5675364833309,83.5597121396993,
76.003284345909));
#122651=CARTESIAN_POINT('Ctrl Pts',(-13.5675364833309,83.4568123740149,
76.2576560644358));
#122652=CARTESIAN_POINT('Ctrl Pts',(-13.5675364833306,83.3421517896857,
76.5072491508691));
#122653=CARTESIAN_POINT('Ctrl Pts',(-13.5675364833306,83.0901412786061,
76.9958065667943));
#122654=CARTESIAN_POINT('Ctrl Pts',(-13.5675364833309,82.9527179931296,
77.2347267130182));
#122655=CARTESIAN_POINT('Ctrl Pts',(-13.5675364833309,82.8047338290467,
77.4669045928492));
#122656=CARTESIAN_POINT('Ctrl Pts',(-13.5667373703007,83.5584173721563,
76.0027980283233));
#122657=CARTESIAN_POINT('Ctrl Pts',(-13.564075594742,83.592340938489,75.9066576672772));
#122658=CARTESIAN_POINT('Ctrl Pts',(-13.5614443082188,83.6246588263767,
75.8099515860624));
#122659=CARTESIAN_POINT('Ctrl Pts',(-13.5528805561748,83.7255380217485,
75.4903852147587));
#122660=CARTESIAN_POINT('Ctrl Pts',(-13.5470489678549,83.7872128263381,
75.2653495867716));
#122661=CARTESIAN_POINT('Ctrl Pts',(-13.5345639614118,83.9002282736153,
74.7800787709895));
#122662=CARTESIAN_POINT('Ctrl Pts',(-13.5279027197026,83.9490273837395,
74.5191127785177));
#122663=CARTESIAN_POINT('Ctrl Pts',(-13.5172661848976,84.0062659030078,
74.1128779791592));
#122664=CARTESIAN_POINT('Ctrl Pts',(-13.5134514878214,84.0229649995657,
73.9689943804952));
#122665=CARTESIAN_POINT('Ctrl Pts',(-13.5006780599591,84.0667101876582,
73.4915677406669));
#122666=CARTESIAN_POINT('Ctrl Pts',(-13.49153011449,84.0786264963019,73.1566509078807));
#122667=CARTESIAN_POINT('Ctrl Pts',(-13.4729263825575,84.0655098046931,
72.4769062914134));
#122668=CARTESIAN_POINT('Ctrl Pts',(-13.4634705515801,84.0392880090477,
72.1320526846346));
#122669=CARTESIAN_POINT('Ctrl Pts',(-13.450356846143,83.9744742638213,71.6448625935257));
#122670=CARTESIAN_POINT('Ctrl Pts',(-13.4464988064657,83.9517277642667,
71.5003802332486));
#122671=CARTESIAN_POINT('Ctrl Pts',(-13.4330174124397,83.8587193348971,
70.989577291242));
#122672=CARTESIAN_POINT('Ctrl Pts',(-13.4237734591929,83.7694743897222,
70.6267028826339));
#122673=CARTESIAN_POINT('Ctrl Pts',(-13.4107623419622,83.6148428033846,
70.1325839685342));
#122674=CARTESIAN_POINT('Ctrl Pts',(-13.4071042783417,83.5682706710727,
69.9954701646365));
#122675=CARTESIAN_POINT('Ctrl Pts',(-13.3997705438625,83.4697062984198,
69.7269846099298));
#122676=CARTESIAN_POINT('Ctrl Pts',(-13.3960969783972,83.4179375018191,
69.5957494947586));
#122677=CARTESIAN_POINT('Ctrl Pts',(-13.3863600580663,83.2744249480845,
69.2556865489435));
#122678=CARTESIAN_POINT('Ctrl Pts',(-13.3802233403998,83.1777076411274,
69.0489260936027));
#122679=CARTESIAN_POINT('Ctrl Pts',(-13.3642353284874,82.9081485026537,
68.5250273260032));
#122680=CARTESIAN_POINT('Ctrl Pts',(-13.3543039465761,82.7237894033983,
68.2137929137039));
#122681=CARTESIAN_POINT('Ctrl Pts',(-13.3385997299704,82.3996390811858,
67.7335478280627));
#122682=CARTESIAN_POINT('Ctrl Pts',(-13.3327347574751,82.2710304442392,
67.5569360377424));
#122683=CARTESIAN_POINT('Ctrl Pts',(-13.3232860326794,82.0497101593525,
67.2747633743399));
#122684=CARTESIAN_POINT('Ctrl Pts',(-13.3196387460536,81.9605972793141,
67.1663678592388));
#122685=CARTESIAN_POINT('Ctrl Pts',(-13.3098868170892,81.7120551150842,
66.877862131313));
#122686=CARTESIAN_POINT('Ctrl Pts',(-13.303869318848,81.5478733964024,66.7018423740798));
#122687=CARTESIAN_POINT('Ctrl Pts',(-13.2918801304206,81.20810462183,66.3655714889457));
#122688=CARTESIAN_POINT('Ctrl Pts',(-13.2859052916122,81.0326107033414,
66.2050781705628));
#122689=CARTESIAN_POINT('Ctrl Pts',(-13.2758786417514,80.7359781736785,
65.9549353524514));
#122690=CARTESIAN_POINT('Ctrl Pts',(-13.2719337647068,80.6186701800267,
65.8609971690494));
#122691=CARTESIAN_POINT('Ctrl Pts',(-13.2578861871576,80.197661633211,65.5408500301459));
#122692=CARTESIAN_POINT('Ctrl Pts',(-13.2475391732826,79.881765707429,65.3307048056643));
#122693=CARTESIAN_POINT('Ctrl Pts',(-13.2278220192659,79.2566252411988,
64.968591485336));
#122694=CARTESIAN_POINT('Ctrl Pts',(-13.2184503864139,78.9494020070053,
64.8130212923133));
#122695=CARTESIAN_POINT('Ctrl Pts',(-13.2053810712702,78.4985829896546,
64.6157036183555));
#122696=CARTESIAN_POINT('Ctrl Pts',(-13.201486622264,78.3612636850413,64.5595283514857));
#122697=CARTESIAN_POINT('Ctrl Pts',(-13.1912751694299,77.9919679476251,
64.4188457528643));
#122698=CARTESIAN_POINT('Ctrl Pts',(-13.1850745512282,77.75771183689,64.3403094362059));
#122699=CARTESIAN_POINT('Ctrl Pts',(-13.1723425719473,77.2703020673871,
64.1988175121525));
#122700=CARTESIAN_POINT('Ctrl Pts',(-13.1658078920904,77.0167147743859,
64.1369466091538));
#122701=CARTESIAN_POINT('Ctrl Pts',(-13.1551134668004,76.6102158677895,
64.05657975247));
#122702=CARTESIAN_POINT('Ctrl Pts',(-13.1510897667258,76.4589428399496,
64.0307232111347));
#122703=CARTESIAN_POINT('Ctrl Pts',(-13.1366065118578,75.9186504014741,
63.9525508618867));
#122704=CARTESIAN_POINT('Ctrl Pts',(-13.1258877181829,75.5265270032235,
63.9217977227068));
#122705=CARTESIAN_POINT('Ctrl Pts',(-13.1061387660654,74.8021638102403,
63.9116218425384));
#122706=CARTESIAN_POINT('Ctrl Pts',(-13.0971038211258,74.4699675554139,
63.9250115406869));
#122707=CARTESIAN_POINT('Ctrl Pts',(-13.0841859521077,73.9860025382002,
63.9708955159304));
#122708=CARTESIAN_POINT('Ctrl Pts',(-13.0801346581054,73.8328673009898,
63.9893202487664));
#122709=CARTESIAN_POINT('Ctrl Pts',(-13.0698525264644,73.4393650210581,
64.0468018451389));
#122710=CARTESIAN_POINT('Ctrl Pts',(-13.0637306563078,73.1998390097788,
64.0916281188541));
#122711=CARTESIAN_POINT('Ctrl Pts',(-13.0512170732183,72.713993539085,64.2030395987611));
#122712=CARTESIAN_POINT('Ctrl Pts',(-13.0448210725716,72.4677631456297,
64.270579210745));
#122713=CARTESIAN_POINT('Ctrl Pts',(-13.0341661133012,72.074517734885,64.3969280041532));
#122714=CARTESIAN_POINT('Ctrl Pts',(-13.0300303888732,71.9256084093377,
64.4491851464445));
#122715=CARTESIAN_POINT('Ctrl Pts',(-13.0134987819331,71.343000767011,64.6710253275285));
#122716=CARTESIAN_POINT('Ctrl Pts',(-13.0007317281315,70.9207089899708,
64.870532135827));
#122717=CARTESIAN_POINT('Ctrl Pts',(-12.9822116127472,70.3287077799567,
65.2074302125292));
#122718=CARTESIAN_POINT('Ctrl Pts',(-12.9763751415612,70.1451578642584,
65.3206270535002));
#122719=CARTESIAN_POINT('Ctrl Pts',(-12.9659649315537,69.8210882501108,
65.5365946790075));
#122720=CARTESIAN_POINT('Ctrl Pts',(-12.9613645499335,69.6790895582943,
65.6371699567346));
#122721=CARTESIAN_POINT('Ctrl Pts',(-12.9474535762678,69.2517199479968,
65.9585632774538));
#122722=CARTESIAN_POINT('Ctrl Pts',(-12.9384722719713,68.9762093686211,
66.1924796443799));
#122723=CARTESIAN_POINT('Ctrl Pts',(-12.9258413535345,68.614300180949,66.5393319777033));
#122724=CARTESIAN_POINT('Ctrl Pts',(-12.9222826170324,68.5151523215405,
66.638924521861));
#122725=CARTESIAN_POINT('Ctrl Pts',(-12.9146013600048,68.3093468719787,
66.8557053345773));
#122726=CARTESIAN_POINT('Ctrl Pts',(-12.9104646050691,68.2033750057172,
66.9734888532676));
#122727=CARTESIAN_POINT('Ctrl Pts',(-12.8939450494719,67.7977178914268,
67.4490636836859));
#122728=CARTESIAN_POINT('Ctrl Pts',(-12.8811816764342,67.5225170413055,
67.8277526797481));
#122729=CARTESIAN_POINT('Ctrl Pts',(-12.8622355477249,67.1568637793898,
68.4211831175986));
#122730=CARTESIAN_POINT('Ctrl Pts',(-12.8559943911129,67.0434249301038,
68.621833338459));
#122731=CARTESIAN_POINT('Ctrl Pts',(-12.8449569971097,66.8539793764485,
68.9884793111014));
#122732=CARTESIAN_POINT('Ctrl Pts',(-12.8401301655231,66.7750908408301,
69.1530037799877));
#122733=CARTESIAN_POINT('Ctrl Pts',(-12.826085500755,66.5564523644054,69.6463250323456));
#122734=CARTESIAN_POINT('Ctrl Pts',(-12.8171801930435,66.4308640256927,
69.981386793575));
#122735=CARTESIAN_POINT('Ctrl Pts',(-12.8045916096158,66.2838228836075,
70.4584977964471));
#122736=CARTESIAN_POINT('Ctrl Pts',(-12.8009903537789,66.2452030472901,
70.5952639474852));
#122737=CARTESIAN_POINT('Ctrl Pts',(-12.7930893845086,66.1688548682222,
70.89279144699));
#122738=CARTESIAN_POINT('Ctrl Pts',(-12.7887744392789,66.1322896222929,
71.0537958023746));
#122739=CARTESIAN_POINT('Ctrl Pts',(-12.7728051907319,66.014833578395,71.6460170351442));
#122740=CARTESIAN_POINT('Ctrl Pts',(-12.7608427566072,65.9609842654104,
72.0825832165419));
#122741=CARTESIAN_POINT('Ctrl Pts',(-12.7422445472057,65.9260444425325,
72.7663239634917));
#122742=CARTESIAN_POINT('Ctrl Pts',(-12.7355782073821,65.9233786337209,
73.012451328927));
#122743=CARTESIAN_POINT('Ctrl Pts',(-12.7238859406409,65.9362073925439,
73.449313466967));
#122744=CARTESIAN_POINT('Ctrl Pts',(-12.7188252174585,65.9477872686935,
73.6401820146338));
#122745=CARTESIAN_POINT('Ctrl Pts',(-12.7047983993841,65.9972648248628,
74.1766531939995));
#122746=CARTESIAN_POINT('Ctrl Pts',(-12.6961131093045,66.0489467690798,
74.5209729009366));
#122747=CARTESIAN_POINT('Ctrl Pts',(-12.6836459088926,66.1505500222828,
75.0046507446182));
#122748=CARTESIAN_POINT('Ctrl Pts',(-12.6799271639989,66.1842224256447,
75.1474594584057));
#122749=CARTESIAN_POINT('Ctrl Pts',(-12.6717235174104,66.2650516639478,
75.4557902382051));
#122750=CARTESIAN_POINT('Ctrl Pts',(-12.6672247126425,66.3134879406318,
75.6208672876483));
#122751=CARTESIAN_POINT('Ctrl Pts',(-12.6531757084016,66.4774940861465,
76.1257904975992));
#122752=CARTESIAN_POINT('Ctrl Pts',(-12.6434503837016,66.6087951896857,
76.4605145900957));
#122753=CARTESIAN_POINT('Ctrl Pts',(-12.6258030342205,66.88135216578,77.0507839403595));
#122754=CARTESIAN_POINT('Ctrl Pts',(-12.6178868748013,67.0160770530749,
77.3093887965338));
#122755=CARTESIAN_POINT('Ctrl Pts',(-12.6044136729505,67.2691109372457,
77.7433825391018));
#122756=CARTESIAN_POINT('Ctrl Pts',(-12.5988062683593,67.3817507577389,
77.922110938651));
#122757=CARTESIAN_POINT('Ctrl Pts',(-12.5882906799113,67.60825280591,78.2553264648053));
#122758=CARTESIAN_POINT('Ctrl Pts',(-12.5833813940964,67.7210573086567,
78.41053531039));
#122759=CARTESIAN_POINT('Ctrl Pts',(-12.5725479478004,67.9836142033438,
78.7486768244862));
#122760=CARTESIAN_POINT('Ctrl Pts',(-12.5666345801389,68.1358541457552,
78.9296633685733));
#122761=CARTESIAN_POINT('Ctrl Pts',(-12.5560814553162,68.4153494079624,
79.2363296886019));
#122762=CARTESIAN_POINT('Ctrl Pts',(-12.5514812092673,68.5393340464195,
79.36438391965));
#122763=CARTESIAN_POINT('Ctrl Pts',(-12.540188094451,68.8482087290248,79.6649048815689));
#122764=CARTESIAN_POINT('Ctrl Pts',(-12.5334414053335,69.0367483922625,
79.8334355772062));
#122765=CARTESIAN_POINT('Ctrl Pts',(-12.5156481711702,69.5472316402805,
80.2528513826252));
#122766=CARTESIAN_POINT('Ctrl Pts',(-12.5045078689187,69.8799499965225,
80.4906817912754));
#122767=CARTESIAN_POINT('Ctrl Pts',(-12.4883226190392,70.3911116671256,
80.8069128989764));
#122768=CARTESIAN_POINT('Ctrl Pts',(-12.4831582287761,70.558496888027,80.9033038675062));
#122769=CARTESIAN_POINT('Ctrl Pts',(-12.4734907321598,70.8813099343359,
81.0758447716644));
#122770=CARTESIAN_POINT('Ctrl Pts',(-12.4689745525381,71.0361780777578,
81.1530610916338));
#122771=CARTESIAN_POINT('Ctrl Pts',(-12.4570631524985,71.4569675669917,
81.3480902085793));
#122772=CARTESIAN_POINT('Ctrl Pts',(-12.4497988475183,71.7266747493541,
81.4577271304391));
#122773=CARTESIAN_POINT('Ctrl Pts',(-12.4383211700839,72.1541234716692,
81.60765414121));
#122774=CARTESIAN_POINT('Ctrl Pts',(-12.4341804007932,72.3083041762663,
81.6570566756748));
#122775=CARTESIAN_POINT('Ctrl Pts',(-12.4244611698138,72.6675205969803,
81.7614196825632));
#122776=CARTESIAN_POINT('Ctrl Pts',(-12.4188637003036,72.8730226382521,
81.813274778027));
#122777=CARTESIAN_POINT('Ctrl Pts',(-12.4004787803361,73.5462611627678,
81.9582469171631));
#122778=CARTESIAN_POINT('Ctrl Pts',(-12.3874564595957,74.0203970767149,
82.021810566711));
#122779=CARTESIAN_POINT('Ctrl Pts',(-12.3671300994806,74.7733760226478,
82.0636494785414));
#122780=CARTESIAN_POINT('Ctrl Pts',(-12.3597133925574,75.0509543705473,
82.0664880196756));
#122781=CARTESIAN_POINT('Ctrl Pts',(-12.3476615880533,75.5102965307628,
82.0502835522977));
#122782=CARTESIAN_POINT('Ctrl Pts',(-12.342950076167,75.6923285086733,82.038400729389));
#122783=CARTESIAN_POINT('Ctrl Pts',(-12.3306517123437,76.1731961781591,
81.9924120218353));
#122784=CARTESIAN_POINT('Ctrl Pts',(-12.3231452386327,76.4711123378138,
81.9488889682233));
#122785=CARTESIAN_POINT('Ctrl Pts',(-12.3106304952259,76.9502484100407,
81.8538526155916));
#122786=CARTESIAN_POINT('Ctrl Pts',(-12.305741722965,77.1331624934673,81.8114969195186));
#122787=CARTESIAN_POINT('Ctrl Pts',(-12.2925180068898,77.6181233127046,
81.6831070298117));
#122788=CARTESIAN_POINT('Ctrl Pts',(-12.284077113479,77.9175165446415,81.5868332732924));
#122789=CARTESIAN_POINT('Ctrl Pts',(-12.2660745886364,78.5407379361755,
81.3503819297233));
#122790=CARTESIAN_POINT('Ctrl Pts',(-12.2565020320278,78.8631153856673,
81.2062563850034));
#122791=CARTESIAN_POINT('Ctrl Pts',(-12.2405850593187,79.3905705659937,
80.9330114673131));
#122792=CARTESIAN_POINT('Ctrl Pts',(-12.2341725776039,79.6006501278721,
80.813440125623));
#122793=CARTESIAN_POINT('Ctrl Pts',(-12.2216027796096,80.0097752838398,
80.5585650532214));
#122794=CARTESIAN_POINT('Ctrl Pts',(-12.2154774447836,80.2088643721971,
80.4233312735564));
#122795=CARTESIAN_POINT('Ctrl Pts',(-12.2046453730353,80.5532762949083,
80.1686665260884));
#122796=CARTESIAN_POINT('Ctrl Pts',(-12.1999090131954,80.7008184544443,
80.0522638025176));
#122797=CARTESIAN_POINT('Ctrl Pts',(-12.1901006111542,80.9939699950065,
79.8055145925463));
#122798=CARTESIAN_POINT('Ctrl Pts',(-12.1850200616843,81.1391421901178,
79.6748897334218));
#122799=CARTESIAN_POINT('Ctrl Pts',(-12.1711816510871,81.5180700576123,
79.3109742306788));
#122800=CARTESIAN_POINT('Ctrl Pts',(-12.1623088331986,81.7436892761096,
79.0690816217196));
#122801=CARTESIAN_POINT('Ctrl Pts',(-12.1438682207081,82.1821064845516,
78.5448370469674));
#122802=CARTESIAN_POINT('Ctrl Pts',(-12.1342946016636,82.3929714160391,
78.2608055499923));
#122803=CARTESIAN_POINT('Ctrl Pts',(-12.1182745618553,82.7215936081313,
77.7602519075173));
#122804=CARTESIAN_POINT('Ctrl Pts',(-12.1117624548681,82.8481742610244,
77.5494630099774));
#122805=CARTESIAN_POINT('Ctrl Pts',(-12.0978616409741,83.1042913307437,
77.0810631266478));
#122806=CARTESIAN_POINT('Ctrl Pts',(-12.0905739617319,83.230546547132,76.8216673697312));
#122807=CARTESIAN_POINT('Ctrl Pts',(-12.0787437540253,83.4145321503588,
76.3922532317014));
#122808=CARTESIAN_POINT('Ctrl Pts',(-12.0741938022211,83.4800754356876,
76.2256666843821));
#122809=CARTESIAN_POINT('Ctrl Pts',(-12.0638001481673,83.6158637370845,
75.8472566058139));
#122810=CARTESIAN_POINT('Ctrl Pts',(-12.0579463729973,83.6832187490197,
75.6348454886013));
#122811=CARTESIAN_POINT('Ctrl Pts',(-12.0385091783984,83.8785318879706,
74.9295902101342));
#122812=CARTESIAN_POINT('Ctrl Pts',(-12.0246654647559,83.9730142509582,
74.427433964592));
#122813=CARTESIAN_POINT('Ctrl Pts',(-12.0026284815655,84.0572939236343,
73.6119406926));
#122814=CARTESIAN_POINT('Ctrl Pts',(-11.9943351321064,84.073543915764,73.3012121215505));
#122815=CARTESIAN_POINT('Ctrl Pts',(-11.9773935617203,84.0743111601728,
72.6535079496331));
#122816=CARTESIAN_POINT('Ctrl Pts',(-11.9688665158948,84.0560336237962,
72.3165311780078));
#122817=CARTESIAN_POINT('Ctrl Pts',(-11.9541824810339,83.9921630770108,
71.7415416566964));
#122818=CARTESIAN_POINT('Ctrl Pts',(-11.9480006684834,83.9558518769487,
71.5034271347825));
#122819=CARTESIAN_POINT('Ctrl Pts',(-11.925413164715,83.7913448027552,70.6559352350277));
#122820=CARTESIAN_POINT('Ctrl Pts',(-11.9085088968384,83.6093139072469,
70.0575986845659));
#122821=CARTESIAN_POINT('Ctrl Pts',(-11.8826053899707,83.2370411383783,
69.16872447229));
#122822=CARTESIAN_POINT('Ctrl Pts',(-11.8734787558732,83.0874641788945,
68.8609537687649));
#122823=CARTESIAN_POINT('Ctrl Pts',(-11.8566200690561,82.7736384453366,
68.2979888438898));
#122824=CARTESIAN_POINT('Ctrl Pts',(-11.8489105905299,82.6129745364498,
68.0407856392821));
#122825=CARTESIAN_POINT('Ctrl Pts',(-11.8361173800603,82.3247164839222,
67.6274886742986));
#122826=CARTESIAN_POINT('Ctrl Pts',(-11.8309988914646,82.2044001390743,
67.4668056975292));
#122827=CARTESIAN_POINT('Ctrl Pts',(-11.8186884328572,81.9073280157545,
67.0969139690612));
#122828=CARTESIAN_POINT('Ctrl Pts',(-11.8114726770941,81.7265066892708,
66.8917785636207));
#122829=CARTESIAN_POINT('Ctrl Pts',(-11.7909036071631,81.1907842154379,
66.3365812720506));
#122830=CARTESIAN_POINT('Ctrl Pts',(-11.7773919869305,80.8152025653093,
66.0063841928442));
#122831=CARTESIAN_POINT('Ctrl Pts',(-11.7577359137786,80.2259325654831,
65.5677402313798));
#122832=CARTESIAN_POINT('Ctrl Pts',(-11.7514533924048,80.0309507826131,
65.4339767474056));
#122833=CARTESIAN_POINT('Ctrl Pts',(-11.7391261110203,79.6336498983422,
65.1835295377725));
#122834=CARTESIAN_POINT('Ctrl Pts',(-11.7330919905038,79.4314422155539,
65.0666522017275));
#122835=CARTESIAN_POINT('Ctrl Pts',(-11.7218739022591,79.0422033436105,
64.8613980133367));
#122836=CARTESIAN_POINT('Ctrl Pts',(-11.7166481683376,78.8560991917015,
64.7712967384883));
#122837=CARTESIAN_POINT('Ctrl Pts',(-11.7051089646206,78.4448254719931,
64.5896135664457));
#122838=CARTESIAN_POINT('Ctrl Pts',(-11.6987660691994,78.2185704367478,
64.50056777215));
#122839=CARTESIAN_POINT('Ctrl Pts',(-11.6848137035157,77.7193217761979,
64.3269818650027));
#122840=CARTESIAN_POINT('Ctrl Pts',(-11.6771777832053,77.4451071848254,
64.2459806907456));
#122841=CARTESIAN_POINT('Ctrl Pts',(-11.652910886625,76.5668494001514,64.0306567087294));
#122842=CARTESIAN_POINT('Ctrl Pts',(-11.6361730259508,75.9508490052193,
63.9442499692642));
#122843=CARTESIAN_POINT('Ctrl Pts',(-11.6138730333825,75.09755207763,63.912029666633));
#122844=CARTESIAN_POINT('Ctrl Pts',(-11.6078376954894,74.8621502508335,
63.912269520108));
#122845=CARTESIAN_POINT('Ctrl Pts',(-11.5935401925601,74.3012374350425,
63.9348905061263));
#122846=CARTESIAN_POINT('Ctrl Pts',(-11.5852322787154,73.9777561566445,
63.9657478053854));
#122847=CARTESIAN_POINT('Ctrl Pts',(-11.564688317689,73.2028988620542,64.0825377978221));
#122848=CARTESIAN_POINT('Ctrl Pts',(-11.5524127609735,72.7554314771851,
64.1853200226825));
#122849=CARTESIAN_POINT('Ctrl Pts',(-11.5268898277826,71.8470843832727,
64.4668238657377));
#122850=CARTESIAN_POINT('Ctrl Pts',(-11.5136411107232,71.387687790774,64.6508499734686));
#122851=CARTESIAN_POINT('Ctrl Pts',(-11.4937288130588,70.707457635515,64.9896193704598));
#122852=CARTESIAN_POINT('Ctrl Pts',(-11.4868639886907,70.473924993594,65.1190168069731));
#122853=CARTESIAN_POINT('Ctrl Pts',(-11.4716617689557,69.9660535818595,
65.4307895649784));
#122854=CARTESIAN_POINT('Ctrl Pts',(-11.4632483507889,69.6964232405937,
65.6176345534709));
#122855=CARTESIAN_POINT('Ctrl Pts',(-11.4470220115368,69.208284502858,65.9971295944645));
#122856=CARTESIAN_POINT('Ctrl Pts',(-11.43931922007,68.9881340287137,66.1859898710082));
#122857=CARTESIAN_POINT('Ctrl Pts',(-11.4120216262576,68.2452570433496,
66.8872342308817));
#122858=CARTESIAN_POINT('Ctrl Pts',(-11.3922149334269,67.7732110023256,
67.4537567647632));
#122859=CARTESIAN_POINT('Ctrl Pts',(-11.3669456680991,67.2454304508019,
68.2695544984007));
#122860=CARTESIAN_POINT('Ctrl Pts',(-11.3608242996976,67.123178986526,68.4760297071188));
#122861=CARTESIAN_POINT('Ctrl Pts',(-11.3475630061663,66.8771307302081,
68.9325669324535));
#122862=CARTESIAN_POINT('Ctrl Pts',(-11.3403681640615,66.7568349349563,
69.1834264553651));
#122863=CARTESIAN_POINT('Ctrl Pts',(-11.3248199603447,66.5257007577464,
69.7287292610446));
#122864=CARTESIAN_POINT('Ctrl Pts',(-11.3164608927144,66.4181790243786,
70.0245316235007));
#122865=CARTESIAN_POINT('Ctrl Pts',(-11.2895635086448,66.1233415939836,
70.9874007142824));
#122866=CARTESIAN_POINT('Ctrl Pts',(-11.2708832047889,65.9956993337317,
71.6730255604155));
#122867=CARTESIAN_POINT('Ctrl Pts',(-11.2459423296123,65.9287622245236,
72.6274682344808));
#122868=CARTESIAN_POINT('Ctrl Pts',(-11.2391899128312,65.9217943497886,
72.8916999445158));
#122869=CARTESIAN_POINT('Ctrl Pts',(-11.2247967392948,65.9319287012176,
73.4531286084572));
#122870=CARTESIAN_POINT('Ctrl Pts',(-11.2170835341397,65.9522349747787,
73.7494401143278));
#122871=CARTESIAN_POINT('Ctrl Pts',(-11.1997593434101,66.0294539077494,
74.4032547996756));
#122872=CARTESIAN_POINT('Ctrl Pts',(-11.1901116721686,66.0935069748745,
74.7601509818632));
#122873=CARTESIAN_POINT('Ctrl Pts',(-11.1636740994005,66.3256054618999,
75.7221353348087));
#122874=CARTESIAN_POINT('Ctrl Pts',(-11.1468391668825,66.5355387126056,
76.3173479064166));
#122875=CARTESIAN_POINT('Ctrl Pts',(-11.1230855295391,66.9259140697659,
77.1409425112817));
#122876=CARTESIAN_POINT('Ctrl Pts',(-11.1158407152713,67.0594948847545,
77.3916337481368));
#122877=CARTESIAN_POINT('Ctrl Pts',(-11.0991516044814,67.3913951984904,
77.948534407531));
#122878=CARTESIAN_POINT('Ctrl Pts',(-11.0896004548305,67.5971897626805,
78.2499532894295));
#122879=CARTESIAN_POINT('Ctrl Pts',(-11.066606918913,68.1292644930105,78.936850578795));
#122880=CARTESIAN_POINT('Ctrl Pts',(-11.053077156272,68.4716321676164,79.3101735682659));
#122881=CARTESIAN_POINT('Ctrl Pts',(-11.0284125191687,69.1515329753655,
79.9388802838722));
#122882=CARTESIAN_POINT('Ctrl Pts',(-11.0172503581122,69.4806030071237,
80.2036409696054));
#122883=CARTESIAN_POINT('Ctrl Pts',(-10.9985390390634,70.0712279150404,
80.614415278307));
#122884=CARTESIAN_POINT('Ctrl Pts',(-10.9909334047949,70.3245754877019,
80.7726454831127));
#122885=CARTESIAN_POINT('Ctrl Pts',(-10.9697548269484,71.0388286659262,
81.1699412959377));
#122886=CARTESIAN_POINT('Ctrl Pts',(-10.9560294121159,71.5135704359081,
81.3823050592927));
#122887=CARTESIAN_POINT('Ctrl Pts',(-10.9223429476978,72.708313125711,81.7995014839169));
#122888=CARTESIAN_POINT('Ctrl Pts',(-10.9023122329795,73.4443011087522,
81.9596064222288));
#122889=CARTESIAN_POINT('Ctrl Pts',(-10.8751584514562,74.4848368720807,
82.0540579166407));
#122890=CARTESIAN_POINT('Ctrl Pts',(-10.8675576584132,74.7822601659039,
82.0662707454521));
#122891=CARTESIAN_POINT('Ctrl Pts',(-10.8434722464501,75.7084594847752,
82.0575451759476));
#122892=CARTESIAN_POINT('Ctrl Pts',(-10.8267691213327,76.3355363323114,
81.9854855858357));
#122893=CARTESIAN_POINT('Ctrl Pts',(-10.7944474624907,77.5216341862379,
81.7244250653333));
#122894=CARTESIAN_POINT('Ctrl Pts',(-10.7788310631899,78.0826746872989,
81.5433290772843));
#122895=CARTESIAN_POINT('Ctrl Pts',(-10.7546809646044,78.9322314538102,
81.1746669638441));
#122896=CARTESIAN_POINT('Ctrl Pts',(-10.7459964850638,79.2354841414371,
81.0222032664891));
#122897=CARTESIAN_POINT('Ctrl Pts',(-10.7256878866019,79.9103259574314,
80.6328063119621));
#122898=CARTESIAN_POINT('Ctrl Pts',(-10.7140980827418,80.2741212462702,
80.3856733475756));
#122899=CARTESIAN_POINT('Ctrl Pts',(-10.6871684528069,81.0706736659949,
79.7565830065856));
#122900=CARTESIAN_POINT('Ctrl Pts',(-10.6717915993553,81.4893718767674,
79.3565348007192));
#122901=CARTESIAN_POINT('Ctrl Pts',(-10.640519778576,82.2659768611267,78.4594683542636));
#122902=CARTESIAN_POINT('Ctrl Pts',(-10.6249072747157,82.6176903657794,
77.9595190933445));
#122903=CARTESIAN_POINT('Ctrl Pts',(-10.5939779030133,83.1934066138114,
76.9294721098776));
#122904=CARTESIAN_POINT('Ctrl Pts',(-10.5789318808566,83.4231942328531,
76.4088603817057));
#122905=CARTESIAN_POINT('Ctrl Pts',(-10.5481810648341,83.7914428882741,
75.3100152504172));
#122906=CARTESIAN_POINT('Ctrl Pts',(-10.5324760203067,83.9253402123738,
74.7299845962427));
#122907=CARTESIAN_POINT('Ctrl Pts',(-10.506040976142,84.0550494842427,73.7246815616173));
#122908=CARTESIAN_POINT('Ctrl Pts',(-10.4952140429273,84.0791260026975,
73.3057698135278));
#122909=CARTESIAN_POINT('Ctrl Pts',(-10.4652701513313,84.0649528968915,
72.1657159863188));
#122910=CARTESIAN_POINT('Ctrl Pts',(-10.4461089964124,83.9699778210984,
71.4466320716153));
#122911=CARTESIAN_POINT('Ctrl Pts',(-10.3954812582148,83.4987543731218,
69.5913065933387));
#122912=CARTESIAN_POINT('Ctrl Pts',(-10.3651611426005,82.9832088330785,
68.5139509363784));
#122913=CARTESIAN_POINT('Ctrl Pts',(-10.3180635153095,81.9168420926899,
67.0873853839914));
#122914=CARTESIAN_POINT('Ctrl Pts',(-10.3024236418362,81.5179256481026,
66.6488212164598));
#122915=CARTESIAN_POINT('Ctrl Pts',(-10.26313876224,80.410269540294,65.6467307993475));
#122916=CARTESIAN_POINT('Ctrl Pts',(-10.2399332767544,79.6574681785045,
65.1498522254083));
#122917=CARTESIAN_POINT('Ctrl Pts',(-10.2006644622652,78.3096069450724,
64.5202404529412));
#122918=CARTESIAN_POINT('Ctrl Pts',(-10.1850172306535,77.749637921637,64.321816495378));
#122919=CARTESIAN_POINT('Ctrl Pts',(-10.1540168337345,76.6070822003054,
64.0382750241231));
#122920=CARTESIAN_POINT('Ctrl Pts',(-10.1388244678694,76.0279702794316,
63.9529979491404));
#122921=CARTESIAN_POINT('Ctrl Pts',(-10.0928504785718,74.2792924799251,
63.869769992767));
#122922=CARTESIAN_POINT('Ctrl Pts',(-10.0620175451159,73.1064692951876,
64.0387582366355));
#122923=CARTESIAN_POINT('Ctrl Pts',(-10.0163541915642,71.4644504576041,
64.610815205128));
#122924=CARTESIAN_POINT('Ctrl Pts',(-10.0013527294429,70.9424093499569,
64.8520339579409));
#122925=CARTESIAN_POINT('Ctrl Pts',(-9.96434722807135,69.7262383344997,
65.5590017814957));
#122926=CARTESIAN_POINT('Ctrl Pts',(-9.94233034594927,69.0618814918381,
66.0776427426821));
#122927=CARTESIAN_POINT('Ctrl Pts',(-9.89823651844638,67.8956325647864,
67.2795378045371));
#122928=CARTESIAN_POINT('Ctrl Pts',(-9.87641089052029,67.4023950609479,
67.9580324679594));
#122929=CARTESIAN_POINT('Ctrl Pts',(-9.85451302005563,67.0084395094767,
68.6917839432004));
#122930=CARTESIAN_POINT('Ctrl Pts',(-13.6367975371279,82.22637258748,78.478439844214));
#122931=CARTESIAN_POINT('Ctrl Pts',(-13.5965727996549,83.15132333764,77.260846746689));
#122932=CARTESIAN_POINT('Ctrl Pts',(-13.5161233247074,84.37134578258,74.349656820311));
#122933=CARTESIAN_POINT('Ctrl Pts',(-13.3954491122865,83.85839097116,69.641309155131));
#122934=CARTESIAN_POINT('Ctrl Pts',(-13.2747748998656,81.12957508313,65.770566029046));
#122935=CARTESIAN_POINT('Ctrl Pts',(-13.1541006874447,76.867728622,63.705144460549));
#122936=CARTESIAN_POINT('Ctrl Pts',(-13.0334264750238,72.13871802361,63.961747337343));
#122937=CARTESIAN_POINT('Ctrl Pts',(-12.9127522626029,68.12536086466,66.476164874831));
#122938=CARTESIAN_POINT('Ctrl Pts',(-12.7920780501819,65.83145073401,70.619512225841));
#122939=CARTESIAN_POINT('Ctrl Pts',(-12.6714038377609,65.83072989138,75.355475184308));
#122940=CARTESIAN_POINT('Ctrl Pts',(-12.5507296253399,68.12337819702,79.499520367104));
#122941=CARTESIAN_POINT('Ctrl Pts',(-12.4300554129189,72.13597072448,82.015161004986));
#122942=CARTESIAN_POINT('Ctrl Pts',(-12.3093812004979,76.86489906758,82.273198436157));
#122943=CARTESIAN_POINT('Ctrl Pts',(-12.1887069880768,81.12738874216,80.209093695038));
#122944=CARTESIAN_POINT('Ctrl Pts',(-12.0680327756558,83.857328421,76.339109722068));
#122945=CARTESIAN_POINT('Ctrl Pts',(-11.9473585632348,84.37192006169,71.631186395751));
#122946=CARTESIAN_POINT('Ctrl Pts',(-11.8266843508137,82.5424567304,67.262844545329));
#122947=CARTESIAN_POINT('Ctrl Pts',(-11.7060101383927,78.82651409889,64.326670680902));
#122948=CARTESIAN_POINT('Ctrl Pts',(-11.5853359259716,74.15350404259,63.557045046897));
#122949=CARTESIAN_POINT('Ctrl Pts',(-11.4646617135509,69.69221506849,65.146462327629));
#122950=CARTESIAN_POINT('Ctrl Pts',(-11.3439875011299,66.55848112866,68.697385897282));
#122951=CARTESIAN_POINT('Ctrl Pts',(-11.2233132887089,65.53609514649,73.3216775732696));
#122952=CARTESIAN_POINT('Ctrl Pts',(-11.1026390762869,66.88077088472,77.862734032643));
#122953=CARTESIAN_POINT('Ctrl Pts',(-10.9819648638659,70.25618517554,81.184770299059));
#122954=CARTESIAN_POINT('Ctrl Pts',(-10.8612906514449,74.81809728471,82.456896282854));
#122955=CARTESIAN_POINT('Ctrl Pts',(-10.7406164390239,79.42550594423,81.360934525046));
#122956=CARTESIAN_POINT('Ctrl Pts',(-10.6199422266029,82.92603048601,78.171001360235));
#122957=CARTESIAN_POINT('Ctrl Pts',(-10.4992680141819,84.44413839523,73.6849452599872));
#122958=CARTESIAN_POINT('Ctrl Pts',(-10.3785938017609,83.60012808368,69.02479742627));
#122959=CARTESIAN_POINT('Ctrl Pts',(-10.2579195893399,80.60510074462,65.356119528941));
#122960=CARTESIAN_POINT('Ctrl Pts',(-10.1372453769189,76.20814999546,63.596538435828));
#122961=CARTESIAN_POINT('Ctrl Pts',(-10.0165711644989,71.50904302936,64.186014661069));
#122962=CARTESIAN_POINT('Ctrl Pts',(-9.89589695207791,67.68300161261,66.977621268753));
#122963=CARTESIAN_POINT('Ctrl Pts',(-9.81544747712991,66.35255094703,69.840029796558));
#122964=CARTESIAN_POINT('Ctrl Pts',(-9.77522273965691,66.0753597154,71.343769089941));
#122965=CARTESIAN_POINT('Ctrl Pts',(-13.7234642037949,82.22637258748,78.478439844214));
#122966=CARTESIAN_POINT('Ctrl Pts',(-13.6832394663209,83.15132333764,77.260846746689));
#122967=CARTESIAN_POINT('Ctrl Pts',(-13.6027899913739,84.37134578258,74.349656820311));
#122968=CARTESIAN_POINT('Ctrl Pts',(-13.4821157789532,83.85839097116,69.641309155131));
#122969=CARTESIAN_POINT('Ctrl Pts',(-13.3614415665323,81.12957508313,65.770566029046));
#122970=CARTESIAN_POINT('Ctrl Pts',(-13.2407673541114,76.867728622,63.705144460549));
#122971=CARTESIAN_POINT('Ctrl Pts',(-13.1200931416905,72.13871802361,63.961747337343));
#122972=CARTESIAN_POINT('Ctrl Pts',(-12.9994189292695,68.12536086466,66.476164874831));
#122973=CARTESIAN_POINT('Ctrl Pts',(-12.8787447168486,65.83145073401,70.619512225841));
#122974=CARTESIAN_POINT('Ctrl Pts',(-12.7580705044276,65.83072989138,75.355475184308));
#122975=CARTESIAN_POINT('Ctrl Pts',(-12.6373962920066,68.12337819702,79.499520367104));
#122976=CARTESIAN_POINT('Ctrl Pts',(-12.5167220795856,72.13597072448,82.015161004986));
#122977=CARTESIAN_POINT('Ctrl Pts',(-12.3960478671645,76.86489906758,82.273198436157));
#122978=CARTESIAN_POINT('Ctrl Pts',(-12.2753736547435,81.12738874216,80.209093695038));
#122979=CARTESIAN_POINT('Ctrl Pts',(-12.1546994423225,83.857328421,76.339109722068));
#122980=CARTESIAN_POINT('Ctrl Pts',(-12.0340252299014,84.37192006169,71.631186395751));
#122981=CARTESIAN_POINT('Ctrl Pts',(-11.9133510174804,82.5424567304,67.262844545329));
#122982=CARTESIAN_POINT('Ctrl Pts',(-11.7926768050593,78.82651409889,64.326670680902));
#122983=CARTESIAN_POINT('Ctrl Pts',(-11.6720025926383,74.15350404259,63.557045046897));
#122984=CARTESIAN_POINT('Ctrl Pts',(-11.5513283802169,69.69221506849,65.146462327629));
#122985=CARTESIAN_POINT('Ctrl Pts',(-11.4306541677959,66.55848112866,68.697385897282));
#122986=CARTESIAN_POINT('Ctrl Pts',(-11.3099799553749,65.53609514649,73.3216775732696));
#122987=CARTESIAN_POINT('Ctrl Pts',(-11.1893057429539,66.88077088472,77.862734032643));
#122988=CARTESIAN_POINT('Ctrl Pts',(-11.0686315305329,70.25618517554,81.184770299059));
#122989=CARTESIAN_POINT('Ctrl Pts',(-10.9479573181119,74.81809728471,82.456896282854));
#122990=CARTESIAN_POINT('Ctrl Pts',(-10.8272831056909,79.42550594423,81.360934525046));
#122991=CARTESIAN_POINT('Ctrl Pts',(-10.7066088932699,82.92603048601,78.171001360235));
#122992=CARTESIAN_POINT('Ctrl Pts',(-10.5859346808489,84.44413839523,73.6849452599872));
#122993=CARTESIAN_POINT('Ctrl Pts',(-10.4652604684279,83.60012808368,69.02479742627));
#122994=CARTESIAN_POINT('Ctrl Pts',(-10.3445862560069,80.60510074462,65.356119528941));
#122995=CARTESIAN_POINT('Ctrl Pts',(-10.2239120435859,76.20814999546,63.596538435828));
#122996=CARTESIAN_POINT('Ctrl Pts',(-10.1032378311649,71.50904302936,64.186014661069));
#122997=CARTESIAN_POINT('Ctrl Pts',(-9.98256361874391,67.68300161261,66.977621268753));
#122998=CARTESIAN_POINT('Ctrl Pts',(-9.90211414379691,66.35255094703,69.840029796558));
#122999=CARTESIAN_POINT('Ctrl Pts',(-9.86188940632291,66.0753597154,71.343769089941));
#123000=CARTESIAN_POINT('Ctrl Pts',(-13.8101308704619,82.22637258748,78.478439844214));
#123001=CARTESIAN_POINT('Ctrl Pts',(-13.7699061329879,83.15132333764,77.260846746689));
#123002=CARTESIAN_POINT('Ctrl Pts',(-13.6894566580409,84.37134578258,74.349656820311));
#123003=CARTESIAN_POINT('Ctrl Pts',(-13.5687824456199,83.85839097116,69.641309155131));
#123004=CARTESIAN_POINT('Ctrl Pts',(-13.448108233199,81.12957508313,65.770566029046));
#123005=CARTESIAN_POINT('Ctrl Pts',(-13.3274340207781,76.867728622,63.705144460549));
#123006=CARTESIAN_POINT('Ctrl Pts',(-13.2067598083571,72.13871802361,63.961747337343));
#123007=CARTESIAN_POINT('Ctrl Pts',(-13.0860855959362,68.12536086466,66.476164874831));
#123008=CARTESIAN_POINT('Ctrl Pts',(-12.9654113835152,65.83145073401,70.619512225841));
#123009=CARTESIAN_POINT('Ctrl Pts',(-12.8447371710942,65.83072989138,75.355475184308));
#123010=CARTESIAN_POINT('Ctrl Pts',(-12.7240629586732,68.12337819702,79.499520367104));
#123011=CARTESIAN_POINT('Ctrl Pts',(-12.6033887462522,72.13597072448,82.015161004986));
#123012=CARTESIAN_POINT('Ctrl Pts',(-12.4827145338312,76.86489906758,82.273198436157));
#123013=CARTESIAN_POINT('Ctrl Pts',(-12.3620403214102,81.12738874216,80.209093695038));
#123014=CARTESIAN_POINT('Ctrl Pts',(-12.2413661089891,83.857328421,76.339109722068));
#123015=CARTESIAN_POINT('Ctrl Pts',(-12.1206918965681,84.37192006169,71.631186395751));
#123016=CARTESIAN_POINT('Ctrl Pts',(-12.000017684147,82.5424567304,67.262844545329));
#123017=CARTESIAN_POINT('Ctrl Pts',(-11.879343471726,78.82651409889,64.326670680902));
#123018=CARTESIAN_POINT('Ctrl Pts',(-11.7586692593049,74.15350404259,63.557045046897));
#123019=CARTESIAN_POINT('Ctrl Pts',(-11.6379950468839,69.69221506849,65.146462327629));
#123020=CARTESIAN_POINT('Ctrl Pts',(-11.5173208344629,66.55848112866,68.697385897282));
#123021=CARTESIAN_POINT('Ctrl Pts',(-11.3966466220419,65.53609514649,73.3216775732696));
#123022=CARTESIAN_POINT('Ctrl Pts',(-11.2759724096209,66.88077088472,77.862734032643));
#123023=CARTESIAN_POINT('Ctrl Pts',(-11.1552981971999,70.25618517554,81.184770299059));
#123024=CARTESIAN_POINT('Ctrl Pts',(-11.0346239847789,74.81809728471,82.456896282854));
#123025=CARTESIAN_POINT('Ctrl Pts',(-10.9139497723579,79.42550594423,81.360934525046));
#123026=CARTESIAN_POINT('Ctrl Pts',(-10.7932755599369,82.92603048601,78.171001360235));
#123027=CARTESIAN_POINT('Ctrl Pts',(-10.6726013475159,84.44413839523,73.6849452599872));
#123028=CARTESIAN_POINT('Ctrl Pts',(-10.5519271350949,83.60012808368,69.02479742627));
#123029=CARTESIAN_POINT('Ctrl Pts',(-10.4312529226739,80.60510074462,65.356119528941));
#123030=CARTESIAN_POINT('Ctrl Pts',(-10.3105787102529,76.20814999546,63.596538435828));
#123031=CARTESIAN_POINT('Ctrl Pts',(-10.1899044978319,71.50904302936,64.186014661069));
#123032=CARTESIAN_POINT('Ctrl Pts',(-10.0692302854109,67.68300161261,66.977621268753));
#123033=CARTESIAN_POINT('Ctrl Pts',(-9.98878081046391,66.35255094703,69.840029796558));
#123034=CARTESIAN_POINT('Ctrl Pts',(-9.94855607298991,66.0753597154,71.343769089941));
#123035=CARTESIAN_POINT('Ctrl Pts',(-13.8967975371279,82.22637258748,78.478439844214));
#123036=CARTESIAN_POINT('Ctrl Pts',(-13.8565727996549,83.15132333764,77.260846746689));
#123037=CARTESIAN_POINT('Ctrl Pts',(-13.7761233247069,84.37134578258,74.349656820311));
#123038=CARTESIAN_POINT('Ctrl Pts',(-13.6554491122869,83.85839097116,69.641309155131));
#123039=CARTESIAN_POINT('Ctrl Pts',(-13.5347748998656,81.12957508313,65.770566029046));
#123040=CARTESIAN_POINT('Ctrl Pts',(-13.4141006874447,76.867728622,63.705144460549));
#123041=CARTESIAN_POINT('Ctrl Pts',(-13.2934264750238,72.13871802361,63.961747337343));
#123042=CARTESIAN_POINT('Ctrl Pts',(-13.1727522626029,68.12536086466,66.476164874831));
#123043=CARTESIAN_POINT('Ctrl Pts',(-13.0520780501819,65.83145073401,70.619512225841));
#123044=CARTESIAN_POINT('Ctrl Pts',(-12.9314038377609,65.83072989138,75.355475184308));
#123045=CARTESIAN_POINT('Ctrl Pts',(-12.8107296253399,68.12337819702,79.499520367104));
#123046=CARTESIAN_POINT('Ctrl Pts',(-12.6900554129189,72.13597072448,82.015161004986));
#123047=CARTESIAN_POINT('Ctrl Pts',(-12.5693812004979,76.86489906758,82.273198436157));
#123048=CARTESIAN_POINT('Ctrl Pts',(-12.4487069880768,81.12738874216,80.209093695038));
#123049=CARTESIAN_POINT('Ctrl Pts',(-12.3280327756558,83.857328421,76.339109722068));
#123050=CARTESIAN_POINT('Ctrl Pts',(-12.2073585632348,84.37192006169,71.631186395751));
#123051=CARTESIAN_POINT('Ctrl Pts',(-12.0866843508137,82.5424567304,67.262844545329));
#123052=CARTESIAN_POINT('Ctrl Pts',(-11.9660101383927,78.82651409889,64.326670680902));
#123053=CARTESIAN_POINT('Ctrl Pts',(-11.8453359259716,74.15350404259,63.557045046897));
#123054=CARTESIAN_POINT('Ctrl Pts',(-11.7246617135505,69.69221506849,65.146462327629));
#123055=CARTESIAN_POINT('Ctrl Pts',(-11.6039875011295,66.55848112866,68.697385897282));
#123056=CARTESIAN_POINT('Ctrl Pts',(-11.4833132887089,65.53609514649,73.3216775732696));
#123057=CARTESIAN_POINT('Ctrl Pts',(-11.3626390762869,66.88077088472,77.862734032643));
#123058=CARTESIAN_POINT('Ctrl Pts',(-11.2419648638659,70.25618517554,81.184770299059));
#123059=CARTESIAN_POINT('Ctrl Pts',(-11.1212906514449,74.81809728471,82.456896282854));
#123060=CARTESIAN_POINT('Ctrl Pts',(-11.0006164390239,79.42550594423,81.360934525046));
#123061=CARTESIAN_POINT('Ctrl Pts',(-10.8799422266029,82.92603048601,78.171001360235));
#123062=CARTESIAN_POINT('Ctrl Pts',(-10.7592680141819,84.44413839523,73.6849452599872));
#123063=CARTESIAN_POINT('Ctrl Pts',(-10.6385938017609,83.60012808368,69.02479742627));
#123064=CARTESIAN_POINT('Ctrl Pts',(-10.5179195893399,80.60510074462,65.356119528941));
#123065=CARTESIAN_POINT('Ctrl Pts',(-10.3972453769189,76.20814999546,63.596538435828));
#123066=CARTESIAN_POINT('Ctrl Pts',(-10.2765711644989,71.50904302936,64.186014661069));
#123067=CARTESIAN_POINT('Ctrl Pts',(-10.1558969520779,67.68300161261,66.977621268753));
#123068=CARTESIAN_POINT('Ctrl Pts',(-10.0754474771299,66.35255094703,69.840029796558));
#123069=CARTESIAN_POINT('Ctrl Pts',(-10.0352227396569,66.0753597154,71.343769089941));
#123070=CARTESIAN_POINT('',(-13.5633022950147,81.8869258507955,67.0921386900969));
#123071=CARTESIAN_POINT('Ctrl Pts',(-13.5675364833309,81.8924678804059,
67.0873924564601));
#123072=CARTESIAN_POINT('Ctrl Pts',(-13.5675364833309,81.9977690181948,
67.2106037724578));
#123073=CARTESIAN_POINT('Ctrl Pts',(-13.5675364833309,82.0992425609522,
67.3359700547413));
#123074=CARTESIAN_POINT('Ctrl Pts',(-13.5675364833309,82.1969937123613,
67.4634099181992));
#123075=CARTESIAN_POINT('Ctrl Pts',(-13.5675364833309,82.2957238032808,
67.592126041995));
#123076=CARTESIAN_POINT('Ctrl Pts',(-13.5675364833309,82.3906568522104,
67.7229578489377));
#123077=CARTESIAN_POINT('Ctrl Pts',(-13.5675364833309,82.4818665253462,
67.8558621259143));
#123078=CARTESIAN_POINT('Ctrl Pts',(-13.5675364833309,82.5735780703432,
67.9894976950288));
#123079=CARTESIAN_POINT('Ctrl Pts',(-13.5675364833309,82.6615254275363,
68.1252289856858));
#123080=CARTESIAN_POINT('Ctrl Pts',(-13.5675364833309,82.7457443938265,
68.2630472884685));
#123081=CARTESIAN_POINT('Ctrl Pts',(-13.5675364833309,82.8298710462911,
68.4007145262914));
#123082=CARTESIAN_POINT('Ctrl Pts',(-13.5675364833309,82.9102777265511,
68.5404646023485));
#123083=CARTESIAN_POINT('Ctrl Pts',(-13.5675364833309,82.9869573381782,
68.6823179698962));
#123084=CARTESIAN_POINT('Ctrl Pts',(-13.5675364833309,83.0632243468457,
68.823408043029));
#123085=CARTESIAN_POINT('Ctrl Pts',(-13.5675364833309,83.135804521286,68.9665792259746));
#123086=CARTESIAN_POINT('Ctrl Pts',(-13.5675364833309,83.2046449902606,
69.111874551974));
#123087=CARTESIAN_POINT('Ctrl Pts',(-13.5675364833309,83.2725207161971,
69.2551336824574));
#123088=CARTESIAN_POINT('Ctrl Pts',(-13.5675364833309,83.336760991513,69.400458221822));
#123089=CARTESIAN_POINT('Ctrl Pts',(-13.5675364833309,83.3972675206113,
69.5479059599801));
#123090=CARTESIAN_POINT('Ctrl Pts',(-13.5675364833309,83.4288997535913,
69.6249902230389));
#123091=CARTESIAN_POINT('Ctrl Pts',(-13.5675364833309,83.4595107091917,
69.7026550175545));
#123092=CARTESIAN_POINT('Ctrl Pts',(-13.5675364833309,83.4890807917262,
69.7809099116504));
#123093=CARTESIAN_POINT('Ctrl Pts',(-13.5675364833309,83.5462497067958,
69.9322029420008));
#123094=CARTESIAN_POINT('Ctrl Pts',(-13.5675364833309,83.5995311272314,
70.0857015184292));
#123095=CARTESIAN_POINT('Ctrl Pts',(-13.5675364833309,83.6488530159178,
70.2414380131213));
#123096=CARTESIAN_POINT('Ctrl Pts',(-13.5675364833309,83.6976829222368,
70.3956210472426));
#123097=CARTESIAN_POINT('Ctrl Pts',(-13.5675364833309,83.742631951158,70.5519980279251));
#123098=CARTESIAN_POINT('Ctrl Pts',(-13.5675364833309,83.7835790887525,
70.7106003983674));
#123099=CARTESIAN_POINT('Ctrl Pts',(-13.5675364833309,83.8216452441033,
70.8580437320634));
#123100=CARTESIAN_POINT('Ctrl Pts',(-13.5675364833309,83.8562524416585,
71.0074106221777));
#123101=CARTESIAN_POINT('Ctrl Pts',(-13.5675364833309,83.8872622912965,
71.1587211275468));
#123102=CARTESIAN_POINT('Ctrl Pts',(-13.5675364833309,83.8940456959048,
71.1918203005962));
#123103=CARTESIAN_POINT('Ctrl Pts',(-13.5675364833309,83.9006568071547,
71.2250124483185));
#123104=CARTESIAN_POINT('Ctrl Pts',(-13.5675364833309,83.907093914309,71.2582977234034));
#123105=CARTESIAN_POINT('Ctrl Pts',(-13.5675364833309,83.910075144381,71.2737131981902));
#123106=CARTESIAN_POINT('Ctrl Pts',(-13.5675364833309,83.9130190507611,
71.289148647634));
#123107=CARTESIAN_POINT('Ctrl Pts',(-13.5675364833309,83.9159254565328,
71.3046040850435));
#123108=CARTESIAN_POINT('Ctrl Pts',(-13.5675364833309,83.9182590717436,
71.317013585527));
#123109=CARTESIAN_POINT('Ctrl Pts',(-13.5675364833309,83.9205689816703,
71.3294386553613));
#123110=CARTESIAN_POINT('Ctrl Pts',(-13.5675364833309,83.9228508036666,
71.3418555967155));
#123111=CARTESIAN_POINT('Ctrl Pts',(-13.5675364833309,83.9522228601566,
71.5016888805896));
#123112=CARTESIAN_POINT('Ctrl Pts',(-13.5675364833309,83.977099558419,71.6609852694542));
#123113=CARTESIAN_POINT('Ctrl Pts',(-13.5675364833309,83.9976830999355,
71.8196936146382));
#123114=CARTESIAN_POINT('Ctrl Pts',(-13.5675364833309,84.0186174256015,
71.9811066630849));
#123115=CARTESIAN_POINT('Ctrl Pts',(-13.5675364833309,84.0351110922124,
72.141911865271));
#123116=CARTESIAN_POINT('Ctrl Pts',(-13.5675364833309,84.0473295499119,
72.3020822045462));
#123117=CARTESIAN_POINT('Ctrl Pts',(-13.5675364833309,84.0601988915448,
72.4707849055154));
#123118=CARTESIAN_POINT('Ctrl Pts',(-13.5675364833309,84.0683258291414,
72.6387836571667));
#123119=CARTESIAN_POINT('Ctrl Pts',(-13.5675364833309,84.071847456582,72.8060705862103));
#123120=CARTESIAN_POINT('Ctrl Pts',(-13.5675364833309,84.0752820285138,
72.9692221406381));
#123121=CARTESIAN_POINT('Ctrl Pts',(-13.5675364833309,84.0743359159924,
73.1316972062282));
#123122=CARTESIAN_POINT('Ctrl Pts',(-13.5675364833309,84.0690840216172,
73.2935029730835));
#123123=CARTESIAN_POINT('Ctrl Pts',(-13.5675364833309,84.0636324489359,
73.4614606346904));
#123124=CARTESIAN_POINT('Ctrl Pts',(-13.5675364833309,84.0535418104486,
73.6286976277291));
#123125=CARTESIAN_POINT('Ctrl Pts',(-13.5675364833309,84.0388373131803,
73.7952298789199));
#123126=CARTESIAN_POINT('Ctrl Pts',(-13.5675364833309,84.0241328159119,
73.9617621301106));
#123127=CARTESIAN_POINT('Ctrl Pts',(-13.5675364833309,84.0048144863583,
74.1275901954544));
#123128=CARTESIAN_POINT('Ctrl Pts',(-13.5675364833309,83.9808477027752,
74.2927296910418));
#123129=CARTESIAN_POINT('Ctrl Pts',(-13.5675364833309,83.9577030737421,
74.4522042551125));
#123130=CARTESIAN_POINT('Ctrl Pts',(-13.5675364833309,83.9302230679344,
74.611037108983));
#123131=CARTESIAN_POINT('Ctrl Pts',(-13.5675364833309,83.8984368670594,
74.769252947345));
#123132=CARTESIAN_POINT('Ctrl Pts',(-13.5675364833309,83.8666355215599,
74.9275441680868));
#123133=CARTESIAN_POINT('Ctrl Pts',(-13.5675364833309,83.8305237251017,
75.0852182238534));
#123134=CARTESIAN_POINT('Ctrl Pts',(-13.5675364833309,83.7900804621859,
75.2422858250677));
#123135=CARTESIAN_POINT('Ctrl Pts',(-13.5675364833309,83.7498958119861,
75.3983490642201));
#123136=CARTESIAN_POINT('Ctrl Pts',(-13.5675364833309,83.7054347308817,
75.5538140031912));
#123137=CARTESIAN_POINT('Ctrl Pts',(-13.5675364833309,83.6566295892481,
75.7086709106651));
#123138=CARTESIAN_POINT('Ctrl Pts',(-13.5675364833309,83.6256590203533,
75.8069393791343));
#123139=CARTESIAN_POINT('Ctrl Pts',(-13.5675364833309,83.5929382246295,
75.9049625778693));
#123140=CARTESIAN_POINT('Ctrl Pts',(-13.5675364833309,83.558440477199,76.0027325471775));
#123141=CARTESIAN_POINT('Ctrl Pts',(-13.5590681066986,81.8921747150299,
67.0870494451112));
#123142=CARTESIAN_POINT('Ctrl Pts',(-13.5542716148093,81.7920287222896,
66.9698818089279));
#123143=CARTESIAN_POINT('Ctrl Pts',(-13.5495044344257,81.6889149671049,
66.8552469756093));
#123144=CARTESIAN_POINT('Ctrl Pts',(-13.5372447085138,81.4124470616348,
66.563205798704));
#123145=CARTESIAN_POINT('Ctrl Pts',(-13.529861101716,81.2345601511849,66.3900885153774));
#123146=CARTESIAN_POINT('Ctrl Pts',(-13.5199226290234,80.9740045601888,
66.156827913568));
#123147=CARTESIAN_POINT('Ctrl Pts',(-13.5170895307345,80.8970775777746,
66.0902902151318));
#123148=CARTESIAN_POINT('Ctrl Pts',(-13.5125120131832,80.7680020470132,
65.9824745318577));
#123149=CARTESIAN_POINT('Ctrl Pts',(-13.5107324021522,80.7165917930754,
65.9404996883744));
#123150=CARTESIAN_POINT('Ctrl Pts',(-13.5071900740137,80.6118804334446,
65.8569317744254));
#123151=CARTESIAN_POINT('Ctrl Pts',(-13.5054283118564,80.5585625821676,
65.8153609276827));
#123152=CARTESIAN_POINT('Ctrl Pts',(-13.5010903681271,80.4243331006755,
65.7131198731638));
#123153=CARTESIAN_POINT('Ctrl Pts',(-13.4985435658636,80.3428494857749,
65.6532011411002));
#123154=CARTESIAN_POINT('Ctrl Pts',(-13.4885613616639,80.0136753562677,
65.4195494435737));
#123155=CARTESIAN_POINT('Ctrl Pts',(-13.481492094847,79.7581702326144,65.2568101746283));
#123156=CARTESIAN_POINT('Ctrl Pts',(-13.4588390414386,78.8891870017602,
64.7620196695988));
#123157=CARTESIAN_POINT('Ctrl Pts',(-13.4441362070671,78.2434647223616,
64.4860491263886));
#123158=CARTESIAN_POINT('Ctrl Pts',(-13.4198273992042,77.217813969253,64.1813375254656));
#123159=CARTESIAN_POINT('Ctrl Pts',(-13.4109965907119,76.8543859453273,
64.0973701782848));
#123160=CARTESIAN_POINT('Ctrl Pts',(-13.3959694872772,76.2561904286052,
63.9984996318914));
#123161=CARTESIAN_POINT('Ctrl Pts',(-13.3900843911558,76.0255742570212,
63.9695480407988));
#123162=CARTESIAN_POINT('Ctrl Pts',(-13.3774389878636,75.5360882992717,
63.9270862755009));
#123163=CARTESIAN_POINT('Ctrl Pts',(-13.3706562147548,75.2770273815881,
63.9157442749326));
#123164=CARTESIAN_POINT('Ctrl Pts',(-13.347732045806,74.4106296861599,63.9145582499049));
#123165=CARTESIAN_POINT('Ctrl Pts',(-13.3312825573389,73.8030388329621,
63.9741128273904));
#123166=CARTESIAN_POINT('Ctrl Pts',(-13.3068741897951,72.9206303161106,
64.150906941191));
#123167=CARTESIAN_POINT('Ctrl Pts',(-13.2989021548328,72.6365043448969,
64.2222676715389));
#123168=CARTESIAN_POINT('Ctrl Pts',(-13.2841430096769,72.11390741135,64.3812599171973));
#123169=CARTESIAN_POINT('Ctrl Pts',(-13.2774143257934,71.8748867859194,
64.4653481326174));
#123170=CARTESIAN_POINT('Ctrl Pts',(-13.26220366846,71.3373124473978,64.6802439653337));
#123171=CARTESIAN_POINT('Ctrl Pts',(-13.2537603715575,71.0411819714063,
64.8176543050313));
#123172=CARTESIAN_POINT('Ctrl Pts',(-13.2347161766478,70.3900011803531,
65.1631713777577));
#123173=CARTESIAN_POINT('Ctrl Pts',(-13.2241240900908,70.0397173233626,
65.3804032542507));
#123174=CARTESIAN_POINT('Ctrl Pts',(-13.2051183934299,69.4482949212431,
65.8047240141437));
#123175=CARTESIAN_POINT('Ctrl Pts',(-13.1967624649786,69.2005327453609,
66.00270251492));
#123176=CARTESIAN_POINT('Ctrl Pts',(-13.1818819584551,68.7862115849624,
66.3710115826409));
#123177=CARTESIAN_POINT('Ctrl Pts',(-13.1754097133126,68.6148257190972,
66.535904073327));
#123178=CARTESIAN_POINT('Ctrl Pts',(-13.1624110166355,68.2799723187363,
66.8849633204276));
#123179=CARTESIAN_POINT('Ctrl Pts',(-13.1559150838736,68.1172195495557,
67.0694098321845));
#123180=CARTESIAN_POINT('Ctrl Pts',(-13.1354655682893,67.6240205700236,
67.6765416477148));
#123181=CARTESIAN_POINT('Ctrl Pts',(-13.1217679375107,67.322809964869,68.123242778279));
#123182=CARTESIAN_POINT('Ctrl Pts',(-13.1015177943972,66.9432140501511,
68.8085880289499));
#123183=CARTESIAN_POINT('Ctrl Pts',(-13.0950997382616,66.8323194547083,
69.0293555972505));
#123184=CARTESIAN_POINT('Ctrl Pts',(-13.0773000587725,66.5537365188385,
69.6448401820738));
#123185=CARTESIAN_POINT('Ctrl Pts',(-13.0655752232905,66.4044147511725,
70.047863266239));
#123186=CARTESIAN_POINT('Ctrl Pts',(-13.0486019735719,66.2296064977183,
70.6489567976515));
#123187=CARTESIAN_POINT('Ctrl Pts',(-13.043332694699,66.1809619688838,70.839625496625));
#123188=CARTESIAN_POINT('Ctrl Pts',(-13.0239654869984,66.0229808213967,
71.5572526921515));
#123189=CARTESIAN_POINT('Ctrl Pts',(-13.0103353904296,65.9546993289936,
72.0927051944972));
#123190=CARTESIAN_POINT('Ctrl Pts',(-12.9885990908377,65.9215169832869,
72.94027813103));
#123191=CARTESIAN_POINT('Ctrl Pts',(-12.9805888307732,65.9251310481666,
73.2512490738343));
#123192=CARTESIAN_POINT('Ctrl Pts',(-12.9675766122192,65.9559266866908,
73.74381766199));
#123193=CARTESIAN_POINT('Ctrl Pts',(-12.9626850690453,65.9728160711133,
73.9260876702788));
#123194=CARTESIAN_POINT('Ctrl Pts',(-12.9484343499011,66.0370404315548,
74.4475702119123));
#123195=CARTESIAN_POINT('Ctrl Pts',(-12.9389457038534,66.098081394884,74.7850890378309));
#123196=CARTESIAN_POINT('Ctrl Pts',(-12.925582513397,66.2141810184528,75.2668037068532));
#123197=CARTESIAN_POINT('Ctrl Pts',(-12.9215223251056,66.2538082057257,
75.4143612272045));
#123198=CARTESIAN_POINT('Ctrl Pts',(-12.9103588328681,66.3746781881217,
75.8224056279332));
#123199=CARTESIAN_POINT('Ctrl Pts',(-12.9033635871439,66.4640962439975,
76.0803740916759));
#123200=CARTESIAN_POINT('Ctrl Pts',(-12.8882860121754,66.6828685200793,
76.6303282834251));
#123201=CARTESIAN_POINT('Ctrl Pts',(-12.880219860982,66.8164302170816,76.9206510033425));
#123202=CARTESIAN_POINT('Ctrl Pts',(-12.8666140533297,67.0629123031222,
77.3903188047085));
#123203=CARTESIAN_POINT('Ctrl Pts',(-12.8611410249638,67.1675695463286,
77.5740349716444));
#123204=CARTESIAN_POINT('Ctrl Pts',(-12.8511834084674,67.3655746794775,
77.8952730849634));
#123205=CARTESIAN_POINT('Ctrl Pts',(-12.8467286199518,67.4565482303131,
78.0342668066983));
#123206=CARTESIAN_POINT('Ctrl Pts',(-12.833995788073,67.7239259088111,78.4194204642622));
#123207=CARTESIAN_POINT('Ctrl Pts',(-12.8256153163989,67.9089901421128,
78.6595736177276));
#123208=CARTESIAN_POINT('Ctrl Pts',(-12.812629429129,68.2185515999683,79.0218455084534));
#123209=CARTESIAN_POINT('Ctrl Pts',(-12.8079363573752,68.3352956683199,
79.1507091594142));
#123210=CARTESIAN_POINT('Ctrl Pts',(-12.7990549287592,68.5677928938533,
79.3926279738622));
#123211=CARTESIAN_POINT('Ctrl Pts',(-12.7948525605507,68.6828733112431,
79.5060229309362));
#123212=CARTESIAN_POINT('Ctrl Pts',(-12.7806824443328,69.085267748706,79.8817244083457));
#123213=CARTESIAN_POINT('Ctrl Pts',(-12.7709327824128,69.3868228250467,
80.1287660236168));
#123214=CARTESIAN_POINT('Ctrl Pts',(-12.7566803432005,69.8424642292089,
80.4559321600454));
#123215=CARTESIAN_POINT('Ctrl Pts',(-12.7522856836234,69.9849367350732,
80.552272782412));
#123216=CARTESIAN_POINT('Ctrl Pts',(-12.7440584346135,70.2528646125522,
80.7226820373419));
#123217=CARTESIAN_POINT('Ctrl Pts',(-12.7402422777692,70.3775937352692,
80.7979062825841));
#123218=CARTESIAN_POINT('Ctrl Pts',(-12.7276119703817,70.7894664750456,
81.0331177540324));
#123219=CARTESIAN_POINT('Ctrl Pts',(-12.7185610917208,71.0836724484624,
81.1807805316131));
#123220=CARTESIAN_POINT('Ctrl Pts',(-12.702293439271,71.6269553837915,81.4174559790179));
#123221=CARTESIAN_POINT('Ctrl Pts',(-12.6950675809478,71.8735050770989,
81.512293743389));
#123222=CARTESIAN_POINT('Ctrl Pts',(-12.6845676398191,72.2467370303841,
81.6371436992725));
#123223=CARTESIAN_POINT('Ctrl Pts',(-12.6811649282168,72.3703507424593,
81.6755062985264));
#123224=CARTESIAN_POINT('Ctrl Pts',(-12.6696724559748,72.7959008790564,
81.7974905154234));
#123225=CARTESIAN_POINT('Ctrl Pts',(-12.6617808167259,73.1014806864576,
81.8679574019711));
#123226=CARTESIAN_POINT('Ctrl Pts',(-12.646439637525,73.7008182023705,81.9739776539254));
#123227=CARTESIAN_POINT('Ctrl Pts',(-12.6389889782674,73.9942699533495,
82.011283164141));
#123228=CARTESIAN_POINT('Ctrl Pts',(-12.6278434068756,74.4232051779274,
82.0448901912824));
#123229=CARTESIAN_POINT('Ctrl Pts',(-12.6243059456231,74.5578259666299,
82.0524580466115));
#123230=CARTESIAN_POINT('Ctrl Pts',(-12.6148482026504,74.9128642445359,
82.0645788122341));
#123231=CARTESIAN_POINT('Ctrl Pts',(-12.6088559346375,75.1334576442571,
82.06416141907));
#123232=CARTESIAN_POINT('Ctrl Pts',(-12.5953156808615,75.6281410419969,
82.0453178066303));
#123233=CARTESIAN_POINT('Ctrl Pts',(-12.5877472401498,75.9020786960933,
82.0224912276371));
#123234=CARTESIAN_POINT('Ctrl Pts',(-12.5754682039387,76.3504212585025,
81.9644199628588));
#123235=CARTESIAN_POINT('Ctrl Pts',(-12.5706936698356,76.5257589578696,
81.9364229349427));
#123236=CARTESIAN_POINT('Ctrl Pts',(-12.5623439346404,76.8364716997386,
81.8772308815007));
#123237=CARTESIAN_POINT('Ctrl Pts',(-12.5587450920961,76.9720237602414,
81.8480940252307));
#123238=CARTESIAN_POINT('Ctrl Pts',(-12.5463814236343,77.4405981239887,
81.7359365737801));
#123239=CARTESIAN_POINT('Ctrl Pts',(-12.5378228793052,77.769782858668,81.6368484111675));
#123240=CARTESIAN_POINT('Ctrl Pts',(-12.5252668781339,78.2367696310233,
81.4670486765995));
#123241=CARTESIAN_POINT('Ctrl Pts',(-12.5213608271997,78.3798637588088,
81.4108881467845));
#123242=CARTESIAN_POINT('Ctrl Pts',(-12.5138496797056,78.6483701795652,
81.2976356180653));
#123243=CARTESIAN_POINT('Ctrl Pts',(-12.5102502760716,78.7740794318261,
81.2412427123319));
#123244=CARTESIAN_POINT('Ctrl Pts',(-12.4945868895627,79.307834183047,80.9872211680897));
#123245=CARTESIAN_POINT('Ctrl Pts',(-12.4820732174252,79.7028366912285,
80.7620305089869));
#123246=CARTESIAN_POINT('Ctrl Pts',(-12.4648059240783,80.227945570971,80.40821904971));
#123247=CARTESIAN_POINT('Ctrl Pts',(-12.4599257936274,80.3740861746635,
80.3033082210613));
#123248=CARTESIAN_POINT('Ctrl Pts',(-12.4511559708814,80.634188495179,80.1044868638146));
#123249=CARTESIAN_POINT('Ctrl Pts',(-12.4472457653971,80.7492164195056,
80.0119814787204));
#123250=CARTESIAN_POINT('Ctrl Pts',(-12.4332795506338,81.1582244220697,
79.6659256628228));
#123251=CARTESIAN_POINT('Ctrl Pts',(-12.4236150142218,81.4380023386033,
79.3958458132811));
#123252=CARTESIAN_POINT('Ctrl Pts',(-12.4100069435382,81.8010927749715,
78.9975352387134));
#123253=CARTESIAN_POINT('Ctrl Pts',(-12.4061747844966,81.9000221752958,
78.8834324251171));
#123254=CARTESIAN_POINT('Ctrl Pts',(-12.3984621213635,82.0906265432574,
78.6522776794879));
#123255=CARTESIAN_POINT('Ctrl Pts',(-12.3945765142021,82.1823911497242,
78.5352973120272));
#123256=CARTESIAN_POINT('Ctrl Pts',(-12.3827850493668,82.4487635846914,
78.1781950435444));
#123257=CARTESIAN_POINT('Ctrl Pts',(-12.3747418122683,82.6147305355668,
77.9315979227482));
#123258=CARTESIAN_POINT('Ctrl Pts',(-12.3588545103332,82.91685114776,77.4318820722629));
#123259=CARTESIAN_POINT('Ctrl Pts',(-12.351012514832,83.0538253470931,77.1792180890642));
#123260=CARTESIAN_POINT('Ctrl Pts',(-12.3379241347035,83.2647422152221,
76.741680778256));
#123261=CARTESIAN_POINT('Ctrl Pts',(-12.3326223872496,83.3451029286835,
76.5599022296358));
#123262=CARTESIAN_POINT('Ctrl Pts',(-12.3230759992552,83.4811363673166,
76.2221284152004));
#123263=CARTESIAN_POINT('Ctrl Pts',(-12.3188237233838,83.5385306234,76.0672737673675));
#123264=CARTESIAN_POINT('Ctrl Pts',(-12.3059762950662,83.7007336782974,
75.589358835331));
#123265=CARTESIAN_POINT('Ctrl Pts',(-12.2975196851177,83.7915195380404,
75.2617906469131));
#123266=CARTESIAN_POINT('Ctrl Pts',(-12.284416541049,83.9002990261761,74.7627277986276));
#123267=CARTESIAN_POINT('Ctrl Pts',(-12.2799483222741,83.9320801054606,
74.5942380095015));
#123268=CARTESIAN_POINT('Ctrl Pts',(-12.2676973283403,84.0053152103195,
74.1357483228414));
#123269=CARTESIAN_POINT('Ctrl Pts',(-12.2598136509086,84.03765462545,73.844267491681));
#123270=CARTESIAN_POINT('Ctrl Pts',(-12.243010956856,84.0765286814414,73.2241921333138));
#123271=CARTESIAN_POINT('Ctrl Pts',(-12.2340817631658,84.0794669516359,
72.8953261693159));
#123272=CARTESIAN_POINT('Ctrl Pts',(-12.2192024854395,84.0543085669752,
72.3413562601775));
#123273=CARTESIAN_POINT('Ctrl Pts',(-12.2131903613112,84.0355885901246,
72.1158209549323));
#123274=CARTESIAN_POINT('Ctrl Pts',(-12.1991156142519,83.9706342828342,
71.5807516670429));
#123275=CARTESIAN_POINT('Ctrl Pts',(-12.1912430531929,83.9166562606102,
71.2732499383507));
#123276=CARTESIAN_POINT('Ctrl Pts',(-12.1785628959082,83.8049388610954,
70.7861645488808));
#123277=CARTESIAN_POINT('Ctrl Pts',(-12.1737622640556,83.7571752478623,
70.6041849778724));
#123278=CARTESIAN_POINT('Ctrl Pts',(-12.1621925259686,83.6306908125787,
70.1765927133141));
#123279=CARTESIAN_POINT('Ctrl Pts',(-12.155381403236,83.5470588002038,69.9324277607096));
#123280=CARTESIAN_POINT('Ctrl Pts',(-12.135766427616,83.2795469543242,69.2470416383225));
#123281=CARTESIAN_POINT('Ctrl Pts',(-12.1228063212596,83.0709738936559,
68.8153488006643));
#123282=CARTESIAN_POINT('Ctrl Pts',(-12.1038849508357,82.7143540404618,
68.2049686009164));
#123283=CARTESIAN_POINT('Ctrl Pts',(-12.0977932247745,82.5913421194022,
68.0115833645262));
#123284=CARTESIAN_POINT('Ctrl Pts',(-12.0859684623677,82.3352464314142,
67.6411035413038));
#123285=CARTESIAN_POINT('Ctrl Pts',(-12.0802589120059,82.2029032967178,
67.4640614477432));
#123286=CARTESIAN_POINT('Ctrl Pts',(-12.0680022595118,81.901768283777,67.0911217221234));
#123287=CARTESIAN_POINT('Ctrl Pts',(-12.0614431166126,81.7312092381388,
66.8976311253861));
#123288=CARTESIAN_POINT('Ctrl Pts',(-12.0350907451483,81.0277197183915,
66.1648734460141));
#123289=CARTESIAN_POINT('Ctrl Pts',(-12.0146415565156,80.4340705962415,
65.6835536311353));
#123290=CARTESIAN_POINT('Ctrl Pts',(-11.9861207020082,79.5260624044424,
65.1177839484425));
#123291=CARTESIAN_POINT('Ctrl Pts',(-11.9778495822136,79.2529846788054,
64.9664801821875));
#123292=CARTESIAN_POINT('Ctrl Pts',(-11.9563975669566,78.516556851685,64.6073049986407));
#123293=CARTESIAN_POINT('Ctrl Pts',(-11.9435203999241,78.0439024990142,
64.4251713358605));
#123294=CARTESIAN_POINT('Ctrl Pts',(-11.8997917000753,76.4413545917399,
63.955826946439));
#123295=CARTESIAN_POINT('Ctrl Pts',(-11.8683582127767,75.2573169088765,
63.8422182709281));
#123296=CARTESIAN_POINT('Ctrl Pts',(-11.8230247640893,73.5295526399705,
64.0160172908243));
#123297=CARTESIAN_POINT('Ctrl Pts',(-11.8081872143295,72.9709249133046,
64.1266639140826));
#123298=CARTESIAN_POINT('Ctrl Pts',(-11.7711827409064,71.6199064620653,
64.5270034009169));
#123299=CARTESIAN_POINT('Ctrl Pts',(-11.738904698618,70.4680384568216,64.9838759366761));
#123300=CARTESIAN_POINT('Ctrl Pts',(-11.683963031582,68.8379068340988,66.3014728066721));
#123301=CARTESIAN_POINT('Ctrl Pts',(-11.6684195253985,68.4099673656422,
66.7237215655609));
#123302=CARTESIAN_POINT('Ctrl Pts',(-11.6445866614158,67.8269749097122,
67.4234734941558));
#123303=CARTESIAN_POINT('Ctrl Pts',(-11.6363748850356,67.6391360600916,
67.6738942448746));
#123304=CARTESIAN_POINT('Ctrl Pts',(-11.6139907705485,67.1672167477589,
68.3756301632476));
#123305=CARTESIAN_POINT('Ctrl Pts',(-11.5995675723112,66.9092625860644,
68.8432102479295));
#123306=CARTESIAN_POINT('Ctrl Pts',(-11.5761640350408,66.5517926648154,
69.6574927779121));
#123307=CARTESIAN_POINT('Ctrl Pts',(-11.5669860779528,66.4288090560081,
69.9894867289769));
#123308=CARTESIAN_POINT('Ctrl Pts',(-11.5416972747449,66.1432248448741,
70.9230510370065));
#123309=CARTESIAN_POINT('Ctrl Pts',(-11.5256205887917,66.0218137197234,
71.5374256873591));
#123310=CARTESIAN_POINT('Ctrl Pts',(-11.5015728944489,65.9379543872354,
72.4382896118954));
#123311=CARTESIAN_POINT('Ctrl Pts',(-11.4939376963333,65.9248703381677,
72.7202149910102));
#123312=CARTESIAN_POINT('Ctrl Pts',(-11.4799783985566,65.9253087201448,
73.2360564909682));
#123313=CARTESIAN_POINT('Ctrl Pts',(-11.4737305181669,65.9346898217129,
73.4691147765804));
#123314=CARTESIAN_POINT('Ctrl Pts',(-11.461462234947,65.9716054716059,73.9330051590798));
#123315=CARTESIAN_POINT('Ctrl Pts',(-11.4554357373374,65.9989288197087,
74.1632051665436));
#123316=CARTESIAN_POINT('Ctrl Pts',(-11.436431174078,66.1134062822752,74.8894375070278));
#123317=CARTESIAN_POINT('Ctrl Pts',(-11.4235929510636,66.2331522473532,
75.3804019438939));
#123318=CARTESIAN_POINT('Ctrl Pts',(-11.4039580363381,66.4715142352684,
76.0963920715314));
#123319=CARTESIAN_POINT('Ctrl Pts',(-11.3973588721539,66.5606049907156,
76.3313660082699));
#123320=CARTESIAN_POINT('Ctrl Pts',(-11.3855131280604,66.7346096341848,
76.7386951469584));
#123321=CARTESIAN_POINT('Ctrl Pts',(-11.380299463487,66.8155544511462,76.9127505942496));
#123322=CARTESIAN_POINT('Ctrl Pts',(-11.3676148063142,67.0251092041908,
77.3281676202458));
#123323=CARTESIAN_POINT('Ctrl Pts',(-11.360145787446,67.1594163536749,77.5668108127286));
#123324=CARTESIAN_POINT('Ctrl Pts',(-11.3470740162834,67.4204480446439,
77.9840353655374));
#123325=CARTESIAN_POINT('Ctrl Pts',(-11.341390207838,67.5427478377599,78.164464478255));
#123326=CARTESIAN_POINT('Ctrl Pts',(-11.3278575667772,67.8521077144758,
78.5871696700794));
#123327=CARTESIAN_POINT('Ctrl Pts',(-11.3200632355294,68.045343253798,78.824924085721));
#123328=CARTESIAN_POINT('Ctrl Pts',(-11.303856794792,68.4695769470887,79.2965611134832));
#123329=CARTESIAN_POINT('Ctrl Pts',(-11.295439055484,68.7023320071261,79.528916990291));
#123330=CARTESIAN_POINT('Ctrl Pts',(-11.2822070002329,69.0783193405568,
79.8659813912701));
#123331=CARTESIAN_POINT('Ctrl Pts',(-11.2775251264432,69.2132061360693,
79.9800526775385));
#123332=CARTESIAN_POINT('Ctrl Pts',(-11.2635480851696,69.6188891659272,
80.3034138395053));
#123333=CARTESIAN_POINT('Ctrl Pts',(-11.2540666495126,69.8984948524752,
80.5016572189363));
#123334=CARTESIAN_POINT('Ctrl Pts',(-11.2402553948987,70.3294348510951,
80.7715033277092));
#123335=CARTESIAN_POINT('Ctrl Pts',(-11.2357957702606,70.4726147436903,
80.8556940786965));
#123336=CARTESIAN_POINT('Ctrl Pts',(-11.226031295672,70.7966107214824,81.0341546158046));
#123337=CARTESIAN_POINT('Ctrl Pts',(-11.2207595596775,70.9781670271131,
81.1262131508542));
#123338=CARTESIAN_POINT('Ctrl Pts',(-11.2077292262514,71.4386085384673,
81.3404794186449));
#123339=CARTESIAN_POINT('Ctrl Pts',(-11.2000345207221,71.7210793827409,
81.4549782229865));
#123340=CARTESIAN_POINT('Ctrl Pts',(-11.1849992988541,72.2792537971876,
81.6494725518392));
#123341=CARTESIAN_POINT('Ctrl Pts',(-11.1776627778634,72.5544204164013,
81.7310975951903));
#123342=CARTESIAN_POINT('Ctrl Pts',(-11.1661861333091,72.9796903608049,
81.8358593485588));
#123343=CARTESIAN_POINT('Ctrl Pts',(-11.1621696184886,73.1274980702723,
81.8684154793323));
#123344=CARTESIAN_POINT('Ctrl Pts',(-11.1536965122738,73.4362445673246,
81.9284303650665));
#123345=CARTESIAN_POINT('Ctrl Pts',(-11.14923889819,73.5973034419281,81.9552859638776));
#123346=CARTESIAN_POINT('Ctrl Pts',(-11.1354479115498,74.095608384285,82.0246398185578));
#123347=CARTESIAN_POINT('Ctrl Pts',(-11.1260611004602,74.4348687842597,
82.0526069627284));
#123348=CARTESIAN_POINT('Ctrl Pts',(-11.1132847863632,74.9137958663528,
82.0645609659671));
#123349=CARTESIAN_POINT('Ctrl Pts',(-11.1096344325108,75.0528851330426,
82.0647569843448));
#123350=CARTESIAN_POINT('Ctrl Pts',(-11.097451488835,75.5222664236924,82.0545033550214));
#123351=CARTESIAN_POINT('Ctrl Pts',(-11.0891109015025,75.8522790135066,
82.0290056159743));
#123352=CARTESIAN_POINT('Ctrl Pts',(-11.0731591278899,76.4779139290216,
81.9463295571717));
#123353=CARTESIAN_POINT('Ctrl Pts',(-11.0655487002234,76.773957797436,81.8922289112971));
#123354=CARTESIAN_POINT('Ctrl Pts',(-11.0541089926271,77.2027813124686,
81.7919009598897));
#123355=CARTESIAN_POINT('Ctrl Pts',(-11.0504324152805,77.3382213250744,
81.7569309772833));
#123356=CARTESIAN_POINT('Ctrl Pts',(-11.0395110816555,77.7319107042377,
81.6456185433552));
#123357=CARTESIAN_POINT('Ctrl Pts',(-11.0321327395218,77.9878144579349,
81.560936713203));
#123358=CARTESIAN_POINT('Ctrl Pts',(-11.0160723366018,78.5345152964866,
81.3526799100089));
#123359=CARTESIAN_POINT('Ctrl Pts',(-11.0073864060271,78.8237214348501,
81.2249110123661));
#123360=CARTESIAN_POINT('Ctrl Pts',(-10.995523273993,79.2203641592331,81.0238803300764));
#123361=CARTESIAN_POINT('Ctrl Pts',(-10.9921389815689,79.3338722568417,
80.9632120031192));
#123362=CARTESIAN_POINT('Ctrl Pts',(-10.9851430172786,79.5687433371426,
80.8310605102586));
#123363=CARTESIAN_POINT('Ctrl Pts',(-10.9815399342954,79.6897131415036,
80.759182953659));
#123364=CARTESIAN_POINT('Ctrl Pts',(-10.970129390683,80.0701013964238,80.5209530187167));
#123365=CARTESIAN_POINT('Ctrl Pts',(-10.9624233072592,80.3228815115587,
80.3440073690476));
#123366=CARTESIAN_POINT('Ctrl Pts',(-10.9494508315752,80.7266720984723,
80.0298384114745));
#123367=CARTESIAN_POINT('Ctrl Pts',(-10.9442447135714,80.883087339794,79.8995387813573));
#123368=CARTESIAN_POINT('Ctrl Pts',(-10.9352272618405,81.1406594814284,
79.6700506114573));
#123369=CARTESIAN_POINT('Ctrl Pts',(-10.931468298786,81.2441438311538,79.5734655898293));
#123370=CARTESIAN_POINT('Ctrl Pts',(-10.9229822704551,81.470005458756,79.3526661384571));
#123371=CARTESIAN_POINT('Ctrl Pts',(-10.9182350454293,81.5912007312285,
79.2272356724659));
#123372=CARTESIAN_POINT('Ctrl Pts',(-10.9020030173533,81.9911897640813,
78.7888296477144));
#123373=CARTESIAN_POINT('Ctrl Pts',(-10.8904187287239,82.2523713314234,
78.4597671882362));
#123374=CARTESIAN_POINT('Ctrl Pts',(-10.8758390717496,82.5626442097709,
78.0067722268572));
#123375=CARTESIAN_POINT('Ctrl Pts',(-10.872443510504,82.6335816113649,77.8981809201727));
#123376=CARTESIAN_POINT('Ctrl Pts',(-10.8615128088464,82.8571960949351,
77.5389438864602));
#123377=CARTESIAN_POINT('Ctrl Pts',(-10.854151008882,82.9998691784603,77.2823937818435));
#123378=CARTESIAN_POINT('Ctrl Pts',(-10.8398330113968,83.2520152333316,
76.7724142411953));
#123379=CARTESIAN_POINT('Ctrl Pts',(-10.8328778790993,83.3629621935259,
76.5197172542601));
#123380=CARTESIAN_POINT('Ctrl Pts',(-10.8220340017719,83.5134344201952,
76.1302013555007));
#123381=CARTESIAN_POINT('Ctrl Pts',(-10.8182906544755,83.5614911438892,
75.9966613381224));
#123382=CARTESIAN_POINT('Ctrl Pts',(-10.8100790459964,83.6589444655758,
75.7047932533741));
#123383=CARTESIAN_POINT('Ctrl Pts',(-10.805596054612,83.707201183287,75.5460768921971));
#123384=CARTESIAN_POINT('Ctrl Pts',(-10.7905233374584,83.8539709219854,
75.0116408948854));
#123385=CARTESIAN_POINT('Ctrl Pts',(-10.7798132579853,83.9330152256115,
74.6305418036001));
#123386=CARTESIAN_POINT('Ctrl Pts',(-10.7648866957545,84.0103282714376,
74.0816038978186));
#123387=CARTESIAN_POINT('Ctrl Pts',(-10.7604640999119,84.0289311753907,
73.91663382697));
#123388=CARTESIAN_POINT('Ctrl Pts',(-10.7518282430458,84.0566969974354,
73.5881549578561));
#123389=CARTESIAN_POINT('Ctrl Pts',(-10.7476287681822,84.0659508983708,
73.4249268254314));
#123390=CARTESIAN_POINT('Ctrl Pts',(-10.7369089950463,84.0783125154229,
73.0034218628282));
#123391=CARTESIAN_POINT('Ctrl Pts',(-10.7304495321392,84.0747281652656,
72.7449048836405));
#123392=CARTESIAN_POINT('Ctrl Pts',(-10.7189021956243,84.0489699557529,
72.2887506864487));
#123393=CARTESIAN_POINT('Ctrl Pts',(-10.7138396085273,84.0312872964701,
72.0908628998149));
#123394=CARTESIAN_POINT('Ctrl Pts',(-10.7040256390475,83.9856008159391,
71.717068354512));
#123395=CARTESIAN_POINT('Ctrl Pts',(-10.6993074056721,83.9588552189296,
71.5410052129082));
#123396=CARTESIAN_POINT('Ctrl Pts',(-10.6883676563367,83.8857880556542,
71.1390987168748));
#123397=CARTESIAN_POINT('Ctrl Pts',(-10.6821126698903,83.8360159121452,
70.913866793063));
#123398=CARTESIAN_POINT('Ctrl Pts',(-10.6647578788761,83.6748783135999,
70.2963632020085));
#123399=CARTESIAN_POINT('Ctrl Pts',(-10.6536314488456,83.5455642563476,
69.9087429247327));
#123400=CARTESIAN_POINT('Ctrl Pts',(-10.6387704893156,83.3320061063279,
69.3894003495198));
#123401=CARTESIAN_POINT('Ctrl Pts',(-10.6347472808774,83.2698176549128,
69.2485817466867));
#123402=CARTESIAN_POINT('Ctrl Pts',(-10.6267493833386,83.1369122834732,
68.9676880493098));
#123403=CARTESIAN_POINT('Ctrl Pts',(-10.622775296033,83.0661878347582,68.8278812557266));
#123404=CARTESIAN_POINT('Ctrl Pts',(-10.6106636336823,82.8388717217479,
68.40621890752));
#123405=CARTESIAN_POINT('Ctrl Pts',(-10.60255735847,82.6706398329936,68.1306584318951));
#123406=CARTESIAN_POINT('Ctrl Pts',(-10.5885771942367,82.3668852831137,
67.6875722247586));
#123407=CARTESIAN_POINT('Ctrl Pts',(-10.5828885964537,82.2391850817937,
67.5146839739715));
#123408=CARTESIAN_POINT('Ctrl Pts',(-10.5692504803771,81.921960006923,67.1153221651725));
#123409=CARTESIAN_POINT('Ctrl Pts',(-10.5612512148942,81.727165806553,66.8929947304493));
#123410=CARTESIAN_POINT('Ctrl Pts',(-10.5435319075459,81.2722102448684,
66.4218138464385));
#123411=CARTESIAN_POINT('Ctrl Pts',(-10.5338183891719,81.0070363711832,
66.1777518799018));
#123412=CARTESIAN_POINT('Ctrl Pts',(-10.5194676891263,80.5855150542378,
65.8341332595257));
#123413=CARTESIAN_POINT('Ctrl Pts',(-10.5146683306702,80.4392027997058,
65.7221643306107));
#123414=CARTESIAN_POINT('Ctrl Pts',(-10.5047176744966,80.1239421895527,
65.4961505584553));
#123415=CARTESIAN_POINT('Ctrl Pts',(-10.499576210428,79.9545533087552,65.383294232073));
#123416=CARTESIAN_POINT('Ctrl Pts',(-10.4888830249124,79.5967004160453,
65.1619505119251));
#123417=CARTESIAN_POINT('Ctrl Pts',(-10.4833082953928,79.4077355140865,
65.0542964008141));
#123418=CARTESIAN_POINT('Ctrl Pts',(-10.4702868364309,78.9660838679099,
64.8231668544518));
#123419=CARTESIAN_POINT('Ctrl Pts',(-10.4628034926422,78.7109646074756,
64.7043176959357));
#123420=CARTESIAN_POINT('Ctrl Pts',(-10.4429926927163,78.0283863439525,
64.4236983412069));
#123421=CARTESIAN_POINT('Ctrl Pts',(-10.4305578883603,77.5927797074079,
64.2814987911854));
#123422=CARTESIAN_POINT('Ctrl Pts',(-10.4117972714492,76.9121080083537,
64.1147808037987));
#123423=CARTESIAN_POINT('Ctrl Pts',(-10.4053261437037,76.6728659880689,
64.0663019989242));
#123424=CARTESIAN_POINT('Ctrl Pts',(-10.3924704747258,76.1857043884102,
63.9881669547922));
#123425=CARTESIAN_POINT('Ctrl Pts',(-10.3861511257801,75.9386255716942,
63.959137783098));
#123426=CARTESIAN_POINT('Ctrl Pts',(-10.3713108958127,75.3523051671442,
63.9148915114114));
#123427=CARTESIAN_POINT('Ctrl Pts',(-10.362733387284,75.0128591344745,63.9085165958738));
#123428=CARTESIAN_POINT('Ctrl Pts',(-10.3401166534282,74.1289295276929,
63.9410628493276));
#123429=CARTESIAN_POINT('Ctrl Pts',(-10.3260052712222,73.5854220383952,
64.0099614259926));
#123430=CARTESIAN_POINT('Ctrl Pts',(-10.3026746214761,72.7193661825693,
64.1994590185667));
#123431=CARTESIAN_POINT('Ctrl Pts',(-10.2935997285093,72.3903230828583,
64.29100020586));
#123432=CARTESIAN_POINT('Ctrl Pts',(-10.2771851687998,71.8164515781705,
64.4864564148652));
#123433=CARTESIAN_POINT('Ctrl Pts',(-10.2699644152529,71.569986256241,64.5828222381821));
#123434=CARTESIAN_POINT('Ctrl Pts',(-10.2547777509193,71.0769910820738,
64.8014282605783));
#123435=CARTESIAN_POINT('Ctrl Pts',(-10.2467455153074,70.8317810443425,
64.9238945174778));
#123436=CARTESIAN_POINT('Ctrl Pts',(-10.2197265688772,70.0470125104654,
65.3610879081932));
#123437=CARTESIAN_POINT('Ctrl Pts',(-10.1998805061955,69.5325629390287,
65.7212544317407));
#123438=CARTESIAN_POINT('Ctrl Pts',(-10.1710850937717,68.8153166755438,
66.3412913225327));
#123439=CARTESIAN_POINT('Ctrl Pts',(-10.1614971478665,68.5817403100494,
66.565910497724));
#123440=CARTESIAN_POINT('Ctrl Pts',(-10.1496876337135,68.2943085028007,
66.8737771833284));
#123441=CARTESIAN_POINT('Ctrl Pts',(-10.1469980858286,68.2288702338781,
66.9461926427268));
#123442=CARTESIAN_POINT('Ctrl Pts',(-10.1426652596873,68.1232727188615,
67.0669657211208));
#123443=CARTESIAN_POINT('Ctrl Pts',(-10.1409904959236,68.082410690264,67.1147062631595));
#123444=CARTESIAN_POINT('Ctrl Pts',(-10.1377322385359,68.0027565016216,
67.209789323264));
#123445=CARTESIAN_POINT('Ctrl Pts',(-10.1361495029794,67.9639758520655,
67.2570649985359));
#123446=CARTESIAN_POINT('Ctrl Pts',(-10.1320253387701,67.8627351097104,
67.3831132172281));
#123447=CARTESIAN_POINT('Ctrl Pts',(-10.1295231532016,67.8011406699431,
67.4625170228407));
#123448=CARTESIAN_POINT('Ctrl Pts',(-10.1209819085711,67.5911480164043,
67.742829592026));
#123449=CARTESIAN_POINT('Ctrl Pts',(-10.1152119461978,67.4497532638925,
67.9489759575478));
#123450=CARTESIAN_POINT('Ctrl Pts',(-10.1050291723372,67.2082880174862,
68.334092729626));
#123451=CARTESIAN_POINT('Ctrl Pts',(-10.1005588812509,67.1053631655791,
68.5112665138926));
#123452=CARTESIAN_POINT('Ctrl Pts',(-10.0961244884418,67.0084911154305,
68.691687827272));
#123453=CARTESIAN_POINT('Ctrl Pts',(-13.4857787351653,83.53086080835,69.194683933252));
#123454=CARTESIAN_POINT('Ctrl Pts',(-13.4107459268847,82.33835458422,66.513462598172));
#123455=CARTESIAN_POINT('Ctrl Pts',(-13.2981967144638,78.53320802489,63.458709829566));
#123456=CARTESIAN_POINT('Ctrl Pts',(-13.1481310979025,72.48811911993,63.63322643035));
#123457=CARTESIAN_POINT('Ctrl Pts',(-13.0355818854816,68.51429278678,65.790797832361));
#123458=CARTESIAN_POINT('Ctrl Pts',(-12.9230326730606,65.95227475056,69.522686716285));
#123459=CARTESIAN_POINT('Ctrl Pts',(-12.8104834606397,65.36509547432,74.009771845382));
#123460=CARTESIAN_POINT('Ctrl Pts',(-12.6979342482187,66.87977327092,78.274405364341));
#123461=CARTESIAN_POINT('Ctrl Pts',(-12.5853850357977,70.16613638824,81.385801227635));
#123462=CARTESIAN_POINT('Ctrl Pts',(-12.4728358233767,74.50710712086,82.665227893767));
#123463=CARTESIAN_POINT('Ctrl Pts',(-12.3602866109557,78.95561877133,81.83352216413));
#123464=CARTESIAN_POINT('Ctrl Pts',(-12.2477373985346,82.54111542822,79.072147533527));
#123465=CARTESIAN_POINT('Ctrl Pts',(-12.1351881861136,84.48133587032,74.983562774911));
#123466=CARTESIAN_POINT('Ctrl Pts',(-12.0226389736926,84.35297372718,70.459791926131));
#123467=CARTESIAN_POINT('Ctrl Pts',(-11.9100897612715,82.18403440969,66.487804766612));
#123468=CARTESIAN_POINT('Ctrl Pts',(-11.7975405488505,78.44772440513,63.934186298037));
#123469=CARTESIAN_POINT('Ctrl Pts',(-11.6849913364294,73.95921002211,63.356070078148));
#123470=CARTESIAN_POINT('Ctrl Pts',(-11.5724421240084,69.69776911955,64.879586131319));
#123471=CARTESIAN_POINT('Ctrl Pts',(-11.4598929115869,66.59313798963,68.172342617968));
#123472=CARTESIAN_POINT('Ctrl Pts',(-11.3473436991659,65.32266693424,72.5159451614496));
#123473=CARTESIAN_POINT('Ctrl Pts',(-11.2347944867449,66.16353987442,76.962731892397));
#123474=CARTESIAN_POINT('Ctrl Pts',(-11.1222452743239,68.93230019525,80.542528950631));
#123475=CARTESIAN_POINT('Ctrl Pts',(-11.0096960619029,73.02487543835,82.474316725385));
#123476=CARTESIAN_POINT('Ctrl Pts',(-10.8971468494819,77.5483732915,82.336630496769));
#123477=CARTESIAN_POINT('Ctrl Pts',(-10.7845976370609,81.5158764696,80.159504403197));
#123478=CARTESIAN_POINT('Ctrl Pts',(-10.6720484246399,84.06180417873,76.417951402524));
#123479=CARTESIAN_POINT('Ctrl Pts',(-10.5594992122189,84.63060417684,71.928205926366));
#123480=CARTESIAN_POINT('Ctrl Pts',(-10.4469499997979,83.09853951678,67.670097151854));
#123481=CARTESIAN_POINT('Ctrl Pts',(-10.3344007873769,79.79852165914,64.571579248221));
#123482=CARTESIAN_POINT('Ctrl Pts',(-10.2218515749559,75.45555056223,63.312606598678));
#123483=CARTESIAN_POINT('Ctrl Pts',(-10.0717859583949,69.51269706816,64.433342187813));
#123484=CARTESIAN_POINT('Ctrl Pts',(-9.95923674597391,66.44785978885,68.230370929682));
#123485=CARTESIAN_POINT('Ctrl Pts',(-9.88420393769391,65.8555809379,71.104431594487));
#123486=CARTESIAN_POINT('Ctrl Pts',(-13.7163617470419,83.16594445251,69.356984978657));
#123487=CARTESIAN_POINT('Ctrl Pts',(-13.6413289387609,82.02444891012,66.790455647208));
#123488=CARTESIAN_POINT('Ctrl Pts',(-13.5287797263401,78.38207141327,63.866373073948));
#123489=CARTESIAN_POINT('Ctrl Pts',(-13.3787141097789,72.59556741124,64.033424547414));
#123490=CARTESIAN_POINT('Ctrl Pts',(-13.2661648973579,68.79172559158,66.09870361091));
#123491=CARTESIAN_POINT('Ctrl Pts',(-13.153615684937,66.33930051512,69.670957104856));
#123492=CARTESIAN_POINT('Ctrl Pts',(-13.041066472516,65.77723843707,73.9661025469177));
#123493=CARTESIAN_POINT('Ctrl Pts',(-12.928517260095,67.22712433115,78.048311975543));
#123494=CARTESIAN_POINT('Ctrl Pts',(-12.815968047674,70.37290988194,81.026614676792));
#123495=CARTESIAN_POINT('Ctrl Pts',(-12.703418835253,74.5281911213,82.251312549785));
#123496=CARTESIAN_POINT('Ctrl Pts',(-12.590869622832,78.78641310501,81.455183889208));
#123497=CARTESIAN_POINT('Ctrl Pts',(-12.478320410411,82.2185364502,78.811929902003));
#123498=CARTESIAN_POINT('Ctrl Pts',(-12.3657711979899,84.07576196493,74.898238566719));
#123499=CARTESIAN_POINT('Ctrl Pts',(-12.2532219855689,83.95289064466,70.567976674408));
#123500=CARTESIAN_POINT('Ctrl Pts',(-12.1406727731479,81.87672993999,66.765895355836));
#123501=CARTESIAN_POINT('Ctrl Pts',(-12.0281235607268,78.3002444434,64.321510546861));
#123502=CARTESIAN_POINT('Ctrl Pts',(-11.9155743483058,74.00373088522,63.768123843582));
#123503=CARTESIAN_POINT('Ctrl Pts',(-11.8030251358847,69.92457750553,65.2264699287));
#123504=CARTESIAN_POINT('Ctrl Pts',(-11.6904759234637,66.95275016922,68.378375365861));
#123505=CARTESIAN_POINT('Ctrl Pts',(-11.5779267110427,65.73662482149,72.5361758376591));
#123506=CARTESIAN_POINT('Ctrl Pts',(-11.4653774986219,66.54152855574,76.792746687058));
#123507=CARTESIAN_POINT('Ctrl Pts',(-11.3528282862009,69.19185230266,80.219414239796));
#123508=CARTESIAN_POINT('Ctrl Pts',(-11.2402790737799,73.10936342534,82.068567803219));
#123509=CARTESIAN_POINT('Ctrl Pts',(-11.1277298613589,77.4393639997,81.936771244833));
#123510=CARTESIAN_POINT('Ctrl Pts',(-11.0151806489379,81.23715314378,79.852773961851));
#123511=CARTESIAN_POINT('Ctrl Pts',(-10.9026314365169,83.67417617347,76.271269743701));
#123512=CARTESIAN_POINT('Ctrl Pts',(-10.7900822240959,84.21864516594,71.973577753657));
#123513=CARTESIAN_POINT('Ctrl Pts',(-10.6775330116749,82.75211614938,67.897613966809));
#123514=CARTESIAN_POINT('Ctrl Pts',(-10.5649837992539,79.59325995385,64.931638357232));
#123515=CARTESIAN_POINT('Ctrl Pts',(-10.4524345868329,75.43606391784,63.726519559207));
#123516=CARTESIAN_POINT('Ctrl Pts',(-10.3023689702719,69.7474221017,64.799314529419));
#123517=CARTESIAN_POINT('Ctrl Pts',(-10.1898197578509,66.81368639306,68.433921456821));
#123518=CARTESIAN_POINT('Ctrl Pts',(-10.1147869495699,66.24674287986,71.185041217093));
#123519=CARTESIAN_POINT('Ctrl Pts',(-13.9469447589179,82.80102809666,69.519286024043));
#123520=CARTESIAN_POINT('Ctrl Pts',(-13.8719119506369,81.710543236,67.067448696223));
#123521=CARTESIAN_POINT('Ctrl Pts',(-13.7593627382169,78.23093480162,64.274036318316));
#123522=CARTESIAN_POINT('Ctrl Pts',(-13.6092971216549,72.7030157025,64.433622664488));
#123523=CARTESIAN_POINT('Ctrl Pts',(-13.4967479092343,69.06915839634,66.406609389489));
#123524=CARTESIAN_POINT('Ctrl Pts',(-13.3841986968133,66.72632627966,69.819227493478));
#123525=CARTESIAN_POINT('Ctrl Pts',(-13.2716494843923,66.18938139983,73.9224332485153));
#123526=CARTESIAN_POINT('Ctrl Pts',(-13.1591002719714,67.57447539142,77.822218586803));
#123527=CARTESIAN_POINT('Ctrl Pts',(-13.0465510595504,70.57968337571,80.667428125987));
#123528=CARTESIAN_POINT('Ctrl Pts',(-12.9340018471294,74.54927512182,81.837397205809));
#123529=CARTESIAN_POINT('Ctrl Pts',(-12.8214526347083,78.61720743877,81.076845614251));
#123530=CARTESIAN_POINT('Ctrl Pts',(-12.7089034222873,81.89595747223,78.551712270407));
#123531=CARTESIAN_POINT('Ctrl Pts',(-12.5963542098663,83.67018805956,74.812914358431));
#123532=CARTESIAN_POINT('Ctrl Pts',(-12.4838049974453,83.55280756212,70.676161422585));
#123533=CARTESIAN_POINT('Ctrl Pts',(-12.3712557850242,81.56942547021,67.043985944979));
#123534=CARTESIAN_POINT('Ctrl Pts',(-12.2587065726032,78.15276448156,64.708834795646));
#123535=CARTESIAN_POINT('Ctrl Pts',(-12.1461573601821,74.04825174822,64.180177609028));
#123536=CARTESIAN_POINT('Ctrl Pts',(-12.0336081477611,70.15138589142,65.573353726144));
#123537=CARTESIAN_POINT('Ctrl Pts',(-11.92105893534,67.31236234875,68.584408113854));
#123538=CARTESIAN_POINT('Ctrl Pts',(-11.808509722919,66.15058270873,72.5564065139833));
#123539=CARTESIAN_POINT('Ctrl Pts',(-11.695960510498,66.9195172371,76.622761481822));
#123540=CARTESIAN_POINT('Ctrl Pts',(-11.5834112980769,69.45140441015,79.89629952903));
#123541=CARTESIAN_POINT('Ctrl Pts',(-11.4708620856559,73.19385141245,81.662818881074));
#123542=CARTESIAN_POINT('Ctrl Pts',(-11.3583128732349,77.330354708,81.53691199287));
#123543=CARTESIAN_POINT('Ctrl Pts',(-11.2457636608139,80.95842981803,79.54604352044));
#123544=CARTESIAN_POINT('Ctrl Pts',(-11.1332144483929,83.28654816823,76.124588084795));
#123545=CARTESIAN_POINT('Ctrl Pts',(-11.0206652359719,83.80668615503,72.0189495808697));
#123546=CARTESIAN_POINT('Ctrl Pts',(-10.9081160235509,82.40569278195,68.125130781709));
#123547=CARTESIAN_POINT('Ctrl Pts',(-10.7955668111299,79.38799824851,65.291697466218));
#123548=CARTESIAN_POINT('Ctrl Pts',(-10.6830175987089,75.4165772734,64.140432519737));
#123549=CARTESIAN_POINT('Ctrl Pts',(-10.5329519821479,69.98214713522,65.165286871043));
#123550=CARTESIAN_POINT('Ctrl Pts',(-10.4204027697269,67.17951299727,68.637471983962));
#123551=CARTESIAN_POINT('Ctrl Pts',(-10.3453699614459,66.63790482183,71.265650839687));
#123552=CARTESIAN_POINT('Ctrl Pts',(-14.1775277707939,82.43611174083,69.681587069447));
#123553=CARTESIAN_POINT('Ctrl Pts',(-14.1024949625139,81.3966375619,67.344441745258));
#123554=CARTESIAN_POINT('Ctrl Pts',(-13.9899457500929,78.07979819,64.681699562697));
#123555=CARTESIAN_POINT('Ctrl Pts',(-13.8398801335319,72.8104639938,64.833820781552));
#123556=CARTESIAN_POINT('Ctrl Pts',(-13.7273309211109,69.34659120114,66.714515168039));
#123557=CARTESIAN_POINT('Ctrl Pts',(-13.6147817086899,67.11335204423,69.967497882051));
#123558=CARTESIAN_POINT('Ctrl Pts',(-13.5022324962687,66.60152436258,73.878763950054));
#123559=CARTESIAN_POINT('Ctrl Pts',(-13.3896832838477,67.92182645165,77.596125198008));
#123560=CARTESIAN_POINT('Ctrl Pts',(-13.2771340714267,70.78645686942,80.308241575145));
#123561=CARTESIAN_POINT('Ctrl Pts',(-13.1645848590057,74.57035912226,81.423481861828));
#123562=CARTESIAN_POINT('Ctrl Pts',(-13.0520356465847,78.44800177245,80.698507339327));
#123563=CARTESIAN_POINT('Ctrl Pts',(-12.9394864341637,81.57337849421,78.29149463888));
#123564=CARTESIAN_POINT('Ctrl Pts',(-12.8269372217426,83.26461415418,74.727590150234));
#123565=CARTESIAN_POINT('Ctrl Pts',(-12.7143880093216,83.1527244796,70.784346170858));
#123566=CARTESIAN_POINT('Ctrl Pts',(-12.6018387969006,81.26212100051,67.322076534199));
#123567=CARTESIAN_POINT('Ctrl Pts',(-12.4892895844795,78.00528451983,65.096159044468));
#123568=CARTESIAN_POINT('Ctrl Pts',(-12.3767403720585,74.09277261133,64.592231374463));
#123569=CARTESIAN_POINT('Ctrl Pts',(-12.2641911596374,70.37819427741,65.920237523529));
#123570=CARTESIAN_POINT('Ctrl Pts',(-12.1516419472164,67.67197452834,68.790440861752));
#123571=CARTESIAN_POINT('Ctrl Pts',(-12.0390927347954,66.56454059598,72.5766371901982));
#123572=CARTESIAN_POINT('Ctrl Pts',(-11.9265435223743,67.29750591841,76.452776276488));
#123573=CARTESIAN_POINT('Ctrl Pts',(-11.8139943099533,69.71095651757,79.573184818198));
#123574=CARTESIAN_POINT('Ctrl Pts',(-11.7014450975323,73.27833939945,81.257069958908));
#123575=CARTESIAN_POINT('Ctrl Pts',(-11.5888958851113,77.22134541621,81.137052740933));
#123576=CARTESIAN_POINT('Ctrl Pts',(-11.4763466726899,80.67970649221,79.239313079091));
#123577=CARTESIAN_POINT('Ctrl Pts',(-11.3637974602689,82.89892016296,75.977906425967));
#123578=CARTESIAN_POINT('Ctrl Pts',(-11.2512482478479,83.39472714413,72.0643214081573));
#123579=CARTESIAN_POINT('Ctrl Pts',(-11.1386990354269,82.05926941456,68.352647596662));
#123580=CARTESIAN_POINT('Ctrl Pts',(-11.0261498230059,79.18273654321,65.651756575228));
#123581=CARTESIAN_POINT('Ctrl Pts',(-10.9136006105849,75.39709062901,64.554345480267));
#123582=CARTESIAN_POINT('Ctrl Pts',(-10.7635349940239,70.21687216876,65.53125921265));
#123583=CARTESIAN_POINT('Ctrl Pts',(-10.6509857816029,67.54533960148,68.841022511101));
#123584=CARTESIAN_POINT('Ctrl Pts',(-10.5759529733229,67.02906676379,71.346260462292));
#123585=CARTESIAN_POINT('Ctrl Pts',(-13.5675364833309,80.6475155947738,
66.0116637084142));
#123586=CARTESIAN_POINT('Ctrl Pts',(-13.5675364833309,80.8673931721485,
66.1731545541286));
#123587=CARTESIAN_POINT('Ctrl Pts',(-13.5675364833309,81.0802488986569,
66.3442606841591));
#123588=CARTESIAN_POINT('Ctrl Pts',(-13.5675364833309,81.4923702907423,
66.7063307057292));
#123589=CARTESIAN_POINT('Ctrl Pts',(-13.5675364833309,81.6915016168863,
66.8975231489235));
#123590=CARTESIAN_POINT('Ctrl Pts',(-13.5675364833309,81.881676986561,67.0972279350825));
#123591=CARTESIAN_POINT('Origin',(-13.5675364833309,75.,72.98888938658));
#123592=CARTESIAN_POINT('Origin',(-15.5675364832709,-75.,72.98888938658));
#123593=CARTESIAN_POINT('',(-15.5675364832709,-81.062177826491,72.98888938658));
#123594=CARTESIAN_POINT('',(-15.5675364832709,-78.0310889132455,78.23888938658));
#123595=CARTESIAN_POINT('',(-15.5675364832709,-78.0310889132455,78.23888938658));
#123596=CARTESIAN_POINT('',(-15.5675364832709,-71.9689110867544,78.23888938658));
#123597=CARTESIAN_POINT('',(-15.5675364832709,-71.9689110867544,78.23888938658));
#123598=CARTESIAN_POINT('',(-15.5675364832709,-68.9378221735089,72.98888938658));
#123599=CARTESIAN_POINT('',(-15.5675364832709,-68.9378221735089,72.98888938658));
#123600=CARTESIAN_POINT('',(-15.5675364832709,-71.9689110867545,67.73888938658));
#123601=CARTESIAN_POINT('',(-15.5675364832709,-71.9689110867545,67.73888938658));
#123602=CARTESIAN_POINT('',(-15.5675364832709,-78.0310889132455,67.73888938658));
#123603=CARTESIAN_POINT('',(-15.5675364832709,-78.0310889132455,67.73888938658));
#123604=CARTESIAN_POINT('',(-15.5675364832709,-81.062177826491,72.98888938658));
#123605=CARTESIAN_POINT('Origin',(-25.5675364832709,-78.0310889132455,78.23888938658));
#123606=CARTESIAN_POINT('',(-25.5675364832709,-81.062177826491,72.98888938658));
#123607=CARTESIAN_POINT('',(-25.5675364832709,-78.0310889132455,78.23888938658));
#123608=CARTESIAN_POINT('Origin',(-25.5675364832709,-71.9689110867544,78.23888938658));
#123609=CARTESIAN_POINT('',(-25.5675364832709,-71.9689110867544,78.23888938658));
#123610=CARTESIAN_POINT('Origin',(-25.5675364832709,-68.9378221735089,72.98888938658));
#123611=CARTESIAN_POINT('',(-25.5675364832709,-68.9378221735089,72.98888938658));
#123612=CARTESIAN_POINT('Origin',(-25.5675364832709,-71.9689110867545,67.73888938658));
#123613=CARTESIAN_POINT('',(-25.5675364832709,-71.9689110867545,67.73888938658));
#123614=CARTESIAN_POINT('Origin',(-25.5675364832709,-78.0310889132455,67.73888938658));
#123615=CARTESIAN_POINT('',(-25.5675364832709,-78.0310889132455,67.73888938658));
#123616=CARTESIAN_POINT('Origin',(-25.5675364832709,-81.062177826491,72.98888938658));
#123617=CARTESIAN_POINT('Origin',(-18.5675364832709,-75.,72.98888938658));
#123618=CARTESIAN_POINT('Origin',(-20.5675364832709,-75.,72.98888938658));
#123619=CARTESIAN_POINT('Ctrl Pts',(11.7737028196091,-21.80503453548,82.974463848657));
#123620=CARTESIAN_POINT('Ctrl Pts',(11.7842119497491,-21.8209908852,82.976752059407));
#123621=CARTESIAN_POINT('Ctrl Pts',(11.9074330236891,-22.0118587646,83.00150321689));
#123622=CARTESIAN_POINT('Ctrl Pts',(12.1327094234791,-22.44912871337,82.99331681448));
#123623=CARTESIAN_POINT('Ctrl Pts',(12.3872208177991,-23.19361457716,82.796143394484));
#123624=CARTESIAN_POINT('Ctrl Pts',(12.4980497482091,-23.77070951624,82.495844470338));
#123625=CARTESIAN_POINT('Ctrl Pts',(12.5268844558191,-24.09442226678,82.2737301581291));
#123626=CARTESIAN_POINT('Ctrl Pts',(12.5306001626891,-24.14726018536,82.236125320949));
#123627=CARTESIAN_POINT('Ctrl Pts',(11.8797038575791,-21.71767911338,82.436822495267));
#123628=CARTESIAN_POINT('Ctrl Pts',(11.8865435901191,-21.73097889939,82.438814682516));
#123629=CARTESIAN_POINT('Ctrl Pts',(11.9662971783691,-21.8903986298,82.4607304615951));
#123630=CARTESIAN_POINT('Ctrl Pts',(12.1018554065891,-22.26337977053,82.463312214956));
#123631=CARTESIAN_POINT('Ctrl Pts',(12.2277242566991,-22.91758315467,82.330367392035));
#123632=CARTESIAN_POINT('Ctrl Pts',(12.2549645866691,-23.44051817093,82.115603938798));
#123633=CARTESIAN_POINT('Ctrl Pts',(12.2436931578091,-23.7395527805,81.954214255122));
#123634=CARTESIAN_POINT('Ctrl Pts',(12.2410774442991,-23.78850636215,81.926839572217));
#123635=CARTESIAN_POINT('Ctrl Pts',(12.2573963950691,-21.44250482709,82.137598971116));
#123636=CARTESIAN_POINT('Ctrl Pts',(12.2635341762291,-21.45619889632,82.1383257760441));
#123637=CARTESIAN_POINT('Ctrl Pts',(12.3343464866891,-21.61991088389,82.1449108583021));
#123638=CARTESIAN_POINT('Ctrl Pts',(12.4352004835491,-21.99123106393,82.109689603077));
#123639=CARTESIAN_POINT('Ctrl Pts',(12.4740260820391,-22.60719182595,81.935724156804));
#123640=CARTESIAN_POINT('Ctrl Pts',(12.4201268319991,-23.08268362029,81.721934479734));
#123641=CARTESIAN_POINT('Ctrl Pts',(12.3623316865191,-23.35150381325,81.575321364862));
#123642=CARTESIAN_POINT('Ctrl Pts',(12.3521581962191,-23.39540043164,81.550724432541));
#123643=CARTESIAN_POINT('Ctrl Pts',(12.7032417518891,-21.12780322461,82.238044969419));
#123644=CARTESIAN_POINT('Ctrl Pts',(12.7120233098291,-21.14472994457,82.237218948315));
#123645=CARTESIAN_POINT('Ctrl Pts',(12.8132390090491,-21.34616149612,82.224239734821));
#123646=CARTESIAN_POINT('Ctrl Pts',(12.9531048408191,-21.77934365529,82.123016365173));
#123647=CARTESIAN_POINT('Ctrl Pts',(12.9933941281391,-22.42971061916,81.824887107694));
#123648=CARTESIAN_POINT('Ctrl Pts',(12.9045304751091,-22.89004306637,81.526984743628));
#123649=CARTESIAN_POINT('Ctrl Pts',(12.8188656848891,-23.13939512993,81.341237038185));
#123650=CARTESIAN_POINT('Ctrl Pts',(12.8039809507391,-23.17978735852,81.310468521703));
#123651=CARTESIAN_POINT('',(11.9367309803807,-21.8592780094232,82.7099370787206));
#123652=CARTESIAN_POINT('',(12.6211149266398,-23.1949866874293,81.5466536447308));
#123653=CARTESIAN_POINT('Ctrl Pts',(11.9367361538315,-21.8592750801367,
82.7099405001105));
#123654=CARTESIAN_POINT('Ctrl Pts',(11.9622030980227,-21.8915999880229,
82.6991156916996));
#123655=CARTESIAN_POINT('Ctrl Pts',(11.9881073830353,-21.9253909044623,
82.686248515633));
#123656=CARTESIAN_POINT('Ctrl Pts',(12.0142120213475,-21.96058406732,82.6711822410034));
#123657=CARTESIAN_POINT('Ctrl Pts',(12.0397543732084,-21.9950191795043,
82.6564404896249));
#123658=CARTESIAN_POINT('Ctrl Pts',(12.0654879223436,-22.0307968926114,
82.6395928765279));
#123659=CARTESIAN_POINT('Ctrl Pts',(12.091184141745,-22.0678087196869,82.6204972631129));
#123660=CARTESIAN_POINT('Ctrl Pts',(12.111834171334,-22.0975522127786,82.6051516211771));
#123661=CARTESIAN_POINT('Ctrl Pts',(12.1324598146958,-22.1280917768807,
82.5883541804234));
#123662=CARTESIAN_POINT('Ctrl Pts',(12.1529436620966,-22.159347265805,82.5700366962959));
#123663=CARTESIAN_POINT('Ctrl Pts',(12.1778034947841,-22.1972798968201,
82.5478060292853));
#123664=CARTESIAN_POINT('Ctrl Pts',(12.202453650089,-22.2362680889833,82.5233356680296));
#123665=CARTESIAN_POINT('Ctrl Pts',(12.2266946108567,-22.2761267814906,
82.496519371568));
#123666=CARTESIAN_POINT('Ctrl Pts',(12.2375690653905,-22.2940073244114,
82.4844896257411));
#123667=CARTESIAN_POINT('Ctrl Pts',(12.2483613802324,-22.3120624442134,
82.4719880522356));
#123668=CARTESIAN_POINT('Ctrl Pts',(12.2590548093192,-22.3302726084963,
82.4590065396343));
#123669=CARTESIAN_POINT('Ctrl Pts',(12.2656381470914,-22.3414835737899,
82.4510145586191));
#123670=CARTESIAN_POINT('Ctrl Pts',(12.2721840230251,-22.3527532703367,
82.4428406920455));
#123671=CARTESIAN_POINT('Ctrl Pts',(12.2786887204933,-22.364076830813,82.4344832478605));
#123672=CARTESIAN_POINT('Ctrl Pts',(12.2892432084479,-22.3824503805796,
82.4209225028125));
#123673=CARTESIAN_POINT('Ctrl Pts',(12.2996892145748,-22.4009658161235,
82.4068783698921));
#123674=CARTESIAN_POINT('Ctrl Pts',(12.3100118138469,-22.4196011341924,
82.3923445214752));
#123675=CARTESIAN_POINT('Ctrl Pts',(12.3183540060871,-22.4346612369525,
82.3805990149134));
#123676=CARTESIAN_POINT('Ctrl Pts',(12.3266156437967,-22.4497997587411,
82.3685336671056));
#123677=CARTESIAN_POINT('Ctrl Pts',(12.3347894358396,-22.4650042051673,
82.3561457565399));
#123678=CARTESIAN_POINT('Ctrl Pts',(12.3398113417301,-22.4743456832313,
82.3485347333192));
#123679=CARTESIAN_POINT('Ctrl Pts',(12.3446189812725,-22.4833743225494,
82.3410841813665));
#123680=CARTESIAN_POINT('Ctrl Pts',(12.3495471969363,-22.4927104514669,
82.3332749532429));
#123681=CARTESIAN_POINT('Ctrl Pts',(12.3526402805277,-22.4985700625578,
82.3283736670537));
#123682=CARTESIAN_POINT('Ctrl Pts',(12.3557800676704,-22.504550607999,82.3233305968092));
#123683=CARTESIAN_POINT('Ctrl Pts',(12.3590406769578,-22.5108028429602,
82.3180120668465));
#123684=CARTESIAN_POINT('Ctrl Pts',(12.3824229780028,-22.5556385246324,
82.2798721188351));
#123685=CARTESIAN_POINT('Ctrl Pts',(12.4041003709132,-22.5998921737425,
82.240400081111));
#123686=CARTESIAN_POINT('Ctrl Pts',(12.4241951999649,-22.6433365148074,
82.1997161277026));
#123687=CARTESIAN_POINT('Ctrl Pts',(12.4446093426681,-22.6874712011915,
82.1583856924713));
#123688=CARTESIAN_POINT('Ctrl Pts',(12.4633908163091,-22.7307703672997,
82.1158049661513));
#123689=CARTESIAN_POINT('Ctrl Pts',(12.4806936617776,-22.773042052157,82.0721100489682));
#123690=CARTESIAN_POINT('Ctrl Pts',(12.4984950964185,-22.8165318143765,
82.0271560433517));
#123691=CARTESIAN_POINT('Ctrl Pts',(12.5147320846937,-22.8589338308361,
81.9810231648695));
#123692=CARTESIAN_POINT('Ctrl Pts',(12.5295900954036,-22.900091637856,81.9338632672124));
#123693=CARTESIAN_POINT('Ctrl Pts',(12.5447043782732,-22.9419593380302,
81.8858899518606));
#123694=CARTESIAN_POINT('Ctrl Pts',(12.5583923685859,-22.982539647835,81.8368543167831));
#123695=CARTESIAN_POINT('Ctrl Pts',(12.5708573524237,-23.0217220410528,
81.7869130407606));
#123696=CARTESIAN_POINT('Ctrl Pts',(12.5836915758153,-23.0620651007883,
81.7354923970383));
#123697=CARTESIAN_POINT('Ctrl Pts',(12.595229903226,-23.1009263988723,81.6831120651281));
#123698=CARTESIAN_POINT('Ctrl Pts',(12.6056925681694,-23.1382400019589,
81.6299332280271));
#123699=CARTESIAN_POINT('Ctrl Pts',(12.6111132368744,-23.1575720441887,
81.6023814656797));
#123700=CARTESIAN_POINT('Ctrl Pts',(12.6162450821,-23.1764895136934,81.5746151666791));
#123701=CARTESIAN_POINT('Ctrl Pts',(12.6211177605568,-23.194988395035,81.5466552684072));
#123702=CARTESIAN_POINT('',(12.5172257454391,-21.43204530223,82.22390472213));
#123703=CARTESIAN_POINT('Ctrl Pts',(11.9367208753803,-21.8592837299615,
82.7099303959673));
#123704=CARTESIAN_POINT('Ctrl Pts',(11.9491160482679,-21.848141643132,82.6816498425584));
#123705=CARTESIAN_POINT('Ctrl Pts',(11.9628731595236,-21.8361810914248,
82.6538570180536));
#123706=CARTESIAN_POINT('Ctrl Pts',(11.9779676352564,-21.8234463126838,
82.6268031589723));
#123707=CARTESIAN_POINT('Ctrl Pts',(11.9928703653537,-21.8108733042677,
82.6000929659777));
#123708=CARTESIAN_POINT('Ctrl Pts',(12.0090767055389,-21.7975457050617,
82.5741039294356));
#123709=CARTESIAN_POINT('Ctrl Pts',(12.0265202200287,-21.7835329478403,
82.5490727877408));
#123710=CARTESIAN_POINT('Ctrl Pts',(12.0438587432357,-21.7696045324158,
82.5241923067215));
#123711=CARTESIAN_POINT('Ctrl Pts',(12.0624194312919,-21.7549993785506,
82.5002590484555));
#123712=CARTESIAN_POINT('Ctrl Pts',(12.0820955779931,-21.7398102759138,
82.4774879979392));
#123713=CARTESIAN_POINT('Ctrl Pts',(12.1016867174577,-21.7246867950505,
82.4548153256321));
#123714=CARTESIAN_POINT('Ctrl Pts',(12.1223833406148,-21.7089847118948,
82.433295570755));
#123715=CARTESIAN_POINT('Ctrl Pts',(12.1440427643665,-21.6928162797401,
82.413111864013));
#123716=CARTESIAN_POINT('Ctrl Pts',(12.1544146354514,-21.6850738348868,
82.4034466574616));
#123717=CARTESIAN_POINT('Ctrl Pts',(12.165006766415,-21.6772247283014,82.3940873195626));
#123718=CARTESIAN_POINT('Ctrl Pts',(12.175800879479,-21.6692826127025,82.3850508899748));
#123719=CARTESIAN_POINT('Ctrl Pts',(12.1983165878219,-21.6527159566566,
82.3662015772193));
#123720=CARTESIAN_POINT('Ctrl Pts',(12.221712471054,-21.6357439101918,82.3487602726554));
#123721=CARTESIAN_POINT('Ctrl Pts',(12.2458031684748,-21.6184980794134,
82.3328492103853));
#123722=CARTESIAN_POINT('Ctrl Pts',(12.2700378782506,-21.6011491543716,
82.3168430329964));
#123723=CARTESIAN_POINT('Ctrl Pts',(12.2949750489175,-21.5835236405448,
82.3023857528171));
#123724=CARTESIAN_POINT('Ctrl Pts',(12.3204084032296,-21.5657611169978,
82.289552276764));
#123725=CARTESIAN_POINT('Ctrl Pts',(12.3459603671866,-21.5479157570861,
82.2766589511913));
#123726=CARTESIAN_POINT('Ctrl Pts',(12.3720124086933,-21.5299325919223,
82.2654046417675));
#123727=CARTESIAN_POINT('Ctrl Pts',(12.3983485415761,-21.5119514677974,
82.2558129175903));
#123728=CARTESIAN_POINT('Ctrl Pts',(12.4249913690804,-21.4937609464128,
82.2461094940141));
#123729=CARTESIAN_POINT('Ctrl Pts',(12.4519242002296,-21.4755729740054,
82.2381074290571));
#123730=CARTESIAN_POINT('Ctrl Pts',(12.4789278146413,-21.4575233831369,
82.2317786261044));
#123731=CARTESIAN_POINT('Ctrl Pts',(12.4916861066886,-21.4489955635597,
82.2287884813353));
#123732=CARTESIAN_POINT('Ctrl Pts',(12.5044603332855,-21.4404984616105,
82.2261711119611));
#123733=CARTESIAN_POINT('Ctrl Pts',(12.5172284057885,-21.4320453006202,
82.2239198161667));
#123734=CARTESIAN_POINT('Ctrl Pts',(12.5172257454391,-21.43204530223,82.22390472213));
#123735=CARTESIAN_POINT('Ctrl Pts',(12.6340357992967,-21.713678275013,82.2033623527417));
#123736=CARTESIAN_POINT('Ctrl Pts',(12.692894450305,-22.0223140153352,82.1188254444615));
#123737=CARTESIAN_POINT('Ctrl Pts',(12.7189823415742,-22.623367521142,81.8782087798771));
#123738=CARTESIAN_POINT('Ctrl Pts',(12.6874951393621,-22.9152905983023,
81.7236169057246));
#123739=CARTESIAN_POINT('Ctrl Pts',(12.6211129829291,-23.19498551621,81.546652531098));
#123740=CARTESIAN_POINT('Origin',(18.2606283043191,-15.,57.49100545192));
#123741=CARTESIAN_POINT('',(19.1777592571107,-16.3235270075928,58.627271032273));
#123742=CARTESIAN_POINT('',(20.4074538435026,-16.3235291382987,65.6012398999359));
#123743=CARTESIAN_POINT('',(19.1777552349091,-16.32352916975,58.62727005114));
#123744=CARTESIAN_POINT('',(21.1895064189377,-15.0000003990606,65.4633429305542));
#123745=CARTESIAN_POINT('Origin',(19.7122947894255,-15.,65.7238151970535));
#123746=CARTESIAN_POINT('',(19.9598072782762,-15.0000003739637,58.4893725505111));
#123747=CARTESIAN_POINT('',(19.9598072256691,-15.00000060839,58.48937225217));
#123748=CARTESIAN_POINT('Origin',(18.4825957015691,-15.,58.74984511652));
#123749=CARTESIAN_POINT('Ctrl Pts',(12.5199362278991,-23.49480870114,81.306473853632));
#123750=CARTESIAN_POINT('Ctrl Pts',(12.3430034024391,-23.49480870114,81.620480433794));
#123751=CARTESIAN_POINT('Ctrl Pts',(11.9272160718391,-23.49480870114,82.318177658235));
#123752=CARTESIAN_POINT('Ctrl Pts',(11.2242863296091,-23.49480870114,83.3524350127001));
#123753=CARTESIAN_POINT('Ctrl Pts',(10.4115975050891,-23.49480870114,84.38086299568));
#123754=CARTESIAN_POINT('Ctrl Pts',(9.55586525979908,-23.49480870114,85.31060223946));
#123755=CARTESIAN_POINT('Ctrl Pts',(8.6576193448791,-23.49480870114,86.1471009819601));
#123756=CARTESIAN_POINT('Ctrl Pts',(7.70893043203909,-23.49480870114,86.90213314277));
#123757=CARTESIAN_POINT('Ctrl Pts',(6.71139644797909,-23.49480870114,87.57700589972));
#123758=CARTESIAN_POINT('Ctrl Pts',(5.68377226408909,-23.49480870114,88.16713174316));
#123759=CARTESIAN_POINT('Ctrl Pts',(4.61844145667909,-23.49480870114,88.69058723386));
#123760=CARTESIAN_POINT('Ctrl Pts',(3.47639771609909,-23.49480870114,89.1742936871701));
#123761=CARTESIAN_POINT('Ctrl Pts',(2.24422019413909,-23.49480870114,89.62822366128));
#123762=CARTESIAN_POINT('Ctrl Pts',(1.38880489860909,-23.49480870114,89.9114551536101));
#123763=CARTESIAN_POINT('Ctrl Pts',(0.957537393149087,-23.49480870114,90.05047159017));
#123764=CARTESIAN_POINT('Ctrl Pts',(13.5266301189791,-22.19079082182,81.873739112569));
#123765=CARTESIAN_POINT('Ctrl Pts',(13.3404943832391,-22.19079082182,82.2040797061641));
#123766=CARTESIAN_POINT('Ctrl Pts',(12.9022454213091,-22.19079082182,82.939551587252));
#123767=CARTESIAN_POINT('Ctrl Pts',(12.1577492774591,-22.19079082182,84.03519946655));
#123768=CARTESIAN_POINT('Ctrl Pts',(11.2923354682991,-22.19079082182,85.13056199279));
#123769=CARTESIAN_POINT('Ctrl Pts',(10.3768252729191,-22.19079082182,86.12540154234));
#123770=CARTESIAN_POINT('Ctrl Pts',(9.4127272028091,-22.19079082182,87.0233027811901));
#123771=CARTESIAN_POINT('Ctrl Pts',(8.39331680038909,-22.19079082182,87.83461537407));
#123772=CARTESIAN_POINT('Ctrl Pts',(7.32308119035909,-22.19079082182,88.5585788914901));
#123773=CARTESIAN_POINT('Ctrl Pts',(6.22576052973909,-22.19079082182,89.18856810325));
#123774=CARTESIAN_POINT('Ctrl Pts',(5.09676735478909,-22.19079082182,89.74312289588));
#123775=CARTESIAN_POINT('Ctrl Pts',(3.89863512110909,-22.19079082182,90.2503735744501));
#123776=CARTESIAN_POINT('Ctrl Pts',(2.62244286138909,-22.19079082182,90.7203026262499));
#123777=CARTESIAN_POINT('Ctrl Pts',(1.74918245929909,-22.19079082182,91.0093591043299));
#123778=CARTESIAN_POINT('Ctrl Pts',(1.31205504332909,-22.19079082182,91.1502619594));
#123779=CARTESIAN_POINT('Ctrl Pts',(12.7677580370791,-20.68183777369,81.446119781757));
#123780=CARTESIAN_POINT('Ctrl Pts',(12.5885596948691,-20.68183777369,81.7641473704861));
#123781=CARTESIAN_POINT('Ctrl Pts',(12.1672428958191,-20.68183777369,82.471143731272));
#123782=CARTESIAN_POINT('Ctrl Pts',(11.4540805884091,-20.68183777369,83.5205138335801));
#123783=CARTESIAN_POINT('Ctrl Pts',(10.6284122462891,-20.68183777369,84.56541935731));
#123784=CARTESIAN_POINT('Ctrl Pts',(9.75796422704909,-20.68183777369,85.51118460035));
#123785=CARTESIAN_POINT('Ctrl Pts',(8.8435072271191,-20.68183777369,86.3627990377701));
#123786=CARTESIAN_POINT('Ctrl Pts',(7.87740852601909,-20.68183777369,87.13168597471));
#123787=CARTESIAN_POINT('Ctrl Pts',(6.86197729568909,-20.68183777369,87.81864359795));
#123788=CARTESIAN_POINT('Ctrl Pts',(5.81719565499909,-20.68183777369,88.41858276414));
#123789=CARTESIAN_POINT('Ctrl Pts',(4.73619283124909,-20.68183777369,88.9496940927601));
#123790=CARTESIAN_POINT('Ctrl Pts',(3.58034156490909,-20.68183777369,89.43919652094));
#123791=CARTESIAN_POINT('Ctrl Pts',(2.33732876120909,-20.68183777369,89.89706505117));
#123792=CARTESIAN_POINT('Ctrl Pts',(1.47752046534909,-20.68183777369,90.1817305032401));
#123793=CARTESIAN_POINT('Ctrl Pts',(1.04481040258909,-20.68183777369,90.3212113268901));
#123794=CARTESIAN_POINT('Ctrl Pts',(11.2805063366991,-21.03030703232,80.6080634188521));
#123795=CARTESIAN_POINT('Ctrl Pts',(11.1149040280891,-21.03030703232,80.9019597503359));
#123796=CARTESIAN_POINT('Ctrl Pts',(10.7267711985491,-21.03030703232,81.5531492538179));
#123797=CARTESIAN_POINT('Ctrl Pts',(10.0750175298891,-21.03030703232,82.511823303176));
#123798=CARTESIAN_POINT('Ctrl Pts',(9.32724309746908,-21.03030703232,83.4578422496101));
#123799=CARTESIAN_POINT('Ctrl Pts',(8.54510877389908,-21.03030703232,84.30743074885));
#123800=CARTESIAN_POINT('Ctrl Pts',(7.72793927182908,-21.03030703232,85.06833144705));
#123801=CARTESIAN_POINT('Ctrl Pts',(6.86632184011909,-21.03030703232,85.7540717899401));
#123802=CARTESIAN_POINT('Ctrl Pts',(5.95829725822909,-21.03030703232,86.3685045695999));
#123803=CARTESIAN_POINT('Ctrl Pts',(5.01648257150909,-21.03030703232,86.9095510944));
#123804=CARTESIAN_POINT('Ctrl Pts',(4.02953213566909,-21.03030703232,87.3947174837801));
#123805=CARTESIAN_POINT('Ctrl Pts',(2.95654389997909,-21.03030703232,87.84943655887));
#123806=CARTESIAN_POINT('Ctrl Pts',(1.77855681476909,-21.03030703232,88.2836686533401));
#123807=CARTESIAN_POINT('Ctrl Pts',(0.945112208319089,-21.03030703232,88.5597284904799));
#123808=CARTESIAN_POINT('Ctrl Pts',(0.521059356999088,-21.03030703232,88.6964223903801));
#123809=CARTESIAN_POINT('',(1.21025704777005,-22.7988943080295,90.3337993035096));
#123810=CARTESIAN_POINT('Ctrl Pts',(1.21023413007473,-22.798879208848,90.3337286710351));
#123811=CARTESIAN_POINT('Ctrl Pts',(1.51039343408459,-22.8242058549175,
90.2309309413167));
#123812=CARTESIAN_POINT('Ctrl Pts',(1.81144147252023,-22.8489329406032,
90.1251809362156));
#123813=CARTESIAN_POINT('Ctrl Pts',(2.11324772692397,-22.8729680300164,
90.0151018754575));
#123814=CARTESIAN_POINT('Ctrl Pts',(2.19524318765021,-22.8794979418431,
89.9851953272284));
#123815=CARTESIAN_POINT('Ctrl Pts',(2.27729447866082,-22.8859768914643,
89.9549690246212));
#123816=CARTESIAN_POINT('Ctrl Pts',(2.35939866739142,-22.8924032818193,
89.9243947585409));
#123817=CARTESIAN_POINT('Ctrl Pts',(2.61750826452643,-22.9126058202183,
89.8282789376222));
#123818=CARTESIAN_POINT('Ctrl Pts',(2.87614185551581,-22.9322881533364,
89.7287273974561));
#123819=CARTESIAN_POINT('Ctrl Pts',(3.13505901007745,-22.9514075662278,
89.6248336129083));
#123820=CARTESIAN_POINT('Ctrl Pts',(3.29875079872078,-22.9634951812772,
89.5591502113957));
#123821=CARTESIAN_POINT('Ctrl Pts',(3.46255562440981,-22.9753580097105,
89.4917304938924));
#123822=CARTESIAN_POINT('Ctrl Pts',(3.62640905193442,-22.9869873315234,
89.422335216172));
#123823=CARTESIAN_POINT('Ctrl Pts',(3.86411883991196,-23.0038585295461,
89.3216602592743));
#123824=CARTESIAN_POINT('Ctrl Pts',(4.10193181500926,-23.0202380107857,
89.216829570639));
#123825=CARTESIAN_POINT('Ctrl Pts',(4.33950678287984,-23.0361047359754,
89.1071648584239));
#123826=CARTESIAN_POINT('Ctrl Pts',(4.41586782947864,-23.0412045987785,
89.0719165649073));
#123827=CARTESIAN_POINT('Ctrl Pts',(4.49220414898786,-23.0462515375288,
89.0361685057209));
#123828=CARTESIAN_POINT('Ctrl Pts',(4.56850399330538,-23.0512449880405,
88.9998970643313));
#123829=CARTESIAN_POINT('Ctrl Pts',(4.62986114399214,-23.0552605125574,
88.9707290848305));
#123830=CARTESIAN_POINT('Ctrl Pts',(4.69120662481904,-23.0592406305492,
88.9412176853075));
#123831=CARTESIAN_POINT('Ctrl Pts',(4.75254164044052,-23.0631825590175,
88.9113475912022));
#123832=CARTESIAN_POINT('Ctrl Pts',(4.93441452521425,-23.0748713129018,
88.822775669791));
#123833=CARTESIAN_POINT('Ctrl Pts',(5.11619655591822,-23.0862237242864,
88.7310530645164));
#123834=CARTESIAN_POINT('Ctrl Pts',(5.29786541494919,-23.0971723853635,
88.6358318752671));
#123835=CARTESIAN_POINT('Ctrl Pts',(5.45867598089911,-23.1068639769416,
88.5515434979674));
#123836=CARTESIAN_POINT('Ctrl Pts',(5.61939791126611,-23.1162393502448,
88.4645135318602));
#123837=CARTESIAN_POINT('Ctrl Pts',(5.78000322652552,-23.1252563837044,
88.3744691485403));
#123838=CARTESIAN_POINT('Ctrl Pts',(5.93597595541102,-23.1340133249855,
88.2870220539998));
#123839=CARTESIAN_POINT('Ctrl Pts',(6.09183893182038,-23.1424323589763,
88.1967316702881));
#123840=CARTESIAN_POINT('Ctrl Pts',(6.2475397577679,-23.1504782711739,88.1033934457889));
#123841=CARTESIAN_POINT('Ctrl Pts',(6.41231567943124,-23.1589931431401,
88.004614959068));
#123842=CARTESIAN_POINT('Ctrl Pts',(6.57693499166336,-23.1670818041468,
87.9024144337999));
#123843=CARTESIAN_POINT('Ctrl Pts',(6.74135405556885,-23.1746592334894,
87.7965118526924));
#123844=CARTESIAN_POINT('Ctrl Pts',(6.76510788714164,-23.1757539543574,
87.7812119719183));
#123845=CARTESIAN_POINT('Ctrl Pts',(6.7888574945791,-23.1768380148025,87.7658347455952));
#123846=CARTESIAN_POINT('Ctrl Pts',(6.81260269912841,-23.1779111680061,
87.7503792501723));
#123847=CARTESIAN_POINT('Ctrl Pts',(6.90290661273152,-23.1819924103465,
87.691601414822));
#123848=CARTESIAN_POINT('Ctrl Pts',(6.99314705828,-23.1859158714207,87.6316918366667));
#123849=CARTESIAN_POINT('Ctrl Pts',(7.0833163338459,-23.189668226085,87.570615127344));
#123850=CARTESIAN_POINT('Ctrl Pts',(7.22231302199292,-23.1954525120052,
87.4764648719994));
#123851=CARTESIAN_POINT('Ctrl Pts',(7.36114570487625,-23.2008334359504,
87.3795376940918));
#123852=CARTESIAN_POINT('Ctrl Pts',(7.49978323223744,-23.2057581195249,
87.2796812183491));
#123853=CARTESIAN_POINT('Ctrl Pts',(7.56910199591804,-23.2082204613121,
87.2297529804777));
#123854=CARTESIAN_POINT('Ctrl Pts',(7.63837141634081,-23.2105683901063,
87.1790924778903));
#123855=CARTESIAN_POINT('Ctrl Pts',(7.70758513080529,-23.2127935346573,
87.1276801626053));
#123856=CARTESIAN_POINT('Ctrl Pts',(7.74219198803752,-23.2139061069327,
87.1019740049629));
#123857=CARTESIAN_POINT('Ctrl Pts',(7.7767849042651,-23.21498797025,87.0760798768848));
#123858=CARTESIAN_POINT('Ctrl Pts',(7.81136296286751,-23.2160379809069,
87.0499952636164));
#123859=CARTESIAN_POINT('Ctrl Pts',(7.81422474291771,-23.2161248828231,
87.0478364256456));
#123860=CARTESIAN_POINT('Ctrl Pts',(7.81708642119755,-23.2162115663482,
87.0456762829635));
#123861=CARTESIAN_POINT('Ctrl Pts',(7.81994799711031,-23.2162980310548,
87.0435148340046));
#123862=CARTESIAN_POINT('Ctrl Pts',(7.83437421723199,-23.2167339303383,
87.0326182024236));
#123863=CARTESIAN_POINT('Ctrl Pts',(7.84879783586087,-23.2171642683021,
87.0216883716409));
#123864=CARTESIAN_POINT('Ctrl Pts',(7.86321881976802,-23.2175889901186,
87.010725206942));
#123865=CARTESIAN_POINT('Ctrl Pts',(7.87185958035186,-23.2178434748025,
87.0041563013795));
#123866=CARTESIAN_POINT('Ctrl Pts',(7.88049939494386,-23.2180959434931,
86.9975754281851));
#123867=CARTESIAN_POINT('Ctrl Pts',(7.88913825598689,-23.2183463846371,
86.9909825578367));
#123868=CARTESIAN_POINT('Ctrl Pts',(7.89777711702992,-23.2185968257811,
86.9843896874883));
#123869=CARTESIAN_POINT('Ctrl Pts',(7.9080894630654,-23.2188930037954,86.976502007423));
#123870=CARTESIAN_POINT('Ctrl Pts',(7.91505197072149,-23.2190916136997,
86.9711679255529));
#123871=CARTESIAN_POINT('Ctrl Pts',(8.09134263270587,-23.2241204155669,
86.8361089970165));
#123872=CARTESIAN_POINT('Ctrl Pts',(8.26579962669912,-23.2285515297506,
86.6969431825184));
#123873=CARTESIAN_POINT('Ctrl Pts',(8.43834390340455,-23.2323917796661,
86.5535726536806));
#123874=CARTESIAN_POINT('Ctrl Pts',(8.54726618800008,-23.2348160199957,
86.4630669246999));
#123875=CARTESIAN_POINT('Ctrl Pts',(8.6554255322555,-23.2370047142792,86.3708849085284));
#123876=CARTESIAN_POINT('Ctrl Pts',(8.76279353307567,-23.2389586523644,
86.2769955028744));
#123877=CARTESIAN_POINT('Ctrl Pts',(8.93583566793336,-23.2421077621092,
86.1256764592974));
#123878=CARTESIAN_POINT('Ctrl Pts',(9.10682452799498,-23.2446473763279,
85.9699232692661));
#123879=CARTESIAN_POINT('Ctrl Pts',(9.27571672569409,-23.2465765880523,
85.8096667102436));
#123880=CARTESIAN_POINT('Ctrl Pts',(9.40440547155385,-23.2480465661845,
85.6875579575756));
#123881=CARTESIAN_POINT('Ctrl Pts',(9.53187611599803,-23.2491620555429,
85.5628340870123));
#123882=CARTESIAN_POINT('Ctrl Pts',(9.65809042986943,-23.249920494709,85.4354575360454));
#123883=CARTESIAN_POINT('Ctrl Pts',(9.82840053416643,-23.2509439115427,
85.2635791411569));
#123884=CARTESIAN_POINT('Ctrl Pts',(9.99642459708762,-23.2513174795469,
85.0868705066055));
#123885=CARTESIAN_POINT('Ctrl Pts',(10.1621489201754,-23.2510291393295,
84.9052620331361));
#123886=CARTESIAN_POINT('Ctrl Pts',(10.2548830078338,-23.2508677932669,
84.803639677501));
#123887=CARTESIAN_POINT('Ctrl Pts',(10.3468961194323,-23.2504990718905,
84.7004829782548));
#123888=CARTESIAN_POINT('Ctrl Pts',(10.4381787520344,-23.2499199044464,
84.5957795828485));
#123889=CARTESIAN_POINT('Ctrl Pts',(10.4661094651373,-23.2497426904544,
84.5637423769241));
#123890=CARTESIAN_POINT('Ctrl Pts',(10.4939715105974,-23.2495454018335,
84.5315609605594));
#123891=CARTESIAN_POINT('Ctrl Pts',(10.5217636141367,-23.24932841804,84.4992356500257));
#123892=CARTESIAN_POINT('Ctrl Pts',(10.6908907477392,-23.2480079765346,
84.3025219645837));
#123893=CARTESIAN_POINT('Ctrl Pts',(10.857429405005,-23.2459586353402,84.1004758835953));
#123894=CARTESIAN_POINT('Ctrl Pts',(11.0212005082572,-23.2432622574743,
83.8931696662918));
#123895=CARTESIAN_POINT('Ctrl Pts',(11.1316471341769,-23.2414438302207,
83.7533631205783));
#123896=CARTESIAN_POINT('Ctrl Pts',(11.2408345983813,-23.2393309822942,
83.6111650785467));
#123897=CARTESIAN_POINT('Ctrl Pts',(11.3487029438601,-23.2369477669547,
83.4666101713744));
#123898=CARTESIAN_POINT('Ctrl Pts',(11.509949909774,-23.2333852181743,83.2505223090267));
#123899=CARTESIAN_POINT('Ctrl Pts',(11.6682489825816,-23.2292184719187,
83.0291657532378));
#123900=CARTESIAN_POINT('Ctrl Pts',(11.8234719698744,-23.2245265773938,
82.8026310036824));
#123901=CARTESIAN_POINT('Ctrl Pts',(11.9273300939928,-23.2213872784251,
82.651058903784));
#123902=CARTESIAN_POINT('Ctrl Pts',(12.0298109606654,-23.2180128492973,
82.4971696001478));
#123903=CARTESIAN_POINT('Ctrl Pts',(12.1308752870379,-23.2144271256202,
82.3410032958163));
#123904=CARTESIAN_POINT('Ctrl Pts',(12.2858032080798,-23.2089303421886,
82.1016060551149));
#123905=CARTESIAN_POINT('Ctrl Pts',(12.4374015621889,-23.2029367897955,
81.8568558748265));
#123906=CARTESIAN_POINT('Ctrl Pts',(12.58557409216,-23.1965347740778,81.6068413665939));
#123907=CARTESIAN_POINT('Ctrl Pts',(12.5974439769964,-23.1960219179545,
81.5868130697111));
#123908=CARTESIAN_POINT('Ctrl Pts',(12.6092918820148,-23.1955064427389,
81.5667510169829));
#123909=CARTESIAN_POINT('Ctrl Pts',(12.6211177605568,-23.194988395035,81.5466552684072));
#123910=CARTESIAN_POINT('',(0.756578721069087,-21.00000000034,88.93560161898));
#123911=CARTESIAN_POINT('Origin',(0.756570553373981,-22.5000441054858,88.9355484040727));
#123912=CARTESIAN_POINT('',(9.42148081258226,-20.999999610319,83.7851764430462));
#123913=CARTESIAN_POINT('Ctrl Pts',(9.42147697938284,-21.000000000085,83.7851937308496));
#123914=CARTESIAN_POINT('Ctrl Pts',(9.27399191800444,-21.0000000000907,
83.9540227648115));
#123915=CARTESIAN_POINT('Ctrl Pts',(9.12456523022954,-20.9999999999873,
84.1177960831894));
#123916=CARTESIAN_POINT('Ctrl Pts',(8.97356867507927,-21.0000000000114,
84.2763877180128));
#123917=CARTESIAN_POINT('Ctrl Pts',(8.89529364447174,-21.000000000024,84.3585999582691));
#123918=CARTESIAN_POINT('Ctrl Pts',(8.81659690184896,-21.0000000000025,
84.4394205773969));
#123919=CARTESIAN_POINT('Ctrl Pts',(8.7375311505406,-20.9999999999974,84.518837464166));
#123920=CARTESIAN_POINT('Ctrl Pts',(8.73449110473416,-20.9999999999972,
84.5218910109873));
#123921=CARTESIAN_POINT('Ctrl Pts',(8.73145051346632,-20.9999999999971,
84.5249424830282));
#123922=CARTESIAN_POINT('Ctrl Pts',(8.72840938028159,-20.9999999999971,
84.5279918800666));
#123923=CARTESIAN_POINT('Ctrl Pts',(8.61933714481441,-20.9999999999971,
84.6373605040659));
#123924=CARTESIAN_POINT('Ctrl Pts',(8.5095545037636,-21.0000000000552,84.7440439198219));
#123925=CARTESIAN_POINT('Ctrl Pts',(8.39886090767497,-21.0000000000394,
84.8483541764564));
#123926=CARTESIAN_POINT('Ctrl Pts',(8.28809191854098,-21.0000000000236,
84.9527354784648));
#123927=CARTESIAN_POINT('Ctrl Pts',(8.17641056141695,-20.9999999999989,
85.0547405710911));
#123928=CARTESIAN_POINT('Ctrl Pts',(8.0635768694174,-20.9999999999973,85.1546476180281));
#123929=CARTESIAN_POINT('Ctrl Pts',(8.04652410682795,-20.9999999999971,
85.1697467530669));
#123930=CARTESIAN_POINT('Ctrl Pts',(8.02944495413355,-20.9999999999971,
85.184797899742));
#123931=CARTESIAN_POINT('Ctrl Pts',(8.01233850907909,-20.9999999999971,
85.1998019455117));
#123932=CARTESIAN_POINT('Ctrl Pts',(7.97871884199685,-20.9999999999971,
85.2292897217305));
#123933=CARTESIAN_POINT('Ctrl Pts',(7.94499438200283,-20.9999999999966,
85.2585958705356));
#123934=CARTESIAN_POINT('Ctrl Pts',(7.91115741286785,-20.9999999999976,
85.2877267368321));
#123935=CARTESIAN_POINT('Ctrl Pts',(7.79875923544382,-21.0000000000009,
85.3844923858313));
#123936=CARTESIAN_POINT('Ctrl Pts',(7.68512207258091,-21.0000000000743,
85.4793270732401));
#123937=CARTESIAN_POINT('Ctrl Pts',(7.56996387602843,-21.0000000001119,
85.5724644706683));
#123938=CARTESIAN_POINT('Ctrl Pts',(7.46879379250766,-21.000000000145,85.6542885922576));
#123939=CARTESIAN_POINT('Ctrl Pts',(7.36644918188812,-20.9999999999971,
85.7348021831151));
#123940=CARTESIAN_POINT('Ctrl Pts',(7.26271916490076,-20.9999999999971,
85.8141369321334));
#123941=CARTESIAN_POINT('Ctrl Pts',(7.18897059090721,-20.9999999999971,
85.8705412862264));
#123942=CARTESIAN_POINT('Ctrl Pts',(7.11453057722115,-21.0000000000856,
85.9263626033712));
#123943=CARTESIAN_POINT('Ctrl Pts',(7.03944495771895,-21.0000000000741,
85.9815486371181));
#123944=CARTESIAN_POINT('Ctrl Pts',(6.89893946022772,-21.0000000000526,
86.0848166287467));
#123945=CARTESIAN_POINT('Ctrl Pts',(6.75617114718754,-21.0000000000048,
86.1858577156669));
#123946=CARTESIAN_POINT('Ctrl Pts',(6.61149924495893,-21.0000000000084,
86.2844218120254));
#123947=CARTESIAN_POINT('Ctrl Pts',(6.56370101073671,-21.0000000000097,
86.3169864613531));
#123948=CARTESIAN_POINT('Ctrl Pts',(6.51569527322402,-20.9999999999971,
86.3492810398185));
#123949=CARTESIAN_POINT('Ctrl Pts',(6.46749581550409,-20.9999999999971,
86.3812974551033));
#123950=CARTESIAN_POINT('Ctrl Pts',(6.34746269045993,-20.9999999999971,
86.4610292728694));
#123951=CARTESIAN_POINT('Ctrl Pts',(6.22623198433834,-21.0000000001373,
86.5390531423975));
#123952=CARTESIAN_POINT('Ctrl Pts',(6.10431565800804,-21.0000000001907,
86.615112577885));
#123953=CARTESIAN_POINT('Ctrl Pts',(5.9818449747345,-21.0000000002444,86.6915178577514));
#123954=CARTESIAN_POINT('Ctrl Pts',(5.85868278370828,-21.0000000001471,
86.7659410902819));
#123955=CARTESIAN_POINT('Ctrl Pts',(5.73538690640595,-21.0000000000453,
86.838212150071));
#123956=CARTESIAN_POINT('Ctrl Pts',(5.70324379362019,-21.0000000000188,
86.8570531435963));
#123957=CARTESIAN_POINT('Ctrl Pts',(5.67109173256492,-20.9999999999971,
86.8757481081935));
#123958=CARTESIAN_POINT('Ctrl Pts',(5.63894088385909,-20.9999999999971,
86.8942945284283));
#123959=CARTESIAN_POINT('Ctrl Pts',(5.50244658861362,-20.9999999999971,
86.9730321251381));
#123960=CARTESIAN_POINT('Ctrl Pts',(5.36594890838618,-20.9999999999385,
87.0490545898275));
#123961=CARTESIAN_POINT('Ctrl Pts',(5.22930121456414,-21.0000000000313,
87.1227204573118));
#123962=CARTESIAN_POINT('Ctrl Pts',(5.19957341189603,-21.0000000000515,
87.1387465190088));
#123963=CARTESIAN_POINT('Ctrl Pts',(5.16983838021216,-21.0000000000804,
87.1546608986856));
#123964=CARTESIAN_POINT('Ctrl Pts',(5.14009440103752,-21.0000000001088,
87.1704670447945));
#123965=CARTESIAN_POINT('Ctrl Pts',(5.02785242631964,-21.0000000002158,
87.2301131681836));
#123966=CARTESIAN_POINT('Ctrl Pts',(4.91548405719906,-20.9999999999971,
87.2882194114902));
#123967=CARTESIAN_POINT('Ctrl Pts',(4.80288878060909,-20.9999999999971,
87.3449847521551));
#123968=CARTESIAN_POINT('Ctrl Pts',(4.70564380844993,-20.9999999999971,
87.3940111779496));
#123969=CARTESIAN_POINT('Ctrl Pts',(4.60821980374707,-21.0000000005356,
87.4420125406706));
#123970=CARTESIAN_POINT('Ctrl Pts',(4.50998723134151,-21.0000000008011,
87.4893476966616));
#123971=CARTESIAN_POINT('Ctrl Pts',(4.40901116245255,-21.000000001074,87.5380048564524));
#123972=CARTESIAN_POINT('Ctrl Pts',(4.30718057840428,-21.0000000010355,
87.5859579974302));
#123973=CARTESIAN_POINT('Ctrl Pts',(4.20378538799987,-21.0000000007123,
87.6335491764987));
#123974=CARTESIAN_POINT('Ctrl Pts',(4.19363316767935,-21.0000000006805,
87.6382220837522));
#123975=CARTESIAN_POINT('Ctrl Pts',(4.18346584369122,-21.0000000006469,
87.6428914648658));
#123976=CARTESIAN_POINT('Ctrl Pts',(4.17328273148044,-21.0000000006121,
87.647557620073));
#123977=CARTESIAN_POINT('Ctrl Pts',(4.09799686416734,-21.0000000003543,
87.682055476379));
#123978=CARTESIAN_POINT('Ctrl Pts',(4.02184851305395,-20.9999999999971,
87.7163779316246));
#123979=CARTESIAN_POINT('Ctrl Pts',(3.94455679822576,-20.9999999999971,
87.7506447831067));
#123980=CARTESIAN_POINT('Ctrl Pts',(3.72588698588882,-20.9999999999971,
87.8475908270601));
#123981=CARTESIAN_POINT('Ctrl Pts',(3.49813393978502,-21.0000000001597,
87.9441897501269));
#123982=CARTESIAN_POINT('Ctrl Pts',(3.25999551214122,-21.000000000035,88.0406735965696));
#123983=CARTESIAN_POINT('Ctrl Pts',(3.20802281016991,-21.0000000000077,
88.0617307869014));
#123984=CARTESIAN_POINT('Ctrl Pts',(3.15555560316831,-20.9999999999999,
88.0827825845688));
#123985=CARTESIAN_POINT('Ctrl Pts',(3.10258068301365,-20.9999999999979,
88.1038316430887));
#123986=CARTESIAN_POINT('Ctrl Pts',(3.0677194107392,-20.9999999999966,88.117683423479));
#123987=CARTESIAN_POINT('Ctrl Pts',(3.03263827309266,-20.9999999999971,
88.1315340188204));
#123988=CARTESIAN_POINT('Ctrl Pts',(2.99733338629909,-20.9999999999971,
88.1453845195516));
#123989=CARTESIAN_POINT('Ctrl Pts',(2.84718752884044,-20.9999999999971,
88.2042884135275));
#123990=CARTESIAN_POINT('Ctrl Pts',(2.6930013806397,-21.0000000000004,88.2632001191942));
#123991=CARTESIAN_POINT('Ctrl Pts',(2.53487949972314,-21.0000000000036,
88.3221003830513));
#123992=CARTESIAN_POINT('Ctrl Pts',(2.37929265912228,-21.0000000000068,
88.3800563465837));
#123993=CARTESIAN_POINT('Ctrl Pts',(2.21989523490024,-21.0000000000046,
88.4380011683893));
#123994=CARTESIAN_POINT('Ctrl Pts',(2.05680785367107,-20.9999999999995,
88.4959626190292));
#123995=CARTESIAN_POINT('Ctrl Pts',(2.01608671892802,-20.9999999999982,
88.5104349590939));
#123996=CARTESIAN_POINT('Ctrl Pts',(1.97513564045399,-20.9999999999971,
88.5249085661768));
#123997=CARTESIAN_POINT('Ctrl Pts',(1.93395670865826,-20.9999999999971,
88.5393843373408));
#123998=CARTESIAN_POINT('Ctrl Pts',(1.91643441811195,-20.9999999999971,
88.5455440082491));
#123999=CARTESIAN_POINT('Ctrl Pts',(1.89887083619214,-20.9999999999973,
88.5517040899185));
#124000=CARTESIAN_POINT('Ctrl Pts',(1.88126597856944,-20.9999999999978,
88.5578647064176));
#124001=CARTESIAN_POINT('Ctrl Pts',(1.71400566050106,-21.0000000000031,
88.6163955220154));
#124002=CARTESIAN_POINT('Ctrl Pts',(1.54301816142452,-21.000000000055,88.6749706246985));
#124003=CARTESIAN_POINT('Ctrl Pts',(1.36830996496456,-21.0000000001698,
88.7337291107176));
#124004=CARTESIAN_POINT('Ctrl Pts',(1.19842766148794,-21.0000000002815,
88.7908645351338));
#124005=CARTESIAN_POINT('Ctrl Pts',(1.0250273328815,-21.0000000004429,88.8481732337227));
#124006=CARTESIAN_POINT('Ctrl Pts',(0.848131604814033,-21.0000000004876,
88.9058299251113));
#124007=CARTESIAN_POINT('Ctrl Pts',(0.81771720783072,-21.0000000004953,
88.915743072929));
#124008=CARTESIAN_POINT('Ctrl Pts',(0.787199523968459,-21.0000000004994,
88.9256666252834));
#124009=CARTESIAN_POINT('Ctrl Pts',(0.756578721069087,-21.0000000004994,
88.93560161898));
#124010=CARTESIAN_POINT('Ctrl Pts',(9.42148468716754,-20.9999998370474,
83.7851849075908));
#124011=CARTESIAN_POINT('Ctrl Pts',(9.4941219370757,-20.9999987247078,83.7542551887972));
#124012=CARTESIAN_POINT('Ctrl Pts',(9.56349342993131,-21.0011753932936,
83.7247364896096));
#124013=CARTESIAN_POINT('Ctrl Pts',(9.62942675509781,-21.0033031504389,
83.6966742681167));
#124014=CARTESIAN_POINT('Ctrl Pts',(9.70159869602387,-21.0056322361116,
83.6659567972971));
#124015=CARTESIAN_POINT('Ctrl Pts',(9.76965086116896,-21.0091004632847,
83.6369844447678));
#124016=CARTESIAN_POINT('Ctrl Pts',(9.83339225163773,-21.0133592125468,
83.6097967955185));
#124017=CARTESIAN_POINT('Ctrl Pts',(9.86821381453554,-21.0156857433019,
83.5949443357366));
#124018=CARTESIAN_POINT('Ctrl Pts',(9.9017494968727,-21.0182473659859,83.5806241620194));
#124019=CARTESIAN_POINT('Ctrl Pts',(9.93397208322834,-21.0209827456319,
83.5668406521577));
#124020=CARTESIAN_POINT('Ctrl Pts',(10.0012249953719,-21.0266918542982,
83.5380725958777));
#124021=CARTESIAN_POINT('Ctrl Pts',(10.0627624804275,-21.0331595220266,
83.5116677566652));
#124022=CARTESIAN_POINT('Ctrl Pts',(10.118432381711,-21.0398462117802,83.4877507581234));
#124023=CARTESIAN_POINT('Ctrl Pts',(10.1228137575912,-21.0403724728392,
83.4858684238975));
#124024=CARTESIAN_POINT('Ctrl Pts',(10.1271587990794,-21.0409000994819,
83.4840014909435));
#124025=CARTESIAN_POINT('Ctrl Pts',(10.1314674224592,-21.041428840755,83.4821500212401));
#124026=CARTESIAN_POINT('Ctrl Pts',(10.1609944869985,-21.045052313108,83.4694618699199));
#124027=CARTESIAN_POINT('Ctrl Pts',(10.1888130136579,-21.0487283218401,
83.4575006696735));
#124028=CARTESIAN_POINT('Ctrl Pts',(10.2149085149073,-21.0523803329437,
83.4462874670011));
#124029=CARTESIAN_POINT('Ctrl Pts',(10.227956265532,-21.0542063384956,83.4406808656649));
#124030=CARTESIAN_POINT('Ctrl Pts',(10.2405732483423,-21.0560263866187,
83.4352612547228));
#124031=CARTESIAN_POINT('Ctrl Pts',(10.2527582877196,-21.0578314278658,
83.4300313071825));
#124032=CARTESIAN_POINT('Ctrl Pts',(10.2588508074083,-21.0587339484893,
83.4274163334123));
#124033=CARTESIAN_POINT('Ctrl Pts',(10.2648353402489,-21.0596327218206,
83.4248487747094));
#124034=CARTESIAN_POINT('Ctrl Pts',(10.2707117489126,-21.0605266486678,
83.4223289593342));
#124035=CARTESIAN_POINT('Ctrl Pts',(10.2736499532444,-21.0609736120914,
83.4210690516466));
#124036=CARTESIAN_POINT('Ctrl Pts',(10.2765611264585,-21.0614193642047,
83.4198210797331));
#124037=CARTESIAN_POINT('Ctrl Pts',(10.2794452533187,-21.0618637701409,
83.4185850844988));
#124038=CARTESIAN_POINT('Ctrl Pts',(10.2823293801789,-21.0623081760772,
83.4173490892646));
#124039=CARTESIAN_POINT('Ctrl Pts',(10.2836807391676,-21.0625162915106,
83.4167699199381));
#124040=CARTESIAN_POINT('Ctrl Pts',(10.2880164799651,-21.063192816072,83.4149130695255));
#124041=CARTESIAN_POINT('Ctrl Pts',(10.3573883327262,-21.0740172090535,
83.3852034629241));
#124042=CARTESIAN_POINT('Ctrl Pts',(10.4244790085951,-21.0860937750086,
83.356489243626));
#124043=CARTESIAN_POINT('Ctrl Pts',(10.4891589927194,-21.0992619090558,
83.3288037272593));
#124044=CARTESIAN_POINT('Ctrl Pts',(10.5538389768437,-21.1124300431029,
83.3011182108926));
#124045=CARTESIAN_POINT('Ctrl Pts',(10.6161083609051,-21.126689375742,83.2744613038628));
#124046=CARTESIAN_POINT('Ctrl Pts',(10.6758773896147,-21.1418390982324,
83.2488498686012));
#124047=CARTESIAN_POINT('Ctrl Pts',(10.6944286648869,-21.146541310704,83.240900520989));
#124048=CARTESIAN_POINT('Ctrl Pts',(10.7127383054214,-21.1513290015203,
83.2330530884892));
#124049=CARTESIAN_POINT('Ctrl Pts',(10.7308053753453,-21.1561961057732,
83.2253085040455));
#124050=CARTESIAN_POINT('Ctrl Pts',(10.7709473075054,-21.1670099770626,
83.2081013650542));
#124051=CARTESIAN_POINT('Ctrl Pts',(10.8098908809428,-21.1782162765483,
83.191402349222));
#124052=CARTESIAN_POINT('Ctrl Pts',(10.8476102714308,-21.1897492289399,
83.1752272556387));
#124053=CARTESIAN_POINT('Ctrl Pts',(10.8749583331879,-21.1981110791757,
83.1634996679836));
#124054=CARTESIAN_POINT('Ctrl Pts',(10.9016637920612,-21.2066447958269,
83.1520473918412));
#124055=CARTESIAN_POINT('Ctrl Pts',(10.9277205287919,-21.2153245551945,
83.1408772706061));
#124056=CARTESIAN_POINT('Ctrl Pts',(10.9407488971573,-21.2196644348783,
83.1352922099885));
#124057=CARTESIAN_POINT('Ctrl Pts',(10.9536150958344,-21.2240407993215,
83.129777696196));
#124058=CARTESIAN_POINT('Ctrl Pts',(10.9663185903961,-21.2284503766631,
83.1243346726393));
#124059=CARTESIAN_POINT('Ctrl Pts',(10.9757077232876,-21.2317094883551,
83.1203117424717));
#124060=CARTESIAN_POINT('Ctrl Pts',(10.9844456080701,-21.2347871993304,
83.1165686325483));
#124061=CARTESIAN_POINT('Ctrl Pts',(10.9937795634143,-21.2381236045094,
83.1125716339291));
#124062=CARTESIAN_POINT('Ctrl Pts',(10.9970744474234,-21.2393013547414,
83.1111606943703));
#124063=CARTESIAN_POINT('Ctrl Pts',(11.000443387423,-21.2405117232215,83.1097182138103));
#124064=CARTESIAN_POINT('Ctrl Pts',(11.0039404737775,-21.2417753992659,
83.1082210540086));
#124065=CARTESIAN_POINT('Ctrl Pts',(11.0631942380401,-21.2631868128966,
83.082853549476));
#124066=CARTESIAN_POINT('Ctrl Pts',(11.1203932699226,-21.2859004072948,
83.0584395184106));
#124067=CARTESIAN_POINT('Ctrl Pts',(11.1754531134644,-21.3098087790778,
83.0349755843049));
#124068=CARTESIAN_POINT('Ctrl Pts',(11.1976469963221,-21.3194459223848,
83.0255175878519));
#124069=CARTESIAN_POINT('Ctrl Pts',(11.2194937986439,-21.3292768923882,
83.0162137952532));
#124070=CARTESIAN_POINT('Ctrl Pts',(11.2409899698962,-21.3392935161446,
83.0070633299919));
#124071=CARTESIAN_POINT('Ctrl Pts',(11.2895857629332,-21.3619378172754,
82.9863771291417));
#124072=CARTESIAN_POINT('Ctrl Pts',(11.3363860415459,-21.3855316806876,
82.9664757873883));
#124073=CARTESIAN_POINT('Ctrl Pts',(11.3812882123752,-21.4099625974059,
82.9473763273766));
#124074=CARTESIAN_POINT('Ctrl Pts',(11.4271082844229,-21.4348929369317,
82.9278864315065));
#124075=CARTESIAN_POINT('Ctrl Pts',(11.4709518791844,-21.4606946924684,
82.9092315100768));
#124076=CARTESIAN_POINT('Ctrl Pts',(11.5127604257083,-21.4872375191448,
82.8914122362505));
#124077=CARTESIAN_POINT('Ctrl Pts',(11.5296285630557,-21.4979465268285,
82.8842228459624));
#124078=CARTESIAN_POINT('Ctrl Pts',(11.5461659945948,-21.5087760641745,
82.8771692907715));
#124079=CARTESIAN_POINT('Ctrl Pts',(11.5623710988165,-21.5197172131263,
82.8702508527974));
#124080=CARTESIAN_POINT('Ctrl Pts',(11.5907328843161,-21.5388661501183,
82.8581423682649));
#124081=CARTESIAN_POINT('Ctrl Pts',(11.6180670866337,-21.5583481139389,
82.8464481889862));
#124082=CARTESIAN_POINT('Ctrl Pts',(11.6443762493541,-21.5781278394007,
82.8351789009517));
#124083=CARTESIAN_POINT('Ctrl Pts',(11.6824031463224,-21.6067171787951,
82.818890429154));
#124084=CARTESIAN_POINT('Ctrl Pts',(11.7182857209953,-21.6359274631247,
82.803491035106));
#124085=CARTESIAN_POINT('Ctrl Pts',(11.7519727657735,-21.6655985418644,
82.7890322234246));
#124086=CARTESIAN_POINT('Ctrl Pts',(11.7875315792775,-21.6969182483662,
82.7737700301556));
#124087=CARTESIAN_POINT('Ctrl Pts',(11.8206442207179,-21.7287515826067,
82.7595557971992));
#124088=CARTESIAN_POINT('Ctrl Pts',(11.8513026624327,-21.7609228338839,
82.7464223763073));
#124089=CARTESIAN_POINT('Ctrl Pts',(11.881683577325,-21.7928028640605,82.7334078419721));
#124090=CARTESIAN_POINT('Ctrl Pts',(11.9096550578661,-21.825015029524,82.7214543109823));
#124091=CARTESIAN_POINT('Ctrl Pts',(11.9352533773051,-21.8573962950116,
82.7105706050017));
#124092=CARTESIAN_POINT('Ctrl Pts',(11.9357484417354,-21.8580225397456,
82.710360117133));
#124093=CARTESIAN_POINT('Ctrl Pts',(11.9362426197884,-21.8586488478941,
82.7101500287686));
#124094=CARTESIAN_POINT('Ctrl Pts',(11.9367359116729,-21.8592752175941,
82.7099403399791));
#124095=CARTESIAN_POINT('Origin',(-6.52065461870091,-20.,86.59621775143));
#124096=CARTESIAN_POINT('',(-5.93853418689289,-20.99999960112,86.4935742132807));
#124097=CARTESIAN_POINT('',(-6.11218254686295,-20.0000000000124,85.5087654262472));
#124098=CARTESIAN_POINT('Origin',(-5.93853418689091,-20.,86.49357421328));
#124099=CARTESIAN_POINT('',(9.24780733902467,-20.0000000000007,82.8003857150944));
#124100=CARTESIAN_POINT('',(-6.11218263803291,-20.00000000001,85.50876490924));
#124101=CARTESIAN_POINT('Origin',(9.42145554646909,-19.99999972872,83.78519359989));
#124102=CARTESIAN_POINT('',(-5.93853418689091,-20.99999920224,86.49357421328));
#124103=CARTESIAN_POINT('Ctrl Pts',(9.31777244213909,-20.94531685512,84.14178879308));
#124104=CARTESIAN_POINT('Ctrl Pts',(9.36640017655909,-20.94770345583,84.1219806875601));
#124105=CARTESIAN_POINT('Ctrl Pts',(9.65757640544909,-20.96509256254,84.00275491356));
#124106=CARTESIAN_POINT('Ctrl Pts',(10.1549539983791,-21.02844485154,83.7926499217099));
#124107=CARTESIAN_POINT('Ctrl Pts',(10.7546658021091,-21.18754199612,83.5266079797999));
#124108=CARTESIAN_POINT('Ctrl Pts',(11.2403353151791,-21.40098020438,83.30037335394));
#124109=CARTESIAN_POINT('Ctrl Pts',(11.6099495725991,-21.65243696673,83.11889690529));
#124110=CARTESIAN_POINT('Ctrl Pts',(11.8190595633691,-21.87547143775,83.0102334421199));
#124111=CARTESIAN_POINT('Ctrl Pts',(11.9040610043191,-22.00823653322,82.964473853835));
#124112=CARTESIAN_POINT('Ctrl Pts',(11.9241977534391,-22.04372273473,82.9535566484859));
#124113=CARTESIAN_POINT('Ctrl Pts',(9.17645376799909,-21.25096624947,83.2879897269701));
#124114=CARTESIAN_POINT('Ctrl Pts',(9.22142272969909,-21.24328720155,83.2651886209901));
#124115=CARTESIAN_POINT('Ctrl Pts',(9.49214864496909,-21.19958401021,83.12878887307));
#124116=CARTESIAN_POINT('Ctrl Pts',(9.97085285597909,-21.15021821319,82.897289550365));
#124117=CARTESIAN_POINT('Ctrl Pts',(10.5934314779391,-21.16468088244,82.619908795121));
#124118=CARTESIAN_POINT('Ctrl Pts',(11.1469282254291,-21.2664360337,82.394534196853));
#124119=CARTESIAN_POINT('Ctrl Pts',(11.6180848277091,-21.4560997606,82.2199954501849));
#124120=CARTESIAN_POINT('Ctrl Pts',(11.9207663248691,-21.68120338254,82.117675714632));
#124121=CARTESIAN_POINT('Ctrl Pts',(12.0537280986091,-21.83843148824,82.074956833363));
#124122=CARTESIAN_POINT('Ctrl Pts',(12.0857902240491,-21.88190130568,82.0647465697241));
#124123=CARTESIAN_POINT('Ctrl Pts',(9.04133139198908,-20.62712475778,82.628500914342));
#124124=CARTESIAN_POINT('Ctrl Pts',(9.0929323218291,-20.61138663654,82.6119687700661));
#124125=CARTESIAN_POINT('Ctrl Pts',(9.40552780613909,-20.52047148252,82.5136949694449));
#124126=CARTESIAN_POINT('Ctrl Pts',(9.97906646707909,-20.40232051245,82.353473063821));
#124127=CARTESIAN_POINT('Ctrl Pts',(10.7708010393391,-20.37411518934,82.1731360077631));
#124128=CARTESIAN_POINT('Ctrl Pts',(11.5138296365191,-20.49600614651,82.034557857099));
#124129=CARTESIAN_POINT('Ctrl Pts',(12.1780168724191,-20.77496047938,81.932042963468));
#124130=CARTESIAN_POINT('Ctrl Pts',(12.6233299940891,-21.13270407263,81.8735317226859));
#124131=CARTESIAN_POINT('Ctrl Pts',(12.8231734110491,-21.39071629538,81.8493699294251));
#124132=CARTESIAN_POINT('Ctrl Pts',(12.8715846172591,-21.46248197016,81.84356917358));
#124133=CARTESIAN_POINT('Ctrl Pts',(9.05705447055909,-19.74161771142,82.869308315871));
#124134=CARTESIAN_POINT('Ctrl Pts',(9.11847855545909,-19.7284543691,82.8615961416661));
#124135=CARTESIAN_POINT('Ctrl Pts',(9.49044191549909,-19.65474822197,82.815934198766));
#124136=CARTESIAN_POINT('Ctrl Pts',(10.1708021213091,-19.58537985194,82.743358638735));
#124137=CARTESIAN_POINT('Ctrl Pts',(11.0968995137491,-19.66214931145,82.6645620454749));
#124138=CARTESIAN_POINT('Ctrl Pts',(11.9482698149491,-19.91443945991,82.605800745851));
#124139=CARTESIAN_POINT('Ctrl Pts',(12.6903357471891,-20.33818201501,82.563293973608));
#124140=CARTESIAN_POINT('Ctrl Pts',(13.1746527682191,-20.81714466972,82.539158789408));
#124141=CARTESIAN_POINT('Ctrl Pts',(13.3887020165791,-21.14437223204,82.529205012765));
#124142=CARTESIAN_POINT('Ctrl Pts',(13.4403842380291,-21.23445515355,82.526795931394));
#124143=CARTESIAN_POINT('Ctrl Pts',(9.2478073367568,-19.9999999999995,82.8003857022309));
#124144=CARTESIAN_POINT('Ctrl Pts',(9.44746232363843,-19.9999947893509,
82.7651858109517));
#124145=CARTESIAN_POINT('Ctrl Pts',(9.63275874640372,-20.0102049333749,
82.732512666375));
#124146=CARTESIAN_POINT('Ctrl Pts',(9.8878093209807,-20.0353935839062,82.6875380030807));
#124147=CARTESIAN_POINT('Ctrl Pts',(9.96902609894511,-20.0454254995066,
82.6732164866477));
#124148=CARTESIAN_POINT('Ctrl Pts',(10.0850995196626,-20.0622046672562,
82.6527499742875));
#124149=CARTESIAN_POINT('Ctrl Pts',(10.1228331636278,-20.0680856223673,
82.6460969388893));
#124150=CARTESIAN_POINT('Ctrl Pts',(10.1779943238935,-20.0772527547499,
82.6363715837551));
#124151=CARTESIAN_POINT('Ctrl Pts',(10.1961413085924,-20.0803664121402,
82.6331721758484));
#124152=CARTESIAN_POINT('Ctrl Pts',(10.2319541510883,-20.0866967255136,
82.6268581999328));
#124153=CARTESIAN_POINT('Ctrl Pts',(10.2510600419059,-20.0901829259522,
82.6234897459459));
#124154=CARTESIAN_POINT('Ctrl Pts',(10.3949250479738,-20.1171116810494,
82.59812551849));
#124155=CARTESIAN_POINT('Ctrl Pts',(10.5440152508577,-20.149477090711,82.5718364035666));
#124156=CARTESIAN_POINT('Ctrl Pts',(10.7965591891663,-20.2221388834674,
82.5272998102366));
#124157=CARTESIAN_POINT('Ctrl Pts',(10.8855418190081,-20.2504210618513,
82.5116080062251));
#124158=CARTESIAN_POINT('Ctrl Pts',(11.0254757509608,-20.3008841383642,
82.4869377685761));
#124159=CARTESIAN_POINT('Ctrl Pts',(11.0731867261691,-20.319054786091,82.4785267513243));
#124160=CARTESIAN_POINT('Ctrl Pts',(11.146183705256,-20.348647486402,82.4656568172526));
#124161=CARTESIAN_POINT('Ctrl Pts',(11.1830392891995,-20.3640284868325,
82.4591586062959));
#124162=CARTESIAN_POINT('Ctrl Pts',(11.226619501312,-20.3830693031182,82.4514740645984));
#124163=CARTESIAN_POINT('Ctrl Pts',(11.2454164624666,-20.3914727212221,
82.4481594349195));
#124164=CARTESIAN_POINT('Ctrl Pts',(11.2579738094765,-20.3971299277008,
82.4459450591596));
#124165=CARTESIAN_POINT('Ctrl Pts',(11.2657286922385,-20.4006553367271,
82.4445775325265));
#124166=CARTESIAN_POINT('Ctrl Pts',(11.3480297246391,-20.4383043456372,
82.4300640878185));
#124167=CARTESIAN_POINT('Ctrl Pts',(11.421888665082,-20.4753509528145,82.4170367346209));
#124168=CARTESIAN_POINT('Ctrl Pts',(11.5272732330714,-20.5327179132995,
82.3984528739781));
#124169=CARTESIAN_POINT('Ctrl Pts',(11.561502672334,-20.5521388404709,82.3924175625728));
#124170=CARTESIAN_POINT('Ctrl Pts',(11.6031750904849,-20.5767194020878,
82.3850720577672));
#124171=CARTESIAN_POINT('Ctrl Pts',(11.6123888516415,-20.58221902437,82.3834480849646));
#124172=CARTESIAN_POINT('Ctrl Pts',(11.6240309445655,-20.5892103236488,
82.3813961661963));
#124173=CARTESIAN_POINT('Ctrl Pts',(11.6419615202763,-20.6000380415341,
82.3782359971482));
#124174=CARTESIAN_POINT('Ctrl Pts',(11.6612775281911,-20.6119196074362,
82.3748318879259));
#124175=CARTESIAN_POINT('Ctrl Pts',(11.7017026635763,-20.6371825857324,
82.367707745307));
#124176=CARTESIAN_POINT('Ctrl Pts',(11.7310477696397,-20.6560203002695,
82.3625363705117));
#124177=CARTESIAN_POINT('Ctrl Pts',(11.7783737270488,-20.6877204153845,
82.354195088854));
#124178=CARTESIAN_POINT('Ctrl Pts',(11.7946994328715,-20.6988620468004,
82.3513174598515));
#124179=CARTESIAN_POINT('Ctrl Pts',(11.8283908526668,-20.7223825537064,
82.3453782383267));
#124180=CARTESIAN_POINT('Ctrl Pts',(11.8401311157668,-20.7307794729597,
82.3433083872193));
#124181=CARTESIAN_POINT('Ctrl Pts',(11.8792669632643,-20.759194418091,82.3364080799073));
#124182=CARTESIAN_POINT('Ctrl Pts',(11.9179182184663,-20.7883420314512,
82.3295918309551));
#124183=CARTESIAN_POINT('Ctrl Pts',(11.9620834760337,-20.8236468981876,
82.3218011143799));
#124184=CARTESIAN_POINT('Ctrl Pts',(11.9839243744912,-20.8416259125265,
82.3179480447014));
#124185=CARTESIAN_POINT('Ctrl Pts',(11.9932319197662,-20.8494013637813,
82.3163059961232));
#124186=CARTESIAN_POINT('Ctrl Pts',(11.9994250927753,-20.8546006075963,
82.3152133794341));
#124187=CARTESIAN_POINT('Ctrl Pts',(12.0039591773524,-20.8584317976343,
82.3144134551576));
#124188=CARTESIAN_POINT('Ctrl Pts',(12.0318603467978,-20.8820869136747,
82.3094909807558));
#124189=CARTESIAN_POINT('Ctrl Pts',(12.0824933910368,-20.9240074051633,
82.3005552708056));
#124190=CARTESIAN_POINT('Ctrl Pts',(12.1616638165423,-21.0000768353195,
82.2865925876594));
#124191=CARTESIAN_POINT('Ctrl Pts',(12.1707604794478,-21.0089379861606,
82.2849883614701));
#124192=CARTESIAN_POINT('Ctrl Pts',(12.1895177034974,-21.0275141712816,
82.2816805550659));
#124193=CARTESIAN_POINT('Ctrl Pts',(12.1938078445007,-21.0318455932408,
82.2809240187919));
#124194=CARTESIAN_POINT('Ctrl Pts',(12.2118934559253,-21.0501437800382,
82.2777347242169));
#124195=CARTESIAN_POINT('Ctrl Pts',(12.2236629025068,-21.0622900912216,
82.2756592661729));
#124196=CARTESIAN_POINT('Ctrl Pts',(12.2581217968457,-21.0985357629434,
82.2695825526892));
#124197=CARTESIAN_POINT('Ctrl Pts',(12.2809075638514,-21.1235159463043,
82.2655641269728));
#124198=CARTESIAN_POINT('Ctrl Pts',(12.3799394395816,-21.2359287811547,
82.2480979874625));
#124199=CARTESIAN_POINT('Ctrl Pts',(12.4526737390527,-21.3312614384013,
82.2352611547935));
#124200=CARTESIAN_POINT('Ctrl Pts',(12.5172257454391,-21.43204530223,82.22390472213));
#124201=CARTESIAN_POINT('Ctrl Pts',(10.7887201262991,-22.10443025328,82.17467014195));
#124202=CARTESIAN_POINT('Ctrl Pts',(10.8047337967191,-22.08320647671,82.173219921734));
#124203=CARTESIAN_POINT('Ctrl Pts',(11.0973679846591,-21.6977322454,82.146617864881));
#124204=CARTESIAN_POINT('Ctrl Pts',(11.6742414050491,-21.01672713982,82.090586401544));
#124205=CARTESIAN_POINT('Ctrl Pts',(12.5401712418891,-20.15025725843,81.996296778919));
#124206=CARTESIAN_POINT('Ctrl Pts',(13.3705524233291,-19.42440302238,81.897353491595));
#124207=CARTESIAN_POINT('Ctrl Pts',(14.1538154081591,-18.81497810678,81.7971741645661));
#124208=CARTESIAN_POINT('Ctrl Pts',(14.8829524524591,-18.30350003294,81.698540745942));
#124209=CARTESIAN_POINT('Ctrl Pts',(15.5555809773291,-17.87418996261,81.6034015345329));
#124210=CARTESIAN_POINT('Ctrl Pts',(16.1720623735391,-17.513706038,81.513033347234));
#124211=CARTESIAN_POINT('Ctrl Pts',(16.7343651483591,-17.21078913064,81.4281925355089));
#124212=CARTESIAN_POINT('Ctrl Pts',(17.2456693404391,-16.95583958766,81.349208818485));
#124213=CARTESIAN_POINT('Ctrl Pts',(17.6465406780691,-16.77007568858,81.2860730452739));
#124214=CARTESIAN_POINT('Ctrl Pts',(17.8774928558391,-16.66870970371,81.2492359042699));
#124215=CARTESIAN_POINT('Ctrl Pts',(17.9533920306691,-16.63600339584,81.237081512272));
#124216=CARTESIAN_POINT('Ctrl Pts',(11.5977514399991,-22.56749970211,82.742377900034));
#124217=CARTESIAN_POINT('Ctrl Pts',(11.6135348286791,-22.54809608191,82.73977119412));
#124218=CARTESIAN_POINT('Ctrl Pts',(11.9019007421091,-22.19570125639,82.692043649529));
#124219=CARTESIAN_POINT('Ctrl Pts',(12.4682941702191,-21.57382709283,82.59463865837));
#124220=CARTESIAN_POINT('Ctrl Pts',(13.3124318802591,-20.78368851256,82.4397023567349));
#124221=CARTESIAN_POINT('Ctrl Pts',(14.1165688943791,-20.12241917829,82.284501810265));
#124222=CARTESIAN_POINT('Ctrl Pts',(14.8705665392591,-19.56763806237,82.13324984309));
#124223=CARTESIAN_POINT('Ctrl Pts',(15.5687371062291,-19.10232611625,81.989006399952));
#124224=CARTESIAN_POINT('Ctrl Pts',(16.2097847874691,-18.71200397957,81.853549425408));
#124225=CARTESIAN_POINT('Ctrl Pts',(16.7949185413491,-18.38444768917,81.727752369711));
#124226=CARTESIAN_POINT('Ctrl Pts',(17.3267225057291,-18.10935418506,81.611888543045));
#124227=CARTESIAN_POINT('Ctrl Pts',(17.8087865331191,-17.87794738429,81.505773672536));
#124228=CARTESIAN_POINT('Ctrl Pts',(18.1857031536891,-17.70942521826,81.4221360479911));
#124229=CARTESIAN_POINT('Ctrl Pts',(18.4024472122491,-17.61750301323,81.373802591825));
#124230=CARTESIAN_POINT('Ctrl Pts',(18.4736338331591,-17.58784766122,81.357904139968));
#124231=CARTESIAN_POINT('Ctrl Pts',(12.4259640368191,-23.15463944465,82.3416426964909));
#124232=CARTESIAN_POINT('Ctrl Pts',(12.4401412767391,-23.13665861788,82.33780158716));
#124233=CARTESIAN_POINT('Ctrl Pts',(12.6992171930991,-22.80992651895,82.2675629739351));
#124234=CARTESIAN_POINT('Ctrl Pts',(13.2099574421591,-22.22741757786,82.127448594009));
#124235=CARTESIAN_POINT('Ctrl Pts',(13.9753360388591,-21.47531598229,81.913721537321));
#124236=CARTESIAN_POINT('Ctrl Pts',(14.7074100844491,-20.8373796579,81.707070463445));
#124237=CARTESIAN_POINT('Ctrl Pts',(15.3960509033691,-20.29596035334,81.511532543162));
#124238=CARTESIAN_POINT('Ctrl Pts',(16.0354203056491,-19.83722693452,81.329600240346));
#124239=CARTESIAN_POINT('Ctrl Pts',(16.6238567262691,-19.44888644012,81.162238962755));
#124240=CARTESIAN_POINT('Ctrl Pts',(17.1621028148391,-19.12021905677,81.0094715701341));
#124241=CARTESIAN_POINT('Ctrl Pts',(17.6522333898591,-18.84198037761,80.870794099851));
#124242=CARTESIAN_POINT('Ctrl Pts',(18.0973044970791,-18.60613730024,80.745333020243));
#124243=CARTESIAN_POINT('Ctrl Pts',(18.4458601500391,-18.43311625794,80.647472162088));
#124244=CARTESIAN_POINT('Ctrl Pts',(18.6465294124491,-18.33821558922,80.591313309216));
#124245=CARTESIAN_POINT('Ctrl Pts',(18.7124620135991,-18.30754110383,80.572882098526));
#124246=CARTESIAN_POINT('Ctrl Pts',(12.6103453412591,-23.3958239894,81.2932667992599));
#124247=CARTESIAN_POINT('Ctrl Pts',(12.6228263425391,-23.37772959822,81.289101551044));
#124248=CARTESIAN_POINT('Ctrl Pts',(12.8510381860091,-23.0486996543,81.212987170427));
#124249=CARTESIAN_POINT('Ctrl Pts',(13.3055043469091,-22.45427700608,81.063017870605));
#124250=CARTESIAN_POINT('Ctrl Pts',(13.9982062138891,-21.67146816858,80.839419997635));
#124251=CARTESIAN_POINT('Ctrl Pts',(14.6700873664091,-20.9969340879,80.627313039042));
#124252=CARTESIAN_POINT('Ctrl Pts',(15.3096002530191,-20.41689801836,80.4297282763071));
#124253=CARTESIAN_POINT('Ctrl Pts',(15.9094061513291,-19.91988918978,80.2481995028229));
#124254=CARTESIAN_POINT('Ctrl Pts',(16.4663180120191,-19.4949376737,80.082887870565));
#124255=CARTESIAN_POINT('Ctrl Pts',(16.9796715957291,-19.13200993825,79.933199351765));
#124256=CARTESIAN_POINT('Ctrl Pts',(17.4503151792491,-18.82217532617,79.798180712975));
#124257=CARTESIAN_POINT('Ctrl Pts',(17.8802547115591,-18.55746834489,79.676645672238));
#124258=CARTESIAN_POINT('Ctrl Pts',(18.2187470731791,-18.36180932168,79.582226384286));
#124259=CARTESIAN_POINT('Ctrl Pts',(18.4143432878591,-18.25389230802,79.52817755149));
#124260=CARTESIAN_POINT('Ctrl Pts',(18.4786864263191,-18.21894445124,79.510452443262));
#124261=CARTESIAN_POINT('',(15.1826284143117,-20.4790209964007,80.7654348671615));
#124262=CARTESIAN_POINT('',(13.3597754116033,-20.4707120255044,82.0753347888772));
#124263=CARTESIAN_POINT('Ctrl Pts',(15.1826281951692,-20.4790210042571,
80.7654347832022));
#124264=CARTESIAN_POINT('Ctrl Pts',(15.1191106435012,-20.4831595772132,
80.9316095253303));
#124265=CARTESIAN_POINT('Ctrl Pts',(15.0202333632624,-20.4881017533022,
81.0852214233996));
#124266=CARTESIAN_POINT('Ctrl Pts',(14.7692951009453,-20.496465001043,81.3804070169615));
#124267=CARTESIAN_POINT('Ctrl Pts',(14.6067129985061,-20.4996164325595,
81.5206692599665));
#124268=CARTESIAN_POINT('Ctrl Pts',(14.2708648919509,-20.5002922526295,
81.7486174057977));
#124269=CARTESIAN_POINT('Ctrl Pts',(14.0952875735918,-20.4982343136608,
81.8417267900461));
#124270=CARTESIAN_POINT('Ctrl Pts',(13.7352155159587,-20.4885488872977,
81.9876049764954));
#124271=CARTESIAN_POINT('Ctrl Pts',(13.5489239184334,-20.4809898307412,
82.041981658877));
#124272=CARTESIAN_POINT('Ctrl Pts',(13.359775386349,-20.470712025504,82.0753346456572));
#124273=CARTESIAN_POINT('Ctrl Pts',(12.6211112025166,-23.1949844434374,
81.546651511011));
#124274=CARTESIAN_POINT('Ctrl Pts',(12.7010796583489,-23.0859335125774,
81.5217614922825));
#124275=CARTESIAN_POINT('Ctrl Pts',(12.7873020478414,-22.9720163830221,
81.4948559993584));
#124276=CARTESIAN_POINT('Ctrl Pts',(12.8801975478467,-22.8535598950672,
81.4659316626286));
#124277=CARTESIAN_POINT('Ctrl Pts',(12.9693469700448,-22.7398802501308,
81.4381737205671));
#124278=CARTESIAN_POINT('Ctrl Pts',(13.0646433628694,-22.6220200826152,
81.4085560004937));
#124279=CARTESIAN_POINT('Ctrl Pts',(13.1664350211465,-22.5002998917991,
81.3770989552872));
#124280=CARTESIAN_POINT('Ctrl Pts',(13.2060171790742,-22.4529684316637,
81.3648667375164));
#124281=CARTESIAN_POINT('Ctrl Pts',(13.2465829275287,-22.4050546552067,
81.3523520386674));
#124282=CARTESIAN_POINT('Ctrl Pts',(13.2881527164378,-22.3565825378578,
81.3395481591552));
#124283=CARTESIAN_POINT('Ctrl Pts',(13.3557321339824,-22.2777821026487,
81.3187330734294));
#124284=CARTESIAN_POINT('Ctrl Pts',(13.4259653175262,-22.197505741631,81.2971535838656));
#124285=CARTESIAN_POINT('Ctrl Pts',(13.4989513338155,-22.115863929788,81.2747791284266));
#124286=CARTESIAN_POINT('Ctrl Pts',(13.5578921034289,-22.0499330642976,
81.256710357307));
#124287=CARTESIAN_POINT('Ctrl Pts',(13.6186279276438,-21.9831129698786,
81.2381219473619));
#124288=CARTESIAN_POINT('Ctrl Pts',(13.6812085868739,-21.9154695454829,
81.2189866650971));
#124289=CARTESIAN_POINT('Ctrl Pts',(13.712498916489,-21.881647833285,81.2094190239647));
#124290=CARTESIAN_POINT('Ctrl Pts',(13.7442504334845,-21.847620273801,81.1997146534683));
#124291=CARTESIAN_POINT('Ctrl Pts',(13.7764690753335,-21.8133956591303,
81.1898691502691));
#124292=CARTESIAN_POINT('Ctrl Pts',(13.7925783962579,-21.7962833517949,
81.1849463986695));
#124293=CARTESIAN_POINT('Ctrl Pts',(13.8088044961137,-21.7791217787972,
81.1799883628294));
#124294=CARTESIAN_POINT('Ctrl Pts',(13.8251480981321,-21.7619120485684,
81.1749944576721));
#124295=CARTESIAN_POINT('Ctrl Pts',(13.8333198991413,-21.7533071834539,
81.1724975050935));
#124296=CARTESIAN_POINT('Ctrl Pts',(13.8415210755324,-21.7446902788946,
81.1699915851153));
#124297=CARTESIAN_POINT('Ctrl Pts',(13.8497517162525,-21.7360614749796,
81.1674766209594));
#124298=CARTESIAN_POINT('Ctrl Pts',(13.8538670366125,-21.7317470730221,
81.1662191388814));
#124299=CARTESIAN_POINT('Ctrl Pts',(13.8579897230441,-21.7274296962161,
81.1649593957544));
#124300=CARTESIAN_POINT('Ctrl Pts',(13.8621197865673,-21.7231093621754,
81.1636973817387));
#124301=CARTESIAN_POINT('Ctrl Pts',(13.8662498500906,-21.7187890281346,
81.162435367723));
#124302=CARTESIAN_POINT('Ctrl Pts',(13.8718575245007,-21.7129311569294,
81.1607218127025));
#124303=CARTESIAN_POINT('Ctrl Pts',(13.8745321193775,-21.7101395059708,
81.1599045171018));
#124304=CARTESIAN_POINT('Ctrl Pts',(13.9127985873755,-21.6701982711336,
81.1482111514188));
#124305=CARTESIAN_POINT('Ctrl Pts',(13.9540072554889,-21.6275871585619,
81.1356238056198));
#124306=CARTESIAN_POINT('Ctrl Pts',(13.9982420814259,-21.5823867839551,
81.1221332886392));
#124307=CARTESIAN_POINT('Ctrl Pts',(14.0529431604893,-21.5264917010042,
81.1054508258889));
#124308=CARTESIAN_POINT('Ctrl Pts',(14.112271257553,-21.4666361954175,81.0873872566257));
#124309=CARTESIAN_POINT('Ctrl Pts',(14.1764050690305,-21.4029997983481,
81.0679228150623));
#124310=CARTESIAN_POINT('Ctrl Pts',(14.2344033461055,-21.3454513491875,
81.0503204919055));
#124311=CARTESIAN_POINT('Ctrl Pts',(14.2963323407058,-21.2848124726741,
81.0315700508687));
#124312=CARTESIAN_POINT('Ctrl Pts',(14.362335166225,-21.221246127599,81.0116327158677));
#124313=CARTESIAN_POINT('Ctrl Pts',(14.3953365789847,-21.1894629550614,
81.0016640483672));
#124314=CARTESIAN_POINT('Ctrl Pts',(14.4293565867576,-21.1569483381342,
80.9913983362014));
#124315=CARTESIAN_POINT('Ctrl Pts',(14.4644136947065,-21.1237252347141,
80.9808285409277));
#124316=CARTESIAN_POINT('Ctrl Pts',(14.4819422486809,-21.107113683004,80.9755436432908));
#124317=CARTESIAN_POINT('Ctrl Pts',(14.4997300874212,-21.0903250186968,
80.9701827288884));
#124318=CARTESIAN_POINT('Ctrl Pts',(14.5177795393016,-21.0733622970361,
80.9647447272958));
#124319=CARTESIAN_POINT('Ctrl Pts',(14.5268042652417,-21.0648809362057,
80.9620257264995));
#124320=CARTESIAN_POINT('Ctrl Pts',(14.5358943949757,-21.0563560614945,
80.9592874541226));
#124321=CARTESIAN_POINT('Ctrl Pts',(14.5450502210561,-21.0477880619624,
80.9565297708572));
#124322=CARTESIAN_POINT('Ctrl Pts',(14.5496281340964,-21.0435040621964,
80.9551509292245));
#124323=CARTESIAN_POINT('Ctrl Pts',(14.5542224712529,-21.0392092812524,
80.953767234882));
#124324=CARTESIAN_POINT('Ctrl Pts',(14.5588332691131,-21.0349037684304,
80.9523786696975));
#124325=CARTESIAN_POINT('Ctrl Pts',(14.5634440669733,-21.0305982556084,
80.9509901045129));
#124326=CARTESIAN_POINT('Ctrl Pts',(14.5671550748878,-21.0271357486057,
80.9498725694768));
#124327=CARTESIAN_POINT('Ctrl Pts',(14.5727150814534,-21.0219550838904,
80.9481983432867));
#124328=CARTESIAN_POINT('Ctrl Pts',(14.6124113807312,-20.9849671389,80.9362450149736));
#124329=CARTESIAN_POINT('Ctrl Pts',(14.6503266609049,-20.9499779898511,
80.9248393076686));
#124330=CARTESIAN_POINT('Ctrl Pts',(14.6864107610285,-20.9169365199115,
80.9139933493658));
#124331=CARTESIAN_POINT('Ctrl Pts',(14.7443878671627,-20.863848073672,80.8965669129716));
#124332=CARTESIAN_POINT('Ctrl Pts',(14.7976358817662,-20.8157860004258,
80.880585953442));
#124333=CARTESIAN_POINT('Ctrl Pts',(14.8459839415778,-20.7725674980799,
80.8660905655735));
#124334=CARTESIAN_POINT('Ctrl Pts',(14.8949868311436,-20.7287636410915,
80.8513988510827));
#124335=CARTESIAN_POINT('Ctrl Pts',(14.9389562888953,-20.6899353059313,
80.8382331285868));
#124336=CARTESIAN_POINT('Ctrl Pts',(14.977753356939,-20.655927835926,80.8266253191512));
#124337=CARTESIAN_POINT('Ctrl Pts',(15.0167645805568,-20.6217326484042,
80.8149534358764));
#124338=CARTESIAN_POINT('Ctrl Pts',(15.0505463171594,-20.5924116099799,
80.804856625578));
#124339=CARTESIAN_POINT('Ctrl Pts',(15.0789939351,-20.5678449536711,80.796358861458));
#124340=CARTESIAN_POINT('Ctrl Pts',(15.1076083817696,-20.5431342282155,
80.7878112628952));
#124341=CARTESIAN_POINT('Ctrl Pts',(15.1308260759889,-20.5232337366539,
80.78088145753));
#124342=CARTESIAN_POINT('Ctrl Pts',(15.1485754243984,-20.5080606018071,
80.7755864184812));
#124343=CARTESIAN_POINT('Ctrl Pts',(15.1641398050169,-20.4947552995232,
80.7709432056013));
#124344=CARTESIAN_POINT('Ctrl Pts',(15.1754998459937,-20.4850856751023,
80.7675569223367));
#124345=CARTESIAN_POINT('Ctrl Pts',(15.1826283063839,-20.4790208829906,
80.7654348287324));
#124346=CARTESIAN_POINT('Ctrl Pts',(12.5172248390746,-21.4320453024142,
82.2238995806392));
#124347=CARTESIAN_POINT('Ctrl Pts',(12.6294093254391,-21.2933908624356,
82.2041182404801));
#124348=CARTESIAN_POINT('Ctrl Pts',(12.7416585985438,-21.1594801400756,
82.1843245397865));
#124349=CARTESIAN_POINT('Ctrl Pts',(12.8535950144248,-21.0300306251832,
82.164587125004));
#124350=CARTESIAN_POINT('Ctrl Pts',(12.9612121273082,-20.9055761931985,
82.145611320053));
#124351=CARTESIAN_POINT('Ctrl Pts',(13.0685405940468,-20.785245355736,82.1266873294237));
#124352=CARTESIAN_POINT('Ctrl Pts',(13.175286560664,-20.6688012397128,82.1078652991768));
#124353=CARTESIAN_POINT('Ctrl Pts',(13.1820061662658,-20.6614711404209,
82.1066804617174));
#124354=CARTESIAN_POINT('Ctrl Pts',(13.1887234763875,-20.6541564475408,
82.1054960251714));
#124355=CARTESIAN_POINT('Ctrl Pts',(13.1954384320464,-20.6468571100375,
82.1043120005116));
#124356=CARTESIAN_POINT('Ctrl Pts',(13.2503880070708,-20.5871254432717,
82.0946229340191));
#124357=CARTESIAN_POINT('Ctrl Pts',(13.305175381437,-20.5284202730709,82.084962261829));
#124358=CARTESIAN_POINT('Ctrl Pts',(13.3597753863499,-20.4707120255048,
82.0753346456571));
#124359=CARTESIAN_POINT('Origin',(22.8854471965091,-9.5,80.840271512642));
#124360=CARTESIAN_POINT('',(21.1895064189391,-9.49999999533099,65.4633429305539));
#124361=CARTESIAN_POINT('',(20.0012895469927,-9.49999999792378,58.7246301887194));
#124362=CARTESIAN_POINT('',(24.2283495281091,-9.49999999533099,82.697478608263));
#124363=CARTESIAN_POINT('',(20.2047119979795,-8.50000000009162,65.6369887574203));
#124364=CARTESIAN_POINT('Origin',(20.2046986659336,-9.5,65.6369911082197));
#124365=CARTESIAN_POINT('',(19.0165457197942,-8.50000000044727,58.8982964289324));
#124366=CARTESIAN_POINT('Ctrl Pts',(20.2047119979795,-8.50000000009162,
65.6369887574203));
#124367=CARTESIAN_POINT('Ctrl Pts',(19.8086377232276,-8.50000000004136,
63.3907613048375));
#124368=CARTESIAN_POINT('Ctrl Pts',(19.4125634484756,-8.50000000001177,
61.1445338522548));
#124369=CARTESIAN_POINT('Ctrl Pts',(19.0165457198591,-8.5,58.89829642895));
#124370=CARTESIAN_POINT('Ctrl Pts',(20.0012895473071,-9.49999999792378,
58.7246301886641));
#124371=CARTESIAN_POINT('Ctrl Pts',(20.0012899795185,-9.46762591868316,
58.7246326402436));
#124372=CARTESIAN_POINT('Ctrl Pts',(19.9997391442553,-9.43457989065709,
58.7249081307818));
#124373=CARTESIAN_POINT('Ctrl Pts',(19.9964623697764,-9.40109896318049,
58.725487577709));
#124374=CARTESIAN_POINT('Ctrl Pts',(19.9932143516384,-9.36791185786638,
58.7260619395216));
#124375=CARTESIAN_POINT('Ctrl Pts',(19.9882701017658,-9.33429788673468,
58.7269350260154));
#124376=CARTESIAN_POINT('Ctrl Pts',(19.9814984743018,-9.3005197579655,58.728130076751));
#124377=CARTESIAN_POINT('Ctrl Pts',(19.9747974261233,-9.26709369171103,
58.7293126717177));
#124378=CARTESIAN_POINT('Ctrl Pts',(19.966306563625,-9.23350740803131,58.7308106127281));
#124379=CARTESIAN_POINT('Ctrl Pts',(19.9559429296749,-9.20003957605674,
58.7326386388117));
#124380=CARTESIAN_POINT('Ctrl Pts',(19.9488851771946,-9.17724760219227,
58.7338835453463));
#124381=CARTESIAN_POINT('Ctrl Pts',(19.9409598030488,-9.15451106970619,
58.7352813743508));
#124382=CARTESIAN_POINT('Ctrl Pts',(19.932153557986,-9.13192242870445,58.7368344972254));
#124383=CARTESIAN_POINT('Ctrl Pts',(19.9201566287579,-9.10114945730447,
58.738950348542));
#124384=CARTESIAN_POINT('Ctrl Pts',(19.9065243780912,-9.07065704605179,
58.7413544985239));
#124385=CARTESIAN_POINT('Ctrl Pts',(19.8912777345561,-9.04071403997275,
58.7440432534581));
#124386=CARTESIAN_POINT('Ctrl Pts',(19.8761507537896,-9.01100604056889,
58.7467109057897));
#124387=CARTESIAN_POINT('Ctrl Pts',(19.8594347467946,-8.98183953430048,
58.7496586911272));
#124388=CARTESIAN_POINT('Ctrl Pts',(19.8412003847823,-8.95346833657049,
58.7528741448684));
#124389=CARTESIAN_POINT('Ctrl Pts',(19.8227496569657,-8.92476049108652,
58.7561277526309));
#124390=CARTESIAN_POINT('Ctrl Pts',(19.8027444542824,-8.89686767177941,
58.7596553963031));
#124391=CARTESIAN_POINT('Ctrl Pts',(19.781307980834,-8.8700331238014,58.7634353481959));
#124392=CARTESIAN_POINT('Ctrl Pts',(19.7598715073857,-8.84319857582339,
58.7672153000887));
#124393=CARTESIAN_POINT('Ctrl Pts',(19.7370041494664,-8.81742294259417,
58.7712474920879));
#124394=CARTESIAN_POINT('Ctrl Pts',(19.7128747804019,-8.79291951777192,
58.7755021437878));
#124395=CARTESIAN_POINT('Ctrl Pts',(19.6888397304775,-8.76851187423399,
58.7797401645063));
#124396=CARTESIAN_POINT('Ctrl Pts',(19.6635614323748,-8.74537551707984,
58.7841973371116));
#124397=CARTESIAN_POINT('Ctrl Pts',(19.6372473957868,-8.72368004516574,
58.7888370761684));
#124398=CARTESIAN_POINT('Ctrl Pts',(19.61117460253,-8.70218347424117,58.7934342787599));
#124399=CARTESIAN_POINT('Ctrl Pts',(19.5840856193093,-8.68210179550079,
58.7982106020061));
#124400=CARTESIAN_POINT('Ctrl Pts',(19.5562104876184,-8.66355581926994,
58.8031254873951));
#124401=CARTESIAN_POINT('Ctrl Pts',(19.5279484762274,-8.64475244293768,
58.8081085866101));
#124402=CARTESIAN_POINT('Ctrl Pts',(19.4988789808644,-8.62752803875613,
58.813234008398));
#124403=CARTESIAN_POINT('Ctrl Pts',(19.4692613061491,-8.61195770978641,
58.8184560345373));
#124404=CARTESIAN_POINT('Ctrl Pts',(19.4396436314338,-8.59638738081669,
58.8236780606767));
#124405=CARTESIAN_POINT('Ctrl Pts',(19.409478491668,-8.58247119127859,58.8289965652168));
#124406=CARTESIAN_POINT('Ctrl Pts',(19.3790342951517,-8.57023085295102,
58.8343642247118));
#124407=CARTESIAN_POINT('Ctrl Pts',(19.3463554205598,-8.55709204401731,
58.8401258834697));
#124408=CARTESIAN_POINT('Ctrl Pts',(19.3133623206699,-8.54588566789205,
58.8459428927352));
#124409=CARTESIAN_POINT('Ctrl Pts',(19.2803417007415,-8.53656112194488,
58.8517651620618));
#124410=CARTESIAN_POINT('Ctrl Pts',(19.2471142663819,-8.5271781745906,58.8576238973702));
#124411=CARTESIAN_POINT('Ctrl Pts',(19.2138595521797,-8.51970040815207,
58.8634878555077));
#124412=CARTESIAN_POINT('Ctrl Pts',(19.1808509606665,-8.51402658730199,
58.8693093004204));
#124413=CARTESIAN_POINT('Ctrl Pts',(19.147412530532,-8.50827888182916,58.8752065523197));
#124414=CARTESIAN_POINT('Ctrl Pts',(19.1142272133837,-8.50438203527085,
58.8810600816113));
#124415=CARTESIAN_POINT('Ctrl Pts',(19.0815514632307,-8.50218500580683,
58.8868251594106));
#124416=CARTESIAN_POINT('Ctrl Pts',(19.0596311897744,-8.50071114563782,
58.8906926171205));
#124417=CARTESIAN_POINT('Ctrl Pts',(19.0379396363874,-8.50000130130795,
58.8945203748651));
#124418=CARTESIAN_POINT('Ctrl Pts',(19.016545719859,-8.50000000178909,58.89829642895));
#124419=CARTESIAN_POINT('Origin',(23.0888233837291,-10.,78.836701365196));
#124420=CARTESIAN_POINT('',(-3.18510217627065,-9.99999863269069,84.9926432467801));
#124421=CARTESIAN_POINT('',(-4.19326724970536,-8.5,83.6472700340011));
#124422=CARTESIAN_POINT('Ctrl Pts',(-3.18510142355444,-10.,84.9926431156534));
#124423=CARTESIAN_POINT('Ctrl Pts',(-3.28774654871392,-9.81347742952627,
85.0107420480117));
#124424=CARTESIAN_POINT('Ctrl Pts',(-3.40138324898531,-9.61104424048628,
84.9933696737421));
#124425=CARTESIAN_POINT('Ctrl Pts',(-3.6218722462137,-9.23231631838246,
84.8715546372826));
#124426=CARTESIAN_POINT('Ctrl Pts',(-3.72887381127769,-9.05615862658819,
84.7669564448341));
#124427=CARTESIAN_POINT('Ctrl Pts',(-3.90143678101031,-8.79358573018847,
84.5186556652058));
#124428=CARTESIAN_POINT('Ctrl Pts',(-3.98029199297708,-8.68400566943748,
84.3669625950309));
#124429=CARTESIAN_POINT('Ctrl Pts',(-4.10991781742065,-8.53714553683044,
84.0232533567387));
#124430=CARTESIAN_POINT('Ctrl Pts',(-4.16082961889395,-8.5,83.8312329798933));
#124431=CARTESIAN_POINT('Ctrl Pts',(-4.19326724970496,-8.5,83.6472700340034));
#124432=CARTESIAN_POINT('',(-6.54682286478236,-9.99999999999981,85.5854053073669));
#124433=CARTESIAN_POINT('',(-1.48527513867091,-9.99999794132199,84.6929178719));
#124434=CARTESIAN_POINT('',(-6.8072945644184,-8.50000000000003,84.1081934941563));
#124435=CARTESIAN_POINT('Origin',(-6.80729512863291,-10.,84.10819367738));
#124436=CARTESIAN_POINT('',(-2.24409325564091,-8.5,83.30357806876));
#124437=CARTESIAN_POINT('Ctrl Pts',(19.9312442464691,-9.83434173672299,
58.58808248603));
#124438=CARTESIAN_POINT('Ctrl Pts',(19.9318133015791,-9.83251988519099,
58.59130975793));
#124439=CARTESIAN_POINT('Ctrl Pts',(19.9372671952991,-9.81590682367799,
58.62224032621));
#124440=CARTESIAN_POINT('Ctrl Pts',(19.9474515848891,-9.79777453008298,
58.67999886974));
#124441=CARTESIAN_POINT('Ctrl Pts',(19.9576520930091,-9.79674919137799,
58.73784882602));
#124442=CARTESIAN_POINT('Ctrl Pts',(19.9616392603091,-9.79878222958499,
58.76046117542));
#124443=CARTESIAN_POINT('Ctrl Pts',(20.1262752009291,-9.06820471416898,
58.12191241983));
#124444=CARTESIAN_POINT('Ctrl Pts',(20.1286905848491,-9.06047995653799,
58.13561074275));
#124445=CARTESIAN_POINT('Ctrl Pts',(20.1516207901991,-8.99069547653899,
58.26565439945));
#124446=CARTESIAN_POINT('Ctrl Pts',(20.1910945955491,-8.92247834065099,
58.48952147411));
#124447=CARTESIAN_POINT('Ctrl Pts',(20.2290936722891,-8.91832092631999,
58.70502494718));
#124448=CARTESIAN_POINT('Ctrl Pts',(20.2440720102891,-8.926020544672,58.7899713231901));
#124449=CARTESIAN_POINT('Ctrl Pts',(19.4324748633591,-8.50077447479,57.9244548090799));
#124450=CARTESIAN_POINT('Ctrl Pts',(19.4362577086691,-8.48867780022699,
57.94590839094));
#124451=CARTESIAN_POINT('Ctrl Pts',(19.4721315355791,-8.37951254390298,
58.14935897332));
#124452=CARTESIAN_POINT('Ctrl Pts',(19.5332981970591,-8.27420066749899,
58.49625234851));
#124453=CARTESIAN_POINT('Ctrl Pts',(19.5918859517691,-8.267723518747,58.8285200166801));
#124454=CARTESIAN_POINT('Ctrl Pts',(19.6150047691491,-8.27962002203299,
58.95963334533));
#124455=CARTESIAN_POINT('Ctrl Pts',(18.5925509242691,-8.73948053367298,
58.2070864406));
#124456=CARTESIAN_POINT('Ctrl Pts',(18.5957585071091,-8.72922303331798,
58.22527754688));
#124457=CARTESIAN_POINT('Ctrl Pts',(18.6261872225791,-8.63662444767899,
58.3978473677));
#124458=CARTESIAN_POINT('Ctrl Pts',(18.6782281522391,-8.54691755440599,
58.69298614594));
#124459=CARTESIAN_POINT('Ctrl Pts',(18.7281546798291,-8.54141626950999,
58.97613355421));
#124460=CARTESIAN_POINT('Ctrl Pts',(18.7478489674291,-8.55154723089699,
59.08782540944));
#124461=CARTESIAN_POINT('',(19.0913785491043,-8.64603879443074,58.2486575231502));
#124462=CARTESIAN_POINT('Ctrl Pts',(19.0913788008791,-8.64603683958299,
58.24865662762));
#124463=CARTESIAN_POINT('Ctrl Pts',(19.0831160153987,-8.61192581016859,
58.3206480322238));
#124464=CARTESIAN_POINT('Ctrl Pts',(19.0729896736748,-8.57628931983382,
58.4100917669793));
#124465=CARTESIAN_POINT('Ctrl Pts',(19.04805521017,-8.52029418216068,58.6267491454393));
#124466=CARTESIAN_POINT('Ctrl Pts',(19.0331814385135,-8.4999991684141,58.7541918345667));
#124467=CARTESIAN_POINT('Ctrl Pts',(19.0165457198591,-8.5,58.89829642895));
#124468=CARTESIAN_POINT('',(19.9598076682562,-9.54867899952217,58.4893752699909));
#124469=CARTESIAN_POINT('Origin',(18.9749976915275,-9.54867463823461,58.6630340457145));
#124470=CARTESIAN_POINT('Origin',(19.9995178579382,-9.97190853039367,58.7145825449128));
#124471=CARTESIAN_POINT('Origin',(24.2283495281091,-1.25,82.697478608263));
#124472=CARTESIAN_POINT('',(21.1895064189391,-1.25,65.4633429305539));
#124473=CARTESIAN_POINT('',(19.9598077382391,-9.54867899952299,58.48937525765));
#124474=CARTESIAN_POINT('Ctrl Pts',(19.1714182688491,-10.74749523148,58.64157228471));
#124475=CARTESIAN_POINT('Ctrl Pts',(19.2001402692091,-10.7360962773,58.6139545222));
#124476=CARTESIAN_POINT('Ctrl Pts',(19.2671048399391,-10.70358813109,58.5547842577801));
#124477=CARTESIAN_POINT('Ctrl Pts',(19.3727076110191,-10.63072812626,58.47790542142));
#124478=CARTESIAN_POINT('Ctrl Pts',(19.4816021301791,-10.53268886688,58.41849876533));
#124479=CARTESIAN_POINT('Ctrl Pts',(19.5798624371291,-10.42553809768,58.38451859051));
#124480=CARTESIAN_POINT('Ctrl Pts',(19.6666859921691,-10.31512361264,58.37413803989));
#124481=CARTESIAN_POINT('Ctrl Pts',(19.7421160173891,-10.20561091184,58.3851490096));
#124482=CARTESIAN_POINT('Ctrl Pts',(19.8072433379691,-10.09866844348,58.41581498618));
#124483=CARTESIAN_POINT('Ctrl Pts',(19.8629533250291,-9.99480870780799,
58.46596105467));
#124484=CARTESIAN_POINT('Ctrl Pts',(19.9090928496691,-9.894926057294,58.53693056153));
#124485=CARTESIAN_POINT('Ctrl Pts',(19.9440264651791,-9.80174293293698,
58.63026741436));
#124486=CARTESIAN_POINT('Ctrl Pts',(19.9586138434991,-9.74464988774498,
58.71150611838));
#124487=CARTESIAN_POINT('Ctrl Pts',(19.9627402380791,-9.71822700826899,
58.75847349534));
#124488=CARTESIAN_POINT('Ctrl Pts',(19.9631169183391,-9.71562037545599,
58.76321536219));
#124489=CARTESIAN_POINT('Ctrl Pts',(19.4389951139891,-10.92142136616,57.90619534373));
#124490=CARTESIAN_POINT('Ctrl Pts',(19.4698150313491,-10.87387824357,57.8709868808));
#124491=CARTESIAN_POINT('Ctrl Pts',(19.5403451857891,-10.75993068367,57.8001893243101));
#124492=CARTESIAN_POINT('Ctrl Pts',(19.6471278826591,-10.56375960732,57.72415385788));
#124493=CARTESIAN_POINT('Ctrl Pts',(19.7525232043691,-10.34198300414,57.68551084602));
#124494=CARTESIAN_POINT('Ctrl Pts',(19.8436599230991,-10.12537489763,57.68693560855));
#124495=CARTESIAN_POINT('Ctrl Pts',(19.9206973644291,-9.91948599561099,
57.7224735366501));
#124496=CARTESIAN_POINT('Ctrl Pts',(19.9844091841491,-9.72750230791499,
57.78683436066));
#124497=CARTESIAN_POINT('Ctrl Pts',(20.0362321565991,-9.54902868193599,
57.87682821331));
#124498=CARTESIAN_POINT('Ctrl Pts',(20.0770494080691,-9.38266419984499,
57.9922002653601));
#124499=CARTESIAN_POINT('Ctrl Pts',(20.1064831635191,-9.22819950554099,
58.1349559086));
#124500=CARTESIAN_POINT('Ctrl Pts',(20.1226504432591,-9.08837963333299,
58.30711118863));
#124501=CARTESIAN_POINT('Ctrl Pts',(20.1225325579991,-9.00485278376398,
58.44835364564));
#124502=CARTESIAN_POINT('Ctrl Pts',(20.1184343085791,-8.96657204339798,
58.52818750154));
#124503=CARTESIAN_POINT('Ctrl Pts',(20.1179829255791,-8.96279955198799,
58.53623155663));
#124504=CARTESIAN_POINT('Ctrl Pts',(19.1652394686491,-10.56072968227,57.2444908451201));
#124505=CARTESIAN_POINT('Ctrl Pts',(19.1934686882291,-10.48562637282,57.22576151961));
#124506=CARTESIAN_POINT('Ctrl Pts',(19.2551219195491,-10.31444099589,57.1952629814201));
#124507=CARTESIAN_POINT('Ctrl Pts',(19.3403057354091,-10.04843890404,57.18919599896));
#124508=CARTESIAN_POINT('Ctrl Pts',(19.4162870129891,-9.77434356831699,
57.22757500333));
#124509=CARTESIAN_POINT('Ctrl Pts',(19.4752171934691,-9.526002199897,57.3005463023901));
#124510=CARTESIAN_POINT('Ctrl Pts',(19.5191579447891,-9.30450735442199,
57.39946609893));
#124511=CARTESIAN_POINT('Ctrl Pts',(19.5501871442691,-9.10911142993699,
57.5177279503601));
#124512=CARTESIAN_POINT('Ctrl Pts',(19.5703028373991,-8.93619395275799,
57.6522092200201));
#124513=CARTESIAN_POINT('Ctrl Pts',(19.5806370647691,-8.78210021717399,
57.80293835391));
#124514=CARTESIAN_POINT('Ctrl Pts',(19.5812333396291,-8.64489440002398,
57.9717607872401));
#124515=CARTESIAN_POINT('Ctrl Pts',(19.5712315886491,-8.52540487218098,
58.16008290365));
#124516=CARTESIAN_POINT('Ctrl Pts',(19.5558276663491,-8.45644720816198,
58.30540130949));
#124517=CARTESIAN_POINT('Ctrl Pts',(19.5449631456091,-8.425280107705,58.38543455065));
#124518=CARTESIAN_POINT('Ctrl Pts',(19.5438477623991,-8.42221325699699,
58.39347965143));
#124519=CARTESIAN_POINT('Ctrl Pts',(18.5989027611591,-9.99316710698298,
57.25772470602));
#124520=CARTESIAN_POINT('Ctrl Pts',(18.6222067375291,-9.92413049439999,
57.26457038522));
#124521=CARTESIAN_POINT('Ctrl Pts',(18.6706066640791,-9.77191874230598,
57.28967897792));
#124522=CARTESIAN_POINT('Ctrl Pts',(18.7310388805491,-9.55301850062899,
57.35912787143));
#124523=CARTESIAN_POINT('Ctrl Pts',(18.7784186996691,-9.34556310230998,
57.46080026331));
#124524=CARTESIAN_POINT('Ctrl Pts',(18.8093242582891,-9.17204736543399,
57.57644805921));
#124525=CARTESIAN_POINT('Ctrl Pts',(18.8269314570391,-9.02899558215699,
57.69862040094));
#124526=CARTESIAN_POINT('Ctrl Pts',(18.8340110856991,-8.91234674184498,
57.82235662252));
#124527=CARTESIAN_POINT('Ctrl Pts',(18.8328277769991,-8.817024057061,57.94606081245));
#124528=CARTESIAN_POINT('Ctrl Pts',(18.8247874658691,-8.73882659643499,
58.07015047993));
#124529=CARTESIAN_POINT('Ctrl Pts',(18.8106180795391,-8.67503808675099,
58.19563444819));
#124530=CARTESIAN_POINT('Ctrl Pts',(18.7908234139491,-8.62437257846199,
58.32278161578));
#124531=CARTESIAN_POINT('Ctrl Pts',(18.7734425263991,-8.59774862058898,
58.41254450536));
#124532=CARTESIAN_POINT('Ctrl Pts',(18.7634183625491,-8.58620276459499,
58.4599288642401));
#124533=CARTESIAN_POINT('Ctrl Pts',(18.7624063941091,-8.58507186480098,
58.46467291799));
#124534=CARTESIAN_POINT('',(18.8782773267445,-10.0000000019723,57.3029715768249));
#124535=CARTESIAN_POINT('Ctrl Pts',(18.8783268875783,-10.,57.302985115163));
#124536=CARTESIAN_POINT('Ctrl Pts',(18.8938428301929,-9.95326836354297,
57.3072289031713));
#124537=CARTESIAN_POINT('Ctrl Pts',(18.9083223436148,-9.90758142138574,
57.3134594588141));
#124538=CARTESIAN_POINT('Ctrl Pts',(18.9218376118847,-9.8631161205231,57.3213913093735));
#124539=CARTESIAN_POINT('Ctrl Pts',(18.9357793183205,-9.81724783594088,
57.3295734282767));
#124540=CARTESIAN_POINT('Ctrl Pts',(18.9486951127055,-9.77267940607304,
57.3395653884218));
#124541=CARTESIAN_POINT('Ctrl Pts',(18.9606650515343,-9.72954964117205,
57.3510561920399));
#124542=CARTESIAN_POINT('Ctrl Pts',(18.973479323177,-9.6833775987557,57.3633575313416));
#124543=CARTESIAN_POINT('Ctrl Pts',(18.9852097700432,-9.63885449218422,
57.3773759762135));
#124544=CARTESIAN_POINT('Ctrl Pts',(18.9959530202418,-9.59608710933202,
57.3927418875215));
#124545=CARTESIAN_POINT('Ctrl Pts',(19.0066962704403,-9.55331972647982,
57.4081077988295));
#124546=CARTESIAN_POINT('Ctrl Pts',(19.0164524568694,-9.51230744604947,
57.4248207583032));
#124547=CARTESIAN_POINT('Ctrl Pts',(19.0253143161839,-9.47310040316696,
57.4425306909256));
#124548=CARTESIAN_POINT('Ctrl Pts',(19.0342882072661,-9.43339770421921,
57.4604645128002));
#124549=CARTESIAN_POINT('Ctrl Pts',(19.042345123411,-9.39554564575364,57.4794203451349));
#124550=CARTESIAN_POINT('Ctrl Pts',(19.0495778675271,-9.35954753176827,
57.4990608309867));
#124551=CARTESIAN_POINT('Ctrl Pts',(19.0570664813153,-9.32227592801514,
57.5193961298439));
#124552=CARTESIAN_POINT('Ctrl Pts',(19.0636717003723,-9.28699131720336,
57.5404649911381));
#124553=CARTESIAN_POINT('Ctrl Pts',(19.0694884995562,-9.25365191702527,
57.5619262349102));
#124554=CARTESIAN_POINT('Ctrl Pts',(19.0740301794008,-9.22762095445684,
57.5786828901084));
#124555=CARTESIAN_POINT('Ctrl Pts',(19.0780910568302,-9.20277482937547,
57.5956794254871));
#124556=CARTESIAN_POINT('Ctrl Pts',(19.0817125082702,-9.17907826869883,
57.6127686736064));
#124557=CARTESIAN_POINT('Ctrl Pts',(19.0837152207405,-9.16597374462739,
57.6222192629302));
#124558=CARTESIAN_POINT('Ctrl Pts',(19.0855505911153,-9.15346508141529,
57.6315179556795));
#124559=CARTESIAN_POINT('Ctrl Pts',(19.0872733852832,-9.14119469554508,
57.6408911412512));
#124560=CARTESIAN_POINT('Ctrl Pts',(19.0890134403464,-9.12880137110741,
57.6503582379696));
#124561=CARTESIAN_POINT('Ctrl Pts',(19.0906385994655,-9.11665094506254,
57.6599015274696));
#124562=CARTESIAN_POINT('Ctrl Pts',(19.0921933332106,-9.10440424433379,
57.6697959537671));
#124563=CARTESIAN_POINT('Ctrl Pts',(19.0923631759237,-9.10306638639855,
57.6708768437986));
#124564=CARTESIAN_POINT('Ctrl Pts',(19.0925321668134,-9.10172741006866,
57.671961963764));
#124565=CARTESIAN_POINT('Ctrl Pts',(19.0927003554822,-9.10038689612429,
57.6730517011598));
#124566=CARTESIAN_POINT('Ctrl Pts',(19.0980544282457,-9.05771333644073,
57.7077421077707));
#124567=CARTESIAN_POINT('Ctrl Pts',(19.1021295422428,-9.01730565368886,
57.7440102458586));
#124568=CARTESIAN_POINT('Ctrl Pts',(19.1050219213473,-8.97924705484321,
57.7815126843629));
#124569=CARTESIAN_POINT('Ctrl Pts',(19.1079843594873,-8.94026660286906,
57.8199235047129));
#124570=CARTESIAN_POINT('Ctrl Pts',(19.1097062135066,-8.90375023790228,
57.8596286926656));
#124571=CARTESIAN_POINT('Ctrl Pts',(19.110288386314,-8.86973433764281,57.9002739713109));
#124572=CARTESIAN_POINT('Ctrl Pts',(19.1108784273267,-8.83525870431884,
57.9414685806624));
#124573=CARTESIAN_POINT('Ctrl Pts',(19.1102978994856,-8.8033512522251,57.9836284817762));
#124574=CARTESIAN_POINT('Ctrl Pts',(19.1086472825267,-8.77400002787252,
58.0264061375439));
#124575=CARTESIAN_POINT('Ctrl Pts',(19.1069602796114,-8.74400178946377,
58.0701267776396));
#124576=CARTESIAN_POINT('Ctrl Pts',(19.104155613855,-8.71667339410396,58.114492336582));
#124577=CARTESIAN_POINT('Ctrl Pts',(19.1003338768725,-8.69195530435059,
58.1591597238884));
#124578=CARTESIAN_POINT('Ctrl Pts',(19.0977902289464,-8.67550359194224,
58.1888891656587));
#124579=CARTESIAN_POINT('Ctrl Pts',(19.0947958862835,-8.66020725328719,
58.2187529102463));
#124580=CARTESIAN_POINT('Ctrl Pts',(19.0913785491043,-8.64603879443074,
58.2486575231502));
#124581=CARTESIAN_POINT('Ctrl Pts',(19.9598074414544,-9.54867899952064,
58.4893753099853));
#124582=CARTESIAN_POINT('Ctrl Pts',(19.9542411823548,-9.55326652103831,
58.4578102133941));
#124583=CARTESIAN_POINT('Ctrl Pts',(19.9476045455276,-9.55822494497135,
58.4260920838297));
#124584=CARTESIAN_POINT('Ctrl Pts',(19.9398484081562,-9.56355305469618,
58.3942993779954));
#124585=CARTESIAN_POINT('Ctrl Pts',(19.9372948498576,-9.56530723182746,
58.383832244172));
#124586=CARTESIAN_POINT('Ctrl Pts',(19.9346200002808,-9.56710131672924,
58.3733574086514));
#124587=CARTESIAN_POINT('Ctrl Pts',(19.931822301245,-9.56893477895819,58.3628787978499));
#124588=CARTESIAN_POINT('Ctrl Pts',(19.9230863039181,-9.57465988409868,
58.3301586536235));
#124589=CARTESIAN_POINT('Ctrl Pts',(19.9131513284052,-9.58077050467405,
58.2973984067014));
#124590=CARTESIAN_POINT('Ctrl Pts',(19.9019681612585,-9.58727342913176,
58.2646820321185));
#124591=CARTESIAN_POINT('Ctrl Pts',(19.8956843679744,-9.59092740590757,
58.2462987841365));
#124592=CARTESIAN_POINT('Ctrl Pts',(19.8890067452488,-9.59470485515314,
58.2279302044197));
#124593=CARTESIAN_POINT('Ctrl Pts',(19.8819290491294,-9.59860407484053,
58.2095973349305));
#124594=CARTESIAN_POINT('Ctrl Pts',(19.874816160293,-9.60252268277692,58.1911733081669));
#124595=CARTESIAN_POINT('Ctrl Pts',(19.8672991829115,-9.60656426155635,
58.1727853912745));
#124596=CARTESIAN_POINT('Ctrl Pts',(19.8593707036486,-9.61073258786585,
58.1544516284897));
#124597=CARTESIAN_POINT('Ctrl Pts',(19.8458919321712,-9.61781893013978,
58.1232834068547));
#124598=CARTESIAN_POINT('Ctrl Pts',(19.8312239210235,-9.62526905939209,
58.0922727289796));
#124599=CARTESIAN_POINT('Ctrl Pts',(19.8153419026997,-9.63307328270873,
58.061521164123));
#124600=CARTESIAN_POINT('Ctrl Pts',(19.8029377456224,-9.63916852891185,
58.0375036096107));
#124601=CARTESIAN_POINT('Ctrl Pts',(19.7897933314337,-9.64547947752553,
58.0136448082272));
#124602=CARTESIAN_POINT('Ctrl Pts',(19.7758983977501,-9.65201328479347,
57.9899949949436));
#124603=CARTESIAN_POINT('Ctrl Pts',(19.7616084921664,-9.65873281948774,
57.9656729214027));
#124604=CARTESIAN_POINT('Ctrl Pts',(19.7465252268148,-9.66568418437979,
57.9415725405707));
#124605=CARTESIAN_POINT('Ctrl Pts',(19.7306431945115,-9.67286709491166,
57.9177510229782));
#124606=CARTESIAN_POINT('Ctrl Pts',(19.7289172210685,-9.67364769481126,
57.9151622291796));
#124607=CARTESIAN_POINT('Ctrl Pts',(19.7271818233574,-9.67443102682133,
57.9125767380664));
#124608=CARTESIAN_POINT('Ctrl Pts',(19.7254369924547,-9.67521710892549,
57.909994624528));
#124609=CARTESIAN_POINT('Ctrl Pts',(19.7172273866166,-9.67891570471584,
57.8978455192213));
#124610=CARTESIAN_POINT('Ctrl Pts',(19.7086434471657,-9.68274570879777,
57.8855333625138));
#124611=CARTESIAN_POINT('Ctrl Pts',(19.6999083684738,-9.68661195124135,
57.8734007870112));
#124612=CARTESIAN_POINT('Ctrl Pts',(19.6910441422571,-9.69053535580778,
57.8610888322324));
#124613=CARTESIAN_POINT('Ctrl Pts',(19.6820244432216,-9.69449595062049,
57.8489619683201));
#124614=CARTESIAN_POINT('Ctrl Pts',(19.6731171416485,-9.69837585202093,
57.8373408913688));
#124615=CARTESIAN_POINT('Ctrl Pts',(19.6717701967348,-9.69896256320545,
57.835583574592));
#124616=CARTESIAN_POINT('Ctrl Pts',(19.6704258816302,-9.69954739803375,
57.8338377535858));
#124617=CARTESIAN_POINT('Ctrl Pts',(19.669085184134,-9.70012991688436,57.832104463319));
#124618=CARTESIAN_POINT('Ctrl Pts',(19.6545934277506,-9.70642643141944,
57.813369125661));
#124619=CARTESIAN_POINT('Ctrl Pts',(19.6392416893483,-9.71304394409325,
57.7944386211372));
#124620=CARTESIAN_POINT('Ctrl Pts',(19.6229683979434,-9.71997398145692,
57.7753944714038));
#124621=CARTESIAN_POINT('Ctrl Pts',(19.6011612990038,-9.72926060987679,
57.7498742710262));
#124622=CARTESIAN_POINT('Ctrl Pts',(19.5776981983314,-9.73910833703785,
57.7241483916085));
#124623=CARTESIAN_POINT('Ctrl Pts',(19.5524383006595,-9.74951075760174,
57.6984455580634));
#124624=CARTESIAN_POINT('Ctrl Pts',(19.5320199393966,-9.75791935782019,
57.677669157952));
#124625=CARTESIAN_POINT('Ctrl Pts',(19.5104276008589,-9.76669025045359,
57.6569084037166));
#124626=CARTESIAN_POINT('Ctrl Pts',(19.4876002219506,-9.7758198446224,57.6363054400513));
#124627=CARTESIAN_POINT('Ctrl Pts',(19.4614826753149,-9.78626531023744,
57.6127329192411));
#124628=CARTESIAN_POINT('Ctrl Pts',(19.4337470744814,-9.79717991205959,
57.5893665362372));
#124629=CARTESIAN_POINT('Ctrl Pts',(19.4043265244434,-9.80858109390736,
57.5664510660148));
#124630=CARTESIAN_POINT('Ctrl Pts',(19.3908862087655,-9.81378954456305,
57.5559824937652));
#124631=CARTESIAN_POINT('Ctrl Pts',(19.3770947553912,-9.81909963101177,
57.5456084732102));
#124632=CARTESIAN_POINT('Ctrl Pts',(19.3629486740691,-9.82451356155939,
57.5353545818722));
#124633=CARTESIAN_POINT('Ctrl Pts',(19.3490675385454,-9.82982609313166,
57.5252927384494));
#124634=CARTESIAN_POINT('Ctrl Pts',(19.3348478695568,-9.83525106947039,
57.5153486013066));
#124635=CARTESIAN_POINT('Ctrl Pts',(19.3202822274548,-9.84078167951122,
57.5055433568592));
#124636=CARTESIAN_POINT('Ctrl Pts',(19.2897062331762,-9.85239145955266,
57.4849603234422));
#124637=CARTESIAN_POINT('Ctrl Pts',(19.2576029146744,-9.86446624259593,
57.4649867936472));
#124638=CARTESIAN_POINT('Ctrl Pts',(19.2239336798893,-9.87694380377314,
57.4458454060012));
#124639=CARTESIAN_POINT('Ctrl Pts',(19.1927256677699,-9.88850925463423,
57.4281032547034));
#124640=CARTESIAN_POINT('Ctrl Pts',(19.1601720310806,-9.90042058302751,
57.4110763933475));
#124641=CARTESIAN_POINT('Ctrl Pts',(19.1262789226855,-9.91263776729008,
57.3949732486323));
#124642=CARTESIAN_POINT('Ctrl Pts',(19.1236059396619,-9.91360127661915,
57.3937032726847));
#124643=CARTESIAN_POINT('Ctrl Pts',(19.1209246469674,-9.91456669436537,
57.3924390573872));
#124644=CARTESIAN_POINT('Ctrl Pts',(19.1182350589379,-9.91553400419153,
57.3911807128345));
#124645=CARTESIAN_POINT('Ctrl Pts',(19.0841674648025,-9.92778640797961,
57.3752419255427));
#124646=CARTESIAN_POINT('Ctrl Pts',(19.0487653579397,-9.94034008511723,
57.3602447619451));
#124647=CARTESIAN_POINT('Ctrl Pts',(19.0120652193687,-9.95324402795822,
57.3464036888154));
#124648=CARTESIAN_POINT('Ctrl Pts',(18.9756752032899,-9.96603893025964,
57.3326795751376));
#124649=CARTESIAN_POINT('Ctrl Pts',(18.9380089288395,-9.97917838906926,
57.3200930197138));
#124650=CARTESIAN_POINT('Ctrl Pts',(18.8991462603499,-9.99273593367285,
57.3088485005585));
#124651=CARTESIAN_POINT('Ctrl Pts',(18.8922438986108,-9.99514387632795,
57.3068513721623));
#124652=CARTESIAN_POINT('Ctrl Pts',(18.8853039100555,-9.99756506874135,
57.3048965453963));
#124653=CARTESIAN_POINT('Ctrl Pts',(18.8783268876145,-9.99999999999996,
57.3029851150307));
#124654=CARTESIAN_POINT('Origin',(18.4825957014091,-15.00000011529,58.74984511558));
#124655=CARTESIAN_POINT('',(18.8783357567019,-14.999996024641,57.302989036439));
#124656=CARTESIAN_POINT('Origin',(18.4825952511691,-15.00000013862,58.74984256216));
#124657=CARTESIAN_POINT('Origin',(18.4826085813491,-14.99999405365,58.74984854358));
#124658=CARTESIAN_POINT('Origin',(17.7894674803291,1.4210854715202E-14,
100.88908350184));
#124659=CARTESIAN_POINT('',(15.282105101301,-17.8079464603878,57.8022959605294));
#124660=CARTESIAN_POINT('',(18.9921129410137,-17.0122601925885,65.8508014704009));
#124661=CARTESIAN_POINT('Ctrl Pts',(15.282105101301,-17.8079464603878,57.8022959605294));
#124662=CARTESIAN_POINT('Ctrl Pts',(15.3505394572593,-17.7947650778713,
57.9206881482452));
#124663=CARTESIAN_POINT('Ctrl Pts',(15.4184424259051,-17.7815460140866,
58.0393944742722));
#124664=CARTESIAN_POINT('Ctrl Pts',(15.4858175145022,-17.7683020806319,
58.1584148517074));
#124665=CARTESIAN_POINT('Ctrl Pts',(15.684876581833,-17.7291730034586,58.5100594405155));
#124666=CARTESIAN_POINT('Ctrl Pts',(15.8793283335588,-17.6898288245895,
58.8644420115123));
#124667=CARTESIAN_POINT('Ctrl Pts',(16.0692882733122,-17.6505598703399,
59.2214906008568));
#124668=CARTESIAN_POINT('Ctrl Pts',(16.2599229789274,-17.6111514269444,
59.5798074797121));
#124669=CARTESIAN_POINT('Ctrl Pts',(16.4460340568941,-17.5718183397561,
59.9408092387024));
#124670=CARTESIAN_POINT('Ctrl Pts',(16.6277296627721,-17.532830229838,60.3044694396092));
#124671=CARTESIAN_POINT('Ctrl Pts',(16.80927596144,-17.4938741581515,60.6678308050557));
#124672=CARTESIAN_POINT('Ctrl Pts',(16.9864141980048,-17.4552620670934,
61.0338461524315));
#124673=CARTESIAN_POINT('Ctrl Pts',(17.1592414060169,-17.4172454697713,
61.4025367311538));
#124674=CARTESIAN_POINT('Ctrl Pts',(17.3247218718306,-17.3808449266747,
61.7555545771854));
#124675=CARTESIAN_POINT('Ctrl Pts',(17.4862500986103,-17.3449898813006,
62.1110252596489));
#124676=CARTESIAN_POINT('Ctrl Pts',(17.6438998504956,-17.3098916204539,
62.4690096849072));
#124677=CARTESIAN_POINT('Ctrl Pts',(17.8025545590757,-17.2745696216578,
62.8292761235559));
#124678=CARTESIAN_POINT('Ctrl Pts',(17.957281269496,-17.240013832677,63.1920878397201));
#124679=CARTESIAN_POINT('Ctrl Pts',(18.1080982043483,-17.2064151462286,
63.5573650366903));
#124680=CARTESIAN_POINT('Ctrl Pts',(18.2637636032691,-17.1717363289306,
63.9343851680085));
#124681=CARTESIAN_POINT('Ctrl Pts',(18.4152641332005,-17.1380767231858,
64.3140315907342));
#124682=CARTESIAN_POINT('Ctrl Pts',(18.5626024828262,-17.1056465582174,
64.6962722974421));
#124683=CARTESIAN_POINT('Ctrl Pts',(18.7099408324519,-17.0732163932491,
65.0785130041501));
#124684=CARTESIAN_POINT('Ctrl Pts',(18.8531172838998,-17.042015217014,65.4633480320533));
#124685=CARTESIAN_POINT('Ctrl Pts',(18.9921129410137,-17.0122601925885,
65.8508014704009));
#124686=CARTESIAN_POINT('Origin',(11.8338327653321,1.4210854715202E-14,
67.1130006183879));
#124687=CARTESIAN_POINT('Ctrl Pts',(15.2821062552024,-17.8079506230211,
57.8022957570331));
#124688=CARTESIAN_POINT('Ctrl Pts',(15.4823121359235,-17.7542554209139,
57.8391951328845));
#124689=CARTESIAN_POINT('Ctrl Pts',(15.6878488274998,-17.6958698358612,
57.8779860861533));
#124690=CARTESIAN_POINT('Ctrl Pts',(15.8984493855906,-17.632250897153,57.9186971735126));
#124691=CARTESIAN_POINT('Ctrl Pts',(16.1060975495705,-17.5695238277811,
57.9588375350598));
#124692=CARTESIAN_POINT('Ctrl Pts',(16.3186688001434,-17.5017088209382,
58.0008445354996));
#124693=CARTESIAN_POINT('Ctrl Pts',(16.5358605764418,-17.4282679911826,
58.0447537793855));
#124694=CARTESIAN_POINT('Ctrl Pts',(16.7482639330329,-17.3564463089037,
58.0876949576643));
#124695=CARTESIAN_POINT('Ctrl Pts',(16.9650864343223,-17.2792438249526,
58.132455407181));
#124696=CARTESIAN_POINT('Ctrl Pts',(17.1859979209596,-17.1961450662185,
58.1790767468365));
#124697=CARTESIAN_POINT('Ctrl Pts',(17.4041564194499,-17.1140818801533,
58.2251170936362));
#124698=CARTESIAN_POINT('Ctrl Pts',(17.626302786287,-17.0262681635225,58.2729722104596));
#124699=CARTESIAN_POINT('Ctrl Pts',(17.8520704187426,-16.9321996968654,
58.3226907549545));
#124700=CARTESIAN_POINT('Ctrl Pts',(18.0732551795446,-16.8400407320471,
58.3714000595255));
#124701=CARTESIAN_POINT('Ctrl Pts',(18.2979157487183,-16.7418780652835,
58.4218978960706));
#124702=CARTESIAN_POINT('Ctrl Pts',(18.5256588509806,-16.6372345008744,
58.4742385791027));
#124703=CARTESIAN_POINT('Ctrl Pts',(18.7404075568062,-16.5385616110849,
58.5235928463957));
#124704=CARTESIAN_POINT('Ctrl Pts',(18.957896824941,-16.4341260375928,58.5745857071687));
#124705=CARTESIAN_POINT('Ctrl Pts',(19.1777550979457,-16.323528908982,58.6272700752903));
#124706=CARTESIAN_POINT('Origin',(11.833832765324,1.4210854715202E-14,67.1130006183894));
#124707=CARTESIAN_POINT('',(14.883373594419,-20.2647763837508,66.5752842914479));
#124708=CARTESIAN_POINT('Ctrl Pts',(18.9921131492666,-17.012260192524,65.8508026512244));
#124709=CARTESIAN_POINT('Ctrl Pts',(18.1865537652697,-17.3617579185958,
65.9928445051859));
#124710=CARTESIAN_POINT('Ctrl Pts',(17.4282361956689,-17.8163218667055,
66.1265563526508));
#124711=CARTESIAN_POINT('Ctrl Pts',(16.0411085625388,-18.9125487124957,
66.3711443800578));
#124712=CARTESIAN_POINT('Ctrl Pts',(15.4171051316011,-19.5523187044817,
66.4811730209878));
#124713=CARTESIAN_POINT('Ctrl Pts',(14.883373594419,-20.2647763837508,66.575284291448));
#124714=CARTESIAN_POINT('',(-6.53751764820717,-8.5,70.352365368344));
#124715=CARTESIAN_POINT('Origin',(11.833832765324,1.4210854715202E-14,67.1130006183894));
#124716=CARTESIAN_POINT('',(-12.1462360205204,-8.5,71.3413337445779));
#124717=CARTESIAN_POINT('Origin',(11.833832765324,1.4210854715202E-14,67.1130006183894));
#124718=CARTESIAN_POINT('',(15.6158353372468,-20.1981065744412,68.3761083647154));
#124719=CARTESIAN_POINT('Ctrl Pts',(15.6157934551793,-20.1981142180028,
68.3761244855819));
#124720=CARTESIAN_POINT('Ctrl Pts',(15.5010475555325,-20.2085914269983,
68.07304656518));
#124721=CARTESIAN_POINT('Ctrl Pts',(15.3826186459966,-20.2194631831356,
67.7713940591794));
#124722=CARTESIAN_POINT('Ctrl Pts',(15.1384505677303,-20.2417654565994,
67.1710527205433));
#124723=CARTESIAN_POINT('Ctrl Pts',(15.0127177613177,-20.2531953410346,
66.8723797468496));
#124724=CARTESIAN_POINT('Ctrl Pts',(14.8833735944191,-20.2647763837508,
66.5752842914479));
#124725=CARTESIAN_POINT('',(15.9984098127276,-20.3875455450126,78.3830072931938));
#124726=CARTESIAN_POINT('Ctrl Pts',(15.9983959512983,-20.3875469025234,
78.3830030094886));
#124727=CARTESIAN_POINT('Ctrl Pts',(16.4328372437242,-20.3164621615951,
76.9546891450724));
#124728=CARTESIAN_POINT('Ctrl Pts',(16.7037780449221,-20.2204258112703,
75.2444468274443));
#124729=CARTESIAN_POINT('Ctrl Pts',(16.5602362046653,-20.1331659697557,
71.6438394681868));
#124730=CARTESIAN_POINT('Ctrl Pts',(16.217560034564,-20.1431511202205,69.965049899536));
#124731=CARTESIAN_POINT('Ctrl Pts',(15.615877218811,-20.198098930694,68.3760922412998));
#124732=CARTESIAN_POINT('Ctrl Pts',(15.1826286361355,-20.4790209859242,
80.7654349522145));
#124733=CARTESIAN_POINT('Ctrl Pts',(15.3308715299447,-20.4693621419826,
80.3776179869579));
#124734=CARTESIAN_POINT('Ctrl Pts',(15.4722327090839,-20.4566516001834,
79.9871295969088));
#124735=CARTESIAN_POINT('Ctrl Pts',(15.7443617489847,-20.4259089142243,
79.1929667922874));
#124736=CARTESIAN_POINT('Ctrl Pts',(15.874915709885,-20.4077502433841,78.7889060427433));
#124737=CARTESIAN_POINT('Ctrl Pts',(15.9984236741293,-20.387544187533,78.3830115786004));
#124738=CARTESIAN_POINT('Origin',(14.4385554303262,1.4210854715202E-14,
81.8851169135651));
#124739=CARTESIAN_POINT('',(-6.53751764820717,-8.5,70.352365368344));
#124740=CARTESIAN_POINT('Ctrl Pts',(20.1035333418991,-16.60682578431,65.661400313719));
#124741=CARTESIAN_POINT('Ctrl Pts',(20.4910764161291,-16.50426328115,66.404263622412));
#124742=CARTESIAN_POINT('Ctrl Pts',(21.2622024424291,-16.31712154271,68.2147622085249));
#124743=CARTESIAN_POINT('Ctrl Pts',(21.9472426402291,-16.25946392932,71.32939250689));
#124744=CARTESIAN_POINT('Ctrl Pts',(21.9575487565991,-16.51641000933,74.855943101759));
#124745=CARTESIAN_POINT('Ctrl Pts',(21.2210210639291,-17.03764923711,78.150815900789));
#124746=CARTESIAN_POINT('Ctrl Pts',(20.3317361244091,-17.46566964773,80.057299005597));
#124747=CARTESIAN_POINT('Ctrl Pts',(19.8425295031191,-17.6668669887,80.890276924625));
#124748=CARTESIAN_POINT('Ctrl Pts',(16.1484715971691,-17.81257432064,67.611225517012));
#124749=CARTESIAN_POINT('Ctrl Pts',(16.4410317598291,-17.71210035932,68.160095145162));
#124750=CARTESIAN_POINT('Ctrl Pts',(17.0247629322891,-17.52936000758,69.505370284895));
#124751=CARTESIAN_POINT('Ctrl Pts',(17.5404653675491,-17.47323219871,71.836115329147));
#124752=CARTESIAN_POINT('Ctrl Pts',(17.5346243142291,-17.72370055013,74.470228345905));
#124753=CARTESIAN_POINT('Ctrl Pts',(16.9597507724791,-18.2350065912,76.900867930413));
#124754=CARTESIAN_POINT('Ctrl Pts',(16.2859520423791,-18.65955113028,78.274474857878));
#124755=CARTESIAN_POINT('Ctrl Pts',(15.9214324846391,-18.86042280821,78.865755836276));
#124756=CARTESIAN_POINT('Ctrl Pts',(13.8455860593191,-21.47087538256,69.098352900055));
#124757=CARTESIAN_POINT('Ctrl Pts',(14.0473884300291,-21.37673816115,69.4909848960241));
#124758=CARTESIAN_POINT('Ctrl Pts',(14.4481518263091,-21.20735183567,70.444214760764));
#124759=CARTESIAN_POINT('Ctrl Pts',(14.8055693836991,-21.15586552985,72.0760640565359));
#124760=CARTESIAN_POINT('Ctrl Pts',(14.8175681434991,-21.38668013034,73.9261073698239));
#124761=CARTESIAN_POINT('Ctrl Pts',(14.4432251927491,-21.86784838863,75.6694251557751));
#124762=CARTESIAN_POINT('Ctrl Pts',(13.9813565266591,-22.2818469605,76.694122020234));
#124763=CARTESIAN_POINT('Ctrl Pts',(13.7242846805491,-22.48173056057,77.146151574849));
#124764=CARTESIAN_POINT('Ctrl Pts',(14.1821041658691,-26.01344642904,69.485263605966));
#124765=CARTESIAN_POINT('Ctrl Pts',(14.3362809575091,-25.92717763912,69.826391761791));
#124766=CARTESIAN_POINT('Ctrl Pts',(14.6369403842691,-25.77437322202,70.628820996858));
#124767=CARTESIAN_POINT('Ctrl Pts',(14.9149813289091,-25.72865034491,71.94637471107));
#124768=CARTESIAN_POINT('Ctrl Pts',(14.9711591085391,-25.93506056796,73.456840206672));
#124769=CARTESIAN_POINT('Ctrl Pts',(14.7502574305891,-26.37880625846,74.9843966174541));
#124770=CARTESIAN_POINT('Ctrl Pts',(14.4059100677191,-26.77970973387,75.993724308785));
#124771=CARTESIAN_POINT('Ctrl Pts',(14.1929846615191,-26.97836642181,76.46864385711));
#124772=CARTESIAN_POINT('Origin',(22.9322443087252,-26.6270894131141,80.1832188051537));
#124773=CARTESIAN_POINT('Origin',(22.9323739056077,-25.6803623351439,65.7952890379436));
#124774=CARTESIAN_POINT('Ctrl Pts',(20.3703076195591,-17.48636025246,80.6160118299));
#124775=CARTESIAN_POINT('Ctrl Pts',(20.1881103583291,-17.59469264276,81.383197007755));
#124776=CARTESIAN_POINT('Ctrl Pts',(19.7633142133291,-17.81559800981,82.9726719728399));
#124777=CARTESIAN_POINT('Ctrl Pts',(19.0018167096191,-18.10372872761,85.2475673257499));
#124778=CARTESIAN_POINT('Ctrl Pts',(18.1317679720991,-18.32477803286,87.36843783982));
#124779=CARTESIAN_POINT('Ctrl Pts',(17.2370610827991,-18.45951303147,89.2032198305499));
#124780=CARTESIAN_POINT('Ctrl Pts',(16.3494952333791,-18.51446227549,90.7700178089799));
#124781=CARTESIAN_POINT('Ctrl Pts',(15.4867758268391,-18.50123398135,92.10529605495));
#124782=CARTESIAN_POINT('Ctrl Pts',(14.6453959780491,-18.43037008788,93.26267617499));
#124783=CARTESIAN_POINT('Ctrl Pts',(13.8009845953991,-18.30490819777,94.3025568640399));
#124784=CARTESIAN_POINT('Ctrl Pts',(12.9307100320291,-18.12021817286,95.2628709280001));
#124785=CARTESIAN_POINT('Ctrl Pts',(12.0275979803391,-17.86955305763,96.15310194351));
#124786=CARTESIAN_POINT('Ctrl Pts',(11.1010176724691,-17.54986176095,96.96608256951));
#124787=CARTESIAN_POINT('Ctrl Pts',(10.1635981391591,-17.16111541643,97.6955323958101));
#124788=CARTESIAN_POINT('Ctrl Pts',(9.27968364505908,-16.73052720888,98.30286534269));
#124789=CARTESIAN_POINT('Ctrl Pts',(8.71271538374908,-16.41504543997,98.64913661867));
#124790=CARTESIAN_POINT('Ctrl Pts',(8.45819912877909,-16.26514131694,98.79644286584));
#124791=CARTESIAN_POINT('Ctrl Pts',(14.7248846521991,-18.94108804276,77.911688731006));
#124792=CARTESIAN_POINT('Ctrl Pts',(14.5694350031491,-18.93552267139,78.561742613804));
#124793=CARTESIAN_POINT('Ctrl Pts',(14.2134049487491,-18.91245218656,79.908309787637));
#124794=CARTESIAN_POINT('Ctrl Pts',(13.6004443439491,-18.832257487,81.827642780919));
#124795=CARTESIAN_POINT('Ctrl Pts',(12.9289464995691,-18.69869734538,83.60280410874));
#124796=CARTESIAN_POINT('Ctrl Pts',(12.2646619608891,-18.52485132822,85.12309497776));
#124797=CARTESIAN_POINT('Ctrl Pts',(11.6278705382591,-18.32183553005,86.4073429830001));
#124798=CARTESIAN_POINT('Ctrl Pts',(11.0263774792591,-18.09933417041,87.4904580833699));
#124799=CARTESIAN_POINT('Ctrl Pts',(10.4529512601791,-17.86094059021,88.4205103504401));
#124800=CARTESIAN_POINT('Ctrl Pts',(9.88731078157909,-17.60178133109,89.249386304));
#124801=CARTESIAN_POINT('Ctrl Pts',(9.31126387016909,-17.31409529898,90.0096973799401));
#124802=CARTESIAN_POINT('Ctrl Pts',(8.71693645522909,-16.9926399648,90.7110627126001));
#124803=CARTESIAN_POINT('Ctrl Pts',(8.10624510203909,-16.63664836235,91.35001588189));
#124804=CARTESIAN_POINT('Ctrl Pts',(7.48260991328909,-16.24618559887,91.92364883475));
#124805=CARTESIAN_POINT('Ctrl Pts',(6.88447228887909,-15.84456366131,92.40307208249));
#124806=CARTESIAN_POINT('Ctrl Pts',(6.49233429628909,-15.56370842049,92.67816808986));
#124807=CARTESIAN_POINT('Ctrl Pts',(6.31420645011909,-15.43222415467,92.79562051845));
#124808=CARTESIAN_POINT('Ctrl Pts',(12.5063401363191,-24.60762905604,75.845594438731));
#124809=CARTESIAN_POINT('Ctrl Pts',(12.2868497584891,-24.55389093248,76.4322774261809));
#124810=CARTESIAN_POINT('Ctrl Pts',(11.7948949593591,-24.42464703364,77.649532278307));
#124811=CARTESIAN_POINT('Ctrl Pts',(10.9814946228591,-24.17202064863,79.385448634424));
#124812=CARTESIAN_POINT('Ctrl Pts',(10.1222707621991,-23.85736527914,80.987352988331));
#124813=CARTESIAN_POINT('Ctrl Pts',(9.29846527963909,-23.5105055521,82.353880287081));
#124814=CARTESIAN_POINT('Ctrl Pts',(8.52998276490909,-23.14741348718,83.50305548649));
#124815=CARTESIAN_POINT('Ctrl Pts',(7.82085548590909,-22.77957706661,84.4682620618799));
#124816=CARTESIAN_POINT('Ctrl Pts',(7.15797738393909,-22.40870352106,85.2944825448601));
#124817=CARTESIAN_POINT('Ctrl Pts',(6.5147643722091,-22.02537234206,86.0295402695));
#124818=CARTESIAN_POINT('Ctrl Pts',(5.86851416204909,-21.61846160989,86.7038509520601));
#124819=CARTESIAN_POINT('Ctrl Pts',(5.20849832309909,-21.1819420503,87.32752168855));
#124820=CARTESIAN_POINT('Ctrl Pts',(4.53433886995909,-20.71577757791,87.89907590832));
#124821=CARTESIAN_POINT('Ctrl Pts',(3.84677854591909,-20.22008924508,88.41723900531));
#124822=CARTESIAN_POINT('Ctrl Pts',(3.18516755758909,-19.72283039656,88.85636793195));
#124823=CARTESIAN_POINT('Ctrl Pts',(2.74853368799909,-19.38098595465,89.11251172142));
#124824=CARTESIAN_POINT('Ctrl Pts',(2.54938093874909,-19.22185467038,89.22278927536));
#124825=CARTESIAN_POINT('Ctrl Pts',(15.3202955475791,-30.38495224307,75.913018023323));
#124826=CARTESIAN_POINT('Ctrl Pts',(14.9923241307591,-30.38363031797,76.535953769073));
#124827=CARTESIAN_POINT('Ctrl Pts',(14.2581262150091,-30.36285605286,77.831078640661));
#124828=CARTESIAN_POINT('Ctrl Pts',(13.0403732440191,-30.25848525137,79.688467729779));
#124829=CARTESIAN_POINT('Ctrl Pts',(11.7430089211191,-30.06731245317,81.414958143033));
#124830=CARTESIAN_POINT('Ctrl Pts',(10.4851888796891,-29.80822108623,82.899732333371));
#124831=CARTESIAN_POINT('Ctrl Pts',(9.29785820693909,-29.4987931119,84.15906778619));
#124832=CARTESIAN_POINT('Ctrl Pts',(8.19013397563909,-29.15474260213,85.2259540885799));
#124833=CARTESIAN_POINT('Ctrl Pts',(7.14513725765909,-28.78231819477,86.14698476448));
#124834=CARTESIAN_POINT('Ctrl Pts',(6.12414964407909,-28.37420716695,86.97330959057));
#124835=CARTESIAN_POINT('Ctrl Pts',(5.09407323602909,-27.91812922517,87.73786331633));
#124836=CARTESIAN_POINT('Ctrl Pts',(4.04143642525909,-27.40554656753,88.4512402521699));
#124837=CARTESIAN_POINT('Ctrl Pts',(2.97038542110909,-26.83507178681,89.11080249674));
#124838=CARTESIAN_POINT('Ctrl Pts',(1.88745485450909,-26.20680336296,89.71398781054));
#124839=CARTESIAN_POINT('Ctrl Pts',(0.859057681899087,-25.55851947637,90.2295998987501));
#124840=CARTESIAN_POINT('Ctrl Pts',(0.190804675379086,-25.10420966072,90.53273076058));
#124841=CARTESIAN_POINT('Ctrl Pts',(-0.111569990190912,-24.89137338738,
90.6637050372499));
#124842=CARTESIAN_POINT('',(0.214736886699964,-24.69203306784,90.5121335896162));
#124843=CARTESIAN_POINT('Ctrl Pts',(14.2241127701603,-26.6269674540423,
76.3859510179931));
#124844=CARTESIAN_POINT('Ctrl Pts',(14.1795412520668,-26.6539472170917,
76.4881804929476));
#124845=CARTESIAN_POINT('Ctrl Pts',(14.1312457138014,-26.6826870736875,
76.5972642426185));
#124846=CARTESIAN_POINT('Ctrl Pts',(14.0789302636491,-26.7130501592952,
76.7131194761497));
#124847=CARTESIAN_POINT('Ctrl Pts',(14.0273555139025,-26.7429833537376,
76.8273343908414));
#124848=CARTESIAN_POINT('Ctrl Pts',(13.9718738149409,-26.7744943394918,
76.9481305583616));
#124849=CARTESIAN_POINT('Ctrl Pts',(13.9121646105711,-26.8074240326092,
77.0754103633617));
#124850=CARTESIAN_POINT('Ctrl Pts',(13.853945332469,-26.8395320297204,77.1995141500777));
#124851=CARTESIAN_POINT('Ctrl Pts',(13.7917067792004,-26.8729889715799,
77.3297821645709));
#124852=CARTESIAN_POINT('Ctrl Pts',(13.7251177195424,-26.9076180913397,
77.4661043804653));
#124853=CARTESIAN_POINT('Ctrl Pts',(13.6768759464196,-26.9327058482096,
77.564865730221));
#124854=CARTESIAN_POINT('Ctrl Pts',(13.6263500841447,-26.9584082502522,
77.6668042823383));
#124855=CARTESIAN_POINT('Ctrl Pts',(13.5734030099601,-26.9846472826072,
77.7718708996449));
#124856=CARTESIAN_POINT('Ctrl Pts',(13.5418538420831,-27.0002821340026,
77.8344761407981));
#124857=CARTESIAN_POINT('Ctrl Pts',(13.5094448380976,-27.0161073377719,
77.8981918866019));
#124858=CARTESIAN_POINT('Ctrl Pts',(13.4761453842481,-27.0321046935293,
77.9630065865777));
#124859=CARTESIAN_POINT('Ctrl Pts',(13.401736918055,-27.0678511868629,78.1078366619823));
#124860=CARTESIAN_POINT('Ctrl Pts',(13.3228842458205,-27.1044596343681,
78.2581554643632));
#124861=CARTESIAN_POINT('Ctrl Pts',(13.2392274815457,-27.1417034896578,
78.4138206406379));
#124862=CARTESIAN_POINT('Ctrl Pts',(13.157955967163,-27.1778854355779,78.5650474388788));
#124863=CARTESIAN_POINT('Ctrl Pts',(13.0721503004761,-27.2146672208158,
78.7213201750395));
#124864=CARTESIAN_POINT('Ctrl Pts',(12.9814542693971,-27.2518065680707,
78.8824858105204));
#124865=CARTESIAN_POINT('Ctrl Pts',(12.932154265861,-27.2719945512626,78.9700912581302));
#124866=CARTESIAN_POINT('Ctrl Pts',(12.8814088429243,-27.292287566873,79.0591420216869));
#124867=CARTESIAN_POINT('Ctrl Pts',(12.8291575446481,-27.3126419570784,
79.1496104415529));
#124868=CARTESIAN_POINT('Ctrl Pts',(12.7805568352331,-27.3315742675917,
79.2337581953925));
#124869=CARTESIAN_POINT('Ctrl Pts',(12.7306532976543,-27.3505596547148,
79.3191324189104));
#124870=CARTESIAN_POINT('Ctrl Pts',(12.6793964907654,-27.3695601212508,
79.4057090153605));
#124871=CARTESIAN_POINT('Ctrl Pts',(12.653768087321,-27.3790603545189,79.4489973135856));
#124872=CARTESIAN_POINT('Ctrl Pts',(12.6278013340391,-27.38856435764,79.4925861857176));
#124873=CARTESIAN_POINT('Ctrl Pts',(12.6014897686547,-27.3980670555022,
79.5364724335371));
#124874=CARTESIAN_POINT('Ctrl Pts',(12.5883339859625,-27.4028184044332,
79.5584155574468));
#124875=CARTESIAN_POINT('Ctrl Pts',(12.5750919981576,-27.4075694270496,
79.5804330240537));
#124876=CARTESIAN_POINT('Ctrl Pts',(12.5617629862613,-27.4123194787753,
79.6025244237642));
#124877=CARTESIAN_POINT('Ctrl Pts',(12.5550984803131,-27.4146945046381,
79.6135701236194));
#124878=CARTESIAN_POINT('Ctrl Pts',(12.5484122182105,-27.4170692877783,
79.624634306671));
#124879=CARTESIAN_POINT('Ctrl Pts',(12.5417040969433,-27.4194437464173,
79.6357169209848));
#124880=CARTESIAN_POINT('Ctrl Pts',(12.5349959756761,-27.4218182050562,
79.6467995352986));
#124881=CARTESIAN_POINT('Ctrl Pts',(12.5272565546748,-27.4245472203708,
79.6595629761372));
#124882=CARTESIAN_POINT('Ctrl Pts',(12.5215140521559,-27.4265660666789,
79.6690200053765));
#124883=CARTESIAN_POINT('Ctrl Pts',(12.4895955835732,-27.4377873908745,
79.7215848740324));
#124884=CARTESIAN_POINT('Ctrl Pts',(12.457820218365,-27.4487628534799,79.773516535532));
#124885=CARTESIAN_POINT('Ctrl Pts',(12.4262002963281,-27.459497966512,79.8248182666612));
#124886=CARTESIAN_POINT('Ctrl Pts',(12.3102039383348,-27.4988792784873,
80.0130165159416));
#124887=CARTESIAN_POINT('Ctrl Pts',(12.1963034536775,-27.5350256110503,
80.1927364770569));
#124888=CARTESIAN_POINT('Ctrl Pts',(12.0850861408458,-27.568225675283,80.3641442765277));
#124889=CARTESIAN_POINT('Ctrl Pts',(11.9732291346555,-27.6016166977403,
80.5365379695448));
#124890=CARTESIAN_POINT('Ctrl Pts',(11.8640862653525,-27.6320278504697,
80.7005239682551));
#124891=CARTESIAN_POINT('Ctrl Pts',(11.7582030352789,-27.6597560315795,
80.8562805060204));
#124892=CARTESIAN_POINT('Ctrl Pts',(11.6520919177104,-27.687543890749,81.0123722712543));
#124893=CARTESIAN_POINT('Ctrl Pts',(11.549254468362,-27.7126376176627,81.1601994727069));
#124894=CARTESIAN_POINT('Ctrl Pts',(11.4501877554424,-27.7353332633818,
81.2999452956347));
#124895=CARTESIAN_POINT('Ctrl Pts',(11.4098317685165,-27.7445786007401,
81.3568723949279));
#124896=CARTESIAN_POINT('Ctrl Pts',(11.3701009140853,-27.7534259261453,
81.4124584548637));
#124897=CARTESIAN_POINT('Ctrl Pts',(11.3310263390456,-27.7618948858452,
81.466715831748));
#124898=CARTESIAN_POINT('Ctrl Pts',(11.2369289677487,-27.782289396715,81.5973756414347));
#124899=CARTESIAN_POINT('Ctrl Pts',(11.1466408422166,-27.8004908673477,
81.7203306552685));
#124900=CARTESIAN_POINT('Ctrl Pts',(11.0605649669356,-27.8167694213073,
81.8357518458604));
#124901=CARTESIAN_POINT('Ctrl Pts',(10.9902945781751,-27.830058862878,81.9299790832555));
#124902=CARTESIAN_POINT('Ctrl Pts',(10.9228306223314,-27.8420665444725,
82.0191852159257));
#124903=CARTESIAN_POINT('Ctrl Pts',(10.8583685231998,-27.8529305219237,
82.1034591713792));
#124904=CARTESIAN_POINT('Ctrl Pts',(10.8270363034821,-27.8582110283468,
82.1444210718496));
#124905=CARTESIAN_POINT('Ctrl Pts',(10.7964129542786,-27.8632212016962,
82.1842176753842));
#124906=CARTESIAN_POINT('Ctrl Pts',(10.7665191005272,-27.8679760853578,
82.2228587759127));
#124907=CARTESIAN_POINT('Ctrl Pts',(10.7515721736515,-27.8703535271885,
82.2421793261769));
#124908=CARTESIAN_POINT('Ctrl Pts',(10.7368076068207,-27.8726671465973,
82.2612109899799));
#124909=CARTESIAN_POINT('Ctrl Pts',(10.7222278619699,-27.8749187597034,
82.2799549691001));
#124910=CARTESIAN_POINT('Ctrl Pts',(10.7149379895445,-27.8760445662565,
82.2893269586601));
#124911=CARTESIAN_POINT('Ctrl Pts',(10.7076943217371,-27.8771548712339,
82.2986270263737));
#124912=CARTESIAN_POINT('Ctrl Pts',(10.7004971602225,-27.8782498996363,
82.3078553194231));
#124913=CARTESIAN_POINT('Ctrl Pts',(10.6968985794652,-27.8787974138375,
82.3124694659478));
#124914=CARTESIAN_POINT('Ctrl Pts',(10.6933116252264,-27.8793411088949,
82.3170656687637));
#124915=CARTESIAN_POINT('Ctrl Pts',(10.6897363347735,-27.8798810126956,
82.3216439461571));
#124916=CARTESIAN_POINT('Ctrl Pts',(10.6861610443206,-27.8804209164962,
82.3262222235505));
#124917=CARTESIAN_POINT('Ctrl Pts',(10.6837523045838,-27.8807839390271,
82.3293056274602));
#124918=CARTESIAN_POINT('Ctrl Pts',(10.6790454917869,-27.881489378141,82.335325020227));
#124919=CARTESIAN_POINT('Ctrl Pts',(10.5292564252777,-27.9039391909764,
82.5268854800133));
#124920=CARTESIAN_POINT('Ctrl Pts',(10.3793236309,-27.9229735484718,82.7133951355727));
#124921=CARTESIAN_POINT('Ctrl Pts',(10.2295971511516,-27.9387427501686,
82.8949065634546));
#124922=CARTESIAN_POINT('Ctrl Pts',(10.0307485928665,-27.9596854920803,
83.1359680363966));
#124923=CARTESIAN_POINT('Ctrl Pts',(9.83226532157518,-27.9748691529642,
83.3682129997933));
#124924=CARTESIAN_POINT('Ctrl Pts',(9.63493943597387,-27.9847086285095,
83.5918178861406));
#124925=CARTESIAN_POINT('Ctrl Pts',(9.47468391907635,-27.992699623886,83.7734155337742));
#124926=CARTESIAN_POINT('Ctrl Pts',(9.3151911459906,-27.9971661307136,83.9493151099293));
#124927=CARTESIAN_POINT('Ctrl Pts',(9.15686623641873,-27.9983390449081,
84.1196252339744));
#124928=CARTESIAN_POINT('Ctrl Pts',(8.95410134268431,-27.9998411826489,
84.3377394542653));
#124929=CARTESIAN_POINT('Ctrl Pts',(8.753253301804,-27.9959415990584,84.5466860940465));
#124930=CARTESIAN_POINT('Ctrl Pts',(8.55512279127164,-27.9871686188701,
84.7467468079522));
#124931=CARTESIAN_POINT('Ctrl Pts',(8.41451149554765,-27.9809425201823,
84.8887279502314));
#124932=CARTESIAN_POINT('Ctrl Pts',(8.27526800369909,-27.9722620931865,
85.0262340307359));
#124933=CARTESIAN_POINT('Ctrl Pts',(8.13766371803501,-27.9613185539669,
85.1593713327432));
#124934=CARTESIAN_POINT('Ctrl Pts',(7.95933531701222,-27.9471362642138,
85.3319107421728));
#124935=CARTESIAN_POINT('Ctrl Pts',(7.78376096012283,-27.9291534161313,
85.4971131132777));
#124936=CARTESIAN_POINT('Ctrl Pts',(7.61149075125023,-27.907799918818,85.6552372156831));
#124937=CARTESIAN_POINT('Ctrl Pts',(7.54331604267503,-27.899349424296,85.717813703346));
#124938=CARTESIAN_POINT('Ctrl Pts',(7.47565842835141,-27.8903710309361,
85.779281690035));
#124939=CARTESIAN_POINT('Ctrl Pts',(7.40855047216036,-27.8808912939398,
85.8396573807588));
#124940=CARTESIAN_POINT('Ctrl Pts',(7.37499649406485,-27.8761514254417,
85.8698452261206));
#124941=CARTESIAN_POINT('Ctrl Pts',(7.34157992495571,-27.8712862210344,
85.8997599913057));
#124942=CARTESIAN_POINT('Ctrl Pts',(7.30830474045628,-27.8662989906185,
85.9294037186682));
#124943=CARTESIAN_POINT('Ctrl Pts',(7.29166714820657,-27.8638053754106,
85.9442255823494));
#124944=CARTESIAN_POINT('Ctrl Pts',(7.27506490174535,-27.8612812537005,
85.9589796861728));
#124945=CARTESIAN_POINT('Ctrl Pts',(7.25849849392102,-27.8587270387572,
85.9736662847182));
#124946=CARTESIAN_POINT('Ctrl Pts',(7.2430603299745,-27.8563467768762,85.9873526625114));
#124947=CARTESIAN_POINT('Ctrl Pts',(7.22880377733608,-27.8541223276371,
85.999964745298));
#124948=CARTESIAN_POINT('Ctrl Pts',(7.21251286320198,-27.8515454028678,
86.0143422730012));
#124949=CARTESIAN_POINT('Ctrl Pts',(7.21132229907794,-27.8513570773904,
86.015393004012));
#124950=CARTESIAN_POINT('Ctrl Pts',(7.21012085734284,-27.8511668541592,
86.0164531517114));
#124951=CARTESIAN_POINT('Ctrl Pts',(7.20890727669436,-27.8509745272833,
86.0175238184091));
#124952=CARTESIAN_POINT('Ctrl Pts',(7.19212008865412,-27.8483141128838,
86.0323341099262));
#124953=CARTESIAN_POINT('Ctrl Pts',(7.17532881181902,-27.8456172063041,
86.0471115463409));
#124954=CARTESIAN_POINT('Ctrl Pts',(7.158533668051,-27.842883885024,86.0618561108206));
#124955=CARTESIAN_POINT('Ctrl Pts',(6.88863339131123,-27.7989590350725,
86.29880329558));
#124956=CARTESIAN_POINT('Ctrl Pts',(6.61773200244552,-27.7456271040454,
86.5272593346919));
#124957=CARTESIAN_POINT('Ctrl Pts',(6.34672839360205,-27.6832456329547,
86.7472348456383));
#124958=CARTESIAN_POINT('Ctrl Pts',(6.29242554817431,-27.6707458312117,
86.7913128423107));
#124959=CARTESIAN_POINT('Ctrl Pts',(6.2381186830817,-27.657882802054,86.8350504199427));
#124960=CARTESIAN_POINT('Ctrl Pts',(6.18381514071596,-27.6446596060459,
86.8784477931218));
#124961=CARTESIAN_POINT('Ctrl Pts',(5.91249637583059,-27.5785920706245,
87.0952756680128));
#124962=CARTESIAN_POINT('Ctrl Pts',(5.64125923124188,-27.5035299731285,
87.3036091507583));
#124963=CARTESIAN_POINT('Ctrl Pts',(5.37099723920783,-27.4198773606199,
87.5035499473392));
#124964=CARTESIAN_POINT('Ctrl Pts',(5.30487001435339,-27.3994093877638,
87.5524711068169));
#124965=CARTESIAN_POINT('Ctrl Pts',(5.23880123116859,-27.378427332939,87.6008899271453));
#124966=CARTESIAN_POINT('Ctrl Pts',(5.17280406231213,-27.3569375245363,
87.6488081242018));
#124967=CARTESIAN_POINT('Ctrl Pts',(4.99448569078833,-27.2988740090079,
87.7782787517077));
#124968=CARTESIAN_POINT('Ctrl Pts',(4.81669010245746,-27.2371030146491,
87.9040944119933));
#124969=CARTESIAN_POINT('Ctrl Pts',(4.63967111765496,-27.1717492493324,
88.0263075399396));
#124970=CARTESIAN_POINT('Ctrl Pts',(4.49833896028284,-27.1195707293002,
88.1238826393061));
#124971=CARTESIAN_POINT('Ctrl Pts',(4.35750189809531,-27.0651085905577,
88.2191613816254));
#124972=CARTESIAN_POINT('Ctrl Pts',(4.21728870287524,-27.0084307638643,
88.3121724045632));
#124973=CARTESIAN_POINT('Ctrl Pts',(4.18619065250119,-26.9958601216588,
88.3328014293289));
#124974=CARTESIAN_POINT('Ctrl Pts',(4.15512327995206,-26.9831804716333,
88.3533189145229));
#124975=CARTESIAN_POINT('Ctrl Pts',(4.12408798694208,-26.9703925946575,
88.3737251833332));
#124976=CARTESIAN_POINT('Ctrl Pts',(4.08515816083398,-26.9543518301381,
88.3993222510343));
#124977=CARTESIAN_POINT('Ctrl Pts',(4.04627881053809,-26.938140774818,88.4247443251059));
#124978=CARTESIAN_POINT('Ctrl Pts',(4.00745267935975,-26.9217608738289,
88.4499921950428));
#124979=CARTESIAN_POINT('Ctrl Pts',(3.97256330064477,-26.9070418031521,
88.4726800722337));
#124980=CARTESIAN_POINT('Ctrl Pts',(3.93771690956971,-26.8921864059705,
88.4952272722382));
#124981=CARTESIAN_POINT('Ctrl Pts',(3.90291546573732,-26.8771956934937,
88.5176343908025));
#124982=CARTESIAN_POINT('Ctrl Pts',(3.88551474382113,-26.8697003372553,
88.5288379500847));
#124983=CARTESIAN_POINT('Ctrl Pts',(3.86812525873783,-26.8621711521931,
88.5400064890187));
#124984=CARTESIAN_POINT('Ctrl Pts',(3.85074725861327,-26.8546082721214,
88.5511400802268));
#124985=CARTESIAN_POINT('Ctrl Pts',(3.8333692584887,-26.8470453920496,88.5622736714349));
#124986=CARTESIAN_POINT('Ctrl Pts',(3.81691551857993,-26.8398501240272,
88.5727904156976));
#124987=CARTESIAN_POINT('Ctrl Pts',(3.79864795992528,-26.8318186793894,
88.584436084294));
#124988=CARTESIAN_POINT('Ctrl Pts',(3.55361646487997,-26.7240890739074,
88.7406450031161));
#124989=CARTESIAN_POINT('Ctrl Pts',(3.30660909204321,-26.6077717064107,
88.8926491666568));
#124990=CARTESIAN_POINT('Ctrl Pts',(3.05812708824525,-26.4827613689761,
89.0402227961973));
#124991=CARTESIAN_POINT('Ctrl Pts',(2.79976957900169,-26.3527827028528,
89.1936614950784));
#124992=CARTESIAN_POINT('Ctrl Pts',(2.53981823571299,-26.2134059636382,
89.3423100176492));
#124993=CARTESIAN_POINT('Ctrl Pts',(2.27889797695919,-26.064512216502,89.4859651894051));
#124994=CARTESIAN_POINT('Ctrl Pts',(2.18168862608131,-26.0090398488981,
89.5394858553102));
#124995=CARTESIAN_POINT('Ctrl Pts',(2.08434511443063,-25.9522468182292,
89.592313669351));
#124996=CARTESIAN_POINT('Ctrl Pts',(1.98690080831514,-25.8941281785326,
89.6444390289528));
#124997=CARTESIAN_POINT('Ctrl Pts',(1.72144171495565,-25.7358005961816,
89.7864396368133));
#124998=CARTESIAN_POINT('Ctrl Pts',(1.45523313112368,-25.5676326544185,
89.9232247222671));
#124999=CARTESIAN_POINT('Ctrl Pts',(1.18899435962219,-25.3894973442791,
90.0546604194468));
#125000=CARTESIAN_POINT('Ctrl Pts',(1.09880780979761,-25.3291552350784,
90.099183356454));
#125001=CARTESIAN_POINT('Ctrl Pts',(1.00861796167179,-25.2676697047823,
90.1430927451011));
#125002=CARTESIAN_POINT('Ctrl Pts',(0.918453200391034,-25.2050367529372,
90.1863842595382));
#125003=CARTESIAN_POINT('Ctrl Pts',(0.683510322579977,-25.0418336817674,
90.2991892272681));
#125004=CARTESIAN_POINT('Ctrl Pts',(0.448737285098761,-24.8708383520767,
90.4077974543601));
#125005=CARTESIAN_POINT('Ctrl Pts',(0.214737593717178,-24.6920330679193,
90.5121351745855));
#125006=CARTESIAN_POINT('Origin',(4.0920067733132,-24.696099145329,99.1931566746257));
#125007=CARTESIAN_POINT('Ctrl Pts',(1.36163900653909,-23.0868350636,90.18857710052));
#125008=CARTESIAN_POINT('Ctrl Pts',(1.33629755400909,-23.0868350636,90.1973864042999));
#125009=CARTESIAN_POINT('Ctrl Pts',(1.18340487400909,-23.0868350636,90.24974235902));
#125010=CARTESIAN_POINT('Ctrl Pts',(0.88596103596909,-23.0868350636,90.3426923710499));
#125011=CARTESIAN_POINT('Ctrl Pts',(0.460669337409092,-23.0868350636,90.4582699612699));
#125012=CARTESIAN_POINT('Ctrl Pts',(0.0027641290990888,-23.0868350636,90.5675700300099));
#125013=CARTESIAN_POINT('Ctrl Pts',(-0.472046391840912,-23.0868350636,90.6688291289299));
#125014=CARTESIAN_POINT('Ctrl Pts',(-0.870003116440913,-23.0868350636,90.74660632017));
#125015=CARTESIAN_POINT('Ctrl Pts',(-1.10812696320091,-23.0868350636,90.7911946280099));
#125016=CARTESIAN_POINT('Ctrl Pts',(-1.18647142001091,-23.0868350636,90.80570636327));
#125017=CARTESIAN_POINT('Ctrl Pts',(1.53839445242909,-21.82055408281,90.69703431954));
#125018=CARTESIAN_POINT('Ctrl Pts',(1.51147927430909,-21.82055408281,90.7063904444401));
#125019=CARTESIAN_POINT('Ctrl Pts',(1.34927535701909,-21.82055408281,90.76193375724));
#125020=CARTESIAN_POINT('Ctrl Pts',(1.03585658491909,-21.82055408281,90.8598359761601));
#125021=CARTESIAN_POINT('Ctrl Pts',(0.592965254849087,-21.82055408281,90.98015107536));
#125022=CARTESIAN_POINT('Ctrl Pts',(0.120694188719086,-21.82055408281,91.09284990719));
#125023=CARTESIAN_POINT('Ctrl Pts',(-0.364876444990915,-21.82055408281,
91.19638270328));
#125024=CARTESIAN_POINT('Ctrl Pts',(-0.768844937710913,-21.82055408281,
91.27532498826));
#125025=CARTESIAN_POINT('Ctrl Pts',(-1.00940150886091,-21.82055408281,91.3203684735299));
#125026=CARTESIAN_POINT('Ctrl Pts',(-1.08843051722092,-21.82055408281,91.33500702056));
#125027=CARTESIAN_POINT('Ctrl Pts',(1.25251305092909,-20.75508811698,89.87466383106));
#125028=CARTESIAN_POINT('Ctrl Pts',(1.22814319113909,-20.75508811698,89.88313553631));
#125029=CARTESIAN_POINT('Ctrl Pts',(1.08099911855909,-20.75508811698,89.93352366767));
#125030=CARTESIAN_POINT('Ctrl Pts',(0.793417946619087,-20.75508811698,90.0234162672001));
#125031=CARTESIAN_POINT('Ctrl Pts',(0.378991976119086,-20.75508811698,90.1360689959401));
#125032=CARTESIAN_POINT('Ctrl Pts',(-0.0700439837509129,-20.75508811698,
90.24327072329));
#125033=CARTESIAN_POINT('Ctrl Pts',(-0.538211384980914,-20.75508811698,
90.34312607832));
#125034=CARTESIAN_POINT('Ctrl Pts',(-0.932456541100915,-20.75508811698,
90.42018395951));
#125035=CARTESIAN_POINT('Ctrl Pts',(-1.16907846314091,-20.75508811698,90.46449124816));
#125036=CARTESIAN_POINT('Ctrl Pts',(-1.24700028889091,-20.75508811698,90.47892469189));
#125037=CARTESIAN_POINT('Ctrl Pts',(0.809841866079087,-21.03031417726,88.60126963119));
#125038=CARTESIAN_POINT('Ctrl Pts',(0.78941328779909,-21.03031417726,88.60837186262));
#125039=CARTESIAN_POINT('Ctrl Pts',(0.665588533179087,-21.03031417726,88.6507774870499));
#125040=CARTESIAN_POINT('Ctrl Pts',(0.418015424089088,-21.03031417726,88.72826764384));
#125041=CARTESIAN_POINT('Ctrl Pts',(0.0476664532790877,-21.03031417726,
88.8290556252));
#125042=CARTESIAN_POINT('Ctrl Pts',(-0.36539125839091,-21.03031417726,88.9277453971099));
#125043=CARTESIAN_POINT('Ctrl Pts',(-0.80661073819091,-21.03031417726,89.02190644259));
#125044=CARTESIAN_POINT('Ctrl Pts',(-1.18579985743091,-21.03031417726,89.09604643108));
#125045=CARTESIAN_POINT('Ctrl Pts',(-1.41632919778091,-21.03031417726,89.13921376088));
#125046=CARTESIAN_POINT('Ctrl Pts',(-1.49253661387091,-21.03031417726,89.15332961377));
#125047=CARTESIAN_POINT('',(-1.00776358327158,-22.5000393642437,90.8939758070015));
#125048=CARTESIAN_POINT('',(-1.28514186019175,-21.0000000000091,89.4198403356738));
#125049=CARTESIAN_POINT('Origin',(-1.28514465536091,-22.5,89.4198456395));
#125050=CARTESIAN_POINT('Ctrl Pts',(0.756578721069087,-21.00000000034,88.93560161898));
#125051=CARTESIAN_POINT('Ctrl Pts',(0.653003740499087,-21.00000000034,88.96920956699));
#125052=CARTESIAN_POINT('Ctrl Pts',(0.429939155889087,-20.99999999984,89.03708519515));
#125053=CARTESIAN_POINT('Ctrl Pts',(0.0394814676090878,-21.00000000004,
89.14048085679));
#125054=CARTESIAN_POINT('Ctrl Pts',(-0.384836251440913,-20.99999999999,
89.23943098501));
#125055=CARTESIAN_POINT('Ctrl Pts',(-0.831136955090912,-21.,89.33289755051));
#125056=CARTESIAN_POINT('Ctrl Pts',(-1.13262274867091,-21.,89.39113259042));
#125057=CARTESIAN_POINT('Ctrl Pts',(-1.28513819680091,-21.00000000001,89.41983964605));
#125058=CARTESIAN_POINT('Ctrl Pts',(1.21025704777005,-22.7988943080295,
90.3337993035096));
#125059=CARTESIAN_POINT('Ctrl Pts',(1.11883424343817,-22.7853130337259,
90.3663681552013));
#125060=CARTESIAN_POINT('Ctrl Pts',(1.02596857595066,-22.7717048756296,
90.3976542109587));
#125061=CARTESIAN_POINT('Ctrl Pts',(0.931813726174482,-22.7580801782437,
90.4277751577328));
#125062=CARTESIAN_POINT('Ctrl Pts',(0.840202022289285,-22.7448234873202,
90.4570825302491));
#125063=CARTESIAN_POINT('Ctrl Pts',(0.747372442868353,-22.7315511422234,
90.485287389861));
#125064=CARTESIAN_POINT('Ctrl Pts',(0.653326688054345,-22.7182727250757,
90.5125156428743));
#125065=CARTESIAN_POINT('Ctrl Pts',(0.602522516857858,-22.7110996317305,
90.5272245346281));
#125066=CARTESIAN_POINT('Ctrl Pts',(0.551363182508309,-22.7039247670197,
90.5416492614627));
#125067=CARTESIAN_POINT('Ctrl Pts',(0.499847108697976,-22.696749642616,
90.5558157707814));
#125068=CARTESIAN_POINT('Ctrl Pts',(0.395200362092091,-22.6821745135387,
90.5845927912591));
#125069=CARTESIAN_POINT('Ctrl Pts',(0.289081810103877,-22.6675983181277,
90.6123016588467));
#125070=CARTESIAN_POINT('Ctrl Pts',(0.181529294844612,-22.653033691233,
90.6390726080421));
#125071=CARTESIAN_POINT('Ctrl Pts',(0.133050478942922,-22.6464687507088,
90.6511394938274));
#125072=CARTESIAN_POINT('Ctrl Pts',(0.0842802116893185,-22.6399061596043,
90.6630165007185));
#125073=CARTESIAN_POINT('Ctrl Pts',(0.0352214027325707,-22.6333470682069,
90.6747190033485));
#125074=CARTESIAN_POINT('Ctrl Pts',(-0.0778601668898635,-22.6182282268349,
90.7016935140235));
#125075=CARTESIAN_POINT('Ctrl Pts',(-0.192474304323062,-22.60312799504,
90.7277376446242));
#125076=CARTESIAN_POINT('Ctrl Pts',(-0.30858246594518,-22.58806032326,90.7530081683137));
#125077=CARTESIAN_POINT('Ctrl Pts',(-0.35395508725891,-22.5821721948442,
90.7628833561192));
#125078=CARTESIAN_POINT('Ctrl Pts',(-0.39955594211883,-22.576289036217,
90.7726409553093));
#125079=CARTESIAN_POINT('Ctrl Pts',(-0.445383055984327,-22.5704116694695,
90.782292479886));
#125080=CARTESIAN_POINT('Ctrl Pts',(-0.566668934225101,-22.5548566513245,
90.8078361708562));
#125081=CARTESIAN_POINT('Ctrl Pts',(-0.689539096038413,-22.5393422305868,
90.832633381094));
#125082=CARTESIAN_POINT('Ctrl Pts',(-0.813956921433526,-22.5238833956251,
90.856869529174));
#125083=CARTESIAN_POINT('Ctrl Pts',(-0.852043593115456,-22.5191511511103,
90.8642886768069));
#125084=CARTESIAN_POINT('Ctrl Pts',(-0.890275349954781,-22.5144241126308,
90.8716556097766));
#125085=CARTESIAN_POINT('Ctrl Pts',(-0.928651288068415,-22.5097027021494,
90.8789766224509));
#125086=CARTESIAN_POINT('Ctrl Pts',(-0.954936548950239,-22.5064688136157,
90.8839910856152));
#125087=CARTESIAN_POINT('Ctrl Pts',(-0.981289452544953,-22.5032375653443,
90.8889840167774));
#125088=CARTESIAN_POINT('Ctrl Pts',(-1.00770989807145,-22.500009091799,
90.8939570738426));
#125089=CARTESIAN_POINT('Ctrl Pts',(-6.25976359311891,-21.0101086723,86.80605952089));
#125090=CARTESIAN_POINT('Ctrl Pts',(-6.20991132790791,-20.99698855152,86.80345236223));
#125091=CARTESIAN_POINT('Ctrl Pts',(-6.05600621273991,-20.963809122,86.7954056045899));
#125092=CARTESIAN_POINT('Ctrl Pts',(-5.89752936873391,-20.95187439198,86.78709081339));
#125093=CARTESIAN_POINT('Ctrl Pts',(-5.79082527707091,-20.95374691807,86.7814767506699));
#125094=CARTESIAN_POINT('Ctrl Pts',(-6.36253180399691,-21.23537119951,85.92231661493));
#125095=CARTESIAN_POINT('Ctrl Pts',(-6.31814829585091,-21.22933598386,85.92215256487));
#125096=CARTESIAN_POINT('Ctrl Pts',(-6.18252552805991,-21.21729456478,85.92204034661));
#125097=CARTESIAN_POINT('Ctrl Pts',(-6.04735840947691,-21.22429001182,85.92328042834));
#125098=CARTESIAN_POINT('Ctrl Pts',(-5.95842995311291,-21.23703750146,85.9247493404201));
#125099=CARTESIAN_POINT('Ctrl Pts',(-6.62085321050291,-20.57398746247,85.34080893105));
#125100=CARTESIAN_POINT('Ctrl Pts',(-6.55589593677591,-20.56692097113,85.33267979129));
#125101=CARTESIAN_POINT('Ctrl Pts',(-6.35811797501791,-20.55529791815,85.3082833307501));
#125102=CARTESIAN_POINT('Ctrl Pts',(-6.16331684750191,-20.57308609787,85.2855875247701));
#125103=CARTESIAN_POINT('Ctrl Pts',(-6.03626442425791,-20.59714856909,85.2714418523801));
#125104=CARTESIAN_POINT('Ctrl Pts',(-6.75819841819991,-19.73395935219,85.68403218053));
#125105=CARTESIAN_POINT('Ctrl Pts',(-6.66864877990991,-19.71884937032,85.6660562680899));
#125106=CARTESIAN_POINT('Ctrl Pts',(-6.39481433463891,-19.68647718414,85.61115271986));
#125107=CARTESIAN_POINT('Ctrl Pts',(-6.12127282288791,-19.69536718519,85.55665329315));
#125108=CARTESIAN_POINT('Ctrl Pts',(-5.94100799531891,-19.71907212904,85.52091066777));
#125109=CARTESIAN_POINT('',(-6.21291707614173,-21.0225426194874,86.5058300720823));
#125110=CARTESIAN_POINT('',(-6.5468225705719,-20.0375665162624,85.5854070569733));
#125111=CARTESIAN_POINT('Origin',(-6.37317299992691,-20.0375768096,86.57021276289));
#125112=CARTESIAN_POINT('Origin',(-6.11241447398738,-22.6085115286827,85.5088316030536));
#125113=CARTESIAN_POINT('Origin',(-5.9375029357236,-22.6813923363259,86.5223306616674));
#125114=CARTESIAN_POINT('Origin',(155.459720656869,-21.,57.01928063319));
#125115=CARTESIAN_POINT('',(-5.70733054565492,-21.0000000000039,87.0513884694139));
#125116=CARTESIAN_POINT('Origin',(-2.02513312664091,-21.00000000001,85.48888938658));
#125117=CARTESIAN_POINT('Origin',(27.4324635166691,-21.,72.98888938658));
#125118=CARTESIAN_POINT('Ctrl Pts',(-9.31134522286991,-23.33493700796,85.4554385022599));
#125119=CARTESIAN_POINT('Ctrl Pts',(-9.28499288372891,-23.28758267006,85.50448598234));
#125120=CARTESIAN_POINT('Ctrl Pts',(-9.19047003471491,-23.12655314471,85.66856307458));
#125121=CARTESIAN_POINT('Ctrl Pts',(-9.0098363850229,-22.86492193384,85.9192200995));
#125122=CARTESIAN_POINT('Ctrl Pts',(-8.75884674055692,-22.5625884577,86.18264969547));
#125123=CARTESIAN_POINT('Ctrl Pts',(-8.49981345722091,-22.29401394629,86.39371900856));
#125124=CARTESIAN_POINT('Ctrl Pts',(-8.23984516015692,-22.05730715509,86.5593464839501));
#125125=CARTESIAN_POINT('Ctrl Pts',(-7.98398752470691,-21.85037332061,86.6857732052299));
#125126=CARTESIAN_POINT('Ctrl Pts',(-7.73566246859491,-21.67095709777,86.77861968057));
#125127=CARTESIAN_POINT('Ctrl Pts',(-7.4973815228969,-21.51699185038,86.84277779335));
#125128=CARTESIAN_POINT('Ctrl Pts',(-7.27102440704691,-21.386549034,86.88261210473));
#125129=CARTESIAN_POINT('Ctrl Pts',(-7.05796092602491,-21.2777684576,86.90210334931));
#125130=CARTESIAN_POINT('Ctrl Pts',(-6.85943856171691,-21.18897387943,86.9049046154299));
#125131=CARTESIAN_POINT('Ctrl Pts',(-6.67670949594691,-21.11854136463,86.8945490446601));
#125132=CARTESIAN_POINT('Ctrl Pts',(-6.51034314219591,-21.06450784875,86.87448931141));
#125133=CARTESIAN_POINT('Ctrl Pts',(-6.35927469654491,-21.02446132003,86.84768246284));
#125134=CARTESIAN_POINT('Ctrl Pts',(-6.22090131047091,-20.99596779402,86.81617682313));
#125135=CARTESIAN_POINT('Ctrl Pts',(-6.10579036137791,-20.97909200866,86.78485289377));
#125136=CARTESIAN_POINT('Ctrl Pts',(-6.03665598268991,-20.97241818335,86.7637314788699));
#125137=CARTESIAN_POINT('Ctrl Pts',(-6.00965782959991,-20.97035997432,86.7551449868199));
#125138=CARTESIAN_POINT('Ctrl Pts',(-8.4350370823869,-23.50439686796,85.39546316836));
#125139=CARTESIAN_POINT('Ctrl Pts',(-8.40984591433391,-23.45695203024,85.4275369102899));
#125140=CARTESIAN_POINT('Ctrl Pts',(-8.32096735149791,-23.295774178,85.53371911941));
#125141=CARTESIAN_POINT('Ctrl Pts',(-8.15928441830591,-23.0347138024,85.68952154615));
#125142=CARTESIAN_POINT('Ctrl Pts',(-7.94691404596691,-22.73437091822,85.84244627094));
#125143=CARTESIAN_POINT('Ctrl Pts',(-7.73767036549491,-22.46881609534,85.95482781482));
#125144=CARTESIAN_POINT('Ctrl Pts',(-7.53628477743691,-22.23597796783,86.0332540986199));
#125145=CARTESIAN_POINT('Ctrl Pts',(-7.34594773687791,-22.03361870056,86.08348958725));
#125146=CARTESIAN_POINT('Ctrl Pts',(-7.16868354027591,-21.85935874251,86.11059919866));
#125147=CARTESIAN_POINT('Ctrl Pts',(-7.0058965082479,-21.71100809099,86.11900317502));
#125148=CARTESIAN_POINT('Ctrl Pts',(-6.85853254906791,-21.58650051732,86.11268429546));
#125149=CARTESIAN_POINT('Ctrl Pts',(-6.7271147517219,-21.48381351961,86.09531628731));
#125150=CARTESIAN_POINT('Ctrl Pts',(-6.61192983251291,-21.40106859032,86.07035403811));
#125151=CARTESIAN_POINT('Ctrl Pts',(-6.51295284246591,-21.33639303747,86.0411390717));
#125152=CARTESIAN_POINT('Ctrl Pts',(-6.42933637844591,-21.28756622125,86.01071140893));
#125153=CARTESIAN_POINT('Ctrl Pts',(-6.35905177532891,-21.25197480454,85.98135155073));
#125154=CARTESIAN_POINT('Ctrl Pts',(-6.29925123788791,-21.22705685392,85.95440275155));
#125155=CARTESIAN_POINT('Ctrl Pts',(-6.25250368986091,-21.21251241075,85.93304888243));
#125156=CARTESIAN_POINT('Ctrl Pts',(-6.22536410282091,-21.20680909012,85.92116194032));
#125157=CARTESIAN_POINT('Ctrl Pts',(-6.21483774804991,-21.20505475476,85.91669105491));
#125158=CARTESIAN_POINT('Ctrl Pts',(-7.94712863324292,-23.04130212549,84.80577059714));
#125159=CARTESIAN_POINT('Ctrl Pts',(-7.93348145948992,-22.99410460291,84.82813589426));
#125160=CARTESIAN_POINT('Ctrl Pts',(-7.88483370393191,-22.83333209387,84.90272578354));
#125161=CARTESIAN_POINT('Ctrl Pts',(-7.79354048754991,-22.57071175704,85.01536177068));
#125162=CARTESIAN_POINT('Ctrl Pts',(-7.66920664452491,-22.26492904381,85.13152091435));
#125163=CARTESIAN_POINT('Ctrl Pts',(-7.54292338971691,-21.99112210811,85.2225126459599));
#125164=CARTESIAN_POINT('Ctrl Pts',(-7.41794917868591,-21.74771181434,85.29191458303));
#125165=CARTESIAN_POINT('Ctrl Pts',(-7.29656245333991,-21.53285130916,85.3429175053));
#125166=CARTESIAN_POINT('Ctrl Pts',(-7.18027985650291,-21.34450046779,85.3783690288999));
#125167=CARTESIAN_POINT('Ctrl Pts',(-7.07019785162091,-21.18080641974,85.40075005732));
#125168=CARTESIAN_POINT('Ctrl Pts',(-6.96711552884591,-21.04007919563,85.41228205909));
#125169=CARTESIAN_POINT('Ctrl Pts',(-6.8715811492079,-20.9207398517,85.41499958511));
#125170=CARTESIAN_POINT('Ctrl Pts',(-6.78405515274891,-20.82146262628,85.41078684325));
#125171=CARTESIAN_POINT('Ctrl Pts',(-6.70493563279891,-20.74105462321,85.40146619008));
#125172=CARTESIAN_POINT('Ctrl Pts',(-6.63423230918392,-20.6779990968,85.3887722936999));
#125173=CARTESIAN_POINT('Ctrl Pts',(-6.57118663989192,-20.63023288573,85.37412460379));
#125174=CARTESIAN_POINT('Ctrl Pts',(-6.51437698962792,-20.59554371159,85.35845791767));
#125175=CARTESIAN_POINT('Ctrl Pts',(-6.46773244924391,-20.57462824752,85.34399614184));
#125176=CARTESIAN_POINT('Ctrl Pts',(-6.4399101321309,-20.56627276126,85.33475936856));
#125177=CARTESIAN_POINT('Ctrl Pts',(-6.42905981978291,-20.56368800922,85.33107841599));
#125178=CARTESIAN_POINT('Ctrl Pts',(-8.35461977250192,-22.42686803145,84.29912753498));
#125179=CARTESIAN_POINT('Ctrl Pts',(-8.35090371515592,-22.37999864658,84.3291380087));
#125180=CARTESIAN_POINT('Ctrl Pts',(-8.3352682829919,-22.2197639469,84.4312666422201));
#125181=CARTESIAN_POINT('Ctrl Pts',(-8.29265977640492,-21.95507385353,84.5972798544901));
#125182=CARTESIAN_POINT('Ctrl Pts',(-8.21429839509991,-21.64207357524,84.7886168945501));
#125183=CARTESIAN_POINT('Ctrl Pts',(-8.11793979130091,-21.35731773644,84.95774354849));
#125184=CARTESIAN_POINT('Ctrl Pts',(-8.00780433526691,-21.0998802927,85.1056754455199));
#125185=CARTESIAN_POINT('Ctrl Pts',(-7.8871493623079,-20.86843314535,85.2336070050299));
#125186=CARTESIAN_POINT('Ctrl Pts',(-7.7584013469319,-20.66138652028,85.34281089274));
#125187=CARTESIAN_POINT('Ctrl Pts',(-7.6234681520699,-20.47733485406,85.43437619933));
#125188=CARTESIAN_POINT('Ctrl Pts',(-7.48394160578191,-20.31508739811,85.50921378337));
#125189=CARTESIAN_POINT('Ctrl Pts',(-7.34124087217191,-20.17365372159,85.5680901662));
#125190=CARTESIAN_POINT('Ctrl Pts',(-7.19695408294091,-20.05244144602,85.61157853619));
#125191=CARTESIAN_POINT('Ctrl Pts',(-7.05316295123591,-19.95115962835,85.64023314414));
#125192=CARTESIAN_POINT('Ctrl Pts',(-6.91211759795191,-19.86922544959,85.6549470362799));
#125193=CARTESIAN_POINT('Ctrl Pts',(-6.77524376654791,-19.80530572163,85.6569888494899));
#125194=CARTESIAN_POINT('Ctrl Pts',(-6.64273512392691,-19.75765208834,85.64760597632));
#125195=CARTESIAN_POINT('Ctrl Pts',(-6.52782615951691,-19.72828355387,85.6297965517001));
#125196=CARTESIAN_POINT('Ctrl Pts',(-6.45735303533591,-19.71640917432,85.61387177559));
#125197=CARTESIAN_POINT('Ctrl Pts',(-6.42971964328091,-19.71272262543,85.6068342398));
#125198=CARTESIAN_POINT('Ctrl Pts',(-8.23395173885433,-22.5,84.5714980228305));
#125199=CARTESIAN_POINT('Ctrl Pts',(-8.21609487741167,-22.4068116375628,
84.6264627209876));
#125200=CARTESIAN_POINT('Ctrl Pts',(-8.19563729693556,-22.316592985688,
84.6786894498294));
#125201=CARTESIAN_POINT('Ctrl Pts',(-8.17316811952911,-22.2295003482217,
84.7281880289493));
#125202=CARTESIAN_POINT('Ctrl Pts',(-8.16832056716124,-22.2107107809253,
84.7388669670376));
#125203=CARTESIAN_POINT('Ctrl Pts',(-8.16337943807854,-22.1920665946948,
84.7494190677838));
#125204=CARTESIAN_POINT('Ctrl Pts',(-8.1583507236139,-22.1735691653645,
84.7598446655152));
#125205=CARTESIAN_POINT('Ctrl Pts',(-8.15717124053408,-22.1692306002961,
84.7622899855285));
#125206=CARTESIAN_POINT('Ctrl Pts',(-8.15598693964693,-22.1649001132339,
84.7647283456416));
#125207=CARTESIAN_POINT('Ctrl Pts',(-8.15479788384955,-22.1605776812017,
84.7671597802231));
#125208=CARTESIAN_POINT('Ctrl Pts',(-8.13546187554057,-22.09028780761,84.8066989165476));
#125209=CARTESIAN_POINT('Ctrl Pts',(-8.11487172341013,-22.0221309939227,
84.8444053993864));
#125210=CARTESIAN_POINT('Ctrl Pts',(-8.09327142289032,-21.9560751966656,
84.8803769914104));
#125211=CARTESIAN_POINT('Ctrl Pts',(-8.08428709169013,-21.9286002474302,
84.8953388525311));
#125212=CARTESIAN_POINT('Ctrl Pts',(-8.07512753850495,-21.9014883623869,
84.9100007460101));
#125213=CARTESIAN_POINT('Ctrl Pts',(-8.06580839124876,-21.8747356121368,
84.9243703323895));
#125214=CARTESIAN_POINT('Ctrl Pts',(-8.0630516692208,-21.8668218090929,
84.9286210384053));
#125215=CARTESIAN_POINT('Ctrl Pts',(-8.06028098400575,-21.8589394443409,
84.9328461531074));
#125216=CARTESIAN_POINT('Ctrl Pts',(-8.05749675602641,-21.8510884665214,
84.9370458299792));
#125217=CARTESIAN_POINT('Ctrl Pts',(-8.0321399670793,-21.7795872859154,
84.9752935312716));
#125218=CARTESIAN_POINT('Ctrl Pts',(-8.00566235701005,-21.7106926989649,
85.0114295529073));
#125219=CARTESIAN_POINT('Ctrl Pts',(-7.97833258524892,-21.6443451374452,
85.0455700289277));
#125220=CARTESIAN_POINT('Ctrl Pts',(-7.97262937400217,-21.6304996446119,
85.0526945065308));
#125221=CARTESIAN_POINT('Ctrl Pts',(-7.96688894881453,-21.6167649379167,
85.0597321527015));
#125222=CARTESIAN_POINT('Ctrl Pts',(-7.96111358632208,-21.6031402786599,
85.0666841259067));
#125223=CARTESIAN_POINT('Ctrl Pts',(-7.95655569992873,-21.5923877676058,
85.0721705874267));
#125224=CARTESIAN_POINT('Ctrl Pts',(-7.95197608277586,-21.5817039214224,
85.0776036540415));
#125225=CARTESIAN_POINT('Ctrl Pts',(-7.94737578754198,-21.5710882773315,
85.0829839580058));
#125226=CARTESIAN_POINT('Ctrl Pts',(-7.9189919510701,-21.5055897189562,
85.1161804508671));
#125227=CARTESIAN_POINT('Ctrl Pts',(-7.88982332230086,-21.442690854516,
85.1473666462622));
#125228=CARTESIAN_POINT('Ctrl Pts',(-7.86008135930843,-21.382298961433,
85.1766706697932));
#125229=CARTESIAN_POINT('Ctrl Pts',(-7.85605227772784,-21.3741177978663,
85.18064042463));
#125230=CARTESIAN_POINT('Ctrl Pts',(-7.85201262971751,-21.3659825840344,
85.1845756664998));
#125231=CARTESIAN_POINT('Ctrl Pts',(-7.84796289870774,-21.3578930384239,
85.1884767380341));
#125232=CARTESIAN_POINT('Ctrl Pts',(-7.84150175753707,-21.3449865772121,
85.1947007005242));
#125233=CARTESIAN_POINT('Ctrl Pts',(-7.83501500635689,-21.3321966058346,
85.2008376333083));
#125234=CARTESIAN_POINT('Ctrl Pts',(-7.82850443275156,-21.3195216462603,
85.2068890661026));
#125235=CARTESIAN_POINT('Ctrl Pts',(-7.79757970098214,-21.2593165477873,
85.2356329137769));
#125236=CARTESIAN_POINT('Ctrl Pts',(-7.76612012353127,-21.2017094488401,
85.2624463516647));
#125237=CARTESIAN_POINT('Ctrl Pts',(-7.73428116833124,-21.1465576100225,
85.2874725851855));
#125238=CARTESIAN_POINT('Ctrl Pts',(-7.7325816659029,-21.1436137105318,
85.288808437583));
#125239=CARTESIAN_POINT('Ctrl Pts',(-7.7308810746105,-21.1406767981643,
85.2901392012988));
#125240=CARTESIAN_POINT('Ctrl Pts',(-7.72917941540612,-21.1377468484969,
85.2914648991735));
#125241=CARTESIAN_POINT('Ctrl Pts',(-7.7207908080919,-21.1233031824875,
85.2980001436337));
#125242=CARTESIAN_POINT('Ctrl Pts',(-7.71237638460782,-21.1090291814494,
85.3044121822821));
#125243=CARTESIAN_POINT('Ctrl Pts',(-7.70393847386822,-21.094921727032,
85.3107038484261));
#125244=CARTESIAN_POINT('Ctrl Pts',(-7.67184699656642,-21.0412675622518,
85.3346326226784));
#125245=CARTESIAN_POINT('Ctrl Pts',(-7.63941827929952,-20.9900251945777,
85.3568192087859));
#125246=CARTESIAN_POINT('Ctrl Pts',(-7.60675049093118,-20.9410460703631,
85.3773953104988));
#125247=CARTESIAN_POINT('Ctrl Pts',(-7.59644995709495,-20.9256023825152,
85.3838831948184));
#125248=CARTESIAN_POINT('Ctrl Pts',(-7.58612566976997,-20.9103839950355,
85.3902108619718));
#125249=CARTESIAN_POINT('Ctrl Pts',(-7.57578194958231,-20.89538828511,85.3963815542268));
#125250=CARTESIAN_POINT('Ctrl Pts',(-7.54469546302359,-20.8503209469976,
85.4149266364955));
#125251=CARTESIAN_POINT('Ctrl Pts',(-7.51343434563313,-20.807267573974,
85.4320523721681));
#125252=CARTESIAN_POINT('Ctrl Pts',(-7.48210528888147,-20.7661744671713,
85.4478328690123));
#125253=CARTESIAN_POINT('Ctrl Pts',(-7.46993905493201,-20.7502164906821,
85.4539610208417));
#125254=CARTESIAN_POINT('Ctrl Pts',(-7.4577626784941,-20.7345546856784,
85.4598863994543));
#125255=CARTESIAN_POINT('Ctrl Pts',(-7.44558104050676,-20.7191833921662,
85.4656144281874));
#125256=CARTESIAN_POINT('Ctrl Pts',(-7.41595632336812,-20.6818017015572,
85.4795445114125));
#125257=CARTESIAN_POINT('Ctrl Pts',(-7.38630150114422,-20.6461400595536,
85.4923065228914));
#125258=CARTESIAN_POINT('Ctrl Pts',(-7.3566796152423,-20.6121347464711,
85.5039653794934));
#125259=CARTESIAN_POINT('Ctrl Pts',(-7.34275950248185,-20.5961547445857,
85.5094441865853));
#125260=CARTESIAN_POINT('Ctrl Pts',(-7.32884685141897,-20.5805413456455,
85.514679426976));
#125261=CARTESIAN_POINT('Ctrl Pts',(-7.31494462205447,-20.5652838484883,
85.5196794165379));
#125262=CARTESIAN_POINT('Ctrl Pts',(-7.28709819590326,-20.5347227955304,
85.5296944894045));
#125263=CARTESIAN_POINT('Ctrl Pts',(-7.25929464945993,-20.5055906815646,
85.5387654561346));
#125264=CARTESIAN_POINT('Ctrl Pts',(-7.23155263669677,-20.477820081468,
85.5469457005477));
#125265=CARTESIAN_POINT('Ctrl Pts',(-7.21598901700505,-20.462240423921,
85.5515349210241));
#125266=CARTESIAN_POINT('Ctrl Pts',(-7.20044538808841,-20.4470894585749,
85.5558434744203));
#125267=CARTESIAN_POINT('Ctrl Pts',(-7.184933585593,-20.4323636783849,85.5598786279935));
#125268=CARTESIAN_POINT('Ctrl Pts',(-7.15899174990591,-20.4077363811918,
85.5666269920859));
#125269=CARTESIAN_POINT('Ctrl Pts',(-7.13313936171369,-20.3842994707439,
85.5726100926947));
#125270=CARTESIAN_POINT('Ctrl Pts',(-7.10743707658413,-20.3620447045031,
85.5778590282367));
#125271=CARTESIAN_POINT('Ctrl Pts',(-7.09034758997357,-20.3472474781951,
85.5813490530812));
#125272=CARTESIAN_POINT('Ctrl Pts',(-7.07332502324638,-20.3329726384921,
85.5845144972691));
#125273=CARTESIAN_POINT('Ctrl Pts',(-7.05639340493283,-20.3192185126292,
85.5873657595805));
#125274=CARTESIAN_POINT('Ctrl Pts',(-7.03263357576654,-20.2999176002897,
85.5913668836416));
#125275=CARTESIAN_POINT('Ctrl Pts',(-7.00905319070198,-20.2816430035672,
85.5947488602904));
#125276=CARTESIAN_POINT('Ctrl Pts',(-6.9857261746476,-20.2643903645038,
85.5975435664691));
#125277=CARTESIAN_POINT('Ctrl Pts',(-6.96742649372553,-20.2508559377606,
85.5997359699561));
#125278=CARTESIAN_POINT('Ctrl Pts',(-6.94928267677856,-20.237951007443,
85.6015674054324));
#125279=CARTESIAN_POINT('Ctrl Pts',(-6.93131002919188,-20.2256539965921,
85.6030583215737));
#125280=CARTESIAN_POINT('Ctrl Pts',(-6.91004642120851,-20.2111052876811,
85.6048222384486));
#125281=CARTESIAN_POINT('Ctrl Pts',(-6.88902273918636,-20.1974077367977,
85.606109504425));
#125282=CARTESIAN_POINT('Ctrl Pts',(-6.86826729763053,-20.1845277817933,
85.6069539388812));
#125283=CARTESIAN_POINT('Ctrl Pts',(-6.84914188148638,-20.172659352075,
85.6077320558072));
#125284=CARTESIAN_POINT('Ctrl Pts',(-6.83024405342614,-20.1614855334301,
85.6081344160708));
#125285=CARTESIAN_POINT('Ctrl Pts',(-6.81157466760304,-20.1509669364568,
85.6081875725525));
#125286=CARTESIAN_POINT('Ctrl Pts',(-6.79285868093349,-20.140422083905,
85.6082408617186));
#125287=CARTESIAN_POINT('Ctrl Pts',(-6.77437236819119,-20.1305356928375,
85.6079432628828));
#125288=CARTESIAN_POINT('Ctrl Pts',(-6.75611755799409,-20.1212710245048,
85.6073201220557));
#125289=CARTESIAN_POINT('Ctrl Pts',(-6.73638327829304,-20.111255496858,
85.6066464784931));
#125290=CARTESIAN_POINT('Ctrl Pts',(-6.71691930222018,-20.1019677281025,
85.6055929164435));
#125291=CARTESIAN_POINT('Ctrl Pts',(-6.69768443571138,-20.0933512015893,
85.6041834821669));
#125292=CARTESIAN_POINT('Ctrl Pts',(-6.68137792897692,-20.0860464746472,
85.6029886233665));
#125293=CARTESIAN_POINT('Ctrl Pts',(-6.6652359218369,-20.0792242508093,
85.6015378792598));
#125294=CARTESIAN_POINT('Ctrl Pts',(-6.64923350344088,-20.072855918317,
85.599842182004));
#125295=CARTESIAN_POINT('Ctrl Pts',(-6.62896111745131,-20.0647883068349,
85.5976940173679));
#125296=CARTESIAN_POINT('Ctrl Pts',(-6.60891363092771,-20.0574444366806,
85.5951518701932));
#125297=CARTESIAN_POINT('Ctrl Pts',(-6.58913563150429,-20.0508103664085,
85.5922443617696));
#125298=CARTESIAN_POINT('Ctrl Pts',(-6.57488563962315,-20.0460305377973,
85.5901495102861));
#125299=CARTESIAN_POINT('Ctrl Pts',(-6.56077545734654,-20.0416189903231,
85.5878650765649));
#125300=CARTESIAN_POINT('Ctrl Pts',(-6.54682296816177,-20.0375665177092,
85.5854047998161));
#125301=CARTESIAN_POINT('Ctrl Pts',(-8.23395173885433,-22.5,84.5714980228305));
#125302=CARTESIAN_POINT('Ctrl Pts',(-8.21516313921569,-22.4637909993162,
84.6293396005463));
#125303=CARTESIAN_POINT('Ctrl Pts',(-8.19537632053088,-22.4283109296505,
84.6855617234812));
#125304=CARTESIAN_POINT('Ctrl Pts',(-8.17476407227142,-22.393589005892,
84.7401422899255));
#125305=CARTESIAN_POINT('Ctrl Pts',(-8.15671077006665,-22.3631777002037,
84.7879468500163));
#125306=CARTESIAN_POINT('Ctrl Pts',(-8.13802383025153,-22.3333487538864,
84.8344926324756));
#125307=CARTESIAN_POINT('Ctrl Pts',(-8.11881620643752,-22.3041412702589,
84.8797910935868));
#125308=CARTESIAN_POINT('Ctrl Pts',(-8.11710382636405,-22.3015373920569,
84.88382949953));
#125309=CARTESIAN_POINT('Ctrl Pts',(-8.11538731317498,-22.2989384496591,
84.8878579869973));
#125310=CARTESIAN_POINT('Ctrl Pts',(-8.11366673296642,-22.2963444085858,
84.8918765846372));
#125311=CARTESIAN_POINT('Ctrl Pts',(-8.0897968412713,-22.2603568509209,
84.9476272494163));
#125312=CARTESIAN_POINT('Ctrl Pts',(-8.06514684457484,-22.2253110021173,
85.0014709552372));
#125313=CARTESIAN_POINT('Ctrl Pts',(-8.03987636784091,-22.1911816240943,
85.0534715425807));
#125314=CARTESIAN_POINT('Ctrl Pts',(-8.02320821822501,-22.1686702332261,
85.0877706014818));
#125315=CARTESIAN_POINT('Ctrl Pts',(-8.0062694224247,-22.1465580108257,
85.1212686975038));
#125316=CARTESIAN_POINT('Ctrl Pts',(-7.98909910267082,-22.1248416438096,
85.1539936246758));
#125317=CARTESIAN_POINT('Ctrl Pts',(-7.98534474887514,-22.1200932799991,
85.1611490508008));
#125318=CARTESIAN_POINT('Ctrl Pts',(-7.98157932470578,-22.1153638238704,
85.1682674700585));
#125319=CARTESIAN_POINT('Ctrl Pts',(-7.9778032608764,-22.1106532030564,
85.175349023635));
#125320=CARTESIAN_POINT('Ctrl Pts',(-7.94852432800735,-22.0741278801764,
85.2302581409442));
#125321=CARTESIAN_POINT('Ctrl Pts',(-7.91860782492171,-22.0387338144514,
85.2829470085377));
#125322=CARTESIAN_POINT('Ctrl Pts',(-7.88822657837118,-22.004449586861,
85.3335014088525));
#125323=CARTESIAN_POINT('Ctrl Pts',(-7.87547986902107,-21.9900653487534,
85.3547119357514));
#125324=CARTESIAN_POINT('Ctrl Pts',(-7.86265104172624,-21.9758766378046,
85.3755472904137));
#125325=CARTESIAN_POINT('Ctrl Pts',(-7.84975157984563,-21.9618824200467,
85.3960160906175));
#125326=CARTESIAN_POINT('Ctrl Pts',(-7.84380464228576,-21.9554307757863,
85.4054526607522));
#125327=CARTESIAN_POINT('Ctrl Pts',(-7.83784275699324,-21.949020523473,
85.4148111914716));
#125328=CARTESIAN_POINT('Ctrl Pts',(-7.83186694184561,-21.9426512253961,
85.4240923487898));
#125329=CARTESIAN_POINT('Ctrl Pts',(-7.79856222503536,-21.9071535295188,
85.4758185666391));
#125330=CARTESIAN_POINT('Ctrl Pts',(-7.76482751222371,-21.8729277948954,
85.5251380270165));
#125331=CARTESIAN_POINT('Ctrl Pts',(-7.73082285967433,-21.8399335685685,
85.5721737374828));
#125332=CARTESIAN_POINT('Ctrl Pts',(-7.72208232225891,-21.8314527505603,
85.5842637709449));
#125333=CARTESIAN_POINT('Ctrl Pts',(-7.71332377777891,-21.8230533025536,
85.596203127984));
#125334=CARTESIAN_POINT('Ctrl Pts',(-7.70454958924842,-21.8147345355726,
85.6079943060831));
#125335=CARTESIAN_POINT('Ctrl Pts',(-7.69638193440349,-21.8069908203333,
85.6189703949367));
#125336=CARTESIAN_POINT('Ctrl Pts',(-7.68820087496758,-21.7993171648251,
85.6298178953534));
#125337=CARTESIAN_POINT('Ctrl Pts',(-7.68000800769289,-21.791712453889,
85.6405386121853));
#125338=CARTESIAN_POINT('Ctrl Pts',(-7.64389923360224,-21.7581958863665,
85.6877884856661));
#125339=CARTESIAN_POINT('Ctrl Pts',(-7.60756450920095,-21.7260191702926,
85.7325732292101));
#125340=CARTESIAN_POINT('Ctrl Pts',(-7.57112643839262,-21.6951172731443,
85.7750551354326));
#125341=CARTESIAN_POINT('Ctrl Pts',(-7.56619751991202,-21.6909372238562,
85.7808015936843));
#125342=CARTESIAN_POINT('Ctrl Pts',(-7.56126664530471,-21.6867804895583,
85.7865059566646));
#125343=CARTESIAN_POINT('Ctrl Pts',(-7.55633405710516,-21.6826468987909,
85.7921686615137));
#125344=CARTESIAN_POINT('Ctrl Pts',(-7.54599295193706,-21.6739808810496,
85.8040404464694));
#125345=CARTESIAN_POINT('Ctrl Pts',(-7.53564465326263,-21.665416940057,
85.8157289319937));
#125346=CARTESIAN_POINT('Ctrl Pts',(-7.52529102525006,-21.6569528433106,
85.8272375230484));
#125347=CARTESIAN_POINT('Ctrl Pts',(-7.48591297578626,-21.6247612656395,
85.8710082541641));
#125348=CARTESIAN_POINT('Ctrl Pts',(-7.44646243495958,-21.5940151597803,
85.9121755393748));
#125349=CARTESIAN_POINT('Ctrl Pts',(-7.40703126209498,-21.5646271272466,
85.9509322071749));
#125350=CARTESIAN_POINT('Ctrl Pts',(-7.39459833707732,-21.5553608747269,
85.9631524560209));
#125351=CARTESIAN_POINT('Ctrl Pts',(-7.38216737807832,-21.5462301568784,
85.9751332185511));
#125352=CARTESIAN_POINT('Ctrl Pts',(-7.36974224252354,-21.5372329843712,
85.9868776265169));
#125353=CARTESIAN_POINT('Ctrl Pts',(-7.33239980939396,-21.5101929322747,
86.0221742047455));
#125354=CARTESIAN_POINT('Ctrl Pts',(-7.29511245957576,-21.4843604653004,
86.0553350106453));
#125355=CARTESIAN_POINT('Ctrl Pts',(-7.25799097947772,-21.4597047804485,
86.0864591384738));
#125356=CARTESIAN_POINT('Ctrl Pts',(-7.24357553249829,-21.4501301967631,
86.0985456235306));
#125357=CARTESIAN_POINT('Ctrl Pts',(-7.22918530724825,-21.4407334617653,
86.1103252009181));
#125358=CARTESIAN_POINT('Ctrl Pts',(-7.21482430868666,-21.4315109200846,
86.1218036380714));
#125359=CARTESIAN_POINT('Ctrl Pts',(-7.17989907466988,-21.4090821575549,
86.1497186261558));
#125360=CARTESIAN_POINT('Ctrl Pts',(-7.1451486333736,-21.3876844720568,
86.1758528094717));
#125361=CARTESIAN_POINT('Ctrl Pts',(-7.11063583301104,-21.3672816186261,
86.2003008191494));
#125362=CARTESIAN_POINT('Ctrl Pts',(-7.09441751541707,-21.357693872825,
86.2117894720934));
#125363=CARTESIAN_POINT('Ctrl Pts',(-7.07825187942197,-21.3483262000986,
86.2229060358246));
#125364=CARTESIAN_POINT('Ctrl Pts',(-7.06214060964175,-21.3391720258857,
86.2336599246193));
#125365=CARTESIAN_POINT('Ctrl Pts',(-7.0298691387285,-21.3208358754224,
86.2552003627211));
#125366=CARTESIAN_POINT('Ctrl Pts',(-6.99781709896481,-21.3033565079906,
86.27528664282));
#125367=CARTESIAN_POINT('Ctrl Pts',(-6.96600003195233,-21.2866931565165,
86.2940024449842));
#125368=CARTESIAN_POINT('Ctrl Pts',(-6.94815056474316,-21.2773449678347,
86.3045020644775));
#125369=CARTESIAN_POINT('Ctrl Pts',(-6.93037501697478,-21.2682542386513,
86.3145713105324));
#125370=CARTESIAN_POINT('Ctrl Pts',(-6.9126858637405,-21.2594190155966,
86.3242147374989));
#125371=CARTESIAN_POINT('Ctrl Pts',(-6.88310196576389,-21.2446427098013,
86.340342709016));
#125372=CARTESIAN_POINT('Ctrl Pts',(-6.85375997369321,-21.230581377448,
86.3552799987662));
#125373=CARTESIAN_POINT('Ctrl Pts',(-6.8247237715537,-21.2172277935325,
86.3690639227611));
#125374=CARTESIAN_POINT('Ctrl Pts',(-6.80541826317748,-21.2083493002333,
86.3782285393615));
#125375=CARTESIAN_POINT('Ctrl Pts',(-6.78624741907278,-21.1997836333197,
86.3868840470772));
#125376=CARTESIAN_POINT('Ctrl Pts',(-6.76723753695952,-21.1915311822395,
86.3950378247371));
#125377=CARTESIAN_POINT('Ctrl Pts',(-6.74056004148214,-21.1799501148213,
86.4064804189285));
#125378=CARTESIAN_POINT('Ctrl Pts',(-6.71419947662327,-21.1689861593937,
86.4169351580929));
#125379=CARTESIAN_POINT('Ctrl Pts',(-6.68823034809353,-21.158635001424,
86.4264373456855));
#125380=CARTESIAN_POINT('Ctrl Pts',(-6.66785902462152,-21.150515099092,
86.4338912784163));
#125381=CARTESIAN_POINT('Ctrl Pts',(-6.64772783612135,-21.1427714979923,
86.4407584809481));
#125382=CARTESIAN_POINT('Ctrl Pts',(-6.62785299516616,-21.1353933240402,
86.4470647112304));
#125383=CARTESIAN_POINT('Ctrl Pts',(-6.6043375045663,-21.1266636249897,
86.454526109249));
#125384=CARTESIAN_POINT('Ctrl Pts',(-6.58118076088298,-21.1184454494094,
86.461202477795));
#125385=CARTESIAN_POINT('Ctrl Pts',(-6.55840481740494,-21.1107171824041,
86.4671409404535));
#125386=CARTESIAN_POINT('Ctrl Pts',(-6.53741878493808,-21.1035962628056,
86.4726127124693));
#125387=CARTESIAN_POINT('Ctrl Pts',(-6.51675554276146,-21.0968907643728,
86.4774570680671));
#125388=CARTESIAN_POINT('Ctrl Pts',(-6.49641502090829,-21.0905794474349,
86.4817141253824));
#125389=CARTESIAN_POINT('Ctrl Pts',(-6.47602248136917,-21.0842519902964,
86.4859820694523));
#125390=CARTESIAN_POINT('Ctrl Pts',(-6.45595416530781,-21.078320662806,
86.4896597311807));
#125391=CARTESIAN_POINT('Ctrl Pts',(-6.43620364679814,-21.0727627584111,
86.4927862263515));
#125392=CARTESIAN_POINT('Ctrl Pts',(-6.41485383265773,-21.0667548034412,
86.4961658890564));
#125393=CARTESIAN_POINT('Ctrl Pts',(-6.39387591799712,-21.0611827407742,
86.4989005495489));
#125394=CARTESIAN_POINT('Ctrl Pts',(-6.37322590319923,-21.0560128857335,
86.5010337758867));
#125395=CARTESIAN_POINT('Ctrl Pts',(-6.35571836562928,-21.051629768712,
86.5028423721815));
#125396=CARTESIAN_POINT('Ctrl Pts',(-6.33844642442226,-21.0475358633691,
86.5042184324612));
#125397=CARTESIAN_POINT('Ctrl Pts',(-6.32137803192766,-21.0437131274736,
86.5051841797176));
#125398=CARTESIAN_POINT('Ctrl Pts',(-6.29975624133946,-21.0388705862072,
86.5064075629357));
#125399=CARTESIAN_POINT('Ctrl Pts',(-6.27846158278878,-21.0344644269352,
86.5069734461553));
#125400=CARTESIAN_POINT('Ctrl Pts',(-6.25754083755047,-21.0304847535283,
86.5069156039064));
#125401=CARTESIAN_POINT('Ctrl Pts',(-6.24246729728511,-21.0276173715752,
86.5068739281699));
#125402=CARTESIAN_POINT('Ctrl Pts',(-6.22758792701389,-21.0249712982746,
86.5065084226784));
#125403=CARTESIAN_POINT('Ctrl Pts',(-6.2129177451068,-21.0225402179311,
86.5058302683033));
#125404=CARTESIAN_POINT('Origin',(-8.75366715310791,111.0724296188,85.97453149762));
#125405=CARTESIAN_POINT('',(-6.54682286637191,-10.,85.58540530765));
#125406=CARTESIAN_POINT('Origin',(-6.80729512863291,-10.,84.10819367738));
#125407=CARTESIAN_POINT('Origin',(-6.80729512863291,-10.,84.10819367738));
#125408=CARTESIAN_POINT('Origin',(-6.80729512863291,-10.,84.10819367738));
#125409=CARTESIAN_POINT('Origin',(-9.10739291134991,-8.5,88.57546942229));
#125410=CARTESIAN_POINT('',(-5.70733149011427,-8.50000000000053,58.9263899029757));
#125411=CARTESIAN_POINT('Origin',(27.4324635166691,-8.5,72.98888938658));
#125412=CARTESIAN_POINT('',(-2.22484390946918,-8.50000000000039,56.4938787766194));
#125413=CARTESIAN_POINT('Origin',(-2.02513312664091,-8.50000000000099,60.48888938658));
#125414=CARTESIAN_POINT('Origin',(1.07038457110909,-8.5,122.41156512159));
#125415=CARTESIAN_POINT('Origin',(1.07038457110909,-10.,122.41156512159));
#125416=CARTESIAN_POINT('',(-2.29973550275294,-10.,54.9957487971695));
#125417=CARTESIAN_POINT('Origin',(-2.22484394585091,-10.,56.49387804884));
#125418=CARTESIAN_POINT('Origin',(1.07038457110909,-10.,122.41156512159));
#125419=CARTESIAN_POINT('Origin',(18.4825952511691,-2.36409272922499,58.74984256216));
#125420=CARTESIAN_POINT('',(18.8781175927891,-10.0002140775,57.30292794298));
#125421=CARTESIAN_POINT('Ctrl Pts',(-3.58430183424491,-12.77734752092,56.71623037308));
#125422=CARTESIAN_POINT('Ctrl Pts',(-2.82654579637091,-13.56823877579,56.66356760301));
#125423=CARTESIAN_POINT('Ctrl Pts',(-1.22510960093091,-14.96301005098,56.57763219321));
#125424=CARTESIAN_POINT('Ctrl Pts',(1.36103340034909,-16.52464473566,56.54069563469));
#125425=CARTESIAN_POINT('Ctrl Pts',(3.87584585923909,-17.55452762874,56.60358098145));
#125426=CARTESIAN_POINT('Ctrl Pts',(6.19710063835909,-18.15797232338,56.74716429009));
#125427=CARTESIAN_POINT('Ctrl Pts',(8.31505282592909,-18.45204200109,56.94959224141));
#125428=CARTESIAN_POINT('Ctrl Pts',(10.3190076082391,-18.5227178858,57.20308600798));
#125429=CARTESIAN_POINT('Ctrl Pts',(12.2966611152891,-18.39728886114,57.51358361024));
#125430=CARTESIAN_POINT('Ctrl Pts',(14.2762842352891,-18.07077538528,57.88694259276));
#125431=CARTESIAN_POINT('Ctrl Pts',(16.1913087147191,-17.5550687573,58.30881641828));
#125432=CARTESIAN_POINT('Ctrl Pts',(18.0106355730791,-16.87094604643,58.76532096745));
#125433=CARTESIAN_POINT('Ctrl Pts',(19.7936798013391,-16.00018983021,59.26535024511));
#125434=CARTESIAN_POINT('Ctrl Pts',(21.6152587953191,-14.87219739396,59.8316118168));
#125435=CARTESIAN_POINT('Ctrl Pts',(23.5037332083091,-13.38226243744,60.48072054854));
#125436=CARTESIAN_POINT('Ctrl Pts',(25.4089773760291,-11.42609024385,61.20195839564));
#125437=CARTESIAN_POINT('Ctrl Pts',(27.1843832993891,-8.93696435445999,
61.93748494782));
#125438=CARTESIAN_POINT('Ctrl Pts',(28.5837262234791,-5.98779183204199,
62.56306222481));
#125439=CARTESIAN_POINT('Ctrl Pts',(29.4131721215591,-2.80038937228799,
62.95281639517));
#125440=CARTESIAN_POINT('Ctrl Pts',(29.5612752799991,-0.620166171525686,
63.023935917286));
#125441=CARTESIAN_POINT('Ctrl Pts',(29.5343220504091,0.444915684091514,
63.011087634094));
#125442=CARTESIAN_POINT('Ctrl Pts',(29.5338703742191,0.461774656562614,
63.0108722771));
#125443=CARTESIAN_POINT('Ctrl Pts',(-3.72288960953291,-12.85329830414,55.62299833527));
#125444=CARTESIAN_POINT('Ctrl Pts',(-2.94901860386991,-13.64890746123,55.56862071173));
#125445=CARTESIAN_POINT('Ctrl Pts',(-1.31349980804092,-15.05199668853,55.47970165767));
#125446=CARTESIAN_POINT('Ctrl Pts',(1.32767713553909,-16.6228801163,55.44051598947));
#125447=CARTESIAN_POINT('Ctrl Pts',(3.89588111527909,-17.65877088157,55.5036943663299));
#125448=CARTESIAN_POINT('Ctrl Pts',(6.26621663463909,-18.26566107639,55.64967374489));
#125449=CARTESIAN_POINT('Ctrl Pts',(8.42872386496909,-18.56136755362,55.8560400985301));
#125450=CARTESIAN_POINT('Ctrl Pts',(10.4746065168291,-18.63242271852,56.11476044379));
#125451=CARTESIAN_POINT('Ctrl Pts',(12.4933994745791,-18.50631935278,56.431858726));
#125452=CARTESIAN_POINT('Ctrl Pts',(14.5139561217791,-18.17810478474,56.81330363737));
#125453=CARTESIAN_POINT('Ctrl Pts',(16.4683569012591,-17.65977495691,57.24442226139));
#125454=CARTESIAN_POINT('Ctrl Pts',(18.3249224039791,-16.97222998037,57.71101147142));
#125455=CARTESIAN_POINT('Ctrl Pts',(20.1443477633591,-16.09715278017,58.22215868751));
#125456=CARTESIAN_POINT('Ctrl Pts',(22.0030374225591,-14.96355146807,58.80109378072));
#125457=CARTESIAN_POINT('Ctrl Pts',(23.9300250610891,-13.46607983077,59.4648497644901));
#125458=CARTESIAN_POINT('Ctrl Pts',(25.8743271231091,-11.49961504094,60.20254853862));
#125459=CARTESIAN_POINT('Ctrl Pts',(27.6865453689491,-8.99647741870398,
60.9551385269801));
#125460=CARTESIAN_POINT('Ctrl Pts',(29.1154374711391,-6.02908615362698,
61.59554524518));
#125461=CARTESIAN_POINT('Ctrl Pts',(29.9627342908991,-2.82017517727099,
61.99473019848));
#125462=CARTESIAN_POINT('Ctrl Pts',(30.1140601046791,-0.624535642130786,
62.06759020103));
#125463=CARTESIAN_POINT('Ctrl Pts',(30.0865221951591,0.448052485067714,
62.05442854821));
#125464=CARTESIAN_POINT('Ctrl Pts',(30.0860607192791,0.465030265795814,
62.05420793871));
#125465=CARTESIAN_POINT('Ctrl Pts',(-3.17320105054691,-12.28484166745,54.85174559045));
#125466=CARTESIAN_POINT('Ctrl Pts',(-2.42508695642091,-13.04513949903,54.80503919576));
#125467=CARTESIAN_POINT('Ctrl Pts',(-0.844253174050915,-14.3859726853,54.73047035947));
#125468=CARTESIAN_POINT('Ctrl Pts',(1.70866986857909,-15.8876335301,54.70700946437));
#125469=CARTESIAN_POINT('Ctrl Pts',(4.19228482572909,-16.87855813869,54.77837472681));
#125470=CARTESIAN_POINT('Ctrl Pts',(6.48653288913908,-17.45966035134,54.92597342556));
#125471=CARTESIAN_POINT('Ctrl Pts',(8.58186134395909,-17.74311613794,55.12908301981));
#125472=CARTESIAN_POINT('Ctrl Pts',(10.5664452653491,-17.81133256526,55.38081209437));
#125473=CARTESIAN_POINT('Ctrl Pts',(12.5270981927391,-17.69027633198,55.68738173201));
#125474=CARTESIAN_POINT('Ctrl Pts',(14.4918977503591,-17.37479365556,56.05469422228));
#125475=CARTESIAN_POINT('Ctrl Pts',(16.3945506037791,-16.87609727056,56.4687746378201));
#125476=CARTESIAN_POINT('Ctrl Pts',(18.2036342066391,-16.21416637664,56.91612646381));
#125477=CARTESIAN_POINT('Ctrl Pts',(19.9776601847591,-15.37142975168,57.40549259896));
#125478=CARTESIAN_POINT('Ctrl Pts',(21.7905301121891,-14.27980829232,57.95894164));
#125479=CARTESIAN_POINT('Ctrl Pts',(23.6696227303091,-12.83874523999,58.59230118133));
#125480=CARTESIAN_POINT('Ctrl Pts',(25.5636008457491,-10.94931579331,59.29438635056));
#125481=CARTESIAN_POINT('Ctrl Pts',(27.3248106085391,-8.55104953890899,
60.00792469414));
#125482=CARTESIAN_POINT('Ctrl Pts',(28.7082158942091,-5.72001717281198,
60.61198629947));
#125483=CARTESIAN_POINT('Ctrl Pts',(29.5252295808991,-2.67208753843899,
60.98663314509));
#125484=CARTESIAN_POINT('Ctrl Pts',(29.6707996220691,-0.591832166815786,
61.0548216514));
#125485=CARTESIAN_POINT('Ctrl Pts',(29.6442913120391,0.424574974273814,
61.04249344665));
#125486=CARTESIAN_POINT('Ctrl Pts',(29.6438471072391,0.440663529910414,
61.04228680651));
#125487=CARTESIAN_POINT('Ctrl Pts',(-2.38244347352091,-11.53445397631,55.02993629904));
#125488=CARTESIAN_POINT('Ctrl Pts',(-1.68100325115091,-12.24813930956,54.99404617299));
#125489=CARTESIAN_POINT('Ctrl Pts',(-0.199132288740913,-13.50679179131,
54.93948658306));
#125490=CARTESIAN_POINT('Ctrl Pts',(2.19404928560909,-14.91707579071,54.93693122039));
#125491=CARTESIAN_POINT('Ctrl Pts',(4.52391333623909,-15.8486431004,55.0177166612));
#125492=CARTESIAN_POINT('Ctrl Pts',(6.67880783080909,-16.3957040456,55.16484050833));
#125493=CARTESIAN_POINT('Ctrl Pts',(8.6498779854791,-16.6629883833,55.36014776661));
#125494=CARTESIAN_POINT('Ctrl Pts',(10.5198070717491,-16.72745755252,55.5983555735));
#125495=CARTESIAN_POINT('Ctrl Pts',(12.3703411755791,-16.61306375545,55.88583297768));
#125496=CARTESIAN_POINT('Ctrl Pts',(14.2280550377091,-16.31438773435,56.22829233863));
#125497=CARTESIAN_POINT('Ctrl Pts',(16.0299360351191,-15.84160835493,56.61291322706));
#125498=CARTESIAN_POINT('Ctrl Pts',(17.7454468009191,-15.21348917344,57.02735648449));
#125499=CARTESIAN_POINT('Ctrl Pts',(19.4292282283691,-14.41344352614,57.47976284219));
#125500=CARTESIAN_POINT('Ctrl Pts',(21.1506253523991,-13.37723731351,57.99030081481));
#125501=CARTESIAN_POINT('Ctrl Pts',(22.9343804115591,-12.01063606723,58.57294969782));
#125502=CARTESIAN_POINT('Ctrl Pts',(24.7295945359991,-10.22289665205,59.2163207090301));
#125503=CARTESIAN_POINT('Ctrl Pts',(26.3934737214891,-7.96306520251299,
59.86646337428));
#125504=CARTESIAN_POINT('Ctrl Pts',(27.6933626732391,-5.31203256334299,
60.41257442068));
#125505=CARTESIAN_POINT('Ctrl Pts',(28.4565964661691,-2.47660536052199,
60.74867761106));
#125506=CARTESIAN_POINT('Ctrl Pts',(28.5921150013391,-0.548662145128386,
60.80958320983));
#125507=CARTESIAN_POINT('Ctrl Pts',(28.5674129242191,0.393583630375914,
60.79855720673));
#125508=CARTESIAN_POINT('Ctrl Pts',(28.5669990101191,0.408498369893214,
60.79837239285));
#125509=CARTESIAN_POINT('',(-2.29980340878172,-12.0404106862218,54.9957613512899));
#125510=CARTESIAN_POINT('Ctrl Pts',(-2.29980340878172,-12.0404106862218,
54.9957613512899));
#125511=CARTESIAN_POINT('Ctrl Pts',(-2.11823697781814,-12.2161790760666,
54.9866899612617));
#125512=CARTESIAN_POINT('Ctrl Pts',(-1.93310846652742,-12.3876152127252,
54.9781755580477));
#125513=CARTESIAN_POINT('Ctrl Pts',(-1.74444833532541,-12.5547517442881,
54.9703033857551));
#125514=CARTESIAN_POINT('Ctrl Pts',(-1.55486486079395,-12.7227062780466,
54.9623926853552));
#125515=CARTESIAN_POINT('Ctrl Pts',(-1.36171473698319,-12.8863192680378,
54.9551303640825));
#125516=CARTESIAN_POINT('Ctrl Pts',(-1.16499499631772,-13.0455840037535,
54.9486081660288));
#125517=CARTESIAN_POINT('Ctrl Pts',(-1.03792296467273,-13.1484618007063,
54.944395121854));
#125518=CARTESIAN_POINT('Ctrl Pts',(-0.909360813004725,-13.2495244394935,
54.9404910116767));
#125519=CARTESIAN_POINT('Ctrl Pts',(-0.779301391391256,-13.3487605877945,
54.9369221775477));
#125520=CARTESIAN_POINT('Ctrl Pts',(-0.611246867493417,-13.476987235655,
54.9323107567604));
#125521=CARTESIAN_POINT('Ctrl Pts',(-0.440702356432936,-13.6021849644138,
54.9282592889589));
#125522=CARTESIAN_POINT('Ctrl Pts',(-0.267676715340883,-13.7243431957544,
54.924828715228));
#125523=CARTESIAN_POINT('Ctrl Pts',(-0.166953501828351,-13.7954550236891,
54.9228316793657));
#125524=CARTESIAN_POINT('Ctrl Pts',(-0.0653892044135112,-13.8655365188882,
54.921045112895));
#125525=CARTESIAN_POINT('Ctrl Pts',(0.0370171584764496,-13.9345929491547,
54.9194792680636));
#125526=CARTESIAN_POINT('Ctrl Pts',(0.176178845081396,-14.0284348651803,
54.917351415833));
#125527=CARTESIAN_POINT('Ctrl Pts',(0.316893525903645,-14.1203783761309,
54.9156311299842));
#125528=CARTESIAN_POINT('Ctrl Pts',(0.459158674092703,-14.2104234819286,
54.9143456426954));
#125529=CARTESIAN_POINT('Ctrl Pts',(0.530291248187232,-14.2554460348274,
54.913702899051));
#125530=CARTESIAN_POINT('Ctrl Pts',(0.601811440288151,-14.2999939864225,
54.9131688810108));
#125531=CARTESIAN_POINT('Ctrl Pts',(0.673718918977216,-14.3440673366463,
54.9127471525551));
#125532=CARTESIAN_POINT('Ctrl Pts',(0.709672658321749,-14.3661040117582,
54.9125362883272));
#125533=CARTESIAN_POINT('Ctrl Pts',(0.745723219351884,-14.388022036527,
54.9123534981929));
#125534=CARTESIAN_POINT('Ctrl Pts',(0.781870558597959,-14.4098214109445,
54.912199237989));
#125535=CARTESIAN_POINT('Ctrl Pts',(0.808981063032514,-14.4261709417575,
54.9120835428361));
#125536=CARTESIAN_POINT('Ctrl Pts',(0.836146005216066,-14.4424537317479,
54.9119838959101));
#125537=CARTESIAN_POINT('Ctrl Pts',(0.86336536634066,-14.4586697809128,
54.9119004921109));
#125538=CARTESIAN_POINT('Ctrl Pts',(0.872438486715524,-14.4640751306344,
54.9118726908444));
#125539=CARTESIAN_POINT('Ctrl Pts',(0.882845358372333,-14.4702608301792,
54.9118431601062));
#125540=CARTESIAN_POINT('Ctrl Pts',(0.890602866371274,-14.4748635831357,
54.9118225100166));
#125541=CARTESIAN_POINT('Ctrl Pts',(1.12238678087696,-14.6123876563195,
54.9112055130879));
#125542=CARTESIAN_POINT('Ctrl Pts',(1.35703325424795,-14.7444222465215,
54.9117700146229));
#125543=CARTESIAN_POINT('Ctrl Pts',(1.59451843150642,-14.8709914875867,
54.9136088011056));
#125544=CARTESIAN_POINT('Ctrl Pts',(1.78986036435338,-14.9751002175464,
54.9151212833151));
#125545=CARTESIAN_POINT('Ctrl Pts',(1.98712346942663,-15.0755104066668,
54.9174960503598));
#125546=CARTESIAN_POINT('Ctrl Pts',(2.18630472440888,-15.1722117185856,
54.9207900375331));
#125547=CARTESIAN_POINT('Ctrl Pts',(2.26366130372528,-15.2097678766996,
54.9220693325153));
#125548=CARTESIAN_POINT('Ctrl Pts',(2.34130728992583,-15.2467643796092,
54.9234873317818));
#125549=CARTESIAN_POINT('Ctrl Pts',(2.4192417879567,-15.2832011533707,54.925046539226));
#125550=CARTESIAN_POINT('Ctrl Pts',(2.66203537948802,-15.3967146215894,
54.9299040232015));
#125551=CARTESIAN_POINT('Ctrl Pts',(2.90762907197283,-15.504802566863,54.9361310672224));
#125552=CARTESIAN_POINT('Ctrl Pts',(3.15600542837689,-15.6074668205158,
54.9438115552215));
#125553=CARTESIAN_POINT('Ctrl Pts',(3.17491982026466,-15.6152849234729,
54.9443964408443));
#125554=CARTESIAN_POINT('Ctrl Pts',(3.1938503567678,-15.6230715505705,54.9449897614188));
#125555=CARTESIAN_POINT('Ctrl Pts',(3.21279703372886,-15.6308266911595,
54.9455915571066));
#125556=CARTESIAN_POINT('Ctrl Pts',(3.34667052785487,-15.6856229897515,
54.949843727112));
#125557=CARTESIAN_POINT('Ctrl Pts',(3.48134941726851,-15.7388486429223,
54.9545189197661));
#125558=CARTESIAN_POINT('Ctrl Pts',(3.61683074223619,-15.7905036503555,
54.9596318684309));
#125559=CARTESIAN_POINT('Ctrl Pts',(3.68457140472003,-15.816331154072,54.9621883427633));
#125560=CARTESIAN_POINT('Ctrl Pts',(3.75251267553316,-15.8417659963483,
54.9648542730921));
#125561=CARTESIAN_POINT('Ctrl Pts',(3.82065417045425,-15.8668081771434,
54.9676316045845));
#125562=CARTESIAN_POINT('Ctrl Pts',(3.85472491791479,-15.879329267541,54.9690202703307));
#125563=CARTESIAN_POINT('Ctrl Pts',(3.88884572134119,-15.8917521925685,
54.9704367874654));
#125564=CARTESIAN_POINT('Ctrl Pts',(3.92301653121896,-15.9040769522236,
54.9718814057418));
#125565=CARTESIAN_POINT('Ctrl Pts',(3.94864463862729,-15.9133205219649,
54.9729648694492));
#125566=CARTESIAN_POINT('Ctrl Pts',(3.97430087465893,-15.9225088736842,
54.9740641401396));
#125567=CARTESIAN_POINT('Ctrl Pts',(3.99998521807188,-15.9316420073814,
54.9751793248278));
#125568=CARTESIAN_POINT('Ctrl Pts',(4.0085466658762,-15.9346863852804,54.9755510530572));
#125569=CARTESIAN_POINT('Ctrl Pts',(4.01841638730849,-15.9381865207366,
54.9759817156855));
#125570=CARTESIAN_POINT('Ctrl Pts',(4.02567892979854,-15.9407567350712,
54.9762998182153));
#125571=CARTESIAN_POINT('Ctrl Pts',(4.19513949895062,-16.0007288432664,
54.9837222650809));
#125572=CARTESIAN_POINT('Ctrl Pts',(4.36540762168142,-16.0581700333998,
54.9918196982076));
#125573=CARTESIAN_POINT('Ctrl Pts',(4.53647535322449,-16.1130769852884,
55.0006148639831));
#125574=CARTESIAN_POINT('Ctrl Pts',(4.79577701300262,-16.1963040417861,
55.0139464319126));
#125575=CARTESIAN_POINT('Ctrl Pts',(5.05691578284093,-16.2737107959004,
55.0288804604544));
#125576=CARTESIAN_POINT('Ctrl Pts',(5.31987357742345,-16.3453019227047,
55.0454711014457));
#125577=CARTESIAN_POINT('Ctrl Pts',(5.35926275247959,-16.3560257555184,
55.0479562594283));
#125578=CARTESIAN_POINT('Ctrl Pts',(5.39869274909326,-16.3666190063023,
55.0504786131046));
#125579=CARTESIAN_POINT('Ctrl Pts',(5.43816351149184,-16.3770815939634,
55.053038370818));
#125580=CARTESIAN_POINT('Ctrl Pts',(5.67656967670919,-16.4402763551221,
55.0684994864194));
#125581=CARTESIAN_POINT('Ctrl Pts',(5.91646148577811,-16.4987080922576,
55.0853243446279));
#125582=CARTESIAN_POINT('Ctrl Pts',(6.15782167811788,-16.5523768050417,
55.1035638143412));
#125583=CARTESIAN_POINT('Ctrl Pts',(6.27850177428777,-16.5792111614337,
55.1126835491979));
#125584=CARTESIAN_POINT('Ctrl Pts',(6.3995489559653,-16.6048547617057,55.1221570798402));
#125585=CARTESIAN_POINT('Ctrl Pts',(6.52096086026782,-16.6293076058599,
55.1319916333416));
#125586=CARTESIAN_POINT('Ctrl Pts',(6.58166681241908,-16.641534027937,55.1369089100924));
#125587=CARTESIAN_POINT('Ctrl Pts',(6.64246394417776,-16.6534627609877,
55.141916451863));
#125588=CARTESIAN_POINT('Ctrl Pts',(6.70335194954774,-16.6650938050292,
55.1470152184466));
#125589=CARTESIAN_POINT('Ctrl Pts',(6.70722592634993,-16.6658338259007,
55.147339625583));
#125590=CARTESIAN_POINT('Ctrl Pts',(6.71110027104119,-16.6665726417745,
55.1476644020211));
#125591=CARTESIAN_POINT('Ctrl Pts',(6.71497498351283,-16.6673102525422,
55.1479895480109));
#125592=CARTESIAN_POINT('Ctrl Pts',(6.76438739306036,-16.6767166602704,
55.1521359838887));
#125593=CARTESIAN_POINT('Ctrl Pts',(6.81385961344467,-16.6859270892099,
55.1563425176269));
#125594=CARTESIAN_POINT('Ctrl Pts',(6.86339149624892,-16.6949415412016,
55.1606094699931));
#125595=CARTESIAN_POINT('Ctrl Pts',(6.87102234822951,-16.6963303022367,
55.1612668341002));
#125596=CARTESIAN_POINT('Ctrl Pts',(6.87987773679538,-16.6979354380448,
55.1620314192965));
#125597=CARTESIAN_POINT('Ctrl Pts',(6.88628829968681,-16.6990938701348,
55.162585865581));
#125598=CARTESIAN_POINT('Ctrl Pts',(7.09142631221265,-16.736163697014,55.1803281466857));
#125599=CARTESIAN_POINT('Ctrl Pts',(7.29906866836621,-16.7699660342097,
55.1992345884685));
#125600=CARTESIAN_POINT('Ctrl Pts',(7.50920025566267,-16.8005008816512,
55.2193722461986));
#125601=CARTESIAN_POINT('Ctrl Pts',(7.6142660493109,-16.8157683053719,55.2294410750636));
#125602=CARTESIAN_POINT('Ctrl Pts',(7.71995414520202,-16.8302188565267,
55.2398177960984));
#125603=CARTESIAN_POINT('Ctrl Pts',(7.82626245270495,-16.8438525347216,
55.2505113355578));
#125604=CARTESIAN_POINT('Ctrl Pts',(7.88848917012429,-16.8518328991949,
55.256770713341));
#125605=CARTESIAN_POINT('Ctrl Pts',(7.9516382434093,-16.8596206660257,55.2632112213451));
#125606=CARTESIAN_POINT('Ctrl Pts',(8.01446306451706,-16.8670588826418,
55.2697083472482));
#125607=CARTESIAN_POINT('Ctrl Pts',(8.05896835301694,-16.8723281372229,
55.2743109303935));
#125608=CARTESIAN_POINT('Ctrl Pts',(8.10331079659642,-16.8774230378983,
55.2789416187177));
#125609=CARTESIAN_POINT('Ctrl Pts',(8.14704586474734,-16.8823029504198,
55.2835517443369));
#125610=CARTESIAN_POINT('Ctrl Pts',(8.3264698772246,-16.9023228914453,55.3024648790727));
#125611=CARTESIAN_POINT('Ctrl Pts',(8.50485641498181,-16.9197600629979,
55.3219956359713));
#125612=CARTESIAN_POINT('Ctrl Pts',(8.68198013956874,-16.9345906189262,
55.3420966134434));
#125613=CARTESIAN_POINT('Ctrl Pts',(8.92133811413511,-16.954632043851,55.3692602769545));
#125614=CARTESIAN_POINT('Ctrl Pts',(9.15839074252427,-16.9699118174646,
55.3974658526435));
#125615=CARTESIAN_POINT('Ctrl Pts',(9.39257368191784,-16.9804287123046,
55.426561672554));
#125616=CARTESIAN_POINT('Ctrl Pts',(9.5963122636134,-16.9895783849669,55.4518749643642));
#125617=CARTESIAN_POINT('Ctrl Pts',(9.79845889006155,-16.9955813380872,
55.4779328650654));
#125618=CARTESIAN_POINT('Ctrl Pts',(9.99901038774821,-16.9984375726291,
55.5046948396689));
#125619=CARTESIAN_POINT('Ctrl Pts',(10.0992861365915,-16.9998656899,55.5180758269706));
#125620=CARTESIAN_POINT('Ctrl Pts',(10.1991630943723,-17.0005071275631,
55.5316328999386));
#125621=CARTESIAN_POINT('Ctrl Pts',(10.2986408939489,-17.0003618855091,
55.5453613709104));
#125622=CARTESIAN_POINT('Ctrl Pts',(10.3622868047177,-17.0002689596217,
55.5541448486529));
#125623=CARTESIAN_POINT('Ctrl Pts',(10.4251100046831,-16.9998594984302,
55.5629062774401));
#125624=CARTESIAN_POINT('Ctrl Pts',(10.4883760042335,-16.9991254956933,
55.5718207460435));
#125625=CARTESIAN_POINT('Ctrl Pts',(10.4931746518341,-16.9990698224961,
55.572496897431));
#125626=CARTESIAN_POINT('Ctrl Pts',(10.4979758457689,-16.9990122583866,
55.5731739361208));
#125627=CARTESIAN_POINT('Ctrl Pts',(10.5027801376696,-16.9989527881453,
55.5738519418908));
#125628=CARTESIAN_POINT('Ctrl Pts',(10.5336357439578,-16.9985708400058,
55.5782064398132));
#125629=CARTESIAN_POINT('Ctrl Pts',(10.5646191521784,-16.9981104984623,
55.5826007620461));
#125630=CARTESIAN_POINT('Ctrl Pts',(10.5958764208502,-16.9975661198121,
55.5870564767843));
#125631=CARTESIAN_POINT('Ctrl Pts',(10.7964545168402,-16.994072838479,55.6156488271859));
#125632=CARTESIAN_POINT('Ctrl Pts',(10.9986788730587,-16.9872735133215,
55.6453989040006));
#125633=CARTESIAN_POINT('Ctrl Pts',(11.2025344927777,-16.9771681456159,
55.6763506604447));
#125634=CARTESIAN_POINT('Ctrl Pts',(11.3110439159274,-16.9717892032941,
55.6928258365612));
#125635=CARTESIAN_POINT('Ctrl Pts',(11.4195641712537,-16.96549941776,55.7095718230664));
#125636=CARTESIAN_POINT('Ctrl Pts',(11.5288140096561,-16.9582626105621,
55.7267056358984));
#125637=CARTESIAN_POINT('Ctrl Pts',(11.6248108020557,-16.9519036970079,
55.7417609540344));
#125638=CARTESIAN_POINT('Ctrl Pts',(11.7213709309547,-16.9448129094927,
55.7571159141607));
#125639=CARTESIAN_POINT('Ctrl Pts',(11.8189787193469,-16.9369339119195,
55.7728589214683));
#125640=CARTESIAN_POINT('Ctrl Pts',(12.0087112421133,-16.9216185143365,
55.8034605828888));
#125641=CARTESIAN_POINT('Ctrl Pts',(12.1981250333715,-16.903544034879,55.8348412411284));
#125642=CARTESIAN_POINT('Ctrl Pts',(12.3872110443822,-16.8827131212053,
55.8669978109124));
#125643=CARTESIAN_POINT('Ctrl Pts',(12.6140848726673,-16.8577192620268,
55.9055806973587));
#125644=CARTESIAN_POINT('Ctrl Pts',(12.8404870703923,-16.8287575946014,
55.945280530211));
#125645=CARTESIAN_POINT('Ctrl Pts',(13.0664108967834,-16.7958240268103,
55.9860824040969));
#125646=CARTESIAN_POINT('Ctrl Pts',(13.273519930093,-16.7656331456729,56.023486323784));
#125647=CARTESIAN_POINT('Ctrl Pts',(13.480225796256,-16.7321059811549,56.0618162294752));
#125648=CARTESIAN_POINT('Ctrl Pts',(13.6865207180361,-16.695242533248,56.1010641528426));
#125649=CARTESIAN_POINT('Ctrl Pts',(13.7896681789261,-16.6768108092946,
56.1206881145263));
#125650=CARTESIAN_POINT('Ctrl Pts',(13.8927128932393,-16.657545014482,56.1405416383219));
#125651=CARTESIAN_POINT('Ctrl Pts',(13.9956538238716,-16.6374451487844,
56.160624077633));
#125652=CARTESIAN_POINT('Ctrl Pts',(14.0471242891877,-16.6273952159356,
56.1706652972885));
#125653=CARTESIAN_POINT('Ctrl Pts',(14.0985688077801,-16.6171367653659,
56.180763749469));
#125654=CARTESIAN_POINT('Ctrl Pts',(14.1499872456801,-16.6066697970753,
56.1909193754892));
#125655=CARTESIAN_POINT('Ctrl Pts',(14.188520764919,-16.5988257407315,56.1985301086545));
#125656=CARTESIAN_POINT('Ctrl Pts',(14.2279621434588,-16.5906724585696,
56.2063564186179));
#125657=CARTESIAN_POINT('Ctrl Pts',(14.2662370443747,-16.5826408526218,
56.2139860715531));
#125658=CARTESIAN_POINT('Ctrl Pts',(14.2750639199052,-16.5807886208899,
56.2157456057436));
#125659=CARTESIAN_POINT('Ctrl Pts',(14.2838288110896,-16.5789430676027,
56.2174946280228));
#125660=CARTESIAN_POINT('Ctrl Pts',(14.2925063727919,-16.5771098442795,
56.2192279890994));
#125661=CARTESIAN_POINT('Ctrl Pts',(14.2964107562995,-16.5762850034827,
56.2200078978609));
#125662=CARTESIAN_POINT('Ctrl Pts',(14.3002974607726,-16.5754626606167,
56.2207846356224));
#125663=CARTESIAN_POINT('Ctrl Pts',(14.3041641799629,-16.5746433390449,
56.2215577311178));
#125664=CARTESIAN_POINT('Ctrl Pts',(14.5915131589416,-16.5137567823796,
56.2790090717243));
#125665=CARTESIAN_POINT('Ctrl Pts',(14.8766803030032,-16.4466339001003,
56.3379743812551));
#125666=CARTESIAN_POINT('Ctrl Pts',(15.1596819051769,-16.3733807048929,
56.398376378207));
#125667=CARTESIAN_POINT('Ctrl Pts',(15.4451387650363,-16.2994919815855,
56.4593024091789));
#125668=CARTESIAN_POINT('Ctrl Pts',(15.7283927043861,-16.2193660075623,
56.5216903084838));
#125669=CARTESIAN_POINT('Ctrl Pts',(16.0094473939293,-16.1330620148757,
56.585473450932));
#125670=CARTESIAN_POINT('Ctrl Pts',(16.051085209621,-16.1202762124157,56.594922824411));
#125671=CARTESIAN_POINT('Ctrl Pts',(16.0926747273626,-16.1073547287579,
56.6044028408523));
#125672=CARTESIAN_POINT('Ctrl Pts',(16.1342159274268,-16.0942976671956,
56.6139133040204));
#125673=CARTESIAN_POINT('Ctrl Pts',(16.425505046536,-16.0027408524006,56.6806011809788));
#125674=CARTESIAN_POINT('Ctrl Pts',(16.7144204396943,-15.9045221819093,
56.7487852650238));
#125675=CARTESIAN_POINT('Ctrl Pts',(17.0009678150187,-15.7996448168294,
56.8183790298192));
#125676=CARTESIAN_POINT('Ctrl Pts',(17.2875151903431,-15.6947674517495,
56.8879727946147));
#125677=CARTESIAN_POINT('Ctrl Pts',(17.5716949479418,-15.5832312167085,
56.9589764659462));
#125678=CARTESIAN_POINT('Ctrl Pts',(17.853484767978,-15.4649874495282,57.0313116212954));
#125679=CARTESIAN_POINT('Ctrl Pts',(18.1244197179,-15.3512985691583,57.1008603427135));
#125680=CARTESIAN_POINT('Ctrl Pts',(18.3931454302537,-15.2314085628236,
57.171640227598));
#125681=CARTESIAN_POINT('Ctrl Pts',(18.6596279924013,-15.105223090577,57.2435655992374));
#125682=CARTESIAN_POINT('Ctrl Pts',(18.7326997853566,-15.0706219571007,
57.2632881500201));
#125683=CARTESIAN_POINT('Ctrl Pts',(18.8056027326372,-15.0355472259604,
57.2830968401248));
#125684=CARTESIAN_POINT('Ctrl Pts',(18.8783357065489,-14.9999964140997,
57.3029899158076));
#125685=CARTESIAN_POINT('',(4.86118769045346,-16.9627432173458,55.1997076232029));
#125686=CARTESIAN_POINT('Ctrl Pts',(-2.29980340878007,-12.0404106862236,
54.9957613512899));
#125687=CARTESIAN_POINT('Ctrl Pts',(-2.06567740026702,-12.2943912214082,
54.9840649350874));
#125688=CARTESIAN_POINT('Ctrl Pts',(-1.82554507595862,-12.5407219961361,
54.9736741258264));
#125689=CARTESIAN_POINT('Ctrl Pts',(-1.58014432233485,-12.7792889509596,
54.9649000176596));
#125690=CARTESIAN_POINT('Ctrl Pts',(-1.34235247712726,-13.0104588864848,
54.9563979599428));
#125691=CARTESIAN_POINT('Ctrl Pts',(-1.09961332086077,-13.2343393853548,
54.9494138090859));
#125692=CARTESIAN_POINT('Ctrl Pts',(-0.852552136993808,-13.4508341796129,
54.944230727073));
#125693=CARTESIAN_POINT('Ctrl Pts',(-0.692492947152338,-13.5910908594825,
54.9408728547643));
#125694=CARTESIAN_POINT('Ctrl Pts',(-0.530618838552155,-13.7282478118966,
54.9382709254756));
#125695=CARTESIAN_POINT('Ctrl Pts',(-0.367090522438706,-13.8622794667611,
54.9365021757409));
#125696=CARTESIAN_POINT('Ctrl Pts',(-0.274164418016843,-13.9384438880172,
54.9354970713868));
#125697=CARTESIAN_POINT('Ctrl Pts',(-0.180704010652601,-14.0135991241281,
54.934761014906));
#125698=CARTESIAN_POINT('Ctrl Pts',(-0.0867375050534825,-14.0877495088467,
54.9343060611869));
#125699=CARTESIAN_POINT('Ctrl Pts',(0.0429253377670358,-14.1900684108592,
54.9336782779977));
#125700=CARTESIAN_POINT('Ctrl Pts',(0.173551750225582,-14.2904740468692,
54.9335857285551));
#125701=CARTESIAN_POINT('Ctrl Pts',(0.305069580466433,-14.3889768459098,
54.9340602809736));
#125702=CARTESIAN_POINT('Ctrl Pts',(0.370828495586858,-14.4382282454301,
54.9342975571829));
#125703=CARTESIAN_POINT('Ctrl Pts',(0.436810266016493,-14.4870039344858,
54.9346766178456));
#125704=CARTESIAN_POINT('Ctrl Pts',(0.503006110322588,-14.535305081866,
54.9352014595083));
#125705=CARTESIAN_POINT('Ctrl Pts',(0.536104032475637,-14.5594556555561,
54.9354638803397));
#125706=CARTESIAN_POINT('Ctrl Pts',(0.569255473146564,-14.5834875937639,
54.9357627469423));
#125707=CARTESIAN_POINT('Ctrl Pts',(0.602459340381778,-14.6074010376774,
54.9360985608908));
#125708=CARTESIAN_POINT('Ctrl Pts',(0.619061273999385,-14.6193577596341,
54.9362664678651));
#125709=CARTESIAN_POINT('Ctrl Pts',(0.635676314261408,-14.6312848580121,
54.9364436117096));
#125710=CARTESIAN_POINT('Ctrl Pts',(0.652304325438487,-14.6431823499626,
54.9366300551795));
#125711=CARTESIAN_POINT('Ctrl Pts',(0.664775333821296,-14.6521054689255,
54.9367698877819));
#125712=CARTESIAN_POINT('Ctrl Pts',(0.677253638344097,-14.6610119342725,
54.9369149514262));
#125713=CARTESIAN_POINT('Ctrl Pts',(0.689739181907747,-14.6699017531266,
54.9370652726049));
#125714=CARTESIAN_POINT('Ctrl Pts',(0.693901029762297,-14.6728650260779,
54.9371153796645));
#125715=CARTESIAN_POINT('Ctrl Pts',(0.696714681788608,-14.6748675183456,
54.9371494568424));
#125716=CARTESIAN_POINT('Ctrl Pts',(0.702227136384261,-14.6787860234036,
54.9372173472754));
#125717=CARTESIAN_POINT('Ctrl Pts',(0.935316961053932,-14.8444769404133,
54.9400880410572));
#125718=CARTESIAN_POINT('Ctrl Pts',(1.16882069079971,-15.0029006935076,
54.9447710833822));
#125719=CARTESIAN_POINT('Ctrl Pts',(1.40215622931578,-15.1543843049336,
54.9513409451183));
#125720=CARTESIAN_POINT('Ctrl Pts',(1.60396128131111,-15.2853980299524,
54.9570230255149));
#125721=CARTESIAN_POINT('Ctrl Pts',(1.80564149725469,-15.4112205074094,
54.9641162477073));
#125722=CARTESIAN_POINT('Ctrl Pts',(2.00685028315897,-15.5320598165629,
54.9726602222318));
#125723=CARTESIAN_POINT('Ctrl Pts',(2.24133468443142,-15.6728833543111,
54.982617186794));
#125724=CARTESIAN_POINT('Ctrl Pts',(2.47517761250087,-15.8069400864488,
54.9945443759754));
#125725=CARTESIAN_POINT('Ctrl Pts',(2.70784486479394,-15.9345930464969,
55.0084597313433));
#125726=CARTESIAN_POINT('Ctrl Pts',(2.94360679681554,-16.0639439035367,
55.0225601732145));
#125727=CARTESIAN_POINT('Ctrl Pts',(3.17816178474359,-16.186719595967,55.0387021617065));
#125728=CARTESIAN_POINT('Ctrl Pts',(3.41100385579573,-16.3032809225961,
55.056892462709));
#125729=CARTESIAN_POINT('Ctrl Pts',(3.64796053047498,-16.4219020301537,
55.0754042085353));
#125730=CARTESIAN_POINT('Ctrl Pts',(3.88314339365675,-16.5340872788256,
55.0960374899752));
#125731=CARTESIAN_POINT('Ctrl Pts',(4.11606747139699,-16.6401981973185,
55.1187846528849));
#125732=CARTESIAN_POINT('Ctrl Pts',(4.18606844953421,-16.6720878506236,
55.1256208875455));
#125733=CARTESIAN_POINT('Ctrl Pts',(4.2558657319487,-16.7034287456591,55.1326479351931));
#125734=CARTESIAN_POINT('Ctrl Pts',(4.32544694935167,-16.7342303598792,
55.1398652916536));
#125735=CARTESIAN_POINT('Ctrl Pts',(4.50554310797927,-16.8139537767382,
55.1585458813659));
#125736=CARTESIAN_POINT('Ctrl Pts',(4.68419074392955,-16.8900651847476,
55.1785017228101));
#125737=CARTESIAN_POINT('Ctrl Pts',(4.86118763155564,-16.9627435466136,
55.1997069862893));
#125738=CARTESIAN_POINT('Ctrl Pts',(4.86118763155564,-16.9627435466136,
55.1997069862893));
#125739=CARTESIAN_POINT('Ctrl Pts',(5.13408696149748,-17.0747940674125,
55.2323981770183));
#125740=CARTESIAN_POINT('Ctrl Pts',(5.41104329099708,-17.1804252386101,
55.2682238076182));
#125741=CARTESIAN_POINT('Ctrl Pts',(5.69165293468597,-17.2792384440373,
55.3072587814995));
#125742=CARTESIAN_POINT('Ctrl Pts',(5.83195775653042,-17.3286450467509,
55.3267762684401));
#125743=CARTESIAN_POINT('Ctrl Pts',(5.97317512545962,-17.3763471920351,
55.3470957603042));
#125744=CARTESIAN_POINT('Ctrl Pts',(6.11524996609304,-17.4222956096913,
55.3682246325463));
#125745=CARTESIAN_POINT('Ctrl Pts',(6.18628738640975,-17.4452698185194,
55.3787890686673));
#125746=CARTESIAN_POINT('Ctrl Pts',(6.25753917329986,-17.4678056092315,
55.3895558296405));
#125747=CARTESIAN_POINT('Ctrl Pts',(6.32899810955315,-17.4898968769833,
55.4005257120424));
#125748=CARTESIAN_POINT('Ctrl Pts',(6.36472757767979,-17.5009425108593,
55.4060106532433));
#125749=CARTESIAN_POINT('Ctrl Pts',(6.40050883304789,-17.5118770148992,
55.411546373421));
#125750=CARTESIAN_POINT('Ctrl Pts',(6.43634096453578,-17.5226996315496,
55.4171329644763));
#125751=CARTESIAN_POINT('Ctrl Pts',(6.45425703027973,-17.5281109398747,
55.419926260004));
#125752=CARTESIAN_POINT('Ctrl Pts',(6.47218581504866,-17.5334942764124,
55.4227322731676));
#125753=CARTESIAN_POINT('Ctrl Pts',(6.4901272038462,-17.5388495467521,55.4255510149582));
#125754=CARTESIAN_POINT('Ctrl Pts',(6.49909789824497,-17.5415271819219,
55.4269603858535));
#125755=CARTESIAN_POINT('Ctrl Pts',(6.50807174365058,-17.544197800546,55.4283729389003));
#125756=CARTESIAN_POINT('Ctrl Pts',(6.51704872561684,-17.5468613908419,
55.4297886754419));
#125757=CARTESIAN_POINT('Ctrl Pts',(6.51794605115068,-17.5471276392975,
55.4299301903244));
#125758=CARTESIAN_POINT('Ctrl Pts',(6.51886222152525,-17.5473993989782,
55.4300747038184));
#125759=CARTESIAN_POINT('Ctrl Pts',(6.51979159730476,-17.547674988676,55.4302213294836));
#125760=CARTESIAN_POINT('Ctrl Pts',(6.52815983905417,-17.5501564404902,
55.4315415694125));
#125761=CARTESIAN_POINT('Ctrl Pts',(6.53759930005029,-17.5529464639317,
55.4330338954395));
#125762=CARTESIAN_POINT('Ctrl Pts',(6.54398906712212,-17.5548310661202,
55.4340454359284));
#125763=CARTESIAN_POINT('Ctrl Pts',(6.68482944491206,-17.5963706216668,
55.4563413573604));
#125764=CARTESIAN_POINT('Ctrl Pts',(6.83166069154892,-17.6378547174454,
55.4803409554723));
#125765=CARTESIAN_POINT('Ctrl Pts',(6.984546755397,-17.6788176469995,55.5062351627957));
#125766=CARTESIAN_POINT('Ctrl Pts',(7.13416335766372,-17.7189045861522,
55.5315756236631));
#125767=CARTESIAN_POINT('Ctrl Pts',(7.28957895861548,-17.7584923310297,
55.5587307194324));
#125768=CARTESIAN_POINT('Ctrl Pts',(7.45082986615249,-17.797101452478,55.5878880173816));
#125769=CARTESIAN_POINT('Ctrl Pts',(7.52348653070042,-17.814498005641,55.6010257543939));
#125770=CARTESIAN_POINT('Ctrl Pts',(7.59732754358988,-17.8316952951325,
55.6145700863502));
#125771=CARTESIAN_POINT('Ctrl Pts',(7.67235428721205,-17.8486465937323,
55.6285385959872));
#125772=CARTESIAN_POINT('Ctrl Pts',(7.74096883591555,-17.8641491418532,
55.6413132805667));
#125773=CARTESIAN_POINT('Ctrl Pts',(7.81057508931384,-17.8794459293272,
55.6544427411163));
#125774=CARTESIAN_POINT('Ctrl Pts',(7.88117307932695,-17.8944998967529,
55.667940560898));
#125775=CARTESIAN_POINT('Ctrl Pts',(7.91647207433351,-17.9020268804658,
55.6746894707888));
#125776=CARTESIAN_POINT('Ctrl Pts',(7.95201900356004,-17.9094931491135,
55.6815304811982));
#125777=CARTESIAN_POINT('Ctrl Pts',(7.98781375337589,-17.9168939410521,
55.6884652887162));
#125778=CARTESIAN_POINT('Ctrl Pts',(8.00571112828382,-17.9205943370214,
55.6919326924753));
#125779=CARTESIAN_POINT('Ctrl Pts',(8.02367045834657,-17.9242783632166,
55.6954235461614));
#125780=CARTESIAN_POINT('Ctrl Pts',(8.04169172558814,-17.9279454187725,
55.6989380638335));
#125781=CARTESIAN_POINT('Ctrl Pts',(8.05070235920893,-17.9297789465505,
55.7006953226695));
#125782=CARTESIAN_POINT('Ctrl Pts',(8.05972847712441,-17.9316082316297,
55.7024584975425));
#125783=CARTESIAN_POINT('Ctrl Pts',(8.06877007664731,-17.9334331984247,
55.7042276152159));
#125784=CARTESIAN_POINT('Ctrl Pts',(8.07781167617023,-17.9352581652196,
55.7059967328893));
#125785=CARTESIAN_POINT('Ctrl Pts',(8.08877438449428,-17.9374603051664,
55.7081458861864));
#125786=CARTESIAN_POINT('Ctrl Pts',(8.09594131721416,-17.9388950681421,
55.7095528234899));
#125787=CARTESIAN_POINT('Ctrl Pts',(8.24515499940074,-17.9687664615305,
55.7388448935938));
#125788=CARTESIAN_POINT('Ctrl Pts',(8.39258291270406,-17.9962919149135,
55.7686163247889));
#125789=CARTESIAN_POINT('Ctrl Pts',(8.53813373952569,-18.0216103412977,
55.7987959487959));
#125790=CARTESIAN_POINT('Ctrl Pts',(8.76031886400935,-18.0602592300793,
55.8448655154433));
#125791=CARTESIAN_POINT('Ctrl Pts',(8.97812767280675,-18.0937657232564,
55.8918855519334));
#125792=CARTESIAN_POINT('Ctrl Pts',(9.19129301389337,-18.1226368286976,
55.9395949763453));
#125793=CARTESIAN_POINT('Ctrl Pts',(9.40660253590258,-18.1517983419189,
55.987784298836));
#125794=CARTESIAN_POINT('Ctrl Pts',(9.61717482294331,-18.1762309612043,
56.0366767735567));
#125795=CARTESIAN_POINT('Ctrl Pts',(9.82278558814653,-18.1964489204329,
56.0860161043764));
#125796=CARTESIAN_POINT('Ctrl Pts',(9.89514614563819,-18.2035642229789,
56.1033800856876));
#125797=CARTESIAN_POINT('Ctrl Pts',(9.96689264452012,-18.2101574312165,
56.1207995386339));
#125798=CARTESIAN_POINT('Ctrl Pts',(10.0380167407446,-18.2162506428644,
56.1382637195788));
#125799=CARTESIAN_POINT('Ctrl Pts',(10.1387466453931,-18.2248801884174,
56.1629974648876));
#125800=CARTESIAN_POINT('Ctrl Pts',(10.2382280323521,-18.2325068870764,
56.1878208824132));
#125801=CARTESIAN_POINT('Ctrl Pts',(10.3364396630195,-18.2391928519174,
56.2127042782402));
#125802=CARTESIAN_POINT('Ctrl Pts',(10.3662481283228,-18.2412221263488,
56.2202567018798));
#125803=CARTESIAN_POINT('Ctrl Pts',(10.3959396301051,-18.2431647334506,
56.2278146535373));
#125804=CARTESIAN_POINT('Ctrl Pts',(10.4255136353887,-18.2450223953613,
56.2353773236462));
#125805=CARTESIAN_POINT('Ctrl Pts',(10.4446592011181,-18.246225005149,56.2402732312607));
#125806=CARTESIAN_POINT('Ctrl Pts',(10.4637555247294,-18.2473920143967,
56.2451711165242));
#125807=CARTESIAN_POINT('Ctrl Pts',(10.4828024737685,-18.248523895181,56.2500707531901));
#125808=CARTESIAN_POINT('Ctrl Pts',(10.5070367847156,-18.24996403926,56.2563047866958));
#125809=CARTESIAN_POINT('Ctrl Pts',(10.5311911582704,-18.2513473167322,
56.2625416565715));
#125810=CARTESIAN_POINT('Ctrl Pts',(10.5552653290177,-18.2526746938239,
56.268780896882));
#125811=CARTESIAN_POINT('Ctrl Pts',(10.5673024143913,-18.2533383823697,
56.2719005170373));
#125812=CARTESIAN_POINT('Ctrl Pts',(10.5793194490533,-18.2539880957524,
56.2750207298374));
#125813=CARTESIAN_POINT('Ctrl Pts',(10.5913163998402,-18.2546239547716,
56.2781414779492));
#125814=CARTESIAN_POINT('Ctrl Pts',(10.6033133506272,-18.2552598137908,
56.281262226061));
#125815=CARTESIAN_POINT('Ctrl Pts',(10.6136892177232,-18.255800371469,56.2839655080025));
#125816=CARTESIAN_POINT('Ctrl Pts',(10.627246968054,-18.2564900891339,56.2875052709587));
#125817=CARTESIAN_POINT('Ctrl Pts',(10.9015920746051,-18.2704467310282,
56.3591334261967));
#125818=CARTESIAN_POINT('Ctrl Pts',(11.1720029145194,-18.2775353472381,
56.4327922782982));
#125819=CARTESIAN_POINT('Ctrl Pts',(11.4381033505419,-18.2781754605747,
56.5081406300829));
#125820=CARTESIAN_POINT('Ctrl Pts',(11.7013982102515,-18.2788088250053,
56.5826945617075));
#125821=CARTESIAN_POINT('Ctrl Pts',(11.9604729780913,-18.2731289229042,
56.6589021614018));
#125822=CARTESIAN_POINT('Ctrl Pts',(12.2150117560152,-18.261557173146,56.7364262203268));
#125823=CARTESIAN_POINT('Ctrl Pts',(12.2719104662312,-18.2589704645841,
56.7537556779423));
#125824=CARTESIAN_POINT('Ctrl Pts',(12.3285827161712,-18.2560894089725,
56.7711509039483));
#125825=CARTESIAN_POINT('Ctrl Pts',(12.3850253198193,-18.2529188169293,
56.7886081168881));
#125826=CARTESIAN_POINT('Ctrl Pts',(12.6280044057201,-18.2392697733585,
56.8637594630048));
#125827=CARTESIAN_POINT('Ctrl Pts',(12.8667244425015,-18.2202541755889,
56.9400591331704));
#125828=CARTESIAN_POINT('Ctrl Pts',(13.1009783143073,-18.1962710403985,
57.0171918416888));
#125829=CARTESIAN_POINT('Ctrl Pts',(13.3454540417339,-18.1712413818642,
57.0976902978213));
#125830=CARTESIAN_POINT('Ctrl Pts',(13.5850649647323,-18.1408012563723,
57.1790956310876));
#125831=CARTESIAN_POINT('Ctrl Pts',(13.8196238143751,-18.1054157572537,
57.2610588229446));
#125832=CARTESIAN_POINT('Ctrl Pts',(14.0016511419414,-18.0779551525953,
57.3246656354577));
#125833=CARTESIAN_POINT('Ctrl Pts',(14.1806369067664,-18.0475165221978,
57.3886085529791));
#125834=CARTESIAN_POINT('Ctrl Pts',(14.3565139790441,-18.0143210898017,
57.4527306528993));
#125835=CARTESIAN_POINT('Ctrl Pts',(14.5849508451095,-17.9712054042491,
57.5360152525438));
#125836=CARTESIAN_POINT('Ctrl Pts',(14.808142012816,-17.9234390099083,57.6196010152843));
#125837=CARTESIAN_POINT('Ctrl Pts',(15.0260000176933,-17.8715129210895,
57.7031512683577));
#125838=CARTESIAN_POINT('Ctrl Pts',(15.1122043556141,-17.8509662622235,
57.7362113078699));
#125839=CARTESIAN_POINT('Ctrl Pts',(15.197574179134,-17.8297683615518,57.7692660605151));
#125840=CARTESIAN_POINT('Ctrl Pts',(15.2821060147948,-17.8079497558195,
57.8022957994193));
#125841=CARTESIAN_POINT('Ctrl Pts',(4.94558033465909,-16.73691709796,55.07275817496));
#125842=CARTESIAN_POINT('Ctrl Pts',(5.28026245545909,-16.877827078,55.10599062996));
#125843=CARTESIAN_POINT('Ctrl Pts',(6.08156567048909,-17.18655968786,55.19564711277));
#125844=CARTESIAN_POINT('Ctrl Pts',(7.32238711382909,-17.56623194746,55.37236882206));
#125845=CARTESIAN_POINT('Ctrl Pts',(8.60269693009909,-17.85372405277,55.59911231378));
#125846=CARTESIAN_POINT('Ctrl Pts',(9.75286163943908,-18.0317753553,55.8397251211601));
#125847=CARTESIAN_POINT('Ctrl Pts',(10.8188407317891,-18.13130923193,56.09418879665));
#125848=CARTESIAN_POINT('Ctrl Pts',(11.8646555289291,-18.16653886356,56.3744521454));
#125849=CARTESIAN_POINT('Ctrl Pts',(12.9185497408191,-18.13616215699,56.68933508407));
#125850=CARTESIAN_POINT('Ctrl Pts',(13.9431659298891,-18.03863753101,57.02804389316));
#125851=CARTESIAN_POINT('Ctrl Pts',(14.8522303901791,-17.89093940842,57.3563849417));
#125852=CARTESIAN_POINT('Ctrl Pts',(15.4050401168391,-17.76756499744,57.57011599991));
#125853=CARTESIAN_POINT('Ctrl Pts',(15.6447528874391,-17.7074511508,57.66533851275));
#125854=CARTESIAN_POINT('Ctrl Pts',(1.34059656653909,-19.36072534028,56.89732226648));
#125855=CARTESIAN_POINT('Ctrl Pts',(1.74623295480909,-19.53025176889,57.0298489626201));
#125856=CARTESIAN_POINT('Ctrl Pts',(2.69773504947909,-19.86856616523,57.34298332191));
#125857=CARTESIAN_POINT('Ctrl Pts',(4.10404431957909,-20.19175246157,57.82133063031));
#125858=CARTESIAN_POINT('Ctrl Pts',(5.48295515591909,-20.33570170296,58.30871066767));
#125859=CARTESIAN_POINT('Ctrl Pts',(6.66706436789909,-20.33231978859,58.74039296884));
#125860=CARTESIAN_POINT('Ctrl Pts',(7.72117288249909,-20.22891362284,59.13262578937));
#125861=CARTESIAN_POINT('Ctrl Pts',(8.71648603674909,-20.03904678401,59.50701950141));
#125862=CARTESIAN_POINT('Ctrl Pts',(9.68245645954909,-19.76211419568,59.87017792638));
#125863=CARTESIAN_POINT('Ctrl Pts',(10.5890305168591,-19.4126839085,60.20557239847));
#125864=CARTESIAN_POINT('Ctrl Pts',(11.3702963784091,-19.03754467514,60.4854871058399));
#125865=CARTESIAN_POINT('Ctrl Pts',(11.8361982920691,-18.77679247185,60.64563044228));
#125866=CARTESIAN_POINT('Ctrl Pts',(12.0369318547391,-18.657705851,60.71311141309));
#125867=CARTESIAN_POINT('Ctrl Pts',(-1.75622200369091,-22.80586325942,55.57455847696));
#125868=CARTESIAN_POINT('Ctrl Pts',(-1.27988520209091,-23.08527728226,55.82753333339));
#125869=CARTESIAN_POINT('Ctrl Pts',(-0.164033475360911,-23.64821979482,
56.42532032641));
#125870=CARTESIAN_POINT('Ctrl Pts',(1.47552702563909,-24.21351924158,57.33972030603));
#125871=CARTESIAN_POINT('Ctrl Pts',(3.06337678448909,-24.51022608242,58.27488614442));
#125872=CARTESIAN_POINT('Ctrl Pts',(4.40638925420909,-24.57683508764,59.10793062424));
#125873=CARTESIAN_POINT('Ctrl Pts',(5.58071779312909,-24.48672687027,59.87004703943));
#125874=CARTESIAN_POINT('Ctrl Pts',(6.66586605652908,-24.26362966974,60.60326872942));
#125875=CARTESIAN_POINT('Ctrl Pts',(7.6915675903991,-23.90746855691,61.32138257166));
#125876=CARTESIAN_POINT('Ctrl Pts',(8.62353581161909,-23.43716483225,61.9914774074));
#125877=CARTESIAN_POINT('Ctrl Pts',(9.39869767618908,-22.91856774323,62.55627460265));
#125878=CARTESIAN_POINT('Ctrl Pts',(9.84576389899909,-22.55231998127,62.8815147844301));
#125879=CARTESIAN_POINT('Ctrl Pts',(10.0354867964191,-22.3841506822,63.018780147989));
#125880=CARTESIAN_POINT('Ctrl Pts',(-2.89864469832391,-25.46343319653,51.72220450345));
#125881=CARTESIAN_POINT('Ctrl Pts',(-2.38487880508091,-25.88268787062,52.0605315104));
#125882=CARTESIAN_POINT('Ctrl Pts',(-1.16727884272091,-26.76040230889,52.87121160649));
#125883=CARTESIAN_POINT('Ctrl Pts',(0.664366732859086,-27.75334589591,54.152452422));
#125884=CARTESIAN_POINT('Ctrl Pts',(2.47391773298909,-28.42777219138,55.51343497556));
#125885=CARTESIAN_POINT('Ctrl Pts',(4.02658355238909,-28.78311012245,56.77069605527));
#125886=CARTESIAN_POINT('Ctrl Pts',(5.39707932946909,-28.91632763189,57.96207291656));
#125887=CARTESIAN_POINT('Ctrl Pts',(6.67044598217909,-28.86738493337,59.15124563255));
#125888=CARTESIAN_POINT('Ctrl Pts',(7.87563878198909,-28.63632279394,60.3652287628));
#125889=CARTESIAN_POINT('Ctrl Pts',(8.96457825374909,-28.23262639115,61.55173181993));
#125890=CARTESIAN_POINT('Ctrl Pts',(9.85818132202908,-27.72155028017,62.60167870114));
#125891=CARTESIAN_POINT('Ctrl Pts',(10.3632803435291,-27.33095617795,63.233599193963));
#125892=CARTESIAN_POINT('Ctrl Pts',(10.5751031573891,-27.14651616736,63.505585203961));
#125893=CARTESIAN_POINT('',(0.214753670929088,-21.31105119265,55.46569744597));
#125894=CARTESIAN_POINT('Ctrl Pts',(4.86118780824909,-16.96274255881,55.19970889703));
#125895=CARTESIAN_POINT('Ctrl Pts',(3.24795847665787,-18.1787189357449,
55.9775434950793));
#125896=CARTESIAN_POINT('Ctrl Pts',(1.63141885578447,-19.6797052340533,
56.0974256036295));
#125897=CARTESIAN_POINT('Ctrl Pts',(0.214753670929088,-21.31105119265,55.46569744597));
#125898=CARTESIAN_POINT('',(10.422120832449,-26.9525721548983,63.3189206077878));
#125899=CARTESIAN_POINT('Ctrl Pts',(0.214753670929088,-21.31105119265,55.46569744597));
#125900=CARTESIAN_POINT('Ctrl Pts',(0.290187002274114,-21.4155332695987,
55.4996802294028));
#125901=CARTESIAN_POINT('Ctrl Pts',(0.44074324512562,-21.6239539292895,
55.5672851854211));
#125902=CARTESIAN_POINT('Ctrl Pts',(0.673504421678082,-21.9280409589524,
55.6749490529411));
#125903=CARTESIAN_POINT('Ctrl Pts',(0.910137783129716,-22.2247972557687,
55.7869376302151));
#125904=CARTESIAN_POINT('Ctrl Pts',(1.15078407677516,-22.5137264542137,
55.9037690189854));
#125905=CARTESIAN_POINT('Ctrl Pts',(1.39501754485644,-22.7949068800299,
56.0253588111342));
#125906=CARTESIAN_POINT('Ctrl Pts',(1.64265138383823,-23.0681707206839,
56.1517636676972));
#125907=CARTESIAN_POINT('Ctrl Pts',(1.89341726172454,-23.3334286266629,
56.2830032944462));
#125908=CARTESIAN_POINT('Ctrl Pts',(2.14706268673953,-23.5905979055829,
56.4191130640057));
#125909=CARTESIAN_POINT('Ctrl Pts',(2.40331415145427,-23.8396233403112,
56.5601306035357));
#125910=CARTESIAN_POINT('Ctrl Pts',(2.66190654374435,-24.0804379098326,
56.7060819271997));
#125911=CARTESIAN_POINT('Ctrl Pts',(2.92260263037789,-24.312940414964,56.8569721248615));
#125912=CARTESIAN_POINT('Ctrl Pts',(3.18514629285495,-24.537043024692,57.0128078932314));
#125913=CARTESIAN_POINT('Ctrl Pts',(3.44928284702211,-24.7526663920023,
57.1735971708211));
#125914=CARTESIAN_POINT('Ctrl Pts',(3.71474257272434,-24.9597539591783,
57.3393510545193));
#125915=CARTESIAN_POINT('Ctrl Pts',(3.98128843413907,-25.1582070270359,
57.5100682063123));
#125916=CARTESIAN_POINT('Ctrl Pts',(4.248667984514,-25.3479921026865,57.6857082905432));
#125917=CARTESIAN_POINT('Ctrl Pts',(4.51673610366451,-25.5287769949927,
57.8663174785204));
#125918=CARTESIAN_POINT('Ctrl Pts',(4.80979204127848,-25.7174013418108,
58.0688292490302));
#125919=CARTESIAN_POINT('Ctrl Pts',(5.34984032046011,-26.0368282294947,
58.4529844481055));
#125920=CARTESIAN_POINT('Ctrl Pts',(6.00395547931118,-26.3813417007364,
58.9484029796231));
#125921=CARTESIAN_POINT('Ctrl Pts',(6.76922502482267,-26.7008669853632,
59.5749062650414));
#125922=CARTESIAN_POINT('Ctrl Pts',(7.44523296529213,-26.9154311025405,
60.1638164809444));
#125923=CARTESIAN_POINT('Ctrl Pts',(8.05943260808658,-27.0474061126848,
60.7373939732686));
#125924=CARTESIAN_POINT('Ctrl Pts',(8.58328127952353,-27.1133122218592,
61.2563918549296));
#125925=CARTESIAN_POINT('Ctrl Pts',(8.99487194315013,-27.1362136993778,
61.6824057705528));
#125926=CARTESIAN_POINT('Ctrl Pts',(9.38423160485021,-27.1299300466065,
62.1028527403915));
#125927=CARTESIAN_POINT('Ctrl Pts',(9.75118830050383,-27.0960867289846,
62.5160177603512));
#125928=CARTESIAN_POINT('Ctrl Pts',(10.0969192926289,-27.0393423587567,
62.9200265760865));
#125929=CARTESIAN_POINT('Ctrl Pts',(10.3150222716872,-26.9811488497848,
63.1875477293253));
#125930=CARTESIAN_POINT('Ctrl Pts',(10.4221208324491,-26.9525721549,63.318920607788));
#125931=CARTESIAN_POINT('Origin',(17.8170477102388,-26.9525619812102,57.3553028688338));
#125932=CARTESIAN_POINT('Ctrl Pts',(15.3838087950991,-17.76813627932,57.47088283762));
#125933=CARTESIAN_POINT('Ctrl Pts',(15.5136776391891,-17.7399793982,57.61873928627));
#125934=CARTESIAN_POINT('Ctrl Pts',(16.6719036715191,-17.48466648861,58.96026165475));
#125935=CARTESIAN_POINT('Ctrl Pts',(18.6380558813391,-16.98952718735,61.62070291459));
#125936=CARTESIAN_POINT('Ctrl Pts',(20.1925743271491,-16.57554208156,64.475671438406));
#125937=CARTESIAN_POINT('Ctrl Pts',(20.8483496278291,-16.41007917736,65.90602790217));
#125938=CARTESIAN_POINT('Ctrl Pts',(11.8147841629991,-18.75274562585,60.55324082484));
#125939=CARTESIAN_POINT('Ctrl Pts',(11.9272368286891,-18.72450512001,60.68095860922));
#125940=CARTESIAN_POINT('Ctrl Pts',(12.9302993033491,-18.46854961149,61.83994096131));
#125941=CARTESIAN_POINT('Ctrl Pts',(14.6355320841891,-17.97406652798,64.141414936219));
#125942=CARTESIAN_POINT('Ctrl Pts',(15.9859865671191,-17.5628505011,66.6161169938171));
#125943=CARTESIAN_POINT('Ctrl Pts',(16.5558929421091,-17.3987396548,67.85685075686));
#125944=CARTESIAN_POINT('Ctrl Pts',(9.83041017598908,-22.50758332692,62.8274075721));
#125945=CARTESIAN_POINT('Ctrl Pts',(9.93119743901908,-22.47902391565,62.94546639158));
#125946=CARTESIAN_POINT('Ctrl Pts',(10.8283385940591,-22.22061783658,64.014699314213));
#125947=CARTESIAN_POINT('Ctrl Pts',(12.3248185130891,-21.72863725946,66.102727503159));
#125948=CARTESIAN_POINT('Ctrl Pts',(13.4841962641491,-21.32798119921,68.290608316712));
#125949=CARTESIAN_POINT('Ctrl Pts',(13.9709785907491,-21.16902646686,69.377215769556));
#125950=CARTESIAN_POINT('Ctrl Pts',(10.3574012282691,-27.27911795738,63.231333751354));
#125951=CARTESIAN_POINT('Ctrl Pts',(10.4577216764591,-27.25015329071,63.354724099072));
#125952=CARTESIAN_POINT('Ctrl Pts',(11.3476496329491,-26.98863310041,64.468911693823));
#125953=CARTESIAN_POINT('Ctrl Pts',(12.7850320790991,-26.49983263301,66.58869604085));
#125954=CARTESIAN_POINT('Ctrl Pts',(13.8555542937391,-26.11259586023,68.717148050722));
#125955=CARTESIAN_POINT('Ctrl Pts',(14.3007768717191,-25.96019336214,69.757103482774));
#125956=CARTESIAN_POINT('Ctrl Pts',(10.4221208324491,-26.9525721549,63.318920607788));
#125957=CARTESIAN_POINT('Ctrl Pts',(10.4905170530396,-26.9326350193341,
63.4037419898396));
#125958=CARTESIAN_POINT('Ctrl Pts',(11.3467766751192,-26.6801389649098,
64.4784607693732));
#125959=CARTESIAN_POINT('Ctrl Pts',(12.7315159791238,-26.2103421355703,
66.51344276841));
#125960=CARTESIAN_POINT('Ctrl Pts',(13.7906434600985,-25.8290501580449,
68.5975758543698));
#125961=CARTESIAN_POINT('Ctrl Pts',(14.2241252549691,-25.68032884552,69.591853101251));
#125962=CARTESIAN_POINT('Origin',(-10.9843331791359,-89.,80.581991049076));
#125963=CARTESIAN_POINT('',(12.8491777764712,-90.5,70.1914310155131));
#125964=CARTESIAN_POINT('Origin',(12.8491780888091,-89.,70.191430879345));
#125965=CARTESIAN_POINT('',(0.214666886482069,-89.,55.465613970957));
#125966=CARTESIAN_POINT('Origin',(-10.9843331791359,-89.,80.581991049076));
#125967=CARTESIAN_POINT('',(-0.396188736334104,-90.4999999999959,56.8356005834295));
#125968=CARTESIAN_POINT('Origin',(-0.396187662550911,-89.,56.83559817522));
#125969=CARTESIAN_POINT('Origin',(-10.9843331791359,-90.5,80.581991049076));
#125970=CARTESIAN_POINT('Origin',(6.43246351666909,-89.,72.98888938658));
#125971=CARTESIAN_POINT('',(12.8491777757672,-90.5,75.7863477573401));
#125972=CARTESIAN_POINT('Origin',(12.8491780888091,-89.,75.786347893815));
#125973=CARTESIAN_POINT('Origin',(6.43246351666909,-90.5,72.98888938658));
#125974=CARTESIAN_POINT('Origin',(-10.9843331791359,-89.,65.395787724084));
#125975=CARTESIAN_POINT('',(-0.39618873597521,-90.4999999999959,89.1421781905352));
#125976=CARTESIAN_POINT('',(0.214666886482189,-89.,90.5121648022033));
#125977=CARTESIAN_POINT('Origin',(-0.396187662550911,-89.,89.14218059794));
#125978=CARTESIAN_POINT('Origin',(-10.9843331791359,-89.,65.395787724084));
#125979=CARTESIAN_POINT('Origin',(-10.9843331791359,-90.5,65.395787724084));
#125980=CARTESIAN_POINT('Origin',(-10.9843331791359,-92.5,65.395787724084));
#125981=CARTESIAN_POINT('',(0.21473688718606,-24.69203306784,90.5121335898666));
#125982=CARTESIAN_POINT('Ctrl Pts',(8.76687408897909,-16.44294428525,98.6115064056));
#125983=CARTESIAN_POINT('Ctrl Pts',(8.50448839268907,-16.29482593816,98.7748340168099));
#125984=CARTESIAN_POINT('Ctrl Pts',(7.73803846225909,-15.84050813694,99.1889282148399));
#125985=CARTESIAN_POINT('Ctrl Pts',(6.5349477692391,-15.02004513321,99.57986765328));
#125986=CARTESIAN_POINT('Ctrl Pts',(5.27236547025909,-14.00812222941,99.71688058005));
#125987=CARTESIAN_POINT('Ctrl Pts',(4.18367013900909,-13.00986029655,99.6525682338999));
#125988=CARTESIAN_POINT('Ctrl Pts',(3.20714073810909,-11.9973978225,99.4540121251699));
#125989=CARTESIAN_POINT('Ctrl Pts',(2.30415558486909,-10.93738557134,99.14726582813));
#125990=CARTESIAN_POINT('Ctrl Pts',(1.48684448748909,-9.84723726948199,
98.7638938018301));
#125991=CARTESIAN_POINT('Ctrl Pts',(0.762911702719089,-8.74553579959698,
98.3366761029799));
#125992=CARTESIAN_POINT('Ctrl Pts',(0.112673674949087,-7.60752902450998,
97.87904754731));
#125993=CARTESIAN_POINT('Ctrl Pts',(-0.488386309690911,-6.37224922945299,
97.3887134898101));
#125994=CARTESIAN_POINT('Ctrl Pts',(-1.04213634100091,-4.97114208044499,
96.8726660516999));
#125995=CARTESIAN_POINT('Ctrl Pts',(-1.51067364081091,-3.36802983074299,
96.3809404461301));
#125996=CARTESIAN_POINT('Ctrl Pts',(-1.81701727702091,-1.61981132427399,
96.0275490175501));
#125997=CARTESIAN_POINT('Ctrl Pts',(-1.87689058580091,-0.403435681896786,
95.95525979127));
#125998=CARTESIAN_POINT('Ctrl Pts',(-1.86852961382091,0.200651371990514,
95.9651297134299));
#125999=CARTESIAN_POINT('Ctrl Pts',(6.48819653156909,-15.56528785696,92.69131734964));
#126000=CARTESIAN_POINT('Ctrl Pts',(6.38630096531909,-15.47758556196,92.78395944648));
#126001=CARTESIAN_POINT('Ctrl Pts',(6.06771745324909,-15.21581444004,93.0220629079301));
#126002=CARTESIAN_POINT('Ctrl Pts',(5.4599981715091,-14.7540110982,93.25770281466));
#126003=CARTESIAN_POINT('Ctrl Pts',(4.67600680749909,-14.1542490297,93.3348504985));
#126004=CARTESIAN_POINT('Ctrl Pts',(3.89225004337909,-13.51762150969,93.2708681228701));
#126005=CARTESIAN_POINT('Ctrl Pts',(3.10219061563909,-12.82180106148,93.10110938746));
#126006=CARTESIAN_POINT('Ctrl Pts',(2.29351899611909,-12.03547497051,92.8361696333));
#126007=CARTESIAN_POINT('Ctrl Pts',(1.49269764718909,-11.16347023105,92.4954481808701));
#126008=CARTESIAN_POINT('Ctrl Pts',(0.723899763099089,-10.21566958806,92.10308906725));
#126009=CARTESIAN_POINT('Ctrl Pts',(-0.0200535606409112,-9.16446753653399,
91.66798555359));
#126010=CARTESIAN_POINT('Ctrl Pts',(-0.760996247700911,-7.93604781061299,
91.18364248321));
#126011=CARTESIAN_POINT('Ctrl Pts',(-1.50146348324091,-6.42271318686499,
90.65003751555));
#126012=CARTESIAN_POINT('Ctrl Pts',(-2.18733220258091,-4.52156727656799,
90.1121766327));
#126013=CARTESIAN_POINT('Ctrl Pts',(-2.67864361223591,-2.24136809065099,
89.70052285778));
#126014=CARTESIAN_POINT('Ctrl Pts',(-2.78026244461691,-0.556674570830786,
89.61294403093));
#126015=CARTESIAN_POINT('Ctrl Pts',(-2.76634006182491,0.277047208448614,
89.6246271184));
#126016=CARTESIAN_POINT('Ctrl Pts',(2.72889798757909,-19.34707978044,89.1447316619801));
#126017=CARTESIAN_POINT('Ctrl Pts',(2.66091020417909,-19.26097438926,89.20317193542));
#126018=CARTESIAN_POINT('Ctrl Pts',(2.42996072068909,-19.00901506437,89.3612231288901));
#126019=CARTESIAN_POINT('Ctrl Pts',(1.89825599140909,-18.57235792605,89.54995470502));
#126020=CARTESIAN_POINT('Ctrl Pts',(1.10699433400909,-17.98310305551,89.64471299023));
#126021=CARTESIAN_POINT('Ctrl Pts',(0.252027388659088,-17.32630382037,89.6293082806));
#126022=CARTESIAN_POINT('Ctrl Pts',(-0.654644487020914,-16.5759732809,89.5211787480401));
#126023=CARTESIAN_POINT('Ctrl Pts',(-1.61859475251091,-15.69330276297,89.32252842609));
#126024=CARTESIAN_POINT('Ctrl Pts',(-2.60190967346991,-14.67920705201,89.04432012876));
#126025=CARTESIAN_POINT('Ctrl Pts',(-3.56872088692091,-13.5426076308,88.7048190356501));
#126026=CARTESIAN_POINT('Ctrl Pts',(-4.52340351538191,-12.24737090716,88.3108681836801));
#126027=CARTESIAN_POINT('Ctrl Pts',(-5.49218708965691,-10.69472182793,87.8542655723));
#126028=CARTESIAN_POINT('Ctrl Pts',(-6.47884434265791,-8.73212611500698,
87.33045821777));
#126029=CARTESIAN_POINT('Ctrl Pts',(-7.41072188100292,-6.20174180863199,
86.77974038575));
#126030=CARTESIAN_POINT('Ctrl Pts',(-8.09046417872891,-3.09478014856899,
86.34080207947));
#126031=CARTESIAN_POINT('Ctrl Pts',(-8.23255272084991,-0.768163226373987,
86.24527748657));
#126032=CARTESIAN_POINT('Ctrl Pts',(-8.21314998798691,0.382355724809714,
86.2578544693));
#126033=CARTESIAN_POINT('Ctrl Pts',(0.196332399109088,-25.06476693734,90.52591274045));
#126034=CARTESIAN_POINT('Ctrl Pts',(0.011250503809089,-24.92028925106,90.61126618974));
#126035=CARTESIAN_POINT('Ctrl Pts',(-0.555409203350912,-24.48834062706,
90.84285524963));
#126036=CARTESIAN_POINT('Ctrl Pts',(-1.58520004181091,-23.72520655934,91.1268519171499));
#126037=CARTESIAN_POINT('Ctrl Pts',(-2.86435733527191,-22.73723822501,91.3040139279599));
#126038=CARTESIAN_POINT('Ctrl Pts',(-4.11539939684391,-21.69298831769,91.35045014482));
#126039=CARTESIAN_POINT('Ctrl Pts',(-5.35778473735791,-20.55625239098,91.29239781524));
#126040=CARTESIAN_POINT('Ctrl Pts',(-6.61477798365991,-19.27659173514,91.13677980334));
#126041=CARTESIAN_POINT('Ctrl Pts',(-7.84814243484691,-17.86250092626,90.8959268123599));
#126042=CARTESIAN_POINT('Ctrl Pts',(-9.02351089959392,-16.33037133773,90.58921613446));
#126043=CARTESIAN_POINT('Ctrl Pts',(-10.1541748021089,-14.63600828855,90.2254084335399));
#126044=CARTESIAN_POINT('Ctrl Pts',(-11.2746720699649,-12.6615424041,89.79831775978));
#126045=CARTESIAN_POINT('Ctrl Pts',(-12.3896921849461,-10.2361987255,89.30460716211));
#126046=CARTESIAN_POINT('Ctrl Pts',(-13.4190864676907,-7.19853323577899,
88.78356996623));
#126047=CARTESIAN_POINT('Ctrl Pts',(-14.1550194975079,-3.56544121650899,
88.3679745890099));
#126048=CARTESIAN_POINT('Ctrl Pts',(-14.3071566503109,-0.885592743395686,
88.2775704089799));
#126049=CARTESIAN_POINT('Ctrl Pts',(-14.2863014408449,0.440736329119914,
88.28947825565));
#126050=CARTESIAN_POINT('Ctrl Pts',(0.214736886699963,-24.69203306784,90.5121335896161));
#126051=CARTESIAN_POINT('Ctrl Pts',(0.135114761630916,-24.5692710385346,
90.5476371811463));
#126052=CARTESIAN_POINT('Ctrl Pts',(0.052735907442164,-24.4383412814108,
90.5820965139287));
#126053=CARTESIAN_POINT('Ctrl Pts',(-0.0321695795334493,-24.2989037853877,
90.6151059543716));
#126054=CARTESIAN_POINT('Ctrl Pts',(-0.114946239082119,-24.1629623928139,
90.6472877521653));
#126055=CARTESIAN_POINT('Ctrl Pts',(-0.200124190341312,-24.0189345404467,
90.6780910702463));
#126056=CARTESIAN_POINT('Ctrl Pts',(-0.287451667108242,-23.866505156519,
90.7071710142038));
#126057=CARTESIAN_POINT('Ctrl Pts',(-0.373795459489902,-23.7157927854992,
90.7359233924528));
#126058=CARTESIAN_POINT('Ctrl Pts',(-0.462240397255042,-23.5568670919221,
90.7629906234067));
#126059=CARTESIAN_POINT('Ctrl Pts',(-0.552508207420546,-23.3894235317423,
90.7880757248107));
#126060=CARTESIAN_POINT('Ctrl Pts',(-0.641604436653361,-23.2241532123008,
90.8128352480662));
#126061=CARTESIAN_POINT('Ctrl Pts',(-0.732476223101845,-23.0505846972385,
90.8356634669094));
#126062=CARTESIAN_POINT('Ctrl Pts',(-0.824825740468708,-22.8684251472527,
90.8563154157583));
#126063=CARTESIAN_POINT('Ctrl Pts',(-0.885203755326287,-22.749329429927,
90.869817637643));
#126064=CARTESIAN_POINT('Ctrl Pts',(-0.946212818488541,-22.6265614486943,
90.8823904467332));
#126065=CARTESIAN_POINT('Ctrl Pts',(-1.00776358327158,-22.5000393642437,
90.8939758070014));
#126066=CARTESIAN_POINT('Origin',(-2.02513312664091,-22.5,85.48888938658));
#126067=CARTESIAN_POINT('Origin',(-5.70733270705591,-22.5,87.05138938658));
#126068=CARTESIAN_POINT('Origin',(-2.02513312664091,-22.5,85.48888938658));
#126069=CARTESIAN_POINT('Origin',(27.4324635166691,-22.5,72.98888938658));
#126070=CARTESIAN_POINT('Origin',(-6.80729512863291,91.08441266238,84.10819367738));
#126071=CARTESIAN_POINT('Origin',(27.4324635166691,-10.,72.98888938658));
#126072=CARTESIAN_POINT('Origin',(-5.70733270705591,-10.,58.92638938658));
#126073=CARTESIAN_POINT('Origin',(-2.02513312664091,-10.,60.48888938658));
#126074=CARTESIAN_POINT('Origin',(-2.02513312664091,-10.,60.48888938658));
#126075=CARTESIAN_POINT('Origin',(1.07038457110909,25.,122.41156512159));
#126076=CARTESIAN_POINT('',(-2.29980363729091,-12.04041068638,54.99575678068));
#126077=CARTESIAN_POINT('Ctrl Pts',(-2.14405189383092,-11.77841163181,54.98461154933));
#126078=CARTESIAN_POINT('Ctrl Pts',(-2.10733458956091,-11.8187886285,54.98225755956));
#126079=CARTESIAN_POINT('Ctrl Pts',(-1.81762989816091,-12.13455643069,54.96398728809));
#126080=CARTESIAN_POINT('Ctrl Pts',(-1.26179089513091,-12.69950422949,54.933471617));
#126081=CARTESIAN_POINT('Ctrl Pts',(-0.446514994060916,-13.4374136371,54.90142190873));
#126082=CARTESIAN_POINT('Ctrl Pts',(0.421832340659087,-14.13773705744,54.88216946334));
#126083=CARTESIAN_POINT('Ctrl Pts',(1.37110882200909,-14.81739036068,54.87937527486));
#126084=CARTESIAN_POINT('Ctrl Pts',(2.42408380219909,-15.48145775016,54.89986692453));
#126085=CARTESIAN_POINT('Ctrl Pts',(3.59645485546909,-16.12374680622,54.954373838));
#126086=CARTESIAN_POINT('Ctrl Pts',(4.53992671491909,-16.5656803246,55.02943094317));
#126087=CARTESIAN_POINT('Ctrl Pts',(5.09008858763909,-16.7974718924,55.08714039026));
#126088=CARTESIAN_POINT('Ctrl Pts',(5.21318854215909,-16.84808010424,55.10078336932));
#126089=CARTESIAN_POINT('Ctrl Pts',(-4.28237251991691,-12.90485596602,55.1580085027501));
#126090=CARTESIAN_POINT('Ctrl Pts',(-4.24372968062391,-12.94840060018,55.15907732619));
#126091=CARTESIAN_POINT('Ctrl Pts',(-3.93840831922691,-13.28959911889,55.16788641051));
#126092=CARTESIAN_POINT('Ctrl Pts',(-3.34715337824091,-13.90827595377,55.19058747105));
#126093=CARTESIAN_POINT('Ctrl Pts',(-2.48081635714091,-14.71143693515,55.23984234275));
#126094=CARTESIAN_POINT('Ctrl Pts',(-1.55944190911091,-15.46716013561,55.31045650299));
#126095=CARTESIAN_POINT('Ctrl Pts',(-0.557170387470911,-16.1876489274,55.40933310786));
#126096=CARTESIAN_POINT('Ctrl Pts',(0.548874055019088,-16.87559341254,55.54601184312));
#126097=CARTESIAN_POINT('Ctrl Pts',(1.76798737872909,-17.51338121009,55.7316611044));
#126098=CARTESIAN_POINT('Ctrl Pts',(2.73528991332909,-17.92273736427,55.91074213052));
#126099=CARTESIAN_POINT('Ctrl Pts',(3.29175315981909,-18.1226855046,56.02609352246));
#126100=CARTESIAN_POINT('Ctrl Pts',(3.41585682087909,-18.16550598283,56.0524294903401));
#126101=CARTESIAN_POINT('Ctrl Pts',(-6.33980068353391,-13.96283635342,54.43755959959));
#126102=CARTESIAN_POINT('Ctrl Pts',(-6.30013246113791,-14.01063098128,54.44188653861));
#126103=CARTESIAN_POINT('Ctrl Pts',(-5.98625783669891,-14.38591317071,54.47649765105));
#126104=CARTESIAN_POINT('Ctrl Pts',(-5.37248291156191,-15.07664932369,54.5503049645301));
#126105=CARTESIAN_POINT('Ctrl Pts',(-4.47094738816091,-15.97723355204,54.67900680025));
#126106=CARTESIAN_POINT('Ctrl Pts',(-3.50976072054391,-16.82815842919,54.83934263413));
#126107=CARTESIAN_POINT('Ctrl Pts',(-2.46460587503091,-17.63890746411,55.04250813135));
#126108=CARTESIAN_POINT('Ctrl Pts',(-1.31102675741091,-18.41248543844,55.3026771825401));
#126109=CARTESIAN_POINT('Ctrl Pts',(-0.0441936566409133,-19.12227138079,
55.63466619505));
#126110=CARTESIAN_POINT('Ctrl Pts',(0.954446004809087,-19.56714593259,55.93839568086));
#126111=CARTESIAN_POINT('Ctrl Pts',(1.52418405419909,-19.77714734994,56.12781832211));
#126112=CARTESIAN_POINT('Ctrl Pts',(1.65098036279909,-19.82165893627,56.17076531156));
#126113=CARTESIAN_POINT('Ctrl Pts',(-8.03244000396691,-14.8063662618,52.92267673657));
#126114=CARTESIAN_POINT('Ctrl Pts',(-7.99278803894591,-14.85890679976,52.92964751905));
#126115=CARTESIAN_POINT('Ctrl Pts',(-7.67860378938091,-15.27222254309,52.98522301204));
#126116=CARTESIAN_POINT('Ctrl Pts',(-7.05831227750691,-16.04340511569,53.10097414993));
#126117=CARTESIAN_POINT('Ctrl Pts',(-6.14229777174491,-17.06014121543,53.29630276114));
#126118=CARTESIAN_POINT('Ctrl Pts',(-5.16000730910191,-18.03293316272,53.5338349975401));
#126119=CARTESIAN_POINT('Ctrl Pts',(-4.08799815650491,-18.97091254114,53.82951707404));
#126120=CARTESIAN_POINT('Ctrl Pts',(-2.89897827285191,-19.88006417146,54.20343973087));
#126121=CARTESIAN_POINT('Ctrl Pts',(-1.59003255186091,-20.72841292249,54.67677305415));
#126122=CARTESIAN_POINT('Ctrl Pts',(-0.556873398130915,-21.27200059043,
55.10857579009));
#126123=CARTESIAN_POINT('Ctrl Pts',(0.0312811456690863,-21.53256477732,
55.37827818613));
#126124=CARTESIAN_POINT('Ctrl Pts',(0.162087495049087,-21.58801296415,55.43946214072));
#126125=CARTESIAN_POINT('Ctrl Pts',(-2.29980340877935,-12.0404106863416,
54.9957613525836));
#126126=CARTESIAN_POINT('Ctrl Pts',(-2.29979627965971,-12.0404473675576,
54.9957609965661));
#126127=CARTESIAN_POINT('Ctrl Pts',(-2.29978915050876,-12.0404840487877,
54.9957606405607));
#126128=CARTESIAN_POINT('Ctrl Pts',(-2.29978202132649,-12.0405207300321,
54.9957602845673));
#126129=CARTESIAN_POINT('Ctrl Pts',(-2.27572901261885,-12.1642788632817,
54.9945592054126));
#126130=CARTESIAN_POINT('Ctrl Pts',(-2.2513175691152,-12.2882021978735,
54.993495270802));
#126131=CARTESIAN_POINT('Ctrl Pts',(-2.22648966927543,-12.4123811458191,
54.9925841664874));
#126132=CARTESIAN_POINT('Ctrl Pts',(-2.20172610202318,-12.5362383286098,
54.9916754229724));
#126133=CARTESIAN_POINT('Ctrl Pts',(-2.1765480591974,-12.6603501622916,
54.9909187023437));
#126134=CARTESIAN_POINT('Ctrl Pts',(-2.15092231702737,-12.7847590309372,
54.9903311614157));
#126135=CARTESIAN_POINT('Ctrl Pts',(-2.12529657485734,-12.9091678995828,
54.9897436204878));
#126136=CARTESIAN_POINT('Ctrl Pts',(-2.09922294790261,-13.0338741904353,
54.9893252401201));
#126137=CARTESIAN_POINT('Ctrl Pts',(-2.07269530706027,-13.1588672637238,
54.9890950393045));
#126138=CARTESIAN_POINT('Ctrl Pts',(-2.00845697777614,-13.4615457509614,
54.9885375937375));
#126139=CARTESIAN_POINT('Ctrl Pts',(-1.94157305345321,-13.7658810338058,
54.9890823794828));
#126140=CARTESIAN_POINT('Ctrl Pts',(-1.87208962015349,-14.0716870597456,
54.9910178180691));
#126141=CARTESIAN_POINT('Ctrl Pts',(-1.85651589013135,-14.1402291605164,
54.9914516192874));
#126142=CARTESIAN_POINT('Ctrl Pts',(-1.8408114204113,-14.2088450198168,
54.991955403005));
#126143=CARTESIAN_POINT('Ctrl Pts',(-1.82497643282323,-14.2775323299277,
54.9925326544939));
#126144=CARTESIAN_POINT('Ctrl Pts',(-1.78082973392649,-14.4690271435882,
54.9941419862047));
#126145=CARTESIAN_POINT('Ctrl Pts',(-1.735666691271,-14.6610810017041,54.9963214523107));
#126146=CARTESIAN_POINT('Ctrl Pts',(-1.68945916723778,-14.8536488722862,
54.9991469932073));
#126147=CARTESIAN_POINT('Ctrl Pts',(-1.64325164320455,-15.0462167428683,
55.001972534104));
#126148=CARTESIAN_POINT('Ctrl Pts',(-1.59599946347008,-15.2392990217843,
55.0054438945215));
#126149=CARTESIAN_POINT('Ctrl Pts',(-1.54769772308862,-15.4328022255565,
55.0096508046892));
#126150=CARTESIAN_POINT('Ctrl Pts',(-1.53176134994561,-15.4966454584365,
55.0110388062329));
#126151=CARTESIAN_POINT('Ctrl Pts',(-1.51571096741508,-15.5605340258221,
55.0125070139342));
#126152=CARTESIAN_POINT('Ctrl Pts',(-1.49954709930578,-15.6244654940096,
55.0140584675908));
#126153=CARTESIAN_POINT('Ctrl Pts',(-1.47759392156854,-15.7112948887208,
55.0161655955163));
#126154=CARTESIAN_POINT('Ctrl Pts',(-1.45543143911073,-15.798203392864,
55.0184262598809));
#126155=CARTESIAN_POINT('Ctrl Pts',(-1.43306031387933,-15.8851854425692,
55.0208484533193));
#126156=CARTESIAN_POINT('Ctrl Pts',(-1.42187475126362,-15.9286764674218,
55.0220595500385));
#126157=CARTESIAN_POINT('Ctrl Pts',(-1.41063702858815,-15.9721858786649,
55.0233110347678));
#126158=CARTESIAN_POINT('Ctrl Pts',(-1.39934713818154,-16.0157130538162,
55.0246039542798));
#126159=CARTESIAN_POINT('Ctrl Pts',(-1.39370219297824,-16.0374766413918,
55.0252504140358));
#126160=CARTESIAN_POINT('Ctrl Pts',(-1.38804420588604,-16.0592446699445,
55.0259072329045));
#126161=CARTESIAN_POINT('Ctrl Pts',(-1.38237317309397,-16.0810170640224,
55.0265745446507));
#126162=CARTESIAN_POINT('Ctrl Pts',(-1.37953765669793,-16.0919032610614,
55.0269082005238));
#126163=CARTESIAN_POINT('Ctrl Pts',(-1.37669887888011,-16.1027905494816,
55.0272444796433));
#126164=CARTESIAN_POINT('Ctrl Pts',(-1.3738568388251,-16.113678920125,55.027583398937));
#126165=CARTESIAN_POINT('Ctrl Pts',(-1.37101479877008,-16.1245672907683,
55.0279223182307));
#126166=CARTESIAN_POINT('Ctrl Pts',(-1.36865251609714,-16.133610081709,
55.0282055102779));
#126167=CARTESIAN_POINT('Ctrl Pts',(-1.36532093103418,-16.1463472696511,
55.0286080943937));
#126168=CARTESIAN_POINT('Ctrl Pts',(-1.32033570854725,-16.3183330429714,
55.0340440462533));
#126169=CARTESIAN_POINT('Ctrl Pts',(-1.27477572945593,-16.4896151849966,
55.040113685044));
#126170=CARTESIAN_POINT('Ctrl Pts',(-1.22867726285142,-16.6601973448782,
55.0468623692584));
#126171=CARTESIAN_POINT('Ctrl Pts',(-1.16978974220244,-16.8781039522402,
55.0554833345595));
#126172=CARTESIAN_POINT('Ctrl Pts',(-1.11001923437359,-17.0948742436374,
55.0652120839941));
#126173=CARTESIAN_POINT('Ctrl Pts',(-1.04940924672357,-17.3104263127349,
55.0761380260064));
#126174=CARTESIAN_POINT('Ctrl Pts',(-0.988799259073545,-17.5259783818323,
55.0870639680186));
#126175=CARTESIAN_POINT('Ctrl Pts',(-0.927349920031676,-17.7403122086757,
55.0991866017856));
#126176=CARTESIAN_POINT('Ctrl Pts',(-0.865126498396156,-17.9532975613375,
55.1126099267491));
#126177=CARTESIAN_POINT('Ctrl Pts',(-0.861262891894302,-17.9665223498771,
55.1134434142727));
#126178=CARTESIAN_POINT('Ctrl Pts',(-0.857396307508481,-17.9797419240376,
55.1142819226883));
#126179=CARTESIAN_POINT('Ctrl Pts',(-0.853526763430693,-17.9929562465901,
55.1151254794357));
#126180=CARTESIAN_POINT('Ctrl Pts',(-0.828492501792921,-18.0784471471962,
55.1205829234907));
#126181=CARTESIAN_POINT('Ctrl Pts',(-0.803334389201592,-18.163718240567,
55.1262516375727));
#126182=CARTESIAN_POINT('Ctrl Pts',(-0.778057158148713,-18.248764113097,
55.1321368969883));
#126183=CARTESIAN_POINT('Ctrl Pts',(-0.763464992700593,-18.2978598166588,
55.1355343687651));
#126184=CARTESIAN_POINT('Ctrl Pts',(-0.748833131789826,-18.3468804357216,
55.1390040107368));
#126185=CARTESIAN_POINT('Ctrl Pts',(-0.734162426679192,-18.3958249557652,
55.1425469019139));
#126186=CARTESIAN_POINT('Ctrl Pts',(-0.726827074123874,-18.4202972157869,
55.1443183475024));
#126187=CARTESIAN_POINT('Ctrl Pts',(-0.719482010669794,-18.4447504510539,
55.1461081059892));
#126188=CARTESIAN_POINT('Ctrl Pts',(-0.712127340211664,-18.4691845275153,
55.1479163168723));
#126189=CARTESIAN_POINT('Ctrl Pts',(-0.706611337368068,-18.4875100848613,
55.1492724750347));
#126190=CARTESIAN_POINT('Ctrl Pts',(-0.701089930596245,-18.5058248653791,
55.150639012722));
#126191=CARTESIAN_POINT('Ctrl Pts',(-0.695563163090249,-18.5241288135701,
55.1520159900027));
#126192=CARTESIAN_POINT('Ctrl Pts',(-0.693720907254918,-18.5302301296337,
55.1524749824295));
#126193=CARTESIAN_POINT('Ctrl Pts',(-0.692327278617444,-18.5348440206536,
55.1528227186659));
#126194=CARTESIAN_POINT('Ctrl Pts',(-0.690034610190422,-18.5424291489228,
55.1533964494393));
#126195=CARTESIAN_POINT('Ctrl Pts',(-0.614956638884621,-18.7908192064774,
55.1721844006473));
#126196=CARTESIAN_POINT('Ctrl Pts',(-0.539153626642809,-19.0361926767024,
55.1928330519685));
#126197=CARTESIAN_POINT('Ctrl Pts',(-0.462786056000691,-19.2784783689272,
55.2154576486142));
#126198=CARTESIAN_POINT('Ctrl Pts',(-0.44434194325563,-19.336994628988,
55.2209218870054));
#126199=CARTESIAN_POINT('Ctrl Pts',(-0.425864730362313,-19.3953308171107,
55.2265015432689));
#126200=CARTESIAN_POINT('Ctrl Pts',(-0.407356350425952,-19.4534860061815,
55.2321985735646));
#126201=CARTESIAN_POINT('Ctrl Pts',(-0.328708790148578,-19.7006045413324,
55.2564069340542));
#126202=CARTESIAN_POINT('Ctrl Pts',(-0.249496603748653,-19.9444575557464,
55.2827320599704));
#126203=CARTESIAN_POINT('Ctrl Pts',(-0.169859166644958,-20.18488117157,
55.311268127787));
#126204=CARTESIAN_POINT('Ctrl Pts',(-0.09455233110252,-20.4122307995318,
55.3382524337146));
#126205=CARTESIAN_POINT('Ctrl Pts',(-0.0188656993732753,-20.6365133872874,
55.367212997343));
#126206=CARTESIAN_POINT('Ctrl Pts',(0.0570693465599587,-20.8575662264015,
55.3982676679193));
#126207=CARTESIAN_POINT('Ctrl Pts',(0.0757505374372732,-20.9119486295556,
55.4059075951958));
#126208=CARTESIAN_POINT('Ctrl Pts',(0.0944467137683982,-20.9661354554094,
55.4136744827716));
#126209=CARTESIAN_POINT('Ctrl Pts',(0.113155831545745,-21.0201240906044,
55.421570535909));
#126210=CARTESIAN_POINT('Ctrl Pts',(0.146987875206053,-21.1177527380272,
55.4358491148174));
#126211=CARTESIAN_POINT('Ctrl Pts',(0.180862205655314,-21.2147333141768,
55.4505500132441));
#126212=CARTESIAN_POINT('Ctrl Pts',(0.214763979944339,-21.3110511932278,
55.4656743286618));
#126213=CARTESIAN_POINT('Origin',(-10.9843331791359,-92.5,80.581991049076));
#126214=CARTESIAN_POINT('',(0.214770326079967,-21.31105119265,55.4656600933121));
#126215=CARTESIAN_POINT('Origin',(-2.02513312664091,-89.,60.48888938658));
#126216=CARTESIAN_POINT('',(-7.08815755064836,-89.,58.3404518887897));
#126217=CARTESIAN_POINT('Origin',(-2.02513312664091,-89.,60.48888938658));
#126218=CARTESIAN_POINT('',(-5.70733025545361,-90.4999999999959,58.9263904268899));
#126219=CARTESIAN_POINT('Origin',(-5.70733270705591,-89.,58.92638938658));
#126220=CARTESIAN_POINT('Origin',(-2.02513312664091,-90.49999999999,60.48888938658));
#126221=CARTESIAN_POINT('Origin',(-2.27593483123091,-90.5,69.192338555332));
#126222=CARTESIAN_POINT('',(-5.70733025554977,-90.4999999999959,87.0513883463108));
#126223=CARTESIAN_POINT('Origin',(27.4324635166691,-90.5,72.98888938658));
#126224=CARTESIAN_POINT('Origin',(-2.02513312664091,-90.49999999999,85.48888938658));
#126225=CARTESIAN_POINT('Origin',(-2.02513312664091,-89.,85.48888938658));
#126226=CARTESIAN_POINT('',(-7.08815755202979,-89.,87.6373268811148));
#126227=CARTESIAN_POINT('Origin',(-5.70733270705591,-89.,87.05138938658));
#126228=CARTESIAN_POINT('Origin',(-2.02513312664091,-89.,85.48888938658));
#126229=CARTESIAN_POINT('Origin',(-2.02513312664091,-92.5,85.48888938658));
#126230=CARTESIAN_POINT('',(-7.08838180624485,-85.174012662148,87.6374220205403));
#126231=CARTESIAN_POINT('',(-7.08815755434906,25.,87.6373268756495));
#126232=CARTESIAN_POINT('Ctrl Pts',(-7.08838180624485,-85.174012662148,
87.6374220205403));
#126233=CARTESIAN_POINT('Ctrl Pts',(-7.06379631478045,-84.9618158750809,
87.6953760007039));
#126234=CARTESIAN_POINT('Ctrl Pts',(-7.03898074672462,-84.748459068266,
87.7510083865588));
#126235=CARTESIAN_POINT('Ctrl Pts',(-7.01416074376767,-84.5339843926944,
87.8044020256059));
#126236=CARTESIAN_POINT('Ctrl Pts',(-6.98859134290818,-84.3130340179738,
87.8594077950456));
#126237=CARTESIAN_POINT('Ctrl Pts',(-6.96301669278039,-84.0908972668471,
87.9120376933239));
#126238=CARTESIAN_POINT('Ctrl Pts',(-6.93764503641729,-83.8675829154453,
87.9623644050187));
#126239=CARTESIAN_POINT('Ctrl Pts',(-6.91121161522479,-83.6349232016113,
88.0147972122593));
#126240=CARTESIAN_POINT('Ctrl Pts',(-6.88499796602311,-83.400985352606,
88.0647302007003));
#126241=CARTESIAN_POINT('Ctrl Pts',(-6.85920704409652,-83.1657384765946,
88.1122242130556));
#126242=CARTESIAN_POINT('Ctrl Pts',(-6.85103788991991,-83.0912251263091,
88.1272677198562));
#126243=CARTESIAN_POINT('Ctrl Pts',(-6.84291094610431,-83.0165801426965,
88.1420663642715));
#126244=CARTESIAN_POINT('Ctrl Pts',(-6.83483216441449,-82.9418017191346,
88.1566216159116));
#126245=CARTESIAN_POINT('Ctrl Pts',(-6.82950767478839,-82.8925174389302,
88.1662145581817));
#126246=CARTESIAN_POINT('Ctrl Pts',(-6.82420410061484,-82.8431751901153,
88.1757017737205));
#126247=CARTESIAN_POINT('Ctrl Pts',(-6.81892303812862,-82.7937759979044,
88.185084240871));
#126248=CARTESIAN_POINT('Ctrl Pts',(-6.79460184830759,-82.5662749725138,
88.2282938724841));
#126249=CARTESIAN_POINT('Ctrl Pts',(-6.77075938383651,-82.3375651317986,
88.2692827739492));
#126250=CARTESIAN_POINT('Ctrl Pts',(-6.74754396638005,-82.1076627398156,
88.3081343431746));
#126251=CARTESIAN_POINT('Ctrl Pts',(-6.7295030810263,-81.929003764413,88.3383262062985));
#126252=CARTESIAN_POINT('Ctrl Pts',(-6.71184063768807,-81.7496235979736,
88.3672266692105));
#126253=CARTESIAN_POINT('Ctrl Pts',(-6.69462624070162,-81.5695127023199,
88.3948617495597));
#126254=CARTESIAN_POINT('Ctrl Pts',(-6.67494310539971,-81.3635718766673,
88.4264600115273));
#126255=CARTESIAN_POINT('Ctrl Pts',(-6.65584272326395,-81.1566825793778,
88.4564089810734));
#126256=CARTESIAN_POINT('Ctrl Pts',(-6.63741409551801,-80.9488448097589,
88.4847575516344));
#126257=CARTESIAN_POINT('Ctrl Pts',(-6.62819978164503,-80.8449259249494,
88.4989318369149));
#126258=CARTESIAN_POINT('Ctrl Pts',(-6.61915331092193,-80.740769922046,
88.5127059616475));
#126259=CARTESIAN_POINT('Ctrl Pts',(-6.61028508149103,-80.6363768009134,
88.526086081745));
#126260=CARTESIAN_POINT('Ctrl Pts',(-6.60585096677558,-80.5841802403472,
88.5327761417938));
#126261=CARTESIAN_POINT('Ctrl Pts',(-6.6014614077024,-80.5319244002237,
88.5393676980408));
#126262=CARTESIAN_POINT('Ctrl Pts',(-6.59711767521138,-80.479609280531,
88.5458615114224));
#126263=CARTESIAN_POINT('Ctrl Pts',(-6.59494580896587,-80.4534517206847,
88.5491084181132));
#126264=CARTESIAN_POINT('Ctrl Pts',(-6.5927853991295,-80.4272793409462,
88.5523308889536));
#126265=CARTESIAN_POINT('Ctrl Pts',(-6.59063660249566,-80.4010921413147,
88.5555290194189));
#126266=CARTESIAN_POINT('Ctrl Pts',(-6.58848780586183,-80.3749049416833,
88.5587271498841));
#126267=CARTESIAN_POINT('Ctrl Pts',(-6.58644354173115,-80.3498490744125,
88.561763247515));
#126268=CARTESIAN_POINT('Ctrl Pts',(-6.58422520796802,-80.3224860827418,
88.5650504850222));
#126269=CARTESIAN_POINT('Ctrl Pts',(-6.5641013055288,-80.0742591549545,
88.594871086408));
#126270=CARTESIAN_POINT('Ctrl Pts',(-6.54513483205179,-79.8256135763339,
88.622367628329));
#126271=CARTESIAN_POINT('Ctrl Pts',(-6.52746563345973,-79.5765104364289,
88.6476204732732));
#126272=CARTESIAN_POINT('Ctrl Pts',(-6.51570540126308,-79.410712833842,
88.6644282146444));
#126273=CARTESIAN_POINT('Ctrl Pts',(-6.50452000859505,-79.2447115819987,
88.6802414043915));
#126274=CARTESIAN_POINT('Ctrl Pts',(-6.49395442975159,-79.0784852886401,
88.6950766706492));
#126275=CARTESIAN_POINT('Ctrl Pts',(-6.47849511246648,-78.8352667155519,
88.7167832985099));
#126276=CARTESIAN_POINT('Ctrl Pts',(-6.46436081725034,-78.5915678258629,
88.7363976088991));
#126277=CARTESIAN_POINT('Ctrl Pts',(-6.45152907111565,-78.3474341596224,
88.7540024507364));
#126278=CARTESIAN_POINT('Ctrl Pts',(-6.43850088405651,-78.099563056358,
88.7718768047171));
#126279=CARTESIAN_POINT('Ctrl Pts',(-6.42681516618875,-77.8512432568754,
88.787679653157));
#126280=CARTESIAN_POINT('Ctrl Pts',(-6.41648321794231,-77.6024927608509,
88.8014696460193));
#126281=CARTESIAN_POINT('Ctrl Pts',(-6.4060523720161,-77.3513612185502,
88.8153916370552));
#126282=CARTESIAN_POINT('Ctrl Pts',(-6.3970010649043,-77.0997901362597,
88.8272620102371));
#126283=CARTESIAN_POINT('Ctrl Pts',(-6.38938018142158,-76.8477761615928,
88.8371134105489));
#126284=CARTESIAN_POINT('Ctrl Pts',(-6.38178064370192,-76.5964680671039,
88.8469372175172));
#126285=CARTESIAN_POINT('Ctrl Pts',(-6.37560331098471,-76.3447189675036,
88.8547532740801));
#126286=CARTESIAN_POINT('Ctrl Pts',(-6.37094103456924,-76.0925125845702,
88.8605674847034));
#126287=CARTESIAN_POINT('Ctrl Pts',(-6.3663487990775,-75.8440950735223,
88.8662943490076));
#126288=CARTESIAN_POINT('Ctrl Pts',(-6.36322629828271,-75.5952333553235,
88.870078969759));
#126289=CARTESIAN_POINT('Ctrl Pts',(-6.36170597022165,-75.345907828253,
88.8719025711441));
#126290=CARTESIAN_POINT('Ctrl Pts',(-6.36100416191559,-75.2308150859092,
88.8727443753782));
#126291=CARTESIAN_POINT('Ctrl Pts',(-6.36064438933148,-75.1156235047724,
88.8731679708493));
#126292=CARTESIAN_POINT('Ctrl Pts',(-6.36064303502447,-75.0003313582817,
88.8731697877795));
#126293=CARTESIAN_POINT('Ctrl Pts',(-6.36064303474443,-75.0003075183965,
88.8731697881552));
#126294=CARTESIAN_POINT('Ctrl Pts',(-6.36064303447919,-75.0002836785154,
88.8731697885135));
#126295=CARTESIAN_POINT('Ctrl Pts',(-6.36064303422876,-75.0002598386384,
88.8731697888545));
#126296=CARTESIAN_POINT('Ctrl Pts',(-6.36064040478154,-74.749954905453,
88.873173369011));
#126297=CARTESIAN_POINT('Ctrl Pts',(-6.36226546725732,-74.5001035131016,
88.8712654272117));
#126298=CARTESIAN_POINT('Ctrl Pts',(-6.36540095128621,-74.2506871861409,
88.8674288772245));
#126299=CARTESIAN_POINT('Ctrl Pts',(-6.36856865307248,-73.9987080540005,
88.8635529058799));
#126300=CARTESIAN_POINT('Ctrl Pts',(-6.37327831247089,-73.7471724121695,
88.8577085442994));
#126301=CARTESIAN_POINT('Ctrl Pts',(-6.37945535068582,-73.4960730086243,
88.8498538881179));
#126302=CARTESIAN_POINT('Ctrl Pts',(-6.38565345904744,-73.2441170940647,
88.8419724393617));
#126303=CARTESIAN_POINT('Ctrl Pts',(-6.39332933367653,-72.9925998472497,
88.8320670081214));
#126304=CARTESIAN_POINT('Ctrl Pts',(-6.40244871597262,-72.7415341444287,
88.8200701793989));
#126305=CARTESIAN_POINT('Ctrl Pts',(-6.40753807971511,-72.6014188774695,
88.8133749644004));
#126306=CARTESIAN_POINT('Ctrl Pts',(-6.41307773369852,-72.4614446543939,
88.8060279205458));
#126307=CARTESIAN_POINT('Ctrl Pts',(-6.41906664530995,-72.3216174025011,
88.7980138504433));
#126308=CARTESIAN_POINT('Ctrl Pts',(-6.42961412702571,-72.0753580688533,
88.7838997236438));
#126309=CARTESIAN_POINT('Ctrl Pts',(-6.44153217487,-71.8295371924908,88.7677456148225));
#126310=CARTESIAN_POINT('Ctrl Pts',(-6.45477307066889,-71.5841478194717,
88.749542707656));
#126311=CARTESIAN_POINT('Ctrl Pts',(-6.46538522433686,-71.3874761006909,
88.7349536608884));
#126312=CARTESIAN_POINT('Ctrl Pts',(-6.4768478731557,-71.1910816029631,
88.7190480585771));
#126313=CARTESIAN_POINT('Ctrl Pts',(-6.48915450788134,-70.9949691674386,
88.7018075585331));
#126314=CARTESIAN_POINT('Ctrl Pts',(-6.49071134690436,-70.9701601518685,
88.6996265656099));
#126315=CARTESIAN_POINT('Ctrl Pts',(-6.49228157490731,-70.9453555172984,
88.6974243856275));
#126316=CARTESIAN_POINT('Ctrl Pts',(-6.4938652542253,-70.9205553918243,
88.6952008885181));
#126317=CARTESIAN_POINT('Ctrl Pts',(-6.50635089886465,-70.7250325039749,
88.6776709539853));
#126318=CARTESIAN_POINT('Ctrl Pts',(-6.51967225333885,-70.5297886023269,
88.6588166712615));
#126319=CARTESIAN_POINT('Ctrl Pts',(-6.53376669716175,-70.3348221400914,
88.6385974917835));
#126320=CARTESIAN_POINT('Ctrl Pts',(-6.54170778878621,-70.2249741347525,
88.627205601559));
#126321=CARTESIAN_POINT('Ctrl Pts',(-6.54989441621222,-70.1152143819194,
88.6153802361868));
#126322=CARTESIAN_POINT('Ctrl Pts',(-6.55831520320439,-70.0055428830087,
88.6031139835115));
#126323=CARTESIAN_POINT('Ctrl Pts',(-6.56252559670048,-69.9507071335534,
88.5969808571739));
#126324=CARTESIAN_POINT('Ctrl Pts',(-6.56679452679293,-69.8958934475535,
88.5907375074315));
#126325=CARTESIAN_POINT('Ctrl Pts',(-6.57112054094054,-69.8411018250717,
88.5843830071542));
#126326=CARTESIAN_POINT('Ctrl Pts',(-6.57328354801434,-69.8137060138308,
88.5812057570156));
#126327=CARTESIAN_POINT('Ctrl Pts',(-6.57546082583398,-69.7863157184686,
88.5780007191089));
#126328=CARTESIAN_POINT('Ctrl Pts',(-6.57765219046004,-69.7589309389883,
88.574767777654));
#126329=CARTESIAN_POINT('Ctrl Pts',(-6.5798435550861,-69.7315461595081,
88.5715348361991));
#126330=CARTESIAN_POINT('Ctrl Pts',(-6.58214338518519,-69.7030028197464,
88.5681341312207));
#126331=CARTESIAN_POINT('Ctrl Pts',(-6.58426835938578,-69.6767931481951,
88.5649851265532));
#126332=CARTESIAN_POINT('Ctrl Pts',(-6.60448470513764,-69.4274424586774,
88.5350264724128));
#126333=CARTESIAN_POINT('Ctrl Pts',(-6.62580950443919,-69.1794547193134,
88.5028101608645));
#126334=CARTESIAN_POINT('Ctrl Pts',(-6.64806081890539,-68.9327838372194,
88.4683145058022));
#126335=CARTESIAN_POINT('Ctrl Pts',(-6.66995243203797,-68.6901004878794,
88.434376486701));
#126336=CARTESIAN_POINT('Ctrl Pts',(-6.69274146521221,-68.4486914334156,
88.3982322076366));
#126337=CARTESIAN_POINT('Ctrl Pts',(-6.71626520022788,-68.2085505509096,
88.3598306420088));
#126338=CARTESIAN_POINT('Ctrl Pts',(-6.73899437491936,-67.9765208980757,
88.3227261646374));
#126339=CARTESIAN_POINT('Ctrl Pts',(-6.76240999994988,-67.7456750207067,
88.2835142412598));
#126340=CARTESIAN_POINT('Ctrl Pts',(-6.78636679563562,-67.5160464093315,
88.242121012596));
#126341=CARTESIAN_POINT('Ctrl Pts',(-6.80235411105814,-67.3628061726886,
88.2144976771682));
#126342=CARTESIAN_POINT('Ctrl Pts',(-6.81858245485541,-67.2101088308579,
88.1859023530971));
#126343=CARTESIAN_POINT('Ctrl Pts',(-6.8350072566281,-67.0579751615403,
88.1563059844045));
#126344=CARTESIAN_POINT('Ctrl Pts',(-6.85993106443988,-66.8271199957825,
88.1113949884954));
#126345=CARTESIAN_POINT('Ctrl Pts',(-6.8853085719417,-66.5975613278129,
88.0641797110285));
#126346=CARTESIAN_POINT('Ctrl Pts',(-6.91096401058241,-66.3692379839661,
88.0146005159368));
#126347=CARTESIAN_POINT('Ctrl Pts',(-6.9359277552185,-66.1470704455322,
87.9663580211244));
#126348=CARTESIAN_POINT('Ctrl Pts',(-6.96115522877894,-65.9260725236057,
87.9158772269839));
#126349=CARTESIAN_POINT('Ctrl Pts',(-6.98645999388353,-65.7062244363269,
87.8630827857479));
#126350=CARTESIAN_POINT('Ctrl Pts',(-7.01070555469572,-65.4955787279977,
87.8124982088809));
#126351=CARTESIAN_POINT('Ctrl Pts',(-7.03502249709539,-65.2859887012326,
87.7597894706709));
#126352=CARTESIAN_POINT('Ctrl Pts',(-7.05921693797329,-65.077470153448,
87.7048733754824));
#126353=CARTESIAN_POINT('Ctrl Pts',(-7.06896378908785,-64.9934674170285,
87.6827501527844));
#126354=CARTESIAN_POINT('Ctrl Pts',(-7.07869037563948,-64.9096389534572,
87.6602685078946));
#126355=CARTESIAN_POINT('Ctrl Pts',(-7.08838231939817,-64.8259873690431,
87.6374222559034));
#126356=CARTESIAN_POINT('Origin',(-2.02513312664091,25.,60.48888938658));
#126357=CARTESIAN_POINT('',(-6.36087450269922,-74.999999801042,57.1044283173086));
#126358=CARTESIAN_POINT('Ctrl Pts',(-7.08825603872491,-64.825987319,58.34041012264));
#126359=CARTESIAN_POINT('Ctrl Pts',(-6.99794665049256,-65.6045290148126,
58.1278601811754));
#126360=CARTESIAN_POINT('Ctrl Pts',(-6.9052605176683,-66.3985891148802,
57.94616482494));
#126361=CARTESIAN_POINT('Ctrl Pts',(-6.77559174784533,-67.6129568713641,
57.7156393481809));
#126362=CARTESIAN_POINT('Ctrl Pts',(-6.73388211710599,-68.0216257245892,
57.6457863578687));
#126363=CARTESIAN_POINT('Ctrl Pts',(-6.67482143432723,-68.6404484060224,
57.5508991529112));
#126364=CARTESIAN_POINT('Ctrl Pts',(-6.64616303810798,-68.9513145971379,
57.5059287097987));
#126365=CARTESIAN_POINT('Ctrl Pts',(-6.6144832189235,-69.3165378083041,
57.457666220138));
#126366=CARTESIAN_POINT('Ctrl Pts',(-6.60130426161773,-69.4736076105606,
57.4378700643154));
#126367=CARTESIAN_POINT('Ctrl Pts',(-6.59260914456376,-69.5784420495982,
57.4248685010235));
#126368=CARTESIAN_POINT('Ctrl Pts',(-6.58847553231003,-69.6288394451349,
57.4187153470913));
#126369=CARTESIAN_POINT('Ctrl Pts',(-6.44248193445931,-71.4312631171058,
57.202390535774));
#126370=CARTESIAN_POINT('Ctrl Pts',(-6.36088862142065,-73.2034436053334,
57.1049235992306));
#126371=CARTESIAN_POINT('Ctrl Pts',(-6.36082055131842,-74.9999998096187,
57.1044704220667));
#126372=CARTESIAN_POINT('',(-7.08824189517591,-85.17401265925,58.3404161122));
#126373=CARTESIAN_POINT('Ctrl Pts',(-6.36082055131591,-74.99999987577,57.10447042205));
#126374=CARTESIAN_POINT('Ctrl Pts',(-6.36078005345576,-75.8984830421777,
57.104784515926));
#126375=CARTESIAN_POINT('Ctrl Pts',(-6.38054797589447,-76.7906363769049,
57.1296675300475));
#126376=CARTESIAN_POINT('Ctrl Pts',(-6.43768917687825,-78.1193716314746,
57.2055448111296));
#126377=CARTESIAN_POINT('Ctrl Pts',(-6.46127749702327,-78.5607009250776,
57.2372938612818));
#126378=CARTESIAN_POINT('Ctrl Pts',(-6.50284708023062,-79.220321178602,
57.2950452555082));
#126379=CARTESIAN_POINT('Ctrl Pts',(-6.52517453823015,-79.5495378836441,
57.3264553750152));
#126380=CARTESIAN_POINT('Ctrl Pts',(-6.55374130281479,-79.9325855515165,
57.3676563681427));
#126381=CARTESIAN_POINT('Ctrl Pts',(-6.56650133766688,-80.0965263046025,
57.3863044363751));
#126382=CARTESIAN_POINT('Ctrl Pts',(-6.5751203655941,-80.2057706881831,
57.3989582017931));
#126383=CARTESIAN_POINT('Ctrl Pts',(-6.57964866975663,-80.2623756631579,
57.4056368678187));
#126384=CARTESIAN_POINT('Ctrl Pts',(-6.72015992204332,-81.9970282825598,
57.6138171149191));
#126385=CARTESIAN_POINT('Ctrl Pts',(-6.90771485277002,-83.6167188709601,
57.9152192285855));
#126386=CARTESIAN_POINT('Ctrl Pts',(-7.08824189517591,-85.17401265925,58.3404161122));
#126387=CARTESIAN_POINT('',(-7.08815755158619,25.,58.3404518909995));
#126388=CARTESIAN_POINT('Origin',(27.4324635166691,25.,72.98888938658));
#126389=CARTESIAN_POINT('',(-8.15021171484832,-89.0000000007984,61.1515796381337));
#126390=CARTESIAN_POINT('Ctrl Pts',(-7.08815755570517,-85.17401265925,58.3404519007063));
#126391=CARTESIAN_POINT('Ctrl Pts',(-7.17009088674586,-85.5332934006639,
58.5335366223212));
#126392=CARTESIAN_POINT('Ctrl Pts',(-7.25466994278313,-85.8832477134225,
58.7373493420429));
#126393=CARTESIAN_POINT('Ctrl Pts',(-7.34134732186451,-86.2238755975257,
58.9520777911399));
#126394=CARTESIAN_POINT('Ctrl Pts',(-7.38468601140521,-86.3941895395773,
59.0594420156884));
#126395=CARTESIAN_POINT('Ctrl Pts',(-7.42854839638355,-86.5621718744651,
59.1695353419165));
#126396=CARTESIAN_POINT('Ctrl Pts',(-7.47286045458535,-86.727822602189,
59.2823814993839));
#126397=CARTESIAN_POINT('Ctrl Pts',(-7.49501648368625,-86.8106479660509,
59.3388045781176));
#126398=CARTESIAN_POINT('Ctrl Pts',(-7.51728487970092,-86.8928904281219,
59.395915884714));
#126399=CARTESIAN_POINT('Ctrl Pts',(-7.53965601887953,-86.974549988402,
59.4537183425445));
#126400=CARTESIAN_POINT('Ctrl Pts',(-7.56202715805814,-87.056209548682,
59.5115208003749));
#126401=CARTESIAN_POINT('Ctrl Pts',(-7.58475892257956,-87.1382060307662,
59.5706907776505));
#126402=CARTESIAN_POINT('Ctrl Pts',(-7.6070678306237,-87.2177799638692,
59.6292021536361));
#126403=CARTESIAN_POINT('Ctrl Pts',(-7.69754835975279,-87.5405161353482,
59.8665127494201));
#126404=CARTESIAN_POINT('Ctrl Pts',(-7.78908991439444,-87.8523241301438,
60.1138381553492));
#126405=CARTESIAN_POINT('Ctrl Pts',(-7.88109427946115,-88.1532039481646,
60.371336700763));
#126406=CARTESIAN_POINT('Ctrl Pts',(-7.97056691853573,-88.4458043192783,
60.6217495414943));
#126407=CARTESIAN_POINT('Ctrl Pts',(-8.06047707269029,-88.7280696699181,
60.8817836000023));
#126408=CARTESIAN_POINT('Ctrl Pts',(-8.15022843089587,-89.,61.15157407589));
#126409=CARTESIAN_POINT('Origin',(27.4324635166691,-89.,72.98888938658));
#126410=CARTESIAN_POINT('Origin',(27.4324635166691,-89.,72.98888938658));
#126411=CARTESIAN_POINT('',(-9.69875398068591,-89.98547710816,72.9888884257558));
#126412=CARTESIAN_POINT('Ctrl Pts',(-8.15021171484831,-89.0000000007984,
61.1515796381337));
#126413=CARTESIAN_POINT('Ctrl Pts',(-8.18209401555367,-89.016084121901,
61.247394756252));
#126414=CARTESIAN_POINT('Ctrl Pts',(-8.21351914995864,-89.0320746553665,
61.3439406457586));
#126415=CARTESIAN_POINT('Ctrl Pts',(-8.24446559888565,-89.0479569881628,
61.441196198803));
#126416=CARTESIAN_POINT('Ctrl Pts',(-8.29197525924787,-89.0723398903396,
61.5905050356386));
#126417=CARTESIAN_POINT('Ctrl Pts',(-8.33835843912484,-89.0964700937086,
61.7414879393347));
#126418=CARTESIAN_POINT('Ctrl Pts',(-8.38362243092968,-89.1203436093358,
61.8941276178605));
#126419=CARTESIAN_POINT('Ctrl Pts',(-8.42888642273451,-89.1442171249629,
62.0467672963862));
#126420=CARTESIAN_POINT('Ctrl Pts',(-8.47303075616557,-89.1678336747818,
62.2010637343623));
#126421=CARTESIAN_POINT('Ctrl Pts',(-8.51603088739236,-89.1911430500894,
62.3569811977979));
#126422=CARTESIAN_POINT('Ctrl Pts',(-8.54388046912763,-89.2062396633859,
62.4579631254809));
#126423=CARTESIAN_POINT('Ctrl Pts',(-8.57124991958204,-89.2212197737176,
62.55963207447));
#126424=CARTESIAN_POINT('Ctrl Pts',(-8.59812340744795,-89.2360643190087,
62.6619701173454));
#126425=CARTESIAN_POINT('Ctrl Pts',(-8.62625664141202,-89.2516047307279,
62.7691054515457));
#126426=CARTESIAN_POINT('Ctrl Pts',(-8.65384642235063,-89.2669966465503,
62.8769743529093));
#126427=CARTESIAN_POINT('Ctrl Pts',(-8.68089332036743,-89.282247619279,
62.9855784771597));
#126428=CARTESIAN_POINT('Ctrl Pts',(-8.70733466723629,-89.2971571390234,
63.0917510711077));
#126429=CARTESIAN_POINT('Ctrl Pts',(-8.73325657894745,-89.3119259141199,
63.1986202964528));
#126430=CARTESIAN_POINT('Ctrl Pts',(-8.7586549986539,-89.3265499257272,
63.3061769093053));
#126431=CARTESIAN_POINT('Ctrl Pts',(-8.77135420850712,-89.3338619315309,
63.3599552157315));
#126432=CARTESIAN_POINT('Ctrl Pts',(-8.7839224900317,-89.3411377408504,
63.4139053859424));
#126433=CARTESIAN_POINT('Ctrl Pts',(-8.79635897506002,-89.3483768140945,
63.4680263665213));
#126434=CARTESIAN_POINT('Ctrl Pts',(-8.80504617371202,-89.353433489448,
63.5058312373075));
#126435=CARTESIAN_POINT('Ctrl Pts',(-8.8135248704471,-89.3583844131764,
63.5430801157702));
#126436=CARTESIAN_POINT('Ctrl Pts',(-8.82209708340818,-89.3634146593055,
63.5811113108075));
#126437=CARTESIAN_POINT('Ctrl Pts',(-8.82579674339726,-89.365585650673,
63.5975250993187));
#126438=CARTESIAN_POINT('Ctrl Pts',(-8.82951373013669,-89.3677709458225,
63.6140850461936));
#126439=CARTESIAN_POINT('Ctrl Pts',(-8.83327191475055,-89.369983233208,
63.6309007518484));
#126440=CARTESIAN_POINT('Ctrl Pts',(-8.8572936644153,-89.3841238407679,
63.7383842081388));
#126441=CARTESIAN_POINT('Ctrl Pts',(-8.88059574867455,-89.3979965883317,
63.8456211319469));
#126442=CARTESIAN_POINT('Ctrl Pts',(-8.9031979127015,-89.41159584742,63.9525808563939));
#126443=CARTESIAN_POINT('Ctrl Pts',(-8.93881407811077,-89.4330253645474,
64.1211264537753));
#126444=CARTESIAN_POINT('Ctrl Pts',(-8.97269344987008,-89.4537784137391,
64.2889863577911));
#126445=CARTESIAN_POINT('Ctrl Pts',(-9.00495691259786,-89.4738783490184,
64.456129214163));
#126446=CARTESIAN_POINT('Ctrl Pts',(-9.03722037532564,-89.4939782842977,
64.623272070535));
#126447=CARTESIAN_POINT('Ctrl Pts',(-9.067867221227,-89.5134242699625,64.7896971699235));
#126448=CARTESIAN_POINT('Ctrl Pts',(-9.09700654351357,-89.5321971028266,
64.9553440727831));
#126449=CARTESIAN_POINT('Ctrl Pts',(-9.11569946399035,-89.544239904248,
65.0616068180841));
#126450=CARTESIAN_POINT('Ctrl Pts',(-9.1337712008358,-89.5560112179457,
65.1675566042376));
#126451=CARTESIAN_POINT('Ctrl Pts',(-9.15124299591421,-89.5675125901354,
65.2731732755662));
#126452=CARTESIAN_POINT('Ctrl Pts',(-9.16964894930865,-89.5796289021427,
65.3844369162756));
#126453=CARTESIAN_POINT('Ctrl Pts',(-9.18738923923466,-89.5914456250726,
65.4953311385514));
#126454=CARTESIAN_POINT('Ctrl Pts',(-9.20449991765006,-89.6029672745584,
65.6058534556344));
#126455=CARTESIAN_POINT('Ctrl Pts',(-9.22117638648685,-89.6141965446045,
65.7135711002455));
#126456=CARTESIAN_POINT('Ctrl Pts',(-9.23725367603251,-89.6251457653554,
65.8209307443482));
#126457=CARTESIAN_POINT('Ctrl Pts',(-9.25276003570989,-89.6358193485331,
65.9279223147034));
#126458=CARTESIAN_POINT('Ctrl Pts',(-9.26051321554857,-89.6411561401219,
65.981418099881));
#126459=CARTESIAN_POINT('Ctrl Pts',(-9.26812362181095,-89.6464240048523,
66.0348218752061));
#126460=CARTESIAN_POINT('Ctrl Pts',(-9.27559453031638,-89.6516234702577,
66.0881325230372));
#126461=CARTESIAN_POINT('Ctrl Pts',(-9.27932998456911,-89.6542232029604,
66.1147878469527));
#126462=CARTESIAN_POINT('Ctrl Pts',(-9.28303056205811,-89.6568058346514,
66.1414198894198));
#126463=CARTESIAN_POINT('Ctrl Pts',(-9.28669665832162,-89.6593714261074,
66.1680285154141));
#126464=CARTESIAN_POINT('Ctrl Pts',(-9.28852970645337,-89.6606542218354,
66.1813328284112));
#126465=CARTESIAN_POINT('Ctrl Pts',(-9.29035413414395,-89.6619327574292,
66.1946312873125));
#126466=CARTESIAN_POINT('Ctrl Pts',(-9.2921699899623,-89.6632070403074,
66.2079238756842));
#126467=CARTESIAN_POINT('Ctrl Pts',(-9.29307791787148,-89.6638441817465,
66.2145701698701));
#126468=CARTESIAN_POINT('Ctrl Pts',(-9.29398370280446,-89.6644802600019,
66.2212149964247));
#126469=CARTESIAN_POINT('Ctrl Pts',(-9.29488735077875,-89.66511527599,66.2278583533219));
#126470=CARTESIAN_POINT('Ctrl Pts',(-9.29579099875305,-89.6657502919782,
66.2345017102192));
#126471=CARTESIAN_POINT('Ctrl Pts',(-9.29651740248539,-89.6662610229698,
66.239850723387));
#126472=CARTESIAN_POINT('Ctrl Pts',(-9.29759188980969,-89.6670171380553,
66.2477840130256));
#126473=CARTESIAN_POINT('Ctrl Pts',(-9.31182399920604,-89.6770322516533,
66.3528643089539));
#126474=CARTESIAN_POINT('Ctrl Pts',(-9.32551671844582,-89.6867588740448,
66.457480530125));
#126475=CARTESIAN_POINT('Ctrl Pts',(-9.33868951779708,-89.6962118077819,
66.5616189265927));
#126476=CARTESIAN_POINT('Ctrl Pts',(-9.36621604052355,-89.7159651182519,
66.7792315889151));
#126477=CARTESIAN_POINT('Ctrl Pts',(-9.3914768363582,-89.7345241980598,
66.994757794308));
#126478=CARTESIAN_POINT('Ctrl Pts',(-9.41474181762129,-89.7519385865142,
67.2081436914698));
#126479=CARTESIAN_POINT('Ctrl Pts',(-9.434138334951,-89.7664573382649,67.3860481224001));
#126480=CARTESIAN_POINT('Ctrl Pts',(-9.45214578494019,-89.7801797718888,
67.5624644758447));
#126481=CARTESIAN_POINT('Ctrl Pts',(-9.46889638665283,-89.7931234924939,
67.7373665660249));
#126482=CARTESIAN_POINT('Ctrl Pts',(-9.47600631428016,-89.7986175588151,
67.8116051649949));
#126483=CARTESIAN_POINT('Ctrl Pts',(-9.48289068462014,-89.8039692324113,
67.8855695517355));
#126484=CARTESIAN_POINT('Ctrl Pts',(-9.48955517202189,-89.8091856646797,
67.9592604516609));
#126485=CARTESIAN_POINT('Ctrl Pts',(-9.50466375404086,-89.8210114646285,
68.1263198124878));
#126486=CARTESIAN_POINT('Ctrl Pts',(-9.5186447410226,-89.8321414282993,
68.2919706567794));
#126487=CARTESIAN_POINT('Ctrl Pts',(-9.53162797150561,-89.8425937213016,
68.4561895503427));
#126488=CARTESIAN_POINT('Ctrl Pts',(-9.54098307770475,-89.8501251528039,
68.5745179733959));
#126489=CARTESIAN_POINT('Ctrl Pts',(-9.54981726512395,-89.8573080437861,
68.6921043252551));
#126490=CARTESIAN_POINT('Ctrl Pts',(-9.55816846897785,-89.8641521140158,
68.8089439460119));
#126491=CARTESIAN_POINT('Ctrl Pts',(-9.5623440709048,-89.8675741491307,
68.8673637563902));
#126492=CARTESIAN_POINT('Ctrl Pts',(-9.56639886080588,-89.870911431891,
68.9255968914723));
#126493=CARTESIAN_POINT('Ctrl Pts',(-9.57033720511539,-89.8741650071343,
68.9836429109746));
#126494=CARTESIAN_POINT('Ctrl Pts',(-9.57230637727014,-89.8757917947559,
69.0126659207258));
#126495=CARTESIAN_POINT('Ctrl Pts',(-9.57424643505923,-89.8773976532099,
69.0416421518496));
#126496=CARTESIAN_POINT('Ctrl Pts',(-9.57615790736035,-89.8789827019431,
69.0705715529551));
#126497=CARTESIAN_POINT('Ctrl Pts',(-9.57711364351091,-89.8797752263098,
69.0850362535078));
#126498=CARTESIAN_POINT('Ctrl Pts',(-9.5780622331368,-89.8805625481215,
69.0994892465667));
#126499=CARTESIAN_POINT('Ctrl Pts',(-9.57900374133827,-89.8813446818348,
69.1139305261119));
#126500=CARTESIAN_POINT('Ctrl Pts',(-9.57970987248937,-89.8819312821198,
69.1247614857708));
#126501=CARTESIAN_POINT('Ctrl Pts',(-9.58041202032738,-89.8825149640896,
69.1355858565792));
#126502=CARTESIAN_POINT('Ctrl Pts',(-9.5811102120887,-89.8830957337268,
69.1464036360814));
#126503=CARTESIAN_POINT('Ctrl Pts',(-9.58134294267581,-89.8832893236059,
69.1500095625822));
#126504=CARTESIAN_POINT('Ctrl Pts',(-9.5814788872496,-89.8834024123336,
69.1521169202122));
#126505=CARTESIAN_POINT('Ctrl Pts',(-9.58180708615587,-89.8836755328058,
69.1572192183974));
#126506=CARTESIAN_POINT('Ctrl Pts',(-9.59057123577426,-89.890968880334,
69.2934698390995));
#126507=CARTESIAN_POINT('Ctrl Pts',(-9.59875323496047,-89.8978406637106,
69.429383537476));
#126508=CARTESIAN_POINT('Ctrl Pts',(-9.60637084586831,-89.9043168788772,
69.5650066938047));
#126509=CARTESIAN_POINT('Ctrl Pts',(-9.6151037548574,-89.9117412798249,
69.7204865017603));
#126510=CARTESIAN_POINT('Ctrl Pts',(-9.62309536810506,-89.9186454307002,
69.8755816217704));
#126511=CARTESIAN_POINT('Ctrl Pts',(-9.63040876584963,-89.925030666439,
70.0302322420457));
#126512=CARTESIAN_POINT('Ctrl Pts',(-9.63791116337966,-89.9315809155174,
70.1888794908479));
#126513=CARTESIAN_POINT('Ctrl Pts',(-9.64469942220319,-89.9375852668526,
70.3470593513853));
#126514=CARTESIAN_POINT('Ctrl Pts',(-9.65083230009781,-89.9430469783969,
70.5047651994685));
#126515=CARTESIAN_POINT('Ctrl Pts',(-9.65730123938662,-89.9488079736425,
70.6711128056447));
#126516=CARTESIAN_POINT('Ctrl Pts',(-9.66304052990155,-89.9539654654836,
70.836933200003));
#126517=CARTESIAN_POINT('Ctrl Pts',(-9.66811581934112,-89.9585219861143,
71.0022782405352));
#126518=CARTESIAN_POINT('Ctrl Pts',(-9.67230014378107,-89.962278611399,
71.1385970263627));
#126519=CARTESIAN_POINT('Ctrl Pts',(-9.67603295014039,-89.9656267811013,
71.2745939771198));
#126520=CARTESIAN_POINT('Ctrl Pts',(-9.67935298844021,-89.9685655423977,
71.4103244434226));
#126521=CARTESIAN_POINT('Ctrl Pts',(-9.6832714542365,-89.9720340070909,
71.5705199416948));
#126522=CARTESIAN_POINT('Ctrl Pts',(-9.68661369895617,-89.9749328318067,
71.7303422457988));
#126523=CARTESIAN_POINT('Ctrl Pts',(-9.68935269073222,-89.9772973600029,
71.8897156366769));
#126524=CARTESIAN_POINT('Ctrl Pts',(-9.69223792563923,-89.9797881375766,
72.0575984593386));
#126525=CARTESIAN_POINT('Ctrl Pts',(-9.69445346644508,-89.981686222432,
72.2249840222755));
#126526=CARTESIAN_POINT('Ctrl Pts',(-9.69599245988841,-89.9830179188359,
72.3918357271171));
#126527=CARTESIAN_POINT('Ctrl Pts',(-9.69764057859723,-89.9844440417134,
72.5705183703347));
#126528=CARTESIAN_POINT('Ctrl Pts',(-9.69851227080421,-89.9852209484255,
72.7485899466107));
#126529=CARTESIAN_POINT('Ctrl Pts',(-9.69863352861823,-89.9853599569616,
72.926047324153));
#126530=CARTESIAN_POINT('Ctrl Pts',(-9.69864784763287,-89.9853763721121,
72.9470027966594));
#126531=CARTESIAN_POINT('Ctrl Pts',(-9.69865174465511,-89.9853838658523,
72.9679497363086));
#126532=CARTESIAN_POINT('Ctrl Pts',(-9.69864529703997,-89.9853824355062,
72.9888881602058));
#126533=CARTESIAN_POINT('',(-8.1502284310481,-88.9999999997697,84.8262046968124));
#126534=CARTESIAN_POINT('Ctrl Pts',(-9.69875398068591,-89.98547710816,72.9888884257558));
#126535=CARTESIAN_POINT('Ctrl Pts',(-9.69890573883026,-89.9848877911751,
73.9716069035248));
#126536=CARTESIAN_POINT('Ctrl Pts',(-9.67912136001599,-89.9640632821437,
74.9856759988131));
#126537=CARTESIAN_POINT('Ctrl Pts',(-9.60195490217224,-89.8977852775027,
76.5544514555789));
#126538=CARTESIAN_POINT('Ctrl Pts',(-9.56819216649599,-89.8697589747,77.0852934680504));
#126539=CARTESIAN_POINT('Ctrl Pts',(-9.50208752038253,-89.8176498462862,
77.8929954127754));
#126540=CARTESIAN_POINT('Ctrl Pts',(-9.47746662247536,-89.7985988344223,
78.1641308573158));
#126541=CARTESIAN_POINT('Ctrl Pts',(-9.43614470342231,-89.7673400574451,
78.5735759435839));
#126542=CARTESIAN_POINT('Ctrl Pts',(-9.41438517235184,-89.7510400643076,
78.7789833001031));
#126543=CARTESIAN_POINT('Ctrl Pts',(-9.38695474897263,-89.730815278714,
79.0197918353817));
#126544=CARTESIAN_POINT('Ctrl Pts',(-9.37271249123869,-89.7203966553879,
79.1404831516953));
#126545=CARTESIAN_POINT('Ctrl Pts',(-9.36545758383888,-89.715110269035,
79.2008999758989));
#126546=CARTESIAN_POINT('Ctrl Pts',(-9.36231945271429,-89.71282810399,79.2268080846274));
#126547=CARTESIAN_POINT('Ctrl Pts',(-9.36022092200985,-89.7113029721415,
79.2440835239248));
#126548=CARTESIAN_POINT('Ctrl Pts',(-9.35901417344777,-89.710426596697,
79.2539855590541));
#126549=CARTESIAN_POINT('Ctrl Pts',(-9.24272592603309,-89.6260229082353,
80.2058056935545));
#126550=CARTESIAN_POINT('Ctrl Pts',(-9.09014305109249,-89.5253628372099,
81.1460397672208));
#126551=CARTESIAN_POINT('Ctrl Pts',(-8.69368888297694,-89.2881476313874,
83.006160518697));
#126552=CARTESIAN_POINT('Ctrl Pts',(-8.4496752067201,-89.1513839217613,
83.9260746582551));
#126553=CARTESIAN_POINT('Ctrl Pts',(-8.15022843089591,-89.,84.82620469727));
#126554=CARTESIAN_POINT('Origin',(27.4324635166691,-89.,72.98888938658));
#126555=CARTESIAN_POINT('Origin',(27.4324635166691,25.,72.98888938658));
#126556=CARTESIAN_POINT('Ctrl Pts',(-8.15022843089586,-89.,84.82620469727));
#126557=CARTESIAN_POINT('Ctrl Pts',(-8.0592727893093,-88.7244220625868,
85.0996152207309));
#126558=CARTESIAN_POINT('Ctrl Pts',(-7.96815107952594,-88.4382163304836,
85.3630149775318));
#126559=CARTESIAN_POINT('Ctrl Pts',(-7.87748303577277,-88.1413827738554,
85.6165445316851));
#126560=CARTESIAN_POINT('Ctrl Pts',(-7.83214901389618,-87.9929659955412,
85.7433093087617));
#126561=CARTESIAN_POINT('Ctrl Pts',(-7.7869276544551,-87.8418922610958,
85.8676067479479));
#126562=CARTESIAN_POINT('Ctrl Pts',(-7.7418919204437,-87.6881615705191,
85.989455512086));
#126563=CARTESIAN_POINT('Ctrl Pts',(-7.719374053438,-87.6112962252308,86.050379894155));
#126564=CARTESIAN_POINT('Ctrl Pts',(-7.69690255497006,-87.5337666409097,
86.1106920933842));
#126565=CARTESIAN_POINT('Ctrl Pts',(-7.67448625331229,-87.4555728175557,
86.1703945300757));
#126566=CARTESIAN_POINT('Ctrl Pts',(-7.65206995165452,-87.3773789942017,
86.2300969667672));
#126567=CARTESIAN_POINT('Ctrl Pts',(-7.62999301043884,-87.2995343704679,
86.2884442841026));
#126568=CARTESIAN_POINT('Ctrl Pts',(-7.60741161314129,-87.2189986303954,
86.3476749184798));
#126569=CARTESIAN_POINT('Ctrl Pts',(-7.51708602403756,-86.8968556704137,
86.5845974557616));
#126570=CARTESIAN_POINT('Ctrl Pts',(-7.42825142502899,-86.5653686931437,
86.8104033987204));
#126571=CARTESIAN_POINT('Ctrl Pts',(-7.34151639358491,-86.2245376985853,
87.0252821283513));
#126572=CARTESIAN_POINT('Ctrl Pts',(-7.25478136214084,-85.8837067040269,
87.2401608579821));
#126573=CARTESIAN_POINT('Ctrl Pts',(-7.17014580984083,-85.5335316921802,
87.4441127186809));
#126574=CARTESIAN_POINT('Ctrl Pts',(-7.08815755482003,-85.1740126630452,
87.6373268745396));
#126575=CARTESIAN_POINT('Ctrl Pts',(-7.03188518854192,-85.51135559513,87.78728732497));
#126576=CARTESIAN_POINT('Ctrl Pts',(-6.88609751019091,-84.8164336540901,
88.13174534986));
#126577=CARTESIAN_POINT('Ctrl Pts',(-6.48107502706592,-82.93977280408,88.90591654473));
#126578=CARTESIAN_POINT('Ctrl Pts',(-5.85681573002491,-79.41119109238,89.73590455514));
#126579=CARTESIAN_POINT('Ctrl Pts',(-5.56514360048591,-74.999772686,90.0489960419));
#126580=CARTESIAN_POINT('Ctrl Pts',(-5.85684197555091,-70.58850343071,89.73588726852));
#126581=CARTESIAN_POINT('Ctrl Pts',(-6.48119721132191,-67.05962993044,88.90572058463));
#126582=CARTESIAN_POINT('Ctrl Pts',(-6.88619857614591,-65.18309553123,88.13154378191));
#126583=CARTESIAN_POINT('Ctrl Pts',(-7.03199309806391,-64.48813202086,87.78703389719));
#126584=CARTESIAN_POINT('Ctrl Pts',(-7.61748505797291,-84.28363064449,86.1725311745699));
#126585=CARTESIAN_POINT('Ctrl Pts',(-7.51829975074291,-83.66265636758,86.47777956431));
#126586=CARTESIAN_POINT('Ctrl Pts',(-7.23957840814891,-81.99276209823,87.16157935315));
#126587=CARTESIAN_POINT('Ctrl Pts',(-6.79943451186591,-78.87943948555,87.89696709168));
#126588=CARTESIAN_POINT('Ctrl Pts',(-6.59060359545691,-74.99979991999,88.17713587471));
#126589=CARTESIAN_POINT('Ctrl Pts',(-6.79945368327691,-71.12029257632,87.8969512836301));
#126590=CARTESIAN_POINT('Ctrl Pts',(-7.23966353825691,-68.0067086013501,
87.16140622182));
#126591=CARTESIAN_POINT('Ctrl Pts',(-7.51836905611891,-66.33692462081,86.47760140457));
#126592=CARTESIAN_POINT('Ctrl Pts',(-7.61755845601991,-65.7159117191401,
86.1723066272));
#126593=CARTESIAN_POINT('Ctrl Pts',(-8.94180725924391,-83.1405774216701,
84.9904520841));
#126594=CARTESIAN_POINT('Ctrl Pts',(-8.87784551922691,-82.57791839499,85.27891283488));
#126595=CARTESIAN_POINT('Ctrl Pts',(-8.69724304976191,-81.08162805277,85.91955509897));
#126596=CARTESIAN_POINT('Ctrl Pts',(-8.40920175141591,-78.35538419096,86.60152333573));
#126597=CARTESIAN_POINT('Ctrl Pts',(-8.27170075666791,-74.99982653108,86.86227405379));
#126598=CARTESIAN_POINT('Ctrl Pts',(-8.40921447291491,-71.64438573464,86.60150867591));
#126599=CARTESIAN_POINT('Ctrl Pts',(-8.69729849347391,-68.91790285567,85.9193939094799));
#126600=CARTESIAN_POINT('Ctrl Pts',(-8.87789036104291,-67.42170567277,85.27874554859));
#126601=CARTESIAN_POINT('Ctrl Pts',(-8.94185458683591,-66.85900818197,84.99023987675));
#126602=CARTESIAN_POINT('Ctrl Pts',(-10.7849815469809,-82.27197103756,84.43730442383));
#126603=CARTESIAN_POINT('Ctrl Pts',(-10.7390165867829,-81.74231307311,84.73418669521));
#126604=CARTESIAN_POINT('Ctrl Pts',(-10.6120605629239,-80.3576414581,85.38605053251));
#126605=CARTESIAN_POINT('Ctrl Pts',(-10.4188562658489,-77.92603135117,86.06464899639));
#126606=CARTESIAN_POINT('Ctrl Pts',(-10.3293313697989,-74.99984810118,86.32271016737));
#126607=CARTESIAN_POINT('Ctrl Pts',(-10.4188642324849,-72.07377047682,86.06463496379));
#126608=CARTESIAN_POINT('Ctrl Pts',(-10.6120986166669,-69.64193190681,85.38588841531));
#126609=CARTESIAN_POINT('Ctrl Pts',(-10.7390483236119,-68.25733819811,84.73401594236));
#126610=CARTESIAN_POINT('Ctrl Pts',(-10.7850155734819,-67.72763911956,84.43708596738));
#126611=CARTESIAN_POINT('',(-10.5124641215422,-67.7275765921281,84.5902475699691));
#126612=CARTESIAN_POINT('Origin',(-13.9923868665804,-64.8259016968275,90.5664476682519));
#126613=CARTESIAN_POINT('',(-10.5124533883332,-82.2723820629486,84.5902806024135));
#126614=CARTESIAN_POINT('Ctrl Pts',(-7.08822305920791,-85.17401266098,87.6373546719));
#126615=CARTESIAN_POINT('Ctrl Pts',(-7.69414323235493,-84.0874541957658,
86.2096035275483));
#126616=CARTESIAN_POINT('Ctrl Pts',(-8.88948386358317,-83.0746694882491,
85.1457926978883));
#126617=CARTESIAN_POINT('Ctrl Pts',(-10.5124533883332,-82.2723820629485,
84.5902806024135));
#126618=CARTESIAN_POINT('',(-9.07682641225685,-75.0000006726261,86.7031084130407));
#126619=CARTESIAN_POINT('Ctrl Pts',(-9.07682655323991,-75.00000067265,86.70310871249));
#126620=CARTESIAN_POINT('Ctrl Pts',(-9.07712527162583,-75.7710653833458,
86.703079548411));
#126621=CARTESIAN_POINT('Ctrl Pts',(-9.14270874172081,-76.5105174064079,
86.6375317298765));
#126622=CARTESIAN_POINT('Ctrl Pts',(-9.35334858385702,-77.8974408785069,
86.4100699179464));
#126623=CARTESIAN_POINT('Ctrl Pts',(-9.49860676910191,-78.5448431892613,
86.2490985948516));
#126624=CARTESIAN_POINT('Ctrl Pts',(-9.80522934488242,-79.7518959795621,
85.8621453182158));
#126625=CARTESIAN_POINT('Ctrl Pts',(-9.96585902065113,-80.3121962983374,
85.6360301024058));
#126626=CARTESIAN_POINT('Ctrl Pts',(-10.2616504213497,-81.3517147132588,
85.1408733798662));
#126627=CARTESIAN_POINT('Ctrl Pts',(-10.3972012330611,-81.831526988694,
84.8713589226467));
#126628=CARTESIAN_POINT('Ctrl Pts',(-10.5124534169749,-82.27238204879,84.59028059261));
#126629=CARTESIAN_POINT('Ctrl Pts',(-10.5124650377649,-67.72757582813,84.59024914348));
#126630=CARTESIAN_POINT('Ctrl Pts',(-10.4327423171429,-68.0325174777516,
84.7846763698828));
#126631=CARTESIAN_POINT('Ctrl Pts',(-10.3563334338288,-68.3071255764948,
84.9428892616601));
#126632=CARTESIAN_POINT('Ctrl Pts',(-10.2548365651166,-68.6670586204727,
85.1382149877773));
#126633=CARTESIAN_POINT('Ctrl Pts',(-10.223125993645,-68.7784239097236,
85.1962985864462));
#126634=CARTESIAN_POINT('Ctrl Pts',(-10.1646839277008,-68.9833111354606,
85.3001142621517));
#126635=CARTESIAN_POINT('Ctrl Pts',(-10.137524099967,-69.0783222991939,
85.3465564639887));
#126636=CARTESIAN_POINT('Ctrl Pts',(-10.0666768665712,-69.3268944073992,
85.4651755558802));
#126637=CARTESIAN_POINT('Ctrl Pts',(-10.0065160646104,-69.5382359356507,
85.5619916181195));
#126638=CARTESIAN_POINT('Ctrl Pts',(-9.8977910040944,-69.927385302646,85.7233076444201));
#126639=CARTESIAN_POINT('Ctrl Pts',(-9.85850403230828,-70.0691379356638,
85.7797140223083));
#126640=CARTESIAN_POINT('Ctrl Pts',(-9.79563566630381,-70.3003928382042,
85.8665387091036));
#126641=CARTESIAN_POINT('Ctrl Pts',(-9.77402788007526,-70.3805828396457,
85.8958465728976));
#126642=CARTESIAN_POINT('Ctrl Pts',(-9.74076713746608,-70.5056027949893,
85.940114802761));
#126643=CARTESIAN_POINT('Ctrl Pts',(-9.7239250814145,-70.5692965693181,
85.962325255793));
#126644=CARTESIAN_POINT('Ctrl Pts',(-9.70394026882669,-70.645695140865,
85.9883150254738));
#126645=CARTESIAN_POINT('Ctrl Pts',(-9.69386879831417,-70.6844189512115,
86.0013220886582));
#126646=CARTESIAN_POINT('Ctrl Pts',(-9.68953604802536,-70.7011275081655,
86.0068983758215));
#126647=CARTESIAN_POINT('Ctrl Pts',(-9.68664396323484,-70.7122916036429,
86.0106162205642));
#126648=CARTESIAN_POINT('Ctrl Pts',(-9.68488025991898,-70.7191079772815,
86.0128804243338));
#126649=CARTESIAN_POINT('Ctrl Pts',(-9.53862940322314,-71.2848144523634,
86.2004563984907));
#126650=CARTESIAN_POINT('Ctrl Pts',(-9.38875606960968,-71.9186428381076,
86.3702386471311));
#126651=CARTESIAN_POINT('Ctrl Pts',(-9.1579878314319,-73.3455803154869,
86.621969533406));
#126652=CARTESIAN_POINT('Ctrl Pts',(-9.07716137299026,-74.1401369689079,
86.7030186524931));
#126653=CARTESIAN_POINT('Ctrl Pts',(-9.07682655323991,-75.00000067265,86.70310871249));
#126654=CARTESIAN_POINT('Ctrl Pts',(-6.92065457530891,-65.0085199552,88.04213796552));
#126655=CARTESIAN_POINT('Ctrl Pts',(-7.12075460565991,-64.0617034611701,
87.58903703014));
#126656=CARTESIAN_POINT('Ctrl Pts',(-7.57373925880491,-62.21199765049,86.51254138381));
#126657=CARTESIAN_POINT('Ctrl Pts',(-8.29170030411691,-59.88527159252,84.5296397505));
#126658=CARTESIAN_POINT('Ctrl Pts',(-8.94052593337591,-58.09298635035,82.330744365395));
#126659=CARTESIAN_POINT('Ctrl Pts',(-9.43809466145892,-56.85575438086,80.175556126363));
#126660=CARTESIAN_POINT('Ctrl Pts',(-9.78504368857292,-56.04942203172,78.151265483228));
#126661=CARTESIAN_POINT('Ctrl Pts',(-10.0084080082939,-55.55161389672,76.24295421649));
#126662=CARTESIAN_POINT('Ctrl Pts',(-10.1306719411089,-55.28587008401,74.370377310615));
#126663=CARTESIAN_POINT('Ctrl Pts',(-10.1545766833119,-55.23449747153,72.4633569248084));
#126664=CARTESIAN_POINT('Ctrl Pts',(-10.0742919226589,-55.40774496076,70.54498904177));
#126665=CARTESIAN_POINT('Ctrl Pts',(-9.89754394190891,-55.79679141717,68.694837416293));
#126666=CARTESIAN_POINT('Ctrl Pts',(-9.63436051758492,-56.39594592554,66.889026863432));
#126667=CARTESIAN_POINT('Ctrl Pts',(-9.27716813710291,-57.24836476724,65.062303256644));
#126668=CARTESIAN_POINT('Ctrl Pts',(-8.80090929958791,-58.46683609555,63.14889932481));
#126669=CARTESIAN_POINT('Ctrl Pts',(-8.20270682605691,-60.16216466129,61.19431102613));
#126670=CARTESIAN_POINT('Ctrl Pts',(-7.53829930230291,-62.35228602585,59.3803617293));
#126671=CARTESIAN_POINT('Ctrl Pts',(-7.11363397064091,-64.09507808025,58.37279234099));
#126672=CARTESIAN_POINT('Ctrl Pts',(-6.92079475816891,-65.00772646722,57.93600906651));
#126673=CARTESIAN_POINT('Ctrl Pts',(-7.63686846205491,-66.3621040647101,
86.13865710204));
#126674=CARTESIAN_POINT('Ctrl Pts',(-7.76950703063191,-65.54018993106,85.74905955785));
#126675=CARTESIAN_POINT('Ctrl Pts',(-8.07016186809891,-63.92982350139,84.82480089674));
#126676=CARTESIAN_POINT('Ctrl Pts',(-8.54916445708991,-61.88218169553,83.12176196493));
#126677=CARTESIAN_POINT('Ctrl Pts',(-8.98476748958292,-60.28053161396,81.222506221777));
#126678=CARTESIAN_POINT('Ctrl Pts',(-9.32101949477791,-59.15720375094,79.345376616387));
#126679=CARTESIAN_POINT('Ctrl Pts',(-9.5568109059989,-58.41509188199,77.567583873189));
#126680=CARTESIAN_POINT('Ctrl Pts',(-9.70924409102191,-57.95233484547,75.880638307014));
#126681=CARTESIAN_POINT('Ctrl Pts',(-9.79291036296791,-57.70366775115,74.217967928337));
#126682=CARTESIAN_POINT('Ctrl Pts',(-9.80928988049891,-57.65544493246,72.5212298562295));
#126683=CARTESIAN_POINT('Ctrl Pts',(-9.75430501765591,-57.81788267456,70.815731431435));
#126684=CARTESIAN_POINT('Ctrl Pts',(-9.63352487119791,-58.18069632678,69.176762924934));
#126685=CARTESIAN_POINT('Ctrl Pts',(-9.45430378327291,-58.73477501893,67.585691843247));
#126686=CARTESIAN_POINT('Ctrl Pts',(-9.21211183497991,-59.51491229764,65.986727637278));
#126687=CARTESIAN_POINT('Ctrl Pts',(-8.89088286577791,-60.61594879951,64.324292302119));
#126688=CARTESIAN_POINT('Ctrl Pts',(-8.48972710545391,-62.12654662001,62.63793056294));
#126689=CARTESIAN_POINT('Ctrl Pts',(-8.04663367869591,-64.05203475839,61.08013396196));
#126690=CARTESIAN_POINT('Ctrl Pts',(-7.76477879250591,-65.56916470704,60.21501006199));
#126691=CARTESIAN_POINT('Ctrl Pts',(-7.63695856837891,-66.36141690504,59.8394398311601));
#126692=CARTESIAN_POINT('Ctrl Pts',(-9.30568646040191,-67.5925100747501,
84.84655826695));
#126693=CARTESIAN_POINT('Ctrl Pts',(-9.38430344193091,-66.8864512848699,
84.49764454981));
#126694=CARTESIAN_POINT('Ctrl Pts',(-9.56256965368191,-65.50055373805,83.67212409033));
#126695=CARTESIAN_POINT('Ctrl Pts',(-9.84698595988291,-63.72418521299,82.154388156787));
#126696=CARTESIAN_POINT('Ctrl Pts',(-10.1060740212189,-62.31869562594,80.456822147596));
#126697=CARTESIAN_POINT('Ctrl Pts',(-10.3064235701329,-61.32140256381,78.769328788008));
#126698=CARTESIAN_POINT('Ctrl Pts',(-10.4471274598089,-60.65609648668,77.161368332835));
#126699=CARTESIAN_POINT('Ctrl Pts',(-10.5381893031789,-60.23829278713,75.6280051070961));
#126700=CARTESIAN_POINT('Ctrl Pts',(-10.5882066814419,-60.01274187767,74.111586341137));
#126701=CARTESIAN_POINT('Ctrl Pts',(-10.5980020454079,-59.96890586323,72.561632978805));
#126702=CARTESIAN_POINT('Ctrl Pts',(-10.5651238429639,-60.11644815221,71.0046224172161));
#126703=CARTESIAN_POINT('Ctrl Pts',(-10.4929458682419,-60.44475452627,69.512475580624));
#126704=CARTESIAN_POINT('Ctrl Pts',(-10.3859423486419,-60.94317745813,68.069876677003));
#126705=CARTESIAN_POINT('Ctrl Pts',(-10.2415081737819,-61.6397769585701,
66.627215680196));
#126706=CARTESIAN_POINT('Ctrl Pts',(-10.0502091869879,-62.61390026386,65.135327797585));
#126707=CARTESIAN_POINT('Ctrl Pts',(-9.81168369918191,-63.93662258829,63.629051184382));
#126708=CARTESIAN_POINT('Ctrl Pts',(-9.54861819276191,-65.60577043727,62.24063178495));
#126709=CARTESIAN_POINT('Ctrl Pts',(-9.38149959755591,-66.91134741848,61.4678544918301));
#126710=CARTESIAN_POINT('Ctrl Pts',(-9.30573940932591,-67.59192210557,61.1315047603));
#126711=CARTESIAN_POINT('Ctrl Pts',(-11.5646178953289,-68.43247654302,84.4465034494));
#126712=CARTESIAN_POINT('Ctrl Pts',(-11.6143874109131,-67.80806067473,84.10661689733));
#126713=CARTESIAN_POINT('Ctrl Pts',(-11.7267907129605,-66.583003723,83.30488853365));
#126714=CARTESIAN_POINT('Ctrl Pts',(-11.9032597796691,-65.01117314613,81.837645484982));
#126715=CARTESIAN_POINT('Ctrl Pts',(-12.0608820228823,-63.7647605769001,
80.200009462762));
#126716=CARTESIAN_POINT('Ctrl Pts',(-12.1802633017076,-62.87825648365,78.57253830883));
#126717=CARTESIAN_POINT('Ctrl Pts',(-12.2626041075034,-62.2856582147501,
77.02085457485));
#126718=CARTESIAN_POINT('Ctrl Pts',(-12.3151851184271,-61.91294559539,75.539930091032));
#126719=CARTESIAN_POINT('Ctrl Pts',(-12.3438113818399,-61.71152917766,74.074340121796));
#126720=CARTESIAN_POINT('Ctrl Pts',(-12.3493938338451,-61.67236410253,72.5757901676427));
#126721=CARTESIAN_POINT('Ctrl Pts',(-12.3306271776957,-61.80416073374,71.070632227735));
#126722=CARTESIAN_POINT('Ctrl Pts',(-12.2891286387917,-62.09718082047,69.629053886055));
#126723=CARTESIAN_POINT('Ctrl Pts',(-12.2269112507223,-62.54145725969,68.23640962794));
#126724=CARTESIAN_POINT('Ctrl Pts',(-12.1417578310604,-63.16140834367,66.844644399399));
#126725=CARTESIAN_POINT('Ctrl Pts',(-12.0270663262746,-64.02670740855,65.4058375265251));
#126726=CARTESIAN_POINT('Ctrl Pts',(-11.8814290941622,-65.19921867886,63.9523875906491));
#126727=CARTESIAN_POINT('Ctrl Pts',(-11.7180007421678,-66.67599988134,62.60977879472));
#126728=CARTESIAN_POINT('Ctrl Pts',(-11.6126219518349,-67.83008530504,61.85919024876));
#126729=CARTESIAN_POINT('Ctrl Pts',(-11.5646546770989,-68.43195908097,61.53154922964));
#126730=CARTESIAN_POINT('',(-10.5124610812362,-67.7276344807769,61.3874942276418));
#126731=CARTESIAN_POINT('Ctrl Pts',(-7.08825603872491,-64.825987319,58.34041012264));
#126732=CARTESIAN_POINT('Ctrl Pts',(-7.69416695291821,-65.9125766751487,
59.7681366846271));
#126733=CARTESIAN_POINT('Ctrl Pts',(-8.88950139818992,-66.9253426838604,
60.8319665772906));
#126734=CARTESIAN_POINT('Ctrl Pts',(-10.5124619777589,-67.72763373312,61.38749268805));
#126735=CARTESIAN_POINT('Ctrl Pts',(-10.5124561093177,-67.7276386264893,
61.3875027668017));
#126736=CARTESIAN_POINT('Ctrl Pts',(-10.5438023417544,-67.6076229168416,
61.4640236233382));
#126737=CARTESIAN_POINT('Ctrl Pts',(-10.576340043582,-67.4844449032088,
61.5453107016493));
#126738=CARTESIAN_POINT('Ctrl Pts',(-10.6098920208526,-67.3584444482681,
61.6317332225431));
#126739=CARTESIAN_POINT('Ctrl Pts',(-10.6430841483886,-67.2337953661514,
61.7172288495922));
#126740=CARTESIAN_POINT('Ctrl Pts',(-10.6772689260462,-67.1063838842474,
61.8077504324841));
#126741=CARTESIAN_POINT('Ctrl Pts',(-10.7122657704729,-66.9765786831478,
61.9036851495562));
#126742=CARTESIAN_POINT('Ctrl Pts',(-10.7465708814531,-66.849339159057,
61.9977236598827));
#126743=CARTESIAN_POINT('Ctrl Pts',(-10.7816562679877,-66.7197994639639,
62.0969635646312));
#126744=CARTESIAN_POINT('Ctrl Pts',(-10.8173430910532,-66.5883473939177,
62.2017966028244));
#126745=CARTESIAN_POINT('Ctrl Pts',(-10.8465046193832,-66.4809311843642,
62.2874610400198));
#126746=CARTESIAN_POINT('Ctrl Pts',(-10.8760675936279,-66.3722386719903,
62.3768607253668));
#126747=CARTESIAN_POINT('Ctrl Pts',(-10.905929980847,-66.2625034493625,
62.4702223439506));
#126748=CARTESIAN_POINT('Ctrl Pts',(-10.9314965512758,-66.1685540515048,
62.5501535423291));
#126749=CARTESIAN_POINT('Ctrl Pts',(-10.9572825668611,-66.0738408708389,
62.6329889654811));
#126750=CARTESIAN_POINT('Ctrl Pts',(-10.9832185102277,-65.9785092162543,
62.7188774816556));
#126751=CARTESIAN_POINT('Ctrl Pts',(-11.026670215868,-65.8187956120613,
62.8627705519772));
#126752=CARTESIAN_POINT('Ctrl Pts',(-11.0705064137141,-65.6573614979089,
63.0151950488345));
#126753=CARTESIAN_POINT('Ctrl Pts',(-11.1143817956528,-65.4951382027885,
63.1767142242415));
#126754=CARTESIAN_POINT('Ctrl Pts',(-11.1560082078672,-65.3412301692834,
63.3299542298881));
#126755=CARTESIAN_POINT('Ctrl Pts',(-11.1976696927773,-65.1866119558448,
63.4913808424263));
#126756=CARTESIAN_POINT('Ctrl Pts',(-11.2390529797762,-65.032118176574,
63.6614748088734));
#126757=CARTESIAN_POINT('Ctrl Pts',(-11.2609077837574,-64.9505289286642,
63.751302624996));
#126758=CARTESIAN_POINT('Ctrl Pts',(-11.282686080715,-64.868981940792,63.8435429374389));
#126759=CARTESIAN_POINT('Ctrl Pts',(-11.3043495221077,-64.7876164372335,
63.9382629119894));
#126760=CARTESIAN_POINT('Ctrl Pts',(-11.3248151405692,-64.7107498248809,
64.0277455950355));
#126761=CARTESIAN_POINT('Ctrl Pts',(-11.3451782345556,-64.6340451386831,
64.1194414174417));
#126762=CARTESIAN_POINT('Ctrl Pts',(-11.3654052810579,-64.5576276447232,
64.2133953716165));
#126763=CARTESIAN_POINT('Ctrl Pts',(-11.3862242573906,-64.478973848284,
64.3100988200467));
#126764=CARTESIAN_POINT('Ctrl Pts',(-11.406899835192,-64.4006233060692,
64.4091961323424));
#126765=CARTESIAN_POINT('Ctrl Pts',(-11.4273972521796,-64.3227181963433,
64.5107349606021));
#126766=CARTESIAN_POINT('Ctrl Pts',(-11.4376459606734,-64.2837656414803,
64.5615043747319));
#126767=CARTESIAN_POINT('Ctrl Pts',(-11.4478501704006,-64.2449246102199,
64.612884080549));
#126768=CARTESIAN_POINT('Ctrl Pts',(-11.4580056783908,-64.2062137707468,
64.6648794653407));
#126769=CARTESIAN_POINT('Ctrl Pts',(-11.4630834323859,-64.1868583510102,
64.6908771577365));
#126770=CARTESIAN_POINT('Ctrl Pts',(-11.468149010096,-64.1675354801149,
64.7170287702674));
#126771=CARTESIAN_POINT('Ctrl Pts',(-11.4732018890547,-64.1482475470137,
64.7433349320655));
#126772=CARTESIAN_POINT('Ctrl Pts',(-11.4757283285341,-64.1386035804631,
64.7564880129645));
#126773=CARTESIAN_POINT('Ctrl Pts',(-11.4782515932834,-64.1289683484049,
64.7696797312012));
#126774=CARTESIAN_POINT('Ctrl Pts',(-11.4807716179499,-64.1193421511978,
64.7829101641624));
#126775=CARTESIAN_POINT('Ctrl Pts',(-11.482976639533,-64.1109192286416,
64.7944867930035));
#126776=CARTESIAN_POINT('Ctrl Pts',(-11.4851791804248,-64.1025032233963,
64.8060930628069));
#126777=CARTESIAN_POINT('Ctrl Pts',(-11.487379196887,-64.094094337761,64.8177290245631));
#126778=CARTESIAN_POINT('Ctrl Pts',(-11.487693484953,-64.0928930683846,
64.819391304814));
#126779=CARTESIAN_POINT('Ctrl Pts',(-11.4877849049776,-64.0925436650061,
64.8198744603236));
#126780=CARTESIAN_POINT('Ctrl Pts',(-11.4883219064042,-64.0904909661437,
64.822717683314));
#126781=CARTESIAN_POINT('Ctrl Pts',(-11.5258190563035,-63.9471573488824,
65.0212511571591));
#126782=CARTESIAN_POINT('Ctrl Pts',(-11.5609964063703,-63.8111425419701,
65.2209281352053));
#126783=CARTESIAN_POINT('Ctrl Pts',(-11.594015105858,-63.6821643659619,
65.4211892538843));
#126784=CARTESIAN_POINT('Ctrl Pts',(-11.6274131721106,-63.5517043013831,
65.6237512630868));
#126785=CARTESIAN_POINT('Ctrl Pts',(-11.6586031518168,-63.4284436783251,
65.8269094954421));
#126786=CARTESIAN_POINT('Ctrl Pts',(-11.6877753102132,-63.312096759407,
66.0300444814576));
#126787=CARTESIAN_POINT('Ctrl Pts',(-11.7174950675559,-63.1935658591276,
66.2369925725164));
#126788=CARTESIAN_POINT('Ctrl Pts',(-11.7451206692197,-63.0822108218853,
66.4439166065601));
#126789=CARTESIAN_POINT('Ctrl Pts',(-11.7708581256066,-62.9777293233036,
66.6502154332417));
#126790=CARTESIAN_POINT('Ctrl Pts',(-11.7801202228301,-62.9401297336867,
66.7244558617095));
#126791=CARTESIAN_POINT('Ctrl Pts',(-11.7891378310711,-62.9034202902373,
66.7986158159301));
#126792=CARTESIAN_POINT('Ctrl Pts',(-11.7979206601765,-62.8675868429193,
66.8726689124244));
#126793=CARTESIAN_POINT('Ctrl Pts',(-11.8039223096278,-62.8431004517058,
66.9232722795869));
#126794=CARTESIAN_POINT('Ctrl Pts',(-11.8098143307674,-62.8190231075782,
66.973825761044));
#126795=CARTESIAN_POINT('Ctrl Pts',(-11.8156000723212,-62.7953502204353,
67.0243199683128));
#126796=CARTESIAN_POINT('Ctrl Pts',(-11.8366325561611,-62.7092939022176,
67.2078778732972));
#126797=CARTESIAN_POINT('Ctrl Pts',(-11.856262485958,-62.6285637495704,
67.3906826664573));
#126798=CARTESIAN_POINT('Ctrl Pts',(-11.8745953081227,-62.5528590078558,
67.5723776005199));
#126799=CARTESIAN_POINT('Ctrl Pts',(-11.8934193020411,-62.4751259897296,
67.7589404931876));
#126800=CARTESIAN_POINT('Ctrl Pts',(-11.9108757973575,-62.4026912023522,
67.9443333953572));
#126801=CARTESIAN_POINT('Ctrl Pts',(-11.9270787481793,-62.3352376974856,
68.128224202014));
#126802=CARTESIAN_POINT('Ctrl Pts',(-11.9310492584917,-62.3187083109794,
68.1732863855755));
#126803=CARTESIAN_POINT('Ctrl Pts',(-11.9349444923878,-62.3024780870216,
68.2182586128735));
#126804=CARTESIAN_POINT('Ctrl Pts',(-11.9387661208648,-62.2865424453986,
68.2631364596983));
#126805=CARTESIAN_POINT('Ctrl Pts',(-11.9542469369982,-62.2219896665453,
68.4449295616027));
#126806=CARTESIAN_POINT('Ctrl Pts',(-11.9685202013225,-62.1622697499585,
68.6251697788815));
#126807=CARTESIAN_POINT('Ctrl Pts',(-11.9817054877579,-62.1070691003341,
68.8035570717619));
#126808=CARTESIAN_POINT('Ctrl Pts',(-11.9905306773405,-62.070122144316,
68.9229554395179));
#126809=CARTESIAN_POINT('Ctrl Pts',(-11.9988683951492,-62.0352000449545,
69.0415248418523));
#126810=CARTESIAN_POINT('Ctrl Pts',(-12.0067537158868,-62.0022120194877,
69.1591878279127));
#126811=CARTESIAN_POINT('Ctrl Pts',(-12.0165282381559,-61.9613205706461,
69.3050410551654));
#126812=CARTESIAN_POINT('Ctrl Pts',(-12.0256045901432,-61.9233962069462,
69.4495053598849));
#126813=CARTESIAN_POINT('Ctrl Pts',(-12.0340260667932,-61.8882498965005,
69.5924495455297));
#126814=CARTESIAN_POINT('Ctrl Pts',(-12.0443085686483,-61.845336756991,
69.7669823400919));
#126815=CARTESIAN_POINT('Ctrl Pts',(-12.053615002802,-61.8065643760454,
69.9392473392475));
#126816=CARTESIAN_POINT('Ctrl Pts',(-12.0620297563089,-61.7715807855154,
70.1090179180091));
#126817=CARTESIAN_POINT('Ctrl Pts',(-12.0707293734922,-61.7354128995448,
70.2845357205214));
#126818=CARTESIAN_POINT('Ctrl Pts',(-12.0784759221661,-61.7032945687419,
70.457387502534));
#126819=CARTESIAN_POINT('Ctrl Pts',(-12.0853584309557,-61.6748564071382,
70.6273760230889));
#126820=CARTESIAN_POINT('Ctrl Pts',(-12.0912109139692,-61.650674257459,
70.7719243207282));
#126821=CARTESIAN_POINT('Ctrl Pts',(-12.096438548449,-61.6291535020079,
70.9144032875922));
#126822=CARTESIAN_POINT('Ctrl Pts',(-12.1010937813383,-61.6100782623838,
71.0547188720989));
#126823=CARTESIAN_POINT('Ctrl Pts',(-12.101742421823,-61.607420399078,71.07426985288));
#126824=CARTESIAN_POINT('Ctrl Pts',(-12.1023799462569,-61.604810030352,
71.0937788696004));
#126825=CARTESIAN_POINT('Ctrl Pts',(-12.1030065055343,-61.6022465427781,
71.1132456782365));
#126826=CARTESIAN_POINT('Ctrl Pts',(-12.1084457844721,-61.5799924249766,
71.2822407055606));
#126827=CARTESIAN_POINT('Ctrl Pts',(-12.1130528169592,-61.5612642377236,
71.4480414148776));
#126828=CARTESIAN_POINT('Ctrl Pts',(-12.116911318386,-61.5456656243764,
71.6104912946339));
#126829=CARTESIAN_POINT('Ctrl Pts',(-12.1200457784369,-61.5329940648827,
71.7424577246135));
#126830=CARTESIAN_POINT('Ctrl Pts',(-12.1226861568724,-61.5223882620892,
71.87221393459));
#126831=CARTESIAN_POINT('Ctrl Pts',(-12.1248747923724,-61.513648042856,
71.9996978758656));
#126832=CARTESIAN_POINT('Ctrl Pts',(-12.1273162086756,-61.5038983546462,
72.1419058280955));
#126833=CARTESIAN_POINT('Ctrl Pts',(-12.1291916676191,-61.4964661468903,
72.2812835408876));
#126834=CARTESIAN_POINT('Ctrl Pts',(-12.1305459358192,-61.4910776631597,
72.4177568917541));
#126835=CARTESIAN_POINT('Ctrl Pts',(-12.1311089653444,-61.488837430807,
72.474494933694));
#126836=CARTESIAN_POINT('Ctrl Pts',(-12.1315818513851,-61.4869505975996,
72.5307311892445));
#126837=CARTESIAN_POINT('Ctrl Pts',(-12.1319676597541,-61.4853982272355,
72.5864611708658));
#126838=CARTESIAN_POINT('Ctrl Pts',(-12.1320458483712,-61.4850836210691,
72.5977555090442));
#126839=CARTESIAN_POINT('Ctrl Pts',(-12.1321204603002,-61.4847827532277,
72.6090290559099));
#126840=CARTESIAN_POINT('Ctrl Pts',(-12.1321915229297,-61.484495458529,
72.6202817765625));
#126841=CARTESIAN_POINT('Ctrl Pts',(-12.1324023774452,-61.4836430078827,
72.6536704504152));
#126842=CARTESIAN_POINT('Ctrl Pts',(-12.1325820021325,-61.482910069771,
72.6868757439766));
#126843=CARTESIAN_POINT('Ctrl Pts',(-12.1327311936757,-61.4822924708232,
72.7198968084425));
#126844=CARTESIAN_POINT('Ctrl Pts',(-12.1328457263696,-61.481818346957,
72.7452467135941));
#126845=CARTESIAN_POINT('Ctrl Pts',(-12.1329392063142,-61.4814268389799,
72.7695145227435));
#126846=CARTESIAN_POINT('Ctrl Pts',(-12.1330192927011,-61.4810814594443,
72.7949419211735));
#126847=CARTESIAN_POINT('Ctrl Pts',(-12.1330435277201,-61.480976943809,
72.8026365308037));
#126848=CARTESIAN_POINT('Ctrl Pts',(-12.1330664824746,-61.4808770019494,
72.8104373358324));
#126849=CARTESIAN_POINT('Ctrl Pts',(-12.1330882249236,-61.4807815611221,
72.8184064724661));
#126850=CARTESIAN_POINT('Ctrl Pts',(-12.1335198815254,-61.4788867578659,
72.9766191208087));
#126851=CARTESIAN_POINT('Ctrl Pts',(-12.1332896604181,-61.4795152831409,
73.1386795008977));
#126852=CARTESIAN_POINT('Ctrl Pts',(-12.1323239957528,-61.4830694277461,
73.3045108131254));
#126853=CARTESIAN_POINT('Ctrl Pts',(-12.1313891342929,-61.4865102006496,
73.4650523636382));
#126854=CARTESIAN_POINT('Ctrl Pts',(-12.1297650083798,-61.4926929857708,
73.6291282763541));
#126855=CARTESIAN_POINT('Ctrl Pts',(-12.1273794940025,-61.5020097389348,
73.7966288939179));
#126856=CARTESIAN_POINT('Ctrl Pts',(-12.1259968230349,-61.5074098338727,
73.8937141360713));
#126857=CARTESIAN_POINT('Ctrl Pts',(-12.1243582631598,-61.5138632821912,
73.9919491456346));
#126858=CARTESIAN_POINT('Ctrl Pts',(-12.1224488799031,-61.5214506542386,
74.0913057436497));
#126859=CARTESIAN_POINT('Ctrl Pts',(-12.1192505880294,-61.5341598001248,
74.2577319437944));
#126860=CARTESIAN_POINT('Ctrl Pts',(-12.1152925857901,-61.5500496941281,
74.4273073862083));
#126861=CARTESIAN_POINT('Ctrl Pts',(-12.1105082832172,-61.5694865436168,
74.5998752133286));
#126862=CARTESIAN_POINT('Ctrl Pts',(-12.1058412023223,-61.5884471648407,
74.7682149027085));
#126863=CARTESIAN_POINT('Ctrl Pts',(-12.1003894003114,-61.6107843636321,
74.9394029220836));
#126864=CARTESIAN_POINT('Ctrl Pts',(-12.094069497973,-61.6368433161217,
75.1132814589855));
#126865=CARTESIAN_POINT('Ctrl Pts',(-12.0890393747711,-61.6575841020577,
75.2516744935554));
#126866=CARTESIAN_POINT('Ctrl Pts',(-12.0834592429624,-61.680682966408,
75.3917711999041));
#126867=CARTESIAN_POINT('Ctrl Pts',(-12.0772848465946,-61.7063238630825,
75.5334705951441));
#126868=CARTESIAN_POINT('Ctrl Pts',(-12.0695748590907,-61.7383417286644,
75.7104110605041));
#126869=CARTESIAN_POINT('Ctrl Pts',(-12.0609382481766,-61.7743231686574,
75.8898518990448));
#126870=CARTESIAN_POINT('Ctrl Pts',(-12.0512938757378,-61.8146144057835,
76.0715772112131));
#126871=CARTESIAN_POINT('Ctrl Pts',(-12.0416495032989,-61.8549056429096,
76.2533025233813));
#126872=CARTESIAN_POINT('Ctrl Pts',(-12.0309973732903,-61.8995066938939,
76.4373127173123));
#126873=CARTESIAN_POINT('Ctrl Pts',(-12.0192532062723,-61.9487789363498,
76.6233402471264));
#126874=CARTESIAN_POINT('Ctrl Pts',(-12.0119610900703,-61.9793727551339,
76.7388473207304));
#126875=CARTESIAN_POINT('Ctrl Pts',(-12.0042493416637,-62.0117709110583,
76.8551362886535));
#126876=CARTESIAN_POINT('Ctrl Pts',(-11.9960865951416,-62.04605383537,76.9721351064428));
#126877=CARTESIAN_POINT('Ctrl Pts',(-11.983203031392,-62.1001638386265,
77.1567986536362));
#126878=CARTESIAN_POINT('Ctrl Pts',(-11.9691959878891,-62.158968700625,
77.3432328300292));
#126879=CARTESIAN_POINT('Ctrl Pts',(-11.953950818084,-62.2227705709226,
77.5311535277543));
#126880=CARTESIAN_POINT('Ctrl Pts',(-11.9391675825026,-62.2846392212027,
77.7133801595713));
#126881=CARTESIAN_POINT('Ctrl Pts',(-11.9232200992943,-62.3512067118891,
77.8970046933264));
#126882=CARTESIAN_POINT('Ctrl Pts',(-11.9060019391879,-62.4227585422542,
78.0817208074706));
#126883=CARTESIAN_POINT('Ctrl Pts',(-11.8924848796091,-62.47893006976,78.2267315812477));
#126884=CARTESIAN_POINT('Ctrl Pts',(-11.8781846626541,-62.5381736325303,
78.3724142381549));
#126885=CARTESIAN_POINT('Ctrl Pts',(-11.8630490617186,-62.6006315321448,
78.518598370791));
#126886=CARTESIAN_POINT('Ctrl Pts',(-11.8527079585239,-62.6433046699995,
78.6184758191628));
#126887=CARTESIAN_POINT('Ctrl Pts',(-11.8419768601538,-62.6874783657934,
78.7185868613273));
#126888=CARTESIAN_POINT('Ctrl Pts',(-11.8308411848522,-62.7331971715572,
78.8188816475872));
#126889=CARTESIAN_POINT('Ctrl Pts',(-11.8088680429328,-62.8234104527664,
79.0167853680701));
#126890=CARTESIAN_POINT('Ctrl Pts',(-11.7853100432508,-62.9196242385598,
79.2153970823566));
#126891=CARTESIAN_POINT('Ctrl Pts',(-11.7600015537594,-63.0221098479846,
79.4142611496952));
#126892=CARTESIAN_POINT('Ctrl Pts',(-11.7374125321294,-63.1135830925194,
79.5917567177362));
#126893=CARTESIAN_POINT('Ctrl Pts',(-11.7134289650972,-63.2100527378074,
79.7694528166375));
#126894=CARTESIAN_POINT('Ctrl Pts',(-11.6879340427069,-63.3117149837188,
79.946990504635));
#126895=CARTESIAN_POINT('Ctrl Pts',(-11.6776109810424,-63.3528786953563,
80.0188766815338));
#126896=CARTESIAN_POINT('Ctrl Pts',(-11.6670390543325,-63.3948936216669,
80.0907377515338));
#126897=CARTESIAN_POINT('Ctrl Pts',(-11.6562097610406,-63.4377703728835,
80.162545776049));
#126898=CARTESIAN_POINT('Ctrl Pts',(-11.6386839781394,-63.507160739649,
80.2787575928594));
#126899=CARTESIAN_POINT('Ctrl Pts',(-11.6204840638948,-63.5788083395828,
80.3948305815524));
#126900=CARTESIAN_POINT('Ctrl Pts',(-11.6015778893442,-63.6527581555802,
80.510661085996));
#126901=CARTESIAN_POINT('Ctrl Pts',(-11.5862836790107,-63.712580095601,
80.6043625428008));
#126902=CARTESIAN_POINT('Ctrl Pts',(-11.5705275262936,-63.7739076751408,
80.6979037327157));
#126903=CARTESIAN_POINT('Ctrl Pts',(-11.5542930734213,-63.8367611427316,
80.7912243017232));
#126904=CARTESIAN_POINT('Ctrl Pts',(-11.5461758469852,-63.868187876527,
80.837884586227));
#126905=CARTESIAN_POINT('Ctrl Pts',(-11.5379390457412,-63.8999960821772,
80.8844897138579));
#126906=CARTESIAN_POINT('Ctrl Pts',(-11.5295806409392,-63.9321880788289,
80.9310318791045));
#126907=CARTESIAN_POINT('Ctrl Pts',(-11.5254014385383,-63.9482840771547,
80.9543029617278));
#126908=CARTESIAN_POINT('Ctrl Pts',(-11.5211918353313,-63.9644760231451,
80.9775583038081));
#126909=CARTESIAN_POINT('Ctrl Pts',(-11.5169515785101,-63.9807642000307,
81.0007969225799));
#126910=CARTESIAN_POINT('Ctrl Pts',(-11.5148314500995,-63.9889082884735,
81.0124162319659));
#126911=CARTESIAN_POINT('Ctrl Pts',(-11.5127036582898,-63.9970764346354,
81.0240313605289));
#126912=CARTESIAN_POINT('Ctrl Pts',(-11.5105681715546,-64.0052686731633,
81.0356421845783));
#126913=CARTESIAN_POINT('Ctrl Pts',(-11.5089665565033,-64.0114128520592,
81.0443503026154));
#126914=CARTESIAN_POINT('Ctrl Pts',(-11.5073606130567,-64.0175705829106,
81.053055999364));
#126915=CARTESIAN_POINT('Ctrl Pts',(-11.5057503279326,-64.0237418801664,
81.0617592224612));
#126916=CARTESIAN_POINT('Ctrl Pts',(-11.5052135662245,-64.0257989792517,
81.0646602968269));
#126917=CARTESIAN_POINT('Ctrl Pts',(-11.5044589032026,-64.0286905507612,
81.0687338632904));
#126918=CARTESIAN_POINT('Ctrl Pts',(-11.5041385950919,-64.0299177000775,
81.0704616190519));
#126919=CARTESIAN_POINT('Ctrl Pts',(-11.4693282359868,-64.1632815049607,
81.2582301971615));
#126920=CARTESIAN_POINT('Ctrl Pts',(-11.4338224094827,-64.2984486344061,
81.4383197181533));
#126921=CARTESIAN_POINT('Ctrl Pts',(-11.3978475310335,-64.4346583969914,
81.6109610394162));
#126922=CARTESIAN_POINT('Ctrl Pts',(-11.3818221835758,-64.4953343149279,
81.687865737307));
#126923=CARTESIAN_POINT('Ctrl Pts',(-11.365703592804,-64.5562176505651,
81.7632928978732));
#126924=CARTESIAN_POINT('Ctrl Pts',(-11.3495109701921,-64.6172436488808,
81.8372649522619));
#126925=CARTESIAN_POINT('Ctrl Pts',(-11.3088630152425,-64.7704357592468,
82.0229552389044));
#126926=CARTESIAN_POINT('Ctrl Pts',(-11.2677500849922,-64.9245238729807,
82.1994752984627));
#126927=CARTESIAN_POINT('Ctrl Pts',(-11.2264661430999,-65.0785573569255,
82.3672898262114));
#126928=CARTESIAN_POINT('Ctrl Pts',(-11.1844002383752,-65.2355084028539,
82.5382829439258));
#126929=CARTESIAN_POINT('Ctrl Pts',(-11.1421568545417,-65.3924027172242,
82.7002380132411));
#126930=CARTESIAN_POINT('Ctrl Pts',(-11.1000240148836,-65.548281736956,
82.8536621198914));
#126931=CARTESIAN_POINT('Ctrl Pts',(-11.0627471787476,-65.6861949828407,
82.9894033927163));
#126932=CARTESIAN_POINT('Ctrl Pts',(-11.0255565497497,-65.8233142083913,
83.1184672839319));
#126933=CARTESIAN_POINT('Ctrl Pts',(-10.9886364195613,-65.9590053830707,
83.2412108269353));
#126934=CARTESIAN_POINT('Ctrl Pts',(-10.966306089561,-66.0410752103776,
83.3154495635453));
#126935=CARTESIAN_POINT('Ctrl Pts',(-10.9440995863303,-66.1226383441794,
83.3873692256676));
#126936=CARTESIAN_POINT('Ctrl Pts',(-10.9220620077695,-66.2035972621863,
83.4570689492617));
#126937=CARTESIAN_POINT('Ctrl Pts',(-10.8850013345343,-66.3397461588291,
83.5742832191318));
#126938=CARTESIAN_POINT('Ctrl Pts',(-10.8484188681295,-66.4741832051189,
83.6852208513242));
#126939=CARTESIAN_POINT('Ctrl Pts',(-10.8125103570658,-66.6064494670023,
83.790334502538));
#126940=CARTESIAN_POINT('Ctrl Pts',(-10.7771834166723,-66.7365735576764,
83.8937457435215));
#126941=CARTESIAN_POINT('Ctrl Pts',(-10.7425087210743,-66.8645970764474,
83.9915201052581));
#126942=CARTESIAN_POINT('Ctrl Pts',(-10.7086632572777,-66.9901294897027,
84.0840601625485));
#126943=CARTESIAN_POINT('Ctrl Pts',(-10.6739820207459,-67.1187617738597,
84.1788853844699));
#126944=CARTESIAN_POINT('Ctrl Pts',(-10.6401714806484,-67.2447785203136,
84.2682147686759));
#126945=CARTESIAN_POINT('Ctrl Pts',(-10.6074124011771,-67.3678047457111,
84.3524499440023));
#126946=CARTESIAN_POINT('Ctrl Pts',(-10.5746533217058,-67.4908309711085,
84.4366851193286));
#126947=CARTESIAN_POINT('Ctrl Pts',(-10.5429456614745,-67.6108669255703,
84.5158261086302));
#126948=CARTESIAN_POINT('Ctrl Pts',(-10.5124609685256,-67.727579221203,
84.5902421548952));
#126949=CARTESIAN_POINT('Ctrl Pts',(-7.03190132271491,-64.48874263761,58.19041163036));
#126950=CARTESIAN_POINT('Ctrl Pts',(-6.87538499698691,-65.23521415548,57.82043934767));
#126951=CARTESIAN_POINT('Ctrl Pts',(-6.44219525657191,-67.23717591574,57.00605633762));
#126952=CARTESIAN_POINT('Ctrl Pts',(-5.81802729745091,-70.88052909333,56.2001657272));
#126953=CARTESIAN_POINT('Ctrl Pts',(-5.65466277349091,-73.83365375479,56.02303478332));
#126954=CARTESIAN_POINT('Ctrl Pts',(-5.66377280622291,-75.2425631386,56.03448007742));
#126955=CARTESIAN_POINT('Ctrl Pts',(-7.61748996822491,-65.7164492576301,
59.80517843096));
#126956=CARTESIAN_POINT('Ctrl Pts',(-7.51101325256191,-66.3834691039,59.4773126071101));
#126957=CARTESIAN_POINT('Ctrl Pts',(-7.21262838267092,-68.16429015863,58.75816291855));
#126958=CARTESIAN_POINT('Ctrl Pts',(-6.77170455789591,-71.37723474796,58.04355709918));
#126959=CARTESIAN_POINT('Ctrl Pts',(-6.65471882509291,-73.97423010814,57.88507987323));
#126960=CARTESIAN_POINT('Ctrl Pts',(-6.66121085611991,-75.21333331973,57.8952394617801));
#126961=CARTESIAN_POINT('Ctrl Pts',(-8.94180688412191,-66.85948039078,60.9872761331401));
#126962=CARTESIAN_POINT('Ctrl Pts',(-8.87314531440391,-67.46383081509,60.6774497334101));
#126963=CARTESIAN_POINT('Ctrl Pts',(-8.67972634156291,-69.0582366384701,
60.0041732311799));
#126964=CARTESIAN_POINT('Ctrl Pts',(-8.39095292952791,-71.86723579451,59.34163138087));
#126965=CARTESIAN_POINT('Ctrl Pts',(-8.31392057053391,-74.11277277759,59.19423894577));
#126966=CARTESIAN_POINT('Ctrl Pts',(-8.31818721880991,-75.18451754242,59.20357135831));
#126967=CARTESIAN_POINT('Ctrl Pts',(-10.7849809204589,-67.72806305548,61.54044568591));
#126968=CARTESIAN_POINT('Ctrl Pts',(-10.7356317320139,-68.29693106613,61.22159666065));
#126969=CARTESIAN_POINT('Ctrl Pts',(-10.5999126060329,-69.77059692297,60.53721706415));
#126970=CARTESIAN_POINT('Ctrl Pts',(-10.4069349481069,-72.2691792786301,
59.87887438407));
#126971=CARTESIAN_POINT('Ctrl Pts',(-10.3567972434249,-74.22628006642,59.73315744833));
#126972=CARTESIAN_POINT('Ctrl Pts',(-10.3596005994849,-75.1608999773,59.74225854723));
#126973=CARTESIAN_POINT('',(-9.07718749353492,-75.0000704107034,59.2746757745282));
#126974=CARTESIAN_POINT('Origin',(-12.2732112378679,-75.0025912594184,52.4899004903005));
#126975=CARTESIAN_POINT('Ctrl Pts',(-9.07715892555361,-75.0000703914058,
59.2747363757385));
#126976=CARTESIAN_POINT('Ctrl Pts',(-9.0773127009558,-74.832857148716,59.2747599930608));
#126977=CARTESIAN_POINT('Ctrl Pts',(-9.08051151357833,-74.6670415245432,
59.2778801351493));
#126978=CARTESIAN_POINT('Ctrl Pts',(-9.08649648450185,-74.50288770246,59.2839023726706));
#126979=CARTESIAN_POINT('Ctrl Pts',(-9.0925301261762,-74.3373989549659,
59.2899735840006));
#126980=CARTESIAN_POINT('Ctrl Pts',(-9.10139524577937,-74.1735991368877,
59.2989940519194));
#126981=CARTESIAN_POINT('Ctrl Pts',(-9.11282574947299,-74.011705812419,
59.3107672755481));
#126982=CARTESIAN_POINT('Ctrl Pts',(-9.12433239231336,-73.8487341085611,
59.3226189211978));
#126983=CARTESIAN_POINT('Ctrl Pts',(-9.13843855877331,-73.6876942906821,
59.3372598927645));
#126984=CARTESIAN_POINT('Ctrl Pts',(-9.15487444279722,-73.5287554860593,
59.3544959235967));
#126985=CARTESIAN_POINT('Ctrl Pts',(-9.17153044121632,-73.3676881242626,
59.3719627846353));
#126986=CARTESIAN_POINT('Ctrl Pts',(-9.19057884342498,-73.2087783349392,
59.3920944476079));
#126987=CARTESIAN_POINT('Ctrl Pts',(-9.21174268813516,-73.052149383601,
59.4146985404614));
#126988=CARTESIAN_POINT('Ctrl Pts',(-9.22410816607753,-72.9606352060292,
59.4279055175213));
#126989=CARTESIAN_POINT('Ctrl Pts',(-9.23719588777561,-72.8698986706841,
59.4419567242433));
#126990=CARTESIAN_POINT('Ctrl Pts',(-9.25095145667989,-72.7799564487297,
59.4568157702803));
#126991=CARTESIAN_POINT('Ctrl Pts',(-9.2740752764921,-72.6287589411269,
59.4817945919875));
#126992=CARTESIAN_POINT('Ctrl Pts',(-9.29905722820936,-72.4796871923342,
59.5090536971147));
#126993=CARTESIAN_POINT('Ctrl Pts',(-9.32558888018677,-72.3328475236606,
59.5384048910294));
#126994=CARTESIAN_POINT('Ctrl Pts',(-9.3361553352476,-72.2743673822239,
59.5500942525417));
#126995=CARTESIAN_POINT('Ctrl Pts',(-9.34696763875273,-72.2162406966429,
59.5621155468557));
#126996=CARTESIAN_POINT('Ctrl Pts',(-9.35800653552035,-72.1584719535309,
59.574457351823));
#126997=CARTESIAN_POINT('Ctrl Pts',(-9.38679592664713,-72.0078113417539,
59.6066447214392));
#126998=CARTESIAN_POINT('Ctrl Pts',(-9.41712538814356,-71.8595886590536,
59.6410108307925));
#126999=CARTESIAN_POINT('Ctrl Pts',(-9.44860522972388,-71.7137833374362,
59.6773583586395));
#127000=CARTESIAN_POINT('Ctrl Pts',(-9.48147079396201,-71.5615597580496,
59.715305881606));
#127001=CARTESIAN_POINT('Ctrl Pts',(-9.51559001782784,-71.4119710067821,
59.7554127840311));
#127002=CARTESIAN_POINT('Ctrl Pts',(-9.55053752099497,-71.2649410788004,
59.7974761241889));
#127003=CARTESIAN_POINT('Ctrl Pts',(-9.58548502416211,-71.1179111508188,
59.8395394643468));
#127004=CARTESIAN_POINT('Ctrl Pts',(-9.62126076092705,-70.9734395747625,
59.8835591509684));
#127005=CARTESIAN_POINT('Ctrl Pts',(-9.65745893337754,-70.8314033385646,
59.9293563090885));
#127006=CARTESIAN_POINT('Ctrl Pts',(-9.69745063613198,-70.6744818545821,
59.9799529610892));
#127007=CARTESIAN_POINT('Ctrl Pts',(-9.73787512708575,-70.5205510584211,
60.0326779352948));
#127008=CARTESIAN_POINT('Ctrl Pts',(-9.77836794971244,-70.3696212117005,
60.0873359005608));
#127009=CARTESIAN_POINT('Ctrl Pts',(-9.81980468036516,-70.2151731144741,
60.1432679704398));
#127010=CARTESIAN_POINT('Ctrl Pts',(-9.86131281739014,-70.0638671796215,
60.201224220966));
#127011=CARTESIAN_POINT('Ctrl Pts',(-9.90252777852388,-69.9156655216722,
60.2610014311872));
#127012=CARTESIAN_POINT('Ctrl Pts',(-9.94565783802503,-69.7605775111613,
60.3235562550359));
#127013=CARTESIAN_POINT('Ctrl Pts',(-9.9884666611632,-69.6088886519274,
60.3881052946684));
#127014=CARTESIAN_POINT('Ctrl Pts',(-10.0305673179908,-69.4605073347355,
60.4544214019772));
#127015=CARTESIAN_POINT('Ctrl Pts',(-10.0464816427542,-69.4044182223903,
60.4794893260496));
#127016=CARTESIAN_POINT('Ctrl Pts',(-10.0622950959451,-69.348801273108,
60.5048097923068));
#127017=CARTESIAN_POINT('Ctrl Pts',(-10.0779879145727,-69.2936500306986,
60.5303706686463));
#127018=CARTESIAN_POINT('Ctrl Pts',(-10.0913798922194,-69.2465849225712,
60.5521838745904));
#127019=CARTESIAN_POINT('Ctrl Pts',(-10.1046840277155,-69.1998589447846,
60.5741721611837));
#127020=CARTESIAN_POINT('Ctrl Pts',(-10.1178881125732,-69.1534664352015,
60.5963277239018));
#127021=CARTESIAN_POINT('Ctrl Pts',(-10.1645098311032,-68.9896611774352,
60.6745558192263));
#127022=CARTESIAN_POINT('Ctrl Pts',(-10.20985514067,-68.830019727719,60.7548568087025));
#127023=CARTESIAN_POINT('Ctrl Pts',(-10.2536478639727,-68.674514504205,
60.8369131460621));
#127024=CARTESIAN_POINT('Ctrl Pts',(-10.2976229428249,-68.5183617475314,
60.9193111709755));
#127025=CARTESIAN_POINT('Ctrl Pts',(-10.3400326286217,-68.3663793370692,
61.0034794657588));
#127026=CARTESIAN_POINT('Ctrl Pts',(-10.3806348632554,-68.2185240971467,
61.0890630067659));
#127027=CARTESIAN_POINT('Ctrl Pts',(-10.421394210819,-68.0700967219673,
61.1749777187295));
#127028=CARTESIAN_POINT('Ctrl Pts',(-10.4603322871068,-67.9258281880866,
61.2623188942037));
#127029=CARTESIAN_POINT('Ctrl Pts',(-10.4972393820192,-67.7856650022798,
61.3506897699846));
#127030=CARTESIAN_POINT('Ctrl Pts',(-10.5023538913183,-67.7662414762911,
61.3629360241811));
#127031=CARTESIAN_POINT('Ctrl Pts',(-10.507429450164,-67.7468967778124,
61.37520199055));
#127032=CARTESIAN_POINT('Ctrl Pts',(-10.5124655500624,-67.7276307548579,
61.387486552728));
#127033=CARTESIAN_POINT('Ctrl Pts',(-5.66390799836291,-74.75737804457,56.03434061462));
#127034=CARTESIAN_POINT('Ctrl Pts',(-5.65535142628591,-76.10467861883,56.0232167771601));
#127035=CARTESIAN_POINT('Ctrl Pts',(-5.80770735786591,-79.026938051,56.19025778671));
#127036=CARTESIAN_POINT('Ctrl Pts',(-6.42570231203591,-82.68817021729,56.97863787517));
#127037=CARTESIAN_POINT('Ctrl Pts',(-6.87092180434491,-84.74323712603,57.80972126602));
#127038=CARTESIAN_POINT('Ctrl Pts',(-7.03202708148491,-85.51176293719,58.190648673));
#127039=CARTESIAN_POINT('Ctrl Pts',(-6.66130762481391,-74.78661230242,57.89514017999));
#127040=CARTESIAN_POINT('Ctrl Pts',(-6.65520895153991,-75.97153049077,57.88529641475));
#127041=CARTESIAN_POINT('Ctrl Pts',(-6.76428650217192,-78.54142323843,58.0346527913201));
#127042=CARTESIAN_POINT('Ctrl Pts',(-7.20118434740491,-81.76946793919,58.7339909933601));
#127043=CARTESIAN_POINT('Ctrl Pts',(-7.50797960521091,-83.59728170036,59.46781607306));
#127044=CARTESIAN_POINT('Ctrl Pts',(-7.61757460804891,-84.28400193635,59.8053942113101));
#127045=CARTESIAN_POINT('Ctrl Pts',(-8.31825718332691,-74.8154343473,59.20351517363));
#127046=CARTESIAN_POINT('Ctrl Pts',(-8.31424878828192,-75.84030625732,59.19451804723));
#127047=CARTESIAN_POINT('Ctrl Pts',(-8.38606722527991,-78.06244770262,59.33332269739));
#127048=CARTESIAN_POINT('Ctrl Pts',(-8.67229125102691,-80.88281314368,59.98168293644));
#127049=CARTESIAN_POINT('Ctrl Pts',(-8.87119507621291,-82.5187403495901,
60.66848706106));
#127050=CARTESIAN_POINT('Ctrl Pts',(-8.94186638725491,-83.14093103373,60.98748931569));
#127051=CARTESIAN_POINT('Ctrl Pts',(-10.3596572459539,-74.8390589230501,
59.74223918064));
#127052=CARTESIAN_POINT('Ctrl Pts',(-10.3570244645989,-75.73279276851,59.73351469424));
#127053=CARTESIAN_POINT('Ctrl Pts',(-10.4037890980549,-77.6695346223,59.8706524028));
#127054=CARTESIAN_POINT('Ctrl Pts',(-10.5947786127089,-80.17541503562,60.51456235328));
#127055=CARTESIAN_POINT('Ctrl Pts',(-10.7342367672979,-81.68668075087,61.21238965717));
#127056=CARTESIAN_POINT('Ctrl Pts',(-10.7850333778129,-82.27233159581,61.54067352347));
#127057=CARTESIAN_POINT('',(-10.5124842662009,-82.2724282582398,61.3875276985405));
#127058=CARTESIAN_POINT('Origin',(-13.992064676801,-85.1738977789521,55.4111095407736));
#127059=CARTESIAN_POINT('Ctrl Pts',(-10.5124867527329,-82.2724303312993,
61.3875234280722));
#127060=CARTESIAN_POINT('Ctrl Pts',(-10.4762711011264,-82.1338625944223,
61.2991699968375));
#127061=CARTESIAN_POINT('Ctrl Pts',(-10.438002373032,-81.9912324976581,
61.2117810269455));
#127062=CARTESIAN_POINT('Ctrl Pts',(-10.3978910917222,-81.8444856272407,
61.1257577565632));
#127063=CARTESIAN_POINT('Ctrl Pts',(-10.3579096744694,-81.698213863659,
61.0400129946334));
#127064=CARTESIAN_POINT('Ctrl Pts',(-10.3160974143833,-81.5478516042782,
60.9556248663313));
#127065=CARTESIAN_POINT('Ctrl Pts',(-10.2726971972061,-81.3933546676573,
60.8729533678949));
#127066=CARTESIAN_POINT('Ctrl Pts',(-10.2295936236166,-81.2399137286455,
60.7908469350617));
#127067=CARTESIAN_POINT('Ctrl Pts',(-10.1849235906381,-81.0823940478829,
60.7104334616942));
#127068=CARTESIAN_POINT('Ctrl Pts',(-10.1389615230731,-80.9207673678253,
60.6320326508068));
#127069=CARTESIAN_POINT('Ctrl Pts',(-10.1319059530302,-80.8959562915974,
60.6199974565272));
#127070=CARTESIAN_POINT('Ctrl Pts',(-10.1248200088764,-80.8710484703209,
60.6080096315989));
#127071=CARTESIAN_POINT('Ctrl Pts',(-10.1177047628883,-80.8460438430459,
60.5960702697948));
#127072=CARTESIAN_POINT('Ctrl Pts',(-10.0996785737433,-80.7826956269042,
60.5658223775208));
#127073=CARTESIAN_POINT('Ctrl Pts',(-10.0814646789748,-80.7187301616859,
60.5358871188695));
#127074=CARTESIAN_POINT('Ctrl Pts',(-10.0630950294152,-80.654132126471,
60.5062841964149));
#127075=CARTESIAN_POINT('Ctrl Pts',(-10.0218969588841,-80.5092565041948,
60.4398929850177));
#127076=CARTESIAN_POINT('Ctrl Pts',(-9.97991351415051,-80.3611963072566,
60.3751730647508));
#127077=CARTESIAN_POINT('Ctrl Pts',(-9.93751558889771,-80.2098428202604,
60.3123409636049));
#127078=CARTESIAN_POINT('Ctrl Pts',(-9.89646762773618,-80.0633084788077,
60.2515094575311));
#127079=CARTESIAN_POINT('Ctrl Pts',(-9.85503123342581,-79.9136868150178,
60.1924473470377));
#127080=CARTESIAN_POINT('Ctrl Pts',(-9.81356958142742,-79.7609190158336,
60.1353567984347));
#127081=CARTESIAN_POINT('Ctrl Pts',(-9.77350619410377,-79.613303201839,
60.0801915879097));
#127082=CARTESIAN_POINT('Ctrl Pts',(-9.73341937574205,-79.4627496238593,
60.0268671777777));
#127083=CARTESIAN_POINT('Ctrl Pts',(-9.69366035730599,-79.3092477597733,
59.975572340852));
#127084=CARTESIAN_POINT('Ctrl Pts',(-9.68152659738807,-79.2624016644964,
59.9599180500579));
#127085=CARTESIAN_POINT('Ctrl Pts',(-9.66942352908825,-79.2152812982283,
59.944452833371));
#127086=CARTESIAN_POINT('Ctrl Pts',(-9.65736155610982,-79.1678872397631,
59.9291821806378));
#127087=CARTESIAN_POINT('Ctrl Pts',(-9.62201461612017,-79.0290015911687,
59.8844323833426));
#127088=CARTESIAN_POINT('Ctrl Pts',(-9.58703968796021,-78.8878078118406,
59.8413703728143));
#127089=CARTESIAN_POINT('Ctrl Pts',(-9.55282750996213,-78.7441854699933,
59.800166502298));
#127090=CARTESIAN_POINT('Ctrl Pts',(-9.5191756918907,-78.6029155128712,
59.7596375083668));
#127091=CARTESIAN_POINT('Ctrl Pts',(-9.48626192830372,-78.4592955945563,
59.7209064168299));
#127092=CARTESIAN_POINT('Ctrl Pts',(-9.45447515147843,-78.3132529060324,
59.6841568027735));
#127093=CARTESIAN_POINT('Ctrl Pts',(-9.42327095192074,-78.1698868383845,
59.6480807231828));
#127094=CARTESIAN_POINT('Ctrl Pts',(-9.39315293618557,-78.0241857785365,
59.6139143499317));
#127095=CARTESIAN_POINT('Ctrl Pts',(-9.36450404991878,-77.8761252320951,
59.5818497633476));
#127096=CARTESIAN_POINT('Ctrl Pts',(-9.35417346630618,-77.8227356573488,
59.5702875026152));
#127097=CARTESIAN_POINT('Ctrl Pts',(-9.34403404331903,-77.7690397248902,
59.558998692747));
#127098=CARTESIAN_POINT('Ctrl Pts',(-9.33410417244265,-77.7150378179831,
59.547992859992));
#127099=CARTESIAN_POINT('Ctrl Pts',(-9.30747413422574,-77.5702149031008,
59.5184772952358));
#127100=CARTESIAN_POINT('Ctrl Pts',(-9.28235096974286,-77.4231876848988,
59.4909962251838));
#127101=CARTESIAN_POINT('Ctrl Pts',(-9.25904243547962,-77.2740527153528,
59.4657370725323));
#127102=CARTESIAN_POINT('Ctrl Pts',(-9.25620601913232,-77.2559044757081,
59.4626632853653));
#127103=CARTESIAN_POINT('Ctrl Pts',(-9.25339647976746,-77.2377250856647,
59.459622413244));
#127104=CARTESIAN_POINT('Ctrl Pts',(-9.25061437593473,-77.2195147713465,
59.4566148033186));
#127105=CARTESIAN_POINT('Ctrl Pts',(-9.22695626991347,-77.0646601818987,
59.4310390668385));
#127106=CARTESIAN_POINT('Ctrl Pts',(-9.20528666567254,-76.9074701121915,
59.407860857459));
#127107=CARTESIAN_POINT('Ctrl Pts',(-9.18587873902337,-76.7480308556771,
59.3872658982294));
#127108=CARTESIAN_POINT('Ctrl Pts',(-9.16679394018577,-76.5912461463984,
59.3670138300373));
#127109=CARTESIAN_POINT('Ctrl Pts',(-9.14989624892856,-76.4322864143346,
59.3492599343375));
#127110=CARTESIAN_POINT('Ctrl Pts',(-9.13545003206928,-76.2712822983254,
59.334193112631));
#127111=CARTESIAN_POINT('Ctrl Pts',(-9.12111676305156,-76.1115369940565,
59.3192440909692));
#127112=CARTESIAN_POINT('Ctrl Pts',(-9.10919691016474,-75.9497790199847,
59.3069405025098));
#127113=CARTESIAN_POINT('Ctrl Pts',(-9.09995150671631,-75.7861860647748,
59.2974758526382));
#127114=CARTESIAN_POINT('Ctrl Pts',(-9.09078434628428,-75.6239775820057,
59.2880913012457));
#127115=CARTESIAN_POINT('Ctrl Pts',(-9.08424670897293,-75.4599649789326,
59.2814980596483));
#127116=CARTESIAN_POINT('Ctrl Pts',(-9.0805937999134,-75.2943723586259,
59.2778904338773));
#127117=CARTESIAN_POINT('Ctrl Pts',(-9.07844141775526,-75.1968011911922,
59.2757647337254));
#127118=CARTESIAN_POINT('Ctrl Pts',(-9.07729057504939,-75.0986824358921,
59.2746756866574));
#127119=CARTESIAN_POINT('Ctrl Pts',(-9.07719325348405,-75.0000704146066,
59.2746634980018));
#127120=CARTESIAN_POINT('Ctrl Pts',(-6.95501045707591,-85.1529137311,58.01387408059));
#127121=CARTESIAN_POINT('Ctrl Pts',(-7.05774004267591,-85.63125128373,58.24814136492));
#127122=CARTESIAN_POINT('Ctrl Pts',(-7.30909908298691,-86.71753851572,58.83656145538));
#127123=CARTESIAN_POINT('Ctrl Pts',(-7.70408428485791,-88.18560403961,59.83257430806));
#127124=CARTESIAN_POINT('Ctrl Pts',(-7.99155039204292,-89.1287412301401,
60.6313043667));
#127125=CARTESIAN_POINT('Ctrl Pts',(-8.11817253279791,-89.52581262105,61.00177960564));
#127126=CARTESIAN_POINT('Ctrl Pts',(-7.61082803413691,-83.8733505902,59.77519556645));
#127127=CARTESIAN_POINT('Ctrl Pts',(-7.68132640632891,-84.29308008815,59.97887993217));
#127128=CARTESIAN_POINT('Ctrl Pts',(-7.85394933178791,-85.24759038451,60.490155777));
#127129=CARTESIAN_POINT('Ctrl Pts',(-8.12583286142491,-86.5433442491299,
61.3549613678501));
#127130=CARTESIAN_POINT('Ctrl Pts',(-8.32426658251891,-87.38107274318,62.04914416167));
#127131=CARTESIAN_POINT('Ctrl Pts',(-8.41178668367091,-87.73491510949,62.37149197426));
#127132=CARTESIAN_POINT('Ctrl Pts',(-9.10619475060691,-82.69410558745,61.0173249886));
#127133=CARTESIAN_POINT('Ctrl Pts',(-9.15027307656091,-83.0587530577401,
61.20050989027));
#127134=CARTESIAN_POINT('Ctrl Pts',(-9.25823067031591,-83.88877557576,61.65978326684));
#127135=CARTESIAN_POINT('Ctrl Pts',(-9.42839777627291,-85.01925517755,62.43508999421));
#127136=CARTESIAN_POINT('Ctrl Pts',(-9.55271238964991,-85.7537033340401,
63.057206833302));
#127137=CARTESIAN_POINT('Ctrl Pts',(-9.60756611401691,-86.06469941247,63.346234090372));
#127138=CARTESIAN_POINT('Ctrl Pts',(-11.1563436524369,-81.83974571622,61.5037200941));
#127139=CARTESIAN_POINT('Ctrl Pts',(-11.1848443441729,-82.16332661371,61.68039275776));
#127140=CARTESIAN_POINT('Ctrl Pts',(-11.2545217931519,-82.89985707379,62.12270842198));
#127141=CARTESIAN_POINT('Ctrl Pts',(-11.3637278730099,-83.90357345901,62.86726820837));
#127142=CARTESIAN_POINT('Ctrl Pts',(-11.4429513703819,-84.55653760648,63.463524128386));
#127143=CARTESIAN_POINT('Ctrl Pts',(-11.4777951321979,-84.83322947472,63.740383029282));
#127144=CARTESIAN_POINT('',(-11.2183622024927,-84.8936594351933,63.5797742587981));
#127145=CARTESIAN_POINT('Origin',(-15.266749813004,-89.0000231752399,58.784173264979));
#127146=CARTESIAN_POINT('Ctrl Pts',(-11.2183618829509,-84.89365911108,63.579774637322));
#127147=CARTESIAN_POINT('Ctrl Pts',(-11.1916862812499,-84.79459105882,63.472429641703));
#127148=CARTESIAN_POINT('Ctrl Pts',(-11.1374145693669,-84.59364149351,63.261778406171));
#127149=CARTESIAN_POINT('Ctrl Pts',(-11.0534807578479,-84.28415018161,62.95789841798));
#127150=CARTESIAN_POINT('Ctrl Pts',(-10.9672526777759,-83.96690341805,62.66606616824));
#127151=CARTESIAN_POINT('Ctrl Pts',(-10.8789867581169,-83.64220144843,62.38623331845));
#127152=CARTESIAN_POINT('Ctrl Pts',(-10.7889753777679,-83.31030668945,62.11833551683));
#127153=CARTESIAN_POINT('Ctrl Pts',(-10.6976076698479,-82.97144101564,61.86230947727));
#127154=CARTESIAN_POINT('Ctrl Pts',(-10.6052835128899,-82.62579823329,61.61807691418));
#127155=CARTESIAN_POINT('Ctrl Pts',(-10.5434296705349,-82.39092106547,61.46307272833));
#127156=CARTESIAN_POINT('Ctrl Pts',(-10.5124834373569,-82.27242756722,61.38752912203));
#127157=CARTESIAN_POINT('Ctrl Pts',(-8.06612779774991,-89.12550208689,60.88625533387));
#127158=CARTESIAN_POINT('Ctrl Pts',(-8.09637982822591,-89.23409807329,60.9678095002));
#127159=CARTESIAN_POINT('Ctrl Pts',(-8.20385936829092,-89.63416343301,61.28679075656));
#127160=CARTESIAN_POINT('Ctrl Pts',(-8.35457669863391,-90.30389549261,61.94147242306));
#127161=CARTESIAN_POINT('Ctrl Pts',(-8.4646874159229,-91.0756228145,62.9334803921));
#127162=CARTESIAN_POINT('Ctrl Pts',(-8.49068670939391,-91.7484865399,64.060395809805));
#127163=CARTESIAN_POINT('Ctrl Pts',(-8.4424810519869,-92.33192150942,65.328224889624));
#127164=CARTESIAN_POINT('Ctrl Pts',(-8.32876960322491,-92.84821811054,66.807276461651));
#127165=CARTESIAN_POINT('Ctrl Pts',(-8.15823859365691,-93.3022201360699,
68.644737618775));
#127166=CARTESIAN_POINT('Ctrl Pts',(-7.99043840954591,-93.61899006591,70.8474005016));
#127167=CARTESIAN_POINT('Ctrl Pts',(-7.95242679364891,-93.68276184645,72.4799516511365));
#127168=CARTESIAN_POINT('Ctrl Pts',(-7.95741734812491,-93.6732941703,73.2720763218484));
#127169=CARTESIAN_POINT('Ctrl Pts',(-8.43949877683291,-87.3537747401099,
62.27006488597));
#127170=CARTESIAN_POINT('Ctrl Pts',(-8.45731359140492,-87.4535563417601,
62.34368555564));
#127171=CARTESIAN_POINT('Ctrl Pts',(-8.52131292219791,-87.82106654726,62.63149311457));
#127172=CARTESIAN_POINT('Ctrl Pts',(-8.61411039860292,-88.43540728025,63.222074263414));
#127173=CARTESIAN_POINT('Ctrl Pts',(-8.68403744008991,-89.13943833049,64.117405994067));
#127174=CARTESIAN_POINT('Ctrl Pts',(-8.70113772340991,-89.7471218280801,
65.132620071883));
#127175=CARTESIAN_POINT('Ctrl Pts',(-8.66952211163591,-90.26679126728,66.269050071176));
#127176=CARTESIAN_POINT('Ctrl Pts',(-8.59296528164791,-90.71932698016,67.5848917653981));
#127177=CARTESIAN_POINT('Ctrl Pts',(-8.47524822121891,-91.1106638471899,
69.204437583702));
#127178=CARTESIAN_POINT('Ctrl Pts',(-8.35657014317891,-91.37998713432,71.128070825606));
#127179=CARTESIAN_POINT('Ctrl Pts',(-8.32937461695891,-91.43389890748,72.5465372663564));
#127180=CARTESIAN_POINT('Ctrl Pts',(-8.33290939283891,-91.42587213809,73.2350085774806));
#127181=CARTESIAN_POINT('Ctrl Pts',(-9.70290977013891,-85.71563863313,63.225929504496));
#127182=CARTESIAN_POINT('Ctrl Pts',(-9.71347226780991,-85.81258521909,63.3042697667619));
#127183=CARTESIAN_POINT('Ctrl Pts',(-9.75155217659191,-86.16920472985,63.607119168682));
#127184=CARTESIAN_POINT('Ctrl Pts',(-9.80734092195292,-86.76321296501,64.208958863088));
#127185=CARTESIAN_POINT('Ctrl Pts',(-9.84976775888791,-87.44130407606,65.092689108936));
#127186=CARTESIAN_POINT('Ctrl Pts',(-9.86024687222591,-88.02252314883,66.068935008635));
#127187=CARTESIAN_POINT('Ctrl Pts',(-9.84088807922991,-88.51301036784,67.134160433264));
#127188=CARTESIAN_POINT('Ctrl Pts',(-9.79367311983191,-88.93113286615,68.3343103616489));
#127189=CARTESIAN_POINT('Ctrl Pts',(-9.72059012292691,-89.2817921413201,
69.767187011365));
#127190=CARTESIAN_POINT('Ctrl Pts',(-9.64644890999391,-89.51483550078,71.418566814176));
#127191=CARTESIAN_POINT('Ctrl Pts',(-9.62940986650091,-89.56052949701,72.6152524275675));
#127192=CARTESIAN_POINT('Ctrl Pts',(-9.63161894838992,-89.55368004058,73.1967232445338));
#127193=CARTESIAN_POINT('Ctrl Pts',(-11.6147520896694,-84.5243630961,63.571054202212));
#127194=CARTESIAN_POINT('Ctrl Pts',(-11.6246340679083,-84.6249961903,63.66586459399));
#127195=CARTESIAN_POINT('Ctrl Pts',(-11.6593120484911,-84.99447215027,64.027094849045));
#127196=CARTESIAN_POINT('Ctrl Pts',(-11.7060805587835,-85.60709500622,64.713399121719));
#127197=CARTESIAN_POINT('Ctrl Pts',(-11.7389496702744,-86.30596314069,65.6728212489209));
#127198=CARTESIAN_POINT('Ctrl Pts',(-11.7463516547408,-86.90449452193,66.690284220663));
#127199=CARTESIAN_POINT('Ctrl Pts',(-11.7325725181496,-87.40596349938,67.7581163994829));
#127200=CARTESIAN_POINT('Ctrl Pts',(-11.7012754818754,-87.82560147568,68.912217015091));
#127201=CARTESIAN_POINT('Ctrl Pts',(-11.6561110576122,-88.16534971416,70.225368387264));
#127202=CARTESIAN_POINT('Ctrl Pts',(-11.6134044513163,-88.3802178611799,
71.663335401016));
#127203=CARTESIAN_POINT('Ctrl Pts',(-11.6039200063252,-88.42090783937,72.6729563753231));
#127204=CARTESIAN_POINT('Ctrl Pts',(-11.6051869982177,-88.4147469583799,
73.1645418273416));
#127205=CARTESIAN_POINT('',(-11.2241290292204,-88.6512992632751,72.9889531634726));
#127206=CARTESIAN_POINT('Origin',(-15.3537166934403,-94.9097718533471,73.0060860461187));
#127207=CARTESIAN_POINT('Ctrl Pts',(-11.2240197558157,-88.6511336051499,
72.9889531154357));
#127208=CARTESIAN_POINT('Ctrl Pts',(-11.2242745255353,-88.6509671919425,
72.9761856442956));
#127209=CARTESIAN_POINT('Ctrl Pts',(-11.2245118171374,-88.6508027974082,
72.9569880187906));
#127210=CARTESIAN_POINT('Ctrl Pts',(-11.2247672217957,-88.6505537102174,
72.9313531986707));
#127211=CARTESIAN_POINT('Ctrl Pts',(-11.2250224784259,-88.6503047673933,
72.905733236053));
#127212=CARTESIAN_POINT('Ctrl Pts',(-11.2252958726478,-88.6499712088215,
72.8736832010589));
#127213=CARTESIAN_POINT('Ctrl Pts',(-11.2256349948435,-88.6494160359053,
72.8352002030464));
#127214=CARTESIAN_POINT('Ctrl Pts',(-11.2259720748059,-88.6488642063049,
72.7969489541183));
#127215=CARTESIAN_POINT('Ctrl Pts',(-11.2263741723918,-88.6480933420174,
72.7523415227726));
#127216=CARTESIAN_POINT('Ctrl Pts',(-11.2268989971422,-88.6469198945246,
72.7013851606149));
#127217=CARTESIAN_POINT('Ctrl Pts',(-11.2272369925059,-88.6461641759504,
72.6685684648564));
#127218=CARTESIAN_POINT('Ctrl Pts',(-11.2276261104829,-88.6452404949846,
72.6331187210802));
#127219=CARTESIAN_POINT('Ctrl Pts',(-11.2280839387327,-88.6440892094085,
72.5950416458244));
#127220=CARTESIAN_POINT('Ctrl Pts',(-11.2287632555083,-88.6423809539531,
72.5385436119001));
#127221=CARTESIAN_POINT('Ctrl Pts',(-11.2295979323301,-88.640170573144,
72.4762570353377));
#127222=CARTESIAN_POINT('Ctrl Pts',(-11.2306657390954,-88.637218963774,
72.4081865053001));
#127223=CARTESIAN_POINT('Ctrl Pts',(-11.2316410246325,-88.634523099669,
72.3460140171672));
#127224=CARTESIAN_POINT('Ctrl Pts',(-11.2328109383719,-88.6312084061529,
72.2790163014364));
#127225=CARTESIAN_POINT('Ctrl Pts',(-11.2342393575461,-88.6270626171519,
72.2072196998836));
#127226=CARTESIAN_POINT('Ctrl Pts',(-11.2357355307736,-88.6227201813865,
72.1320175778403));
#127227=CARTESIAN_POINT('Ctrl Pts',(-11.2375167516463,-88.6174653044088,
72.051546660498));
#127228=CARTESIAN_POINT('Ctrl Pts',(-11.2396643553321,-88.6110151748712,
71.9658383006492));
#127229=CARTESIAN_POINT('Ctrl Pts',(-11.240738157175,-88.6077901101024,
71.9229841207248));
#127230=CARTESIAN_POINT('Ctrl Pts',(-11.2419034100726,-88.6042657527526,
71.8788202239335));
#127231=CARTESIAN_POINT('Ctrl Pts',(-11.2431696669609,-88.6004035007701,
71.8333495265937));
#127232=CARTESIAN_POINT('Ctrl Pts',(-11.243802795405,-88.5984723747788,
71.8106141779239));
#127233=CARTESIAN_POINT('Ctrl Pts',(-11.244461156607,-88.5964567476816,
71.7875521308478));
#127234=CARTESIAN_POINT('Ctrl Pts',(-11.2451459415228,-88.5943515507392,
71.7641637757324));
#127235=CARTESIAN_POINT('Ctrl Pts',(-11.2454883339806,-88.593298952268,
71.7524695981747));
#127236=CARTESIAN_POINT('Ctrl Pts',(-11.2458373311496,-88.5922239595018,
71.7406938437182));
#127237=CARTESIAN_POINT('Ctrl Pts',(-11.2461930770222,-88.5911259259485,
71.7288365623583));
#127238=CARTESIAN_POINT('Ctrl Pts',(-11.2463709499585,-88.5905769091719,
71.7229079216783));
#127239=CARTESIAN_POINT('Ctrl Pts',(-11.2465505099919,-88.5900221320799,
71.7169588992809));
#127240=CARTESIAN_POINT('Ctrl Pts',(-11.2467317749972,-88.5894615129103,
71.7109895015165));
#127241=CARTESIAN_POINT('Ctrl Pts',(-11.2468224074999,-88.5891812033255,
71.7080048026343));
#127242=CARTESIAN_POINT('Ctrl Pts',(-11.2469134662406,-88.5888994332138,
71.7050150099109));
#127243=CARTESIAN_POINT('Ctrl Pts',(-11.2470049534458,-88.5886161922945,
71.7020201241467));
#127244=CARTESIAN_POINT('Ctrl Pts',(-11.2470964406511,-88.5883329513752,
71.6990252383824));
#127245=CARTESIAN_POINT('Ctrl Pts',(-11.2472508047561,-88.5878547041565,
71.6939931057192));
#127246=CARTESIAN_POINT('Ctrl Pts',(-11.2472807026685,-88.5877620467987,
71.6930201885352));
#127247=CARTESIAN_POINT('Ctrl Pts',(-11.2477188332067,-88.5864042256359,
71.6787628475912));
#127248=CARTESIAN_POINT('Ctrl Pts',(-11.2481906728962,-88.5849616586075,
71.6639168877229));
#127249=CARTESIAN_POINT('Ctrl Pts',(-11.2486979846655,-88.5834283333534,
71.6484822011923));
#127250=CARTESIAN_POINT('Ctrl Pts',(-11.2503106722699,-88.5785540631702,
71.5994170520069));
#127251=CARTESIAN_POINT('Ctrl Pts',(-11.2522817326128,-88.5727659906201,
71.5444007021859));
#127252=CARTESIAN_POINT('Ctrl Pts',(-11.2546673042124,-88.5658423347889,
71.4834425465419));
#127253=CARTESIAN_POINT('Ctrl Pts',(-11.2570204709904,-88.5590127276259,
71.4233124264758));
#127254=CARTESIAN_POINT('Ctrl Pts',(-11.2597772685108,-88.5510780541774,
71.3574005696904));
#127255=CARTESIAN_POINT('Ctrl Pts',(-11.2629906638128,-88.5417831055776,
71.2857435995938));
#127256=CARTESIAN_POINT('Ctrl Pts',(-11.2644459367637,-88.5375736367738,
71.2532918031204));
#127257=CARTESIAN_POINT('Ctrl Pts',(-11.2659948166465,-88.5330846099312,
71.2196620993046));
#127258=CARTESIAN_POINT('Ctrl Pts',(-11.2676418836711,-88.5282895140319,
71.1848600200692));
#127259=CARTESIAN_POINT('Ctrl Pts',(-11.2711519048001,-88.5180708115325,
71.1106942261965));
#127260=CARTESIAN_POINT('Ctrl Pts',(-11.2751087946652,-88.5064636760206,
71.0311953045052));
#127261=CARTESIAN_POINT('Ctrl Pts',(-11.2795473902357,-88.4931829448063,
70.9464067805103));
#127262=CARTESIAN_POINT('Ctrl Pts',(-11.2815142287214,-88.4872979632045,
70.9088351366222));
#127263=CARTESIAN_POINT('Ctrl Pts',(-11.2835755289603,-88.4810838644701,
70.8702252769905));
#127264=CARTESIAN_POINT('Ctrl Pts',(-11.2857335898617,-88.4745134816927,
70.8305831879646));
#127265=CARTESIAN_POINT('Ctrl Pts',(-11.2892476854252,-88.4638145468512,
70.7660316782822));
#127266=CARTESIAN_POINT('Ctrl Pts',(-11.293018420646,-88.4521714371299,
70.6987413507889));
#127267=CARTESIAN_POINT('Ctrl Pts',(-11.2970505565863,-88.4394586051646,
70.628738799706));
#127268=CARTESIAN_POINT('Ctrl Pts',(-11.2990666245565,-88.4331021891819,
70.5937375241646));
#127269=CARTESIAN_POINT('Ctrl Pts',(-11.3011479344878,-88.4264781837837,
70.5580582142501));
#127270=CARTESIAN_POINT('Ctrl Pts',(-11.3032946151084,-88.4195697734577,
70.5217045156815));
#127271=CARTESIAN_POINT('Ctrl Pts',(-11.3043679554187,-88.4161155682947,
70.5035276663972));
#127272=CARTESIAN_POINT('Ctrl Pts',(-11.3054576310313,-88.4125902510797,
70.4851822214201));
#127273=CARTESIAN_POINT('Ctrl Pts',(-11.3065636138707,-88.4089916532588,
70.466668651342));
#127274=CARTESIAN_POINT('Ctrl Pts',(-11.3071166052905,-88.4071923543484,
70.4574118663029));
#127275=CARTESIAN_POINT('Ctrl Pts',(-11.3076736730322,-88.405374734581,
70.4481130500982));
#127276=CARTESIAN_POINT('Ctrl Pts',(-11.3082348106141,-88.4035385188914,
70.4387722639503));
#127277=CARTESIAN_POINT('Ctrl Pts',(-11.3087959481959,-88.4017023032017,
70.4294314778024));
#127278=CARTESIAN_POINT('Ctrl Pts',(-11.309459193718,-88.3995248099728,
70.4184256286073));
#127279=CARTESIAN_POINT('Ctrl Pts',(-11.3099304244086,-88.3979738061611,
70.4106240577841));
#127280=CARTESIAN_POINT('Ctrl Pts',(-11.3161893151632,-88.3773733579903,
70.3070035159241));
#127281=CARTESIAN_POINT('Ctrl Pts',(-11.3224767080662,-88.3558955118018,
70.2052254946104));
#127282=CARTESIAN_POINT('Ctrl Pts',(-11.3287287672198,-88.3336575856445,
70.1053181242262));
#127283=CARTESIAN_POINT('Ctrl Pts',(-11.3396427516581,-88.2948376746266,
69.9309135866394));
#127284=CARTESIAN_POINT('Ctrl Pts',(-11.3504467258724,-88.253701523487,
69.7622090979111));
#127285=CARTESIAN_POINT('Ctrl Pts',(-11.3608858503052,-88.2108286042613,
69.5991748821252));
#127286=CARTESIAN_POINT('Ctrl Pts',(-11.3716123989377,-88.166775249399,
69.431651786138));
#127287=CARTESIAN_POINT('Ctrl Pts',(-11.3819537487847,-88.1208883263476,
69.2701150314172));
#127288=CARTESIAN_POINT('Ctrl Pts',(-11.3916854425355,-88.0737898026253,
69.1145168693028));
#127289=CARTESIAN_POINT('Ctrl Pts',(-11.3931999939023,-88.0664598212977,
69.0903010015266));
#127290=CARTESIAN_POINT('Ctrl Pts',(-11.3946998778907,-88.0591004783046,
69.0662289505687));
#127291=CARTESIAN_POINT('Ctrl Pts',(-11.3961843563362,-88.0517141003437,
69.0423005151616));
#127292=CARTESIAN_POINT('Ctrl Pts',(-11.4015341233223,-88.0250950537155,
68.956067162196));
#127293=CARTESIAN_POINT('Ctrl Pts',(-11.4066887884465,-87.9981222265563,
68.8717032079022));
#127294=CARTESIAN_POINT('Ctrl Pts',(-11.4116279620168,-87.9708955175075,
68.7891981885541));
#127295=CARTESIAN_POINT('Ctrl Pts',(-11.4185172356412,-87.9329190735016,
68.6741182777992));
#127296=CARTESIAN_POINT('Ctrl Pts',(-11.4249872025774,-87.8944486596017,
68.562654875211));
#127297=CARTESIAN_POINT('Ctrl Pts',(-11.4310142678285,-87.855743445013,
68.4547791264471));
#127298=CARTESIAN_POINT('Ctrl Pts',(-11.4361883127967,-87.822516241981,
68.3621712067002));
#127299=CARTESIAN_POINT('Ctrl Pts',(-11.4410356293391,-87.7891159936686,
68.2722057637127));
#127300=CARTESIAN_POINT('Ctrl Pts',(-11.4455514956465,-87.7556979118045,
68.1848566034732));
#127301=CARTESIAN_POINT('Ctrl Pts',(-11.4478094288002,-87.7389888708724,
68.1411820233534));
#127302=CARTESIAN_POINT('Ctrl Pts',(-11.4499845038457,-87.7222753760469,
68.0981615098983));
#127303=CARTESIAN_POINT('Ctrl Pts',(-11.4520774016122,-87.7055757548429,
68.0557915330754));
#127304=CARTESIAN_POINT('Ctrl Pts',(-11.4534623527881,-87.6945249713823,
68.0277536851878));
#127305=CARTESIAN_POINT('Ctrl Pts',(-11.4547703837296,-87.683821685813,
68.0008571179604));
#127306=CARTESIAN_POINT('Ctrl Pts',(-11.4560833007314,-87.6727952916227,
67.9733995645209));
#127307=CARTESIAN_POINT('Ctrl Pts',(-11.4567544255561,-87.667158920962,
67.9593640651589));
#127308=CARTESIAN_POINT('Ctrl Pts',(-11.4574267125168,-87.6614374289534,
67.9451823919486));
#127309=CARTESIAN_POINT('Ctrl Pts',(-11.4581103184323,-87.6555367675149,
67.9306298265414));
#127310=CARTESIAN_POINT('Ctrl Pts',(-11.4623071180713,-87.619311373272,
67.8412885849503));
#127311=CARTESIAN_POINT('Ctrl Pts',(-11.4662235340514,-87.5818180497456,
67.7513816670787));
#127312=CARTESIAN_POINT('Ctrl Pts',(-11.4698027840946,-87.5430029926291,
67.6609294029669));
#127313=CARTESIAN_POINT('Ctrl Pts',(-11.475785945847,-87.4781187955625,
67.5097271900694));
#127314=CARTESIAN_POINT('Ctrl Pts',(-11.4808278170763,-87.4095416663116,
67.3569981853293));
#127315=CARTESIAN_POINT('Ctrl Pts',(-11.4846831264988,-87.337022253606,
67.2029120936388));
#127316=CARTESIAN_POINT('Ctrl Pts',(-11.4883729157958,-87.2676163192169,
67.0554413851604));
#127317=CARTESIAN_POINT('Ctrl Pts',(-11.4909758971826,-87.1945991804734,
66.9067274080467));
#127318=CARTESIAN_POINT('Ctrl Pts',(-11.4922587536103,-87.1177441567912,
66.7569628191743));
#127319=CARTESIAN_POINT('Ctrl Pts',(-11.4926072969111,-87.096863173498,
66.7162728066242));
#127320=CARTESIAN_POINT('Ctrl Pts',(-11.4928582814169,-87.0756988479199,
66.6755055098484));
#127321=CARTESIAN_POINT('Ctrl Pts',(-11.4930067714473,-87.0542465467405,
66.6346654152655));
#127322=CARTESIAN_POINT('Ctrl Pts',(-11.493518944891,-86.9802530339186,
66.4937993125153));
#127323=CARTESIAN_POINT('Ctrl Pts',(-11.4928126466536,-86.9028330702812,
66.3520630396957));
#127324=CARTESIAN_POINT('Ctrl Pts',(-11.4907005478281,-86.8218389933892,
66.2097182555379));
#127325=CARTESIAN_POINT('Ctrl Pts',(-11.4885884490026,-86.7408449164971,
66.0673734713802));
#127326=CARTESIAN_POINT('Ctrl Pts',(-11.4850706336615,-86.6562766227845,
65.9244197258589));
#127327=CARTESIAN_POINT('Ctrl Pts',(-11.4799467033179,-86.5679916716801,
65.781175173196));
#127328=CARTESIAN_POINT('Ctrl Pts',(-11.4778444076629,-86.5317692688256,
65.7224034139284));
#127329=CARTESIAN_POINT('Ctrl Pts',(-11.4754702275825,-86.4949212922084,
65.663581338532));
#127330=CARTESIAN_POINT('Ctrl Pts',(-11.4727992458932,-86.457434097807,
65.604715206676));
#127331=CARTESIAN_POINT('Ctrl Pts',(-11.4676289803903,-86.3848694865291,
65.4907670160001));
#127332=CARTESIAN_POINT('Ctrl Pts',(-11.4613470631302,-86.3099097321324,
65.3766505663401));
#127333=CARTESIAN_POINT('Ctrl Pts',(-11.4537794840977,-86.2324876677326,
65.262464666662));
#127334=CARTESIAN_POINT('Ctrl Pts',(-11.4465361633332,-86.1583830109739,
65.1531714442723));
#127335=CARTESIAN_POINT('Ctrl Pts',(-11.4381149629705,-86.0820223655018,
65.0438144674924));
#127336=CARTESIAN_POINT('Ctrl Pts',(-11.4283559618822,-86.0033458151717,
64.9345266511644));
#127337=CARTESIAN_POINT('Ctrl Pts',(-11.4205914636241,-85.9407488411113,
64.8475746104977));
#127338=CARTESIAN_POINT('Ctrl Pts',(-11.411979975111,-85.876685805877,64.7606671320666));
#127339=CARTESIAN_POINT('Ctrl Pts',(-11.4024376136905,-85.811127109965,
64.6738946118772));
#127340=CARTESIAN_POINT('Ctrl Pts',(-11.4010476440789,-85.8015776293827,
64.6612550606308));
#127341=CARTESIAN_POINT('Ctrl Pts',(-11.399638690759,-85.7919965920506,
64.6486194534414));
#127342=CARTESIAN_POINT('Ctrl Pts',(-11.3982101770104,-85.7823838748884,
64.635987712293));
#127343=CARTESIAN_POINT('Ctrl Pts',(-11.3880774781259,-85.7141991839361,
64.5463885540258));
#127344=CARTESIAN_POINT('Ctrl Pts',(-11.3769610614966,-85.6444206348788,
64.4569799346877));
#127345=CARTESIAN_POINT('Ctrl Pts',(-11.3646619607724,-85.5730292249959,
64.3677650832233));
#127346=CARTESIAN_POINT('Ctrl Pts',(-11.352722443728,-85.5037250559967,
64.2811585691726));
#127347=CARTESIAN_POINT('Ctrl Pts',(-11.3396683115244,-85.4329006832326,
64.1947343917873));
#127348=CARTESIAN_POINT('Ctrl Pts',(-11.3253131918183,-85.3605404164633,
64.1085436510511));
#127349=CARTESIAN_POINT('Ctrl Pts',(-11.3115545684955,-85.2911869262528,
64.0259343827223));
#127350=CARTESIAN_POINT('Ctrl Pts',(-11.2966007409571,-85.2204222912503,
63.9435394171877));
#127351=CARTESIAN_POINT('Ctrl Pts',(-11.2802847637017,-85.1482379428458,
63.8614513511311));
#127352=CARTESIAN_POINT('Ctrl Pts',(-11.2744827839982,-85.1225691080715,
63.8322607433176));
#127353=CARTESIAN_POINT('Ctrl Pts',(-11.2685085368507,-85.0967208144483,
63.8031094064044));
#127354=CARTESIAN_POINT('Ctrl Pts',(-11.262354457998,-85.0706929373549,
63.7740031019365));
#127355=CARTESIAN_POINT('Ctrl Pts',(-11.2486127761017,-85.0125742788164,
63.7090105032463));
#127356=CARTESIAN_POINT('Ctrl Pts',(-11.2339742973963,-84.9535597088113,
63.6442408305321));
#127357=CARTESIAN_POINT('Ctrl Pts',(-11.2183631611147,-84.8936604075354,
63.579773123225));
#127358=CARTESIAN_POINT('Ctrl Pts',(-7.95814792783791,-93.67295473434,72.7059852969892));
#127359=CARTESIAN_POINT('Ctrl Pts',(-7.95271346435991,-93.6874724926401,
73.9073476595992));
#127360=CARTESIAN_POINT('Ctrl Pts',(-8.06439460568691,-93.50423865288,76.59995736407));
#127361=CARTESIAN_POINT('Ctrl Pts',(-8.42970521090091,-92.66068586414,80.031694782438));
#127362=CARTESIAN_POINT('Ctrl Pts',(-8.53434685477391,-91.35085311195,82.802279089842));
#127363=CARTESIAN_POINT('Ctrl Pts',(-8.31596425941191,-90.05403658787,84.34463821187));
#127364=CARTESIAN_POINT('Ctrl Pts',(-8.1057478610679,-89.26927616764,84.98339808023));
#127365=CARTESIAN_POINT('Ctrl Pts',(-8.06516310420291,-89.12509080528,85.09190979212));
#127366=CARTESIAN_POINT('Ctrl Pts',(-8.33354804813591,-91.42591365382,72.7430411923306));
#127367=CARTESIAN_POINT('Ctrl Pts',(-8.32981191803891,-91.43826407759,73.7872734245095));
#127368=CARTESIAN_POINT('Ctrl Pts',(-8.40995296574992,-91.28362370523,76.126620078171));
#127369=CARTESIAN_POINT('Ctrl Pts',(-8.66300469726491,-90.56112912654,79.150030229971));
#127370=CARTESIAN_POINT('Ctrl Pts',(-8.72873058528991,-89.39410231427,81.640904005726));
#127371=CARTESIAN_POINT('Ctrl Pts',(-8.58890642680991,-88.20699181858,83.0342999759601));
#127372=CARTESIAN_POINT('Ctrl Pts',(-8.46279625181091,-87.48612778525,83.61026163649));
#127373=CARTESIAN_POINT('Ctrl Pts',(-8.43880080502891,-87.3536321469,83.70816700881));
#127374=CARTESIAN_POINT('Ctrl Pts',(-9.63185731428291,-89.5539832136501,
72.781364998818));
#127375=CARTESIAN_POINT('Ctrl Pts',(-9.62954009343191,-89.56450050364,73.6635123434199));
#127376=CARTESIAN_POINT('Ctrl Pts',(-9.67979255886791,-89.43456846233,75.636780916767));
#127377=CARTESIAN_POINT('Ctrl Pts',(-9.83705040271291,-88.79415684226,78.3069686379569));
#127378=CARTESIAN_POINT('Ctrl Pts',(-9.87680294572491,-87.68882950106,80.657534553207));
#127379=CARTESIAN_POINT('Ctrl Pts',(-9.79176044324591,-86.54376161791,82.044574788622));
#127380=CARTESIAN_POINT('Ctrl Pts',(-9.71654265497591,-85.8444122705301,
82.648215408587));
#127381=CARTESIAN_POINT('Ctrl Pts',(-9.70229630805891,-85.7156408435,82.752331765737));
#127382=CARTESIAN_POINT('Ctrl Pts',(-11.6048653665117,-88.41503849039,72.8136299831037));
#127383=CARTESIAN_POINT('Ctrl Pts',(-11.603416364145,-88.42440730528,73.5597250211369));
#127384=CARTESIAN_POINT('Ctrl Pts',(-11.6311458484653,-88.31057472766,75.224087177656));
#127385=CARTESIAN_POINT('Ctrl Pts',(-11.7273886361771,-87.6975782204,77.663686258094));
#127386=CARTESIAN_POINT('Ctrl Pts',(-11.7590758209942,-86.56104819585,80.0401709969071));
#127387=CARTESIAN_POINT('Ctrl Pts',(-11.6945650537626,-85.38232181583,81.564678001863));
#127388=CARTESIAN_POINT('Ctrl Pts',(-11.6272962250143,-84.6579922825401,
82.281183093728));
#127389=CARTESIAN_POINT('Ctrl Pts',(-11.6140949378786,-84.52426756057,82.407140345955));
#127390=CARTESIAN_POINT('',(-11.2182878249493,-84.8936697055269,82.3980269273797));
#127391=CARTESIAN_POINT('Origin',(-15.2669619786145,-88.9999686914874,87.1938529810033));
#127392=CARTESIAN_POINT('Ctrl Pts',(-11.2182787039429,-84.89366045326,82.398016121838));
#127393=CARTESIAN_POINT('Ctrl Pts',(-11.3430626531798,-85.3496693368457,
81.9024669884646));
#127394=CARTESIAN_POINT('Ctrl Pts',(-11.4164398924616,-85.7961369782742,
81.3484093064796));
#127395=CARTESIAN_POINT('Ctrl Pts',(-11.4782992679321,-86.4220082696662,
80.4300644193753));
#127396=CARTESIAN_POINT('Ctrl Pts',(-11.4902933546158,-86.6235627591728,
80.1091043375985));
#127397=CARTESIAN_POINT('Ctrl Pts',(-11.4960118930784,-86.9113210240422,
79.6062440989535));
#127398=CARTESIAN_POINT('Ctrl Pts',(-11.4959454832308,-87.0047852362595,
79.4351079792639));
#127399=CARTESIAN_POINT('Ctrl Pts',(-11.4931937770432,-87.1408527017736,
79.1732045109814));
#127400=CARTESIAN_POINT('Ctrl Pts',(-11.4911535852368,-87.207857804048,
79.0409473814055));
#127401=CARTESIAN_POINT('Ctrl Pts',(-11.4876778074931,-87.2841422644907,
78.8843632165692));
#127402=CARTESIAN_POINT('Ctrl Pts',(-11.4856711248064,-87.3218005338773,
78.8055014690377));
#127403=CARTESIAN_POINT('Ctrl Pts',(-11.4845249525581,-87.3418433962271,
78.7631016647935));
#127404=CARTESIAN_POINT('Ctrl Pts',(-11.4839708080131,-87.351160796497,
78.7432736154725));
#127405=CARTESIAN_POINT('Ctrl Pts',(-11.4836494562678,-87.3564761847352,
78.7319331490591));
#127406=CARTESIAN_POINT('Ctrl Pts',(-11.4835239494247,-87.3585369885875,
78.7275313025709));
#127407=CARTESIAN_POINT('Ctrl Pts',(-11.4788357164147,-87.4352505833193,
78.5635820136977));
#127408=CARTESIAN_POINT('Ctrl Pts',(-11.4691050177157,-87.5706949678135,
78.2721609350838));
#127409=CARTESIAN_POINT('Ctrl Pts',(-11.436532125925,-87.8206224854711,
77.6267037058662));
#127410=CARTESIAN_POINT('Ctrl Pts',(-11.422499106422,-87.9113251064847,
77.3766987634165));
#127411=CARTESIAN_POINT('Ctrl Pts',(-11.3963228623726,-88.0493517436767,
76.9476848439182));
#127412=CARTESIAN_POINT('Ctrl Pts',(-11.3867564782335,-88.0956584606176,
76.7956922087132));
#127413=CARTESIAN_POINT('Ctrl Pts',(-11.3713368768106,-88.1642089966755,
76.5540216285056));
#127414=CARTESIAN_POINT('Ctrl Pts',(-11.3633625248204,-88.1982545023846,
76.4297665144432));
#127415=CARTESIAN_POINT('Ctrl Pts',(-11.3536733662997,-88.2372497858451,
76.2787824303504));
#127416=CARTESIAN_POINT('Ctrl Pts',(-11.3487450162542,-88.2565240599301,
76.2017818743169));
#127417=CARTESIAN_POINT('Ctrl Pts',(-11.3466164315199,-88.2647320395063,
76.1684580009983));
#127418=CARTESIAN_POINT('Ctrl Pts',(-11.3451939196021,-88.2701918684418,
76.1461701194819));
#127419=CARTESIAN_POINT('Ctrl Pts',(-11.3443530684592,-88.273401943246,
76.1329833439319));
#127420=CARTESIAN_POINT('Ctrl Pts',(-11.3062141912186,-88.4184339482895,
75.5343934562496));
#127421=CARTESIAN_POINT('Ctrl Pts',(-11.2748698034577,-88.5118391686237,
74.9752281112511));
#127422=CARTESIAN_POINT('Ctrl Pts',(-11.2346789802457,-88.6282672494248,
73.9272753026554));
#127423=CARTESIAN_POINT('Ctrl Pts',(-11.2248258049113,-88.6512540350557,
73.4383979205486));
#127424=CARTESIAN_POINT('Ctrl Pts',(-11.2240831851649,-88.65122976349,72.9889532029839));
#127425=CARTESIAN_POINT('Ctrl Pts',(-8.11808175007291,-89.52553005688,84.97626614071));
#127426=CARTESIAN_POINT('Ctrl Pts',(-7.99010363327091,-89.1241947504099,
85.35070169572));
#127427=CARTESIAN_POINT('Ctrl Pts',(-7.69938772208291,-88.16991851438,86.15798661873));
#127428=CARTESIAN_POINT('Ctrl Pts',(-7.30474282753991,-86.6999882338099,
87.1516158381));
#127429=CARTESIAN_POINT('Ctrl Pts',(-7.05497526331491,-85.61835734781,87.73595158981));
#127430=CARTESIAN_POINT('Ctrl Pts',(-6.95502900065691,-85.15297983312,87.96387367036));
#127431=CARTESIAN_POINT('Ctrl Pts',(-8.41172030319291,-87.7346806391301,
83.6065321030901));
#127432=CARTESIAN_POINT('Ctrl Pts',(-8.32326273657991,-87.3770388479801,
83.93232607158));
#127433=CARTESIAN_POINT('Ctrl Pts',(-8.12258789573591,-86.52944513715,84.63393589531));
#127434=CARTESIAN_POINT('Ctrl Pts',(-7.85094891605191,-85.2321620574,85.49666769891));
#127435=CARTESIAN_POINT('Ctrl Pts',(-7.67942255015891,-84.28177895711,86.00440541648));
#127436=CARTESIAN_POINT('Ctrl Pts',(-7.61083400787491,-83.8734210634099,
86.202573254));
#127437=CARTESIAN_POINT('Ctrl Pts',(-9.60750379728591,-86.06450877549,82.631770479613));
#127438=CARTESIAN_POINT('Ctrl Pts',(-9.55206217138891,-85.75017345838,82.9238877548731));
#127439=CARTESIAN_POINT('Ctrl Pts',(-9.42634334149491,-85.00709560531,83.5526574662701));
#127440=CARTESIAN_POINT('Ctrl Pts',(-9.25633058814091,-83.87535919677,84.32611853891));
#127441=CARTESIAN_POINT('Ctrl Pts',(-9.14905898422491,-83.04894649912,84.7822283658801));
#127442=CARTESIAN_POINT('Ctrl Pts',(-9.10617448690291,-82.6941779,84.96045202937));
#127443=CARTESIAN_POINT('Ctrl Pts',(-11.4777197527979,-84.8330644961,82.237604660585));
#127444=CARTESIAN_POINT('Ctrl Pts',(-11.4425022483259,-84.5534017806,82.517423172522));
#127445=CARTESIAN_POINT('Ctrl Pts',(-11.3623805326309,-83.89277021298,83.12005866634));
#127446=CARTESIAN_POINT('Ctrl Pts',(-11.2532616833429,-82.88795497252,83.86287547546));
#127447=CARTESIAN_POINT('Ctrl Pts',(-11.1840224014209,-82.15462766988,84.30215902993));
#127448=CARTESIAN_POINT('Ctrl Pts',(-11.1562934646479,-81.83981305517,84.47404654791));
#127449=CARTESIAN_POINT('Ctrl Pts',(-10.5124540782072,-82.2723839409002,
84.5902798667472));
#127450=CARTESIAN_POINT('Ctrl Pts',(-10.5589860307587,-82.4505577062519,
84.4766884517136));
#127451=CARTESIAN_POINT('Ctrl Pts',(-10.6048707416816,-82.6240058202091,
84.3601665283034));
#127452=CARTESIAN_POINT('Ctrl Pts',(-10.6498634719091,-82.7927321454252,
84.241090889674));
#127453=CARTESIAN_POINT('Ctrl Pts',(-10.6647639335523,-82.8486100644659,
84.2016560303743));
#127454=CARTESIAN_POINT('Ctrl Pts',(-10.6795667719249,-82.9039704873559,
84.1619410628824));
#127455=CARTESIAN_POINT('Ctrl Pts',(-10.6942637014701,-82.9588146439936,
84.1219596015313));
#127456=CARTESIAN_POINT('Ctrl Pts',(-10.7011862115472,-82.9846471980538,
84.1031276361028));
#127457=CARTESIAN_POINT('Ctrl Pts',(-10.7080853830463,-83.0103652957587,
84.0842364087212));
#127458=CARTESIAN_POINT('Ctrl Pts',(-10.7149605779035,-83.0359688607419,
84.0652873462258));
#127459=CARTESIAN_POINT('Ctrl Pts',(-10.7374211071262,-83.1196129801387,
84.0033827775899));
#127460=CARTESIAN_POINT('Ctrl Pts',(-10.7596256252642,-83.2020345828744,
83.9408609130829));
#127461=CARTESIAN_POINT('Ctrl Pts',(-10.7815513942294,-83.2832401218694,
83.8777695031336));
#127462=CARTESIAN_POINT('Ctrl Pts',(-10.7958700307634,-83.3362714476698,
83.8365676201386));
#127463=CARTESIAN_POINT('Ctrl Pts',(-10.8100698415077,-83.3887839747292,
83.7951229639608));
#127464=CARTESIAN_POINT('Ctrl Pts',(-10.8241461578732,-83.4407780456636,
83.7534493364609));
#127465=CARTESIAN_POINT('Ctrl Pts',(-10.8311843160559,-83.4667750811308,
83.732612522711));
#127466=CARTESIAN_POINT('Ctrl Pts',(-10.8381916040485,-83.4926425056323,
83.7117184715802));
#127467=CARTESIAN_POINT('Ctrl Pts',(-10.8451674543059,-83.5183804254234,
83.6907689146438));
#127468=CARTESIAN_POINT('Ctrl Pts',(-10.8507162070296,-83.5388529624296,
83.6741051522605));
#127469=CARTESIAN_POINT('Ctrl Pts',(-10.8564229129647,-83.5599006965701,
83.6568664032067));
#127470=CARTESIAN_POINT('Ctrl Pts',(-10.8618629080467,-83.5799551092879,
83.640341318734));
#127471=CARTESIAN_POINT('Ctrl Pts',(-10.8632620339316,-83.5851129536458,
83.6360911910982));
#127472=CARTESIAN_POINT('Ctrl Pts',(-10.8646435212819,-83.5902052797057,
83.6318884682935));
#127473=CARTESIAN_POINT('Ctrl Pts',(-10.8660001538151,-83.5952057823778,
83.6277554717686));
#127474=CARTESIAN_POINT('Ctrl Pts',(-10.8932821168994,-83.6957661964699,
83.5446406592721));
#127475=CARTESIAN_POINT('Ctrl Pts',(-10.9215231939352,-83.7996244495179,
83.4562915788775));
#127476=CARTESIAN_POINT('Ctrl Pts',(-10.9505677005548,-83.9063897436635,
83.3623391081002));
#127477=CARTESIAN_POINT('Ctrl Pts',(-10.9741423207597,-83.9930481707976,
83.2860804942117));
#127478=CARTESIAN_POINT('Ctrl Pts',(-10.9982461043705,-84.0816211316533,
83.2061296345882));
#127479=CARTESIAN_POINT('Ctrl Pts',(-11.0227911613409,-84.1718808298857,
83.1222729447451));
#127480=CARTESIAN_POINT('Ctrl Pts',(-11.0523588430011,-84.2806102586782,
83.0212567640396));
#127481=CARTESIAN_POINT('Ctrl Pts',(-11.0825673448688,-84.391789165629,
82.9145725157852));
#127482=CARTESIAN_POINT('Ctrl Pts',(-11.1132477111449,-84.5049638728565,
82.8018482205845));
#127483=CARTESIAN_POINT('Ctrl Pts',(-11.1434088030221,-84.6162230642284,
82.6910318178809));
#127484=CARTESIAN_POINT('Ctrl Pts',(-11.1740259596734,-84.729411220195,
82.5743778595687));
#127485=CARTESIAN_POINT('Ctrl Pts',(-11.2049266350637,-84.8440507040571,
82.4515174287385));
#127486=CARTESIAN_POINT('Ctrl Pts',(-11.2093777150624,-84.8605639196173,
82.4338200289442));
#127487=CARTESIAN_POINT('Ctrl Pts',(-11.2138346564853,-84.8771071660355,
82.4159938285928));
#127488=CARTESIAN_POINT('Ctrl Pts',(-11.2182969218548,-84.8936789311703,
82.398037702481));
#127489=CARTESIAN_POINT('Ctrl Pts',(-8.78823419897191,-74.82614074722,86.78284890078));
#127490=CARTESIAN_POINT('Ctrl Pts',(-8.7830641547019,-75.27337593527,86.78841383868));
#127491=CARTESIAN_POINT('Ctrl Pts',(-8.81909035363991,-76.30222111183,86.7513931298999));
#127492=CARTESIAN_POINT('Ctrl Pts',(-9.02657683691191,-77.8128025443,86.5260662143401));
#127493=CARTESIAN_POINT('Ctrl Pts',(-9.35664843786591,-79.26654580558,86.1326423177499));
#127494=CARTESIAN_POINT('Ctrl Pts',(-9.6889294635519,-80.5040342907,85.6588740936));
#127495=CARTESIAN_POINT('Ctrl Pts',(-9.98045484240391,-81.56707970974,85.1378870544099));
#127496=CARTESIAN_POINT('Ctrl Pts',(-10.1467265870689,-82.21888736454,84.7499607329399));
#127497=CARTESIAN_POINT('Ctrl Pts',(-10.2190780893279,-82.52447496234,84.5512375554));
#127498=CARTESIAN_POINT('Ctrl Pts',(-10.2208467462859,-82.53195984062,84.54635981205));
#127499=CARTESIAN_POINT('Ctrl Pts',(-9.36200580719791,-74.83444576085,86.7229059112));
#127500=CARTESIAN_POINT('Ctrl Pts',(-9.35704322394791,-75.26072541529,86.72795887141));
#127501=CARTESIAN_POINT('Ctrl Pts',(-9.39143229143391,-76.2407078089901,
86.69443228383));
#127502=CARTESIAN_POINT('Ctrl Pts',(-9.59050034074491,-77.69241237804,86.4878381930401));
#127503=CARTESIAN_POINT('Ctrl Pts',(-9.91209801158591,-79.1100671474,86.11982387127));
#127504=CARTESIAN_POINT('Ctrl Pts',(-10.2428814792609,-80.34262221862,85.66384781911));
#127505=CARTESIAN_POINT('Ctrl Pts',(-10.5367862747679,-81.4145391991,85.1527501983101));
#127506=CARTESIAN_POINT('Ctrl Pts',(-10.7064485902869,-82.07950817142,84.76549076934));
#127507=CARTESIAN_POINT('Ctrl Pts',(-10.7804334814949,-82.39193104589,84.56605530898));
#127508=CARTESIAN_POINT('Ctrl Pts',(-10.7822421679279,-82.39958375107,84.56115953279));
#127509=CARTESIAN_POINT('Ctrl Pts',(-9.69871563901291,-74.8448186684699,
86.25448988185));
#127510=CARTESIAN_POINT('Ctrl Pts',(-9.69387480135591,-75.24465675332,86.25906511337));
#127511=CARTESIAN_POINT('Ctrl Pts',(-9.72730314117991,-76.16342344133,86.22876881924));
#127512=CARTESIAN_POINT('Ctrl Pts',(-9.92143095043291,-77.53286478316,86.04033581316));
#127513=CARTESIAN_POINT('Ctrl Pts',(-10.2380558140759,-78.88352999808,85.69971076668));
#127514=CARTESIAN_POINT('Ctrl Pts',(-10.5679604608069,-80.07432532315,85.2691364616501));
#127515=CARTESIAN_POINT('Ctrl Pts',(-10.8632615836509,-81.11812953757,84.78024447856));
#127516=CARTESIAN_POINT('Ctrl Pts',(-11.0349136081859,-81.77043206243,84.4055551387));
#127517=CARTESIAN_POINT('Ctrl Pts',(-11.1098570308209,-82.07731007429,84.21193509085));
#127518=CARTESIAN_POINT('Ctrl Pts',(-11.1116892079909,-82.0848272083201,
84.20718173107));
#127519=CARTESIAN_POINT('Ctrl Pts',(-9.5727563378399,-74.8503092594,85.69145592527));
#127520=CARTESIAN_POINT('Ctrl Pts',(-9.56786995654791,-75.23593651453,85.69590777201));
#127521=CARTESIAN_POINT('Ctrl Pts',(-9.6016576936139,-76.12215123656,85.6664135340699));
#127522=CARTESIAN_POINT('Ctrl Pts',(-9.79763359022991,-77.44106222501,85.48340131111));
#127523=CARTESIAN_POINT('Ctrl Pts',(-10.1161187242309,-78.73872216599,85.1537934685601));
#127524=CARTESIAN_POINT('Ctrl Pts',(-10.4463521278369,-79.87891190224,84.73921042734));
#127525=CARTESIAN_POINT('Ctrl Pts',(-10.7411309005779,-80.876455559,84.26996174785));
#127526=CARTESIAN_POINT('Ctrl Pts',(-10.9120385977019,-81.49875083394,83.9113232946299));
#127527=CARTESIAN_POINT('Ctrl Pts',(-10.9866234446819,-81.79141909568,83.7261498249799));
#127528=CARTESIAN_POINT('Ctrl Pts',(-10.9884468342349,-81.79858809794,83.72160390688));
#127529=CARTESIAN_POINT('Ctrl Pts',(-9.44679703666692,-74.85579985033,85.12842196869));
#127530=CARTESIAN_POINT('Ctrl Pts',(-9.44186511173891,-75.2272162757499,
85.13275043066));
#127531=CARTESIAN_POINT('Ctrl Pts',(-9.47601224604791,-76.0808790318,85.10405824889));
#127532=CARTESIAN_POINT('Ctrl Pts',(-9.67383623002691,-77.34925966686,84.92646680905));
#127533=CARTESIAN_POINT('Ctrl Pts',(-9.99418163438691,-78.5939143339,84.60787617043));
#127534=CARTESIAN_POINT('Ctrl Pts',(-10.3247437948669,-79.68349848133,84.20928439302));
#127535=CARTESIAN_POINT('Ctrl Pts',(-10.6190002175039,-80.63478158042,83.75967901714));
#127536=CARTESIAN_POINT('Ctrl Pts',(-10.7891635872179,-81.22706960545,83.41709145055));
#127537=CARTESIAN_POINT('Ctrl Pts',(-10.8633898585419,-81.50552811708,83.2403645591));
#127538=CARTESIAN_POINT('Ctrl Pts',(-10.8652044604789,-81.51234898755,83.23602608269));
#127539=CARTESIAN_POINT('Ctrl Pts',(-8.94256573703792,-74.85272923674,84.84802251592));
#127540=CARTESIAN_POINT('Ctrl Pts',(-8.93745149507291,-75.23168732494,84.85266460914));
#127541=CARTESIAN_POINT('Ctrl Pts',(-8.97303734281391,-76.1032728097299,
84.82180884061));
#127542=CARTESIAN_POINT('Ctrl Pts',(-9.17825945844692,-77.38671306824,84.63326576812));
#127543=CARTESIAN_POINT('Ctrl Pts',(-9.50605176455791,-78.6278621281099,
84.30193835036));
#127544=CARTESIAN_POINT('Ctrl Pts',(-9.83792998113391,-79.6919023574,83.89921264773));
#127545=CARTESIAN_POINT('Ctrl Pts',(-10.1300953690529,-80.60977329784,83.45352654133));
#127546=CARTESIAN_POINT('Ctrl Pts',(-10.2972791003129,-81.17481917682,83.1197160038201));
#127547=CARTESIAN_POINT('Ctrl Pts',(-10.3700699471209,-81.4399240801001,
82.9484073536091));
#127548=CARTESIAN_POINT('Ctrl Pts',(-10.3718493710999,-81.44641751861,82.94420235099));
#127549=CARTESIAN_POINT('Ctrl Pts',(-8.3979150344609,-74.84315483705,85.03813500131));
#127550=CARTESIAN_POINT('Ctrl Pts',(-8.3926038608449,-75.24635390287,85.0433175979099));
#127551=CARTESIAN_POINT('Ctrl Pts',(-8.42974374991891,-76.17432795641,85.0087822784299));
#127552=CARTESIAN_POINT('Ctrl Pts',(-8.6429570346969,-77.52832734109,84.8002531342));
#127553=CARTESIAN_POINT('Ctrl Pts',(-8.9787931894819,-78.8178193399,84.4409690414599));
#127554=CARTESIAN_POINT('Ctrl Pts',(-9.31209295778892,-79.89849263975,84.01675409896));
#127555=CARTESIAN_POINT('Ctrl Pts',(-9.6019996927279,-80.81818713473,83.5566371803699));
#127556=CARTESIAN_POINT('Ctrl Pts',(-9.76596493640291,-81.37700916158,83.21844889811));
#127557=CARTESIAN_POINT('Ctrl Pts',(-9.83720529443491,-81.63856398261,83.04589974118));
#127558=CARTESIAN_POINT('Ctrl Pts',(-9.83894672057291,-81.64497007984,83.04166481234));
#127559=CARTESIAN_POINT('Origin',(-10.0948648922209,-81.92420577264,83.87306935796));
#127560=CARTESIAN_POINT('Ctrl Pts',(-9.07682613029074,-75.0000006725783,
86.7031078141421));
#127561=CARTESIAN_POINT('Ctrl Pts',(-9.10399999504518,-74.9999907514271,
86.6903141483888));
#127562=CARTESIAN_POINT('Ctrl Pts',(-9.13088724151304,-74.9999811036892,
86.6759898162106));
#127563=CARTESIAN_POINT('Ctrl Pts',(-9.1572412637087,-74.999971777649,86.6601431358597));
#127564=CARTESIAN_POINT('Ctrl Pts',(-9.18329122530418,-74.9999625592083,
86.6444792872262));
#127565=CARTESIAN_POINT('Ctrl Pts',(-9.20881934010855,-74.9999536552907,
86.6273278788702));
#127566=CARTESIAN_POINT('Ctrl Pts',(-9.23358406665683,-74.9999451130034,
86.6087473498612));
#127567=CARTESIAN_POINT('Ctrl Pts',(-9.25813552876659,-74.9999366442791,
86.5903268293255));
#127568=CARTESIAN_POINT('Ctrl Pts',(-9.28193582084024,-74.9999285311918,
86.5705018011061));
#127569=CARTESIAN_POINT('Ctrl Pts',(-9.30475915361208,-74.9999208170244,
86.5493793145265));
#127570=CARTESIAN_POINT('Ctrl Pts',(-9.32745319920907,-74.9999131465553,
86.5283764803502));
#127571=CARTESIAN_POINT('Ctrl Pts',(-9.34918050304556,-74.9999058706931,
86.506091191989));
#127572=CARTESIAN_POINT('Ctrl Pts',(-9.3697412764515,-74.9998990263766,
86.4826751026726));
#127573=CARTESIAN_POINT('Ctrl Pts',(-9.39024645363464,-74.9998922005671,
86.4593223303381));
#127574=CARTESIAN_POINT('Ctrl Pts',(-9.40959070386907,-74.9998858041356,
86.434845429367));
#127575=CARTESIAN_POINT('Ctrl Pts',(-9.4276093994838,-74.9998798654377,
86.4094343007998));
#127576=CARTESIAN_POINT('Ctrl Pts',(-9.44563283269752,-74.9998739251784,
86.3840164909646));
#127577=CARTESIAN_POINT('Ctrl Pts',(-9.46232950020998,-74.9998684430116,
86.3576647027707));
#127578=CARTESIAN_POINT('Ctrl Pts',(-9.47757741530284,-74.9998634368882,
86.330598712092));
#127579=CARTESIAN_POINT('Ctrl Pts',(-9.49293759605705,-74.9998583939063,
86.3033334429334));
#127580=CARTESIAN_POINT('Ctrl Pts',(-9.50682728712112,-74.9998538340757,
86.2753442715325));
#127581=CARTESIAN_POINT('Ctrl Pts',(-9.51917165228492,-74.9998497636995,
86.2468739512399));
#127582=CARTESIAN_POINT('Ctrl Pts',(-9.53159872212772,-74.9998456660525,
86.218212885723));
#127583=CARTESIAN_POINT('Ctrl Pts',(-9.54245964807191,-74.9998420644443,
86.189065122376));
#127584=CARTESIAN_POINT('Ctrl Pts',(-9.55173123092076,-74.9998389525596,
86.1596830567581));
#127585=CARTESIAN_POINT('Ctrl Pts',(-9.56108916788417,-74.9998358116912,
86.1300273310433));
#127586=CARTESIAN_POINT('Ctrl Pts',(-9.56882823591605,-74.9998331696532,
86.1001338087774));
#127587=CARTESIAN_POINT('Ctrl Pts',(-9.57497724561255,-74.9998310074135,
86.0702529880118));
#127588=CARTESIAN_POINT('Ctrl Pts',(-9.58119948158175,-74.9998288194246,
86.0400163276497));
#127589=CARTESIAN_POINT('Ctrl Pts',(-9.58579401693701,-74.9998271226158,
86.0097934597263));
#127590=CARTESIAN_POINT('Ctrl Pts',(-9.58883927510594,-74.9998258857931,
85.9798218969432));
#127591=CARTESIAN_POINT('Ctrl Pts',(-9.59195555286494,-74.9998246201261,
85.9491513562788));
#127592=CARTESIAN_POINT('Ctrl Pts',(-9.59345005338149,-74.9998238360011,
85.9187446672511));
#127593=CARTESIAN_POINT('Ctrl Pts',(-9.5934493444679,-74.9998234900437,
85.8888219184142));
#127594=CARTESIAN_POINT('Ctrl Pts',(-9.59344862496583,-74.999823138919,
85.8584522370923));
#127595=CARTESIAN_POINT('Ctrl Pts',(-9.59190851333374,-74.9998232389509,
85.8285814699716));
#127596=CARTESIAN_POINT('Ctrl Pts',(-9.58899358054596,-74.9998237373645,
85.7993962358241));
#127597=CARTESIAN_POINT('Ctrl Pts',(-9.58600511871662,-74.9998242483505,
85.7694748055271));
#127598=CARTESIAN_POINT('Ctrl Pts',(-9.58157246621915,-74.9998251778617,
85.7402741621824));
#127599=CARTESIAN_POINT('Ctrl Pts',(-9.5758936539825,-74.9998264644108,
85.7119449365536));
#127600=CARTESIAN_POINT('Ctrl Pts',(-9.57457467685541,-74.9998267632284,
85.705365109809));
#127601=CARTESIAN_POINT('Ctrl Pts',(-9.57318852871841,-74.9998270812952,
85.6988320763153));
#127602=CARTESIAN_POINT('Ctrl Pts',(-9.57173776914569,-74.9998274178246,
85.6923473348233));
#127603=CARTESIAN_POINT('Ctrl Pts',(-9.56551370279836,-74.9998288616072,
85.6645264180766));
#127604=CARTESIAN_POINT('Ctrl Pts',(-9.55783270403854,-74.9998306249665,
85.6364049762161));
#127605=CARTESIAN_POINT('Ctrl Pts',(-9.54857347396069,-74.9998327271977,
85.6081918997131));
#127606=CARTESIAN_POINT('Ctrl Pts',(-9.53951690601265,-74.9998347834162,
85.5805963391509));
#127607=CARTESIAN_POINT('Ctrl Pts',(-9.52894976120909,-74.9998371640152,
85.5529135806603));
#127608=CARTESIAN_POINT('Ctrl Pts',(-9.51679285414336,-74.9998398786314,
85.525374443191));
#127609=CARTESIAN_POINT('Ctrl Pts',(-9.50486790627308,-74.9998425414514,
85.4983607647169));
#127610=CARTESIAN_POINT('Ctrl Pts',(-9.49141274535437,-74.9998455258108,
85.4714859248127));
#127611=CARTESIAN_POINT('Ctrl Pts',(-9.47639499415803,-74.9998488301971,
85.444993978127));
#127612=CARTESIAN_POINT('Ctrl Pts',(-9.46162100402897,-74.9998520809482,
85.4189320362478));
#127613=CARTESIAN_POINT('Ctrl Pts',(-9.44533438718281,-74.9998556415217,
85.3932414401984));
#127614=CARTESIAN_POINT('Ctrl Pts',(-9.42755231432449,-74.9998594982772,
85.3681696172929));
#127615=CARTESIAN_POINT('Ctrl Pts',(-9.41000756113224,-74.9998633035605,
85.3434324031075));
#127616=CARTESIAN_POINT('Ctrl Pts',(-9.39100687524507,-74.9998673972163,
85.3192984171782));
#127617=CARTESIAN_POINT('Ctrl Pts',(-9.37061743520078,-74.999871753094,
85.2960079213209));
#127618=CARTESIAN_POINT('Ctrl Pts',(-9.34984201493274,-74.9998761914302,
85.2722765270973));
#127619=CARTESIAN_POINT('Ctrl Pts',(-9.32762462572471,-74.9998809020583,
85.2494218850682));
#127620=CARTESIAN_POINT('Ctrl Pts',(-9.30409180453394,-74.9998858428542,
85.2276865690306));
#127621=CARTESIAN_POINT('Ctrl Pts',(-9.28144013241718,-74.9998905986497,
85.2067650973445));
#127622=CARTESIAN_POINT('Ctrl Pts',(-9.25757030985327,-74.9998955675488,
85.186881423829));
#127623=CARTESIAN_POINT('Ctrl Pts',(-9.23264164306874,-74.9999006997037,
85.1682285148043));
#127624=CARTESIAN_POINT('Ctrl Pts',(-9.20779321329438,-74.9999058153399,
85.1496356432322));
#127625=CARTESIAN_POINT('Ctrl Pts',(-9.18189331394207,-74.9999110930441,
85.1322663161802));
#127626=CARTESIAN_POINT('Ctrl Pts',(-9.15513836009451,-74.9999164730492,
85.1162773047068));
#127627=CARTESIAN_POINT('Ctrl Pts',(-9.12839924598703,-74.9999218498692,
85.1002977592108));
#127628=CARTESIAN_POINT('Ctrl Pts',(-9.10080683593486,-74.9999273286825,
85.0856974009578));
#127629=CARTESIAN_POINT('Ctrl Pts',(-9.07258596059659,-74.9999328418655,
85.0725893291592));
#127630=CARTESIAN_POINT('Ctrl Pts',(-9.04430746240289,-74.9999383663057,
85.0594544926158));
#127631=CARTESIAN_POINT('Ctrl Pts',(-9.01539879073536,-74.9999439250373,
85.0478183180839));
#127632=CARTESIAN_POINT('Ctrl Pts',(-8.9861029073353,-74.9999494450838,
85.0377450762627));
#127633=CARTESIAN_POINT('Ctrl Pts',(-8.95654791083695,-74.9999550139534,
85.0275827397088));
#127634=CARTESIAN_POINT('Ctrl Pts',(-8.92659973489103,-74.9999605432158,
85.0190111633963));
#127635=CARTESIAN_POINT('Ctrl Pts',(-8.89651140595007,-74.999965956364,
85.0120433514983));
#127636=CARTESIAN_POINT('Ctrl Pts',(-8.86622517470663,-74.9999714051166,
85.0050297096699));
#127637=CARTESIAN_POINT('Ctrl Pts',(-8.83579781987997,-74.9999767359927,
84.9996407568067));
#127638=CARTESIAN_POINT('Ctrl Pts',(-8.80547732474302,-74.9999818729188,
84.995837732317));
#127639=CARTESIAN_POINT('Ctrl Pts',(-8.77474583349687,-74.9999870794761,
84.9919831576049));
#127640=CARTESIAN_POINT('Ctrl Pts',(-8.74412491066357,-74.9999920865798,
84.9897573534694));
#127641=CARTESIAN_POINT('Ctrl Pts',(-8.71384962962935,-74.9999968203932,
84.9890718459364));
#127642=CARTESIAN_POINT('Ctrl Pts',(-8.70698518555899,-74.999997893711,
84.988916417879));
#127643=CARTESIAN_POINT('Ctrl Pts',(-8.70013839104334,-74.9999989530079,
84.9888399980106));
#127644=CARTESIAN_POINT('Ctrl Pts',(-8.69331176399212,-74.9999999974771,
84.9888412596817));
#127645=CARTESIAN_POINT('Ctrl Pts',(-10.2209979427679,-67.46798896641,84.5463096825499));
#127646=CARTESIAN_POINT('Ctrl Pts',(-10.2196132646019,-67.4738480541,84.5501279961));
#127647=CARTESIAN_POINT('Ctrl Pts',(-10.1480245164719,-67.77630330004,84.7469081971199));
#127648=CARTESIAN_POINT('Ctrl Pts',(-9.98388527989691,-68.42046765222,85.1308217788001));
#127649=CARTESIAN_POINT('Ctrl Pts',(-9.69703741833592,-69.46700133775,85.64545920484));
#127650=CARTESIAN_POINT('Ctrl Pts',(-9.37340189687591,-70.6706622866,86.1104956752401));
#127651=CARTESIAN_POINT('Ctrl Pts',(-9.05098927287391,-72.06834247106,86.4981844835201));
#127652=CARTESIAN_POINT('Ctrl Pts',(-8.82755044173492,-73.59330681594,86.7431130017399));
#127653=CARTESIAN_POINT('Ctrl Pts',(-8.7822484149829,-74.66230448112,86.7892411673399));
#127654=CARTESIAN_POINT('Ctrl Pts',(-8.78824703444391,-75.1740212775,86.7828639942899));
#127655=CARTESIAN_POINT('Ctrl Pts',(-10.7823181781539,-67.6003915011101,
84.56103425336));
#127656=CARTESIAN_POINT('Ctrl Pts',(-10.7809021555679,-67.60638197925,84.56486670678));
#127657=CARTESIAN_POINT('Ctrl Pts',(-10.7076960644999,-67.91560684941,84.76235822432));
#127658=CARTESIAN_POINT('Ctrl Pts',(-10.5401996588409,-68.57280682492,85.14564918501));
#127659=CARTESIAN_POINT('Ctrl Pts',(-10.2509568505849,-69.62827488174,85.65066970524));
#127660=CARTESIAN_POINT('Ctrl Pts',(-9.92861982731791,-70.82766304517,86.09858814927));
#127661=CARTESIAN_POINT('Ctrl Pts',(-9.61403567119891,-72.1924890331,86.46193063502));
#127662=CARTESIAN_POINT('Ctrl Pts',(-9.39940208312791,-73.65946242481,86.68685818601));
#127663=CARTESIAN_POINT('Ctrl Pts',(-9.35621111589692,-74.67798882017,86.72863385846));
#127664=CARTESIAN_POINT('Ctrl Pts',(-9.36195895040191,-75.16571991393,86.72284269434));
#127665=CARTESIAN_POINT('Ctrl Pts',(-11.1116938129149,-67.91511854175,84.2070762476901));
#127666=CARTESIAN_POINT('Ctrl Pts',(-11.1102593978189,-67.921002933,84.21079725143));
#127667=CARTESIAN_POINT('Ctrl Pts',(-11.0361042703119,-68.22474376388,84.40253481458));
#127668=CARTESIAN_POINT('Ctrl Pts',(-10.8666379201759,-68.8694457640601,
84.77340996466));
#127669=CARTESIAN_POINT('Ctrl Pts',(-10.5759897874039,-69.89736182966,85.25658866886));
#127670=CARTESIAN_POINT('Ctrl Pts',(-10.2544147065009,-71.05644978244,85.67978174226));
#127671=CARTESIAN_POINT('Ctrl Pts',(-9.94442419660191,-72.3579693818601,
86.01654748832));
#127672=CARTESIAN_POINT('Ctrl Pts',(-9.73495741411192,-73.74276331425,86.22195023037));
#127673=CARTESIAN_POINT('Ctrl Pts',(-9.69300518998291,-74.69786958715,86.25970207886));
#127674=CARTESIAN_POINT('Ctrl Pts',(-9.69860586703891,-75.15534537984,86.25445790011));
#127675=CARTESIAN_POINT('Ctrl Pts',(-10.9884700791849,-68.20132868183,83.72155861371));
#127676=CARTESIAN_POINT('Ctrl Pts',(-10.9870425449669,-68.20694057842,83.7251172404199));
#127677=CARTESIAN_POINT('Ctrl Pts',(-10.9132424644069,-68.49661756483,83.9084902576501));
#127678=CARTESIAN_POINT('Ctrl Pts',(-10.7445130962709,-69.1116606135,84.26347398636));
#127679=CARTESIAN_POINT('Ctrl Pts',(-10.4543907137839,-70.09399590872,84.7272181967299));
#127680=CARTESIAN_POINT('Ctrl Pts',(-10.1325305802749,-71.20375407453,85.13464253368));
#127681=CARTESIAN_POINT('Ctrl Pts',(-9.82082152723193,-72.45392520214,85.4604053674));
#127682=CARTESIAN_POINT('Ctrl Pts',(-9.60942177518391,-73.78740469336,85.6598394857501));
#127683=CARTESIAN_POINT('Ctrl Pts',(-9.56700612105591,-74.7086282923,85.69659181281));
#127684=CARTESIAN_POINT('Ctrl Pts',(-9.5726618516389,-75.14984776556,85.6914891603501));
#127685=CARTESIAN_POINT('Ctrl Pts',(-10.8652463454549,-68.48753882192,83.23604097973));
#127686=CARTESIAN_POINT('Ctrl Pts',(-10.8638256921159,-68.49287822383,83.2394372294));
#127687=CARTESIAN_POINT('Ctrl Pts',(-10.7903806585019,-68.7684913657901,
83.41444570072));
#127688=CARTESIAN_POINT('Ctrl Pts',(-10.6223882723649,-69.35387546295,83.7535380080601));
#127689=CARTESIAN_POINT('Ctrl Pts',(-10.3327916401629,-70.29062998778,84.1978477246001));
#127690=CARTESIAN_POINT('Ctrl Pts',(-10.0106464540489,-71.3510583666101,
84.5895033251));
#127691=CARTESIAN_POINT('Ctrl Pts',(-9.69721885786292,-72.54988102242,84.90426324647));
#127692=CARTESIAN_POINT('Ctrl Pts',(-9.48388613625691,-73.83204607248,85.09772874113));
#127693=CARTESIAN_POINT('Ctrl Pts',(-9.44100705212892,-74.71938699745,85.13348154676));
#127694=CARTESIAN_POINT('Ctrl Pts',(-9.44671783623892,-75.14435015128,85.12852042059));
#127695=CARTESIAN_POINT('Ctrl Pts',(-10.3719730784129,-68.55349464875,82.94422086921));
#127696=CARTESIAN_POINT('Ctrl Pts',(-10.3705799697159,-68.55857769736,82.947512593833));
#127697=CARTESIAN_POINT('Ctrl Pts',(-10.2985562139839,-68.82096881656,83.11714949015));
#127698=CARTESIAN_POINT('Ctrl Pts',(-10.1335140185879,-69.37940206064,83.44752071946));
#127699=CARTESIAN_POINT('Ctrl Pts',(-9.84602200173092,-70.28308242848,83.8878227876));
#127700=CARTESIAN_POINT('Ctrl Pts',(-9.52273573000191,-71.31819837143,84.2832300510801));
#127701=CARTESIAN_POINT('Ctrl Pts',(-9.20242868482291,-72.51202975347,84.60993193985));
#127702=CARTESIAN_POINT('Ctrl Pts',(-8.98135815021491,-73.80812186411,84.81498348635));
#127703=CARTESIAN_POINT('Ctrl Pts',(-8.93662392322791,-74.71381618721,84.8534306707901));
#127704=CARTESIAN_POINT('Ctrl Pts',(-8.9425550904749,-75.14741240926,84.84811080078));
#127705=CARTESIAN_POINT('Ctrl Pts',(-9.83910307039591,-68.35501114641,83.04159391677));
#127706=CARTESIAN_POINT('Ctrl Pts',(-9.83773971744291,-68.36002571887,83.04490899157));
#127707=CARTESIAN_POINT('Ctrl Pts',(-9.76725133045291,-68.61889431212,83.21576580024));
#127708=CARTESIAN_POINT('Ctrl Pts',(-9.60539614775291,-69.17113967145,83.5504287047001));
#127709=CARTESIAN_POINT('Ctrl Pts',(-9.3201776909509,-70.07640947898,84.0048347668901));
#127710=CARTESIAN_POINT('Ctrl Pts',(-8.99565873474091,-71.1271876013501,
84.4210007850601));
#127711=CARTESIAN_POINT('Ctrl Pts',(-8.66792000354691,-72.36572865333,84.77458937839));
#127712=CARTESIAN_POINT('Ctrl Pts',(-8.43849051508591,-73.73165933346,85.0010199440401));
#127713=CARTESIAN_POINT('Ctrl Pts',(-8.39175222654391,-74.69564784935,85.0440503938199));
#127714=CARTESIAN_POINT('Ctrl Pts',(-8.39792146783991,-75.15698307681,85.0381118389));
#127715=CARTESIAN_POINT('Origin',(-10.0948615431041,-68.0757444516113,83.873039637936));
#127716=CARTESIAN_POINT('Ctrl Pts',(-10.1785854175429,-67.85588330056,61.19532449647));
#127717=CARTESIAN_POINT('Ctrl Pts',(-10.1850298753019,-67.82902615816,61.21159366354));
#127718=CARTESIAN_POINT('Ctrl Pts',(-10.2405662560859,-67.59793547837,61.35266188607));
#127719=CARTESIAN_POINT('Ctrl Pts',(-10.3533091174039,-67.13450494732,61.65463623851));
#127720=CARTESIAN_POINT('Ctrl Pts',(-10.5195786451669,-66.45531759647,62.15428395171));
#127721=CARTESIAN_POINT('Ctrl Pts',(-10.6976369657359,-65.72051916043,62.77307815338));
#127722=CARTESIAN_POINT('Ctrl Pts',(-10.8773515530769,-64.95635886287,63.519467755676));
#127723=CARTESIAN_POINT('Ctrl Pts',(-11.0500634386659,-64.18718474885,64.403598938773));
#127724=CARTESIAN_POINT('Ctrl Pts',(-11.2102175450769,-63.4329994378,65.4436382220611));
#127725=CARTESIAN_POINT('Ctrl Pts',(-11.3532874167409,-62.71533896826,66.6679533293209));
#127726=CARTESIAN_POINT('Ctrl Pts',(-11.4749421508609,-62.0659368475,68.113631709785));
#127727=CARTESIAN_POINT('Ctrl Pts',(-11.5688811502722,-61.5357441304,69.820891505791));
#127728=CARTESIAN_POINT('Ctrl Pts',(-11.6237522292211,-61.21258620971,71.773832111478));
#127729=CARTESIAN_POINT('Ctrl Pts',(-11.6284201506308,-61.1848010717,73.857068402466));
#127730=CARTESIAN_POINT('Ctrl Pts',(-11.5808138773938,-61.46645898683,75.861242610505));
#127731=CARTESIAN_POINT('Ctrl Pts',(-11.4904794662569,-61.98015285862,77.637523541923));
#127732=CARTESIAN_POINT('Ctrl Pts',(-11.3699894781989,-62.62857578264,79.142058916883));
#127733=CARTESIAN_POINT('Ctrl Pts',(-11.2268663935649,-63.35208396897,80.410836525289));
#127734=CARTESIAN_POINT('Ctrl Pts',(-11.0656654745509,-64.11575643041,81.484871784862));
#127735=CARTESIAN_POINT('Ctrl Pts',(-10.8912137555179,-64.89642330348,82.395342195428));
#127736=CARTESIAN_POINT('Ctrl Pts',(-10.7089402192919,-65.67337171062,83.1624171289));
#127737=CARTESIAN_POINT('Ctrl Pts',(-10.5277886673999,-66.42174040101,83.7974836243801));
#127738=CARTESIAN_POINT('Ctrl Pts',(-10.3581235993269,-67.1148137986,84.3098671031399));
#127739=CARTESIAN_POINT('Ctrl Pts',(-10.2425760647809,-67.5895814439499,
84.6199517927501));
#127740=CARTESIAN_POINT('Ctrl Pts',(-10.1854502907699,-67.82725682396,84.7651133990399));
#127741=CARTESIAN_POINT('Ctrl Pts',(-10.1785764846769,-67.85590275553,84.7824661081499));
#127742=CARTESIAN_POINT('Ctrl Pts',(-10.7233079330559,-68.00453699972,61.20971563528));
#127743=CARTESIAN_POINT('Ctrl Pts',(-10.7297606902689,-67.9776801853,61.22566612772));
#127744=CARTESIAN_POINT('Ctrl Pts',(-10.7853820779999,-67.74653156878,61.36401929391));
#127745=CARTESIAN_POINT('Ctrl Pts',(-10.8985266262999,-67.28195020988,61.66103214993));
#127746=CARTESIAN_POINT('Ctrl Pts',(-11.0658987462389,-66.59877623104,62.15484889246));
#127747=CARTESIAN_POINT('Ctrl Pts',(-11.2455867209609,-65.85758537412,62.76912806206));
#127748=CARTESIAN_POINT('Ctrl Pts',(-11.4272960177459,-65.08510007019,63.512959516944));
#127749=CARTESIAN_POINT('Ctrl Pts',(-11.6019946953778,-64.30706109192,64.396071768386));
#127750=CARTESIAN_POINT('Ctrl Pts',(-11.7639748214603,-63.54414794216,65.436512178071));
#127751=CARTESIAN_POINT('Ctrl Pts',(-11.9085537069501,-62.81872865971,66.6619954797));
#127752=CARTESIAN_POINT('Ctrl Pts',(-12.0313720955718,-62.1629201997,68.10924847471));
#127753=CARTESIAN_POINT('Ctrl Pts',(-12.1261231817684,-61.6279818110999,
69.8182781818619));
#127754=CARTESIAN_POINT('Ctrl Pts',(-12.1814253595411,-61.30218855351,71.772869650253));
#127755=CARTESIAN_POINT('Ctrl Pts',(-12.1861300800116,-61.27417565406,73.8577126819013));
#127756=CARTESIAN_POINT('Ctrl Pts',(-12.1381497767974,-61.55812922566,75.863657594818));
#127757=CARTESIAN_POINT('Ctrl Pts',(-12.0470505708238,-62.07633100854,77.64164293623));
#127758=CARTESIAN_POINT('Ctrl Pts',(-11.9254239898882,-62.73106818597,79.147840288293));
#127759=CARTESIAN_POINT('Ctrl Pts',(-11.7808009392146,-63.46234925653,80.417907163538));
#127760=CARTESIAN_POINT('Ctrl Pts',(-11.6177839675048,-64.2347707502,81.4923857304049));
#127761=CARTESIAN_POINT('Ctrl Pts',(-11.4413148751619,-65.0244906302599,
82.401998788017));
#127762=CARTESIAN_POINT('Ctrl Pts',(-11.2570027672979,-65.80998285409,83.16660599563));
#127763=CARTESIAN_POINT('Ctrl Pts',(-11.0741741737809,-66.56495328861,83.79717032534));
#127764=CARTESIAN_POINT('Ctrl Pts',(-10.9033624485049,-67.2621908432,84.30367256423));
#127765=CARTESIAN_POINT('Ctrl Pts',(-10.7873948695429,-67.73817520654,84.6086930769));
#127766=CARTESIAN_POINT('Ctrl Pts',(-10.7301812558329,-67.97591244501,84.75106289439));
#127767=CARTESIAN_POINT('Ctrl Pts',(-10.7232986708699,-68.00455776379,84.76807553907));
#127768=CARTESIAN_POINT('Ctrl Pts',(-11.0265915836499,-68.30671850109,61.57813520514));
#127769=CARTESIAN_POINT('Ctrl Pts',(-11.0330489617269,-68.28068236006,61.59340875318));
#127770=CARTESIAN_POINT('Ctrl Pts',(-11.0887176785409,-68.05656087501,61.72591938424));
#127771=CARTESIAN_POINT('Ctrl Pts',(-11.2020858729929,-67.60548761868,62.01090569511));
#127772=CARTESIAN_POINT('Ctrl Pts',(-11.3700718801319,-66.94081207514,62.48616605829));
#127773=CARTESIAN_POINT('Ctrl Pts',(-11.5506671928959,-66.2184602959799,
63.078991875129));
#127774=CARTESIAN_POINT('Ctrl Pts',(-11.7334870785492,-65.46461996317,63.798576759107));
#127775=CARTESIAN_POINT('Ctrl Pts',(-11.9092919369002,-64.70507433139,64.6541034439819));
#127776=CARTESIAN_POINT('Ctrl Pts',(-12.0722887309123,-63.9602739817501,
65.6629970275841));
#127777=CARTESIAN_POINT('Ctrl Pts',(-12.2177077858624,-63.25239876227,66.851736936753));
#127778=CARTESIAN_POINT('Ctrl Pts',(-12.3411740591877,-62.61281265647,68.255713330532));
#127779=CARTESIAN_POINT('Ctrl Pts',(-12.4363772887007,-62.09139235649,69.913585361883));
#127780=CARTESIAN_POINT('Ctrl Pts',(-12.4919194881749,-61.77398372438,71.809446369507));
#127781=CARTESIAN_POINT('Ctrl Pts',(-12.4966446971569,-61.74669107217,73.8315534842725));
#127782=CARTESIAN_POINT('Ctrl Pts',(-12.4484561463053,-62.02333606787,75.777270406522));
#127783=CARTESIAN_POINT('Ctrl Pts',(-12.3569311276225,-62.5283895667699,
77.501952488849));
#127784=CARTESIAN_POINT('Ctrl Pts',(-12.2346717290096,-63.166882314,78.963124476845));
#127785=CARTESIAN_POINT('Ctrl Pts',(-12.0892135463862,-63.88044861778,80.195157982113));
#127786=CARTESIAN_POINT('Ctrl Pts',(-11.9251854560324,-64.63447944362,81.23707495747));
#127787=CARTESIAN_POINT('Ctrl Pts',(-11.7475931563231,-65.4054610954199,
82.118389008027));
#127788=CARTESIAN_POINT('Ctrl Pts',(-11.5621460385589,-66.17204120784,82.858168756855));
#127789=CARTESIAN_POINT('Ctrl Pts',(-11.3783837232079,-66.90787617342,83.46678987785));
#127790=CARTESIAN_POINT('Ctrl Pts',(-11.2069335767679,-67.5862913034,83.95431827718));
#127791=CARTESIAN_POINT('Ctrl Pts',(-11.0907321308349,-68.04845841504,84.24700650097));
#127792=CARTESIAN_POINT('Ctrl Pts',(-11.0334696108579,-68.27896957299,84.38336540787));
#127793=CARTESIAN_POINT('Ctrl Pts',(-11.0265821381089,-68.30673940993,84.39965592943));
#127794=CARTESIAN_POINT('Ctrl Pts',(-10.8914619965499,-68.56616924746,62.0613048488));
#127795=CARTESIAN_POINT('Ctrl Pts',(-10.8979173157779,-68.54124112046,62.07598283942));
#127796=CARTESIAN_POINT('Ctrl Pts',(-10.9535649448759,-68.32666790684,62.20331802211));
#127797=CARTESIAN_POINT('Ctrl Pts',(-11.0668334926369,-67.89498854316,62.47702364874));
#127798=CARTESIAN_POINT('Ctrl Pts',(-11.2345459791829,-67.2592822743,62.93305408088));
#127799=CARTESIAN_POINT('Ctrl Pts',(-11.4147370228249,-66.56876560972,63.5014215856259));
#127800=CARTESIAN_POINT('Ctrl Pts',(-11.5970620799083,-65.84843083062,64.190818954792));
#127801=CARTESIAN_POINT('Ctrl Pts',(-11.7723740737627,-65.1227258372001,
65.010109503435));
#127802=CARTESIAN_POINT('Ctrl Pts',(-11.9349178861608,-64.411115162,65.975997102607));
#127803=CARTESIAN_POINT('Ctrl Pts',(-12.0799625992957,-63.73469249597,67.113945853266));
#127804=CARTESIAN_POINT('Ctrl Pts',(-12.2031402042661,-63.12342146587,68.457901389867));
#127805=CARTESIAN_POINT('Ctrl Pts',(-12.2981419790039,-62.6250033886,70.04491365903));
#127806=CARTESIAN_POINT('Ctrl Pts',(-12.3535772355771,-62.3215537612,71.859806698113));
#127807=CARTESIAN_POINT('Ctrl Pts',(-12.3582933157977,-62.29546158414,73.7955804875104));
#127808=CARTESIAN_POINT('Ctrl Pts',(-12.3101975507498,-62.55994049022,75.658187143643));
#127809=CARTESIAN_POINT('Ctrl Pts',(-12.2188622551049,-63.0427289581601,
77.309177295583));
#127810=CARTESIAN_POINT('Ctrl Pts',(-12.0968848116561,-63.6529689013,78.707879311435));
#127811=CARTESIAN_POINT('Ctrl Pts',(-11.9517987263592,-64.33483804012,79.887258435538));
#127812=CARTESIAN_POINT('Ctrl Pts',(-11.7882211451067,-65.05528272997,80.884756776892));
#127813=CARTESIAN_POINT('Ctrl Pts',(-11.6111292962042,-65.79190488112,81.728709591473));
#127814=CARTESIAN_POINT('Ctrl Pts',(-11.4261878879259,-66.52439984917,82.437426898831));
#127815=CARTESIAN_POINT('Ctrl Pts',(-11.2428415971309,-67.22779009247,83.02091527749));
#127816=CARTESIAN_POINT('Ctrl Pts',(-11.0716759025169,-67.87662086228,83.48870022348));
#127817=CARTESIAN_POINT('Ctrl Pts',(-10.9555786572129,-68.3189106767101,
83.76979752821));
#127818=CARTESIAN_POINT('Ctrl Pts',(-10.8983379276749,-68.53960095533,83.9008303234899));
#127819=CARTESIAN_POINT('Ctrl Pts',(-10.8914526327039,-68.56618904268,83.9164856622999));
#127820=CARTESIAN_POINT('Ctrl Pts',(-10.7563324094499,-68.82561999382,62.54447449247));
#127821=CARTESIAN_POINT('Ctrl Pts',(-10.7627856698279,-68.80179988086,62.5585569256599));
#127822=CARTESIAN_POINT('Ctrl Pts',(-10.8184122112099,-68.59677493867,62.68071665998));
#127823=CARTESIAN_POINT('Ctrl Pts',(-10.9315811122809,-68.1844894676501,
62.94314160236));
#127824=CARTESIAN_POINT('Ctrl Pts',(-11.0990200782339,-67.57775247346,63.379942103459));
#127825=CARTESIAN_POINT('Ctrl Pts',(-11.2788068527549,-66.91907092346,63.923851296123));
#127826=CARTESIAN_POINT('Ctrl Pts',(-11.4606370812679,-66.23224169808,64.583061150478));
#127827=CARTESIAN_POINT('Ctrl Pts',(-11.6354562106252,-65.540377343,65.366115562889));
#127828=CARTESIAN_POINT('Ctrl Pts',(-11.7975470414093,-64.86195634224,66.288997177629));
#127829=CARTESIAN_POINT('Ctrl Pts',(-11.942217412729,-64.21698622967,67.37615476978));
#127830=CARTESIAN_POINT('Ctrl Pts',(-12.0651063493446,-63.63403027526,68.660089449201));
#127831=CARTESIAN_POINT('Ctrl Pts',(-12.1599066693072,-63.15861442072,70.176241956177));
#127832=CARTESIAN_POINT('Ctrl Pts',(-12.2152349829793,-62.86912379802,71.910167026718));
#127833=CARTESIAN_POINT('Ctrl Pts',(-12.2199419344384,-62.84423209612,73.7596074907483));
#127834=CARTESIAN_POINT('Ctrl Pts',(-12.1719389551942,-63.09654491258,75.539103880765));
#127835=CARTESIAN_POINT('Ctrl Pts',(-12.0807933825874,-63.5570683495501,
77.116402102318));
#127836=CARTESIAN_POINT('Ctrl Pts',(-11.9590978943026,-64.13905548859,78.452634146025));
#127837=CARTESIAN_POINT('Ctrl Pts',(-11.8143839063321,-64.78922746246,79.579358888962));
#127838=CARTESIAN_POINT('Ctrl Pts',(-11.6512568341809,-65.47608601633,80.532438596313));
#127839=CARTESIAN_POINT('Ctrl Pts',(-11.4746654360849,-66.17834866682,81.339030174918));
#127840=CARTESIAN_POINT('Ctrl Pts',(-11.2902297372939,-66.87675849051,82.0166850408071));
#127841=CARTESIAN_POINT('Ctrl Pts',(-11.1072994710539,-67.54770401151,82.57504067714));
#127842=CARTESIAN_POINT('Ctrl Pts',(-10.9364182282669,-68.16695042115,83.02308216978));
#127843=CARTESIAN_POINT('Ctrl Pts',(-10.8204251835919,-68.58936293838,83.2925885554499));
#127844=CARTESIAN_POINT('Ctrl Pts',(-10.7632062444909,-68.80023233767,83.4182952391));
#127845=CARTESIAN_POINT('Ctrl Pts',(-10.7563231272989,-68.82563867543,83.43331539516));
#127846=CARTESIAN_POINT('Ctrl Pts',(-10.2705525273999,-68.8738338756999,
62.8285888422));
#127847=CARTESIAN_POINT('Ctrl Pts',(-10.2769983863809,-68.85068949284,62.84254390307));
#127848=CARTESIAN_POINT('Ctrl Pts',(-10.3325491191389,-68.6515326229,62.96355658686));
#127849=CARTESIAN_POINT('Ctrl Pts',(-10.4453597984549,-68.2519310358,63.222773199426));
#127850=CARTESIAN_POINT('Ctrl Pts',(-10.6118154801089,-67.66581941013,63.652159528043));
#127851=CARTESIAN_POINT('Ctrl Pts',(-10.7901489399979,-67.03129298199,64.184490448952));
#127852=CARTESIAN_POINT('Ctrl Pts',(-10.9702003000219,-66.37106895915,64.82717780351));
#127853=CARTESIAN_POINT('Ctrl Pts',(-11.1432476215749,-65.7064139723,65.5888798818629));
#127854=CARTESIAN_POINT('Ctrl Pts',(-11.3037100202759,-65.05470374144,66.4852275554991));
#127855=CARTESIAN_POINT('Ctrl Pts',(-11.4470346631969,-64.43466710615,67.540533680774));
#127856=CARTESIAN_POINT('Ctrl Pts',(-11.5688858605402,-63.87372908761,68.786685139671));
#127857=CARTESIAN_POINT('Ctrl Pts',(-11.6629619669604,-63.41586028015,70.25829726077));
#127858=CARTESIAN_POINT('Ctrl Pts',(-11.7179058295959,-63.13683705251,71.941603319142));
#127859=CARTESIAN_POINT('Ctrl Pts',(-11.7225799638996,-63.1128463781799,
73.737184164859));
#127860=CARTESIAN_POINT('Ctrl Pts',(-11.6749105420778,-63.3560371312,75.464665840692));
#127861=CARTESIAN_POINT('Ctrl Pts',(-11.5844470083718,-63.79963931423,76.995744338442));
#127862=CARTESIAN_POINT('Ctrl Pts',(-11.4637651259839,-64.35971469293,78.2926343272081));
#127863=CARTESIAN_POINT('Ctrl Pts',(-11.3203887976569,-64.98479353874,79.386281247239));
#127864=CARTESIAN_POINT('Ctrl Pts',(-11.1588812691069,-65.64468375819,80.311933956733));
#127865=CARTESIAN_POINT('Ctrl Pts',(-10.9840889509839,-66.31928118437,81.096367163558));
#127866=CARTESIAN_POINT('Ctrl Pts',(-10.8014712366919,-66.99057019265,81.756898804972));
#127867=CARTESIAN_POINT('Ctrl Pts',(-10.6200365449139,-67.63683369098,82.303255188861));
#127868=CARTESIAN_POINT('Ctrl Pts',(-10.4501778833209,-68.2349480315001,
82.743606443185));
#127869=CARTESIAN_POINT('Ctrl Pts',(-10.3345594314369,-68.64433296274,83.00979126212));
#127870=CARTESIAN_POINT('Ctrl Pts',(-10.2774188271899,-68.84916507436,83.13431579583));
#127871=CARTESIAN_POINT('Ctrl Pts',(-10.2705435389349,-68.87385090858,83.14920024321));
#127872=CARTESIAN_POINT('Ctrl Pts',(-9.74962299603692,-68.67949730555,62.72912345785));
#127873=CARTESIAN_POINT('Ctrl Pts',(-9.75606091807592,-68.65615750078,62.74350205631));
#127874=CARTESIAN_POINT('Ctrl Pts',(-9.8115303569129,-68.4553773527,62.86814106512));
#127875=CARTESIAN_POINT('Ctrl Pts',(-9.92395689456892,-68.05351180776,63.134305424098));
#127876=CARTESIAN_POINT('Ctrl Pts',(-10.0893581442709,-67.46628603603,63.572908639484));
#127877=CARTESIAN_POINT('Ctrl Pts',(-10.2661331318189,-66.83254665104,64.114061097385));
#127878=CARTESIAN_POINT('Ctrl Pts',(-10.4442769094929,-66.17474813376,64.76462187543));
#127879=CARTESIAN_POINT('Ctrl Pts',(-10.6154242202729,-65.51299951022,65.533723174415));
#127880=CARTESIAN_POINT('Ctrl Pts',(-10.7741403581809,-64.8641732358,66.437242013761));
#127881=CARTESIAN_POINT('Ctrl Pts',(-10.9160218996279,-64.24635739527,67.500323013726));
#127882=CARTESIAN_POINT('Ctrl Pts',(-11.0367602698399,-63.68684013021,68.755468049206));
#127883=CARTESIAN_POINT('Ctrl Pts',(-11.1300597606879,-63.22966687071,70.237786913862));
#127884=CARTESIAN_POINT('Ctrl Pts',(-11.1845913545039,-62.95082114388,71.933698569817));
#127885=CARTESIAN_POINT('Ctrl Pts',(-11.1892302970969,-62.92684685694,73.7428738420364));
#127886=CARTESIAN_POINT('Ctrl Pts',(-11.1419185679629,-63.16988410153,75.483218478992));
#127887=CARTESIAN_POINT('Ctrl Pts',(-11.0521864235499,-63.61289869572,77.02556789635));
#127888=CARTESIAN_POINT('Ctrl Pts',(-10.9325914886959,-64.17163444229,78.331795327822));
#127889=CARTESIAN_POINT('Ctrl Pts',(-10.7906496092569,-64.79452149207,79.433424117582));
#127890=CARTESIAN_POINT('Ctrl Pts',(-10.6308788098719,-65.4515763686501,
80.366454544603));
#127891=CARTESIAN_POINT('Ctrl Pts',(-10.4580157480269,-66.12317064763,81.158323495647));
#127892=CARTESIAN_POINT('Ctrl Pts',(-10.2773475624179,-66.79191739163,81.826792191972));
#127893=CARTESIAN_POINT('Ctrl Pts',(-10.0975166606109,-67.43729186041,82.382075997074));
#127894=CARTESIAN_POINT('Ctrl Pts',(-9.9287545712769,-68.03645111936,82.83178482597));
#127895=CARTESIAN_POINT('Ctrl Pts',(-9.8135378166519,-68.44811923391,83.10507469653));
#127896=CARTESIAN_POINT('Ctrl Pts',(-9.75648121534591,-68.65461870147,83.23332881579));
#127897=CARTESIAN_POINT('Ctrl Pts',(-9.74961432250691,-68.6795132254,83.24866516762));
#127898=CARTESIAN_POINT('Origin',(-10.0948830014566,-68.0758056986579,62.1047072263252));
#127899=CARTESIAN_POINT('Ctrl Pts',(-8.78850469721091,-75.17359603956,59.19490760027));
#127900=CARTESIAN_POINT('Ctrl Pts',(-8.78188852477292,-74.58082390223,59.18747495126));
#127901=CARTESIAN_POINT('Ctrl Pts',(-8.83939730088191,-73.4519410195699,
59.24647973494));
#127902=CARTESIAN_POINT('Ctrl Pts',(-9.0876090788949,-71.8919076279,59.52130962477));
#127903=CARTESIAN_POINT('Ctrl Pts',(-9.40574366428991,-70.55021010581,59.90923180519));
#127904=CARTESIAN_POINT('Ctrl Pts',(-9.7179242559119,-69.39113414181,60.36713913229));
#127905=CARTESIAN_POINT('Ctrl Pts',(-9.99356323184191,-68.38469862843,60.8676797454));
#127906=CARTESIAN_POINT('Ctrl Pts',(-10.1509562713109,-67.76495549583,61.2382841953));
#127907=CARTESIAN_POINT('Ctrl Pts',(-10.2198399627489,-67.47399185811,61.42758621355));
#127908=CARTESIAN_POINT('Ctrl Pts',(-10.2212119301449,-67.46818801423,61.43136843613));
#127909=CARTESIAN_POINT('Ctrl Pts',(-9.36212373097791,-75.16592254393,59.25507590282));
#127910=CARTESIAN_POINT('Ctrl Pts',(-9.35580368697291,-74.60107228412,59.24829590499));
#127911=CARTESIAN_POINT('Ctrl Pts',(-9.41070341504091,-73.52317121109,59.30190722471));
#127912=CARTESIAN_POINT('Ctrl Pts',(-9.64914079436791,-72.0227183761,59.5544042459601));
#127913=CARTESIAN_POINT('Ctrl Pts',(-9.9606708405339,-70.70775665002,59.91952962685));
#127914=CARTESIAN_POINT('Ctrl Pts',(-10.2718202607639,-69.55215247787,60.36120446053));
#127915=CARTESIAN_POINT('Ctrl Pts',(-10.5499421585049,-68.53642237687,60.85287618635));
#127916=CARTESIAN_POINT('Ctrl Pts',(-10.7105856685029,-67.90404690096,61.22299765997));
#127917=CARTESIAN_POINT('Ctrl Pts',(-10.7810225640879,-67.6065779882001,
61.4129801104));
#127918=CARTESIAN_POINT('Ctrl Pts',(-10.7824255217669,-67.60064414927,61.41677625211));
#127919=CARTESIAN_POINT('Ctrl Pts',(-9.69865424996091,-75.15593500828,59.72344078075));
#127920=CARTESIAN_POINT('Ctrl Pts',(-9.69250793843191,-74.62620644493,59.71728021902));
#127921=CARTESIAN_POINT('Ctrl Pts',(-9.74587699154091,-73.61389373368,59.76584842473));
#127922=CARTESIAN_POINT('Ctrl Pts',(-9.97857993168691,-72.1976445875,59.9965061873401));
#127923=CARTESIAN_POINT('Ctrl Pts',(-10.2862352301819,-70.9405985037,60.33596972223));
#127924=CARTESIAN_POINT('Ctrl Pts',(-10.5967796833119,-69.82341248365,60.75367197684));
#127925=CARTESIAN_POINT('Ctrl Pts',(-10.8763582603419,-68.83375635653,61.22439153824));
#127926=CARTESIAN_POINT('Ctrl Pts',(-11.0389087547129,-68.21334787189,61.5826002728));
#127927=CARTESIAN_POINT('Ctrl Pts',(-11.1102568833069,-67.92115734446,61.76704648123));
#127928=CARTESIAN_POINT('Ctrl Pts',(-11.1116780223479,-67.91532865455,61.77073220163));
#127929=CARTESIAN_POINT('Ctrl Pts',(-9.57270218655892,-75.15032266631,60.28631102627));
#127930=CARTESIAN_POINT('Ctrl Pts',(-9.56649085280391,-74.63939257487,60.28032181318));
#127931=CARTESIAN_POINT('Ctrl Pts',(-9.62043278610791,-73.6633464358201,
60.32757492167));
#127932=CARTESIAN_POINT('Ctrl Pts',(-9.8552819341209,-72.29952800127,60.55151405768));
#127933=CARTESIAN_POINT('Ctrl Pts',(-10.1643874204499,-71.09278793092,60.87963793134));
#127934=CARTESIAN_POINT('Ctrl Pts',(-10.4751582924339,-70.02323555163,61.28168335214));
#127935=CARTESIAN_POINT('Ctrl Pts',(-10.7541916833609,-69.07755870261,61.73340035548));
#127936=CARTESIAN_POINT('Ctrl Pts',(-10.9160284575699,-68.48570155355,62.07624524263));
#127937=CARTESIAN_POINT('Ctrl Pts',(-10.9870355422719,-68.20703783005,62.25264647826));
#127938=CARTESIAN_POINT('Ctrl Pts',(-10.9884498766409,-68.20147900883,62.25617139248));
#127939=CARTESIAN_POINT('Ctrl Pts',(-9.44675012315791,-75.14471032433,60.84918127178));
#127940=CARTESIAN_POINT('Ctrl Pts',(-9.4404737671749,-74.65257870482,60.84336340734));
#127941=CARTESIAN_POINT('Ctrl Pts',(-9.49498858067491,-73.71279913797,60.88930141861));
#127942=CARTESIAN_POINT('Ctrl Pts',(-9.73198393655491,-72.4014114150499,
61.10652192802));
#127943=CARTESIAN_POINT('Ctrl Pts',(-10.0425396107169,-71.24497735813,61.42330614046));
#127944=CARTESIAN_POINT('Ctrl Pts',(-10.3535369015559,-70.22305861962,61.80969472745));
#127945=CARTESIAN_POINT('Ctrl Pts',(-10.6320251063809,-69.3213610486901,
62.24240917272));
#127946=CARTESIAN_POINT('Ctrl Pts',(-10.7931481604269,-68.7580552352099,
62.56989021246));
#127947=CARTESIAN_POINT('Ctrl Pts',(-10.8638142012379,-68.49291831565,62.7382464752801));
#127948=CARTESIAN_POINT('Ctrl Pts',(-10.8652217309329,-68.48762936311,62.74161058333));
#127949=CARTESIAN_POINT('Ctrl Pts',(-8.94267290200891,-75.1472320879701,
61.12956993419));
#127950=CARTESIAN_POINT('Ctrl Pts',(-8.93613631826291,-74.64498528552,61.12336056877));
#127951=CARTESIAN_POINT('Ctrl Pts',(-8.99294387591691,-73.68786066791,61.17259229674));
#127952=CARTESIAN_POINT('Ctrl Pts',(-9.23852864643891,-72.3620147815,61.4027146666999));
#127953=CARTESIAN_POINT('Ctrl Pts',(-9.55488816877592,-71.21458424523,61.73007623356));
#127954=CARTESIAN_POINT('Ctrl Pts',(-9.86679161854391,-70.2176116156401,
62.11961002449));
#127955=CARTESIAN_POINT('Ctrl Pts',(-10.1430979147259,-69.34834314582,62.54799863675));
#127956=CARTESIAN_POINT('Ctrl Pts',(-10.3013645639899,-68.8110505217,62.8669547831799));
#127957=CARTESIAN_POINT('Ctrl Pts',(-10.3706657009459,-68.55862913711,63.030145528726));
#127958=CARTESIAN_POINT('Ctrl Pts',(-10.3720459974179,-68.55359402616,63.033406146974));
#127959=CARTESIAN_POINT('Ctrl Pts',(-8.39808036486592,-75.1561989854,60.93968441351));
#127960=CARTESIAN_POINT('Ctrl Pts',(-8.39126263749392,-74.62169807166,60.93278290848));
#127961=CARTESIAN_POINT('Ctrl Pts',(-8.45054721911191,-73.60523376996,60.98771117336));
#127962=CARTESIAN_POINT('Ctrl Pts',(-8.7054117803419,-72.20772431819,61.24171476441));
#127963=CARTESIAN_POINT('Ctrl Pts',(-9.02804163640791,-71.02196462817,61.59448643168));
#127964=CARTESIAN_POINT('Ctrl Pts',(-9.34092407782691,-70.01054271518,62.00386093826));
#127965=CARTESIAN_POINT('Ctrl Pts',(-9.6148730939859,-69.14043351377,62.44549770458));
#127966=CARTESIAN_POINT('Ctrl Pts',(-9.7700537543129,-68.60919338644,62.76847752884));
#127967=CARTESIAN_POINT('Ctrl Pts',(-9.83788028297091,-68.36015993432,62.93284186008));
#127968=CARTESIAN_POINT('Ctrl Pts',(-9.83923115734292,-68.35519262538,62.93612561805));
#127969=CARTESIAN_POINT('Ctrl Pts',(-9.07717754188891,-75.00007042599,59.27469685199));
#127970=CARTESIAN_POINT('Ctrl Pts',(-9.16720240148093,-75.0001184241262,
59.3170480141474));
#127971=CARTESIAN_POINT('Ctrl Pts',(-9.25404279049002,-75.0000081264142,
59.3767114129865));
#127972=CARTESIAN_POINT('Ctrl Pts',(-9.40351821239825,-74.9998108011234,
59.5255401835551));
#127973=CARTESIAN_POINT('Ctrl Pts',(-9.46580962876273,-74.9997241032735,
59.6145335066925));
#127974=CARTESIAN_POINT('Ctrl Pts',(-9.5544246386508,-74.9995852537322,
59.8054548367005));
#127975=CARTESIAN_POINT('Ctrl Pts',(-9.58072200049293,-74.9995331268317,
59.9070017703381));
#127976=CARTESIAN_POINT('Ctrl Pts',(-9.5990568491044,-74.999461759626,60.1039339215817));
#127977=CARTESIAN_POINT('Ctrl Pts',(-9.59135343873692,-74.9994422704594,
60.1991266817374));
#127978=CARTESIAN_POINT('Ctrl Pts',(-9.55275050059125,-74.9994255438882,
60.3716696675316));
#127979=CARTESIAN_POINT('Ctrl Pts',(-9.51915258821981,-74.9994305591295,
60.461075888367));
#127980=CARTESIAN_POINT('Ctrl Pts',(-9.41864283736518,-74.9994712546601,
60.6314235011437));
#127981=CARTESIAN_POINT('Ctrl Pts',(-9.35157790424355,-74.9995070680353,
60.7120836753056));
#127982=CARTESIAN_POINT('Ctrl Pts',(-9.19005028283362,-74.9996032866802,
60.8470403630072));
#127983=CARTESIAN_POINT('Ctrl Pts',(-9.09577378900014,-74.999663508245,
60.9010033430434));
#127984=CARTESIAN_POINT('Ctrl Pts',(-8.89712916494651,-74.9997921275302,
60.971943546326));
#127985=CARTESIAN_POINT('Ctrl Pts',(-8.79314519935482,-74.9998601681799,
60.9889116321022));
#127986=CARTESIAN_POINT('Ctrl Pts',(-8.69365830054091,-75.00000003516,60.98889557741));
#127987=CARTESIAN_POINT('Ctrl Pts',(-10.2211081281489,-82.53194766886,61.43143972309));
#127988=CARTESIAN_POINT('Ctrl Pts',(-10.2201357177169,-82.52783508187,61.42875952001));
#127989=CARTESIAN_POINT('Ctrl Pts',(-10.1636466673389,-82.28917485816,61.27340440246));
#127990=CARTESIAN_POINT('Ctrl Pts',(-10.0368070869879,-81.78301134763,60.9658648185301));
#127991=CARTESIAN_POINT('Ctrl Pts',(-9.81630097459091,-80.9666590177,60.53842194595));
#127992=CARTESIAN_POINT('Ctrl Pts',(-9.56244033240291,-80.03767866059,60.13185887577));
#127993=CARTESIAN_POINT('Ctrl Pts',(-9.28898299286992,-78.9779691788,59.7621739654));
#127994=CARTESIAN_POINT('Ctrl Pts',(-9.02433492858491,-77.76063725352,59.45104885705));
#127995=CARTESIAN_POINT('Ctrl Pts',(-8.82681152382191,-76.3599906814101,
59.23360212967));
#127996=CARTESIAN_POINT('Ctrl Pts',(-8.7826942367269,-75.35421730322,59.18826906547));
#127997=CARTESIAN_POINT('Ctrl Pts',(-8.78852660746291,-74.82645883891,59.19489180675));
#127998=CARTESIAN_POINT('Ctrl Pts',(-10.7823639233799,-82.39954255881,61.4167769709));
#127999=CARTESIAN_POINT('Ctrl Pts',(-10.7813694075629,-82.39533735498,61.41408657358));
#128000=CARTESIAN_POINT('Ctrl Pts',(-10.7235982190879,-82.15131047794,61.25815097326));
#128001=CARTESIAN_POINT('Ctrl Pts',(-10.5941274800899,-81.6347455455,60.95074942728));
#128002=CARTESIAN_POINT('Ctrl Pts',(-10.3707861071929,-80.80778684534,60.52861636853));
#128003=CARTESIAN_POINT('Ctrl Pts',(-10.1166516515639,-79.87750579632,60.13360638867));
#128004=CARTESIAN_POINT('Ctrl Pts',(-9.8458315642529,-78.82770723874,59.78020710747));
#128005=CARTESIAN_POINT('Ctrl Pts',(-9.58828415333991,-77.64224093098,59.48963830546));
#128006=CARTESIAN_POINT('Ctrl Pts',(-9.39873529568491,-76.29731610985,59.29012441741));
#128007=CARTESIAN_POINT('Ctrl Pts',(-9.35661561995691,-75.3371255297,59.24892709446));
#128008=CARTESIAN_POINT('Ctrl Pts',(-9.3621874047499,-74.83402387572,59.25497557751));
#128009=CARTESIAN_POINT('Ctrl Pts',(-11.1116909558609,-82.08485676008,61.77071305075));
#128010=CARTESIAN_POINT('Ctrl Pts',(-11.1106834693079,-82.08072576851,61.76810071081));
#128011=CARTESIAN_POINT('Ctrl Pts',(-11.0521599630159,-81.84101032029,61.6166957882701));
#128012=CARTESIAN_POINT('Ctrl Pts',(-10.9211453438879,-81.33416964011,61.31902500224));
#128013=CARTESIAN_POINT('Ctrl Pts',(-10.6961403303939,-80.5265460574199,
60.91344585688));
#128014=CARTESIAN_POINT('Ctrl Pts',(-10.4418452097559,-79.62464188561,60.5380300981801));
#128015=CARTESIAN_POINT('Ctrl Pts',(-10.1725725780889,-78.61395801647,60.20586918788));
#128016=CARTESIAN_POINT('Ctrl Pts',(-9.91919160451791,-77.48554684164,59.93722926782));
#128017=CARTESIAN_POINT('Ctrl Pts',(-9.73432195722691,-76.2175491581999,
59.75515226542));
#128018=CARTESIAN_POINT('Ctrl Pts',(-9.69337441625392,-75.31589529607,59.71782522343));
#128019=CARTESIAN_POINT('Ctrl Pts',(-9.69879329751091,-74.84394649489,59.72332601301));
#128020=CARTESIAN_POINT('Ctrl Pts',(-10.9885024775799,-81.7986701666301,
62.25617781303));
#128021=CARTESIAN_POINT('Ctrl Pts',(-10.9874998428759,-81.7947305082801,
62.25367949842));
#128022=CARTESIAN_POINT('Ctrl Pts',(-10.9292577495199,-81.56611673017,62.10888171807));
#128023=CARTESIAN_POINT('Ctrl Pts',(-10.7988206361079,-81.08261256883,61.8240166475));
#128024=CARTESIAN_POINT('Ctrl Pts',(-10.5744379260799,-80.31131472407,61.43514752791));
#128025=CARTESIAN_POINT('Ctrl Pts',(-10.3202029039939,-79.4484578645,61.07424270354));
#128026=CARTESIAN_POINT('Ctrl Pts',(-10.0503514291499,-78.47989301382,60.7540472192201));
#128027=CARTESIAN_POINT('Ctrl Pts',(-9.79541195285791,-77.39551035263,60.49402055841));
#128028=CARTESIAN_POINT('Ctrl Pts',(-9.60879199433392,-76.17411857882,60.31720507657));
#128029=CARTESIAN_POINT('Ctrl Pts',(-9.56740600318091,-75.30474683854,60.28089049991));
#128030=CARTESIAN_POINT('Ctrl Pts',(-9.57288207972391,-74.84958042058,60.28623701171));
#128031=CARTESIAN_POINT('Ctrl Pts',(-10.8653139992979,-81.51248357318,62.7416425753));
#128032=CARTESIAN_POINT('Ctrl Pts',(-10.8643162164439,-81.50873524805,62.73925828603));
#128033=CARTESIAN_POINT('Ctrl Pts',(-10.8063555360239,-81.2912231400401,
62.60106764788));
#128034=CARTESIAN_POINT('Ctrl Pts',(-10.6764959283279,-80.83105549755,62.32900829277));
#128035=CARTESIAN_POINT('Ctrl Pts',(-10.4527355217649,-80.09608339071,61.95684919894));
#128036=CARTESIAN_POINT('Ctrl Pts',(-10.1985605982329,-79.2722738434,61.6104553089));
#128037=CARTESIAN_POINT('Ctrl Pts',(-9.9281302802099,-78.34582801118,61.30222525055));
#128038=CARTESIAN_POINT('Ctrl Pts',(-9.67163230119791,-77.30547386363,61.050811849));
#128039=CARTESIAN_POINT('Ctrl Pts',(-9.48326203144091,-76.13068799945,60.8792578877099));
#128040=CARTESIAN_POINT('Ctrl Pts',(-9.44143759010691,-75.29359838101,60.8439557764));
#128041=CARTESIAN_POINT('Ctrl Pts',(-9.44697086193691,-74.85521434627,60.84914801041));
#128042=CARTESIAN_POINT('Ctrl Pts',(-10.3721229628409,-81.44648700826,63.033466560404));
#128043=CARTESIAN_POINT('Ctrl Pts',(-10.3711446046019,-81.44291898027,63.031155889041));
#128044=CARTESIAN_POINT('Ctrl Pts',(-10.3143105744929,-81.23586276699,62.8972233234));
#128045=CARTESIAN_POINT('Ctrl Pts',(-10.1867630388899,-80.79701286147,62.63246723488));
#128046=CARTESIAN_POINT('Ctrl Pts',(-9.9654940543779,-80.0910257475,62.26598172626));
#128047=CARTESIAN_POINT('Ctrl Pts',(-9.71155973831091,-79.29077964255,61.9192959056199));
#128048=CARTESIAN_POINT('Ctrl Pts',(-9.4388119936039,-78.3812453924001,
61.60574375877));
#128049=CARTESIAN_POINT('Ctrl Pts',(-9.17607447350191,-77.34240237262,61.34385874115));
#128050=CARTESIAN_POINT('Ctrl Pts',(-8.98069674798891,-76.1526840562,61.16186671292));
#128051=CARTESIAN_POINT('Ctrl Pts',(-8.93711695013291,-75.29999905499,61.12404109126));
#128052=CARTESIAN_POINT('Ctrl Pts',(-8.9428792060599,-74.85278591516,61.12957580007));
#128053=CARTESIAN_POINT('Ctrl Pts',(-9.83927396841091,-81.64488567277,62.93618296021));
#128054=CARTESIAN_POINT('Ctrl Pts',(-9.8383165967389,-81.64136614092,62.93385618928));
#128055=CARTESIAN_POINT('Ctrl Pts',(-9.78269981195991,-81.4371165775,62.79898052422));
#128056=CARTESIAN_POINT('Ctrl Pts',(-9.65765026435391,-81.00328678021,62.53113344782));
#128057=CARTESIAN_POINT('Ctrl Pts',(-9.43907303949791,-80.29952945763,62.15548485613));
#128058=CARTESIAN_POINT('Ctrl Pts',(-9.18539867836992,-79.49157988093,61.79389977818));
#128059=CARTESIAN_POINT('Ctrl Pts',(-8.91014716050591,-78.56242221897,61.4613028198301));
#128060=CARTESIAN_POINT('Ctrl Pts',(-8.64066837191091,-77.48156077165,61.1768753106));
#128061=CARTESIAN_POINT('Ctrl Pts',(-8.4377197144919,-76.22537355638,60.97573715615));
#128062=CARTESIAN_POINT('Ctrl Pts',(-8.39224341023391,-75.3196616209701,
60.93354232254));
#128063=CARTESIAN_POINT('Ctrl Pts',(-8.3982530630859,-74.84392171622,60.93968686546));
#128064=CARTESIAN_POINT('Origin',(-10.0948738970799,-81.9242545390876,62.1047355865488));
#128065=CARTESIAN_POINT('Ctrl Pts',(-10.9000979577359,-85.14899987206,63.654865562155));
#128066=CARTESIAN_POINT('Ctrl Pts',(-10.9000477186829,-85.1487800261801,
63.654626518916));
#128067=CARTESIAN_POINT('Ctrl Pts',(-10.8750123876449,-85.03922772795,63.535516356367));
#128068=CARTESIAN_POINT('Ctrl Pts',(-10.8237192351409,-84.81696300348,63.302245679743));
#128069=CARTESIAN_POINT('Ctrl Pts',(-10.7430009632029,-84.4733922665001,
62.9660343526));
#128070=CARTESIAN_POINT('Ctrl Pts',(-10.6588871180149,-84.1207589005599,
62.64415049315));
#128071=CARTESIAN_POINT('Ctrl Pts',(-10.5716358795289,-83.75942733737,62.33649495227));
#128072=CARTESIAN_POINT('Ctrl Pts',(-10.4815738635699,-83.38968061365,62.04294556664));
#128073=CARTESIAN_POINT('Ctrl Pts',(-10.3891615445639,-83.01173552994,61.76338234176));
#128074=CARTESIAN_POINT('Ctrl Pts',(-10.2950592384889,-82.62625937344,61.49804807824));
#128075=CARTESIAN_POINT('Ctrl Pts',(-10.2315020580689,-82.36404669929,61.33035293551));
#128076=CARTESIAN_POINT('Ctrl Pts',(-10.1997022332309,-82.23195048545,61.24897957104));
#128077=CARTESIAN_POINT('Ctrl Pts',(-11.4503057701359,-85.02149435186,63.648348588485));
#128078=CARTESIAN_POINT('Ctrl Pts',(-11.4502549602019,-85.02127201958,63.648109994586));
#128079=CARTESIAN_POINT('Ctrl Pts',(-11.4249351524119,-84.91048075584,63.529223852626));
#128080=CARTESIAN_POINT('Ctrl Pts',(-11.3730662784169,-84.68574220319,63.296515421712));
#128081=CARTESIAN_POINT('Ctrl Pts',(-11.2914781830179,-84.33853514106,62.96153745929));
#128082=CARTESIAN_POINT('Ctrl Pts',(-11.2065129108719,-83.9824407764401,
62.6413211441));
#128083=CARTESIAN_POINT('Ctrl Pts',(-11.1184473571699,-83.61789787307,62.33578331032));
#128084=CARTESIAN_POINT('Ctrl Pts',(-11.0276490263389,-83.24534740716,62.04487515227));
#128085=CARTESIAN_POINT('Ctrl Pts',(-10.9346294336719,-82.86520152909,61.76854759814));
#128086=CARTESIAN_POINT('Ctrl Pts',(-10.8400644177689,-82.4781916511,61.50699095751));
#128087=CARTESIAN_POINT('Ctrl Pts',(-10.7763175869489,-82.2154961895,61.34218060436));
#128088=CARTESIAN_POINT('Ctrl Pts',(-10.7444583451179,-82.0833195767701,
61.26233610244));
#128089=CARTESIAN_POINT('Ctrl Pts',(-11.7566449436726,-84.63945239913,63.929825092945));
#128090=CARTESIAN_POINT('Ctrl Pts',(-11.7565938158894,-84.63923537938,63.929594055548));
#128091=CARTESIAN_POINT('Ctrl Pts',(-11.7311156199935,-84.53109144801,63.814473228003));
#128092=CARTESIAN_POINT('Ctrl Pts',(-11.678926201576,-84.31174641896,63.589208692137));
#128093=CARTESIAN_POINT('Ctrl Pts',(-11.5968538146156,-83.97298246405,63.265198385424));
#128094=CARTESIAN_POINT('Ctrl Pts',(-11.5114144935289,-83.62570705904,62.95575715306));
#128095=CARTESIAN_POINT('Ctrl Pts',(-11.4228955535879,-83.27038980136,62.66081388226));
#128096=CARTESIAN_POINT('Ctrl Pts',(-11.3316872647659,-82.90755219152,62.3803649164701));
#128097=CARTESIAN_POINT('Ctrl Pts',(-11.2383295603769,-82.53771004922,62.11440489199));
#128098=CARTESIAN_POINT('Ctrl Pts',(-11.1435069215479,-82.16161060535,61.8630870648701));
#128099=CARTESIAN_POINT('Ctrl Pts',(-11.0796544990849,-81.90665320588,61.70502854942));
#128100=CARTESIAN_POINT('Ctrl Pts',(-11.0477621756589,-81.77846676124,61.6285331978));
#128101=CARTESIAN_POINT('Ctrl Pts',(-11.6201560889415,-84.2510004051699,
64.316483348219));
#128102=CARTESIAN_POINT('Ctrl Pts',(-11.6201051027755,-84.2507930465299,
64.316262066733));
#128103=CARTESIAN_POINT('Ctrl Pts',(-11.5946974764085,-84.1474633713399,
64.206002372866));
#128104=CARTESIAN_POINT('Ctrl Pts',(-11.5426508759679,-83.93787626324,63.990228763609));
#128105=CARTESIAN_POINT('Ctrl Pts',(-11.4607942642209,-83.61415126761,63.679797194182));
#128106=CARTESIAN_POINT('Ctrl Pts',(-11.3755661547679,-83.28224709377,63.383240444918));
#128107=CARTESIAN_POINT('Ctrl Pts',(-11.2872492202299,-82.94260064881,63.100487697675));
#128108=CARTESIAN_POINT('Ctrl Pts',(-11.1962235874359,-82.59568424389,62.83152291331));
#128109=CARTESIAN_POINT('Ctrl Pts',(-11.1030165281019,-82.24195835696,62.57632883436));
#128110=CARTESIAN_POINT('Ctrl Pts',(-11.0083086726939,-81.88212745736,62.33506116619));
#128111=CARTESIAN_POINT('Ctrl Pts',(-10.9445032963929,-81.6381032979,62.18323639217));
#128112=CARTESIAN_POINT('Ctrl Pts',(-10.9126257124109,-81.51538607709,62.10973529188));
#128113=CARTESIAN_POINT('Ctrl Pts',(-11.4836672342099,-83.8625484112,64.703141603492));
#128114=CARTESIAN_POINT('Ctrl Pts',(-11.4836163896619,-83.86235071367,64.702930077918));
#128115=CARTESIAN_POINT('Ctrl Pts',(-11.4582793328239,-83.76383529467,64.5975315177281));
#128116=CARTESIAN_POINT('Ctrl Pts',(-11.4063755503609,-83.56400610752,64.391248835081));
#128117=CARTESIAN_POINT('Ctrl Pts',(-11.3247347138269,-83.25532007118,64.09439600294));
#128118=CARTESIAN_POINT('Ctrl Pts',(-11.2397178160059,-82.9387871285,63.810723736779));
#128119=CARTESIAN_POINT('Ctrl Pts',(-11.1516028868719,-82.61481149627,63.540161513093));
#128120=CARTESIAN_POINT('Ctrl Pts',(-11.0607599101069,-82.28381629625,63.282680910147));
#128121=CARTESIAN_POINT('Ctrl Pts',(-10.9677034958279,-81.94620666469,63.038252776739));
#128122=CARTESIAN_POINT('Ctrl Pts',(-10.8731104238399,-81.60264430937,62.8070352675));
#128123=CARTESIAN_POINT('Ctrl Pts',(-10.8093520937009,-81.36955338991,62.66144423492));
#128124=CARTESIAN_POINT('Ctrl Pts',(-10.7774892491629,-81.2523053929401,
62.59093738595));
#128125=CARTESIAN_POINT('Ctrl Pts',(-10.9929963408319,-83.7199759237,64.943857048887));
#128126=CARTESIAN_POINT('Ctrl Pts',(-10.9929460053909,-83.71978596121,64.94365114242));
#128127=CARTESIAN_POINT('Ctrl Pts',(-10.9678626426279,-83.62512498703,64.841052354269));
#128128=CARTESIAN_POINT('Ctrl Pts',(-10.9164722839509,-83.43308060028,64.640143517834));
#128129=CARTESIAN_POINT('Ctrl Pts',(-10.8356071489709,-83.13626195926,64.350661465033));
#128130=CARTESIAN_POINT('Ctrl Pts',(-10.7513495468499,-82.83166930126,64.073614942909));
#128131=CARTESIAN_POINT('Ctrl Pts',(-10.6639608174649,-82.51963186023,63.80892177283));
#128132=CARTESIAN_POINT('Ctrl Pts',(-10.5737744803679,-82.20042580216,63.5564916609381));
#128133=CARTESIAN_POINT('Ctrl Pts',(-10.4812596278459,-81.87427785351,63.316235685092));
#128134=CARTESIAN_POINT('Ctrl Pts',(-10.3870791967539,-81.54177615285,63.088352361282));
#128135=CARTESIAN_POINT('Ctrl Pts',(-10.3234899953139,-81.31571279398,62.94442831965));
#128136=CARTESIAN_POINT('Ctrl Pts',(-10.2916801383709,-81.20186095682,62.87461613406));
#128137=CARTESIAN_POINT('Ctrl Pts',(-10.4668214943349,-83.9158800948,64.88229121328));
#128138=CARTESIAN_POINT('Ctrl Pts',(-10.4667717048379,-83.91569091757,64.882083139652));
#128139=CARTESIAN_POINT('Ctrl Pts',(-10.4419603929409,-83.82142121439,64.778404382196));
#128140=CARTESIAN_POINT('Ctrl Pts',(-10.3911206083559,-83.6301324804899,
64.575262137112));
#128141=CARTESIAN_POINT('Ctrl Pts',(-10.3110873031249,-83.33430210374,64.282155774695));
#128142=CARTESIAN_POINT('Ctrl Pts',(-10.2276439378039,-83.0304638771,64.00117300774));
#128143=CARTESIAN_POINT('Ctrl Pts',(-10.1410339545129,-82.7188784586,63.732215622428));
#128144=CARTESIAN_POINT('Ctrl Pts',(-10.0515517702039,-82.39967273597,63.475122147589));
#128145=CARTESIAN_POINT('Ctrl Pts',(-9.95961766575091,-82.0728878304499,
63.22973483264));
#128146=CARTESIAN_POINT('Ctrl Pts',(-9.86587973341591,-81.73905528501,62.996304253343));
#128147=CARTESIAN_POINT('Ctrl Pts',(-9.80247189848491,-81.51154958802,62.84839778456));
#128148=CARTESIAN_POINT('Ctrl Pts',(-9.7707188632119,-81.39681512848,62.77652950846));
#128149=CARTESIAN_POINT('Origin',(-10.7325612699948,-84.4008983433199,64.1552576107488));
#128150=CARTESIAN_POINT('Ctrl Pts',(-10.9457112853099,-88.7723095427,73.1633008345938));
#128151=CARTESIAN_POINT('Ctrl Pts',(-10.9450018737129,-88.7745370054799,
72.987400423028));
#128152=CARTESIAN_POINT('Ctrl Pts',(-10.9460260077449,-88.77205014386,72.6044578842011));
#128153=CARTESIAN_POINT('Ctrl Pts',(-10.9558737619719,-88.74262773799,71.9944222624584));
#128154=CARTESIAN_POINT('Ctrl Pts',(-10.9769412377749,-88.6771448963399,
71.310998753955));
#128155=CARTESIAN_POINT('Ctrl Pts',(-11.0102164392899,-88.56545006486,70.560459108714));
#128156=CARTESIAN_POINT('Ctrl Pts',(-11.0530137011699,-88.3969466046301,
69.752251524636));
#128157=CARTESIAN_POINT('Ctrl Pts',(-11.0991047356729,-88.1686714004199,
68.920979936926));
#128158=CARTESIAN_POINT('Ctrl Pts',(-11.1393227521459,-87.888632837,68.107252447975));
#128159=CARTESIAN_POINT('Ctrl Pts',(-11.1675251720229,-87.5709448254,67.341066879205));
#128160=CARTESIAN_POINT('Ctrl Pts',(-11.1808972887479,-87.22746712569,66.633570170775));
#128161=CARTESIAN_POINT('Ctrl Pts',(-11.1788763078239,-86.87105465404,65.992404193633));
#128162=CARTESIAN_POINT('Ctrl Pts',(-11.1627503627999,-86.51320748952,65.419759920927));
#128163=CARTESIAN_POINT('Ctrl Pts',(-11.1340216992209,-86.1624575053199,
64.91289537508));
#128164=CARTESIAN_POINT('Ctrl Pts',(-11.0945767098009,-85.8242611711499,
64.466136015972));
#128165=CARTESIAN_POINT('Ctrl Pts',(-11.0458305932859,-85.50274962242,64.073903342735));
#128166=CARTESIAN_POINT('Ctrl Pts',(-10.9894638587469,-85.2010373165,63.730974057673));
#128167=CARTESIAN_POINT('Ctrl Pts',(-10.9440465981759,-84.99834908578,63.514663353308));
#128168=CARTESIAN_POINT('Ctrl Pts',(-10.9192732707999,-84.89780249114,63.41068261844));
#128169=CARTESIAN_POINT('Ctrl Pts',(-10.9177140490529,-84.89150973702,63.404187754761));
#128170=CARTESIAN_POINT('Ctrl Pts',(-11.4761904670739,-88.6404673409601,
73.1593416733101));
#128171=CARTESIAN_POINT('Ctrl Pts',(-11.4754919605259,-88.64261186187,72.9876546744834));
#128172=CARTESIAN_POINT('Ctrl Pts',(-11.4764990546509,-88.64023131728,72.6137103493763));
#128173=CARTESIAN_POINT('Ctrl Pts',(-11.4862124533569,-88.6118783058,72.0173035258748));
#128174=CARTESIAN_POINT('Ctrl Pts',(-11.5069967010369,-88.54872844628,71.348776611085));
#128175=CARTESIAN_POINT('Ctrl Pts',(-11.5399844616029,-88.44039024958,70.61107031933));
#128176=CARTESIAN_POINT('Ctrl Pts',(-11.582615894791,-88.27588931312,69.813090462725));
#128177=CARTESIAN_POINT('Ctrl Pts',(-11.6287959324594,-88.05129587406,68.987787659599));
#128178=CARTESIAN_POINT('Ctrl Pts',(-11.669305562902,-87.77371776389,68.175949983838));
#128179=CARTESIAN_POINT('Ctrl Pts',(-11.6978313787621,-87.45685828132,67.408646414581));
#128180=CARTESIAN_POINT('Ctrl Pts',(-11.7114009845464,-87.11262810213,66.698289589759));
#128181=CARTESIAN_POINT('Ctrl Pts',(-11.7093587965017,-86.75393399862,66.053125508229));
#128182=CARTESIAN_POINT('Ctrl Pts',(-11.6929225816759,-86.39232720817,65.475670662799));
#128183=CARTESIAN_POINT('Ctrl Pts',(-11.6635630956701,-86.0365935910501,
64.963608459124));
#128184=CARTESIAN_POINT('Ctrl Pts',(-11.6230843718873,-85.69193147085,64.510908749976));
#128185=CARTESIAN_POINT('Ctrl Pts',(-11.5728539359695,-85.36268242413,64.112285611781));
#128186=CARTESIAN_POINT('Ctrl Pts',(-11.5144463383459,-85.05180029684,63.76229349374));
#128187=CARTESIAN_POINT('Ctrl Pts',(-11.4670572666889,-84.84139611019,63.540339695315));
#128188=CARTESIAN_POINT('Ctrl Pts',(-11.4410866627279,-84.73653930447,63.43329389282));
#128189=CARTESIAN_POINT('Ctrl Pts',(-11.4394516418749,-84.72997489958,63.426606166869));
#128190=CARTESIAN_POINT('Ctrl Pts',(-11.7472020744045,-88.1658022693401,
73.1521332719869));
#128191=CARTESIAN_POINT('Ctrl Pts',(-11.746509139036,-88.1678377977,72.9878314959629));
#128192=CARTESIAN_POINT('Ctrl Pts',(-11.7475075277997,-88.16558611108,72.6298738240873));
#128193=CARTESIAN_POINT('Ctrl Pts',(-11.7571522868552,-88.1386590847199,
72.058565121298));
#128194=CARTESIAN_POINT('Ctrl Pts',(-11.7777918387362,-88.07865829698,71.417961246875));
#128195=CARTESIAN_POINT('Ctrl Pts',(-11.8106327512531,-87.97536584284,70.709076227008));
#128196=CARTESIAN_POINT('Ctrl Pts',(-11.8531794657527,-87.8179219397101,
69.940253903915));
#128197=CARTESIAN_POINT('Ctrl Pts',(-11.8994049734258,-87.6019786177801,
69.1425609119151));
#128198=CARTESIAN_POINT('Ctrl Pts',(-11.9400635838349,-87.33393685455,68.355683161392));
#128199=CARTESIAN_POINT('Ctrl Pts',(-11.9687546164803,-87.02686944062,67.610366073095));
#128200=CARTESIAN_POINT('Ctrl Pts',(-11.9824251156254,-86.6923642999,66.919355788869));
#128201=CARTESIAN_POINT('Ctrl Pts',(-11.9803720932708,-86.3429766281501,
66.29098910701));
#128202=CARTESIAN_POINT('Ctrl Pts',(-11.9637773675727,-85.98994563365,65.7278882031509));
#128203=CARTESIAN_POINT('Ctrl Pts',(-11.9340956065262,-85.6419386551799,
65.228039708533));
#128204=CARTESIAN_POINT('Ctrl Pts',(-11.8930887677471,-85.3038582790601,
64.78539468191));
#128205=CARTESIAN_POINT('Ctrl Pts',(-11.8421000216054,-84.98003443023,64.394984537295));
#128206=CARTESIAN_POINT('Ctrl Pts',(-11.7826497862989,-84.67324521565,64.051401372673));
#128207=CARTESIAN_POINT('Ctrl Pts',(-11.7342533542964,-84.46477706569,63.832868896649));
#128208=CARTESIAN_POINT('Ctrl Pts',(-11.7076710847639,-84.3606282937899,
63.727283428551));
#128209=CARTESIAN_POINT('Ctrl Pts',(-11.705997339607,-84.35410721095,63.7206861801679));
#128210=CARTESIAN_POINT('Ctrl Pts',(-11.5910801936143,-87.6419739009899,
73.1461352299971));
#128211=CARTESIAN_POINT('Ctrl Pts',(-11.5903840488516,-87.6439418162,72.9878214938683));
#128212=CARTESIAN_POINT('Ctrl Pts',(-11.5913874525196,-87.6417618083599,
72.6429485013794));
#128213=CARTESIAN_POINT('Ctrl Pts',(-11.6010717528755,-87.6157351480201,
72.0926798649851));
#128214=CARTESIAN_POINT('Ctrl Pts',(-11.6217946597851,-87.5577512951999,
71.475750416479));
#128215=CARTESIAN_POINT('Ctrl Pts',(-11.6547201671793,-87.4580720574301,
70.793843819682));
#128216=CARTESIAN_POINT('Ctrl Pts',(-11.6973156856438,-87.30637374418,70.0550700349761));
#128217=CARTESIAN_POINT('Ctrl Pts',(-11.7435149993737,-87.0986973501601,
69.28954660411));
#128218=CARTESIAN_POINT('Ctrl Pts',(-11.7840877867703,-86.8413680052499,
68.535257011051));
#128219=CARTESIAN_POINT('Ctrl Pts',(-11.8126836428455,-86.5469981707199,
67.821428576924));
#128220=CARTESIAN_POINT('Ctrl Pts',(-11.8262960202688,-86.2266790269099,
67.160002425791));
#128221=CARTESIAN_POINT('Ctrl Pts',(-11.8242492392441,-85.89242826919,66.558836652314));
#128222=CARTESIAN_POINT('Ctrl Pts',(-11.8077458270353,-85.5550029313299,
66.02037389564));
#128223=CARTESIAN_POINT('Ctrl Pts',(-11.778249719238,-85.2226526474,65.542594259322));
#128224=CARTESIAN_POINT('Ctrl Pts',(-11.7375471121017,-84.9001296381899,
65.119778448422));
#128225=CARTESIAN_POINT('Ctrl Pts',(-11.6869952063578,-84.5915372927401,
64.747103648563));
#128226=CARTESIAN_POINT('Ctrl Pts',(-11.6281456042038,-84.29957157528,64.419436216352));
#128227=CARTESIAN_POINT('Ctrl Pts',(-11.5803294831087,-84.10149369279,64.21127282023));
#128228=CARTESIAN_POINT('Ctrl Pts',(-11.5540995762679,-84.00263316253,64.110769627984));
#128229=CARTESIAN_POINT('Ctrl Pts',(-11.5524481390529,-83.99644357262,64.104490221532));
#128230=CARTESIAN_POINT('Ctrl Pts',(-11.4349583128239,-87.11814553264,73.1401371880075));
#128231=CARTESIAN_POINT('Ctrl Pts',(-11.4342589586669,-87.1200458347101,
72.9878114917734));
#128232=CARTESIAN_POINT('Ctrl Pts',(-11.4352673772399,-87.11793750563,72.6560231786716));
#128233=CARTESIAN_POINT('Ctrl Pts',(-11.4449912188959,-87.09281121132,72.1267946086722));
#128234=CARTESIAN_POINT('Ctrl Pts',(-11.4657974808339,-87.03684429341,71.533539586084));
#128235=CARTESIAN_POINT('Ctrl Pts',(-11.4988075831059,-86.94077827202,70.878611412355));
#128236=CARTESIAN_POINT('Ctrl Pts',(-11.5414519055349,-86.79482554866,70.169886166037));
#128237=CARTESIAN_POINT('Ctrl Pts',(-11.5876250253216,-86.59541608253,69.436532296305));
#128238=CARTESIAN_POINT('Ctrl Pts',(-11.6281119897057,-86.34879915595,68.714830860709));
#128239=CARTESIAN_POINT('Ctrl Pts',(-11.6566126692108,-86.06712690083,68.032491080753));
#128240=CARTESIAN_POINT('Ctrl Pts',(-11.6701669249123,-85.76099375391,67.400649062714));
#128241=CARTESIAN_POINT('Ctrl Pts',(-11.6681263852174,-85.4418799102201,
66.826684197617));
#128242=CARTESIAN_POINT('Ctrl Pts',(-11.6517142864979,-85.120060229,66.31285958813));
#128243=CARTESIAN_POINT('Ctrl Pts',(-11.6224038319499,-84.8033666396201,
65.8571488101121));
#128244=CARTESIAN_POINT('Ctrl Pts',(-11.5820054564562,-84.49640099733,65.454162214934));
#128245=CARTESIAN_POINT('Ctrl Pts',(-11.5318903911099,-84.20304015525,65.099222759832));
#128246=CARTESIAN_POINT('Ctrl Pts',(-11.4736414221089,-83.9258979349,64.78747106003));
#128247=CARTESIAN_POINT('Ctrl Pts',(-11.4264056119209,-83.73821031989,64.589676743811));
#128248=CARTESIAN_POINT('Ctrl Pts',(-11.4005280677719,-83.6446380312701,
64.494255827417));
#128249=CARTESIAN_POINT('Ctrl Pts',(-11.3988989384989,-83.63877993428,64.488294262896));
#128250=CARTESIAN_POINT('Ctrl Pts',(-10.9482903854889,-86.86922914558,73.139060295455));
#128251=CARTESIAN_POINT('Ctrl Pts',(-10.9475810269089,-86.87114504394,72.9876208540694));
#128252=CARTESIAN_POINT('Ctrl Pts',(-10.9486050780959,-86.86900686913,72.657920188345));
#128253=CARTESIAN_POINT('Ctrl Pts',(-10.9584521791089,-86.84369829509,72.1326568375601));
#128254=CARTESIAN_POINT('Ctrl Pts',(-10.9795182779059,-86.78736836434,71.544181042512));
#128255=CARTESIAN_POINT('Ctrl Pts',(-11.0127920819299,-86.69124765573,70.897697785394));
#128256=CARTESIAN_POINT('Ctrl Pts',(-11.0555885375789,-86.54617447248,70.201322045947));
#128257=CARTESIAN_POINT('Ctrl Pts',(-11.1016800048009,-86.3495342702701,
69.484795244371));
#128258=CARTESIAN_POINT('Ctrl Pts',(-11.1418994390519,-86.10817841465,68.783148983785));
#128259=CARTESIAN_POINT('Ctrl Pts',(-11.1701034312259,-85.83425367749,68.1223190428309));
#128260=CARTESIAN_POINT('Ctrl Pts',(-11.1834765081089,-85.5379910790401,
67.511996026178));
#128261=CARTESIAN_POINT('Ctrl Pts',(-11.1814554240789,-85.23047992381,66.958807276233));
#128262=CARTESIAN_POINT('Ctrl Pts',(-11.1653279705759,-84.92164105655,66.4646622131589));
#128263=CARTESIAN_POINT('Ctrl Pts',(-11.1365962400459,-84.61884793878,66.0272221703121));
#128264=CARTESIAN_POINT('Ctrl Pts',(-11.0971462247829,-84.32679045813,65.641571644434));
#128265=CARTESIAN_POINT('Ctrl Pts',(-11.0483928917579,-84.04904419777,65.302917614327));
#128266=CARTESIAN_POINT('Ctrl Pts',(-10.9920162348879,-83.7882852518,65.006741888935));
#128267=CARTESIAN_POINT('Ctrl Pts',(-10.9465893877049,-83.61301402036,64.819849403497));
#128268=CARTESIAN_POINT('Ctrl Pts',(-10.9218102393719,-83.52603852108,64.729988468514));
#128269=CARTESIAN_POINT('Ctrl Pts',(-10.9202506491019,-83.5205950042099,
64.724375472001));
#128270=CARTESIAN_POINT('Ctrl Pts',(-10.4321617544179,-87.04922107186,73.1435707901278));
#128271=CARTESIAN_POINT('Ctrl Pts',(-10.4314417857939,-87.0512261270099,
72.9873675219955));
#128272=CARTESIAN_POINT('Ctrl Pts',(-10.4324824159229,-87.0489750465499,
72.6474659132869));
#128273=CARTESIAN_POINT('Ctrl Pts',(-10.4424602378649,-87.0225143174599,
72.1066397846169));
#128274=CARTESIAN_POINT('Ctrl Pts',(-10.4638019028829,-86.96366601015,71.501091268797));
#128275=CARTESIAN_POINT('Ctrl Pts',(-10.4973553719879,-86.8638565438999,
70.839294831367));
#128276=CARTESIAN_POINT('Ctrl Pts',(-10.5403131703229,-86.71425270862,70.1299293360159));
#128277=CARTESIAN_POINT('Ctrl Pts',(-10.5863180420969,-86.5131708543901,
69.40447675936));
#128278=CARTESIAN_POINT('Ctrl Pts',(-10.6262537511339,-86.2683698718599,
68.697945218175));
#128279=CARTESIAN_POINT('Ctrl Pts',(-10.6541430958509,-85.99244945822,68.035338875427));
#128280=CARTESIAN_POINT('Ctrl Pts',(-10.6673240261589,-85.69563537809,67.425156634356));
#128281=CARTESIAN_POINT('Ctrl Pts',(-10.6653235755539,-85.3890144863201,
66.873465711372));
#128282=CARTESIAN_POINT('Ctrl Pts',(-10.6494979984179,-85.0825007902901,
66.381866509769));
#128283=CARTESIAN_POINT('Ctrl Pts',(-10.6213800252729,-84.78325215938,65.947595579691));
#128284=CARTESIAN_POINT('Ctrl Pts',(-10.5829357797369,-84.49623044878,65.566062724265));
#128285=CARTESIAN_POINT('Ctrl Pts',(-10.5356266122269,-84.22482162347,65.232168945831));
#128286=CARTESIAN_POINT('Ctrl Pts',(-10.4812356089069,-83.97186993939,64.94159309689));
#128287=CARTESIAN_POINT('Ctrl Pts',(-10.4377272312729,-83.80335960198,64.759390591149));
#128288=CARTESIAN_POINT('Ctrl Pts',(-10.4141129707359,-83.72020822447,64.672127566615));
#128289=CARTESIAN_POINT('Ctrl Pts',(-10.4126271290499,-83.71500588789,64.666678216697));
#128290=CARTESIAN_POINT('Ctrl Pts',(-11.2240831851649,-88.65122976349,72.9889532029839));
#128291=CARTESIAN_POINT('Ctrl Pts',(-11.3032351536548,-88.5991560625599,
72.9890176977034));
#128292=CARTESIAN_POINT('Ctrl Pts',(-11.3769892253945,-88.5321181182094,
72.9888757744761));
#128293=CARTESIAN_POINT('Ctrl Pts',(-11.4995563634225,-88.374992788323,
72.9886266426874));
#128294=CARTESIAN_POINT('Ctrl Pts',(-11.5481347520047,-88.2850759639086,
72.9885197770362));
#128295=CARTESIAN_POINT('Ctrl Pts',(-11.6123569941101,-88.0972289441662,
72.9883528279406));
#128296=CARTESIAN_POINT('Ctrl Pts',(-11.6280120210786,-87.9995855317363,
72.9882927405526));
#128297=CARTESIAN_POINT('Ctrl Pts',(-11.6292320149507,-87.8121305336596,
72.9882159438058));
#128298=CARTESIAN_POINT('Ctrl Pts',(-11.6150356049613,-87.7225667916036,
72.9881989050114));
#128299=CARTESIAN_POINT('Ctrl Pts',(-11.5663507330197,-87.5602645510202,
72.9881945590678));
#128300=CARTESIAN_POINT('Ctrl Pts',(-11.5288061045921,-87.4774628379731,
72.9882110757354));
#128301=CARTESIAN_POINT('Ctrl Pts',(-11.4244552027482,-87.3215153774326,
72.9882855525215));
#128302=CARTESIAN_POINT('Ctrl Pts',(-11.3575532357774,-87.2485944781033,
72.9883436484516));
#128303=CARTESIAN_POINT('Ctrl Pts',(-11.2004148129803,-87.1271549781129,
72.9884929133032));
#128304=CARTESIAN_POINT('Ctrl Pts',(-11.1103290403818,-87.0788809918115,
72.9885838692378));
#128305=CARTESIAN_POINT('Ctrl Pts',(-10.9215320523432,-87.0152878970258,
72.9887780410119));
#128306=CARTESIAN_POINT('Ctrl Pts',(-10.823110509523,-86.9999796268137,
72.9888808467404));
#128307=CARTESIAN_POINT('Ctrl Pts',(-10.7284497219739,-86.99999983559,72.9890778951927));
#128308=CARTESIAN_POINT('Ctrl Pts',(-10.9175000005819,-84.8914604129799,
82.573632476901));
#128309=CARTESIAN_POINT('Ctrl Pts',(-10.9187148702499,-84.8963481517099,
82.568587786684));
#128310=CARTESIAN_POINT('Ctrl Pts',(-10.9496313599749,-85.0212737335599,
82.439453037357));
#128311=CARTESIAN_POINT('Ctrl Pts',(-11.0058431886349,-85.27706754662,82.164507487811));
#128312=CARTESIAN_POINT('Ctrl Pts',(-11.0708521503739,-85.6539729890001,
81.725209488295));
#128313=CARTESIAN_POINT('Ctrl Pts',(-11.1207286557869,-86.03545424853,81.23869304884));
#128314=CARTESIAN_POINT('Ctrl Pts',(-11.1549334002079,-86.40251457695,80.723477204648));
#128315=CARTESIAN_POINT('Ctrl Pts',(-11.1745731186709,-86.7447659739099,
80.192953837545));
#128316=CARTESIAN_POINT('Ctrl Pts',(-11.1807648168209,-87.06062102531,79.650614129966));
#128317=CARTESIAN_POINT('Ctrl Pts',(-11.1760880469139,-87.35492773232,79.088005209122));
#128318=CARTESIAN_POINT('Ctrl Pts',(-11.1616928465779,-87.63400684917,78.48818413759));
#128319=CARTESIAN_POINT('Ctrl Pts',(-11.1372368107129,-87.902076581,77.828950659358));
#128320=CARTESIAN_POINT('Ctrl Pts',(-11.1008128139689,-88.1581700157699,
77.087248046884));
#128321=CARTESIAN_POINT('Ctrl Pts',(-11.0546164356989,-88.3902796938699,
76.256928159294));
#128322=CARTESIAN_POINT('Ctrl Pts',(-11.0064698093009,-88.57829407792,75.361422431816));
#128323=CARTESIAN_POINT('Ctrl Pts',(-10.9692740524649,-88.7055150063399,
74.45212684179));
#128324=CARTESIAN_POINT('Ctrl Pts',(-10.9486889645929,-88.7677494397999,
73.6016671236896));
#128325=CARTESIAN_POINT('Ctrl Pts',(-10.9451851927139,-88.7754227146399,
73.0611701552288));
#128326=CARTESIAN_POINT('Ctrl Pts',(-10.9459672912859,-88.77230539163,72.8146988191757));
#128327=CARTESIAN_POINT('Ctrl Pts',(-11.4392120691599,-84.72970045485,82.5514119589451));
#128328=CARTESIAN_POINT('Ctrl Pts',(-11.4404857879209,-84.73479847883,82.546218425558));
#128329=CARTESIAN_POINT('Ctrl Pts',(-11.4728940472009,-84.86507337982,82.41329139738));
#128330=CARTESIAN_POINT('Ctrl Pts',(-11.5315139643969,-85.1304815547,82.131221295799));
#128331=CARTESIAN_POINT('Ctrl Pts',(-11.598755706812,-85.51811794423,81.683330398921));
#128332=CARTESIAN_POINT('Ctrl Pts',(-11.6499756528862,-85.9073743459,81.190085371289));
#128333=CARTESIAN_POINT('Ctrl Pts',(-11.6849611287431,-86.28001943032,80.66938665616));
#128334=CARTESIAN_POINT('Ctrl Pts',(-11.7050077077243,-86.62644648557,80.133835806426));
#128335=CARTESIAN_POINT('Ctrl Pts',(-11.7113084987726,-86.94510548552,79.587146028598));
#128336=CARTESIAN_POINT('Ctrl Pts',(-11.7065522361436,-87.24050734235,79.021973767765));
#128337=CARTESIAN_POINT('Ctrl Pts',(-11.6919769255882,-87.51959465724,78.4207110295121));
#128338=CARTESIAN_POINT('Ctrl Pts',(-11.667258928563,-87.78680743792,77.760882962257));
#128339=CARTESIAN_POINT('Ctrl Pts',(-11.6305324924398,-88.04095857353,77.020117236076));
#128340=CARTESIAN_POINT('Ctrl Pts',(-11.5842251848039,-88.2694212430601,
76.195453975661));
#128341=CARTESIAN_POINT('Ctrl Pts',(-11.5362920311509,-88.45285201793,75.311618240522));
#128342=CARTESIAN_POINT('Ctrl Pts',(-11.4994922869709,-88.5760310449,74.4195924580851));
#128343=CARTESIAN_POINT('Ctrl Pts',(-11.4791528728089,-88.63611386146,73.5865621709933));
#128344=CARTESIAN_POINT('Ctrl Pts',(-11.4757076647519,-88.6434404726801,
73.058635682904));
#128345=CARTESIAN_POINT('Ctrl Pts',(-11.4764772673159,-88.64043162139,72.8181652199194));
#128346=CARTESIAN_POINT('Ctrl Pts',(-11.7057132270397,-84.35369441765,82.257404991939));
#128347=CARTESIAN_POINT('Ctrl Pts',(-11.7070170071163,-84.35875839185,82.252282259352));
#128348=CARTESIAN_POINT('Ctrl Pts',(-11.7401872926896,-84.48814975745,82.121176924537));
#128349=CARTESIAN_POINT('Ctrl Pts',(-11.8000373105898,-84.75104883033,81.84348205208));
#128350=CARTESIAN_POINT('Ctrl Pts',(-11.868419602882,-85.13319173531,81.404040811101));
#128351=CARTESIAN_POINT('Ctrl Pts',(-11.9203258058273,-85.51527430505,80.921611413094));
#128352=CARTESIAN_POINT('Ctrl Pts',(-11.9557100952138,-85.88002512022,80.413225238712));
#128353=CARTESIAN_POINT('Ctrl Pts',(-11.9759645068405,-86.2185520436701,
79.890676037857));
#128354=CARTESIAN_POINT('Ctrl Pts',(-11.9823210247644,-86.52937136749,79.357690250987));
#128355=CARTESIAN_POINT('Ctrl Pts',(-11.9775241556327,-86.81667491343,78.807753404929));
#128356=CARTESIAN_POINT('Ctrl Pts',(-11.9628568411064,-87.08754421069,78.22340893719));
#128357=CARTESIAN_POINT('Ctrl Pts',(-11.9380050289816,-87.34641096537,77.582692485394));
#128358=CARTESIAN_POINT('Ctrl Pts',(-11.9011241006592,-87.59200141635,76.864268881454));
#128359=CARTESIAN_POINT('Ctrl Pts',(-11.8547601280426,-87.81171865749,76.067026470817));
#128360=CARTESIAN_POINT('Ctrl Pts',(-11.8069360206181,-87.98721342102,75.215676380909));
#128361=CARTESIAN_POINT('Ctrl Pts',(-11.7703385677752,-88.10453079837,74.359470559734));
#128362=CARTESIAN_POINT('Ctrl Pts',(-11.7501246487507,-88.16165500829,73.5606102595776));
#128363=CARTESIAN_POINT('Ctrl Pts',(-11.7467093562876,-88.1685742837001,
73.0551809007065));
#128364=CARTESIAN_POINT('Ctrl Pts',(-11.7474725756366,-88.1657139936001,
72.8251097834962));
#128365=CARTESIAN_POINT('Ctrl Pts',(-11.5521126194759,-83.99608653211,81.873520954723));
#128366=CARTESIAN_POINT('Ctrl Pts',(-11.5533990734129,-84.00089318895,81.868644860704));
#128367=CARTESIAN_POINT('Ctrl Pts',(-11.5861301575113,-84.1237148298,81.743848064745));
#128368=CARTESIAN_POINT('Ctrl Pts',(-11.6452711945686,-84.37353378032,81.47932114015));
#128369=CARTESIAN_POINT('Ctrl Pts',(-11.7129961195329,-84.73735772374,81.060144097334));
#128370=CARTESIAN_POINT('Ctrl Pts',(-11.7645067914674,-85.10175611464,80.599382649326));
#128371=CARTESIAN_POINT('Ctrl Pts',(-11.7996612206877,-85.4500180148699,
80.113486354029));
#128372=CARTESIAN_POINT('Ctrl Pts',(-11.8197958458907,-85.7734570232501,
79.613923491977));
#128373=CARTESIAN_POINT('Ctrl Pts',(-11.8261202450725,-86.0706436476901,
79.104216759278));
#128374=CARTESIAN_POINT('Ctrl Pts',(-11.8213467799047,-86.3456660471901,
78.577887554994));
#128375=CARTESIAN_POINT('Ctrl Pts',(-11.8067324927872,-86.6051758018201,
78.018353542789));
#128376=CARTESIAN_POINT('Ctrl Pts',(-11.7819578063333,-86.85337134828,77.404630081976));
#128377=CARTESIAN_POINT('Ctrl Pts',(-11.7451659211349,-87.0890794363699,
76.716130212862));
#128378=CARTESIAN_POINT('Ctrl Pts',(-11.6988346079466,-87.3003638420499,
75.951106916957));
#128379=CARTESIAN_POINT('Ctrl Pts',(-11.6509476506377,-87.4694803984999,
75.132958453367));
#128380=CARTESIAN_POINT('Ctrl Pts',(-11.61423360516,-87.5827431255899,74.308960051561));
#128381=CARTESIAN_POINT('Ctrl Pts',(-11.5939473557576,-87.6379323021899,
73.539868478611));
#128382=CARTESIAN_POINT('Ctrl Pts',(-11.5905148211427,-87.64463559833,73.0529433677899));
#128383=CARTESIAN_POINT('Ctrl Pts',(-11.5912817195219,-87.64187204039,72.8312357367396));
#128384=CARTESIAN_POINT('Ctrl Pts',(-11.3985120119129,-83.63847864657,81.489636917508));
#128385=CARTESIAN_POINT('Ctrl Pts',(-11.3997811397099,-83.64302798605,81.485007462056));
#128386=CARTESIAN_POINT('Ctrl Pts',(-11.4320730223329,-83.75927990215,81.366519204953));
#128387=CARTESIAN_POINT('Ctrl Pts',(-11.4905050785479,-83.9960187303,81.11516022822));
#128388=CARTESIAN_POINT('Ctrl Pts',(-11.5575726361839,-84.34152371217,80.716247383567));
#128389=CARTESIAN_POINT('Ctrl Pts',(-11.6086877771075,-84.6882379242201,
80.277153885558));
#128390=CARTESIAN_POINT('Ctrl Pts',(-11.6436123461616,-85.02001090952,79.813747469345));
#128391=CARTESIAN_POINT('Ctrl Pts',(-11.6636271849409,-85.32836200283,79.3371709460971));
#128392=CARTESIAN_POINT('Ctrl Pts',(-11.6699194653806,-85.6119159279,78.85074326757));
#128393=CARTESIAN_POINT('Ctrl Pts',(-11.6651694041767,-85.87465718095,78.3480217050591));
#128394=CARTESIAN_POINT('Ctrl Pts',(-11.650608144468,-86.12280739294,77.813298148387));
#128395=CARTESIAN_POINT('Ctrl Pts',(-11.6259105836849,-86.36033173119,77.226567678558));
#128396=CARTESIAN_POINT('Ctrl Pts',(-11.5892077416107,-86.58615745639,76.567991544269));
#128397=CARTESIAN_POINT('Ctrl Pts',(-11.5429090878509,-86.7890090266,75.835187363097));
#128398=CARTESIAN_POINT('Ctrl Pts',(-11.4949592806569,-86.95174737597,75.050240525825));
#128399=CARTESIAN_POINT('Ctrl Pts',(-11.4581286425449,-87.0609554528,74.258449543389));
#128400=CARTESIAN_POINT('Ctrl Pts',(-11.4377700627649,-87.11420959609,73.5191266976445));
#128401=CARTESIAN_POINT('Ctrl Pts',(-11.4343202859979,-87.12069691296,73.0507058348735));
#128402=CARTESIAN_POINT('Ctrl Pts',(-11.4350908634069,-87.11803008719,72.8373616899829));
#128403=CARTESIAN_POINT('Ctrl Pts',(-10.9198461320759,-83.52052975215,81.253394354178));
#128404=CARTESIAN_POINT('Ctrl Pts',(-10.9210612663879,-83.52475771529,81.2490347736811));
#128405=CARTESIAN_POINT('Ctrl Pts',(-10.9519844645779,-83.63281856841,81.13743865198));
#128406=CARTESIAN_POINT('Ctrl Pts',(-11.0082071223769,-83.8539992488999,
80.89989300697));
#128407=CARTESIAN_POINT('Ctrl Pts',(-11.0732261248979,-84.1796941866,80.520520942376));
#128408=CARTESIAN_POINT('Ctrl Pts',(-11.1231086717439,-84.50915551152,80.100541218406));
#128409=CARTESIAN_POINT('Ctrl Pts',(-11.1573169271029,-84.8260470355,79.655886975436));
#128410=CARTESIAN_POINT('Ctrl Pts',(-11.1769584752109,-85.12145769654,79.198059264838));
#128411=CARTESIAN_POINT('Ctrl Pts',(-11.1831506639509,-85.39402078712,78.730082377384));
#128412=CARTESIAN_POINT('Ctrl Pts',(-11.1784735365659,-85.64789670709,78.244734052057));
#128413=CARTESIAN_POINT('Ctrl Pts',(-11.1640775262769,-85.88857428129,77.727362293743));
#128414=CARTESIAN_POINT('Ctrl Pts',(-11.1396203123759,-86.11970476943,77.1588049595881));
#128415=CARTESIAN_POINT('Ctrl Pts',(-11.1031949555669,-86.34044091572,76.519219618205));
#128416=CARTESIAN_POINT('Ctrl Pts',(-11.0569980784489,-86.54038984716,75.803498053924));
#128417=CARTESIAN_POINT('Ctrl Pts',(-11.0088524120349,-86.70225414811,75.0319261570531));
#128418=CARTESIAN_POINT('Ctrl Pts',(-10.9716584360619,-86.81172328639,74.248802525509));
#128419=CARTESIAN_POINT('Ctrl Pts',(-10.9510744529809,-86.8652632226401,
73.5164284997833));
#128420=CARTESIAN_POINT('Ctrl Pts',(-10.9475709444619,-86.8718595485001,
73.0510699681692));
#128421=CARTESIAN_POINT('Ctrl Pts',(-10.9483529868409,-86.86917777529,72.8388787541773));
#128422=CARTESIAN_POINT('Ctrl Pts',(-10.4122773932589,-83.71521774574,81.310962378986));
#128423=CARTESIAN_POINT('Ctrl Pts',(-10.4134352738449,-83.71925911704,81.306728931525));
#128424=CARTESIAN_POINT('Ctrl Pts',(-10.4429071435399,-83.82257558211,81.198344207213));
#128425=CARTESIAN_POINT('Ctrl Pts',(-10.4967869947709,-84.03534630022,80.966710627961));
#128426=CARTESIAN_POINT('Ctrl Pts',(-10.5596337460819,-84.35199707519,80.594065561619));
#128427=CARTESIAN_POINT('Ctrl Pts',(-10.6082092722099,-84.6753115925,80.178819271204));
#128428=CARTESIAN_POINT('Ctrl Pts',(-10.6416579613369,-84.98813663679,79.737577062465));
#128429=CARTESIAN_POINT('Ctrl Pts',(-10.6609036786939,-85.2807609136999,
79.282660284474));
#128430=CARTESIAN_POINT('Ctrl Pts',(-10.6669897319839,-85.5517753356901,
78.81688996442));
#128431=CARTESIAN_POINT('Ctrl Pts',(-10.6623899423179,-85.80568693668,78.331931220347));
#128432=CARTESIAN_POINT('Ctrl Pts',(-10.6481691595579,-86.0474022836899,
77.813716616604));
#128433=CARTESIAN_POINT('Ctrl Pts',(-10.6239668051929,-86.2803723129499,
77.243268394502));
#128434=CARTESIAN_POINT('Ctrl Pts',(-10.5878356887969,-86.50396071259,76.59999083105));
#128435=CARTESIAN_POINT('Ctrl Pts',(-10.5417467338089,-86.70833313634,75.875645948436));
#128436=CARTESIAN_POINT('Ctrl Pts',(-10.4933933817809,-86.87536834288,75.089346899771));
#128437=CARTESIAN_POINT('Ctrl Pts',(-10.4558141288379,-86.9892527291599,
74.285987846374));
#128438=CARTESIAN_POINT('Ctrl Pts',(-10.4349911321279,-87.04512245748,73.5334433267483));
#128439=CARTESIAN_POINT('Ctrl Pts',(-10.4314306474199,-87.05208533402,73.0538104694048));
#128440=CARTESIAN_POINT('Ctrl Pts',(-10.4322248470459,-87.04928618213,72.834848284201));
#128441=CARTESIAN_POINT('Ctrl Pts',(-11.2182969702623,-84.8936789842178,
82.3980377633591));
#128442=CARTESIAN_POINT('Ctrl Pts',(-11.2433855557306,-84.8786414224159,
82.3897381760834));
#128443=CARTESIAN_POINT('Ctrl Pts',(-11.2679068003975,-84.8626035236921,
82.3803586826996));
#128444=CARTESIAN_POINT('Ctrl Pts',(-11.2916243250072,-84.8456399233827,
82.3699174155352));
#128445=CARTESIAN_POINT('Ctrl Pts',(-11.3151598443708,-84.8288064995694,
82.3595562733177));
#128446=CARTESIAN_POINT('Ctrl Pts',(-11.3379030705374,-84.8110617165967,
82.3481495705518));
#128447=CARTESIAN_POINT('Ctrl Pts',(-11.3596341093316,-84.7925135973983,
82.3357505614535));
#128448=CARTESIAN_POINT('Ctrl Pts',(-11.3812224972171,-84.7740872351986,
82.3234329442267));
#128449=CARTESIAN_POINT('Ctrl Pts',(-11.4018111484351,-84.7548684162775,
82.3101361680513));
#128450=CARTESIAN_POINT('Ctrl Pts',(-11.4212078536227,-84.7349936564423,
82.2959465950604));
#128451=CARTESIAN_POINT('Ctrl Pts',(-11.424977064801,-84.7311315486146,
82.2931892454686));
#128452=CARTESIAN_POINT('Ctrl Pts',(-11.4287013583715,-84.7272447543509,
82.290398281619));
#128453=CARTESIAN_POINT('Ctrl Pts',(-11.4323794650856,-84.7233343896316,
82.2875744770987));
#128454=CARTESIAN_POINT('Ctrl Pts',(-11.4512354021245,-84.7032877741644,
82.2730981488187));
#128455=CARTESIAN_POINT('Ctrl Pts',(-11.4688740430804,-84.6826203892961,
82.2577567169767));
#128456=CARTESIAN_POINT('Ctrl Pts',(-11.485147615708,-84.6614963607626,
82.2416701986431));
#128457=CARTESIAN_POINT('Ctrl Pts',(-11.5019402316215,-84.6396985843413,
82.2250706030935));
#128458=CARTESIAN_POINT('Ctrl Pts',(-11.5172785757103,-84.6174151865612,
82.2076780423576));
#128459=CARTESIAN_POINT('Ctrl Pts',(-11.53104990243,-84.5948418128098,82.1896502597164));
#128460=CARTESIAN_POINT('Ctrl Pts',(-11.544511691304,-84.5727758203458,
82.1720276871987));
#128461=CARTESIAN_POINT('Ctrl Pts',(-11.5564761293108,-84.5504334643273,
82.1537988106687));
#128462=CARTESIAN_POINT('Ctrl Pts',(-11.5668892660002,-84.5280015911096,
82.1351267153699));
#128463=CARTESIAN_POINT('Ctrl Pts',(-11.5773770291814,-84.5054089582615,
82.1163208051593));
#128464=CARTESIAN_POINT('Ctrl Pts',(-11.5862912234104,-84.4827261841208,
82.0970659351269));
#128465=CARTESIAN_POINT('Ctrl Pts',(-11.5936293209293,-84.4601379692456,
82.0775350777285));
#128466=CARTESIAN_POINT('Ctrl Pts',(-11.6010391730179,-84.4373288786418,
82.0578132405478));
#128467=CARTESIAN_POINT('Ctrl Pts',(-11.6068422524605,-84.4146167999226,
82.037810619652));
#128468=CARTESIAN_POINT('Ctrl Pts',(-11.6110867946357,-84.392176000142,
82.0177021343215));
#128469=CARTESIAN_POINT('Ctrl Pts',(-11.6154255116511,-84.369237300082,
81.9971474964223));
#128470=CARTESIAN_POINT('Ctrl Pts',(-11.6181362269336,-84.3465825828635,
81.9764828516226));
#128471=CARTESIAN_POINT('Ctrl Pts',(-11.6193176321618,-84.3243726751204,
81.9558821694911));
#128472=CARTESIAN_POINT('Ctrl Pts',(-11.6205146597371,-84.3018690740015,
81.9350090736266));
#128473=CARTESIAN_POINT('Ctrl Pts',(-11.6201423946605,-84.2798224502727,
81.9142021189062));
#128474=CARTESIAN_POINT('Ctrl Pts',(-11.6183421066293,-84.2583678331536,
81.8936208899891));
#128475=CARTESIAN_POINT('Ctrl Pts',(-11.616492258386,-84.2363225908918,
81.8724730794731));
#128476=CARTESIAN_POINT('Ctrl Pts',(-11.6131354923086,-84.214902618432,
81.8515639882498));
#128477=CARTESIAN_POINT('Ctrl Pts',(-11.6084537419359,-84.1942161957235,
81.8310374785355));
#128478=CARTESIAN_POINT('Ctrl Pts',(-11.6042944389499,-84.1758382189213,
81.8128015696655));
#128479=CARTESIAN_POINT('Ctrl Pts',(-11.5990901824507,-84.1580385852257,
81.7948672220324));
#128480=CARTESIAN_POINT('Ctrl Pts',(-11.5929787721051,-84.1408680578277,
81.7773140347692));
#128481=CARTESIAN_POINT('Ctrl Pts',(-11.5860445120705,-84.1213856642106,
81.7573974593739));
#128482=CARTESIAN_POINT('Ctrl Pts',(-11.5776480727554,-84.1018875939657,
81.7371276918464));
#128483=CARTESIAN_POINT('Ctrl Pts',(-11.5676769120622,-84.0825449312996,
81.7166394401541));
#128484=CARTESIAN_POINT('Ctrl Pts',(-11.5574726006912,-84.0627499887989,
81.6956721218904));
#128485=CARTESIAN_POINT('Ctrl Pts',(-11.5456179778182,-84.0431181587144,
81.6744760618832));
#128486=CARTESIAN_POINT('Ctrl Pts',(-11.5320349835769,-84.0238570172672,
81.6532282396095));
#128487=CARTESIAN_POINT('Ctrl Pts',(-11.5194075887975,-84.0059509479106,
81.6334752576613));
#128488=CARTESIAN_POINT('Ctrl Pts',(-11.5052863423841,-83.9883659472882,
81.6136781742483));
#128489=CARTESIAN_POINT('Ctrl Pts',(-11.4896522818661,-83.9712811933441,
81.5940009641816));
#128490=CARTESIAN_POINT('Ctrl Pts',(-11.4742397728455,-83.9544385487876,
81.5746026014014));
#128491=CARTESIAN_POINT('Ctrl Pts',(-11.4573567200337,-83.9380826848318,
81.5553212432214));
#128492=CARTESIAN_POINT('Ctrl Pts',(-11.4390326898169,-83.9223884465296,
81.5363280263991));
#128493=CARTESIAN_POINT('Ctrl Pts',(-11.4209217467494,-83.9068767139568,
81.5175556785877));
#128494=CARTESIAN_POINT('Ctrl Pts',(-11.4014030677723,-83.8920119462866,
81.4990653908471));
#128495=CARTESIAN_POINT('Ctrl Pts',(-11.3805550175105,-83.8779567998221,
81.4810281424953));
#128496=CARTESIAN_POINT('Ctrl Pts',(-11.3598956981088,-83.8640288901903,
81.4631541796955));
#128497=CARTESIAN_POINT('Ctrl Pts',(-11.3379311319091,-83.8508966205834,
81.4457257031722));
#128498=CARTESIAN_POINT('Ctrl Pts',(-11.3147861625713,-83.8387028673069,
81.4289058648591));
#128499=CARTESIAN_POINT('Ctrl Pts',(-11.291811934848,-83.8265990679678,
81.4122101073478));
#128500=CARTESIAN_POINT('Ctrl Pts',(-11.267675062256,-83.8154205147056,
81.3961146293196));
#128501=CARTESIAN_POINT('Ctrl Pts',(-11.2425414819819,-83.8052831936582,
81.3807668276438));
#128502=CARTESIAN_POINT('Ctrl Pts',(-11.2174805704165,-83.7951751826425,
81.3654634010599));
#128503=CARTESIAN_POINT('Ctrl Pts',(-11.1914293085413,-83.7861027995091,
81.3509038563171));
#128504=CARTESIAN_POINT('Ctrl Pts',(-11.1645884150797,-83.7781502842866,
81.3372138112605));
#128505=CARTESIAN_POINT('Ctrl Pts',(-11.137715324457,-83.770188229575,81.3235073442249));
#128506=CARTESIAN_POINT('Ctrl Pts',(-11.1100514689375,-83.7633489876007,
81.3106728816397));
#128507=CARTESIAN_POINT('Ctrl Pts',(-11.0818243842738,-83.7576811857671,
81.2988087855567));
#128508=CARTESIAN_POINT('Ctrl Pts',(-11.0601958237095,-83.7533383215754,
81.2897181081549));
#128509=CARTESIAN_POINT('Ctrl Pts',(-11.0382372286131,-83.7496824821535,
81.2811965966304));
#128510=CARTESIAN_POINT('Ctrl Pts',(-11.0160567890457,-83.7467203804265,
81.2732756023359));
#128511=CARTESIAN_POINT('Ctrl Pts',(-10.9868578190103,-83.7428209843256,
81.2628481771106));
#128512=CARTESIAN_POINT('Ctrl Pts',(-10.9572749163021,-83.7401251164008,
81.2534627663865));
#128513=CARTESIAN_POINT('Ctrl Pts',(-10.9275572528519,-83.7386131255171,
81.2451598069053));
#128514=CARTESIAN_POINT('Ctrl Pts',(-10.8976502687018,-83.7370915022755,
81.2368039522123));
#128515=CARTESIAN_POINT('Ctrl Pts',(-10.8676076690518,-83.7367686166817,
81.2295443295768));
#128516=CARTESIAN_POINT('Ctrl Pts',(-10.837673769809,-83.7375876583117,
81.2233853462825));
#128517=CARTESIAN_POINT('Ctrl Pts',(-10.8073511595244,-83.7384173357271,
81.2171463846068));
#128518=CARTESIAN_POINT('Ctrl Pts',(-10.777140872443,-83.7404183794199,
81.2120366270806));
#128519=CARTESIAN_POINT('Ctrl Pts',(-10.7472743538497,-83.7434992703846,
81.2080249338404));
#128520=CARTESIAN_POINT('Ctrl Pts',(-10.7423430476946,-83.7440079609616,
81.2073625570887));
#128521=CARTESIAN_POINT('Ctrl Pts',(-10.737421049655,-83.7445460278415,
81.2067300423042));
#128522=CARTESIAN_POINT('Ctrl Pts',(-10.7325093222788,-83.7451129887462,
81.2061271649026));
#128523=CARTESIAN_POINT('Ctrl Pts',(-10.1996868022679,-82.23194843945,84.7288031621899));
#128524=CARTESIAN_POINT('Ctrl Pts',(-10.2310549729399,-82.36225217191,84.64853404355));
#128525=CARTESIAN_POINT('Ctrl Pts',(-10.2941852691639,-82.62272957896,84.4820327658399));
#128526=CARTESIAN_POINT('Ctrl Pts',(-10.3878876652799,-83.00658824629,84.21807111946));
#128527=CARTESIAN_POINT('Ctrl Pts',(-10.4803333774059,-83.38465446058,83.93868646342));
#128528=CARTESIAN_POINT('Ctrl Pts',(-10.5704313181939,-83.75452094002,83.64531909529));
#128529=CARTESIAN_POINT('Ctrl Pts',(-10.6577223613839,-84.11597215343,83.33784927704));
#128530=CARTESIAN_POINT('Ctrl Pts',(-10.7418800834869,-84.46872560982,83.01615568715));
#128531=CARTESIAN_POINT('Ctrl Pts',(-10.8226451344339,-84.81241750864,82.680139979899));
#128532=CARTESIAN_POINT('Ctrl Pts',(-10.8743243729249,-85.0362970369799,
82.445396126594));
#128533=CARTESIAN_POINT('Ctrl Pts',(-10.8997098703319,-85.14736683005,82.3246922926509));
#128534=CARTESIAN_POINT('Ctrl Pts',(-10.9001033512449,-85.1490887083899,
82.32282002129));
#128535=CARTESIAN_POINT('Ctrl Pts',(-10.7444620454609,-82.0833175450401,
84.7154537425701));
#128536=CARTESIAN_POINT('Ctrl Pts',(-10.7758888964799,-82.21370092662,84.6366925769601));
#128537=CARTESIAN_POINT('Ctrl Pts',(-10.8392066322589,-82.47465378675,84.47305894541));
#128538=CARTESIAN_POINT('Ctrl Pts',(-10.9333668192599,-82.86002706205,84.21286727656));
#128539=CARTESIAN_POINT('Ctrl Pts',(-11.0264183851959,-83.24028739056,83.93672505408));
#128540=CARTESIAN_POINT('Ctrl Pts',(-11.1172518052149,-83.61295320576,83.64600480045));
#128541=CARTESIAN_POINT('Ctrl Pts',(-11.2053563091919,-83.97761128967,83.34065945251));
#128542=CARTESIAN_POINT('Ctrl Pts',(-11.2903648245519,-84.33382210991,83.0206402545));
#128543=CARTESIAN_POINT('Ctrl Pts',(-11.3719996179599,-84.68114887489,82.685863360081));
#128544=CARTESIAN_POINT('Ctrl Pts',(-11.4242587012799,-84.90751917291,82.4516886974891));
#128545=CARTESIAN_POINT('Ctrl Pts',(-11.4499326462989,-85.01984506826,82.3312125004971));
#128546=CARTESIAN_POINT('Ctrl Pts',(-11.4503305990829,-85.0215864245201,
82.3293437447811));
#128547=CARTESIAN_POINT('Ctrl Pts',(-11.0477735235679,-81.77845486342,84.34924299992));
#128548=CARTESIAN_POINT('Ctrl Pts',(-11.0792330457179,-81.9049022180901,
84.27378555556));
#128549=CARTESIAN_POINT('Ctrl Pts',(-11.1426551411729,-82.15816549389,84.1168578421401));
#128550=CARTESIAN_POINT('Ctrl Pts',(-11.2370702098559,-82.53266637268,83.8668591095801));
#128551=CARTESIAN_POINT('Ctrl Pts',(-11.3304590936439,-82.90261491216,83.601083179));
#128552=CARTESIAN_POINT('Ctrl Pts',(-11.4217020023379,-83.26556115233,83.32082030468));
#128553=CARTESIAN_POINT('Ctrl Pts',(-11.5102594123469,-83.62098684921,83.02606811274));
#128554=CARTESIAN_POINT('Ctrl Pts',(-11.5957416191302,-83.96837243791,82.716822523456));
#128555=CARTESIAN_POINT('Ctrl Pts',(-11.6778606542034,-84.30725103196,82.393010881238));
#128556=CARTESIAN_POINT('Ctrl Pts',(-11.7304425745,-84.52818768737,82.166329389436));
#128557=CARTESIAN_POINT('Ctrl Pts',(-11.7562771168898,-84.63782939136,82.049669415333));
#128558=CARTESIAN_POINT('Ctrl Pts',(-11.7566775594532,-84.63952913831,82.0478598454959));
#128559=CARTESIAN_POINT('Ctrl Pts',(-10.9126188732579,-81.5153702725701,
83.86802669304));
#128560=CARTESIAN_POINT('Ctrl Pts',(-10.9440638372539,-81.636422394,83.7955229542399));
#128561=CARTESIAN_POINT('Ctrl Pts',(-11.0074394303619,-81.87882547258,83.64478390263));
#128562=CARTESIAN_POINT('Ctrl Pts',(-11.1017409245619,-82.23712862778,83.40478070061));
#128563=CARTESIAN_POINT('Ctrl Pts',(-11.1949795005649,-82.59095703495,83.14976196043));
#128564=CARTESIAN_POINT('Ctrl Pts',(-11.2860399423799,-82.93797770321,82.880974608658));
#128565=CARTESIAN_POINT('Ctrl Pts',(-11.3743955388709,-83.27772823833,82.598403949157));
#128566=CARTESIAN_POINT('Ctrl Pts',(-11.4596666702309,-83.60973803331,82.302033671229));
#128567=CARTESIAN_POINT('Ctrl Pts',(-11.5415699287259,-83.9335725497799,
81.991791732945));
#128568=CARTESIAN_POINT('Ctrl Pts',(-11.594007993871,-84.14468032908,81.774660539086));
#128569=CARTESIAN_POINT('Ctrl Pts',(-11.6197709745725,-84.2494409441699,
81.662926717437));
#128570=CARTESIAN_POINT('Ctrl Pts',(-11.6201703076981,-84.25106502002,81.661193562179));
#128571=CARTESIAN_POINT('Ctrl Pts',(-10.7774642229489,-81.25228568173,83.38681038616));
#128572=CARTESIAN_POINT('Ctrl Pts',(-10.8088946287909,-81.36794256992,83.31726035291));
#128573=CARTESIAN_POINT('Ctrl Pts',(-10.8722237195519,-81.5994854512799,
83.17270996312));
#128574=CARTESIAN_POINT('Ctrl Pts',(-10.9664116392669,-81.94159088287,82.942702291641));
#128575=CARTESIAN_POINT('Ctrl Pts',(-11.0594999074859,-82.27929915774,82.698440741869));
#128576=CARTESIAN_POINT('Ctrl Pts',(-11.1503778824219,-82.61039425409,82.441128912633));
#128577=CARTESIAN_POINT('Ctrl Pts',(-11.2385316653959,-82.93446962745,82.170739785574));
#128578=CARTESIAN_POINT('Ctrl Pts',(-11.3235917213319,-83.25110362872,81.887244819002));
#128579=CARTESIAN_POINT('Ctrl Pts',(-11.4052792032479,-83.55989406761,81.590572584651));
#128580=CARTESIAN_POINT('Ctrl Pts',(-11.4575734132419,-83.76117297079,81.382991688735));
#128581=CARTESIAN_POINT('Ctrl Pts',(-11.4832648322549,-83.86105249698,81.27618401954));
#128582=CARTESIAN_POINT('Ctrl Pts',(-11.4836630559429,-83.86260090173,81.274527278862));
#128583=CARTESIAN_POINT('Ctrl Pts',(-10.2916270839719,-81.20185397504,83.10314097868));
#128584=CARTESIAN_POINT('Ctrl Pts',(-10.3230051579719,-81.31416065537,83.03427618836));
#128585=CARTESIAN_POINT('Ctrl Pts',(-10.3861670878749,-81.5387264805201,
82.891377636428));
#128586=CARTESIAN_POINT('Ctrl Pts',(-10.4799467441519,-81.86982936611,82.664675941307));
#128587=CARTESIAN_POINT('Ctrl Pts',(-10.5724947046279,-82.19607927414,82.424575630003));
#128588=CARTESIAN_POINT('Ctrl Pts',(-10.6627167703069,-82.51538654248,82.172304055685));
#128589=CARTESIAN_POINT('Ctrl Pts',(-10.7501450991309,-82.82752507745,81.907772869607));
#128590=CARTESIAN_POINT('Ctrl Pts',(-10.8344464073679,-83.13221937986,81.630892336144));
#128591=CARTESIAN_POINT('Ctrl Pts',(-10.9153582424579,-83.42914104018,81.341580665038));
#128592=CARTESIAN_POINT('Ctrl Pts',(-10.9671353398329,-83.62257973927,81.139404226637));
#128593=CARTESIAN_POINT('Ctrl Pts',(-10.9925695177819,-83.7185515713301,
81.035433078134));
#128594=CARTESIAN_POINT('Ctrl Pts',(-10.9929637534009,-83.72003939198,81.033820349075));
#128595=CARTESIAN_POINT('Ctrl Pts',(-9.77066117414391,-81.3968308051,83.20126320814));
#128596=CARTESIAN_POINT('Ctrl Pts',(-9.80198313241291,-81.51000828017,83.13037012931));
#128597=CARTESIAN_POINT('Ctrl Pts',(-9.86496581478391,-81.73601182397,82.983513714113));
#128598=CARTESIAN_POINT('Ctrl Pts',(-9.95830768786792,-82.0684535513199,
82.751281192542));
#128599=CARTESIAN_POINT('Ctrl Pts',(-10.0502762732979,-82.39534912611,82.506043422008));
#128600=CARTESIAN_POINT('Ctrl Pts',(-10.1397950037739,-82.71466256519,82.249103163521));
#128601=CARTESIAN_POINT('Ctrl Pts',(-10.2264454240119,-83.02635562299,81.980301564201));
#128602=CARTESIAN_POINT('Ctrl Pts',(-10.3099331228039,-83.33030121714,81.699478477315));
#128603=CARTESIAN_POINT('Ctrl Pts',(-10.3900132274179,-83.62623823057,81.40653750512));
#128604=CARTESIAN_POINT('Ctrl Pts',(-10.4412358220089,-83.8189176504501,
81.202109460885));
#128605=CARTESIAN_POINT('Ctrl Pts',(-10.4663941589129,-83.91449325055,81.09704286655));
#128606=CARTESIAN_POINT('Ctrl Pts',(-10.4667841181019,-83.9159749237701,
81.095413160376));
#128607=CARTESIAN_POINT('Origin',(-8.56753648333091,1.4210854715202E-14,
72.98888938658));
#128608=CARTESIAN_POINT('',(-8.56795784296129,-66.4424972638774,69.9758907965238));
#128609=CARTESIAN_POINT('Ctrl Pts',(-8.56753648333091,-72.6784966214787,
81.061721731149));
#128610=CARTESIAN_POINT('Ctrl Pts',(-8.56753648333091,-72.0736574609292,
80.9189296982678));
#128611=CARTESIAN_POINT('Ctrl Pts',(-8.56753648333125,-71.4844480422102,
80.7093614983211));
#128612=CARTESIAN_POINT('Ctrl Pts',(-8.56753648333125,-70.3508022556626,
80.1607120918089));
#128613=CARTESIAN_POINT('Ctrl Pts',(-8.56753648333122,-69.8135934358944,
79.8216225166484));
#128614=CARTESIAN_POINT('Ctrl Pts',(-8.56753648333122,-68.4473368829776,
78.7233837561792));
#128615=CARTESIAN_POINT('Ctrl Pts',(-8.56753648333092,-67.7165424986972,
77.8572780272833));
#128616=CARTESIAN_POINT('Ctrl Pts',(-8.56753648333092,-66.4689218847558,
75.6285559895337));
#128617=CARTESIAN_POINT('Ctrl Pts',(-8.56753648333069,-66.2230924334251,
74.4581989464032));
#128618=CARTESIAN_POINT('Ctrl Pts',(-8.56753648333069,-66.0482530107463,
73.0618974695663));
#128619=CARTESIAN_POINT('Ctrl Pts',(-8.56753648333066,-66.0347923157517,
72.4374342122791));
#128620=CARTESIAN_POINT('Ctrl Pts',(-8.56753648333066,-66.1408479418231,
71.1931468548539));
#128621=CARTESIAN_POINT('Ctrl Pts',(-8.56753648333091,-66.2606244843831,
70.5750930481944));
#128622=CARTESIAN_POINT('Ctrl Pts',(-8.56753648333091,-66.4418053341428,
69.9756606261135));
#128623=CARTESIAN_POINT('',(-8.56568834200734,-73.334592210701,64.0777114412437));
#128624=CARTESIAN_POINT('Ctrl Pts',(-8.56753648333091,-66.4431946200656,
69.976105782015));
#128625=CARTESIAN_POINT('Ctrl Pts',(-8.56753648333091,-66.7099427616035,
69.2296629521477));
#128626=CARTESIAN_POINT('Ctrl Pts',(-8.56753648333093,-67.0759536435953,
68.5186782220475));
#128627=CARTESIAN_POINT('Ctrl Pts',(-8.56753648333093,-67.9733465906314,
67.2115334810726));
#128628=CARTESIAN_POINT('Ctrl Pts',(-8.56753648333091,-68.5055791540009,
66.6142037248065));
#128629=CARTESIAN_POINT('Ctrl Pts',(-8.56753648333091,-69.8717500230355,
65.4338849316529));
#128630=CARTESIAN_POINT('Ctrl Pts',(-8.56753648333092,-70.5858970496848,
65.0401447415795));
#128631=CARTESIAN_POINT('Ctrl Pts',(-8.56753648333092,-71.797320001775,
64.4667419598192));
#128632=CARTESIAN_POINT('Ctrl Pts',(-8.56753648333091,-72.5576048061066,
64.2249906466459));
#128633=CARTESIAN_POINT('Ctrl Pts',(-8.56753648333091,-73.3353239041699,
64.0818175558208));
#128634=CARTESIAN_POINT('Ctrl Pts',(-8.56753648333091,-73.3334510577524,
64.0699842298794));
#128635=CARTESIAN_POINT('Ctrl Pts',(-8.56753648333091,-73.9396539367879,
63.9867207515655));
#128636=CARTESIAN_POINT('Ctrl Pts',(-8.56753648333073,-74.5544091401536,
63.965415257747));
#128637=CARTESIAN_POINT('Ctrl Pts',(-8.56753648333073,-75.7715247557608,
64.0447290124391));
#128638=CARTESIAN_POINT('Ctrl Pts',(-8.56753648333076,-76.3744099119309,
64.144574635375));
#128639=CARTESIAN_POINT('Ctrl Pts',(-8.56753648333076,-78.0901283056316,
64.611417005806));
#128640=CARTESIAN_POINT('Ctrl Pts',(-8.5675364833309,-79.1248322783208,
65.1310007962587));
#128641=CARTESIAN_POINT('Ctrl Pts',(-8.5675364833309,-80.9371209889916,
66.5524367891479));
#128642=CARTESIAN_POINT('Ctrl Pts',(-8.567536483331,-81.6981213556041,67.42795058762));
#128643=CARTESIAN_POINT('Ctrl Pts',(-8.567536483331,-82.5704038623667,68.9625486543065));
#128644=CARTESIAN_POINT('Ctrl Pts',(-8.56753648333101,-82.814707297137,
69.5342669600823));
#128645=CARTESIAN_POINT('Ctrl Pts',(-8.56753648333101,-83.1721280645855,
70.7266324610845));
#128646=CARTESIAN_POINT('Ctrl Pts',(-8.56753648333091,-83.2844104837004,
71.3379527534998));
#128647=CARTESIAN_POINT('Ctrl Pts',(-8.56753648333091,-83.3301907683851,
71.9538361593952));
#128648=CARTESIAN_POINT('Ctrl Pts',(-9.33949250599091,-68.28843467669,68.385749441946));
#128649=CARTESIAN_POINT('Ctrl Pts',(-9.28372478921891,-67.21314456544,69.953566173561));
#128650=CARTESIAN_POINT('Ctrl Pts',(-9.17218935567391,-66.21224057553,73.8663634510705));
#128651=CARTESIAN_POINT('Ctrl Pts',(-9.00488620535791,-68.84902572167,79.327681027565));
#128652=CARTESIAN_POINT('Ctrl Pts',(-8.83758305504191,-74.3860768082,81.799718607153));
#128653=CARTESIAN_POINT('Ctrl Pts',(-8.67027990472591,-80.21224973459,80.119224478064));
#128654=CARTESIAN_POINT('Ctrl Pts',(-8.50297675440891,-83.58160767004,75.077818068246));
#128655=CARTESIAN_POINT('Ctrl Pts',(-8.33567360409291,-82.90653225676,69.051693466476));
#128656=CARTESIAN_POINT('Ctrl Pts',(-8.16837045377691,-78.50298784705,64.8818706633));
#128657=CARTESIAN_POINT('Ctrl Pts',(-8.05683502023291,-74.47097197897,64.648120002453));
#128658=CARTESIAN_POINT('Ctrl Pts',(-8.00106730345991,-72.65076867909,65.196898714115));
#128659=CARTESIAN_POINT('Ctrl Pts',(-9.57007551786691,-67.95907438126,68.159857051868));
#128660=CARTESIAN_POINT('Ctrl Pts',(-9.51430780109491,-66.83101597355,69.804612106664));
#128661=CARTESIAN_POINT('Ctrl Pts',(-9.40277236755091,-65.78099407777,73.9094242130813));
#128662=CARTESIAN_POINT('Ctrl Pts',(-9.23546921723391,-68.54717561549,79.638747997329));
#128663=CARTESIAN_POINT('Ctrl Pts',(-9.06816606691691,-74.3559494215,82.232097221564));
#128664=CARTESIAN_POINT('Ctrl Pts',(-8.90086291659891,-80.46803330067,80.469135290092));
#128665=CARTESIAN_POINT('Ctrl Pts',(-8.73355976628091,-84.00273757062,75.180329201596));
#128666=CARTESIAN_POINT('Ctrl Pts',(-8.56625661596291,-83.29453381444,68.858481309736));
#128667=CARTESIAN_POINT('Ctrl Pts',(-8.39895346564491,-78.67489187492,64.484030524229));
#128668=CARTESIAN_POINT('Ctrl Pts',(-8.28741803209991,-74.4450106992,64.238808890051));
#128669=CARTESIAN_POINT('Ctrl Pts',(-8.23165031532691,-72.5354835728,64.814518117892));
#128670=CARTESIAN_POINT('Ctrl Pts',(-9.80065852974291,-67.62971408584,67.93396466179));
#128671=CARTESIAN_POINT('Ctrl Pts',(-9.74489081297091,-66.44888738166,69.655658039767));
#128672=CARTESIAN_POINT('Ctrl Pts',(-9.63335537942691,-65.34974758001,73.9524849750929));
#128673=CARTESIAN_POINT('Ctrl Pts',(-9.46605222911091,-68.24532550932,79.949814967102));
#128674=CARTESIAN_POINT('Ctrl Pts',(-9.29874907879591,-74.32582203482,82.66447583598));
#128675=CARTESIAN_POINT('Ctrl Pts',(-9.13144592848091,-80.72381686678,80.8190461021));
#128676=CARTESIAN_POINT('Ctrl Pts',(-8.96414277816591,-84.42386747123,75.282840334888));
#128677=CARTESIAN_POINT('Ctrl Pts',(-8.79683962785091,-83.68253537209,68.665269152917));
#128678=CARTESIAN_POINT('Ctrl Pts',(-8.62953647753691,-78.84679590269,64.086190385108));
#128679=CARTESIAN_POINT('Ctrl Pts',(-8.51800104399391,-74.41904941931,63.829497777655));
#128680=CARTESIAN_POINT('Ctrl Pts',(-8.46223332722191,-72.4201984664,64.432137521706));
#128681=CARTESIAN_POINT('Ctrl Pts',(-10.0312415416199,-67.30035379041,67.708072271712));
#128682=CARTESIAN_POINT('Ctrl Pts',(-9.97547382484791,-66.06675878978,69.50670397287));
#128683=CARTESIAN_POINT('Ctrl Pts',(-9.86393839130291,-64.91850108225,73.995545737104));
#128684=CARTESIAN_POINT('Ctrl Pts',(-9.69663524098691,-67.94347540314,80.260881936865));
#128685=CARTESIAN_POINT('Ctrl Pts',(-9.52933209067091,-74.29569464812,83.09685445039));
#128686=CARTESIAN_POINT('Ctrl Pts',(-9.36202894035391,-80.97960043285,81.168956914129));
#128687=CARTESIAN_POINT('Ctrl Pts',(-9.19472579003791,-84.84499737182,75.38535146824));
#128688=CARTESIAN_POINT('Ctrl Pts',(-9.02742263972191,-84.07053692978,68.47205699618));
#128689=CARTESIAN_POINT('Ctrl Pts',(-8.86011948940491,-79.01869993056,63.68835024604));
#128690=CARTESIAN_POINT('Ctrl Pts',(-8.74858405586091,-74.39308813955,63.420186665253));
#128691=CARTESIAN_POINT('Ctrl Pts',(-8.69281633908891,-72.30491336013,64.049756925482));
#128692=CARTESIAN_POINT('',(-9.85448345426765,-67.0071858774639,68.6911520794415));
#128693=CARTESIAN_POINT('Ctrl Pts',(-9.85448345426765,-67.0071858774639,
68.6911520794415));
#128694=CARTESIAN_POINT('Ctrl Pts',(-9.79971249899291,-66.0535515884723,
70.4917741499841));
#128695=CARTESIAN_POINT('Ctrl Pts',(-9.74592499989422,-65.7106640987246,
72.62028225223));
#128696=CARTESIAN_POINT('Ctrl Pts',(-9.63834989066502,-66.4347938378737,
76.617555712199));
#128697=CARTESIAN_POINT('Ctrl Pts',(-9.58456228053448,-67.5188766918498,
78.4829403854034));
#128698=CARTESIAN_POINT('Ctrl Pts',(-9.51732776787134,-69.4294746814203,
80.1653430250265));
#128699=CARTESIAN_POINT('Ctrl Pts',(-9.5038808653387,-69.8393117287546,
80.4693684884601));
#128700=CARTESIAN_POINT('Ctrl Pts',(-9.47698706027345,-70.705657587077,
81.0004575955979));
#128701=CARTESIAN_POINT('Ctrl Pts',(-9.46354015774083,-71.1625234758073,
81.2268973342743));
#128702=CARTESIAN_POINT('Ctrl Pts',(-9.3963056450777,-73.5294734721993,
82.1577931504897));
#128703=CARTESIAN_POINT('Ctrl Pts',(-9.34251803494718,-75.6862304181982,
82.2604177652121));
#128704=CARTESIAN_POINT('Ctrl Pts',(-9.26183661975145,-78.6050687686331,
81.3802459755177));
#128705=CARTESIAN_POINT('Ctrl Pts',(-9.2349428146862,-79.5243766321848,
80.911716381337));
#128706=CARTESIAN_POINT('Ctrl Pts',(-9.16770830202308,-81.577804542804,
79.4008185283445));
#128707=CARTESIAN_POINT('Ctrl Pts',(-9.12736759442522,-82.5896606086484,
78.1891376421487));
#128708=CARTESIAN_POINT('Ctrl Pts',(-9.07357998429472,-83.4468232021015,
76.3465169977388));
#128709=CARTESIAN_POINT('Ctrl Pts',(-9.0601330817621,-83.6196372087911,
75.8667299911412));
#128710=CARTESIAN_POINT('Ctrl Pts',(-8.99289856909898,-84.2755040487159,
73.4089183747913));
#128711=CARTESIAN_POINT('Ctrl Pts',(-8.93911095896847,-84.1348835562278,
71.2546776032613));
#128712=CARTESIAN_POINT('Ctrl Pts',(-8.83153573870747,-82.5254092780411,
67.5221796143094));
#128713=CARTESIAN_POINT('Ctrl Pts',(-8.77774812857696,-81.0499897572754,
65.9468497653013));
#128714=CARTESIAN_POINT('Ctrl Pts',(-8.71051361591392,-78.8096606761766,
64.7397816608276));
#128715=CARTESIAN_POINT('Ctrl Pts',(-8.69706671338133,-78.3418002183133,
64.5364691422482));
#128716=CARTESIAN_POINT('Ctrl Pts',(-8.67017290831613,-77.3775596950603,
64.2160019939825));
#128717=CARTESIAN_POINT('Ctrl Pts',(-8.65672600578354,-76.8811017434786,
64.0990887496991));
#128718=CARTESIAN_POINT('Ctrl Pts',(-8.61640526799513,-75.3716441191094,
63.8760691192961));
#128719=CARTESIAN_POINT('Ctrl Pts',(-8.58953143273933,-74.3378692213475,
63.8972735937159));
#128720=CARTESIAN_POINT('Ctrl Pts',(-8.56568834200734,-73.334592210701,
64.0777114412437));
#128721=CARTESIAN_POINT('',(-9.46541110279056,-67.6020149116865,69.0109979579471));
#128722=CARTESIAN_POINT('Ctrl Pts',(-9.99199816632791,-67.59428425961,67.303209521688));
#128723=CARTESIAN_POINT('Ctrl Pts',(-9.95025389358791,-66.60009764549,68.598158170228));
#128724=CARTESIAN_POINT('Ctrl Pts',(-9.86676534810891,-65.30823381695,71.71969580549));
#128725=CARTESIAN_POINT('Ctrl Pts',(-9.74153252989091,-65.975649193,76.744817636531));
#128726=CARTESIAN_POINT('Ctrl Pts',(-9.61629971167191,-69.0702482942,80.759474381881));
#128727=CARTESIAN_POINT('Ctrl Pts',(-9.49106689345391,-73.75942478415,82.684532165368));
#128728=CARTESIAN_POINT('Ctrl Pts',(-9.36583407523591,-78.78224537899,82.00215805984));
#128729=CARTESIAN_POINT('Ctrl Pts',(-9.24060125701691,-82.78791878897,78.895896207008));
#128730=CARTESIAN_POINT('Ctrl Pts',(-9.11536843879891,-84.6992258503,74.201089045578));
#128731=CARTESIAN_POINT('Ctrl Pts',(-8.99013562057991,-84.00216577159,69.180291345096));
#128732=CARTESIAN_POINT('Ctrl Pts',(-8.86490280236191,-80.88419637879,65.183721669986));
#128733=CARTESIAN_POINT('Ctrl Pts',(-8.73966998414291,-76.18381732287,63.28615857581));
#128734=CARTESIAN_POINT('Ctrl Pts',(-8.61443716592491,-71.16508250412,63.997905008714));
#128735=CARTESIAN_POINT('Ctrl Pts',(-8.48920434770591,-67.17764413613,67.127552977624));
#128736=CARTESIAN_POINT('Ctrl Pts',(-8.36397152948791,-65.29387078721,71.833466448308));
#128737=CARTESIAN_POINT('Ctrl Pts',(-8.23873871126891,-66.02018597587,76.850086687758));
#128738=CARTESIAN_POINT('Ctrl Pts',(-8.11350589305091,-69.16190222137,80.828391821067));
#128739=CARTESIAN_POINT('Ctrl Pts',(-8.03001734757191,-72.30180432462,82.07495675794));
#128740=CARTESIAN_POINT('Ctrl Pts',(-7.98827307483191,-73.92349052215,82.263193053033));
#128741=CARTESIAN_POINT('Ctrl Pts',(-10.2225811782039,-67.91107137654,67.546420332812));
#128742=CARTESIAN_POINT('Ctrl Pts',(-10.1808369054639,-66.95941211861,68.78597621942));
#128743=CARTESIAN_POINT('Ctrl Pts',(-10.0973483599859,-65.72280909565,71.77398686789));
#128744=CARTESIAN_POINT('Ctrl Pts',(-9.97211554176791,-66.36167509171,76.584153937925));
#128745=CARTESIAN_POINT('Ctrl Pts',(-9.84688272354991,-69.32389952966,80.42707960685));
#128746=CARTESIAN_POINT('Ctrl Pts',(-9.72164990533191,-73.81249166652,82.269791061293));
#128747=CARTESIAN_POINT('Ctrl Pts',(-9.59641708711391,-78.6204559381,81.616606210807));
#128748=CARTESIAN_POINT('Ctrl Pts',(-9.47118426889691,-82.45478254308,78.643217907434));
#128749=CARTESIAN_POINT('Ctrl Pts',(-9.34595145067991,-84.28433147665,74.149235956863));
#128750=CARTESIAN_POINT('Ctrl Pts',(-9.22071863246191,-83.61708886061,69.343208048246));
#128751=CARTESIAN_POINT('Ctrl Pts',(-9.09548581424491,-80.63249381933,65.517595756513));
#128752=CARTESIAN_POINT('Ctrl Pts',(-8.97025299602791,-76.13317831779,63.701202877746));
#128753=CARTESIAN_POINT('Ctrl Pts',(-8.84502017781091,-71.32912504901,64.382503624079));
#128754=CARTESIAN_POINT('Ctrl Pts',(-8.71978735959391,-67.51225346334,67.37827767835));
#128755=CARTESIAN_POINT('Ctrl Pts',(-8.59455454137691,-65.70906045929,71.88289085437));
#128756=CARTESIAN_POINT('Ctrl Pts',(-8.46932172315991,-66.40430676786,76.684919997149));
#128757=CARTESIAN_POINT('Ctrl Pts',(-8.34408890494191,-69.41163286577,80.493049031651));
#128758=CARTESIAN_POINT('Ctrl Pts',(-8.26060035946391,-72.41722242321,81.686290869658));
#128759=CARTESIAN_POINT('Ctrl Pts',(-8.21885608672491,-73.96953932369,81.866475163376));
#128760=CARTESIAN_POINT('Ctrl Pts',(-10.4531641900799,-68.22785849346,67.789631143935));
#128761=CARTESIAN_POINT('Ctrl Pts',(-10.4114199173409,-67.31872659173,68.973794268612));
#128762=CARTESIAN_POINT('Ctrl Pts',(-10.3279313718619,-66.13738437435,71.82827793029));
#128763=CARTESIAN_POINT('Ctrl Pts',(-10.2026985536429,-66.74770099042,76.423490239315));
#128764=CARTESIAN_POINT('Ctrl Pts',(-10.0774657354239,-69.57755076511,80.09468483181));
#128765=CARTESIAN_POINT('Ctrl Pts',(-9.95223291720491,-73.86555854886,81.855049957214));
#128766=CARTESIAN_POINT('Ctrl Pts',(-9.82700009898591,-78.45866649718,81.231054361786));
#128767=CARTESIAN_POINT('Ctrl Pts',(-9.70176728076691,-82.12164629715,78.390539607897));
#128768=CARTESIAN_POINT('Ctrl Pts',(-9.57653446254691,-83.86943710299,74.097382868212));
#128769=CARTESIAN_POINT('Ctrl Pts',(-9.45130164432791,-83.23201194965,69.506124751474));
#128770=CARTESIAN_POINT('Ctrl Pts',(-9.32606882610791,-80.38079125995,65.851469843104));
#128771=CARTESIAN_POINT('Ctrl Pts',(-9.20083600788791,-76.08253931283,64.116247179702));
#128772=CARTESIAN_POINT('Ctrl Pts',(-9.07560318966791,-71.49316759404,64.76710223939));
#128773=CARTESIAN_POINT('Ctrl Pts',(-8.95037037144891,-67.84686279065,67.629002378947));
#128774=CARTESIAN_POINT('Ctrl Pts',(-8.82513755322891,-66.1242501314,71.932315260248));
#128775=CARTESIAN_POINT('Ctrl Pts',(-8.69990473500891,-66.78842755977,76.519753306352));
#128776=CARTESIAN_POINT('Ctrl Pts',(-8.57467191678891,-69.66136350999,80.1577062421));
#128777=CARTESIAN_POINT('Ctrl Pts',(-8.49118337130991,-72.53264052159,81.29762498131));
#128778=CARTESIAN_POINT('Ctrl Pts',(-8.44943909856991,-74.01558812501,81.469757273692));
#128779=CARTESIAN_POINT('Ctrl Pts',(-10.6837472019569,-68.54464561039,68.032841955058));
#128780=CARTESIAN_POINT('Ctrl Pts',(-10.6420029292169,-67.67804106486,69.161612317803));
#128781=CARTESIAN_POINT('Ctrl Pts',(-10.5585143837379,-66.55195965305,71.882568992689));
#128782=CARTESIAN_POINT('Ctrl Pts',(-10.4332815655199,-67.13372688913,76.262826540709));
#128783=CARTESIAN_POINT('Ctrl Pts',(-10.3080487473019,-69.83120200056,79.762290056778));
#128784=CARTESIAN_POINT('Ctrl Pts',(-10.1828159290829,-73.91862543122,81.440308853139));
#128785=CARTESIAN_POINT('Ctrl Pts',(-10.0575831108649,-78.29687705629,80.845502512754));
#128786=CARTESIAN_POINT('Ctrl Pts',(-9.93235029264591,-81.78851005125,78.137861308325));
#128787=CARTESIAN_POINT('Ctrl Pts',(-9.80711747442791,-83.45454272935,74.0455297795));
#128788=CARTESIAN_POINT('Ctrl Pts',(-9.68188465620991,-82.84693503866,69.669041454627));
#128789=CARTESIAN_POINT('Ctrl Pts',(-9.55665183799091,-80.1290887005,66.185343929634));
#128790=CARTESIAN_POINT('Ctrl Pts',(-9.43141901977291,-76.03190030776,64.531291481639));
#128791=CARTESIAN_POINT('Ctrl Pts',(-9.30618620155491,-71.65721013894,65.151700854752));
#128792=CARTESIAN_POINT('Ctrl Pts',(-9.18095338333591,-68.18147211787,67.879727079667));
#128793=CARTESIAN_POINT('Ctrl Pts',(-9.05572056511791,-66.53943980348,71.981739666301));
#128794=CARTESIAN_POINT('Ctrl Pts',(-8.93048774689891,-67.17254835176,76.354586615735));
#128795=CARTESIAN_POINT('Ctrl Pts',(-8.80525492868091,-69.91109415439,79.822363452678));
#128796=CARTESIAN_POINT('Ctrl Pts',(-8.72176638320191,-72.64805862017,80.908959093025));
#128797=CARTESIAN_POINT('Ctrl Pts',(-8.68002211046191,-74.06163692655,81.073039384033));
#128798=CARTESIAN_POINT('',(-10.0985254848049,-67.01215254309,68.6936268804507));
#128799=CARTESIAN_POINT('',(-10.0976119119436,-67.0107639369115,68.6928899475042));
#128800=CARTESIAN_POINT('Ctrl Pts',(-10.1056201537506,-67.0100609947306,
68.6927734040079));
#128801=CARTESIAN_POINT('Ctrl Pts',(-10.0858288974105,-66.6260431282916,
69.4150543477338));
#128802=CARTESIAN_POINT('Ctrl Pts',(-10.0673827948632,-66.3411294788075,
70.1900495876074));
#128803=CARTESIAN_POINT('Ctrl Pts',(-10.0353495239254,-66.0633179308166,
71.4200744687751));
#128804=CARTESIAN_POINT('Ctrl Pts',(-10.0232792679854,-65.9963533493792,
71.8592112503599));
#128805=CARTESIAN_POINT('Ctrl Pts',(-10.0020449919732,-65.9382221349775,
72.5860608468921));
#128806=CARTESIAN_POINT('Ctrl Pts',(-9.99345424936893,-65.9286151577416,
72.8724489958298));
#128807=CARTESIAN_POINT('Ctrl Pts',(-9.96978124698292,-65.9394232775651,
73.6637855017629));
#128808=CARTESIAN_POINT('Ctrl Pts',(-9.95478264023665,-65.9884311928924,
74.1682378197038));
#128809=CARTESIAN_POINT('Ctrl Pts',(-9.93276979943483,-66.1405570108522,
74.9827935804844));
#128810=CARTESIAN_POINT('Ctrl Pts',(-9.9250031085192,-66.2175611627718,
75.2952032094914));
#128811=CARTESIAN_POINT('Ctrl Pts',(-9.90660496999056,-66.4505874392876,
76.0577540452807));
#128812=CARTESIAN_POINT('Ctrl Pts',(-9.89614883297556,-66.626578834097,
76.5013880191161));
#128813=CARTESIAN_POINT('Ctrl Pts',(-9.87648446127022,-66.9900401148003,
77.2443161242015));
#128814=CARTESIAN_POINT('Ctrl Pts',(-9.86781300305152,-67.1624496274915,
77.5510235654546));
#128815=CARTESIAN_POINT('Ctrl Pts',(-9.83445661031167,-67.864285454012,
78.6503572119695));
#128816=CARTESIAN_POINT('Ctrl Pts',(-9.80762292083788,-68.500619259633,
79.3771609760621));
#128817=CARTESIAN_POINT('Ctrl Pts',(-9.76803229526134,-69.538252857365,
80.2425287011678));
#128818=CARTESIAN_POINT('Ctrl Pts',(-9.75603894613835,-69.8608619067118,
80.4773256996633));
#128819=CARTESIAN_POINT('Ctrl Pts',(-9.7354525920193,-70.4740212840394,
80.8618096607943));
#128820=CARTESIAN_POINT('Ctrl Pts',(-9.72688917025221,-70.757447065395,
81.0176909946875));
#128821=CARTESIAN_POINT('Ctrl Pts',(-9.70180950486301,-71.6712457260181,
81.4557429774271));
#128822=CARTESIAN_POINT('Ctrl Pts',(-9.68700819128544,-72.3277386010445,
81.6799951258321));
#128823=CARTESIAN_POINT('Ctrl Pts',(-9.66320386310093,-73.3220371140291,
81.9007688530295));
#128824=CARTESIAN_POINT('Ctrl Pts',(-9.65519700831005,-73.6473197544878,
81.9550842937002));
#128825=CARTESIAN_POINT('Ctrl Pts',(-9.62768684262128,-74.6887798708784,
82.0731851906225));
#128826=CARTESIAN_POINT('Ctrl Pts',(-9.60600749490843,-75.4131320814911,
82.0722511733354));
#128827=CARTESIAN_POINT('Ctrl Pts',(-9.5728056010411,-76.5283475754138,
81.938809530694));
#128828=CARTESIAN_POINT('Ctrl Pts',(-9.56099613423051,-76.9266813718286,
81.8640002443785));
#128829=CARTESIAN_POINT('Ctrl Pts',(-9.53752942078241,-77.7541854435951,
81.6481365797571));
#128830=CARTESIAN_POINT('Ctrl Pts',(-9.52652650667813,-78.1764052469984,
81.5016462968993));
#128831=CARTESIAN_POINT('Ctrl Pts',(-9.49549132094949,-79.3626611652649,
80.9849160430836));
#128832=CARTESIAN_POINT('Ctrl Pts',(-9.47577017339058,-80.0888067054271,
80.5359409488921));
#128833=CARTESIAN_POINT('Ctrl Pts',(-9.43839760642428,-81.2371199228423,
79.5921011886046));
#128834=CARTESIAN_POINT('Ctrl Pts',(-9.42135872104697,-81.6912316979897,
79.1337121374095));
#128835=CARTESIAN_POINT('Ctrl Pts',(-9.39220782815627,-82.3240882281726,
78.3463877463461));
#128836=CARTESIAN_POINT('Ctrl Pts',(-9.38097818917659,-82.5379930731196,
78.0449993103856));
#128837=CARTESIAN_POINT('Ctrl Pts',(-9.35775260825943,-82.945334146773,
77.3886404803726));
#128838=CARTESIAN_POINT('Ctrl Pts',(-9.34582770326582,-83.1348815306979,
77.0313987126338));
#128839=CARTESIAN_POINT('Ctrl Pts',(-9.32494003038193,-83.4535024982193,
76.3117296668395));
#128840=CARTESIAN_POINT('Ctrl Pts',(-9.31587772144192,-83.5849139954119,
75.9509159743823));
#128841=CARTESIAN_POINT('Ctrl Pts',(-9.28861783421259,-83.9216282439495,
74.8011690336164));
#128842=CARTESIAN_POINT('Ctrl Pts',(-9.27067335198321,-84.0435701905272,
73.9876456980361));
#128843=CARTESIAN_POINT('Ctrl Pts',(-9.23559857568525,-84.0692658482991,
72.6688868688745));
#128844=CARTESIAN_POINT('Ctrl Pts',(-9.22129912397754,-84.0385238649345,
72.1639069572095));
#128845=CARTESIAN_POINT('Ctrl Pts',(-9.17806499529417,-83.8261976625481,
70.6799500060793));
#128846=CARTESIAN_POINT('Ctrl Pts',(-9.14973443391088,-83.5394059276481,
69.759533298521));
#128847=CARTESIAN_POINT('Ctrl Pts',(-9.11259821608478,-82.8754352936373,
68.457692926074));
#128848=CARTESIAN_POINT('Ctrl Pts',(-9.10120006670172,-82.6205555564293,
68.0464749363187));
#128849=CARTESIAN_POINT('Ctrl Pts',(-9.07117941927312,-81.8617738677188,
67.0142743202317));
#128850=CARTESIAN_POINT('Ctrl Pts',(-9.0526252660902,-81.3037983603748,
66.4320817378967));
#128851=CARTESIAN_POINT('Ctrl Pts',(-9.02101932872785,-80.3960614529603,
65.6984913538591));
#128852=CARTESIAN_POINT('Ctrl Pts',(-9.01027898281615,-80.095877405622,
65.4838148866877));
#128853=CARTESIAN_POINT('Ctrl Pts',(-8.97854614193354,-79.1982942694184,
64.919936575508));
#128854=CARTESIAN_POINT('Ctrl Pts',(-8.95702945793924,-78.5711451652899,
64.6180035181383));
#128855=CARTESIAN_POINT('Ctrl Pts',(-8.93208463483441,-77.6737217783435,
64.3127662936522));
#128856=CARTESIAN_POINT('Ctrl Pts',(-8.92586970758882,-77.4284089827495,
64.2415585305407));
#128857=CARTESIAN_POINT('Ctrl Pts',(-8.90731371882341,-76.656624899155,
64.0536446207396));
#128858=CARTESIAN_POINT('Ctrl Pts',(-8.89561309755475,-76.1209216390034,
63.9745840947576));
#128859=CARTESIAN_POINT('Ctrl Pts',(-8.86487641062158,-74.8360842494938,
63.8986189294642));
#128860=CARTESIAN_POINT('Ctrl Pts',(-8.8454456967949,-74.0835849981138,
63.9451390777231));
#128861=CARTESIAN_POINT('Ctrl Pts',(-8.80150233458386,-72.5160619401253,
64.2314456703135));
#128862=CARTESIAN_POINT('Ctrl Pts',(-8.77624830234048,-71.7038290454958,
64.4962199491525));
#128863=CARTESIAN_POINT('Ctrl Pts',(-8.74167392707594,-70.6373754027766,
65.0238411724459));
#128864=CARTESIAN_POINT('Ctrl Pts',(-8.7322116805582,-70.3402399112782,
65.1935581209927));
#128865=CARTESIAN_POINT('Ctrl Pts',(-8.71444262084913,-69.7582083441322,
65.5740566021455));
#128866=CARTESIAN_POINT('Ctrl Pts',(-8.70610048266984,-69.4763651028232,
65.7836686004065));
#128867=CARTESIAN_POINT('Ctrl Pts',(-8.6828861938593,-68.7101137563505,
66.4260840139121));
#128868=CARTESIAN_POINT('Ctrl Pts',(-8.66847293392533,-68.2575214534165,
66.8969486960608));
#128869=CARTESIAN_POINT('Ctrl Pts',(-8.63968961238916,-67.5604294912633,
67.7914454924441));
#128870=CARTESIAN_POINT('Ctrl Pts',(-8.62604720722989,-67.2920488707874,
68.1971115278178));
#128871=CARTESIAN_POINT('Ctrl Pts',(-8.59751203614483,-66.8162040163527,
69.0551559022318));
#128872=CARTESIAN_POINT('Ctrl Pts',(-8.58263360341257,-66.6102415503235,
69.5086547539668));
#128873=CARTESIAN_POINT('Ctrl Pts',(-8.56837920259168,-66.4431891936119,
69.976120966934));
#128874=CARTESIAN_POINT('Ctrl Pts',(-9.88022273965691,-67.62520219141,67.700413019766));
#128875=CARTESIAN_POINT('Ctrl Pts',(-9.81362168955091,-66.1498345501,69.757818081886));
#128876=CARTESIAN_POINT('Ctrl Pts',(-9.68041958933991,-65.03881684527,75.159924360853));
#128877=CARTESIAN_POINT('Ctrl Pts',(-9.48061643902391,-69.94095953137,81.84418107373));
#128878=CARTESIAN_POINT('Ctrl Pts',(-9.28081328870791,-78.18756436805,82.675374708005));
#128879=CARTESIAN_POINT('Ctrl Pts',(-9.08101013839191,-84.3279816375,77.109502645436));
#128880=CARTESIAN_POINT('Ctrl Pts',(-8.88120698807591,-84.30727308569,68.821968198106));
#128881=CARTESIAN_POINT('Ctrl Pts',(-8.68140383775991,-78.13920519194,63.285515123434));
#128882=CARTESIAN_POINT('Ctrl Pts',(-8.48160068744491,-69.89662703841,64.163123294247));
#128883=CARTESIAN_POINT('Ctrl Pts',(-8.34839858723391,-66.65138462743,68.622440986855));
#128884=CARTESIAN_POINT('Ctrl Pts',(-8.28179753712891,-66.12404568677,71.098635427588));
#128885=CARTESIAN_POINT('Ctrl Pts',(-9.96688940632291,-67.62520219141,67.700413019766));
#128886=CARTESIAN_POINT('Ctrl Pts',(-9.90028835621791,-66.1498345501,69.757818081886));
#128887=CARTESIAN_POINT('Ctrl Pts',(-9.76708625600691,-65.03881684527,75.159924360853));
#128888=CARTESIAN_POINT('Ctrl Pts',(-9.56728310569091,-69.94095953137,81.84418107373));
#128889=CARTESIAN_POINT('Ctrl Pts',(-9.36747995537491,-78.18756436805,82.675374708005));
#128890=CARTESIAN_POINT('Ctrl Pts',(-9.16767680505891,-84.3279816375,77.109502645436));
#128891=CARTESIAN_POINT('Ctrl Pts',(-8.96787365474291,-84.30727308569,68.821968198106));
#128892=CARTESIAN_POINT('Ctrl Pts',(-8.76807050442691,-78.13920519194,63.285515123434));
#128893=CARTESIAN_POINT('Ctrl Pts',(-8.56826735411091,-69.89662703841,64.163123294247));
#128894=CARTESIAN_POINT('Ctrl Pts',(-8.43506525390091,-66.65138462743,68.622440986855));
#128895=CARTESIAN_POINT('Ctrl Pts',(-8.36846420379491,-66.12404568677,71.098635427588));
#128896=CARTESIAN_POINT('Ctrl Pts',(-10.0535560729899,-67.62520219141,67.700413019766));
#128897=CARTESIAN_POINT('Ctrl Pts',(-9.98695502288491,-66.1498345501,69.757818081886));
#128898=CARTESIAN_POINT('Ctrl Pts',(-9.85375292267391,-65.03881684527,75.159924360853));
#128899=CARTESIAN_POINT('Ctrl Pts',(-9.65394977235791,-69.94095953137,81.84418107373));
#128900=CARTESIAN_POINT('Ctrl Pts',(-9.45414662204191,-78.18756436805,82.675374708005));
#128901=CARTESIAN_POINT('Ctrl Pts',(-9.25434347172591,-84.3279816375,77.109502645436));
#128902=CARTESIAN_POINT('Ctrl Pts',(-9.05454032140991,-84.30727308569,68.821968198106));
#128903=CARTESIAN_POINT('Ctrl Pts',(-8.85473717109391,-78.13920519194,63.285515123434));
#128904=CARTESIAN_POINT('Ctrl Pts',(-8.65493402077791,-69.89662703841,64.163123294247));
#128905=CARTESIAN_POINT('Ctrl Pts',(-8.52173192056691,-66.65138462743,68.622440986855));
#128906=CARTESIAN_POINT('Ctrl Pts',(-8.45513087046191,-66.12404568677,71.098635427588));
#128907=CARTESIAN_POINT('Ctrl Pts',(-10.1402227396569,-67.62520219141,67.700413019766));
#128908=CARTESIAN_POINT('Ctrl Pts',(-10.0736216895509,-66.1498345501,69.757818081886));
#128909=CARTESIAN_POINT('Ctrl Pts',(-9.94041958933991,-65.03881684527,75.159924360853));
#128910=CARTESIAN_POINT('Ctrl Pts',(-9.74061643902391,-69.94095953137,81.84418107373));
#128911=CARTESIAN_POINT('Ctrl Pts',(-9.54081328870791,-78.18756436805,82.675374708005));
#128912=CARTESIAN_POINT('Ctrl Pts',(-9.34101013839191,-84.3279816375,77.109502645436));
#128913=CARTESIAN_POINT('Ctrl Pts',(-9.14120698807591,-84.30727308569,68.821968198106));
#128914=CARTESIAN_POINT('Ctrl Pts',(-8.94140383775991,-78.13920519194,63.285515123434));
#128915=CARTESIAN_POINT('Ctrl Pts',(-8.74160068744491,-69.89662703841,64.163123294247));
#128916=CARTESIAN_POINT('Ctrl Pts',(-8.60839858723391,-66.65138462743,68.622440986855));
#128917=CARTESIAN_POINT('Ctrl Pts',(-8.54179753712891,-66.12404568677,71.098635427588));
#128918=CARTESIAN_POINT('Ctrl Pts',(-10.1421465283748,-67.62520219141,67.700413019766));
#128919=CARTESIAN_POINT('Ctrl Pts',(-10.0755454782688,-66.1498345501,69.757818081886));
#128920=CARTESIAN_POINT('Ctrl Pts',(-9.94234337805777,-65.03881684527,75.159924360853));
#128921=CARTESIAN_POINT('Ctrl Pts',(-9.74254022774178,-69.94095953137,81.84418107373));
#128922=CARTESIAN_POINT('Ctrl Pts',(-9.54273707742577,-78.18756436805,82.675374708005));
#128923=CARTESIAN_POINT('Ctrl Pts',(-9.34293392710978,-84.3279816375,77.109502645436));
#128924=CARTESIAN_POINT('Ctrl Pts',(-9.14313077679378,-84.30727308569,68.821968198106));
#128925=CARTESIAN_POINT('Ctrl Pts',(-8.94332762647777,-78.13920519194,63.285515123434));
#128926=CARTESIAN_POINT('Ctrl Pts',(-8.7435244761628,-69.89662703841,64.163123294247));
#128927=CARTESIAN_POINT('Ctrl Pts',(-8.6103223759518,-66.65138462743,68.622440986855));
#128928=CARTESIAN_POINT('Ctrl Pts',(-8.5437213258468,-66.12404568677,71.098635427588));
#128929=CARTESIAN_POINT('Ctrl Pts',(-10.1440703170927,-67.62520219141,67.700413019766));
#128930=CARTESIAN_POINT('Ctrl Pts',(-10.0774692669866,-66.1498345501,69.757818081886));
#128931=CARTESIAN_POINT('Ctrl Pts',(-9.94426716677564,-65.03881684527,75.159924360853));
#128932=CARTESIAN_POINT('Ctrl Pts',(-9.74446401645964,-69.94095953137,81.84418107373));
#128933=CARTESIAN_POINT('Ctrl Pts',(-9.54466086614364,-78.18756436805,82.675374708005));
#128934=CARTESIAN_POINT('Ctrl Pts',(-9.34485771582764,-84.3279816375,77.109502645436));
#128935=CARTESIAN_POINT('Ctrl Pts',(-9.14505456551164,-84.30727308569,68.821968198106));
#128936=CARTESIAN_POINT('Ctrl Pts',(-8.94525141519564,-78.13920519194,63.285515123434));
#128937=CARTESIAN_POINT('Ctrl Pts',(-8.74544826488068,-69.89662703841,64.163123294247));
#128938=CARTESIAN_POINT('Ctrl Pts',(-8.61224616466968,-66.65138462743,68.622440986855));
#128939=CARTESIAN_POINT('Ctrl Pts',(-8.54564511456468,-66.12404568677,71.098635427588));
#128940=CARTESIAN_POINT('Ctrl Pts',(-10.1459941058106,-67.62520219141,67.700413019766));
#128941=CARTESIAN_POINT('Ctrl Pts',(-10.0793930557045,-66.1498345501,69.757818081886));
#128942=CARTESIAN_POINT('Ctrl Pts',(-9.9461909554935,-65.03881684527,75.159924360853));
#128943=CARTESIAN_POINT('Ctrl Pts',(-9.7463878051775,-69.94095953137,81.84418107373));
#128944=CARTESIAN_POINT('Ctrl Pts',(-9.5465846548615,-78.18756436805,82.675374708005));
#128945=CARTESIAN_POINT('Ctrl Pts',(-9.3467815045455,-84.3279816375,77.109502645436));
#128946=CARTESIAN_POINT('Ctrl Pts',(-9.1469783542295,-84.30727308569,68.821968198106));
#128947=CARTESIAN_POINT('Ctrl Pts',(-8.9471752039135,-78.13920519194,63.285515123434));
#128948=CARTESIAN_POINT('Ctrl Pts',(-8.74737205359857,-69.89662703841,64.163123294247));
#128949=CARTESIAN_POINT('Ctrl Pts',(-8.61416995338757,-66.65138462743,68.622440986855));
#128950=CARTESIAN_POINT('Ctrl Pts',(-8.54756890328257,-66.12404568677,71.098635427588));
#128951=CARTESIAN_POINT('',(-9.85448379345391,-67.0101053268475,68.6926900228996));
#128952=CARTESIAN_POINT('Ctrl Pts',(-13.1454639400434,-80.45858984268,79.025262748814));
#128953=CARTESIAN_POINT('Ctrl Pts',(-13.1047676696649,-81.48759917444,78.094747098225));
#128954=CARTESIAN_POINT('Ctrl Pts',(-13.023375128908,-83.05789139581,75.697173136178));
#128955=CARTESIAN_POINT('Ctrl Pts',(-12.9012863177725,-83.35252030674,71.406833513058));
#128956=CARTESIAN_POINT('Ctrl Pts',(-12.779197506637,-81.50958548889,67.521577101676));
#128957=CARTESIAN_POINT('Ctrl Pts',(-12.6571086955016,-78.00102966728,65.03524813757));
#128958=CARTESIAN_POINT('Ctrl Pts',(-12.535019884366,-73.72453794147,64.584146732116));
#128959=CARTESIAN_POINT('Ctrl Pts',(-12.4129310732305,-69.77442198226,66.283678758148));
#128960=CARTESIAN_POINT('Ctrl Pts',(-12.2908422620949,-67.16144589233,69.698967665193));
#128961=CARTESIAN_POINT('Ctrl Pts',(-12.1687534509593,-66.5542301033,73.9560942582189));
#128962=CARTESIAN_POINT('Ctrl Pts',(-12.0466646398237,-68.10815086311,77.965728779761));
#128963=CARTESIAN_POINT('Ctrl Pts',(-11.9245758286881,-71.42558498136,80.70187013362));
#128964=CARTESIAN_POINT('Ctrl Pts',(-11.8024870175525,-75.65765439615,81.464383794463));
#128965=CARTESIAN_POINT('Ctrl Pts',(-11.6803982064169,-79.72144063224,80.058154773716));
#128966=CARTESIAN_POINT('Ctrl Pts',(-11.5583093952809,-82.57708616044,76.843014459137));
#128967=CARTESIAN_POINT('Ctrl Pts',(-11.4362205841459,-83.49387722752,72.6416655369234));
#128968=CARTESIAN_POINT('Ctrl Pts',(-11.3141317730099,-82.23722174699,68.52916561233));
#128969=CARTESIAN_POINT('Ctrl Pts',(-11.1920429618739,-79.12867764146,65.557837261156));
#128970=CARTESIAN_POINT('Ctrl Pts',(-11.0699541507389,-74.96367134257,64.48799561084));
#128971=CARTESIAN_POINT('Ctrl Pts',(-10.9478653396029,-70.80796096272,65.593395929895));
#128972=CARTESIAN_POINT('Ctrl Pts',(-10.8257765284669,-67.72492593816,68.59118405853));
#128973=CARTESIAN_POINT('Ctrl Pts',(-10.7036877173319,-66.50346533712,72.714274237664));
#128974=CARTESIAN_POINT('Ctrl Pts',(-10.5815989061959,-67.45613127848,76.907634016596));
#128975=CARTESIAN_POINT('Ctrl Pts',(-10.4595100950609,-70.33915187332,80.09825008004));
#128976=CARTESIAN_POINT('Ctrl Pts',(-10.3374212839249,-74.4148085262,81.46969511541));
#128977=CARTESIAN_POINT('Ctrl Pts',(-10.2153324727889,-78.64020627051,80.671038351543));
#128978=CARTESIAN_POINT('Ctrl Pts',(-10.0932436616539,-81.93413376206,77.906643386292));
#128979=CARTESIAN_POINT('Ctrl Pts',(-9.97115485051791,-83.45372806371,73.8838737528785));
#128980=CARTESIAN_POINT('Ctrl Pts',(-9.84906603938191,-82.81014898713,69.632093987784));
#128981=CARTESIAN_POINT('Ctrl Pts',(-9.72697722824691,-80.16807974905,66.239256812192));
#128982=CARTESIAN_POINT('Ctrl Pts',(-9.60488841711091,-76.20357708221,64.573569483865));
#128983=CARTESIAN_POINT('Ctrl Pts',(-9.48279960597591,-71.93111689791,65.061124710008));
#128984=CARTESIAN_POINT('Ctrl Pts',(-9.36071079483991,-68.44386550154,67.577649690078));
#128985=CARTESIAN_POINT('Ctrl Pts',(-9.27931825408291,-67.23760922485,70.177481292106));
#128986=CARTESIAN_POINT('Ctrl Pts',(-9.23862198370491,-66.9910877936,71.542745649207));
#128987=CARTESIAN_POINT('Ctrl Pts',(-13.3760469519197,-80.72646219088,79.321488981906));
#128988=CARTESIAN_POINT('Ctrl Pts',(-13.3353506815413,-81.80596865723,78.345309630701));
#128989=CARTESIAN_POINT('Ctrl Pts',(-13.2539581407843,-83.45332068284,75.830078217611));
#128990=CARTESIAN_POINT('Ctrl Pts',(-13.1318693296489,-83.76240807855,71.329196424715));
#128991=CARTESIAN_POINT('Ctrl Pts',(-13.0097805185134,-81.82903391805,67.253276712327));
#128992=CARTESIAN_POINT('Ctrl Pts',(-12.8876917073779,-78.14830082834,64.644934774694));
#128993=CARTESIAN_POINT('Ctrl Pts',(-12.7656028962424,-73.66194649816,64.171696224628));
#128994=CARTESIAN_POINT('Ctrl Pts',(-12.6435140851068,-69.51798435008,65.954630310129));
#128995=CARTESIAN_POINT('Ctrl Pts',(-12.5214252739713,-66.77678026333,69.537519547238));
#128996=CARTESIAN_POINT('Ctrl Pts',(-12.3993364628357,-66.13976624364,74.003558428952));
#128997=CARTESIAN_POINT('Ctrl Pts',(-12.2772476517001,-67.76994340206,78.209959926145));
#128998=CARTESIAN_POINT('Ctrl Pts',(-12.1551588405645,-71.2501757691,81.080373432798));
#128999=CARTESIAN_POINT('Ctrl Pts',(-12.0330700294289,-75.68992782805,81.880306341227));
#129000=CARTESIAN_POINT('Ctrl Pts',(-11.9109812182932,-79.95313845632,80.405068678906));
#129001=CARTESIAN_POINT('Ctrl Pts',(-11.7888924071576,-82.94892063066,77.032150034994));
#129002=CARTESIAN_POINT('Ctrl Pts',(-11.666803596022,-83.91070188439,72.6246260320682));
#129003=CARTESIAN_POINT('Ctrl Pts',(-11.5447147848859,-82.59237786598,68.310311161955));
#129004=CARTESIAN_POINT('Ctrl Pts',(-11.4226259737509,-79.33128648485,65.193169198556));
#129005=CARTESIAN_POINT('Ctrl Pts',(-11.3005371626149,-74.96188856657,64.070826627081));
#129006=CARTESIAN_POINT('Ctrl Pts',(-11.1784483514789,-70.60224275103,65.23047285722));
#129007=CARTESIAN_POINT('Ctrl Pts',(-11.0563595403439,-67.36791227191,68.375373073155));
#129008=CARTESIAN_POINT('Ctrl Pts',(-10.9342707292079,-66.08651027048,72.7007978991383));
#129009=CARTESIAN_POINT('Ctrl Pts',(-10.8121819180719,-67.08592690573,77.0999407032));
#129010=CARTESIAN_POINT('Ctrl Pts',(-10.6900931069369,-70.11042753827,80.447131604038));
#129011=CARTESIAN_POINT('Ctrl Pts',(-10.5680042958009,-74.38609110676,81.885878307519));
#129012=CARTESIAN_POINT('Ctrl Pts',(-10.4459154846659,-78.8188440927,81.048028625887));
#129013=CARTESIAN_POINT('Ctrl Pts',(-10.3238266735299,-82.27441627954,78.147975002984));
#129014=CARTESIAN_POINT('Ctrl Pts',(-10.2017378623939,-83.86858245883,73.9277938074276));
#129015=CARTESIAN_POINT('Ctrl Pts',(-10.0796490512589,-83.19342067618,69.46736414145));
#129016=CARTESIAN_POINT('Ctrl Pts',(-9.95756024012291,-80.4216957374,65.908028421839));
#129017=CARTESIAN_POINT('Ctrl Pts',(-9.83547142898791,-76.26264087496,64.160599913318));
#129018=CARTESIAN_POINT('Ctrl Pts',(-9.71338261785191,-71.78051592832,64.672081202253));
#129019=CARTESIAN_POINT('Ctrl Pts',(-9.59129380671691,-68.12213274751,67.312100981366));
#129020=CARTESIAN_POINT('Ctrl Pts',(-9.50990126595991,-66.8566812005,70.039515533604));
#129021=CARTESIAN_POINT('Ctrl Pts',(-9.46920499558091,-66.59806208898,71.471778251044));
#129022=CARTESIAN_POINT('Ctrl Pts',(-13.6066299637959,-80.99433453906,79.617715215002));
#129023=CARTESIAN_POINT('Ctrl Pts',(-13.5659336934176,-82.12433814002,78.595872163185));
#129024=CARTESIAN_POINT('Ctrl Pts',(-13.4845411526607,-83.84874996986,75.962983299056));
#129025=CARTESIAN_POINT('Ctrl Pts',(-13.3624523415252,-84.17229585037,71.251559336391));
#129026=CARTESIAN_POINT('Ctrl Pts',(-13.2403635303897,-82.14848234721,66.984976322999));
#129027=CARTESIAN_POINT('Ctrl Pts',(-13.1182747192542,-78.29557198944,64.254621411829));
#129028=CARTESIAN_POINT('Ctrl Pts',(-12.9961859081187,-73.59935505488,63.759245717135));
#129029=CARTESIAN_POINT('Ctrl Pts',(-12.8740970969832,-69.26154671793,65.625581862084));
#129030=CARTESIAN_POINT('Ctrl Pts',(-12.7520082858476,-66.39211463435,69.376071429236));
#129031=CARTESIAN_POINT('Ctrl Pts',(-12.629919474712,-65.72530238397,74.051022599625));
#129032=CARTESIAN_POINT('Ctrl Pts',(-12.5078306635764,-67.43173594097,78.454191072474));
#129033=CARTESIAN_POINT('Ctrl Pts',(-12.3857418524408,-71.07476655678,81.458876731945));
#129034=CARTESIAN_POINT('Ctrl Pts',(-12.2636530413052,-75.72220125986,82.296228887996));
#129035=CARTESIAN_POINT('Ctrl Pts',(-12.1415642301696,-80.18483628034,80.751982584142));
#129036=CARTESIAN_POINT('Ctrl Pts',(-12.0194754190339,-83.32075510084,77.221285610932));
#129037=CARTESIAN_POINT('Ctrl Pts',(-11.8973866078983,-84.32752654126,72.6075865273095));
#129038=CARTESIAN_POINT('Ctrl Pts',(-11.7752977967627,-82.94753398501,68.091456711666));
#129039=CARTESIAN_POINT('Ctrl Pts',(-11.653208985627,-79.53389532833,64.828501136008));
#129040=CARTESIAN_POINT('Ctrl Pts',(-11.5311201744909,-74.96010579067,63.653657643322));
#129041=CARTESIAN_POINT('Ctrl Pts',(-11.4090313633559,-70.39652453943,64.867549784492));
#129042=CARTESIAN_POINT('Ctrl Pts',(-11.2869425522199,-67.01089860571,68.159562087686));
#129043=CARTESIAN_POINT('Ctrl Pts',(-11.1648537410839,-65.66955520384,72.6873215605024));
#129044=CARTESIAN_POINT('Ctrl Pts',(-11.0427649299489,-66.71572253294,77.292247389707));
#129045=CARTESIAN_POINT('Ctrl Pts',(-10.9206761188129,-69.88170320312,80.796013127978));
#129046=CARTESIAN_POINT('Ctrl Pts',(-10.7985873076779,-74.35737368722,82.302061499622));
#129047=CARTESIAN_POINT('Ctrl Pts',(-10.6764984965419,-78.99748191481,81.425018900273));
#129048=CARTESIAN_POINT('Ctrl Pts',(-10.5544096854059,-82.61469879698,78.389306619751));
#129049=CARTESIAN_POINT('Ctrl Pts',(-10.4323208742709,-84.28343685395,73.9717138620569));
#129050=CARTESIAN_POINT('Ctrl Pts',(-10.3102320631349,-83.57669236526,69.30263429518));
#129051=CARTESIAN_POINT('Ctrl Pts',(-10.1881432519999,-80.67531172579,65.57680003152));
#129052=CARTESIAN_POINT('Ctrl Pts',(-10.0660544408639,-76.32170466775,63.747630342775));
#129053=CARTESIAN_POINT('Ctrl Pts',(-9.94396562972891,-71.62991495875,64.283037694485));
#129054=CARTESIAN_POINT('Ctrl Pts',(-9.82187681859291,-67.80039999349,67.046552272646));
#129055=CARTESIAN_POINT('Ctrl Pts',(-9.74048427783591,-66.47575317615,69.901549775107));
#129056=CARTESIAN_POINT('Ctrl Pts',(-9.69978800745791,-66.20503638435,71.400810852893));
#129057=CARTESIAN_POINT('Ctrl Pts',(-13.8372129756729,-81.26220688726,79.913941448094));
#129058=CARTESIAN_POINT('Ctrl Pts',(-13.7965167052939,-82.44270762281,78.846434695661));
#129059=CARTESIAN_POINT('Ctrl Pts',(-13.7151241645369,-84.24417925689,76.095888380488));
#129060=CARTESIAN_POINT('Ctrl Pts',(-13.5930353534019,-84.58218362219,71.173922248048));
#129061=CARTESIAN_POINT('Ctrl Pts',(-13.4709465422661,-82.46793077636,66.716675933649));
#129062=CARTESIAN_POINT('Ctrl Pts',(-13.3488577311306,-78.4428431505,63.864308048952));
#129063=CARTESIAN_POINT('Ctrl Pts',(-13.2267689199951,-73.53676361156,63.346795209648));
#129064=CARTESIAN_POINT('Ctrl Pts',(-13.1046801088595,-69.00510908574,65.296533414067));
#129065=CARTESIAN_POINT('Ctrl Pts',(-12.982591297724,-66.00744900535,69.214623311284));
#129066=CARTESIAN_POINT('Ctrl Pts',(-12.8605024865884,-65.31083852431,74.098486770361));
#129067=CARTESIAN_POINT('Ctrl Pts',(-12.7384136754528,-67.09352847992,78.698422218861));
#129068=CARTESIAN_POINT('Ctrl Pts',(-12.6163248643172,-70.89935734453,81.837380031125));
#129069=CARTESIAN_POINT('Ctrl Pts',(-12.4942360531816,-75.75447469176,82.71215143476));
#129070=CARTESIAN_POINT('Ctrl Pts',(-12.3721472420459,-80.41653410443,81.098896489329));
#129071=CARTESIAN_POINT('Ctrl Pts',(-12.2500584309103,-83.69258957107,77.410421186785));
#129072=CARTESIAN_POINT('Ctrl Pts',(-12.1279696197746,-84.74435119813,72.5905470224496));
#129073=CARTESIAN_POINT('Ctrl Pts',(-12.005880808639,-83.302690104,67.872602261286));
#129074=CARTESIAN_POINT('Ctrl Pts',(-11.8837919975033,-79.73650417172,64.463833073406));
#129075=CARTESIAN_POINT('Ctrl Pts',(-11.7617031863677,-74.95832301467,63.236488659563));
#129076=CARTESIAN_POINT('Ctrl Pts',(-11.639614375232,-70.19080632774,64.50462671182));
#129077=CARTESIAN_POINT('Ctrl Pts',(-11.5175255640959,-66.65388493945,67.943751102315));
#129078=CARTESIAN_POINT('Ctrl Pts',(-11.3954367529609,-65.25260013719,72.673845221982));
#129079=CARTESIAN_POINT('Ctrl Pts',(-11.2733479418249,-66.34551816019,77.484554076315));
#129080=CARTESIAN_POINT('Ctrl Pts',(-11.1512591306899,-69.65297886807,81.144894651979));
#129081=CARTESIAN_POINT('Ctrl Pts',(-11.0291703195539,-74.32865626779,82.718244691732));
#129082=CARTESIAN_POINT('Ctrl Pts',(-10.9070815084179,-79.176119737,81.802009174614));
#129083=CARTESIAN_POINT('Ctrl Pts',(-10.7849926972829,-82.95498131447,78.63063823644));
#129084=CARTESIAN_POINT('Ctrl Pts',(-10.6629038861469,-84.69829124907,74.015633916602));
#129085=CARTESIAN_POINT('Ctrl Pts',(-10.5408150750119,-83.95996405431,69.137904448843));
#129086=CARTESIAN_POINT('Ctrl Pts',(-10.4187262638759,-80.92892771414,65.245571641166));
#129087=CARTESIAN_POINT('Ctrl Pts',(-10.2966374527399,-76.3807684605,63.334660772228));
#129088=CARTESIAN_POINT('Ctrl Pts',(-10.1745486416049,-71.47931398915,63.89399418673));
#129089=CARTESIAN_POINT('Ctrl Pts',(-10.0524598304689,-67.47866723947,66.781003563935));
#129090=CARTESIAN_POINT('Ctrl Pts',(-9.97106728971191,-66.0948251518,69.763584016604));
#129091=CARTESIAN_POINT('Ctrl Pts',(-9.93037101933391,-65.81201067972,71.32984345473));
#129092=CARTESIAN_POINT('',(-13.5671411686305,-83.5589497503404,76.0033450387178));
#129093=CARTESIAN_POINT('Ctrl Pts',(-13.5667458539302,-83.5583092465054,
76.0031044421984));
#129094=CARTESIAN_POINT('Ctrl Pts',(-13.5640800181624,-83.5922872145127,
75.9068207927514));
#129095=CARTESIAN_POINT('Ctrl Pts',(-13.5614447593399,-83.6246546966739,
75.8099696689204));
#129096=CARTESIAN_POINT('Ctrl Pts',(-13.5530672454983,-83.7233362399437,
75.4973489808209));
#129097=CARTESIAN_POINT('Ctrl Pts',(-13.5474177830113,-83.7833032435454,
75.2795745744807));
#129098=CARTESIAN_POINT('Ctrl Pts',(-13.5350766693028,-83.8962038299702,
74.8001260870673));
#129099=CARTESIAN_POINT('Ctrl Pts',(-13.5283798935997,-83.9458836624366,
74.5376098343622));
#129100=CARTESIAN_POINT('Ctrl Pts',(-13.5177668235028,-84.0038523401724,
74.1318657443427));
#129101=CARTESIAN_POINT('Ctrl Pts',(-13.5140091710748,-84.0206428553733,
73.9899873829069));
#129102=CARTESIAN_POINT('Ctrl Pts',(-13.5002165626111,-84.069262514367,
73.4739678360416));
#129103=CARTESIAN_POINT('Ctrl Pts',(-13.4899251488299,-84.0810377628333,
73.0979524172502));
#129104=CARTESIAN_POINT('Ctrl Pts',(-13.4703039519722,-84.0594037634423,
72.3811619891736));
#129105=CARTESIAN_POINT('Ctrl Pts',(-13.4609717905523,-84.0299673204892,
72.0402094984997));
#129106=CARTESIAN_POINT('Ctrl Pts',(-13.448222877598,-83.9620661056739,
71.5649788215202));
#129107=CARTESIAN_POINT('Ctrl Pts',(-13.4445894694965,-83.9393892802237,
71.4284087441626));
#129108=CARTESIAN_POINT('Ctrl Pts',(-13.4339896337949,-83.8630274060158,
71.0253456742784));
#129109=CARTESIAN_POINT('Ctrl Pts',(-13.4271842518906,-83.8005219868351,
70.7605125131827));
#129110=CARTESIAN_POINT('Ctrl Pts',(-13.4140566946332,-83.6572722714153,
70.2563978903051));
#129111=CARTESIAN_POINT('Ctrl Pts',(-13.4077344473922,-83.578171160243,
70.0166636317799));
#129112=CARTESIAN_POINT('Ctrl Pts',(-13.3975075655731,-83.4380202727791,
69.6457919580006));
#129113=CARTESIAN_POINT('Ctrl Pts',(-13.3937272172911,-83.3837478006566,
69.5121191198762));
#129114=CARTESIAN_POINT('Ctrl Pts',(-13.3812477757693,-83.1962513613288,
69.0804671876166));
#129115=CARTESIAN_POINT('Ctrl Pts',(-13.3723658901788,-83.0498920388042,
68.7882126092547));
#129116=CARTESIAN_POINT('Ctrl Pts',(-13.3558977290774,-82.7512917519671,
68.2640874293851));
#129117=CARTESIAN_POINT('Ctrl Pts',(-13.3483197841579,-82.6033049797775,
68.0297661795723));
#129118=CARTESIAN_POINT('Ctrl Pts',(-13.3356439017166,-82.3348534023005,
67.6444514316513));
#129119=CARTESIAN_POINT('Ctrl Pts',(-13.3304913444046,-82.2196693095211,
67.4897495021949));
#129120=CARTESIAN_POINT('Ctrl Pts',(-13.3216308651203,-82.0096748178785,
67.2255380783767));
#129121=CARTESIAN_POINT('Ctrl Pts',(-13.3178882932308,-81.916940108937,
67.1143726804648));
#129122=CARTESIAN_POINT('Ctrl Pts',(-13.3064348773527,-81.6210698998257,
66.7763831217991));
#129123=CARTESIAN_POINT('Ctrl Pts',(-13.2988745494577,-81.4090562151365,
66.5573305579049));
#129124=CARTESIAN_POINT('Ctrl Pts',(-13.287872999267,-81.0900536116174,
66.2596318506067));
#129125=CARTESIAN_POINT('Ctrl Pts',(-13.2845263606801,-80.9916661173901,
66.171791176635));
#129126=CARTESIAN_POINT('Ctrl Pts',(-13.2773780454483,-80.7804502592599,
65.9915038295038));
#129127=CARTESIAN_POINT('Ctrl Pts',(-13.2735652493214,-80.667249665329,
65.8996055717503));
#129128=CARTESIAN_POINT('Ctrl Pts',(-13.2569637833204,-80.1708073118262,
65.5162542685411));
#129129=CARTESIAN_POINT('Ctrl Pts',(-13.2437214187867,-79.7660220760457,
65.2526560754908));
#129130=CARTESIAN_POINT('Ctrl Pts',(-13.2249963764698,-79.1622973306626,
64.9239326290828));
#129131=CARTESIAN_POINT('Ctrl Pts',(-13.2194107577164,-78.9781280276051,
64.8315536077034));
#129132=CARTESIAN_POINT('Ctrl Pts',(-13.2094511159405,-78.6401712057606,
64.6760356169752));
#129133=CARTESIAN_POINT('Ctrl Pts',(-13.2050514003971,-78.4873851110901,
64.6106925387327));
#129134=CARTESIAN_POINT('Ctrl Pts',(-13.1960707382152,-78.1668763190988,
64.4838235016176));
#129135=CARTESIAN_POINT('Ctrl Pts',(-13.1915142562595,-77.9988949418862,
64.4229538109884));
#129136=CARTESIAN_POINT('Ctrl Pts',(-13.180415362693,-77.5813063138297,
64.2854135325013));
#129137=CARTESIAN_POINT('Ctrl Pts',(-13.1739176940635,-77.3298340995017,
64.2144287922523));
#129138=CARTESIAN_POINT('Ctrl Pts',(-13.163063039009,-76.9126045445894,
64.1161350615823));
#129139=CARTESIAN_POINT('Ctrl Pts',(-13.158772440825,-76.7486833212321,
64.0823561069267));
#129140=CARTESIAN_POINT('Ctrl Pts',(-13.1496316182324,-76.4040563125874,
64.0214430337194));
#129141=CARTESIAN_POINT('Ctrl Pts',(-13.1447908325575,-76.2236333412628,
63.9952203562065));
#129142=CARTESIAN_POINT('Ctrl Pts',(-13.1283856998445,-75.6163755370945,
63.9256352625226));
#129143=CARTESIAN_POINT('Ctrl Pts',(-13.1165911008828,-75.1866770975472,
63.9071418211856));
#129144=CARTESIAN_POINT('Ctrl Pts',(-13.0998492934382,-74.5700735368246,
63.9237963404925));
#129145=CARTESIAN_POINT('Ctrl Pts',(-13.0947798985282,-74.3824540529019,
63.9346345962008));
#129146=CARTESIAN_POINT('Ctrl Pts',(-13.0855265611452,-74.0365003082374,
63.9653006109643));
#129147=CARTESIAN_POINT('Ctrl Pts',(-13.0813243282303,-73.8780146894078,
63.9835242403866));
#129148=CARTESIAN_POINT('Ctrl Pts',(-13.0709193471626,-73.4806638935296,
64.0397825970281));
#129149=CARTESIAN_POINT('Ctrl Pts',(-13.0648252092706,-73.2425600506697,
64.0831879404041));
#129150=CARTESIAN_POINT('Ctrl Pts',(-13.0520354529743,-72.7455612383279,
64.1945445275424));
#129151=CARTESIAN_POINT('Ctrl Pts',(-13.0453376145367,-72.4870360765741,
64.264634065654));
#129152=CARTESIAN_POINT('Ctrl Pts',(-13.034385538917,-72.0824983766059,
64.3942244165957));
#129153=CARTESIAN_POINT('Ctrl Pts',(-13.030271002386,-71.9342234575551,
64.446095201498));
#129154=CARTESIAN_POINT('Ctrl Pts',(-13.0136565124453,-71.3481710882388,
64.6685101182148));
#129155=CARTESIAN_POINT('Ctrl Pts',(-13.0007741957329,-70.9220142912128,
64.8696380442875));
#129156=CARTESIAN_POINT('Ctrl Pts',(-12.982152422141,-70.3268398396603,
65.2085630953448));
#129157=CARTESIAN_POINT('Ctrl Pts',(-12.976326844472,-70.1436463124613,
65.3215949165373));
#129158=CARTESIAN_POINT('Ctrl Pts',(-12.9659322363181,-69.8200770099199,
65.5373007093749));
#129159=CARTESIAN_POINT('Ctrl Pts',(-12.9613367010879,-69.6782317161318,
65.6377940024871));
#129160=CARTESIAN_POINT('Ctrl Pts',(-12.9474668712654,-69.2521331205604,
65.958296317252));
#129161=CARTESIAN_POINT('Ctrl Pts',(-12.9385186395591,-68.9776493854189,
66.1912805204721));
#129162=CARTESIAN_POINT('Ctrl Pts',(-12.9259108354926,-68.6162479933985,
66.5373953347773));
#129163=CARTESIAN_POINT('Ctrl Pts',(-12.9223398605986,-68.5167177393356,
66.6373160508213));
#129164=CARTESIAN_POINT('Ctrl Pts',(-12.9146492875739,-68.3105958471069,
66.8543448854849));
#129165=CARTESIAN_POINT('Ctrl Pts',(-12.9105158741154,-68.2046724252965,
66.9720243878612));
#129166=CARTESIAN_POINT('Ctrl Pts',(-12.8939773679671,-67.7983988832239,
67.4480995965967));
#129167=CARTESIAN_POINT('Ctrl Pts',(-12.8811892322323,-67.5226375585457,
67.8274973976122));
#129168=CARTESIAN_POINT('Ctrl Pts',(-12.8622215343773,-67.1566058114058,
68.4216312289478));
#129169=CARTESIAN_POINT('Ctrl Pts',(-12.8559830998545,-67.0432252457875,
68.6222022127429));
#129170=CARTESIAN_POINT('Ctrl Pts',(-12.8449495602273,-66.8538563952299,
68.9887312750473));
#129171=CARTESIAN_POINT('Ctrl Pts',(-12.8401238962256,-66.7749905455055,
69.1532203824882));
#129172=CARTESIAN_POINT('Ctrl Pts',(-12.8260882362863,-66.5565002368576,
69.6462360142252));
#129173=CARTESIAN_POINT('Ctrl Pts',(-12.8171900872545,-66.4310078991802,
69.9810141155976));
#129174=CARTESIAN_POINT('Ctrl Pts',(-12.8046090173476,-66.2840149886737,
70.4578371198973));
#129175=CARTESIAN_POINT('Ctrl Pts',(-12.8010077046728,-66.2453827957356,
70.5946070810551));
#129176=CARTESIAN_POINT('Ctrl Pts',(-12.7931083760621,-66.1690244194849,
70.8920803051291));
#129177=CARTESIAN_POINT('Ctrl Pts',(-12.7887950627577,-66.1324577536049,
71.0530276441246));
#129178=CARTESIAN_POINT('Ctrl Pts',(-12.7726402520091,-66.0135761571878,
71.6521427829917));
#129179=CARTESIAN_POINT('Ctrl Pts',(-12.7604785726686,-65.9593325993155,
72.0958671031451));
#129180=CARTESIAN_POINT('Ctrl Pts',(-12.7417813500953,-65.9257357403144,
72.7834136930754));
#129181=CARTESIAN_POINT('Ctrl Pts',(-12.7352087298558,-65.9235134175458,
73.0261761341576));
#129182=CARTESIAN_POINT('Ctrl Pts',(-12.7236478526681,-65.9366908056587,
73.4582749982496));
#129183=CARTESIAN_POINT('Ctrl Pts',(-12.7186260357509,-65.948357594045,
73.6477433913853));
#129184=CARTESIAN_POINT('Ctrl Pts',(-12.7049061682116,-65.9971259901677,
74.172634625439));
#129185=CARTESIAN_POINT('Ctrl Pts',(-12.6964671708652,-66.0469555065457,
74.5068642205268));
#129186=CARTESIAN_POINT('Ctrl Pts',(-12.6842565636745,-66.1452288670634,
74.9811030723674));
#129187=CARTESIAN_POINT('Ctrl Pts',(-12.6805358559911,-66.1785740163575,
75.1242414019398));
#129188=CARTESIAN_POINT('Ctrl Pts',(-12.6723915520485,-66.2581222352044,
75.4310215752946));
#129189=CARTESIAN_POINT('Ctrl Pts',(-12.6679518101771,-66.3055053509249,
75.5943144175234));
#129190=CARTESIAN_POINT('Ctrl Pts',(-12.6516212436858,-66.4944563271868,
76.1826445936466));
#129191=CARTESIAN_POINT('Ctrl Pts',(-12.6394187259343,-66.6633011130804,
76.5989086290332));
#129192=CARTESIAN_POINT('Ctrl Pts',(-12.6204973832283,-66.9719492483717,
77.2242291686741));
#129193=CARTESIAN_POINT('Ctrl Pts',(-12.6137457233882,-67.0914616914067,
77.4433682809365));
#129194=CARTESIAN_POINT('Ctrl Pts',(-12.6018724518322,-67.3199298894286,
77.8244732523635));
#129195=CARTESIAN_POINT('Ctrl Pts',(-12.5967164002634,-67.4255026661867,
77.9884898912608));
#129196=CARTESIAN_POINT('Ctrl Pts',(-12.5853460546946,-67.673796987118,
78.3483727903719));
#129197=CARTESIAN_POINT('Ctrl Pts',(-12.5792117016916,-67.8193138805894,
78.5423053192264));
#129198=CARTESIAN_POINT('Ctrl Pts',(-12.5683096863466,-68.0927037691992,
78.8776387789366));
#129199=CARTESIAN_POINT('Ctrl Pts',(-12.5635236220845,-68.217674991041,
79.0213866934708));
#129200=CARTESIAN_POINT('Ctrl Pts',(-12.5542317363497,-68.4651435564829,
79.2882454482999));
#129201=CARTESIAN_POINT('Ctrl Pts',(-12.5497357559432,-68.5866986269073,
79.4118384285661));
#129202=CARTESIAN_POINT('Ctrl Pts',(-12.5381251345081,-68.9054205928239,
79.7176821663174));
#129203=CARTESIAN_POINT('Ctrl Pts',(-12.5309312787889,-69.1075075161986,
79.8949000650061));
#129204=CARTESIAN_POINT('Ctrl Pts',(-12.5133411163695,-69.6159873837846,
80.302521491647));
#129205=CARTESIAN_POINT('Ctrl Pts',(-12.5028886133086,-69.9301047940802,
80.5233495686275));
#129206=CARTESIAN_POINT('Ctrl Pts',(-12.4860285719784,-70.464264540149,
80.8509991125645));
#129207=CARTESIAN_POINT('Ctrl Pts',(-12.4795352140262,-70.6768760668288,
80.970048415271));
#129208=CARTESIAN_POINT('Ctrl Pts',(-12.4684239451364,-71.0552045178678,
81.1624621476388));
#129209=CARTESIAN_POINT('Ctrl Pts',(-12.4637616215854,-71.2189555267709,
81.2397121151644));
#129210=CARTESIAN_POINT('Ctrl Pts',(-12.4512555091035,-71.6702335519829,
81.4363149037997));
#129211=CARTESIAN_POINT('Ctrl Pts',(-12.4434969476487,-71.9619996094954,
81.5459414268526));
#129212=CARTESIAN_POINT('Ctrl Pts',(-12.4308368744386,-72.432246629013,
81.6949422127961));
#129213=CARTESIAN_POINT('Ctrl Pts',(-12.4260886116885,-72.6074084118894,
81.7445741053388));
#129214=CARTESIAN_POINT('Ctrl Pts',(-12.4106932123179,-73.1730791994157,
81.8864772631894));
#129215=CARTESIAN_POINT('Ctrl Pts',(-12.3998302925292,-73.5687624449072,
81.9580731462943));
#129216=CARTESIAN_POINT('Ctrl Pts',(-12.3783768815432,-74.35582030368,82.0477162622559));
#129217=CARTESIAN_POINT('Ctrl Pts',(-12.3677869869934,-74.7471274668323,
82.0670978702825));
#129218=CARTESIAN_POINT('Ctrl Pts',(-12.3526344492061,-75.3200793364769,
82.0588030438593));
#129219=CARTESIAN_POINT('Ctrl Pts',(-12.347873911003,-75.5020586445725,
82.0507357538656));
#129220=CARTESIAN_POINT('Ctrl Pts',(-12.3356308365092,-75.9767837340445,
82.0153873268272));
#129221=CARTESIAN_POINT('Ctrl Pts',(-12.328282306456,-76.2688704651353,
81.9793459652047));
#129222=CARTESIAN_POINT('Ctrl Pts',(-12.3157260852563,-76.7563694762715,
81.8946079983548));
#129223=CARTESIAN_POINT('Ctrl Pts',(-12.3105740210083,-76.9524881347204,
81.8536303360942));
#129224=CARTESIAN_POINT('Ctrl Pts',(-12.2983032564264,-77.4081668153727,
81.7423142094984));
#129225=CARTESIAN_POINT('Ctrl Pts',(-12.2911459512972,-77.6661252285936,
81.6668766432329));
#129226=CARTESIAN_POINT('Ctrl Pts',(-12.2726493307792,-78.3173925485451,
81.4447294518154));
#129227=CARTESIAN_POINT('Ctrl Pts',(-12.2612227927062,-78.7052121629505,
81.2817875539456));
#129228=CARTESIAN_POINT('Ctrl Pts',(-12.2429374821052,-79.3132607670729,
80.9758038124274));
#129229=CARTESIAN_POINT('Ctrl Pts',(-12.2359833432898,-79.5414862948691,
80.8484830999955));
#129230=CARTESIAN_POINT('Ctrl Pts',(-12.2195299249525,-80.0775160531477,
80.5185476562888));
#129231=CARTESIAN_POINT('Ctrl Pts',(-12.2102794690912,-80.3794929708895,
80.3064921890982));
#129232=CARTESIAN_POINT('Ctrl Pts',(-12.1954914979162,-80.8350893803178,
79.9426080988649));
#129233=CARTESIAN_POINT('Ctrl Pts',(-12.1899920400428,-80.9974964776671,
79.802975437941));
#129234=CARTESIAN_POINT('Ctrl Pts',(-12.1770600988137,-81.3606739236908,
79.4672802425608));
#129235=CARTESIAN_POINT('Ctrl Pts',(-12.1695974691883,-81.5574135001567,
79.2675554631078));
#129236=CARTESIAN_POINT('Ctrl Pts',(-12.1507377520941,-82.0265282874472,
78.7452319839698));
#129237=CARTESIAN_POINT('Ctrl Pts',(-12.1392631758226,-82.2867251066204,
78.4116296283477));
#129238=CARTESIAN_POINT('Ctrl Pts',(-12.1208039387541,-82.6715879988969,
77.8412003225792));
#129239=CARTESIAN_POINT('Ctrl Pts',(-12.113725939776,-82.8108352065244,
77.6141165479128));
#129240=CARTESIAN_POINT('Ctrl Pts',(-12.0989816577469,-83.0847324128818,
77.1201990817444));
#129241=CARTESIAN_POINT('Ctrl Pts',(-12.0914137425593,-83.2167364123384,
76.8519027478229));
#129242=CARTESIAN_POINT('Ctrl Pts',(-12.0793375090851,-83.4057016154436,
76.4139386474057));
#129243=CARTESIAN_POINT('Ctrl Pts',(-12.0748081726496,-83.4714716736889,
76.2480793804726));
#129244=CARTESIAN_POINT('Ctrl Pts',(-12.0644662388748,-83.607794733024,
75.8714583153122));
#129245=CARTESIAN_POINT('Ctrl Pts',(-12.0586414508195,-83.6754985219537,
75.6600669295798));
#129246=CARTESIAN_POINT('Ctrl Pts',(-12.0390058468372,-83.8751177082579,
74.9476081985485));
#129247=CARTESIAN_POINT('Ctrl Pts',(-12.0249158600219,-83.9720370010646,
74.4366951858765));
#129248=CARTESIAN_POINT('Ctrl Pts',(-12.0026358185394,-84.0572776247063,
73.6122150928465));
#129249=CARTESIAN_POINT('Ctrl Pts',(-11.9943402672332,-84.0735397666877,
73.3014068899227));
#129250=CARTESIAN_POINT('Ctrl Pts',(-11.9773923867064,-84.0743154600487,
72.6534647140689));
#129251=CARTESIAN_POINT('Ctrl Pts',(-11.9688614612502,-84.0560248499278,
72.3163295312918));
#129252=CARTESIAN_POINT('Ctrl Pts',(-11.9541753138052,-83.9921224259184,
71.741263674071));
#129253=CARTESIAN_POINT('Ctrl Pts',(-11.9479953932471,-83.9558164733411,
71.503227393253));
#129254=CARTESIAN_POINT('Ctrl Pts',(-11.9254148566645,-83.7913493443104,
70.6560033933371));
#129255=CARTESIAN_POINT('Ctrl Pts',(-11.9085159411425,-83.6093857480237,
70.0578490970235));
#129256=CARTESIAN_POINT('Ctrl Pts',(-11.8826144802468,-83.2371879173642,
69.1690316337926));
#129257=CARTESIAN_POINT('Ctrl Pts',(-11.8734848276452,-83.0875724163114,
68.8611572423334));
#129258=CARTESIAN_POINT('Ctrl Pts',(-11.8566199967557,-82.7736413442767,
68.2979857932564));
#129259=CARTESIAN_POINT('Ctrl Pts',(-11.8489074740658,-82.6129107786165,
68.0406797197332));
#129260=CARTESIAN_POINT('Ctrl Pts',(-11.8361106588257,-82.324560748579,
67.6272750175843));
#129261=CARTESIAN_POINT('Ctrl Pts',(-11.8309916451167,-82.2042288866748,
67.4665816910673));
#129262=CARTESIAN_POINT('Ctrl Pts',(-11.818678293496,-81.9070784219599,
67.0966178448928));
#129263=CARTESIAN_POINT('Ctrl Pts',(-11.8114601160653,-81.7261893091633,
66.8914253334011));
#129264=CARTESIAN_POINT('Ctrl Pts',(-11.7908919240504,-81.190462082797,
66.3362918257294));
#129265=CARTESIAN_POINT('Ctrl Pts',(-11.777383867518,-80.8149659368627,
66.0061964107906));
#129266=CARTESIAN_POINT('Ctrl Pts',(-11.7577317786491,-80.225805379811,
65.567651078504));
#129267=CARTESIAN_POINT('Ctrl Pts',(-11.751449727912,-80.0308352533544,
65.4339001907069));
#129268=CARTESIAN_POINT('Ctrl Pts',(-11.739122124479,-79.6335188690206,
65.1834506279975));
#129269=CARTESIAN_POINT('Ctrl Pts',(-11.7330872672043,-79.4312820732563,
65.0665614617833));
#129270=CARTESIAN_POINT('Ctrl Pts',(-11.7218695882869,-79.0420503425554,
64.8613229085897));
#129271=CARTESIAN_POINT('Ctrl Pts',(-11.7166449615531,-78.8559849360608,
64.7712442010359));
#129272=CARTESIAN_POINT('Ctrl Pts',(-11.7051066279327,-78.4447421435435,
64.5895791838651));
#129273=CARTESIAN_POINT('Ctrl Pts',(-11.6987634650751,-78.2184774724938,
64.5005323416728));
#129274=CARTESIAN_POINT('Ctrl Pts',(-11.684810169018,-77.71919504776,64.3269414567394));
#129275=CARTESIAN_POINT('Ctrl Pts',(-11.6771735870387,-77.4449562289354,
64.24593787506));
#129276=CARTESIAN_POINT('Ctrl Pts',(-11.6529074994395,-76.5667248405637,
64.0306387496498));
#129277=CARTESIAN_POINT('Ctrl Pts',(-11.6361711939247,-75.9507792794544,
63.9442463551502));
#129278=CARTESIAN_POINT('Ctrl Pts',(-11.6138739515497,-75.0975870679637,
63.912031360932));
#129279=CARTESIAN_POINT('Ctrl Pts',(-11.6078398531792,-74.8622347970138,
63.9122696229956));
#129280=CARTESIAN_POINT('Ctrl Pts',(-11.5935419814758,-74.3013077601243,
63.9348828004118));
#129281=CARTESIAN_POINT('Ctrl Pts',(-11.5852325020868,-73.9777636940373,
63.9657446322328));
#129282=CARTESIAN_POINT('Ctrl Pts',(-11.5646853634814,-73.2027886852206,
64.0825572666288));
#129283=CARTESIAN_POINT('Ctrl Pts',(-11.5524082523738,-72.7552675906697,
64.1853590880314));
#129284=CARTESIAN_POINT('Ctrl Pts',(-11.5268837316571,-71.8468711198061,
64.4669025930135));
#129285=CARTESIAN_POINT('Ctrl Pts',(-11.5136349918919,-71.3874765934729,
64.650941098511));
#129286=CARTESIAN_POINT('Ctrl Pts',(-11.4937069948878,-70.7067134752823,
64.989997602512));
#129287=CARTESIAN_POINT('Ctrl Pts',(-11.4868272513075,-70.4726686597408,
65.1197169811987));
#129288=CARTESIAN_POINT('Ctrl Pts',(-11.4716339850267,-69.9651612665699,
65.4314252057549));
#129289=CARTESIAN_POINT('Ctrl Pts',(-11.4632440124045,-69.6963165277426,
65.617753987906));
#129290=CARTESIAN_POINT('Ctrl Pts',(-11.4470462594358,-69.2089929719968,
65.9965466507828));
#129291=CARTESIAN_POINT('Ctrl Pts',(-11.439347003723,-68.988918485167,66.1853004906013));
#129292=CARTESIAN_POINT('Ctrl Pts',(-11.4120393622787,-68.245668214213,
66.8867172062944));
#129293=CARTESIAN_POINT('Ctrl Pts',(-11.3922182362063,-67.7732597186835,
67.4536250804195));
#129294=CARTESIAN_POINT('Ctrl Pts',(-11.366936788712,-67.2452516347224,
68.2698493731437));
#129295=CARTESIAN_POINT('Ctrl Pts',(-11.3608163913894,-67.1230253326142,
68.4762992188587));
#129296=CARTESIAN_POINT('Ctrl Pts',(-11.3475668900671,-66.8772108415422,
68.932436411952));
#129297=CARTESIAN_POINT('Ctrl Pts',(-11.3403831528437,-66.7570892772954,
69.1829057883462));
#129298=CARTESIAN_POINT('Ctrl Pts',(-11.3248512505511,-66.5261303460856,
69.7276262003982));
#129299=CARTESIAN_POINT('Ctrl Pts',(-11.3164971605737,-66.4186286059857,
70.0232446326753));
#129300=CARTESIAN_POINT('Ctrl Pts',(-11.2896150174832,-66.1237919521111,
70.9855319451296));
#129301=CARTESIAN_POINT('Ctrl Pts',(-11.2709446351782,-65.9960640135589,
71.6707490856593));
#129302=CARTESIAN_POINT('Ctrl Pts',(-11.2460031258948,-65.9288496133152,
72.6251134699327));
#129303=CARTESIAN_POINT('Ctrl Pts',(-11.239241899148,-65.9218086926354,
72.8896632608712));
#129304=CARTESIAN_POINT('Ctrl Pts',(-11.2248477107533,-65.9318359002663,
73.4511502989318));
#129305=CARTESIAN_POINT('Ctrl Pts',(-11.2171422305074,-65.9520534110402,
73.7471976633819));
#129306=CARTESIAN_POINT('Ctrl Pts',(-11.1998417502573,-66.0289896609921,
74.4001777604379));
#129307=CARTESIAN_POINT('Ctrl Pts',(-11.1902105720864,-66.0928032406218,
74.75650596556));
#129308=CARTESIAN_POINT('Ctrl Pts',(-11.1637323086314,-66.3248103640701,
75.7200972951544));
#129309=CARTESIAN_POINT('Ctrl Pts',(-11.1468388232568,-66.5353946698986,
76.3173862305834));
#129310=CARTESIAN_POINT('Ctrl Pts',(-11.1230378117483,-66.9267660286225,
77.1425850466735));
#129311=CARTESIAN_POINT('Ctrl Pts',(-11.1158001611499,-67.0602709151533,
77.393018191316));
#129312=CARTESIAN_POINT('Ctrl Pts',(-11.0991110754866,-67.3922405884766,
77.9498465268579));
#129313=CARTESIAN_POINT('Ctrl Pts',(-11.0895530133271,-67.5982301647372,
78.2514307931786));
#129314=CARTESIAN_POINT('Ctrl Pts',(-11.0665262427273,-68.1312114054166,
78.939176623819));
#129315=CARTESIAN_POINT('Ctrl Pts',(-11.0529699195005,-68.4743874713834,
79.3130933754959));
#129316=CARTESIAN_POINT('Ctrl Pts',(-11.0282535705372,-69.1560840092167,
79.9427746266769));
#129317=CARTESIAN_POINT('Ctrl Pts',(-11.0170659596609,-69.4861319311373,
80.2079374301951));
#129318=CARTESIAN_POINT('Ctrl Pts',(-10.9983567631792,-70.07719144732,80.6182380424736));
#129319=CARTESIAN_POINT('Ctrl Pts',(-10.9907753226796,-70.3298606857768,
80.7757836916518));
#129320=CARTESIAN_POINT('Ctrl Pts',(-10.9694617859358,-71.0487938222381,
81.1751307786503));
#129321=CARTESIAN_POINT('Ctrl Pts',(-10.9555724402751,-71.5294163569786,
81.3892160763062));
#129322=CARTESIAN_POINT('Ctrl Pts',(-10.9218765541441,-72.7253853419579,
81.8034386875353));
#129323=CARTESIAN_POINT('Ctrl Pts',(-10.9020080574071,-73.4557989655504,
81.961124441332));
#129324=CARTESIAN_POINT('Ctrl Pts',(-10.8750202645403,-74.4901964527539,
82.0543517725009));
#129325=CARTESIAN_POINT('Ctrl Pts',(-10.8674301257071,-74.7871980771689,
82.0663737775191));
#129326=CARTESIAN_POINT('Ctrl Pts',(-10.843232576932,-75.7176036781963,
82.0571381219942));
#129327=CARTESIAN_POINT('Ctrl Pts',(-10.8264023611081,-76.3492646983437,
81.983744053942));
#129328=CARTESIAN_POINT('Ctrl Pts',(-10.7939437530567,-77.5398607522838,
81.719188310539));
#129329=CARTESIAN_POINT('Ctrl Pts',(-10.7783170880428,-78.1010200303309,
81.5367601632063));
#129330=CARTESIAN_POINT('Ctrl Pts',(-10.7542234072266,-78.9481683680525,
81.1669141646729));
#129331=CARTESIAN_POINT('Ctrl Pts',(-10.7455985843692,-79.2490240312718,
81.0149469874758));
#129332=CARTESIAN_POINT('Ctrl Pts',(-10.7252961957682,-79.9229130642142,
80.6247931408589));
#129333=CARTESIAN_POINT('Ctrl Pts',(-10.7136535989653,-80.2878531273247,
80.3759504681903));
#129334=CARTESIAN_POINT('Ctrl Pts',(-10.6866596950859,-81.0849277124096,
79.7438003105246));
#129335=CARTESIAN_POINT('Ctrl Pts',(-10.6712728449618,-81.5030910693985,
79.3425840826091));
#129336=CARTESIAN_POINT('Ctrl Pts',(-10.640264473015,-82.2714169121863,
78.4511433781504));
#129337=CARTESIAN_POINT('Ctrl Pts',(-10.6249089475234,-82.6170020718191,
77.9593174230282));
#129338=CARTESIAN_POINT('Ctrl Pts',(-10.5943269453012,-83.1875127282136,
76.9413325641774));
#129339=CARTESIAN_POINT('Ctrl Pts',(-10.5793594704117,-83.4169537126725,
76.42375256271));
#129340=CARTESIAN_POINT('Ctrl Pts',(-10.5486920919653,-83.7864617386823,
75.32866985789));
#129341=CARTESIAN_POINT('Ctrl Pts',(-10.5329917514054,-83.9215192221644,
74.7492098724526));
#129342=CARTESIAN_POINT('Ctrl Pts',(-10.5064524109376,-84.0539207745023,
73.7405954091737));
#129343=CARTESIAN_POINT('Ctrl Pts',(-10.4955303508667,-84.078894120976,
73.3178579165979));
#129344=CARTESIAN_POINT('Ctrl Pts',(-10.4655678147656,-84.0657291154148,
72.1769734891154));
#129345=CARTESIAN_POINT('Ctrl Pts',(-10.4464935053981,-83.9721818897685,
71.4609994507493));
#129346=CARTESIAN_POINT('Ctrl Pts',(-10.3959152218326,-83.5050413124618,
69.6067577364375));
#129347=CARTESIAN_POINT('Ctrl Pts',(-10.3655684986034,-82.9909991768275,
68.5274137916928));
#129348=CARTESIAN_POINT('Ctrl Pts',(-10.3184357299047,-81.9259658131339,
67.0981133706526));
#129349=CARTESIAN_POINT('Ctrl Pts',(-10.3027988491642,-81.5278160566466,
66.6590415619498));
#129350=CARTESIAN_POINT('Ctrl Pts',(-10.2630955556355,-80.4101039975176,
65.644636052641));
#129351=CARTESIAN_POINT('Ctrl Pts',(-10.2394869280064,-79.6434187528559,
65.1397751598418));
#129352=CARTESIAN_POINT('Ctrl Pts',(-10.1997971790316,-78.2789760985098,
64.5083161720554));
#129353=CARTESIAN_POINT('Ctrl Pts',(-10.1841445272966,-77.7180805394768,
64.3118157166981));
#129354=CARTESIAN_POINT('Ctrl Pts',(-10.1531620117269,-76.5749408104176,
64.0325708395138));
#129355=CARTESIAN_POINT('Ctrl Pts',(-10.1380002434501,-75.9966210051096,
63.9495786207854));
#129356=CARTESIAN_POINT('Ctrl Pts',(-10.0920399907937,-74.2484621824054,
63.8722749150175));
#129357=CARTESIAN_POINT('Ctrl Pts',(-10.061200132307,-73.0759366879517,
64.0451649366301));
#129358=CARTESIAN_POINT('Ctrl Pts',(-10.0230977550266,-71.7072452821346,
64.5273486670839));
#129359=CARTESIAN_POINT('Ctrl Pts',(-10.0155852308537,-71.4413011270864,
64.6358162931003));
#129360=CARTESIAN_POINT('Ctrl Pts',(-9.98249427654821,-70.2985321732764,
65.1673203799454));
#129361=CARTESIAN_POINT('Ctrl Pts',(-9.95683561054873,-69.482851806251,
65.7207502006352));
#129362=CARTESIAN_POINT('Ctrl Pts',(-9.90543200422985,-68.0615733940599,
67.0581188366673));
#129363=CARTESIAN_POINT('Ctrl Pts',(-9.88009613193941,-67.4686921055001,
67.8345464024768));
#129364=CARTESIAN_POINT('Ctrl Pts',(-9.85451228705275,-67.0084263223619,
68.6918085046015));
#129365=CARTESIAN_POINT('Ctrl Pts',(-13.5675364833309,-82.8095169451273,
77.459392053019));
#129366=CARTESIAN_POINT('Ctrl Pts',(-13.5675364833309,-82.9556776154695,
77.2295778420848));
#129367=CARTESIAN_POINT('Ctrl Pts',(-13.5675364833312,-83.0914974938587,
76.9931764216597));
#129368=CARTESIAN_POINT('Ctrl Pts',(-13.5675364833312,-83.3420981768321,
76.5073540267254));
#129369=CARTESIAN_POINT('Ctrl Pts',(-13.5675364833309,-83.456720060448,
76.2578575306141));
#129370=CARTESIAN_POINT('Ctrl Pts',(-13.5675364833309,-83.5595902541753,
76.0035856352372));
#129371=CARTESIAN_POINT('Ctrl Pts',(-13.4857787351652,-83.53086080835,69.194683933252));
#129372=CARTESIAN_POINT('Ctrl Pts',(-13.4107459268847,-82.33835458422,66.513462598172));
#129373=CARTESIAN_POINT('Ctrl Pts',(-13.2981967144638,-78.53320802489,63.458709829566));
#129374=CARTESIAN_POINT('Ctrl Pts',(-13.1481310979025,-72.48811911993,63.63322643035));
#129375=CARTESIAN_POINT('Ctrl Pts',(-13.0355818854816,-68.51429278678,65.790797832361));
#129376=CARTESIAN_POINT('Ctrl Pts',(-12.9230326730606,-65.95227475056,69.522686716285));
#129377=CARTESIAN_POINT('Ctrl Pts',(-12.8104834606397,-65.36509547432,74.009771845382));
#129378=CARTESIAN_POINT('Ctrl Pts',(-12.6979342482187,-66.87977327092,78.274405364341));
#129379=CARTESIAN_POINT('Ctrl Pts',(-12.5853850357977,-70.16613638824,81.385801227635));
#129380=CARTESIAN_POINT('Ctrl Pts',(-12.4728358233767,-74.50710712086,82.665227893767));
#129381=CARTESIAN_POINT('Ctrl Pts',(-12.3602866109556,-78.95561877133,81.83352216413));
#129382=CARTESIAN_POINT('Ctrl Pts',(-12.2477373985346,-82.54111542822,79.072147533527));
#129383=CARTESIAN_POINT('Ctrl Pts',(-12.1351881861136,-84.48133587032,74.983562774911));
#129384=CARTESIAN_POINT('Ctrl Pts',(-12.0226389736926,-84.35297372718,70.459791926131));
#129385=CARTESIAN_POINT('Ctrl Pts',(-11.9100897612715,-82.18403440969,66.487804766612));
#129386=CARTESIAN_POINT('Ctrl Pts',(-11.7975405488505,-78.44772440513,63.934186298037));
#129387=CARTESIAN_POINT('Ctrl Pts',(-11.6849913364294,-73.95921002211,63.356070078148));
#129388=CARTESIAN_POINT('Ctrl Pts',(-11.5724421240084,-69.69776911955,64.879586131319));
#129389=CARTESIAN_POINT('Ctrl Pts',(-11.4598929115869,-66.59313798963,68.172342617968));
#129390=CARTESIAN_POINT('Ctrl Pts',(-11.3473436991659,-65.32266693424,72.5159451614496));
#129391=CARTESIAN_POINT('Ctrl Pts',(-11.2347944867449,-66.16353987442,76.962731892397));
#129392=CARTESIAN_POINT('Ctrl Pts',(-11.1222452743239,-68.93230019525,80.542528950631));
#129393=CARTESIAN_POINT('Ctrl Pts',(-11.0096960619029,-73.02487543835,82.474316725385));
#129394=CARTESIAN_POINT('Ctrl Pts',(-10.8971468494819,-77.5483732915,82.336630496769));
#129395=CARTESIAN_POINT('Ctrl Pts',(-10.7845976370609,-81.5158764696,80.159504403197));
#129396=CARTESIAN_POINT('Ctrl Pts',(-10.6720484246399,-84.06180417873,76.417951402524));
#129397=CARTESIAN_POINT('Ctrl Pts',(-10.5594992122189,-84.63060417684,71.928205926366));
#129398=CARTESIAN_POINT('Ctrl Pts',(-10.4469499997979,-83.09853951678,67.670097151854));
#129399=CARTESIAN_POINT('Ctrl Pts',(-10.3344007873769,-79.79852165914,64.571579248221));
#129400=CARTESIAN_POINT('Ctrl Pts',(-10.2218515749559,-75.45555056223,63.312606598678));
#129401=CARTESIAN_POINT('Ctrl Pts',(-10.0717859583949,-69.51269706816,64.433342187813));
#129402=CARTESIAN_POINT('Ctrl Pts',(-9.95923674597391,-66.44785978885,68.230370929682));
#129403=CARTESIAN_POINT('Ctrl Pts',(-9.88420393769391,-65.8555809379,71.104431594487));
#129404=CARTESIAN_POINT('Ctrl Pts',(-13.7163617470419,-83.16594445251,69.356984978657));
#129405=CARTESIAN_POINT('Ctrl Pts',(-13.6413289387609,-82.02444891012,66.790455647208));
#129406=CARTESIAN_POINT('Ctrl Pts',(-13.5287797263401,-78.38207141327,63.866373073948));
#129407=CARTESIAN_POINT('Ctrl Pts',(-13.3787141097789,-72.59556741124,64.033424547414));
#129408=CARTESIAN_POINT('Ctrl Pts',(-13.2661648973579,-68.79172559158,66.09870361091));
#129409=CARTESIAN_POINT('Ctrl Pts',(-13.153615684937,-66.33930051512,69.670957104856));
#129410=CARTESIAN_POINT('Ctrl Pts',(-13.041066472516,-65.77723843707,73.9661025469177));
#129411=CARTESIAN_POINT('Ctrl Pts',(-12.928517260095,-67.22712433115,78.048311975543));
#129412=CARTESIAN_POINT('Ctrl Pts',(-12.815968047674,-70.37290988194,81.026614676792));
#129413=CARTESIAN_POINT('Ctrl Pts',(-12.703418835253,-74.5281911213,82.251312549785));
#129414=CARTESIAN_POINT('Ctrl Pts',(-12.590869622832,-78.78641310501,81.455183889208));
#129415=CARTESIAN_POINT('Ctrl Pts',(-12.478320410411,-82.2185364502,78.811929902003));
#129416=CARTESIAN_POINT('Ctrl Pts',(-12.3657711979899,-84.07576196493,74.898238566719));
#129417=CARTESIAN_POINT('Ctrl Pts',(-12.2532219855689,-83.95289064466,70.567976674408));
#129418=CARTESIAN_POINT('Ctrl Pts',(-12.1406727731479,-81.87672993999,66.765895355835));
#129419=CARTESIAN_POINT('Ctrl Pts',(-12.0281235607268,-78.3002444434,64.321510546861));
#129420=CARTESIAN_POINT('Ctrl Pts',(-11.9155743483058,-74.00373088522,63.768123843582));
#129421=CARTESIAN_POINT('Ctrl Pts',(-11.8030251358847,-69.92457750553,65.2264699287));
#129422=CARTESIAN_POINT('Ctrl Pts',(-11.6904759234637,-66.95275016922,68.378375365861));
#129423=CARTESIAN_POINT('Ctrl Pts',(-11.5779267110427,-65.73662482149,72.5361758376591));
#129424=CARTESIAN_POINT('Ctrl Pts',(-11.4653774986219,-66.54152855574,76.792746687058));
#129425=CARTESIAN_POINT('Ctrl Pts',(-11.3528282862009,-69.19185230266,80.219414239796));
#129426=CARTESIAN_POINT('Ctrl Pts',(-11.2402790737799,-73.10936342534,82.068567803219));
#129427=CARTESIAN_POINT('Ctrl Pts',(-11.1277298613589,-77.4393639997,81.936771244834));
#129428=CARTESIAN_POINT('Ctrl Pts',(-11.0151806489379,-81.23715314378,79.852773961851));
#129429=CARTESIAN_POINT('Ctrl Pts',(-10.9026314365169,-83.67417617347,76.271269743701));
#129430=CARTESIAN_POINT('Ctrl Pts',(-10.7900822240959,-84.21864516594,71.973577753657));
#129431=CARTESIAN_POINT('Ctrl Pts',(-10.6775330116749,-82.75211614938,67.89761396681));
#129432=CARTESIAN_POINT('Ctrl Pts',(-10.5649837992539,-79.59325995385,64.931638357232));
#129433=CARTESIAN_POINT('Ctrl Pts',(-10.4524345868329,-75.43606391784,63.726519559207));
#129434=CARTESIAN_POINT('Ctrl Pts',(-10.3023689702719,-69.7474221017,64.799314529419));
#129435=CARTESIAN_POINT('Ctrl Pts',(-10.1898197578509,-66.81368639306,68.433921456821));
#129436=CARTESIAN_POINT('Ctrl Pts',(-10.1147869495699,-66.24674287986,71.185041217093));
#129437=CARTESIAN_POINT('Ctrl Pts',(-13.9469447589179,-82.80102809666,69.519286024043));
#129438=CARTESIAN_POINT('Ctrl Pts',(-13.8719119506369,-81.710543236,67.067448696223));
#129439=CARTESIAN_POINT('Ctrl Pts',(-13.7593627382169,-78.23093480162,64.274036318316));
#129440=CARTESIAN_POINT('Ctrl Pts',(-13.6092971216549,-72.7030157025,64.433622664488));
#129441=CARTESIAN_POINT('Ctrl Pts',(-13.4967479092343,-69.06915839634,66.406609389489));
#129442=CARTESIAN_POINT('Ctrl Pts',(-13.3841986968133,-66.72632627966,69.819227493478));
#129443=CARTESIAN_POINT('Ctrl Pts',(-13.2716494843923,-66.18938139983,73.9224332485153));
#129444=CARTESIAN_POINT('Ctrl Pts',(-13.1591002719714,-67.57447539142,77.822218586803));
#129445=CARTESIAN_POINT('Ctrl Pts',(-13.0465510595504,-70.57968337571,80.667428125987));
#129446=CARTESIAN_POINT('Ctrl Pts',(-12.9340018471294,-74.54927512182,81.837397205809));
#129447=CARTESIAN_POINT('Ctrl Pts',(-12.8214526347083,-78.61720743877,81.076845614251));
#129448=CARTESIAN_POINT('Ctrl Pts',(-12.7089034222873,-81.89595747223,78.551712270408));
#129449=CARTESIAN_POINT('Ctrl Pts',(-12.5963542098663,-83.67018805956,74.81291435843));
#129450=CARTESIAN_POINT('Ctrl Pts',(-12.4838049974453,-83.55280756212,70.676161422585));
#129451=CARTESIAN_POINT('Ctrl Pts',(-12.3712557850242,-81.56942547021,67.043985944979));
#129452=CARTESIAN_POINT('Ctrl Pts',(-12.2587065726032,-78.15276448156,64.708834795646));
#129453=CARTESIAN_POINT('Ctrl Pts',(-12.1461573601821,-74.04825174822,64.180177609028));
#129454=CARTESIAN_POINT('Ctrl Pts',(-12.0336081477611,-70.15138589142,65.573353726144));
#129455=CARTESIAN_POINT('Ctrl Pts',(-11.92105893534,-67.31236234875,68.584408113854));
#129456=CARTESIAN_POINT('Ctrl Pts',(-11.808509722919,-66.15058270873,72.5564065139834));
#129457=CARTESIAN_POINT('Ctrl Pts',(-11.695960510498,-66.9195172371,76.622761481822));
#129458=CARTESIAN_POINT('Ctrl Pts',(-11.5834112980769,-69.45140441015,79.89629952903));
#129459=CARTESIAN_POINT('Ctrl Pts',(-11.4708620856559,-73.19385141245,81.662818881074));
#129460=CARTESIAN_POINT('Ctrl Pts',(-11.3583128732349,-77.330354708,81.53691199287));
#129461=CARTESIAN_POINT('Ctrl Pts',(-11.2457636608139,-80.95842981803,79.54604352044));
#129462=CARTESIAN_POINT('Ctrl Pts',(-11.1332144483929,-83.28654816823,76.124588084794));
#129463=CARTESIAN_POINT('Ctrl Pts',(-11.0206652359719,-83.80668615503,72.0189495808697));
#129464=CARTESIAN_POINT('Ctrl Pts',(-10.9081160235509,-82.40569278195,68.125130781709));
#129465=CARTESIAN_POINT('Ctrl Pts',(-10.7955668111299,-79.38799824851,65.291697466218));
#129466=CARTESIAN_POINT('Ctrl Pts',(-10.6830175987089,-75.4165772734,64.140432519737));
#129467=CARTESIAN_POINT('Ctrl Pts',(-10.5329519821479,-69.98214713522,65.165286871043));
#129468=CARTESIAN_POINT('Ctrl Pts',(-10.4204027697269,-67.17951299727,68.637471983962));
#129469=CARTESIAN_POINT('Ctrl Pts',(-10.3453699614459,-66.63790482183,71.265650839687));
#129470=CARTESIAN_POINT('Ctrl Pts',(-14.1775277707939,-82.43611174083,69.681587069447));
#129471=CARTESIAN_POINT('Ctrl Pts',(-14.1024949625139,-81.3966375619,67.344441745258));
#129472=CARTESIAN_POINT('Ctrl Pts',(-13.9899457500929,-78.07979819,64.681699562697));
#129473=CARTESIAN_POINT('Ctrl Pts',(-13.8398801335319,-72.8104639938,64.833820781552));
#129474=CARTESIAN_POINT('Ctrl Pts',(-13.7273309211109,-69.34659120114,66.714515168039));
#129475=CARTESIAN_POINT('Ctrl Pts',(-13.6147817086899,-67.11335204423,69.967497882051));
#129476=CARTESIAN_POINT('Ctrl Pts',(-13.5022324962687,-66.60152436258,73.878763950054));
#129477=CARTESIAN_POINT('Ctrl Pts',(-13.3896832838477,-67.92182645165,77.596125198008));
#129478=CARTESIAN_POINT('Ctrl Pts',(-13.2771340714267,-70.78645686942,80.308241575145));
#129479=CARTESIAN_POINT('Ctrl Pts',(-13.1645848590057,-74.57035912226,81.423481861828));
#129480=CARTESIAN_POINT('Ctrl Pts',(-13.0520356465847,-78.44800177245,80.698507339327));
#129481=CARTESIAN_POINT('Ctrl Pts',(-12.9394864341637,-81.57337849421,78.29149463888));
#129482=CARTESIAN_POINT('Ctrl Pts',(-12.8269372217426,-83.26461415418,74.727590150234));
#129483=CARTESIAN_POINT('Ctrl Pts',(-12.7143880093216,-83.1527244796,70.784346170858));
#129484=CARTESIAN_POINT('Ctrl Pts',(-12.6018387969006,-81.26212100051,67.322076534199));
#129485=CARTESIAN_POINT('Ctrl Pts',(-12.4892895844795,-78.00528451983,65.096159044468));
#129486=CARTESIAN_POINT('Ctrl Pts',(-12.3767403720585,-74.09277261133,64.592231374463));
#129487=CARTESIAN_POINT('Ctrl Pts',(-12.2641911596374,-70.37819427741,65.920237523529));
#129488=CARTESIAN_POINT('Ctrl Pts',(-12.1516419472164,-67.67197452834,68.790440861752));
#129489=CARTESIAN_POINT('Ctrl Pts',(-12.0390927347954,-66.56454059598,72.5766371901983));
#129490=CARTESIAN_POINT('Ctrl Pts',(-11.9265435223743,-67.29750591841,76.452776276488));
#129491=CARTESIAN_POINT('Ctrl Pts',(-11.8139943099533,-69.71095651757,79.573184818198));
#129492=CARTESIAN_POINT('Ctrl Pts',(-11.7014450975323,-73.27833939945,81.257069958908));
#129493=CARTESIAN_POINT('Ctrl Pts',(-11.5888958851112,-77.22134541621,81.137052740933));
#129494=CARTESIAN_POINT('Ctrl Pts',(-11.4763466726899,-80.67970649221,79.239313079091));
#129495=CARTESIAN_POINT('Ctrl Pts',(-11.3637974602689,-82.89892016296,75.977906425967));
#129496=CARTESIAN_POINT('Ctrl Pts',(-11.2512482478479,-83.39472714413,72.0643214081572));
#129497=CARTESIAN_POINT('Ctrl Pts',(-11.1386990354269,-82.05926941456,68.352647596662));
#129498=CARTESIAN_POINT('Ctrl Pts',(-11.0261498230059,-79.18273654321,65.651756575228));
#129499=CARTESIAN_POINT('Ctrl Pts',(-10.9136006105849,-75.39709062901,64.554345480267));
#129500=CARTESIAN_POINT('Ctrl Pts',(-10.7635349940239,-70.21687216876,65.53125921265));
#129501=CARTESIAN_POINT('Ctrl Pts',(-10.6509857816029,-67.54533960148,68.841022511101));
#129502=CARTESIAN_POINT('Ctrl Pts',(-10.5759529733229,-67.02906676379,71.346260462292));
#129503=CARTESIAN_POINT('',(-13.563311219297,-81.8872991846617,67.092553089091));
#129504=CARTESIAN_POINT('Ctrl Pts',(-13.559085955263,-81.8925473588303,
67.087485454259));
#129505=CARTESIAN_POINT('Ctrl Pts',(-13.5557378489868,-81.8226484187543,
67.0056955122904));
#129506=CARTESIAN_POINT('Ctrl Pts',(-13.5524040041999,-81.7513035648403,
66.9251397154799));
#129507=CARTESIAN_POINT('Ctrl Pts',(-13.5407945360191,-81.4958535332512,
66.6468193919849));
#129508=CARTESIAN_POINT('Ctrl Pts',(-13.5326654402662,-81.3042813848844,
66.4559020117066));
#129509=CARTESIAN_POINT('Ctrl Pts',(-13.5216044230679,-81.0190668043286,
66.1963000811713));
#129510=CARTESIAN_POINT('Ctrl Pts',(-13.5183611378651,-80.932138867054,
66.1202002131299));
#129511=CARTESIAN_POINT('Ctrl Pts',(-13.5133368922477,-80.7915755236166,
66.0019193088781));
#129512=CARTESIAN_POINT('Ctrl Pts',(-13.5115026272737,-80.7389583800737,
65.9586663606433));
#129513=CARTESIAN_POINT('Ctrl Pts',(-13.5079429779001,-80.634394306066,
65.8746963206787));
#129514=CARTESIAN_POINT('Ctrl Pts',(-13.5062160018049,-80.5824778523595,
65.8339426977273));
#129515=CARTESIAN_POINT('Ctrl Pts',(-13.5021175780405,-80.4565479340235,
65.7373147660614));
#129516=CARTESIAN_POINT('Ctrl Pts',(-13.4997684762369,-80.3821031546346,
65.6820031944673));
#129517=CARTESIAN_POINT('Ctrl Pts',(-13.4917599280967,-80.1210357304505,
65.4942033786579));
#129518=CARTESIAN_POINT('Ctrl Pts',(-13.4863033905747,-79.9301647455721,
65.3676160031791));
#129519=CARTESIAN_POINT('Ctrl Pts',(-13.4630988413414,-79.0746195119488,
64.8454007412283));
#129520=CARTESIAN_POINT('Ctrl Pts',(-13.446939288299,-78.3629248291164,
64.5261308523007));
#129521=CARTESIAN_POINT('Ctrl Pts',(-13.4209340605883,-77.2639858617722,
64.1930428150856));
#129522=CARTESIAN_POINT('Ctrl Pts',(-13.4120849370132,-76.8984839701938,
64.1065784692331));
#129523=CARTESIAN_POINT('Ctrl Pts',(-13.3969918678252,-76.2964750450373,
64.0041304265887));
#129524=CARTESIAN_POINT('Ctrl Pts',(-13.3910705329244,-76.0640729471427,
63.9739159071207));
#129525=CARTESIAN_POINT('Ctrl Pts',(-13.3785301259652,-75.5780202632669,
63.9297652567008));
#129526=CARTESIAN_POINT('Ctrl Pts',(-13.3718943919218,-75.3242247504548,
63.9174109355893));
#129527=CARTESIAN_POINT('Ctrl Pts',(-13.3434831198087,-74.2489047375888,
63.9097876203767));
#129528=CARTESIAN_POINT('Ctrl Pts',(-13.3210969350338,-73.4262833985882,
64.0144787652504));
#129529=CARTESIAN_POINT('Ctrl Pts',(-13.2926222433935,-72.4136094699141,
64.2872776090376));
#129530=CARTESIAN_POINT('Ctrl Pts',(-13.2864879360885,-72.196911524819,
64.3546050530603));
#129531=CARTESIAN_POINT('Ctrl Pts',(-13.2630150838093,-71.3647346241283,
64.6485723429744));
#129532=CARTESIAN_POINT('Ctrl Pts',(-13.2462305930131,-70.7711117695441,
64.9345765112858));
#129533=CARTESIAN_POINT('Ctrl Pts',(-13.2210144551986,-69.9428478544483,
65.4487924270168));
#129534=CARTESIAN_POINT('Ctrl Pts',(-13.2127031844204,-69.6798945229241,
65.6317243516277));
#129535=CARTESIAN_POINT('Ctrl Pts',(-13.1966424718445,-69.1982179606711,
66.0058185752753));
#129536=CARTESIAN_POINT('Ctrl Pts',(-13.1888955316257,-68.9776420069283,
66.1946330030121));
#129537=CARTESIAN_POINT('Ctrl Pts',(-13.1773764931447,-68.6676876440164,
66.4870709710263));
#129538=CARTESIAN_POINT('Ctrl Pts',(-13.1736883415841,-68.5708050822243,
66.5827289685801));
#129539=CARTESIAN_POINT('Ctrl Pts',(-13.1634531773245,-68.3063476211814,
66.8561035446628));
#129540=CARTESIAN_POINT('Ctrl Pts',(-13.1569968246614,-68.1440755051959,
67.0383552906632));
#129541=CARTESIAN_POINT('Ctrl Pts',(-13.1366314630471,-67.6506569957674,
67.6398730643821));
#129542=CARTESIAN_POINT('Ctrl Pts',(-13.1229846344129,-67.3484668753696,
68.0831733061487));
#129543=CARTESIAN_POINT('Ctrl Pts',(-13.1026671090003,-66.9635998900805,
68.7692394324011));
#129544=CARTESIAN_POINT('Ctrl Pts',(-13.0961153737121,-66.8492400866051,
68.9943566288763));
#129545=CARTESIAN_POINT('Ctrl Pts',(-13.083431494371,-66.6488881705089,
69.4327296147196));
#129546=CARTESIAN_POINT('Ctrl Pts',(-13.0773086994625,-66.5612676714018,
69.6452604753881));
#129547=CARTESIAN_POINT('Ctrl Pts',(-13.0645429528433,-66.3982345792593,
70.0877189116747));
#129548=CARTESIAN_POINT('Ctrl Pts',(-13.0579148759919,-66.3237102061575,
70.3179694825108));
#129549=CARTESIAN_POINT('Ctrl Pts',(-13.0463406873125,-66.2085000486793,
70.7304437977745));
#129550=CARTESIAN_POINT('Ctrl Pts',(-13.0413850099358,-66.1641151190626,
70.9111354100525));
#129551=CARTESIAN_POINT('Ctrl Pts',(-13.0288741208045,-66.0650095113933,
71.3767387413974));
#129552=CARTESIAN_POINT('Ctrl Pts',(-13.0214032712663,-66.0184056734035,
71.6632455841991));
#129553=CARTESIAN_POINT('Ctrl Pts',(-13.0051273905784,-65.9464198857517,
72.2944176611577));
#129554=CARTESIAN_POINT('Ctrl Pts',(-12.9963384395356,-65.9267882999154,
72.6397606252193));
#129555=CARTESIAN_POINT('Ctrl Pts',(-12.9813320943859,-65.9265458581992,
73.2211658979305));
#129556=CARTESIAN_POINT('Ctrl Pts',(-12.9751799741108,-65.9355563574263,
73.4572664963566));
#129557=CARTESIAN_POINT('Ctrl Pts',(-12.9597906409308,-65.9800744166607,
74.0355245727726));
#129558=CARTESIAN_POINT('Ctrl Pts',(-12.9503423706044,-66.0258024785281,
74.376894732432));
#129559=CARTESIAN_POINT('Ctrl Pts',(-12.936706483897,-66.1201634042575,
74.8664653571157));
#129560=CARTESIAN_POINT('Ctrl Pts',(-12.9324897465908,-66.1533623899488,
75.017630596075));
#129561=CARTESIAN_POINT('Ctrl Pts',(-12.9242274807111,-66.2270688729963,
75.3158989494287));
#129562=CARTESIAN_POINT('Ctrl Pts',(-12.9201940123229,-66.2674172210885,
75.4627941290223));
#129563=CARTESIAN_POINT('Ctrl Pts',(-12.9056351533373,-66.4284273094106,
75.9954678935174));
#129564=CARTESIAN_POINT('Ctrl Pts',(-12.8953959509123,-66.5715638217598,
76.3744766954144));
#129565=CARTESIAN_POINT('Ctrl Pts',(-12.8791747875566,-66.8360786683099,
76.9553847514503));
#129566=CARTESIAN_POINT('Ctrl Pts',(-12.8732144367455,-66.9412535465598,
77.164683710942));
#129567=CARTESIAN_POINT('Ctrl Pts',(-12.862496332028,-67.1416748123932,
77.5281895284742));
#129568=CARTESIAN_POINT('Ctrl Pts',(-12.8577716964445,-67.2337792288395,
77.6841463237772));
#129569=CARTESIAN_POINT('Ctrl Pts',(-12.8426574301479,-67.5377368105897,
78.1656496446993));
#129570=CARTESIAN_POINT('Ctrl Pts',(-12.8319026905027,-67.7659395902239,
78.480884158594));
#129571=CARTESIAN_POINT('Ctrl Pts',(-12.8172087319959,-68.1082589586898,
78.8946606387161));
#129572=CARTESIAN_POINT('Ctrl Pts',(-12.813161188698,-68.2058592810763,
79.0068609964641));
#129573=CARTESIAN_POINT('Ctrl Pts',(-12.8054836864172,-68.3987426811209,
79.2177078607287));
#129574=CARTESIAN_POINT('Ctrl Pts',(-12.8018591577577,-68.4934297980403,
79.3165212196181));
#129575=CARTESIAN_POINT('Ctrl Pts',(-12.7924877187558,-68.7473583304201,
79.5695965652197));
#129576=CARTESIAN_POINT('Ctrl Pts',(-12.7868132265313,-68.9100914481405,
79.7201525763961));
#129577=CARTESIAN_POINT('Ctrl Pts',(-12.7731297896651,-69.3184822447202,
80.0711096023261));
#129578=CARTESIAN_POINT('Ctrl Pts',(-12.7651667228754,-69.569679986819,
80.2650684300452));
#129579=CARTESIAN_POINT('Ctrl Pts',(-12.7519826161154,-69.9944066093667,
80.5592161990268));
#129580=CARTESIAN_POINT('Ctrl Pts',(-12.7468362248654,-70.1623146785122,
80.6675635282834));
#129581=CARTESIAN_POINT('Ctrl Pts',(-12.7377107898938,-70.4601528412897,
80.8462648526309));
#129582=CARTESIAN_POINT('Ctrl Pts',(-12.7337704010071,-70.5885659943192,
80.9191581331012));
#129583=CARTESIAN_POINT('Ctrl Pts',(-12.7205899472585,-71.0185155206958,
81.1496543168899));
#129584=CARTESIAN_POINT('Ctrl Pts',(-12.7111645111972,-71.3273400643339,
81.2936959039509));
#129585=CARTESIAN_POINT('Ctrl Pts',(-12.6978913807998,-71.778492875624,
81.473837303909));
#129586=CARTESIAN_POINT('Ctrl Pts',(-12.6939377820586,-71.9149891906426,
81.5245438986882));
#129587=CARTESIAN_POINT('Ctrl Pts',(-12.6865509171379,-72.1755740522596,
81.6141597880879));
#129588=CARTESIAN_POINT('Ctrl Pts',(-12.6831168399744,-72.2992233922656,
81.6536808195843));
#129589=CARTESIAN_POINT('Ctrl Pts',(-12.6686769484691,-72.8300938688756,
81.8106190406682));
#129590=CARTESIAN_POINT('Ctrl Pts',(-12.6581004599294,-73.2447671539909,
81.9017477773994));
#129591=CARTESIAN_POINT('Ctrl Pts',(-12.6429841521371,-73.8365551857166,
81.9893019522603));
#129592=CARTESIAN_POINT('Ctrl Pts',(-12.6385485030208,-74.0100931116062,
82.009911378161));
#129593=CARTESIAN_POINT('Ctrl Pts',(-12.6303897858426,-74.3256428695035,
82.0382757901307));
#129594=CARTESIAN_POINT('Ctrl Pts',(-12.6266868331992,-74.4675083578769,
82.047710511139));
#129595=CARTESIAN_POINT('Ctrl Pts',(-12.617520560906,-74.8133822434634,
82.0626548227512));
#129596=CARTESIAN_POINT('Ctrl Pts',(-12.6120030923282,-75.0175466471059,
82.0646645233081));
#129597=CARTESIAN_POINT('Ctrl Pts',(-12.5981418281175,-75.5257306599595,
82.052666705461));
#129598=CARTESIAN_POINT('Ctrl Pts',(-12.5897407616311,-75.8295717809301,
82.0303066237215));
#129599=CARTESIAN_POINT('Ctrl Pts',(-12.5776346915689,-76.271213910937,
81.9752554899712));
#129600=CARTESIAN_POINT('Ctrl Pts',(-12.5738318146591,-76.4105098580751,
81.9545707858028));
#129601=CARTESIAN_POINT('Ctrl Pts',(-12.5666397528045,-76.6762659673904,
81.9086642122392));
#129602=CARTESIAN_POINT('Ctrl Pts',(-12.5632489873379,-76.8026940836846,
81.8839939833719));
#129603=CARTESIAN_POINT('Ctrl Pts',(-12.5543979821308,-77.1359613642734,
81.8113936413141));
#129604=CARTESIAN_POINT('Ctrl Pts',(-12.5490142640923,-77.3415385101451,
81.758863685658));
#129605=CARTESIAN_POINT('Ctrl Pts',(-12.5371414791353,-77.7931385035952,
81.6263902756365));
#129606=CARTESIAN_POINT('Ctrl Pts',(-12.5306687199678,-78.0381323963354,
81.5429642811284));
#129607=CARTESIAN_POINT('Ctrl Pts',(-12.5198097905863,-78.4360483812377,
81.3883567270092));
#129608=CARTESIAN_POINT('Ctrl Pts',(-12.5154832156024,-78.5912660416973,
81.3230622102699));
#129609=CARTESIAN_POINT('Ctrl Pts',(-12.5067780224793,-78.8938256450294,
81.1858722808496));
#129610=CARTESIAN_POINT('Ctrl Pts',(-12.5024086538887,-79.0412709331833,
81.1141948716209));
#129611=CARTESIAN_POINT('Ctrl Pts',(-12.4876512850363,-79.527378984235,
80.8615686936808));
#129612=CARTESIAN_POINT('Ctrl Pts',(-12.47705886029,-79.8569878952453,80.6631100560213));
#129613=CARTESIAN_POINT('Ctrl Pts',(-12.4605950155113,-80.354581441332,
80.3186909925396));
#129614=CARTESIAN_POINT('Ctrl Pts',(-12.4546255940102,-80.5318605086843,
80.1861291658312));
#129615=CARTESIAN_POINT('Ctrl Pts',(-12.4451535059546,-80.810645255994,
79.9610489072495));
#129616=CARTESIAN_POINT('Ctrl Pts',(-12.441587635747,-80.9151227787878,
79.8726402084329));
#129617=CARTESIAN_POINT('Ctrl Pts',(-12.4297682171708,-81.2591813213333,
79.5675826799819));
#129618=CARTESIAN_POINT('Ctrl Pts',(-12.4217150343873,-81.4890080079709,
79.3404125362031));
#129619=CARTESIAN_POINT('Ctrl Pts',(-12.4097902796803,-81.8067228412527,
78.9911061652808));
#129620=CARTESIAN_POINT('Ctrl Pts',(-12.4059944973883,-81.9045785673756,
78.8780468884581));
#129621=CARTESIAN_POINT('Ctrl Pts',(-12.3983150778161,-82.0941562183193,
78.6478522649579));
#129622=CARTESIAN_POINT('Ctrl Pts',(-12.3944253424699,-82.1859075482073,
78.5307387402166));
#129623=CARTESIAN_POINT('Ctrl Pts',(-12.3792466122153,-82.5284005675861,
78.0709765756556));
#129624=CARTESIAN_POINT('Ctrl Pts',(-12.3676265905513,-82.7584450752342,
77.7128311661701));
#129625=CARTESIAN_POINT('Ctrl Pts',(-12.3501789095285,-83.0665612399772,
77.1504303401466));
#129626=CARTESIAN_POINT('Ctrl Pts',(-12.3443007404031,-83.1639025978138,
76.9566677648474));
#129627=CARTESIAN_POINT('Ctrl Pts',(-12.3338989010385,-83.3256751822307,
76.603449511283));
#129628=CARTESIAN_POINT('Ctrl Pts',(-12.3293470789259,-83.3927442843099,
76.4452086806175));
#129629=CARTESIAN_POINT('Ctrl Pts',(-12.3188128681221,-83.5396698100925,
76.0685689243611));
#129630=CARTESIAN_POINT('Ctrl Pts',(-12.3129233796486,-83.6155003438947,
75.8490333280528));
#129631=CARTESIAN_POINT('Ctrl Pts',(-12.3017494698807,-83.7437471914812,
75.4254880926722));
#129632=CARTESIAN_POINT('Ctrl Pts',(-12.2964530014789,-83.7977143608655,
75.2217730391077));
#129633=CARTESIAN_POINT('Ctrl Pts',(-12.2866451140008,-83.8831460865559,
74.847307777468));
#129634=CARTESIAN_POINT('Ctrl Pts',(-12.2821484921725,-83.9169005397076,
74.6770802211227));
#129635=CARTESIAN_POINT('Ctrl Pts',(-12.2699862396666,-83.993978017679,
74.2208274413097));
#129636=CARTESIAN_POINT('Ctrl Pts',(-12.2622222761676,-84.0286547814944,
73.9333196481195));
#129637=CARTESIAN_POINT('Ctrl Pts',(-12.2450150622112,-84.07496636679,73.2979981206966));
#129638=CARTESIAN_POINT('Ctrl Pts',(-12.2355493233976,-84.0805245330233,
72.9496900656169));
#129639=CARTESIAN_POINT('Ctrl Pts',(-12.219973209062,-84.0564487416857,
72.370212445068));
#129640=CARTESIAN_POINT('Ctrl Pts',(-12.2137929796483,-84.0378942134671,
72.1385725370326));
#129641=CARTESIAN_POINT('Ctrl Pts',(-12.2014267933846,-83.9817597033124,
71.6687664535025));
#129642=CARTESIAN_POINT('Ctrl Pts',(-12.1953024392983,-83.9435552079869,
71.4314753887407));
#129643=CARTESIAN_POINT('Ctrl Pts',(-12.1824024959074,-83.8426072573388,
70.9328443161101));
#129644=CARTESIAN_POINT('Ctrl Pts',(-12.175606987108,-83.7775697389122,
70.6721752894815));
#129645=CARTESIAN_POINT('Ctrl Pts',(-12.1618712395346,-83.6269495897832,
70.164906507135));
#129646=CARTESIAN_POINT('Ctrl Pts',(-12.1549798667685,-83.5420053403461,
69.9181172023374));
#129647=CARTESIAN_POINT('Ctrl Pts',(-12.1353898234166,-83.2735999437275,
69.2344195535132));
#129648=CARTESIAN_POINT('Ctrl Pts',(-12.1225434617862,-83.0662956243893,
68.8067637860057));
#129649=CARTESIAN_POINT('Ctrl Pts',(-12.1037492686791,-82.7116612292542,
68.2006434754007));
#129650=CARTESIAN_POINT('Ctrl Pts',(-12.0976726041932,-82.5888330849021,
68.0077748431867));
#129651=CARTESIAN_POINT('Ctrl Pts',(-12.0856429660484,-82.3280912483103,
67.6309355267796));
#129652=CARTESIAN_POINT('Ctrl Pts',(-12.0797266482992,-82.1904393974301,
67.4475114577697));
#129653=CARTESIAN_POINT('Ctrl Pts',(-12.0671749847703,-81.8806577161547,
67.0664029530817));
#129654=CARTESIAN_POINT('Ctrl Pts',(-12.0605190336008,-81.7070720184151,
66.8709785133379));
#129655=CARTESIAN_POINT('Ctrl Pts',(-12.035267722196,-81.0308357003993,
66.1726915170404));
#129656=CARTESIAN_POINT('Ctrl Pts',(-12.0161276153687,-80.4762119092328,
65.7198702614967));
#129657=CARTESIAN_POINT('Ctrl Pts',(-11.9885354599265,-79.6047850254594,
65.1632441845259));
#129658=CARTESIAN_POINT('Ctrl Pts',(-11.9799480428361,-79.3232196806061,
65.0037564975032));
#129659=CARTESIAN_POINT('Ctrl Pts',(-11.9555460584312,-78.4902178801228,
64.5896125196323));
#129660=CARTESIAN_POINT('Ctrl Pts',(-11.9401654023462,-77.9226318585693,
64.3769185663475));
#129661=CARTESIAN_POINT('Ctrl Pts',(-11.9095711822706,-76.7974166915148,
64.077714367338));
#129662=CARTESIAN_POINT('Ctrl Pts',(-11.8946383898076,-76.2413160159509,
63.983441562345));
#129663=CARTESIAN_POINT('Ctrl Pts',(-11.8651054933457,-75.1313007927164,
63.8988593087306));
#129664=CARTESIAN_POINT('Ctrl Pts',(-11.8505012040217,-74.5763507546515,
63.9066755440276));
#129665=CARTESIAN_POINT('Ctrl Pts',(-11.8056121264091,-72.8668116532728,
64.0920100148967));
#129666=CARTESIAN_POINT('Ctrl Pts',(-11.7749787653385,-71.7329701178857,
64.4446450603372));
#129667=CARTESIAN_POINT('Ctrl Pts',(-11.7288034797534,-70.1937132121955,
65.2692902920736));
#129668=CARTESIAN_POINT('Ctrl Pts',(-11.7134866021105,-69.7120312900423,
65.5907288589313));
#129669=CARTESIAN_POINT('Ctrl Pts',(-11.6715688233447,-68.4736430122908,
66.6038228064739));
#129670=CARTESIAN_POINT('Ctrl Pts',(-11.6452414234691,-67.7939667727339,
67.3819253526641));
#129671=CARTESIAN_POINT('Ctrl Pts',(-11.6118309935208,-67.1379883663413,
68.4505909544893));
#129672=CARTESIAN_POINT('Ctrl Pts',(-11.6054799560098,-67.0225405329474,
68.6563132895332));
#129673=CARTESIAN_POINT('Ctrl Pts',(-11.5886254045895,-66.7359352067647,
69.2183212618494));
#129674=CARTESIAN_POINT('Ctrl Pts',(-11.5782817421966,-66.5799982454277,
69.5821855594921));
#129675=CARTESIAN_POINT('Ctrl Pts',(-11.5514878718896,-66.236295204117,
70.5541418509554));
#129676=CARTESIAN_POINT('Ctrl Pts',(-11.535146718226,-66.0870511625888,
71.1761051919815));
#129677=CARTESIAN_POINT('Ctrl Pts',(-11.5094703351698,-65.9590926721202,
72.1432071313965));
#129678=CARTESIAN_POINT('Ctrl Pts',(-11.5003872011654,-65.9333107407222,
72.4823240137874));
#129679=CARTESIAN_POINT('Ctrl Pts',(-11.4829997777813,-65.9209453621675,
73.124259887423));
#129680=CARTESIAN_POINT('Ctrl Pts',(-11.4748714117761,-65.9304147698513,
73.4257664585309));
#129681=CARTESIAN_POINT('Ctrl Pts',(-11.4556877679753,-65.9902539903833,
74.1516658337673));
#129682=CARTESIAN_POINT('Ctrl Pts',(-11.4447447212086,-66.0554078580195,
74.5733722865264));
#129683=CARTESIAN_POINT('Ctrl Pts',(-11.4224735425153,-66.2469448313981,
75.4183849888865));
#129684=CARTESIAN_POINT('Ctrl Pts',(-11.41113960832,-66.3754432388486,75.8413030543231));
#129685=CARTESIAN_POINT('Ctrl Pts',(-11.3935752632689,-66.6144863276698,
76.4629018788126));
#129686=CARTESIAN_POINT('Ctrl Pts',(-11.3875512045202,-66.703078855393,
76.670103989202));
#129687=CARTESIAN_POINT('Ctrl Pts',(-11.3735078648652,-66.9240711877018,
77.137935896527));
#129688=CARTESIAN_POINT('Ctrl Pts',(-11.3654708854703,-67.0616573327916,
77.3961033942245));
#129689=CARTESIAN_POINT('Ctrl Pts',(-11.3527699139652,-67.3046267288358,
77.8023906857588));
#129690=CARTESIAN_POINT('Ctrl Pts',(-11.3479887887623,-67.4023484089624,
77.9549881033649));
#129691=CARTESIAN_POINT('Ctrl Pts',(-11.3377039099922,-67.6247424021602,
78.2802199958459));
#129692=CARTESIAN_POINT('Ctrl Pts',(-11.3322193338531,-67.7511630632259,
78.4517057192843));
#129693=CARTESIAN_POINT('Ctrl Pts',(-11.3124185053928,-68.2312664237496,
79.0572791980971));
#129694=CARTESIAN_POINT('Ctrl Pts',(-11.2982657719826,-68.6196423799201,
79.4639972476825));
#129695=CARTESIAN_POINT('Ctrl Pts',(-11.2787715814941,-69.1771042720877,
79.9500337849055));
#129696=CARTESIAN_POINT('Ctrl Pts',(-11.2739662512911,-69.3160426787427,
80.0641532312963));
#129697=CARTESIAN_POINT('Ctrl Pts',(-11.262817305294,-69.6412828963894,
80.3155537500748));
#129698=CARTESIAN_POINT('Ctrl Pts',(-11.2564498950354,-69.8297243550707,
80.4500687474039));
#129699=CARTESIAN_POINT('Ctrl Pts',(-11.2447256892503,-70.1883215496775,
80.6857100721471));
#129700=CARTESIAN_POINT('Ctrl Pts',(-11.2393556625268,-70.3572539516981,
80.7889130438971));
#129701=CARTESIAN_POINT('Ctrl Pts',(-11.2294950337287,-70.6803179939104,
80.971690160875));
#129702=CARTESIAN_POINT('Ctrl Pts',(-11.2249757098433,-70.8333852967702,
81.052492076728));
#129703=CARTESIAN_POINT('Ctrl Pts',(-11.2147842416095,-71.1873142054762,
81.2264846822883));
#129704=CARTESIAN_POINT('Ctrl Pts',(-11.2091430517,-71.3895698597399,81.3168235808343));
#129705=CARTESIAN_POINT('Ctrl Pts',(-11.1928228284033,-71.985184406746,
81.5572487943015));
#129706=CARTESIAN_POINT('Ctrl Pts',(-11.1821830457734,-72.3864812781739,
81.6877900173541));
#129707=CARTESIAN_POINT('Ctrl Pts',(-11.1672197941371,-72.94151884285,81.8270353181207));
#129708=CARTESIAN_POINT('Ctrl Pts',(-11.1632145090628,-73.0891861999772,
81.8602227975301));
#129709=CARTESIAN_POINT('Ctrl Pts',(-11.155076789241,-73.3861335316759,
81.9192649628482));
#129710=CARTESIAN_POINT('Ctrl Pts',(-11.1509507638806,-73.5354179741734,
81.9451126153875));
#129711=CARTESIAN_POINT('Ctrl Pts',(-11.136345270979,-74.0632482480024,
82.0229871572942));
#129712=CARTESIAN_POINT('Ctrl Pts',(-11.1257607190002,-74.4447532345393,
82.0549445472154));
#129713=CARTESIAN_POINT('Ctrl Pts',(-11.1117147504199,-74.9733152347867,
82.0650328851075));
#129714=CARTESIAN_POINT('Ctrl Pts',(-11.1078845385412,-75.1198987599237,
82.064201547195));
#129715=CARTESIAN_POINT('Ctrl Pts',(-11.0994677740146,-75.4453943606477,
82.0543833055328));
#129716=CARTESIAN_POINT('Ctrl Pts',(-11.0949024066108,-75.6242461350268,
82.0436262524113));
#129717=CARTESIAN_POINT('Ctrl Pts',(-11.0787649462341,-76.258124511933,
81.9866335788158));
#129718=CARTESIAN_POINT('Ctrl Pts',(-11.0673216940971,-76.7105666564122,
81.9112406965473));
#129719=CARTESIAN_POINT('Ctrl Pts',(-11.0517603340098,-77.2894569777918,
81.7697555753342));
#129720=CARTESIAN_POINT('Ctrl Pts',(-11.0480914431371,-77.4233479071564,
81.7337998165184));
#129721=CARTESIAN_POINT('Ctrl Pts',(-11.0402828875073,-77.7025558157715,
81.6519880196989));
#129722=CARTESIAN_POINT('Ctrl Pts',(-11.0361393291105,-77.8476910893183,
81.6055027991634));
#129723=CARTESIAN_POINT('Ctrl Pts',(-11.0226028032279,-78.3151379631504,
81.4427744268616));
#129724=CARTESIAN_POINT('Ctrl Pts',(-11.013117398753,-78.632367274265,81.3119098409886));
#129725=CARTESIAN_POINT('Ctrl Pts',(-11.0001390418047,-79.0660376683573,
81.1031778333896));
#129726=CARTESIAN_POINT('Ctrl Pts',(-10.996440079161,-79.1896286560287,
81.0401168218329));
#129727=CARTESIAN_POINT('Ctrl Pts',(-10.9881276344862,-79.4684405309305,
80.8894971637464));
#129728=CARTESIAN_POINT('Ctrl Pts',(-10.9835493630003,-79.6224993875693,
80.8002005014945));
#129729=CARTESIAN_POINT('Ctrl Pts',(-10.9719173868032,-80.0107888351821,
80.559498709591));
#129730=CARTESIAN_POINT('Ctrl Pts',(-10.9649310590942,-80.2409714860484,
80.4015796609635));
#129731=CARTESIAN_POINT('Ctrl Pts',(-10.9520909189305,-80.6463227010311,
80.0953038614243));
#129732=CARTESIAN_POINT('Ctrl Pts',(-10.9462563662033,-80.823996584897,
79.9502453449538));
#129733=CARTESIAN_POINT('Ctrl Pts',(-10.9367398462232,-81.0981567056813,
79.7087565036097));
#129734=CARTESIAN_POINT('Ctrl Pts',(-10.9331400685857,-81.1983222258153,
79.6164897843008));
#129735=CARTESIAN_POINT('Ctrl Pts',(-10.9253018669614,-81.4092241844754,
79.4133595792018));
#129736=CARTESIAN_POINT('Ctrl Pts',(-10.9210528015737,-81.5192815238177,
79.3017862909333));
#129737=CARTESIAN_POINT('Ctrl Pts',(-10.9068397495232,-81.875487434268,
78.921620380461));
#129738=CARTESIAN_POINT('Ctrl Pts',(-10.8967655389423,-82.1087030403898,
78.6408843880499));
#129739=CARTESIAN_POINT('Ctrl Pts',(-10.8828483312068,-82.413679900872,
78.2247447023));
#129740=CARTESIAN_POINT('Ctrl Pts',(-10.8788010458399,-82.500209868164,
78.1001817229147));
#129741=CARTESIAN_POINT('Ctrl Pts',(-10.8706266961558,-82.671333260355,
77.8398668968101));
#129742=CARTESIAN_POINT('Ctrl Pts',(-10.8665121345898,-82.7555152168254,
77.7039405008203));
#129743=CARTESIAN_POINT('Ctrl Pts',(-10.856353382447,-82.9563723238259,
77.3594219109496));
#129744=CARTESIAN_POINT('Ctrl Pts',(-10.8503610923287,-83.068510749718,
77.1481308616468));
#129745=CARTESIAN_POINT('Ctrl Pts',(-10.8381288231242,-83.2790978353818,
76.710575011933));
#129746=CARTESIAN_POINT('Ctrl Pts',(-10.831886352734,-83.3770033625072,
76.4840451405209));
#129747=CARTESIAN_POINT('Ctrl Pts',(-10.8217668907393,-83.5169687353684,
76.1206408386014));
#129748=CARTESIAN_POINT('Ctrl Pts',(-10.8179950385984,-83.5651983130977,
75.9861295767924));
#129749=CARTESIAN_POINT('Ctrl Pts',(-10.8096809863021,-83.6634147315317,
75.690676263741));
#129750=CARTESIAN_POINT('Ctrl Pts',(-10.8051227658235,-83.7121656758757,
75.5293153899842));
#129751=CARTESIAN_POINT('Ctrl Pts',(-10.7899774491732,-83.8583919350915,
74.9922351118796));
#129752=CARTESIAN_POINT('Ctrl Pts',(-10.779276771381,-83.9365571395873,
74.6112262864475));
#129753=CARTESIAN_POINT('Ctrl Pts',(-10.764446174225,-84.0122615806992,
74.0652142323235));
#129754=CARTESIAN_POINT('Ctrl Pts',(-10.7601036036432,-84.0302707333152,
73.903055698679));
#129755=CARTESIAN_POINT('Ctrl Pts',(-10.7514349197537,-84.0577630941967,
73.5730469775939));
#129756=CARTESIAN_POINT('Ctrl Pts',(-10.7471287260413,-84.0669374929368,
73.405428682919));
#129757=CARTESIAN_POINT('Ctrl Pts',(-10.7358619095138,-84.0787625241277,
72.9619473847261));
#129758=CARTESIAN_POINT('Ctrl Pts',(-10.7289707149286,-84.0733941778988,
72.685805038355));
#129759=CARTESIAN_POINT('Ctrl Pts',(-10.7172883315525,-84.0435205228047,
72.225632846293));
#129760=CARTESIAN_POINT('Ctrl Pts',(-10.7125468286424,-84.0258848894152,
72.0411589170452));
#129761=CARTESIAN_POINT('Ctrl Pts',(-10.7028091161632,-83.9791780091691,
71.6713067829865));
#129762=CARTESIAN_POINT('Ctrl Pts',(-10.6978240824464,-83.9499652833923,
71.4859437134095));
#129763=CARTESIAN_POINT('Ctrl Pts',(-10.6859519616658,-83.8677668236538,
71.0514043390162));
#129764=CARTESIAN_POINT('Ctrl Pts',(-10.6790221537907,-83.8100096489346,
70.8031104204124));
#129765=CARTESIAN_POINT('Ctrl Pts',(-10.6625254816767,-83.6480677969372,
70.2187496496713));
#129766=CARTESIAN_POINT('Ctrl Pts',(-10.6529601698758,-83.5345692708946,
69.8852398590506));
#129767=CARTESIAN_POINT('Ctrl Pts',(-10.6395386792417,-83.3435586958817,
69.416262784576));
#129768=CARTESIAN_POINT('Ctrl Pts',(-10.635484714546,-83.2814771857297,
69.2744458777196));
#129769=CARTESIAN_POINT('Ctrl Pts',(-10.6276706720216,-83.1526957541936,
69.0000729422436));
#129770=CARTESIAN_POINT('Ctrl Pts',(-10.6239043064502,-83.0863940754931,
68.8675296775701));
#129771=CARTESIAN_POINT('Ctrl Pts',(-10.6111042815369,-82.8490086757923,
68.420914084305));
#129772=CARTESIAN_POINT('Ctrl Pts',(-10.6021268483587,-82.6623278250407,
68.1151571826957));
#129773=CARTESIAN_POINT('Ctrl Pts',(-10.5867381875179,-82.326115834269,
67.630735462257));
#129774=CARTESIAN_POINT('Ctrl Pts',(-10.5805715462487,-82.1865607801452,
67.4451454461591));
#129775=CARTESIAN_POINT('Ctrl Pts',(-10.5650350745576,-81.8210906315581,
66.9956415649896));
#129776=CARTESIAN_POINT('Ctrl Pts',(-10.5555949762819,-81.5866782437081,
66.7385774415894));
#129777=CARTESIAN_POINT('Ctrl Pts',(-10.5385582191953,-81.1355374615621,
66.2972824871332));
#129778=CARTESIAN_POINT('Ctrl Pts',(-10.5309401020441,-80.9234004412554,
66.1083149121387));
#129779=CARTESIAN_POINT('Ctrl Pts',(-10.5185784955525,-80.558712438817,
65.8132329292415));
#129780=CARTESIAN_POINT('Ctrl Pts',(-10.5137593129423,-80.4110295335681,
65.7011238923676));
#129781=CARTESIAN_POINT('Ctrl Pts',(-10.5032278352579,-80.075827983657,
65.4628829634833));
#129782=CARTESIAN_POINT('Ctrl Pts',(-10.4975397088479,-79.8870655411617,
65.3392252239502));
#129783=CARTESIAN_POINT('Ctrl Pts',(-10.4863052237275,-79.5093908763208,
65.1115097278787));
#129784=CARTESIAN_POINT('Ctrl Pts',(-10.4807413503383,-79.3208662242744,
65.006831185423));
#129785=CARTESIAN_POINT('Ctrl Pts',(-10.4659000199624,-78.8168341624272,
64.7498478759028));
#129786=CARTESIAN_POINT('Ctrl Pts',(-10.4565068000018,-78.495612857664,
64.6086814206857));
#129787=CARTESIAN_POINT('Ctrl Pts',(-10.4328689875357,-77.6742738991775,
64.3024572344422));
#129788=CARTESIAN_POINT('Ctrl Pts',(-10.4185567360137,-77.1652267829833,
64.1609942365449));
#129789=CARTESIAN_POINT('Ctrl Pts',(-10.3998132013467,-76.4650161673287,
64.0310789897881));
#129790=CARTESIAN_POINT('Ctrl Pts',(-10.3949774604576,-76.2811265669053,
64.0028226988203));
#129791=CARTESIAN_POINT('Ctrl Pts',(-10.3854233122192,-75.9102533351739,
63.9577407002902));
#129792=CARTESIAN_POINT('Ctrl Pts',(-10.3807025242223,-75.7234889632973,
63.9410072019634));
#129793=CARTESIAN_POINT('Ctrl Pts',(-10.3598136559066,-74.8969357704687,
63.8928675879046));
#129794=CARTESIAN_POINT('Ctrl Pts',(-10.3434208244558,-74.2534668802988,
63.9237836430573));
#129795=CARTESIAN_POINT('Ctrl Pts',(-10.3163511471999,-73.2248189217987,
64.0816982601024));
#129796=CARTESIAN_POINT('Ctrl Pts',(-10.3058317022822,-72.833207037268,
64.1683093390963));
#129797=CARTESIAN_POINT('Ctrl Pts',(-10.2868973273492,-72.1534178330174,
64.3666454477573));
#129798=CARTESIAN_POINT('Ctrl Pts',(-10.2785506208785,-71.8619117144815,
64.4680682443189));
#129799=CARTESIAN_POINT('Ctrl Pts',(-10.2634506828038,-71.3557661531558,
64.6744071121457));
#129800=CARTESIAN_POINT('Ctrl Pts',(-10.2567170220152,-71.1391476857274,
64.7730143965423));
#129801=CARTESIAN_POINT('Ctrl Pts',(-10.2405995625591,-70.6479643524153,
65.0204229195374));
#129802=CARTESIAN_POINT('Ctrl Pts',(-10.2311102067042,-70.376468234342,
65.1752660712453));
#129803=CARTESIAN_POINT('Ctrl Pts',(-10.2011100154883,-69.5562051963923,
65.7003104258447));
#129804=CARTESIAN_POINT('Ctrl Pts',(-10.1801506924231,-69.0372672770758,
66.1176270367454));
#129805=CARTESIAN_POINT('Ctrl Pts',(-10.1564941020868,-68.4598867081246,
66.6961827051763));
#129806=CARTESIAN_POINT('Ctrl Pts',(-10.152091703178,-68.3528454317604,
66.8091134944626));
#129807=CARTESIAN_POINT('Ctrl Pts',(-10.1457737775871,-68.1990347021608,
66.9800801024668));
#129808=CARTESIAN_POINT('Ctrl Pts',(-10.1437587930829,-68.1499490975946,
67.036025392201));
#129809=CARTESIAN_POINT('Ctrl Pts',(-10.1402109642241,-68.0633659894135,
67.1372354834832));
#129810=CARTESIAN_POINT('Ctrl Pts',(-10.1386658575816,-68.0256028272131,
67.18227159919));
#129811=CARTESIAN_POINT('Ctrl Pts',(-10.1352649287799,-67.9422968840066,
67.2836493022914));
#129812=CARTESIAN_POINT('Ctrl Pts',(-10.1334204988097,-67.8969890987286,
67.3401823061191));
#129813=CARTESIAN_POINT('Ctrl Pts',(-10.1274698000766,-67.7506851965573,
67.5273566676092));
#129814=CARTESIAN_POINT('Ctrl Pts',(-10.123488960456,-67.6526051050933,
67.660273810607));
#129815=CARTESIAN_POINT('Ctrl Pts',(-10.1114123720327,-67.3579075215302,
68.0834662666085));
#129816=CARTESIAN_POINT('Ctrl Pts',(-10.1037158808832,-67.1743297727036,
68.3828182585121));
#129817=CARTESIAN_POINT('Ctrl Pts',(-10.0961244884418,-67.0084911154305,
68.6916878272719));
#129818=CARTESIAN_POINT('Ctrl Pts',(-13.5675364833309,-81.8820510104931,
67.097620723923));
#129819=CARTESIAN_POINT('Ctrl Pts',(-13.5675364833309,-81.6920778341857,
66.8981047934654));
#129820=CARTESIAN_POINT('Ctrl Pts',(-13.5675364833309,-81.4931660627479,
66.7070837578721));
#129821=CARTESIAN_POINT('Ctrl Pts',(-13.5675364833309,-81.0810140826979,
66.3448797285691));
#129822=CARTESIAN_POINT('Ctrl Pts',(-13.5675364833309,-80.8678695555096,
66.1735119454469));
#129823=CARTESIAN_POINT('Ctrl Pts',(-13.5675364833309,-80.6476829122575,
66.0117865989301));
#129824=CARTESIAN_POINT('Ctrl Pts',(-13.6367975371279,-82.22637258748,78.478439844214));
#129825=CARTESIAN_POINT('Ctrl Pts',(-13.5965727996549,-83.15132333764,77.260846746689));
#129826=CARTESIAN_POINT('Ctrl Pts',(-13.5161233247074,-84.37134578258,74.349656820311));
#129827=CARTESIAN_POINT('Ctrl Pts',(-13.3954491122865,-83.85839097116,69.641309155131));
#129828=CARTESIAN_POINT('Ctrl Pts',(-13.2747748998656,-81.12957508313,65.770566029046));
#129829=CARTESIAN_POINT('Ctrl Pts',(-13.1541006874447,-76.867728622,63.705144460549));
#129830=CARTESIAN_POINT('Ctrl Pts',(-13.0334264750238,-72.13871802361,63.961747337343));
#129831=CARTESIAN_POINT('Ctrl Pts',(-12.9127522626029,-68.12536086466,66.476164874831));
#129832=CARTESIAN_POINT('Ctrl Pts',(-12.7920780501819,-65.83145073401,70.619512225841));
#129833=CARTESIAN_POINT('Ctrl Pts',(-12.6714038377609,-65.83072989138,75.355475184308));
#129834=CARTESIAN_POINT('Ctrl Pts',(-12.5507296253399,-68.12337819702,79.499520367103));
#129835=CARTESIAN_POINT('Ctrl Pts',(-12.4300554129189,-72.13597072448,82.015161004986));
#129836=CARTESIAN_POINT('Ctrl Pts',(-12.3093812004979,-76.86489906758,82.273198436157));
#129837=CARTESIAN_POINT('Ctrl Pts',(-12.1887069880768,-81.12738874216,80.209093695038));
#129838=CARTESIAN_POINT('Ctrl Pts',(-12.0680327756558,-83.857328421,76.339109722068));
#129839=CARTESIAN_POINT('Ctrl Pts',(-11.9473585632348,-84.37192006169,71.631186395751));
#129840=CARTESIAN_POINT('Ctrl Pts',(-11.8266843508137,-82.5424567304,67.262844545329));
#129841=CARTESIAN_POINT('Ctrl Pts',(-11.7060101383926,-78.82651409889,64.326670680903));
#129842=CARTESIAN_POINT('Ctrl Pts',(-11.5853359259716,-74.15350404259,63.557045046897));
#129843=CARTESIAN_POINT('Ctrl Pts',(-11.4646617135509,-69.69221506849,65.146462327629));
#129844=CARTESIAN_POINT('Ctrl Pts',(-11.3439875011299,-66.55848112866,68.697385897282));
#129845=CARTESIAN_POINT('Ctrl Pts',(-11.2233132887089,-65.53609514649,73.3216775732695));
#129846=CARTESIAN_POINT('Ctrl Pts',(-11.1026390762869,-66.88077088472,77.862734032643));
#129847=CARTESIAN_POINT('Ctrl Pts',(-10.9819648638659,-70.25618517554,81.184770299059));
#129848=CARTESIAN_POINT('Ctrl Pts',(-10.8612906514449,-74.81809728471,82.456896282854));
#129849=CARTESIAN_POINT('Ctrl Pts',(-10.7406164390239,-79.42550594423,81.360934525046));
#129850=CARTESIAN_POINT('Ctrl Pts',(-10.6199422266029,-82.92603048601,78.171001360235));
#129851=CARTESIAN_POINT('Ctrl Pts',(-10.4992680141819,-84.44413839523,73.6849452599873));
#129852=CARTESIAN_POINT('Ctrl Pts',(-10.3785938017609,-83.60012808368,69.02479742627));
#129853=CARTESIAN_POINT('Ctrl Pts',(-10.2579195893399,-80.60510074462,65.356119528941));
#129854=CARTESIAN_POINT('Ctrl Pts',(-10.1372453769189,-76.20814999546,63.596538435828));
#129855=CARTESIAN_POINT('Ctrl Pts',(-10.0165711644989,-71.50904302936,64.186014661069));
#129856=CARTESIAN_POINT('Ctrl Pts',(-9.89589695207791,-67.68300161261,66.977621268753));
#129857=CARTESIAN_POINT('Ctrl Pts',(-9.81544747712991,-66.35255094703,69.840029796558));
#129858=CARTESIAN_POINT('Ctrl Pts',(-9.77522273965691,-66.0753597154,71.343769089941));
#129859=CARTESIAN_POINT('Ctrl Pts',(-13.7234642037949,-82.22637258748,78.478439844214));
#129860=CARTESIAN_POINT('Ctrl Pts',(-13.6832394663209,-83.15132333764,77.260846746689));
#129861=CARTESIAN_POINT('Ctrl Pts',(-13.6027899913739,-84.37134578258,74.349656820311));
#129862=CARTESIAN_POINT('Ctrl Pts',(-13.4821157789532,-83.85839097116,69.641309155131));
#129863=CARTESIAN_POINT('Ctrl Pts',(-13.3614415665323,-81.12957508313,65.770566029046));
#129864=CARTESIAN_POINT('Ctrl Pts',(-13.2407673541114,-76.867728622,63.705144460549));
#129865=CARTESIAN_POINT('Ctrl Pts',(-13.1200931416905,-72.13871802361,63.961747337343));
#129866=CARTESIAN_POINT('Ctrl Pts',(-12.9994189292695,-68.12536086466,66.476164874831));
#129867=CARTESIAN_POINT('Ctrl Pts',(-12.8787447168486,-65.83145073401,70.619512225841));
#129868=CARTESIAN_POINT('Ctrl Pts',(-12.7580705044276,-65.83072989138,75.355475184308));
#129869=CARTESIAN_POINT('Ctrl Pts',(-12.6373962920066,-68.12337819702,79.499520367103));
#129870=CARTESIAN_POINT('Ctrl Pts',(-12.5167220795856,-72.13597072448,82.015161004986));
#129871=CARTESIAN_POINT('Ctrl Pts',(-12.3960478671645,-76.86489906758,82.273198436157));
#129872=CARTESIAN_POINT('Ctrl Pts',(-12.2753736547435,-81.12738874216,80.209093695038));
#129873=CARTESIAN_POINT('Ctrl Pts',(-12.1546994423225,-83.857328421,76.339109722068));
#129874=CARTESIAN_POINT('Ctrl Pts',(-12.0340252299014,-84.37192006169,71.631186395751));
#129875=CARTESIAN_POINT('Ctrl Pts',(-11.9133510174804,-82.5424567304,67.262844545329));
#129876=CARTESIAN_POINT('Ctrl Pts',(-11.7926768050593,-78.82651409889,64.326670680903));
#129877=CARTESIAN_POINT('Ctrl Pts',(-11.6720025926383,-74.15350404259,63.557045046897));
#129878=CARTESIAN_POINT('Ctrl Pts',(-11.5513283802169,-69.69221506849,65.146462327629));
#129879=CARTESIAN_POINT('Ctrl Pts',(-11.4306541677959,-66.55848112866,68.697385897282));
#129880=CARTESIAN_POINT('Ctrl Pts',(-11.3099799553749,-65.53609514649,73.3216775732695));
#129881=CARTESIAN_POINT('Ctrl Pts',(-11.1893057429539,-66.88077088472,77.862734032643));
#129882=CARTESIAN_POINT('Ctrl Pts',(-11.0686315305329,-70.25618517554,81.184770299059));
#129883=CARTESIAN_POINT('Ctrl Pts',(-10.9479573181119,-74.81809728471,82.456896282854));
#129884=CARTESIAN_POINT('Ctrl Pts',(-10.8272831056909,-79.42550594423,81.360934525046));
#129885=CARTESIAN_POINT('Ctrl Pts',(-10.7066088932699,-82.92603048601,78.171001360235));
#129886=CARTESIAN_POINT('Ctrl Pts',(-10.5859346808489,-84.44413839523,73.6849452599873));
#129887=CARTESIAN_POINT('Ctrl Pts',(-10.4652604684279,-83.60012808368,69.02479742627));
#129888=CARTESIAN_POINT('Ctrl Pts',(-10.3445862560069,-80.60510074462,65.356119528941));
#129889=CARTESIAN_POINT('Ctrl Pts',(-10.2239120435859,-76.20814999546,63.596538435828));
#129890=CARTESIAN_POINT('Ctrl Pts',(-10.1032378311649,-71.50904302936,64.186014661069));
#129891=CARTESIAN_POINT('Ctrl Pts',(-9.98256361874391,-67.68300161261,66.977621268753));
#129892=CARTESIAN_POINT('Ctrl Pts',(-9.90211414379691,-66.35255094703,69.840029796558));
#129893=CARTESIAN_POINT('Ctrl Pts',(-9.86188940632291,-66.0753597154,71.343769089941));
#129894=CARTESIAN_POINT('Ctrl Pts',(-13.8101308704619,-82.22637258748,78.478439844214));
#129895=CARTESIAN_POINT('Ctrl Pts',(-13.7699061329879,-83.15132333764,77.260846746689));
#129896=CARTESIAN_POINT('Ctrl Pts',(-13.6894566580409,-84.37134578258,74.349656820311));
#129897=CARTESIAN_POINT('Ctrl Pts',(-13.5687824456199,-83.85839097116,69.641309155131));
#129898=CARTESIAN_POINT('Ctrl Pts',(-13.448108233199,-81.12957508313,65.770566029046));
#129899=CARTESIAN_POINT('Ctrl Pts',(-13.3274340207781,-76.867728622,63.705144460549));
#129900=CARTESIAN_POINT('Ctrl Pts',(-13.2067598083571,-72.13871802361,63.961747337343));
#129901=CARTESIAN_POINT('Ctrl Pts',(-13.0860855959362,-68.12536086466,66.476164874831));
#129902=CARTESIAN_POINT('Ctrl Pts',(-12.9654113835152,-65.83145073401,70.619512225841));
#129903=CARTESIAN_POINT('Ctrl Pts',(-12.8447371710942,-65.83072989138,75.355475184308));
#129904=CARTESIAN_POINT('Ctrl Pts',(-12.7240629586732,-68.12337819702,79.499520367103));
#129905=CARTESIAN_POINT('Ctrl Pts',(-12.6033887462522,-72.13597072448,82.015161004986));
#129906=CARTESIAN_POINT('Ctrl Pts',(-12.4827145338312,-76.86489906758,82.273198436157));
#129907=CARTESIAN_POINT('Ctrl Pts',(-12.3620403214102,-81.12738874216,80.209093695038));
#129908=CARTESIAN_POINT('Ctrl Pts',(-12.2413661089891,-83.857328421,76.339109722068));
#129909=CARTESIAN_POINT('Ctrl Pts',(-12.1206918965681,-84.37192006169,71.631186395751));
#129910=CARTESIAN_POINT('Ctrl Pts',(-12.000017684147,-82.5424567304,67.262844545329));
#129911=CARTESIAN_POINT('Ctrl Pts',(-11.879343471726,-78.82651409889,64.326670680903));
#129912=CARTESIAN_POINT('Ctrl Pts',(-11.7586692593049,-74.15350404259,63.557045046897));
#129913=CARTESIAN_POINT('Ctrl Pts',(-11.6379950468839,-69.69221506849,65.146462327629));
#129914=CARTESIAN_POINT('Ctrl Pts',(-11.5173208344629,-66.55848112866,68.697385897282));
#129915=CARTESIAN_POINT('Ctrl Pts',(-11.3966466220419,-65.53609514649,73.3216775732695));
#129916=CARTESIAN_POINT('Ctrl Pts',(-11.2759724096209,-66.88077088472,77.862734032643));
#129917=CARTESIAN_POINT('Ctrl Pts',(-11.1552981971999,-70.25618517554,81.184770299059));
#129918=CARTESIAN_POINT('Ctrl Pts',(-11.0346239847789,-74.81809728471,82.456896282854));
#129919=CARTESIAN_POINT('Ctrl Pts',(-10.9139497723579,-79.42550594423,81.360934525046));
#129920=CARTESIAN_POINT('Ctrl Pts',(-10.7932755599369,-82.92603048601,78.171001360235));
#129921=CARTESIAN_POINT('Ctrl Pts',(-10.6726013475159,-84.44413839523,73.6849452599872));
#129922=CARTESIAN_POINT('Ctrl Pts',(-10.5519271350949,-83.60012808368,69.02479742627));
#129923=CARTESIAN_POINT('Ctrl Pts',(-10.4312529226739,-80.60510074462,65.356119528941));
#129924=CARTESIAN_POINT('Ctrl Pts',(-10.3105787102529,-76.20814999546,63.596538435828));
#129925=CARTESIAN_POINT('Ctrl Pts',(-10.1899044978319,-71.50904302936,64.186014661069));
#129926=CARTESIAN_POINT('Ctrl Pts',(-10.0692302854109,-67.68300161261,66.977621268753));
#129927=CARTESIAN_POINT('Ctrl Pts',(-9.98878081046391,-66.35255094703,69.840029796558));
#129928=CARTESIAN_POINT('Ctrl Pts',(-9.94855607298991,-66.0753597154,71.343769089941));
#129929=CARTESIAN_POINT('Ctrl Pts',(-13.8967975371279,-82.22637258748,78.478439844214));
#129930=CARTESIAN_POINT('Ctrl Pts',(-13.8565727996549,-83.15132333764,77.260846746689));
#129931=CARTESIAN_POINT('Ctrl Pts',(-13.7761233247079,-84.37134578258,74.349656820311));
#129932=CARTESIAN_POINT('Ctrl Pts',(-13.6554491122869,-83.85839097116,69.641309155131));
#129933=CARTESIAN_POINT('Ctrl Pts',(-13.5347748998657,-81.12957508313,65.770566029046));
#129934=CARTESIAN_POINT('Ctrl Pts',(-13.4141006874447,-76.867728622,63.705144460549));
#129935=CARTESIAN_POINT('Ctrl Pts',(-13.2934264750238,-72.13871802361,63.961747337343));
#129936=CARTESIAN_POINT('Ctrl Pts',(-13.1727522626029,-68.12536086466,66.476164874831));
#129937=CARTESIAN_POINT('Ctrl Pts',(-13.0520780501819,-65.83145073401,70.619512225841));
#129938=CARTESIAN_POINT('Ctrl Pts',(-12.9314038377609,-65.83072989138,75.355475184308));
#129939=CARTESIAN_POINT('Ctrl Pts',(-12.8107296253399,-68.12337819702,79.499520367103));
#129940=CARTESIAN_POINT('Ctrl Pts',(-12.6900554129189,-72.13597072448,82.015161004986));
#129941=CARTESIAN_POINT('Ctrl Pts',(-12.5693812004979,-76.86489906758,82.273198436157));
#129942=CARTESIAN_POINT('Ctrl Pts',(-12.4487069880768,-81.12738874216,80.209093695038));
#129943=CARTESIAN_POINT('Ctrl Pts',(-12.3280327756558,-83.857328421,76.339109722068));
#129944=CARTESIAN_POINT('Ctrl Pts',(-12.2073585632348,-84.37192006169,71.631186395751));
#129945=CARTESIAN_POINT('Ctrl Pts',(-12.0866843508137,-82.5424567304,67.262844545329));
#129946=CARTESIAN_POINT('Ctrl Pts',(-11.9660101383927,-78.82651409889,64.326670680903));
#129947=CARTESIAN_POINT('Ctrl Pts',(-11.8453359259716,-74.15350404259,63.557045046897));
#129948=CARTESIAN_POINT('Ctrl Pts',(-11.7246617135505,-69.69221506849,65.146462327629));
#129949=CARTESIAN_POINT('Ctrl Pts',(-11.6039875011295,-66.55848112866,68.697385897282));
#129950=CARTESIAN_POINT('Ctrl Pts',(-11.4833132887089,-65.53609514649,73.3216775732695));
#129951=CARTESIAN_POINT('Ctrl Pts',(-11.3626390762869,-66.88077088472,77.862734032643));
#129952=CARTESIAN_POINT('Ctrl Pts',(-11.2419648638659,-70.25618517554,81.184770299059));
#129953=CARTESIAN_POINT('Ctrl Pts',(-11.1212906514449,-74.81809728471,82.456896282854));
#129954=CARTESIAN_POINT('Ctrl Pts',(-11.0006164390239,-79.42550594423,81.360934525046));
#129955=CARTESIAN_POINT('Ctrl Pts',(-10.8799422266029,-82.92603048601,78.171001360235));
#129956=CARTESIAN_POINT('Ctrl Pts',(-10.7592680141819,-84.44413839523,73.6849452599872));
#129957=CARTESIAN_POINT('Ctrl Pts',(-10.6385938017609,-83.60012808368,69.02479742627));
#129958=CARTESIAN_POINT('Ctrl Pts',(-10.5179195893399,-80.60510074462,65.356119528941));
#129959=CARTESIAN_POINT('Ctrl Pts',(-10.3972453769189,-76.20814999546,63.596538435828));
#129960=CARTESIAN_POINT('Ctrl Pts',(-10.2765711644989,-71.50904302936,64.186014661069));
#129961=CARTESIAN_POINT('Ctrl Pts',(-10.1558969520779,-67.68300161261,66.977621268753));
#129962=CARTESIAN_POINT('Ctrl Pts',(-10.0754474771299,-66.35255094703,69.840029796558));
#129963=CARTESIAN_POINT('Ctrl Pts',(-10.0352227396569,-66.0753597154,71.343769089941));
#129964=CARTESIAN_POINT('Ctrl Pts',(-13.5675364833309,-83.5583138245559,
76.0030914693076));
#129965=CARTESIAN_POINT('Ctrl Pts',(-13.5675364833309,-83.8209811139739,
75.2587654320264));
#129966=CARTESIAN_POINT('Ctrl Pts',(-13.5675364833309,-83.9873332505196,
74.480716603791));
#129967=CARTESIAN_POINT('Ctrl Pts',(-13.5675364833309,-84.1078633043029,
72.8969024422775));
#129968=CARTESIAN_POINT('Ctrl Pts',(-13.5675364833309,-84.0638930649032,
72.0991602388659));
#129969=CARTESIAN_POINT('Ctrl Pts',(-13.5675364833309,-83.7739991701906,
70.5423334575277));
#129970=CARTESIAN_POINT('Ctrl Pts',(-13.5675364833309,-83.5285763798928,
69.785555327736));
#129971=CARTESIAN_POINT('Ctrl Pts',(-13.5675364833309,-82.8410434730265,
68.3550103187433));
#129972=CARTESIAN_POINT('Ctrl Pts',(-13.5675364833309,-82.4057128334609,
67.6879975203469));
#129973=CARTESIAN_POINT('Ctrl Pts',(-13.5675364833309,-81.8927835901898,
67.0877618837426));
#129974=CARTESIAN_POINT('Origin',(-13.5675364833309,-75.,72.98888938658));
#129975=CARTESIAN_POINT('Ctrl Pts',(20.4053531221886,-17.1864037180436,
115.724508184767));
#129976=CARTESIAN_POINT('Ctrl Pts',(22.6252113906833,-17.1864037180436,
115.358472943979));
#129977=CARTESIAN_POINT('Ctrl Pts',(27.063989861239,-16.2914328094368,114.626567868827));
#129978=CARTESIAN_POINT('Ctrl Pts',(32.7110101862275,-12.4690426124586,
113.707002820814));
#129979=CARTESIAN_POINT('Ctrl Pts',(36.4883533005745,-6.74813242015872,
113.117112310253));
#129980=CARTESIAN_POINT('Ctrl Pts',(37.8234383481741,1.42212630560579E-14,
112.957857790712));
#129981=CARTESIAN_POINT('Ctrl Pts',(36.5144005272245,6.74813242015874,113.264833473205));
#129982=CARTESIAN_POINT('Ctrl Pts',(32.7631046395276,12.4690426124586,114.002445146718));
#129983=CARTESIAN_POINT('Ctrl Pts',(27.1421315411891,16.2914328094368,115.069731357682));
#129984=CARTESIAN_POINT('Ctrl Pts',(20.5095420287887,17.633889172347,116.315392836574));
#129985=CARTESIAN_POINT('Ctrl Pts',(13.8769525163883,16.2914328094368,117.561054315465));
#129986=CARTESIAN_POINT('Ctrl Pts',(8.25597941804984,12.4690426124586,118.62834052643));
#129987=CARTESIAN_POINT('Ctrl Pts',(4.50468353035287,6.74813242015876,119.365952199943));
#129988=CARTESIAN_POINT('Ctrl Pts',(3.19564570940331,1.55535306856081E-14,
119.672927882436));
#129989=CARTESIAN_POINT('Ctrl Pts',(4.5307307570029,-6.74813242015873,119.513673362895));
#129990=CARTESIAN_POINT('Ctrl Pts',(8.30807387134991,-12.4690426124586,
118.923782852334));
#129991=CARTESIAN_POINT('Ctrl Pts',(13.9550941963384,-16.2914328094368,
118.004217804321));
#129992=CARTESIAN_POINT('Ctrl Pts',(20.6137309353888,-17.633889172347,116.906277488381));
#129993=CARTESIAN_POINT('Ctrl Pts',(27.2723676744393,-16.2914328094368,
115.808337172442));
#129994=CARTESIAN_POINT('Ctrl Pts',(32.9193879994278,-12.4690426124586,
114.888772124429));
#129995=CARTESIAN_POINT('Ctrl Pts',(36.6967311137748,-6.74813242015874,
114.298881613867));
#129996=CARTESIAN_POINT('Ctrl Pts',(38.0318161613744,7.55992490830693E-15,
114.139627094327));
#129997=CARTESIAN_POINT('Ctrl Pts',(36.7227783404248,6.74813242015876,114.446602776819));
#129998=CARTESIAN_POINT('Ctrl Pts',(32.9714824527279,12.4690426124586,115.184214450332));
#129999=CARTESIAN_POINT('Ctrl Pts',(27.3505093543894,16.2914328094368,116.251500661297));
#130000=CARTESIAN_POINT('Ctrl Pts',(20.717919841989,17.633889172347,117.497162140189));
#130001=CARTESIAN_POINT('Ctrl Pts',(14.0853303295886,16.2914328094368,118.74282361908));
#130002=CARTESIAN_POINT('Ctrl Pts',(8.46435723125011,12.4690426124586,119.810109830045));
#130003=CARTESIAN_POINT('Ctrl Pts',(4.71306134355316,6.74813242015877,120.547721503558));
#130004=CARTESIAN_POINT('Ctrl Pts',(3.4040235226036,2.04385119939587E-14,
120.85469718605));
#130005=CARTESIAN_POINT('Ctrl Pts',(4.73910857020318,-6.74813242015873,
120.69544266651));
#130006=CARTESIAN_POINT('Ctrl Pts',(8.51645168455017,-12.4690426124586,
120.105552155948));
#130007=CARTESIAN_POINT('Ctrl Pts',(14.1634720095387,-16.2914328094368,
119.185987107935));
#130008=CARTESIAN_POINT('Ctrl Pts',(20.8221087485891,-17.633889172347,118.088046791996));
#130009=CARTESIAN_POINT('Ctrl Pts',(27.4807454876395,-16.2914328094368,
116.990106476056));
#130010=CARTESIAN_POINT('Ctrl Pts',(33.1277658126281,-12.4690426124586,
116.070541428043));
#130011=CARTESIAN_POINT('Ctrl Pts',(36.905108926975,-6.74813242015875,115.480650917482));
#130012=CARTESIAN_POINT('Ctrl Pts',(38.2401939745746,4.89538964920655E-15,
115.321396397941));
#130013=CARTESIAN_POINT('Ctrl Pts',(36.9311561536251,6.74813242015876,115.628372080434));
#130014=CARTESIAN_POINT('Ctrl Pts',(33.1798602659281,12.4690426124586,116.365983753947));
#130015=CARTESIAN_POINT('Ctrl Pts',(27.5588871675897,16.2914328094368,117.433269964912));
#130016=CARTESIAN_POINT('Ctrl Pts',(20.9262976551893,17.633889172347,118.678931443803));
#130017=CARTESIAN_POINT('Ctrl Pts',(14.293708142789,16.2914328094368,119.924592922695));
#130018=CARTESIAN_POINT('Ctrl Pts',(8.67273504445038,12.4690426124586,120.991879133659));
#130019=CARTESIAN_POINT('Ctrl Pts',(4.92143915675344,6.74813242015876,121.729490807172));
#130020=CARTESIAN_POINT('Ctrl Pts',(3.61240133580388,7.9058287694167E-14,
122.036466489665));
#130021=CARTESIAN_POINT('Ctrl Pts',(4.94748638340347,-6.74813242015874,
121.877211970124));
#130022=CARTESIAN_POINT('Ctrl Pts',(8.72482949775044,-12.4690426124586,
121.287321459563));
#130023=CARTESIAN_POINT('Ctrl Pts',(14.371849822739,-16.2914328094368,120.36775641155));
#130024=CARTESIAN_POINT('Ctrl Pts',(21.0304865617894,-17.633889172347,119.26981609561));
#130025=CARTESIAN_POINT('Ctrl Pts',(27.6891233008398,-16.2914328094368,
118.171875779671));
#130026=CARTESIAN_POINT('Ctrl Pts',(33.3361436258284,-12.4690426124586,
117.252310731658));
#130027=CARTESIAN_POINT('Ctrl Pts',(37.1134867401753,-6.74813242015876,
116.662420221097));
#130028=CARTESIAN_POINT('Ctrl Pts',(38.4485717877749,5.33011135228634E-14,
116.503165701556));
#130029=CARTESIAN_POINT('Ctrl Pts',(37.1395339668254,6.74813242015874,116.810141384049));
#130030=CARTESIAN_POINT('Ctrl Pts',(33.3882380791284,12.4690426124586,117.547753057562));
#130031=CARTESIAN_POINT('Ctrl Pts',(27.7672649807899,16.2914328094368,118.615039268526));
#130032=CARTESIAN_POINT('Ctrl Pts',(21.1346754683896,17.633889172347,119.860700747418));
#130033=CARTESIAN_POINT('Ctrl Pts',(14.5020859559892,16.2914328094368,121.106362226309));
#130034=CARTESIAN_POINT('Ctrl Pts',(8.88111285765067,12.4690426124586,122.173648437274));
#130035=CARTESIAN_POINT('Ctrl Pts',(5.12981696995372,6.74813242015876,122.911260110787));
#130036=CARTESIAN_POINT('Ctrl Pts',(3.82077914900416,8.30550905828176E-14,
123.21823579328));
#130037=CARTESIAN_POINT('Ctrl Pts',(5.15586419660375,-6.74813242015874,
123.058981273739));
#130038=CARTESIAN_POINT('Ctrl Pts',(8.93320731095072,-12.4690426124585,
122.469090763178));
#130039=CARTESIAN_POINT('Ctrl Pts',(14.5802276359393,-16.2914328094368,
121.549525715165));
#130040=CARTESIAN_POINT('Ctrl Pts',(21.2388643749897,-17.633889172347,120.451585399225));
#130041=CARTESIAN_POINT('Ctrl Pts',(27.89750111404,-16.2914328094368,119.353645083286));
#130042=CARTESIAN_POINT('Ctrl Pts',(33.5445214390286,-12.4690426124586,
118.434080035273));
#130043=CARTESIAN_POINT('Ctrl Pts',(37.3218645533756,-6.74813242015877,
117.844189524711));
#130044=CARTESIAN_POINT('Ctrl Pts',(38.6569496009752,4.93043106342128E-14,
117.684935005171));
#130045=CARTESIAN_POINT('Ctrl Pts',(37.3479117800257,6.74813242015873,117.991910687663));
#130046=CARTESIAN_POINT('Ctrl Pts',(33.5966158923287,12.4690426124586,118.729522361176));
#130047=CARTESIAN_POINT('Ctrl Pts',(27.9756427939902,16.2914328094368,119.796808572141));
#130048=CARTESIAN_POINT('Ctrl Pts',(21.3430532815898,17.633889172347,121.042470051032));
#130049=CARTESIAN_POINT('Ctrl Pts',(14.7104637691895,16.2914328094368,122.288131529924));
#130050=CARTESIAN_POINT('Ctrl Pts',(9.08949067085095,12.4690426124586,123.355417740889));
#130051=CARTESIAN_POINT('Ctrl Pts',(5.33819478315401,6.74813242015877,124.093029414402));
#130052=CARTESIAN_POINT('Ctrl Pts',(4.02915696220445,8.70518934714681E-14,
124.400005096894));
#130053=CARTESIAN_POINT('Ctrl Pts',(5.36424200980403,-6.74813242015873,
124.240750577354));
#130054=CARTESIAN_POINT('Ctrl Pts',(9.141585124151,-12.4690426124585,123.650860066792));
#130055=CARTESIAN_POINT('Ctrl Pts',(14.7886054491396,-16.2914328094368,
122.731295018779));
#130056=CARTESIAN_POINT('Ctrl Pts',(21.4472421881899,-17.633889172347,121.63335470284));
#130057=CARTESIAN_POINT('Ctrl Pts',(26.7715870880817,-16.5604411124356,
120.755425308182));
#130058=CARTESIAN_POINT('Ctrl Pts',(29.5464702774019,-15.1257033979806,
120.301649134085));
#130059=CARTESIAN_POINT('Ctrl Pts',(30.3017625288241,-14.6570228943777,
120.178595667035));
#130060=CARTESIAN_POINT('Ctrl Pts',(20.311092103448,-16.2461987828381,115.189927382884));
#130061=CARTESIAN_POINT('Ctrl Pts',(22.4097475821195,-16.2461987828381,
114.84526346408));
#130062=CARTESIAN_POINT('Ctrl Pts',(26.6061717911932,-15.4001884409061,
114.156091984117));
#130063=CARTESIAN_POINT('Ctrl Pts',(31.9449768781284,-11.7869071527165,
113.290873598438));
#130064=CARTESIAN_POINT('Ctrl Pts',(35.5163879178765,-6.37896691532468,
112.737294468822));
#130065=CARTESIAN_POINT('Ctrl Pts',(36.7791478469962,1.33330846363577E-14,
112.590792819052));
#130066=CARTESIAN_POINT('Ctrl Pts',(35.5424351445265,6.3789669153247,112.885015631774));
#130067=CARTESIAN_POINT('Ctrl Pts',(31.9970713314284,11.7869071527165,113.586315924342));
#130068=CARTESIAN_POINT('Ctrl Pts',(26.6843134711433,15.4001884409061,114.599255472972));
#130069=CARTESIAN_POINT('Ctrl Pts',(20.4152810100481,16.6692039538042,115.780812034692));
#130070=CARTESIAN_POINT('Ctrl Pts',(14.146248548953,15.4001884409061,116.962368596411));
#130071=CARTESIAN_POINT('Ctrl Pts',(8.83349068866784,11.7869071527165,117.975308145042));
#130072=CARTESIAN_POINT('Ctrl Pts',(5.28812687556977,6.37896691532472,118.67660843761));
#130073=CARTESIAN_POINT('Ctrl Pts',(4.05141417310005,1.59976198954581E-14,
118.970831250331));
#130074=CARTESIAN_POINT('Ctrl Pts',(5.31417410221981,-6.37896691532469,
118.824329600562));
#130075=CARTESIAN_POINT('Ctrl Pts',(8.88558514196791,-11.7869071527165,
118.270750470945));
#130076=CARTESIAN_POINT('Ctrl Pts',(14.2243902289031,-15.4001884409061,
117.405532085267));
#130077=CARTESIAN_POINT('Ctrl Pts',(20.5194699166483,-16.6692039538041,
116.371696686499));
#130078=CARTESIAN_POINT('Ctrl Pts',(26.8145496043935,-15.4001884409061,
115.337861287731));
#130079=CARTESIAN_POINT('Ctrl Pts',(32.1533546913286,-11.7869071527165,
114.472642902053));
#130080=CARTESIAN_POINT('Ctrl Pts',(35.7247657310767,-6.3789669153247,113.919063772437));
#130081=CARTESIAN_POINT('Ctrl Pts',(36.9875256601965,7.55992490830693E-15,
113.772562122667));
#130082=CARTESIAN_POINT('Ctrl Pts',(35.7508129577268,6.37896691532472,114.066784935388));
#130083=CARTESIAN_POINT('Ctrl Pts',(32.2054491446287,11.7869071527165,114.768085227956));
#130084=CARTESIAN_POINT('Ctrl Pts',(26.8926912843436,15.4001884409061,115.781024776587));
#130085=CARTESIAN_POINT('Ctrl Pts',(20.6236588232484,16.6692039538042,116.962581338306));
#130086=CARTESIAN_POINT('Ctrl Pts',(14.3546263621533,15.4001884409061,118.144137900026));
#130087=CARTESIAN_POINT('Ctrl Pts',(9.04186850186811,11.7869071527165,119.157077448656));
#130088=CARTESIAN_POINT('Ctrl Pts',(5.49650468877006,6.37896691532473,119.858377741224));
#130089=CARTESIAN_POINT('Ctrl Pts',(4.25979198630033,2.04385119939587E-14,
120.152600553946));
#130090=CARTESIAN_POINT('Ctrl Pts',(5.52255191542009,-6.37896691532469,
120.006098904176));
#130091=CARTESIAN_POINT('Ctrl Pts',(9.09396295516817,-11.7869071527165,
119.45251977456));
#130092=CARTESIAN_POINT('Ctrl Pts',(14.4327680421034,-15.4001884409061,
118.587301388881));
#130093=CARTESIAN_POINT('Ctrl Pts',(20.7278477298486,-16.6692039538041,
117.553465990114));
#130094=CARTESIAN_POINT('Ctrl Pts',(27.0229274175937,-15.4001884409061,
116.519630591346));
#130095=CARTESIAN_POINT('Ctrl Pts',(32.3617325045289,-11.7869071527165,
115.654412205667));
#130096=CARTESIAN_POINT('Ctrl Pts',(35.933143544277,-6.3789669153247,115.100833076051));
#130097=CARTESIAN_POINT('Ctrl Pts',(37.1959034733968,5.33947885905661E-15,
114.954331426281));
#130098=CARTESIAN_POINT('Ctrl Pts',(35.9591907709271,6.37896691532471,115.248554239003));
#130099=CARTESIAN_POINT('Ctrl Pts',(32.413826957829,11.7869071527165,115.949854531571));
#130100=CARTESIAN_POINT('Ctrl Pts',(27.1010690975439,15.4001884409061,116.962794080202));
#130101=CARTESIAN_POINT('Ctrl Pts',(20.8320366364487,16.6692039538041,118.144350641921));
#130102=CARTESIAN_POINT('Ctrl Pts',(14.5630041753536,15.4001884409062,119.325907203641));
#130103=CARTESIAN_POINT('Ctrl Pts',(9.25024631506838,11.7869071527165,120.338846752271));
#130104=CARTESIAN_POINT('Ctrl Pts',(5.70488250197034,6.37896691532472,121.040147044839));
#130105=CARTESIAN_POINT('Ctrl Pts',(4.46816979950061,7.50614848055164E-14,
121.334369857561));
#130106=CARTESIAN_POINT('Ctrl Pts',(5.73092972862037,-6.3789669153247,121.187868207791));
#130107=CARTESIAN_POINT('Ctrl Pts',(9.30234076836844,-11.7869071527165,
120.634289078175));
#130108=CARTESIAN_POINT('Ctrl Pts',(14.6411458553037,-15.4001884409061,
119.769070692496));
#130109=CARTESIAN_POINT('Ctrl Pts',(20.9362255430488,-16.6692039538041,
118.735235293728));
#130110=CARTESIAN_POINT('Ctrl Pts',(27.231305230794,-15.4001884409061,117.701399894961));
#130111=CARTESIAN_POINT('Ctrl Pts',(32.5701103177292,-11.7869071527165,
116.836181509282));
#130112=CARTESIAN_POINT('Ctrl Pts',(36.1415213574773,-6.37896691532472,
116.282602379666));
#130113=CARTESIAN_POINT('Ctrl Pts',(37.4042812865971,5.15247566834631E-14,
116.136100729896));
#130114=CARTESIAN_POINT('Ctrl Pts',(36.1675685841274,6.3789669153247,116.430323542618));
#130115=CARTESIAN_POINT('Ctrl Pts',(32.6222047710293,11.7869071527165,117.131623835186));
#130116=CARTESIAN_POINT('Ctrl Pts',(27.3094469107441,15.4001884409062,118.144563383816));
#130117=CARTESIAN_POINT('Ctrl Pts',(21.040414449649,16.6692039538041,119.326119945536));
#130118=CARTESIAN_POINT('Ctrl Pts',(14.7713819885539,15.4001884409062,120.507676507255));
#130119=CARTESIAN_POINT('Ctrl Pts',(9.45862412826867,11.7869071527165,121.520616055886));
#130120=CARTESIAN_POINT('Ctrl Pts',(5.91326031517062,6.37896691532472,122.221916348454));
#130121=CARTESIAN_POINT('Ctrl Pts',(4.6765476127009,7.9058287694167E-14,
122.516139161175));
#130122=CARTESIAN_POINT('Ctrl Pts',(5.93930754182065,-6.37896691532469,
122.369637511406));
#130123=CARTESIAN_POINT('Ctrl Pts',(9.51071858156872,-11.7869071527165,
121.816058381789));
#130124=CARTESIAN_POINT('Ctrl Pts',(14.849523668504,-15.4001884409061,120.950839996111));
#130125=CARTESIAN_POINT('Ctrl Pts',(21.1446033562491,-16.6692039538041,
119.917004597343));
#130126=CARTESIAN_POINT('Ctrl Pts',(27.4396830439942,-15.4001884409061,
118.883169198575));
#130127=CARTESIAN_POINT('Ctrl Pts',(32.7784881309295,-11.7869071527165,
118.017950812897));
#130128=CARTESIAN_POINT('Ctrl Pts',(36.3498991706776,-6.37896691532472,
117.464371683281));
#130129=CARTESIAN_POINT('Ctrl Pts',(37.6126590997973,4.70838645849625E-14,
117.317870033511));
#130130=CARTESIAN_POINT('Ctrl Pts',(36.3759463973276,6.37896691532469,117.612092846232));
#130131=CARTESIAN_POINT('Ctrl Pts',(32.8305825842296,11.7869071527165,118.3133931388));
#130132=CARTESIAN_POINT('Ctrl Pts',(27.5178247239444,15.4001884409062,119.326332687431));
#130133=CARTESIAN_POINT('Ctrl Pts',(21.2487922628493,16.6692039538041,120.50788924915));
#130134=CARTESIAN_POINT('Ctrl Pts',(14.9797598017542,15.4001884409062,121.68944581087));
#130135=CARTESIAN_POINT('Ctrl Pts',(9.66700194146895,11.7869071527165,122.7023853595));
#130136=CARTESIAN_POINT('Ctrl Pts',(6.12163812837091,6.37896691532473,123.403685652068));
#130137=CARTESIAN_POINT('Ctrl Pts',(4.88492542590118,8.26110013729675E-14,
123.69790846479));
#130138=CARTESIAN_POINT('Ctrl Pts',(6.14768535502093,-6.37896691532469,
123.55140681502));
#130139=CARTESIAN_POINT('Ctrl Pts',(9.719096394769,-11.7869071527165,122.997827685404));
#130140=CARTESIAN_POINT('Ctrl Pts',(15.0579014817043,-15.4001884409061,
122.132609299725));
#130141=CARTESIAN_POINT('Ctrl Pts',(21.3529811694494,-16.6692039538041,
121.098773900958));
#130142=CARTESIAN_POINT('Ctrl Pts',(26.3866204477858,-15.6544802890701,
120.272103750824));
#130143=CARTESIAN_POINT('Ctrl Pts',(29.0100321973966,-14.2982317979562,
119.845036078354));
#130144=CARTESIAN_POINT('Ctrl Pts',(29.7240999098662,-13.8551910808817,
119.729251609789));
#130145=CARTESIAN_POINT('',(29.803853834021,-13.9658945114651,119.791289468368));
#130146=CARTESIAN_POINT('Ctrl Pts',(20.5130133806899,-16.2461987828381,
116.335079851501));
#130147=CARTESIAN_POINT('Ctrl Pts',(22.6116688593615,-16.2461987828381,
115.990415932697));
#130148=CARTESIAN_POINT('Ctrl Pts',(26.8080930684351,-15.4001884409061,
115.301244452733));
#130149=CARTESIAN_POINT('Ctrl Pts',(32.1468981553703,-11.7869071527165,
114.436026067055));
#130150=CARTESIAN_POINT('Ctrl Pts',(35.7183091951184,-6.37896691532468,
113.882446937438));
#130151=CARTESIAN_POINT('Ctrl Pts',(36.9810691242382,1.33330846363577E-14,
113.735945287669));
#130152=CARTESIAN_POINT('Ctrl Pts',(35.7443564217685,6.3789669153247,114.03016810039));
#130153=CARTESIAN_POINT('Ctrl Pts',(32.1989926086704,11.7869071527165,114.731468392958));
#130154=CARTESIAN_POINT('Ctrl Pts',(26.8862347483852,15.4001884409061,115.744407941589));
#130155=CARTESIAN_POINT('Ctrl Pts',(20.6172022872901,16.6692039538042,116.925964503308));
#130156=CARTESIAN_POINT('Ctrl Pts',(14.348169826195,15.4001884409061,118.107521065028));
#130157=CARTESIAN_POINT('Ctrl Pts',(9.03541196590979,11.7869071527165,119.120460613658));
#130158=CARTESIAN_POINT('Ctrl Pts',(5.49004815281173,6.37896691532472,119.821760906226));
#130159=CARTESIAN_POINT('Ctrl Pts',(4.253335450342,1.59976198954581E-14,
120.115983718948));
#130160=CARTESIAN_POINT('Ctrl Pts',(5.51609537946176,-6.37896691532469,
119.969482069178));
#130161=CARTESIAN_POINT('Ctrl Pts',(9.08750641920986,-11.7869071527165,
119.415902939562));
#130162=CARTESIAN_POINT('Ctrl Pts',(14.426311506145,-15.4001884409061,118.550684553883));
#130163=CARTESIAN_POINT('Ctrl Pts',(20.7213911938902,-16.6692039538041,
117.516849155116));
#130164=CARTESIAN_POINT('Ctrl Pts',(27.0164708816354,-15.4001884409061,
116.483013756348));
#130165=CARTESIAN_POINT('Ctrl Pts',(32.3552759685706,-11.7869071527165,
115.617795370669));
#130166=CARTESIAN_POINT('Ctrl Pts',(35.9266870083187,-6.3789669153247,115.064216241053));
#130167=CARTESIAN_POINT('Ctrl Pts',(37.1894469374384,7.55992490830693E-15,
114.917714591283));
#130168=CARTESIAN_POINT('Ctrl Pts',(35.9527342349687,6.37896691532472,115.211937404005));
#130169=CARTESIAN_POINT('Ctrl Pts',(32.4073704218707,11.7869071527165,115.913237696573));
#130170=CARTESIAN_POINT('Ctrl Pts',(27.0946125615855,15.4001884409061,116.926177245203));
#130171=CARTESIAN_POINT('Ctrl Pts',(20.8255801004904,16.6692039538042,118.107733806923));
#130172=CARTESIAN_POINT('Ctrl Pts',(14.5565476393952,15.4001884409061,119.289290368642));
#130173=CARTESIAN_POINT('Ctrl Pts',(9.24378977911006,11.7869071527165,120.302229917273));
#130174=CARTESIAN_POINT('Ctrl Pts',(5.69842596601202,6.37896691532473,121.003530209841));
#130175=CARTESIAN_POINT('Ctrl Pts',(4.46171326354229,2.04385119939587E-14,
121.297753022563));
#130176=CARTESIAN_POINT('Ctrl Pts',(5.72447319266205,-6.37896691532469,
121.151251372793));
#130177=CARTESIAN_POINT('Ctrl Pts',(9.29588423241012,-11.7869071527165,
120.597672243177));
#130178=CARTESIAN_POINT('Ctrl Pts',(14.6346893193453,-15.4001884409061,
119.732453857498));
#130179=CARTESIAN_POINT('Ctrl Pts',(20.9297690070905,-16.6692039538041,
118.69861845873));
#130180=CARTESIAN_POINT('Ctrl Pts',(27.2248486948357,-15.4001884409061,
117.664783059963));
#130181=CARTESIAN_POINT('Ctrl Pts',(32.5636537817709,-11.7869071527165,
116.799564674284));
#130182=CARTESIAN_POINT('Ctrl Pts',(36.135064821519,-6.3789669153247,116.245985544668));
#130183=CARTESIAN_POINT('Ctrl Pts',(37.3978247506387,5.33947885905661E-15,
116.099483894898));
#130184=CARTESIAN_POINT('Ctrl Pts',(36.161112048169,6.37896691532471,116.39370670762));
#130185=CARTESIAN_POINT('Ctrl Pts',(32.615748235071,11.7869071527165,117.095007000188));
#130186=CARTESIAN_POINT('Ctrl Pts',(27.3029903747858,15.4001884409061,118.107946548818));
#130187=CARTESIAN_POINT('Ctrl Pts',(21.0339579136907,16.6692039538041,119.289503110538));
#130188=CARTESIAN_POINT('Ctrl Pts',(14.7649254525956,15.4001884409062,120.471059672257));
#130189=CARTESIAN_POINT('Ctrl Pts',(9.45216759231034,11.7869071527165,121.483999220888));
#130190=CARTESIAN_POINT('Ctrl Pts',(5.9068037792123,6.37896691532472,122.185299513456));
#130191=CARTESIAN_POINT('Ctrl Pts',(4.67009107674257,7.50614848055164E-14,
122.479522326177));
#130192=CARTESIAN_POINT('Ctrl Pts',(5.93285100586233,-6.3789669153247,122.333020676407));
#130193=CARTESIAN_POINT('Ctrl Pts',(9.50426204561039,-11.7869071527165,
121.779441546791));
#130194=CARTESIAN_POINT('Ctrl Pts',(14.8430671325457,-15.4001884409061,
120.914223161113));
#130195=CARTESIAN_POINT('Ctrl Pts',(21.1381468202908,-16.6692039538041,
119.880387762345));
#130196=CARTESIAN_POINT('Ctrl Pts',(27.4332265080359,-15.4001884409061,
118.846552363577));
#130197=CARTESIAN_POINT('Ctrl Pts',(32.7720315949712,-11.7869071527165,
117.981333977899));
#130198=CARTESIAN_POINT('Ctrl Pts',(36.3434426347193,-6.37896691532472,
117.427754848282));
#130199=CARTESIAN_POINT('Ctrl Pts',(37.606202563839,5.15247566834631E-14,
117.281253198513));
#130200=CARTESIAN_POINT('Ctrl Pts',(36.3694898613693,6.3789669153247,117.575476011234));
#130201=CARTESIAN_POINT('Ctrl Pts',(32.8241260482713,11.7869071527165,118.276776303802));
#130202=CARTESIAN_POINT('Ctrl Pts',(27.511368187986,15.4001884409062,119.289715852433));
#130203=CARTESIAN_POINT('Ctrl Pts',(21.242335726891,16.6692039538041,120.471272414152));
#130204=CARTESIAN_POINT('Ctrl Pts',(14.9733032657959,15.4001884409062,121.652828975872));
#130205=CARTESIAN_POINT('Ctrl Pts',(9.66054540551062,11.7869071527165,122.665768524502));
#130206=CARTESIAN_POINT('Ctrl Pts',(6.11518159241258,6.37896691532472,123.36706881707));
#130207=CARTESIAN_POINT('Ctrl Pts',(4.87846888994285,7.9058287694167E-14,
123.661291629792));
#130208=CARTESIAN_POINT('Ctrl Pts',(6.14122881906261,-6.37896691532469,
123.514789980022));
#130209=CARTESIAN_POINT('Ctrl Pts',(9.71263985881067,-11.7869071527165,
122.961210850406));
#130210=CARTESIAN_POINT('Ctrl Pts',(15.0514449457459,-15.4001884409061,
122.095992464727));
#130211=CARTESIAN_POINT('Ctrl Pts',(21.3465246334911,-16.6692039538041,
121.06215706596));
#130212=CARTESIAN_POINT('Ctrl Pts',(27.6416043212362,-15.4001884409061,
120.028321667192));
#130213=CARTESIAN_POINT('Ctrl Pts',(32.9804094081715,-11.7869071527165,
119.163103281513));
#130214=CARTESIAN_POINT('Ctrl Pts',(36.5518204479195,-6.37896691532472,
118.609524151897));
#130215=CARTESIAN_POINT('Ctrl Pts',(37.8145803770393,4.70838645849625E-14,
118.463022502127));
#130216=CARTESIAN_POINT('Ctrl Pts',(36.5778676745696,6.37896691532469,118.757245314849));
#130217=CARTESIAN_POINT('Ctrl Pts',(33.0325038614716,11.7869071527165,119.458545607417));
#130218=CARTESIAN_POINT('Ctrl Pts',(27.7197460011863,15.4001884409062,120.471485156047));
#130219=CARTESIAN_POINT('Ctrl Pts',(21.4507135400912,16.6692039538041,121.653041717767));
#130220=CARTESIAN_POINT('Ctrl Pts',(15.1816810789961,15.4001884409062,122.834598279486));
#130221=CARTESIAN_POINT('Ctrl Pts',(9.86892321871091,11.7869071527165,123.847537828117));
#130222=CARTESIAN_POINT('Ctrl Pts',(6.32355940561287,6.37896691532473,124.548838120685));
#130223=CARTESIAN_POINT('Ctrl Pts',(5.08684670314314,8.26110013729675E-14,
124.843060933407));
#130224=CARTESIAN_POINT('Ctrl Pts',(6.34960663226289,-6.37896691532469,
124.696559283637));
#130225=CARTESIAN_POINT('Ctrl Pts',(9.92101767201095,-11.7869071527165,
124.142980154021));
#130226=CARTESIAN_POINT('Ctrl Pts',(15.2598227589462,-15.4001884409061,
123.277761768342));
#130227=CARTESIAN_POINT('Ctrl Pts',(21.5549024466913,-16.6692039538041,
122.243926369574));
#130228=CARTESIAN_POINT('Ctrl Pts',(26.5885417250278,-15.6544802890701,
121.417256219441));
#130229=CARTESIAN_POINT('Ctrl Pts',(29.2119534746386,-14.2982317979562,
120.99018854697));
#130230=CARTESIAN_POINT('Ctrl Pts',(29.9260211871081,-13.8551910808817,
120.874404078406));
#130231=CARTESIAN_POINT('Ctrl Pts',(20.4187523619494,-17.1864037180436,
115.800499049619));
#130232=CARTESIAN_POINT('Ctrl Pts',(22.6386106304441,-17.1864037180436,
115.434463808832));
#130233=CARTESIAN_POINT('Ctrl Pts',(27.0773891009998,-16.2914328094368,
114.702558733679));
#130234=CARTESIAN_POINT('Ctrl Pts',(32.7244094259883,-12.4690426124586,
113.782993685666));
#130235=CARTESIAN_POINT('Ctrl Pts',(36.5017525403353,-6.74813242015872,
113.193103175105));
#130236=CARTESIAN_POINT('Ctrl Pts',(37.8368375879349,1.42212630560579E-14,
113.033848655564));
#130237=CARTESIAN_POINT('Ctrl Pts',(36.5277997669854,6.74813242015874,113.340824338057));
#130238=CARTESIAN_POINT('Ctrl Pts',(32.7765038792884,12.4690426124586,114.07843601157));
#130239=CARTESIAN_POINT('Ctrl Pts',(27.1555307809499,16.2914328094368,115.145722222535));
#130240=CARTESIAN_POINT('Ctrl Pts',(20.5229412685495,17.633889172347,116.391383701426));
#130241=CARTESIAN_POINT('Ctrl Pts',(13.8903517561492,16.2914328094368,117.637045180318));
#130242=CARTESIAN_POINT('Ctrl Pts',(8.26937865781067,12.4690426124586,118.704331391282));
#130243=CARTESIAN_POINT('Ctrl Pts',(4.5180827701137,6.74813242015876,119.441943064795));
#130244=CARTESIAN_POINT('Ctrl Pts',(3.20904494916414,1.55535306856081E-14,
119.748918747288));
#130245=CARTESIAN_POINT('Ctrl Pts',(4.54412999676373,-6.74813242015873,
119.589664227747));
#130246=CARTESIAN_POINT('Ctrl Pts',(8.32147311111074,-12.4690426124586,
118.999773717186));
#130247=CARTESIAN_POINT('Ctrl Pts',(13.9684934360992,-16.2914328094368,
118.080208669173));
#130248=CARTESIAN_POINT('Ctrl Pts',(20.6271301751497,-17.633889172347,116.982268353233));
#130249=CARTESIAN_POINT('Ctrl Pts',(27.2857669142001,-16.2914328094368,
115.884328037294));
#130250=CARTESIAN_POINT('Ctrl Pts',(32.9327872391886,-12.4690426124586,
114.964762989281));
#130251=CARTESIAN_POINT('Ctrl Pts',(36.7101303535356,-6.74813242015874,
114.37487247872));
#130252=CARTESIAN_POINT('Ctrl Pts',(38.0452154011352,7.55992490830693E-15,
114.215617959179));
#130253=CARTESIAN_POINT('Ctrl Pts',(36.7361775801856,6.74813242015876,114.522593641672));
#130254=CARTESIAN_POINT('Ctrl Pts',(32.9848816924887,12.4690426124586,115.260205315185));
#130255=CARTESIAN_POINT('Ctrl Pts',(27.3639085941502,16.2914328094368,116.327491526149));
#130256=CARTESIAN_POINT('Ctrl Pts',(20.7313190817498,17.633889172347,117.573153005041));
#130257=CARTESIAN_POINT('Ctrl Pts',(14.0987295693494,16.2914328094368,118.818814483932));
#130258=CARTESIAN_POINT('Ctrl Pts',(8.47775647101094,12.4690426124586,119.886100694897));
#130259=CARTESIAN_POINT('Ctrl Pts',(4.72646058331399,6.74813242015877,120.62371236841));
#130260=CARTESIAN_POINT('Ctrl Pts',(3.41742276236443,2.04385119939587E-14,
120.930688050903));
#130261=CARTESIAN_POINT('Ctrl Pts',(4.75250780996401,-6.74813242015873,
120.771433531362));
#130262=CARTESIAN_POINT('Ctrl Pts',(8.529850924311,-12.4690426124586,120.181543020801));
#130263=CARTESIAN_POINT('Ctrl Pts',(14.1768712492995,-16.2914328094368,
119.261977972788));
#130264=CARTESIAN_POINT('Ctrl Pts',(20.8355079883499,-17.633889172347,118.164037656848));
#130265=CARTESIAN_POINT('Ctrl Pts',(27.4941447274004,-16.2914328094368,
117.066097340909));
#130266=CARTESIAN_POINT('Ctrl Pts',(33.1411650523889,-12.4690426124586,
116.146532292896));
#130267=CARTESIAN_POINT('Ctrl Pts',(36.9185081667359,-6.74813242015875,
115.556641782334));
#130268=CARTESIAN_POINT('Ctrl Pts',(38.2535932143355,4.89538964920655E-15,
115.397387262794));
#130269=CARTESIAN_POINT('Ctrl Pts',(36.9445553933859,6.74813242015876,115.704362945286));
#130270=CARTESIAN_POINT('Ctrl Pts',(33.193259505689,12.4690426124586,116.441974618799));
#130271=CARTESIAN_POINT('Ctrl Pts',(27.5722864073505,16.2914328094368,117.509260829764));
#130272=CARTESIAN_POINT('Ctrl Pts',(20.9396968949501,17.633889172347,118.754922308655));
#130273=CARTESIAN_POINT('Ctrl Pts',(14.3071073825498,16.2914328094368,120.000583787547));
#130274=CARTESIAN_POINT('Ctrl Pts',(8.68613428421121,12.4690426124586,121.067869998512));
#130275=CARTESIAN_POINT('Ctrl Pts',(4.93483839651427,6.74813242015876,121.805481672025));
#130276=CARTESIAN_POINT('Ctrl Pts',(3.62580057556471,7.9058287694167E-14,
122.112457354517));
#130277=CARTESIAN_POINT('Ctrl Pts',(4.9608856231643,-6.74813242015874,121.953202834977));
#130278=CARTESIAN_POINT('Ctrl Pts',(8.73822873751127,-12.4690426124586,
121.363312324415));
#130279=CARTESIAN_POINT('Ctrl Pts',(14.3852490624999,-16.2914328094368,
120.443747276402));
#130280=CARTESIAN_POINT('Ctrl Pts',(21.0438858015502,-17.633889172347,119.345806960463));
#130281=CARTESIAN_POINT('Ctrl Pts',(27.7025225406006,-16.2914328094368,
118.247866644523));
#130282=CARTESIAN_POINT('Ctrl Pts',(33.3495428655892,-12.4690426124586,
117.32830159651));
#130283=CARTESIAN_POINT('Ctrl Pts',(37.1268859799362,-6.74813242015876,
116.738411085949));
#130284=CARTESIAN_POINT('Ctrl Pts',(38.4619710275358,5.33011135228634E-14,
116.579156566408));
#130285=CARTESIAN_POINT('Ctrl Pts',(37.1529332065862,6.74813242015874,116.886132248901));
#130286=CARTESIAN_POINT('Ctrl Pts',(33.4016373188893,12.4690426124586,117.623743922414));
#130287=CARTESIAN_POINT('Ctrl Pts',(27.7806642205507,16.2914328094368,118.691030133379));
#130288=CARTESIAN_POINT('Ctrl Pts',(21.1480747081504,17.633889172347,119.93669161227));
#130289=CARTESIAN_POINT('Ctrl Pts',(14.5154851957501,16.2914328094368,121.182353091162));
#130290=CARTESIAN_POINT('Ctrl Pts',(8.8945120974115,12.4690426124586,122.249639302126));
#130291=CARTESIAN_POINT('Ctrl Pts',(5.14321620971455,6.74813242015876,122.987250975639));
#130292=CARTESIAN_POINT('Ctrl Pts',(3.83417838876499,8.30550905828176E-14,
123.294226658132));
#130293=CARTESIAN_POINT('Ctrl Pts',(5.16926343636458,-6.74813242015874,
123.134972138591));
#130294=CARTESIAN_POINT('Ctrl Pts',(8.94660655071155,-12.4690426124585,
122.54508162803));
#130295=CARTESIAN_POINT('Ctrl Pts',(14.5936268757001,-16.2914328094368,
121.625516580017));
#130296=CARTESIAN_POINT('Ctrl Pts',(21.2522636147505,-17.633889172347,120.527576264077));
#130297=CARTESIAN_POINT('Ctrl Pts',(27.9109003538009,-16.2914328094368,
119.429635948138));
#130298=CARTESIAN_POINT('Ctrl Pts',(33.5579206787895,-12.4690426124586,
118.510070900125));
#130299=CARTESIAN_POINT('Ctrl Pts',(37.3352637931364,-6.74813242015877,
117.920180389564));
#130300=CARTESIAN_POINT('Ctrl Pts',(38.670348840736,4.93043106342128E-14,
117.760925870023));
#130301=CARTESIAN_POINT('Ctrl Pts',(37.3613110197865,6.74813242015873,118.067901552516));
#130302=CARTESIAN_POINT('Ctrl Pts',(33.6100151320896,12.4690426124586,118.805513226029));
#130303=CARTESIAN_POINT('Ctrl Pts',(27.989042033751,16.2914328094368,119.872799436993));
#130304=CARTESIAN_POINT('Ctrl Pts',(21.3564525213507,17.633889172347,121.118460915885));
#130305=CARTESIAN_POINT('Ctrl Pts',(14.7238630089504,16.2914328094368,122.364122394776));
#130306=CARTESIAN_POINT('Ctrl Pts',(9.10288991061178,12.4690426124586,123.431408605741));
#130307=CARTESIAN_POINT('Ctrl Pts',(5.35159402291484,6.74813242015877,124.169020279254));
#130308=CARTESIAN_POINT('Ctrl Pts',(4.04255620196528,8.70518934714681E-14,
124.475995961747));
#130309=CARTESIAN_POINT('Ctrl Pts',(5.37764124956486,-6.74813242015873,
124.316741442206));
#130310=CARTESIAN_POINT('Ctrl Pts',(9.15498436391183,-12.4690426124585,
123.726850931645));
#130311=CARTESIAN_POINT('Ctrl Pts',(14.8020046889004,-16.2914328094368,
122.807285883632));
#130312=CARTESIAN_POINT('Ctrl Pts',(21.4606414279508,-17.633889172347,121.709345567692));
#130313=CARTESIAN_POINT('Ctrl Pts',(26.7849863278426,-16.5604411124356,
120.831416173035));
#130314=CARTESIAN_POINT('Ctrl Pts',(29.5598695171627,-15.1257033979806,
120.377639998937));
#130315=CARTESIAN_POINT('Ctrl Pts',(30.315161768585,-14.6570228943777,120.254586531888));
#130316=CARTESIAN_POINT('',(30.2384437550856,-14.4989439202996,120.376781885352));
#130317=CARTESIAN_POINT('Origin',(29.8250605484872,-13.8551910808817,120.301827844097));
#130318=CARTESIAN_POINT('Origin',(22.6000197806719,1.4210854715202E-14,
128.171081305147));
#130319=CARTESIAN_POINT('Origin',(20.5162416486691,1.4210854715202E-14,
116.353388269));
#130320=CARTESIAN_POINT('Origin',(13.6416661832291,-6.,84.56419651818));
#130321=CARTESIAN_POINT('',(-5.0395856121756,-6.,84.304212101522));
#130322=CARTESIAN_POINT('',(-6.7204718626933,-5.99999999998125,84.6005928870242));
#130323=CARTESIAN_POINT('',(-0.312555071850913,-6.,83.47070907863));
#130324=CARTESIAN_POINT('',(-7.47066009951181,-6.,70.5169035593534));
#130325=CARTESIAN_POINT('',(-7.47066009951181,-6.,70.5169035593534));
#130326=CARTESIAN_POINT('',(22.1743288589254,-6.0000000159505,65.2896921631773));
#130327=CARTESIAN_POINT('',(10.6028230740595,-6.,67.3300608404729));
#130328=CARTESIAN_POINT('',(21.4524700019691,-6.,61.19591303503));
#130329=CARTESIAN_POINT('',(22.8689360308591,-6.00000009375099,69.228922547753));
#130330=CARTESIAN_POINT('',(21.7837557160991,-6.00001782727999,59.21971079975));
#130331=CARTESIAN_POINT('Origin',(24.4068932609991,-6.,60.67496850203));
#130332=CARTESIAN_POINT('',(-2.24980788089431,-5.99999999999387,55.9944999784261));
#130333=CARTESIAN_POINT('Origin',(1.07038457110909,-5.99999999998499,122.41156512159));
#130334=CARTESIAN_POINT('',(-6.16760615831108,-5.99999999999855,58.7310775215164));
#130335=CARTESIAN_POINT('Origin',(-2.02513312664091,-5.99999999999799,60.48888938658));
#130336=CARTESIAN_POINT('',(-7.28284231406048,-5.99999999998002,84.26262682962));
#130337=CARTESIAN_POINT('Origin',(27.4324635166691,-5.99999999999899,72.98888938658));
#130338=CARTESIAN_POINT('Origin',(-6.80729512863291,-5.99999999995499,84.10819367738));
#130339=CARTESIAN_POINT('Origin',(-9.10739291134991,6.,88.57546942229));
#130340=CARTESIAN_POINT('',(-7.47066009951181,6.,70.5169035593534));
#130341=CARTESIAN_POINT('',(22.1746244425332,5.99999996177058,65.2896400438122));
#130342=CARTESIAN_POINT('',(-12.1462360205204,6.,71.3413337445779));
#130343=CARTESIAN_POINT('',(-5.03958561217587,6.,84.3042121015204));
#130344=CARTESIAN_POINT('',(-7.47066009951181,6.,70.5169035593534));
#130345=CARTESIAN_POINT('',(-6.72047186372468,5.99999999998125,84.6005928811747));
#130346=CARTESIAN_POINT('',(-6.72047103979891,6.,84.60059755389));
#130347=CARTESIAN_POINT('',(-7.28284229737108,5.99999999998,84.2626268242002));
#130348=CARTESIAN_POINT('Origin',(-6.80729512863291,5.99999999995501,84.10819367738));
#130349=CARTESIAN_POINT('',(-6.16760614884715,5.99999999999856,58.7310775255325));
#130350=CARTESIAN_POINT('Origin',(27.4324635166691,5.99999999999901,72.98888938658));
#130351=CARTESIAN_POINT('',(-2.249807880305,5.99999999999389,55.9944999902141));
#130352=CARTESIAN_POINT('Origin',(-2.02513312664091,5.99999999999801,60.48888938658));
#130353=CARTESIAN_POINT('',(21.7835206002327,6.00000000005992,59.219661206118));
#130354=CARTESIAN_POINT('Origin',(1.07038457110909,5.99999999998501,122.41156512159));
#130355=CARTESIAN_POINT('',(21.4524700019691,6.,61.19591303503));
#130356=CARTESIAN_POINT('Origin',(24.4068932609991,6.,60.67496850203));
#130357=CARTESIAN_POINT('',(21.4524700019491,6.,61.1959130349));
#130358=CARTESIAN_POINT('Origin',(-8.75366715310791,111.0724296188,85.97453149762));
#130359=CARTESIAN_POINT('',(33.8591356989091,-12.92363696959,78.460761865691));
#130360=CARTESIAN_POINT('',(29.8285484048191,-12.92381593441,79.171454261306));
#130361=CARTESIAN_POINT('',(33.6423057253991,-11.63783768946,78.49897240947));
#130362=CARTESIAN_POINT('',(33.6423057253991,-11.63783768946,78.49897240947));
#130363=CARTESIAN_POINT('Origin',(36.7188322241242,-11.4176049647123,77.9561983041534));
#130364=CARTESIAN_POINT('Origin',(-8.75366715310791,111.0724296188,85.97453149762));
#130365=CARTESIAN_POINT('',(33.6423056644279,11.63783769022,78.498972064024));
#130366=CARTESIAN_POINT('',(33.6423057253991,-11.63783768946,78.49897240947));
#130367=CARTESIAN_POINT('',(33.8592119939158,12.9236986194734,78.4607301343571));
#130368=CARTESIAN_POINT('',(33.8592136711991,12.92369861938,78.460739645228));
#130369=CARTESIAN_POINT('Origin',(36.7134944496243,11.4180028254251,77.9569478528599));
#130370=CARTESIAN_POINT('Origin',(27.2132013147391,-12.92381190166,78.109462257321));
#130371=CARTESIAN_POINT('',(33.818257678174,-13.7317225406618,78.228144902818));
#130372=CARTESIAN_POINT('Origin',(33.5977564035364,-12.9238122378902,76.9836935245755));
#130373=CARTESIAN_POINT('',(33.6728408920201,-14.3619759694431,77.403275003416));
#130374=CARTESIAN_POINT('Origin',(33.5986100047126,-12.9238119282868,76.9835424355099));
#130375=CARTESIAN_POINT('',(29.6420890790991,-14.36196613703,78.113990728651));
#130376=CARTESIAN_POINT('',(29.6420897207604,-14.3619786049901,78.1139943676928));
#130377=CARTESIAN_POINT('Origin',(29.5680176896579,-12.9236693686975,77.6941105696628));
#130378=CARTESIAN_POINT('Ctrl Pts',(27.5244159794491,-12.80681735949,79.549155074551));
#130379=CARTESIAN_POINT('Ctrl Pts',(27.5827558822291,-12.79405706744,79.538099789147));
#130380=CARTESIAN_POINT('Ctrl Pts',(28.3905563838491,-12.62204439971,79.384761922452));
#130381=CARTESIAN_POINT('Ctrl Pts',(29.2129925125091,-12.51120733417,79.224589989218));
#130382=CARTESIAN_POINT('Ctrl Pts',(29.9816324828591,-12.46457130983,79.071054735497));
#130383=CARTESIAN_POINT('Ctrl Pts',(27.7070605433691,-13.81411105762,79.72010021776));
#130384=CARTESIAN_POINT('Ctrl Pts',(27.7619085286391,-13.80141862852,79.71237284821));
#130385=CARTESIAN_POINT('Ctrl Pts',(28.5216090046891,-13.62979474475,79.605264089276));
#130386=CARTESIAN_POINT('Ctrl Pts',(29.2985927528191,-13.51173676089,79.494180558665));
#130387=CARTESIAN_POINT('Ctrl Pts',(30.0268234514991,-13.45237632462,79.38633904926));
#130388=CARTESIAN_POINT('Ctrl Pts',(27.7062881845591,-14.59938920963,79.041460544841));
#130389=CARTESIAN_POINT('Ctrl Pts',(27.7587276207091,-14.58888856718,79.036271398538));
#130390=CARTESIAN_POINT('Ctrl Pts',(28.4849791691991,-14.44741116539,78.964587688416));
#130391=CARTESIAN_POINT('Ctrl Pts',(29.2264592716991,-14.35719351328,78.893669194586));
#130392=CARTESIAN_POINT('Ctrl Pts',(29.9188937984091,-14.31933226887,78.8260112440331));
#130393=CARTESIAN_POINT('Ctrl Pts',(27.5226758911191,-14.5760123706,78.020211577781));
#130394=CARTESIAN_POINT('Ctrl Pts',(27.5755894451791,-14.56819007155,78.014874790841));
#130395=CARTESIAN_POINT('Ctrl Pts',(28.3080310747691,-14.46409602014,77.941347905091));
#130396=CARTESIAN_POINT('Ctrl Pts',(29.0504791474991,-14.41598192215,77.871665924383));
#130397=CARTESIAN_POINT('Ctrl Pts',(29.7384720137891,-14.41778257326,77.808662352547));
#130398=CARTESIAN_POINT('Ctrl Pts',(28.583810069542,-14.4235289944163,78.2160017822117));
#130399=CARTESIAN_POINT('Ctrl Pts',(28.9401679712898,-14.3897216672816,
78.1843085059736));
#130400=CARTESIAN_POINT('Ctrl Pts',(29.2930910333242,-14.3696365833235,
78.1493275324345));
#130401=CARTESIAN_POINT('Ctrl Pts',(29.6420890790991,-14.36196613703,78.113990728651));
#130402=CARTESIAN_POINT('Origin',(26.6903689106391,-17.,82.263358164095));
#130403=CARTESIAN_POINT('',(23.6515258014693,-10.9473150473928,65.0292224863868));
#130404=CARTESIAN_POINT('',(23.6515258014716,-7.5,65.0292224863863));
#130405=CARTESIAN_POINT('',(23.6515258014693,-17.,65.0292224863868));
#130406=CARTESIAN_POINT('',(22.9355719200891,-10.33193324195,60.96884625134));
#130407=CARTESIAN_POINT('Ctrl Pts',(23.651525801475,-10.9473150473928,65.0292224863858));
#130408=CARTESIAN_POINT('Ctrl Pts',(23.649538794891,-10.9444282998633,65.0179536120707));
#130409=CARTESIAN_POINT('Ctrl Pts',(23.6475480201257,-10.9415421742228,
65.0066633673373));
#130410=CARTESIAN_POINT('Ctrl Pts',(23.645553440154,-10.9386567173531,64.9953515422064));
#130411=CARTESIAN_POINT('Ctrl Pts',(23.6193912182559,-10.9008091685076,
64.8469782087948));
#130412=CARTESIAN_POINT('Ctrl Pts',(23.5925742504193,-10.8631053140448,
64.6948916264451));
#130413=CARTESIAN_POINT('Ctrl Pts',(23.5650981559036,-10.8259116051253,
64.5390669507413));
#130414=CARTESIAN_POINT('Ctrl Pts',(23.5502223202996,-10.8057745547496,
64.4547018945107));
#130415=CARTESIAN_POINT('Ctrl Pts',(23.5351532379843,-10.7857878904675,
64.3692408817632));
#130416=CARTESIAN_POINT('Ctrl Pts',(23.5198899259623,-10.7660159568398,
64.2826783379113));
#130417=CARTESIAN_POINT('Ctrl Pts',(23.5026409053267,-10.7436717571888,
64.1848542809157));
#130418=CARTESIAN_POINT('Ctrl Pts',(23.4851438221287,-10.7216013585723,
64.0856233918126));
#130419=CARTESIAN_POINT('Ctrl Pts',(23.4673981473186,-10.6999293150683,
63.984982668886));
#130420=CARTESIAN_POINT('Ctrl Pts',(23.4445642071311,-10.6720431878624,
63.8554849590316));
#130421=CARTESIAN_POINT('Ctrl Pts',(23.4213212328658,-10.6447569234707,
63.7236675037941));
#130422=CARTESIAN_POINT('Ctrl Pts',(23.3978341137514,-10.61857549495,63.5904654234402));
#130423=CARTESIAN_POINT('Ctrl Pts',(23.3766359460333,-10.5949455933781,
63.4702446323763));
#130424=CARTESIAN_POINT('Ctrl Pts',(23.3552389149002,-10.5722162410661,
63.3488960207313));
#130425=CARTESIAN_POINT('Ctrl Pts',(23.3337672030354,-10.5507173831927,
63.2271238921102));
#130426=CARTESIAN_POINT('Ctrl Pts',(23.3314487146874,-10.5483959636529,
63.2139750913488));
#130427=CARTESIAN_POINT('Ctrl Pts',(23.3291293586053,-10.5460888432694,
63.2008213696401));
#130428=CARTESIAN_POINT('Ctrl Pts',(23.3268092933577,-10.5437964012374,
63.1876636262863));
#130429=CARTESIAN_POINT('Ctrl Pts',(23.309310409464,-10.5265058629688,63.0884225280079));
#130430=CARTESIAN_POINT('Ctrl Pts',(23.2917710596858,-10.5100526735849,
62.9889519597633));
#130431=CARTESIAN_POINT('Ctrl Pts',(23.2742619690445,-10.4946060514652,
62.8896529723304));
#130432=CARTESIAN_POINT('Ctrl Pts',(23.2578463446928,-10.4801240916984,
62.7965553403862));
#130433=CARTESIAN_POINT('Ctrl Pts',(23.2414572804221,-10.4664710978206,
62.7036083027852));
#130434=CARTESIAN_POINT('Ctrl Pts',(23.2252065308699,-10.4537748697727,
62.6114456888268));
#130435=CARTESIAN_POINT('Ctrl Pts',(23.2094400821371,-10.4414570115733,
62.5220296822983));
#130436=CARTESIAN_POINT('Ctrl Pts',(23.1938038426215,-10.430039913861,62.4333521317278));
#130437=CARTESIAN_POINT('Ctrl Pts',(23.1784012188369,-10.4195924205753,
62.3459995053294));
#130438=CARTESIAN_POINT('Ctrl Pts',(23.1629985950523,-10.4091449272895,
62.2586468789311));
#130439=CARTESIAN_POINT('Ctrl Pts',(23.1478295974388,-10.3996672586441,
62.1726192371723));
#130440=CARTESIAN_POINT('Ctrl Pts',(23.1329988176234,-10.3911763876647,
62.0885097389733));
#130441=CARTESIAN_POINT('Ctrl Pts',(23.1186007850307,-10.3829332717514,
62.0068544712464));
#130442=CARTESIAN_POINT('Ctrl Pts',(23.1045215897217,-10.375620358595,61.9270074349582));
#130443=CARTESIAN_POINT('Ctrl Pts',(23.0908595573615,-10.3692172844012,
61.8495262080312));
#130444=CARTESIAN_POINT('Ctrl Pts',(23.0896052918578,-10.368629439572,61.8424129156926));
#130445=CARTESIAN_POINT('Ctrl Pts',(23.0883545424879,-10.3680492269807,
61.8353195639691));
#130446=CARTESIAN_POINT('Ctrl Pts',(23.087107385374,-10.3674766089124,61.8282465845024));
#130447=CARTESIAN_POINT('Ctrl Pts',(23.0666311162332,-10.3580751617747,
61.7121198915922));
#130448=CARTESIAN_POINT('Ctrl Pts',(23.0471148480774,-10.3508869369945,
61.6014375750419));
#130449=CARTESIAN_POINT('Ctrl Pts',(23.0284541449167,-10.3455073057329,
61.4956074781716));
#130450=CARTESIAN_POINT('Ctrl Pts',(23.0103685575805,-10.3402934726752,
61.3930390249216));
#130451=CARTESIAN_POINT('Ctrl Pts',(22.993086486547,-10.3367775742029,61.2950275620653));
#130452=CARTESIAN_POINT('Ctrl Pts',(22.976507171293,-10.3346276973853,61.2010015992793));
#130453=CARTESIAN_POINT('Ctrl Pts',(22.9734133232253,-10.3342265112002,
61.1834555161736));
#130454=CARTESIAN_POINT('Ctrl Pts',(22.9703439336347,-10.3338730176223,
61.1660481433642));
#130455=CARTESIAN_POINT('Ctrl Pts',(22.9672983299519,-10.3335652372066,
61.1487756666496));
#130456=CARTESIAN_POINT('Ctrl Pts',(22.9564298118544,-10.3324668943601,
61.087137237848));
#130457=CARTESIAN_POINT('Ctrl Pts',(22.9458642968996,-10.3319499802198,
61.0272172190325));
#130458=CARTESIAN_POINT('Ctrl Pts',(22.9355719203965,-10.33193324195,60.9688462512858));
#130459=CARTESIAN_POINT('',(22.9355719200891,-10.33193324195,60.96884625134));
#130460=CARTESIAN_POINT('',(22.9296816314691,-7.5,60.93544076845));
#130461=CARTESIAN_POINT('',(22.9296817835391,-10.33198955295,60.93544163085));
#130462=CARTESIAN_POINT('',(24.8670630451391,-7.5,71.922876757467));
#130463=CARTESIAN_POINT('Ctrl Pts',(16.7315271092291,25.77957474242,75.8056538642681));
#130464=CARTESIAN_POINT('Ctrl Pts',(16.8902739491491,25.78276104928,76.726755143248));
#130465=CARTESIAN_POINT('Ctrl Pts',(17.4170423638691,25.68741378017,79.011155596728));
#130466=CARTESIAN_POINT('Ctrl Pts',(18.6971928491291,25.1486541372,82.327981456666));
#130467=CARTESIAN_POINT('Ctrl Pts',(20.3541926191191,24.21296098443,85.29757061493));
#130468=CARTESIAN_POINT('Ctrl Pts',(21.9876235905991,23.12636897321,87.62326197554));
#130469=CARTESIAN_POINT('Ctrl Pts',(23.5303110581191,21.96974605327,89.49482082956));
#130470=CARTESIAN_POINT('Ctrl Pts',(25.0147293345491,20.73535636643,91.08394632963));
#130471=CARTESIAN_POINT('Ctrl Pts',(26.4477039632491,19.42122041898,92.4661164628101));
#130472=CARTESIAN_POINT('Ctrl Pts',(27.8040593501691,18.0525443245,93.66246634875));
#130473=CARTESIAN_POINT('Ctrl Pts',(29.0976297887891,16.61722673478,94.7173081814599));
#130474=CARTESIAN_POINT('Ctrl Pts',(30.3859883571291,15.03805899871,95.692928827));
#130475=CARTESIAN_POINT('Ctrl Pts',(31.6846191544191,13.2490375268,96.6017522016999));
#130476=CARTESIAN_POINT('Ctrl Pts',(32.9283641549091,11.27078505501,97.39922069443));
#130477=CARTESIAN_POINT('Ctrl Pts',(34.0024905191591,9.24026551673301,98.0256740975701));
#130478=CARTESIAN_POINT('Ctrl Pts',(34.8835248980591,7.19980133487202,98.4916705583199));
#130479=CARTESIAN_POINT('Ctrl Pts',(35.5865206621291,5.09129120886101,98.8275149094299));
#130480=CARTESIAN_POINT('Ctrl Pts',(36.0644764908891,2.94897602587201,99.0360923986901));
#130481=CARTESIAN_POINT('Ctrl Pts',(36.2175390832591,1.50759720120401,99.1082321058299));
#130482=CARTESIAN_POINT('Ctrl Pts',(36.2511547877691,0.817200229439614,
99.1309346670101));
#130483=CARTESIAN_POINT('Ctrl Pts',(16.5657307648391,19.34436604072,75.8499470296021));
#130484=CARTESIAN_POINT('Ctrl Pts',(16.7027032210391,19.34727467235,76.647687526976));
#130485=CARTESIAN_POINT('Ctrl Pts',(17.1758927443291,19.26031994756,78.623309386718));
#130486=CARTESIAN_POINT('Ctrl Pts',(18.3744374416091,18.77127275203,81.451029832546));
#130487=CARTESIAN_POINT('Ctrl Pts',(19.9464727370091,17.9342387447,83.90371085737));
#130488=CARTESIAN_POINT('Ctrl Pts',(21.5011129654591,16.97934371574,85.75395997948));
#130489=CARTESIAN_POINT('Ctrl Pts',(22.9701058542891,15.98027083986,87.18714704112));
#130490=CARTESIAN_POINT('Ctrl Pts',(24.3829496628191,14.93205005415,88.35697360021));
#130491=CARTESIAN_POINT('Ctrl Pts',(25.7455828440791,13.83506997747,89.33304121868));
#130492=CARTESIAN_POINT('Ctrl Pts',(27.0338235509591,12.71200151814,90.14134599812));
#130493=CARTESIAN_POINT('Ctrl Pts',(28.2606989614091,11.55431815225,90.82076231519));
#130494=CARTESIAN_POINT('Ctrl Pts',(29.4805515038791,10.30341122855,91.41513380966));
#130495=CARTESIAN_POINT('Ctrl Pts',(30.7073346580191,8.91606547149402,91.92891446662));
#130496=CARTESIAN_POINT('Ctrl Pts',(31.8785519228191,7.42186252822301,92.33283454608));
#130497=CARTESIAN_POINT('Ctrl Pts',(32.8858034194691,5.93611159812901,92.60136415471));
#130498=CARTESIAN_POINT('Ctrl Pts',(33.7077479385191,4.49637949617201,92.75525280737));
#130499=CARTESIAN_POINT('Ctrl Pts',(34.3594477230791,3.06936714330901,92.82352537927));
#130500=CARTESIAN_POINT('Ctrl Pts',(34.7987841186091,1.68933111557601,92.83289655037));
#130501=CARTESIAN_POINT('Ctrl Pts',(34.9379185776691,0.799874261541514,
92.83329103801));
#130502=CARTESIAN_POINT('Ctrl Pts',(34.9680789093591,0.377412282680914,
92.8379453280101));
#130503=CARTESIAN_POINT('Ctrl Pts',(21.0648245475691,14.80356751578,75.088574197736));
#130504=CARTESIAN_POINT('Ctrl Pts',(21.1562893009191,14.80542149402,75.624814594272));
#130505=CARTESIAN_POINT('Ctrl Pts',(21.4915191590391,14.74994267437,76.949273101324));
#130506=CARTESIAN_POINT('Ctrl Pts',(22.4029329257891,14.43645292234,78.850401178621));
#130507=CARTESIAN_POINT('Ctrl Pts',(23.6728411634791,13.89196197301,80.525093828825));
#130508=CARTESIAN_POINT('Ctrl Pts',(24.9938756020691,13.25961078348,81.813737319686));
#130509=CARTESIAN_POINT('Ctrl Pts',(26.2936708744891,12.5864534242,82.832583999374));
#130510=CARTESIAN_POINT('Ctrl Pts',(27.5870975206191,11.86798256843,83.68225710374));
#130511=CARTESIAN_POINT('Ctrl Pts',(28.8717832775691,11.10303997034,84.4077907698501));
#130512=CARTESIAN_POINT('Ctrl Pts',(30.1179515221891,10.306293006,85.0241310085501));
#130513=CARTESIAN_POINT('Ctrl Pts',(31.3323143284891,9.47069299188402,85.55730149859));
#130514=CARTESIAN_POINT('Ctrl Pts',(32.5667384548491,8.55128051724301,86.04034306038));
#130515=CARTESIAN_POINT('Ctrl Pts',(33.8387497469191,7.50960072681501,86.47900335892));
#130516=CARTESIAN_POINT('Ctrl Pts',(35.0880429676691,6.35762147075602,86.85127259704));
#130517=CARTESIAN_POINT('Ctrl Pts',(36.1977391360291,5.17506491544101,87.13119140558));
#130518=CARTESIAN_POINT('Ctrl Pts',(37.1355508905091,3.98655984369701,87.32815521361));
#130519=CARTESIAN_POINT('Ctrl Pts',(37.9083300473991,2.75824145710901,87.46012871543));
#130520=CARTESIAN_POINT('Ctrl Pts',(38.4524854874891,1.51002426311401,87.5351100622101));
#130521=CARTESIAN_POINT('Ctrl Pts',(38.6303209632591,0.670091817760814,
87.56162468684));
#130522=CARTESIAN_POINT('Ctrl Pts',(38.6686985395891,0.267767345835414,
87.57156379687));
#130523=CARTESIAN_POINT('Ctrl Pts',(27.4060955579191,15.00605745049,73.9992175459301));
#130524=CARTESIAN_POINT('Ctrl Pts',(27.4568706345291,15.00674148237,74.299882608077));
#130525=CARTESIAN_POINT('Ctrl Pts',(27.6563153791591,14.98607407549,75.03933020766));
#130526=CARTESIAN_POINT('Ctrl Pts',(28.2552178354491,14.86384274642,76.157719195735));
#130527=CARTESIAN_POINT('Ctrl Pts',(29.1953897033191,14.62223845856,77.28144993045));
#130528=CARTESIAN_POINT('Ctrl Pts',(30.2745666151391,14.3009152899,78.274673456111));
#130529=CARTESIAN_POINT('Ctrl Pts',(31.4158151207291,13.9175608677,79.163166612491));
#130530=CARTESIAN_POINT('Ctrl Pts',(32.6169037455491,13.46553722345,79.992694706598));
#130531=CARTESIAN_POINT('Ctrl Pts',(33.8649399941491,12.93919476597,80.780446952018));
#130532=CARTESIAN_POINT('Ctrl Pts',(35.1214740837291,12.3447503952,81.5213409775531));
#130533=CARTESIAN_POINT('Ctrl Pts',(36.3853570661891,11.67360909312,82.229199358404));
#130534=CARTESIAN_POINT('Ctrl Pts',(37.7082882345091,10.88094645291,82.940678146904));
#130535=CARTESIAN_POINT('Ctrl Pts',(39.1142274982291,9.91205347783502,83.67127064968));
#130536=CARTESIAN_POINT('Ctrl Pts',(40.5432158335391,8.74576233655301,84.3936442258099));
#130537=CARTESIAN_POINT('Ctrl Pts',(41.8604028480391,7.43460302127903,85.0471196915701));
#130538=CARTESIAN_POINT('Ctrl Pts',(43.0163443071791,5.99020112655302,85.6153164434601));
#130539=CARTESIAN_POINT('Ctrl Pts',(44.0066134889891,4.35311312370201,86.1022978834));
#130540=CARTESIAN_POINT('Ctrl Pts',(44.7332634147991,2.52355184883601,86.4665423458501));
#130541=CARTESIAN_POINT('Ctrl Pts',(44.9781481988991,1.19967484028401,86.60065479763));
#130542=CARTESIAN_POINT('Ctrl Pts',(45.0312601718991,0.557056200456914,
86.6358961446099));
#130543=CARTESIAN_POINT('',(29.6421154185267,14.3619794304194,78.1139870084275));
#130544=CARTESIAN_POINT('Ctrl Pts',(29.6421046546614,14.3619829782172,78.1140023840685));
#130545=CARTESIAN_POINT('Ctrl Pts',(29.5145956406364,14.3649991419673,78.1261564978929));
#130546=CARTESIAN_POINT('Ctrl Pts',(29.3820227690687,14.369719041399,78.1388270540191));
#130547=CARTESIAN_POINT('Ctrl Pts',(29.2447491213195,14.3765172160041,78.1520061984839));
#130548=CARTESIAN_POINT('Ctrl Pts',(29.2357685362962,14.3769619596679,78.1528683918425));
#130549=CARTESIAN_POINT('Ctrl Pts',(29.2267678363257,14.3774156051513,78.1537327452661));
#130550=CARTESIAN_POINT('Ctrl Pts',(29.2177471248349,14.3778782601166,78.1545992495703));
#130551=CARTESIAN_POINT('Ctrl Pts',(29.1231957583653,14.3827276180877,78.1636815892615));
#130552=CARTESIAN_POINT('Ctrl Pts',(29.0264438263049,14.3885640451357,78.172998206678));
#130553=CARTESIAN_POINT('Ctrl Pts',(28.9271250708793,14.3955514440818,78.1826054494819));
#130554=CARTESIAN_POINT('Ctrl Pts',(28.872119986792,14.3994212314643,78.1879261685748));
#130555=CARTESIAN_POINT('Ctrl Pts',(28.8163274509837,14.4036448482421,78.1933357668402));
#130556=CARTESIAN_POINT('Ctrl Pts',(28.7596841741806,14.4082565912696,78.1988414060183));
#130557=CARTESIAN_POINT('Ctrl Pts',(28.701932031196,14.4129586151948,78.2044548252797));
#130558=CARTESIAN_POINT('Ctrl Pts',(28.6432962519838,14.4180637104245,78.2101696022246));
#130559=CARTESIAN_POINT('Ctrl Pts',(28.5837302065717,14.4236103462183,78.2159942181859));
#130560=CARTESIAN_POINT('Ctrl Pts',(27.6070995425304,14.9199507410733,75.6071390537838));
#130561=CARTESIAN_POINT('Ctrl Pts',(27.7192629013877,14.8959306840627,75.8250406547776));
#130562=CARTESIAN_POINT('Ctrl Pts',(27.8457646196489,14.8667398375127,76.0382447729958));
#130563=CARTESIAN_POINT('Ctrl Pts',(27.9845985217786,14.8326654832504,76.2466690142022));
#130564=CARTESIAN_POINT('Ctrl Pts',(28.1242452289094,14.7983916402096,76.4563134780127));
#130565=CARTESIAN_POINT('Ctrl Pts',(28.2763688932358,14.7591771556667,76.661121665329));
#130566=CARTESIAN_POINT('Ctrl Pts',(28.4389329606639,14.7153582057326,76.861038443836));
#130567=CARTESIAN_POINT('Ctrl Pts',(28.4556902247096,14.7108413052523,76.8816460620976));
#130568=CARTESIAN_POINT('Ctrl Pts',(28.4725584300046,14.7062755155822,76.9022017328212));
#130569=CARTESIAN_POINT('Ctrl Pts',(28.4895353492335,14.7016612297159,76.9227054145368));
#130570=CARTESIAN_POINT('Ctrl Pts',(28.6751623758138,14.6512082497849,77.1468943512624));
#130571=CARTESIAN_POINT('Ctrl Pts',(28.8735586889575,14.5949456973791,77.3649852820764));
#130572=CARTESIAN_POINT('Ctrl Pts',(29.0821746934216,14.533243265586,77.5774426839974));
#130573=CARTESIAN_POINT('Ctrl Pts',(29.261787491736,14.480119122663,77.7603628227453));
#130574=CARTESIAN_POINT('Ctrl Pts',(29.4489760014774,14.4229617454712,77.9391075942936));
#130575=CARTESIAN_POINT('Ctrl Pts',(29.6421154185267,14.3619794304194,78.1139870084275));
#130576=CARTESIAN_POINT('Origin',(58.0152958556891,-0.499074165591486,68.638644839116));
#130577=CARTESIAN_POINT('',(63.7242586906601,14.99856960786,67.8461534157091));
#130578=CARTESIAN_POINT('Ctrl Pts',(63.7242533230191,14.99854021533,67.846155382807));
#130579=CARTESIAN_POINT('Ctrl Pts',(51.5782329133125,14.9978694358453,69.9878171256976));
#130580=CARTESIAN_POINT('Ctrl Pts',(39.4322140887331,14.9978694371101,72.1294878582915));
#130581=CARTESIAN_POINT('Ctrl Pts',(27.2861971798628,14.9986801148638,74.2711694554112));
#130582=CARTESIAN_POINT('',(63.7044144696626,14.9224864514636,69.2168818788526));
#130583=CARTESIAN_POINT('Ctrl Pts',(63.7044145289691,14.92248985567,69.216882216528));
#130584=CARTESIAN_POINT('Ctrl Pts',(63.6851849469295,14.9336666490122,69.1078885713561));
#130585=CARTESIAN_POINT('Ctrl Pts',(63.6707295798855,14.9437626665518,68.9967717088079));
#130586=CARTESIAN_POINT('Ctrl Pts',(63.6613828168746,14.9526646152637,68.8841400361723));
#130587=CARTESIAN_POINT('Ctrl Pts',(63.6522220369491,14.961389431862,68.7737495229593));
#130588=CARTESIAN_POINT('Ctrl Pts',(63.6479686149546,14.9689673053526,68.6619040795053));
#130589=CARTESIAN_POINT('Ctrl Pts',(63.6489383237461,14.9753434652124,68.5491819025216));
#130590=CARTESIAN_POINT('Ctrl Pts',(63.6499375632273,14.9819137992407,68.4330269798916));
#130591=CARTESIAN_POINT('Ctrl Pts',(63.6564829323108,14.9872078381345,68.3159413010022));
#130592=CARTESIAN_POINT('Ctrl Pts',(63.6689204526746,14.991223439365,68.1985604179833));
#130593=CARTESIAN_POINT('Ctrl Pts',(63.6813579730383,14.9952390405955,68.0811795349645));
#130594=CARTESIAN_POINT('Ctrl Pts',(63.6996876813661,14.9979763340792,67.9635036558599));
#130595=CARTESIAN_POINT('Ctrl Pts',(63.7242555654557,14.9994907873196,67.8461681406557));
#130596=CARTESIAN_POINT('',(66.1162021797537,0.79020098334245,82.8948096732265));
#130597=CARTESIAN_POINT('Origin',(63.4339821949991,-0.499074165591486,67.683184237498));
#130598=CARTESIAN_POINT('',(44.6819013833791,0.790370888696714,86.67422941916));
#130599=CARTESIAN_POINT('',(44.6819028561657,0.790371596722371,86.6742377717481));
#130600=CARTESIAN_POINT('',(37.5050940990142,10.7061722565098,83.1298152725198));
#130601=CARTESIAN_POINT('Ctrl Pts',(37.5051003753486,10.7061762392465,83.1298227805085));
#130602=CARTESIAN_POINT('Ctrl Pts',(38.3763978528178,10.1348334115302,83.5832077696022));
#130603=CARTESIAN_POINT('Ctrl Pts',(39.2226440888349,9.50364223937353,84.0079460340611));
#130604=CARTESIAN_POINT('Ctrl Pts',(40.8102490283764,8.10943081545489,84.7907499725118));
#130605=CARTESIAN_POINT('Ctrl Pts',(41.5520655694067,7.34592818639295,85.1489322811934));
#130606=CARTESIAN_POINT('Ctrl Pts',(42.8580113501118,5.68093119810927,85.776362545284));
#130607=CARTESIAN_POINT('Ctrl Pts',(43.4218825811718,4.77838638362871,86.0454790494045));
#130608=CARTESIAN_POINT('Ctrl Pts',(44.0639229648733,3.33561826274428,86.3569296909199));
#130609=CARTESIAN_POINT('Ctrl Pts',(44.2439337207264,2.84043576288029,86.4453260797462));
#130610=CARTESIAN_POINT('Ctrl Pts',(44.5242936554535,1.82822955706199,86.586853260865));
#130611=CARTESIAN_POINT('Ctrl Pts',(44.6247440186015,1.31135464491908,86.6400205490487));
#130612=CARTESIAN_POINT('Ctrl Pts',(44.6819013833791,0.790370888696714,
86.67422941916));
#130613=CARTESIAN_POINT('',(36.7493876194873,13.6349921310859,78.8488579760133));
#130614=CARTESIAN_POINT('Origin',(35.6454492392491,-0.499074165591586,72.5830523519042));
#130615=CARTESIAN_POINT('',(33.6728394647692,14.3619762585541,77.4032747789144));
#130616=CARTESIAN_POINT('Ctrl Pts',(36.7499023085083,13.6386605077094,78.850394493121));
#130617=CARTESIAN_POINT('Ctrl Pts',(36.7483039859788,13.6431409106807,78.8404660979912));
#130618=CARTESIAN_POINT('Ctrl Pts',(36.7466776914937,13.6470698094342,78.831711908129));
#130619=CARTESIAN_POINT('Ctrl Pts',(36.7450249995319,13.6504651160832,78.8241397777305));
#130620=CARTESIAN_POINT('Ctrl Pts',(36.7441982906584,13.6521635149378,78.8203520498683));
#130621=CARTESIAN_POINT('Ctrl Pts',(36.7433649733905,13.6537282955424,78.8168600514848));
#130622=CARTESIAN_POINT('Ctrl Pts',(36.742525153558,13.6551610905843,78.8136644833911));
#130623=CARTESIAN_POINT('Ctrl Pts',(36.7421052436417,13.6558774881053,78.8120666993442));
#130624=CARTESIAN_POINT('Ctrl Pts',(36.7416837081268,13.6565608828926,78.8105430198817));
#130625=CARTESIAN_POINT('Ctrl Pts',(36.741260559816,13.6572114408692,78.8090935149832));
#130626=CARTESIAN_POINT('Ctrl Pts',(36.7410489856607,13.6575367198576,78.808368762534));
#130627=CARTESIAN_POINT('Ctrl Pts',(36.7408370083007,13.6578537892448,78.8076625535445));
#130628=CARTESIAN_POINT('Ctrl Pts',(36.7406246292619,13.6581626673822,78.8069748956749));
#130629=CARTESIAN_POINT('Ctrl Pts',(36.7405184397425,13.6583171064509,78.8066310667402));
#130630=CARTESIAN_POINT('Ctrl Pts',(36.7405071118863,13.6583391525674,78.8065816613395));
#130631=CARTESIAN_POINT('Ctrl Pts',(36.740448204214,13.6584243401768,78.8063920073941));
#130632=CARTESIAN_POINT('Ctrl Pts',(36.7403892965417,13.6585095277861,78.8062023534488));
#130633=CARTESIAN_POINT('Ctrl Pts',(36.7402828111207,13.6586578767028,78.8058724585813));
#130634=CARTESIAN_POINT('Ctrl Pts',(36.7399862885877,13.6590647448003,78.8049675823703));
#130635=CARTESIAN_POINT('Ctrl Pts',(36.7352419280597,13.6655746343596,78.7904895629937));
#130636=CARTESIAN_POINT('Ctrl Pts',(36.7282234174915,13.6735556178127,78.7727678395045));
#130637=CARTESIAN_POINT('Ctrl Pts',(36.7189266889496,13.6830013954498,78.7518015064668));
#130638=CARTESIAN_POINT('Ctrl Pts',(36.7142783246787,13.6877242842683,78.7413183399479));
#130639=CARTESIAN_POINT('Ctrl Pts',(36.7090604132126,13.6928133730756,78.7300240140316));
#130640=CARTESIAN_POINT('Ctrl Pts',(36.70327253979,13.698267885164,78.7179183561814));
#130641=CARTESIAN_POINT('Ctrl Pts',(36.7003786030787,13.7009951412082,78.7118655272564));
#130642=CARTESIAN_POINT('Ctrl Pts',(36.6973421775542,13.7038137533595,78.7056098641795));
#130643=CARTESIAN_POINT('Ctrl Pts',(36.6941632209318,13.7067236250423,78.6991513408688));
#130644=CARTESIAN_POINT('Ctrl Pts',(36.6911649311007,13.709468122597,78.6930598690224));
#130645=CARTESIAN_POINT('Ctrl Pts',(36.6885450749576,13.7118426094089,78.687789320445));
#130646=CARTESIAN_POINT('Ctrl Pts',(36.6848741180589,13.7151236456254,78.6805062934297));
#130647=CARTESIAN_POINT('Ctrl Pts',(36.6846529186282,13.7153213497562,78.6800674428864));
#130648=CARTESIAN_POINT('Ctrl Pts',(36.6844278930973,13.7155223487087,78.6796212730289));
#130649=CARTESIAN_POINT('Ctrl Pts',(36.6841987246351,13.7157269231489,78.6791671587984));
#130650=CARTESIAN_POINT('Ctrl Pts',(36.6680692169269,13.7301254358376,78.6472053482076));
#130651=CARTESIAN_POINT('Ctrl Pts',(36.6503646181003,13.7445537303848,78.6152586270666));
#130652=CARTESIAN_POINT('Ctrl Pts',(36.6310925009288,13.7590546689286,78.5833421826575));
#130653=CARTESIAN_POINT('Ctrl Pts',(36.6180877346395,13.7688398583326,78.5618050626497));
#130654=CARTESIAN_POINT('Ctrl Pts',(36.6040633494866,13.7788041463262,78.5399779777372));
#130655=CARTESIAN_POINT('Ctrl Pts',(36.589949449959,13.788501639847,78.5188095793515));
#130656=CARTESIAN_POINT('Ctrl Pts',(36.5831475775772,13.7931751259535,78.508607951937));
#130657=CARTESIAN_POINT('Ctrl Pts',(36.5763246574787,13.7977863511604,78.4985596617409));
#130658=CARTESIAN_POINT('Ctrl Pts',(36.5695809276106,13.8022700534891,78.4888012993751));
#130659=CARTESIAN_POINT('Ctrl Pts',(36.559212435832,13.8091637505443,78.4737978069545));
#130660=CARTESIAN_POINT('Ctrl Pts',(36.548971858619,13.8158029081853,78.4593755010848));
#130661=CARTESIAN_POINT('Ctrl Pts',(36.5388588882553,13.8221821595769,78.4455321849782));
#130662=CARTESIAN_POINT('Ctrl Pts',(36.5334905180153,13.8255685220493,78.4381835976159));
#130663=CARTESIAN_POINT('Ctrl Pts',(36.5283454585794,13.8287795761135,78.431215627966));
#130664=CARTESIAN_POINT('Ctrl Pts',(36.5229768883168,13.8320566518634,78.4241131015378));
#130665=CARTESIAN_POINT('Ctrl Pts',(36.5182321114119,13.8349529524748,78.4178358430286));
#130666=CARTESIAN_POINT('Ctrl Pts',(36.5133127821366,13.8379011442613,78.4114528236521));
#130667=CARTESIAN_POINT('Ctrl Pts',(36.5079093897136,13.8410531095132,78.4046389204707));
#130668=CARTESIAN_POINT('Ctrl Pts',(36.5015447951238,13.8447657735989,78.3966129012723));
#130669=CARTESIAN_POINT('Ctrl Pts',(36.4945829395513,13.8487260779931,78.388062192188));
#130670=CARTESIAN_POINT('Ctrl Pts',(36.4870259347947,13.8529298786463,78.3789766395846));
#130671=CARTESIAN_POINT('Ctrl Pts',(36.4844101699437,13.8543849728726,78.375831786575));
#130672=CARTESIAN_POINT('Ctrl Pts',(36.4817230461861,13.8558690534932,78.3726232353304));
#130673=CARTESIAN_POINT('Ctrl Pts',(36.4789644617547,13.8573812806233,78.3693519287813));
#130674=CARTESIAN_POINT('Ctrl Pts',(36.4752711027011,13.8594059414236,78.3649721064627));
#130675=CARTESIAN_POINT('Ctrl Pts',(36.4714496611526,13.8614809894887,78.3604799314432));
#130676=CARTESIAN_POINT('Ctrl Pts',(36.4674996366288,13.8636072933881,78.3558716882688));
#130677=CARTESIAN_POINT('Ctrl Pts',(36.4597877537408,13.8677586110717,78.3468747234483));
#130678=CARTESIAN_POINT('Ctrl Pts',(36.4515871632937,13.8721025800674,78.3374418240048));
#130679=CARTESIAN_POINT('Ctrl Pts',(36.4428975930266,13.8766350377088,78.3275713885573));
#130680=CARTESIAN_POINT('Ctrl Pts',(36.438552807893,13.8789012665295,78.3226361708335));
#130681=CARTESIAN_POINT('Ctrl Pts',(36.4340857780505,13.8812146199161,78.3175915703031));
#130682=CARTESIAN_POINT('Ctrl Pts',(36.4294964723451,13.8835746144666,78.3124374042033));
#130683=CARTESIAN_POINT('Ctrl Pts',(36.4267289688733,13.8849977694122,78.309329271189));
#130684=CARTESIAN_POINT('Ctrl Pts',(36.4243686482471,13.8862050042778,78.3066910306504));
#130685=CARTESIAN_POINT('Ctrl Pts',(36.421598860639,13.8876189102116,78.3035976453758));
#130686=CARTESIAN_POINT('Ctrl Pts',(36.4197755547958,13.8885496613433,78.3015613204858));
#130687=CARTESIAN_POINT('Ctrl Pts',(36.4177747384656,13.8895696444297,78.2993284362583));
#130688=CARTESIAN_POINT('Ctrl Pts',(36.4153616994248,13.8907940838674,78.2966460457519));
#130689=CARTESIAN_POINT('Ctrl Pts',(36.4019716470465,13.8975885484107,78.2817613510696));
#130690=CARTESIAN_POINT('Ctrl Pts',(36.3890010975978,13.9040184390785,78.2676211351411));
#130691=CARTESIAN_POINT('Ctrl Pts',(36.3764337310713,13.910136612886,78.2541341879297));
#130692=CARTESIAN_POINT('Ctrl Pts',(36.3672900523479,13.9145880320081,78.2443214469707));
#130693=CARTESIAN_POINT('Ctrl Pts',(36.3583600601549,13.9188739784771,78.2348555092975));
#130694=CARTESIAN_POINT('Ctrl Pts',(36.3496410325615,13.9230076695007,78.2257166146442));
#130695=CARTESIAN_POINT('Ctrl Pts',(36.3268217375824,13.9338262973593,78.2017984505322));
#130696=CARTESIAN_POINT('Ctrl Pts',(36.3054447977087,13.943598679941,78.1801266659689));
#130697=CARTESIAN_POINT('Ctrl Pts',(36.2855839501909,13.9521935012056,78.1611288208426));
#130698=CARTESIAN_POINT('Ctrl Pts',(36.2808490071319,13.9542425572318,78.1565996226381));
#130699=CARTESIAN_POINT('Ctrl Pts',(36.2761982177636,13.9562293358506,78.1522106338178));
#130700=CARTESIAN_POINT('Ctrl Pts',(36.2716316100593,13.9581542476587,78.1479620137005));
#130701=CARTESIAN_POINT('Ctrl Pts',(36.2686426206986,13.9594141633964,78.1451811572858));
#130702=CARTESIAN_POINT('Ctrl Pts',(36.2640769281232,13.9613255588747,78.1409638939666));
#130703=CARTESIAN_POINT('Ctrl Pts',(36.2592938494356,13.9633073451264,78.1365905752382));
#130704=CARTESIAN_POINT('Ctrl Pts',(36.2567692928829,13.9643533516412,78.1342822940716));
#130705=CARTESIAN_POINT('Ctrl Pts',(36.2541844203468,13.965419258694,78.1319299371098));
#130706=CARTESIAN_POINT('Ctrl Pts',(36.2517412373075,13.9664222308341,78.1297163483021));
#130707=CARTESIAN_POINT('Ctrl Pts',(36.2375970578421,13.9722286799298,78.1169013455558));
#130708=CARTESIAN_POINT('Ctrl Pts',(36.2230046602156,13.9780685655748,78.1040081587856));
#130709=CARTESIAN_POINT('Ctrl Pts',(36.2079638463695,13.9839387279526,78.0910356788575));
#130710=CARTESIAN_POINT('Ctrl Pts',(36.207192383829,13.9842398160737,78.0903703038037));
#130711=CARTESIAN_POINT('Ctrl Pts',(36.2064197402877,13.9845409860667,78.0897047141239));
#130712=CARTESIAN_POINT('Ctrl Pts',(36.2056459158412,13.9848422362319,78.0890389129253));
#130713=CARTESIAN_POINT('Ctrl Pts',(36.1778639481647,13.9956577673124,78.0651352129796));
#130714=CARTESIAN_POINT('Ctrl Pts',(36.148561323177,14.0065748413203,78.0409623999071));
#130715=CARTESIAN_POINT('Ctrl Pts',(36.1177379487843,14.0175855767315,78.0165187379705));
#130716=CARTESIAN_POINT('Ctrl Pts',(36.1159428936046,14.0182268069025,78.0150952169305));
#130717=CARTESIAN_POINT('Ctrl Pts',(36.114142675661,14.0188683610647,78.0136707648243));
#130718=CARTESIAN_POINT('Ctrl Pts',(36.112337293027,14.0195102400722,78.0122453765528));
#130719=CARTESIAN_POINT('Ctrl Pts',(36.0931864763242,14.026319050009,77.9971253964415));
#130720=CARTESIAN_POINT('Ctrl Pts',(36.0730170337921,14.0333203443543,77.9815520871684));
#130721=CARTESIAN_POINT('Ctrl Pts',(36.0520653827686,14.0403913058479,77.9658078664028));
#130722=CARTESIAN_POINT('Ctrl Pts',(36.050604035552,14.0408844951381,77.9647097298804));
#130723=CARTESIAN_POINT('Ctrl Pts',(36.0491388901179,14.041378032158,77.9636107440935));
#130724=CARTESIAN_POINT('Ctrl Pts',(36.0476700299407,14.04187187919,77.9625109968557));
#130725=CARTESIAN_POINT('Ctrl Pts',(36.0257420075874,14.0492443227505,77.9460933130025));
#130726=CARTESIAN_POINT('Ctrl Pts',(36.0029842929834,14.0566841655443,77.9295094191599));
#130727=CARTESIAN_POINT('Ctrl Pts',(35.9796840785309,14.0640627858329,77.9130581508823));
#130728=CARTESIAN_POINT('Ctrl Pts',(35.9564015056663,14.0714358194528,77.8966193385627));
#130729=CARTESIAN_POINT('Ctrl Pts',(35.9325772396664,14.0787477537516,77.8803130083138));
#130730=CARTESIAN_POINT('Ctrl Pts',(35.9085200506683,14.0858906018936,77.8643943068697));
#130731=CARTESIAN_POINT('Ctrl Pts',(35.9000853007769,14.0883949733559,77.8588130120107));
#130732=CARTESIAN_POINT('Ctrl Pts',(35.8916221174696,14.0908787388124,77.8532789794143));
#130733=CARTESIAN_POINT('Ctrl Pts',(35.8831444455004,14.0933378118669,77.8478019599974));
#130734=CARTESIAN_POINT('Ctrl Pts',(35.8818762623415,14.0937056669863,77.8469826473593));
#130735=CARTESIAN_POINT('Ctrl Pts',(35.8806072317308,14.0940731498235,77.8461641921004));
#130736=CARTESIAN_POINT('Ctrl Pts',(35.8793373537139,14.0944402608808,77.8453465942344));
#130737=CARTESIAN_POINT('Ctrl Pts',(35.8396948890402,14.105900564095,77.8198232021532));
#130738=CARTESIAN_POINT('Ctrl Pts',(35.7992265591956,14.1169982935614,77.7951356522314));
#130739=CARTESIAN_POINT('Ctrl Pts',(35.7579333334925,14.1277470638494,77.7712893746665));
#130740=CARTESIAN_POINT('Ctrl Pts',(35.7392147843485,14.1326195673035,77.7604796665146));
#130741=CARTESIAN_POINT('Ctrl Pts',(35.7203267314783,14.1374203733427,77.7498428800502));
#130742=CARTESIAN_POINT('Ctrl Pts',(35.7012692658199,14.1421509171572,77.7393794462338));
#130743=CARTESIAN_POINT('Ctrl Pts',(35.6986329392312,14.1428053199335,77.7379319804861));
#130744=CARTESIAN_POINT('Ctrl Pts',(35.6959933706936,14.1434583783386,77.7364878319158));
#130745=CARTESIAN_POINT('Ctrl Pts',(35.693350560544,14.1441100928129,77.7350470088184));
#130746=CARTESIAN_POINT('Ctrl Pts',(35.6824769884722,14.1467915053646,77.7291188895419));
#130747=CARTESIAN_POINT('Ctrl Pts',(35.6715485390952,14.1494501996738,77.7232469700815));
#130748=CARTESIAN_POINT('Ctrl Pts',(35.6605652265203,14.152086379761,77.7174313304439));
#130749=CARTESIAN_POINT('Ctrl Pts',(35.6523277420891,14.1540635148264,77.7130696007158));
#130750=CARTESIAN_POINT('Ctrl Pts',(35.6440593971144,14.1560279857181,77.7087395284178));
#130751=CARTESIAN_POINT('Ctrl Pts',(35.6357601976009,14.1579798800796,77.7044411476049));
#130752=CARTESIAN_POINT('Ctrl Pts',(35.632993797763,14.1586305115335,77.7030083540006));
#130753=CARTESIAN_POINT('Ctrl Pts',(35.6312566437295,14.159038510211,77.7021099864139));
#130754=CARTESIAN_POINT('Ctrl Pts',(35.6274507134639,14.159927585583,77.700153331884));
#130755=CARTESIAN_POINT('Ctrl Pts',(35.5902453846576,14.1686188487543,77.6810258203259));
#130756=CARTESIAN_POINT('Ctrl Pts',(35.5527081000862,14.1769924264008,77.6626793895717));
#130757=CARTESIAN_POINT('Ctrl Pts',(35.5148349612072,14.1850634367579,77.6451066981544));
#130758=CARTESIAN_POINT('Ctrl Pts',(35.4512220903169,14.1986197501503,77.6155910735347));
#130759=CARTESIAN_POINT('Ctrl Pts',(35.3866613241379,14.2113228793747,77.5882569010224));
#130760=CARTESIAN_POINT('Ctrl Pts',(35.3211605362392,14.2232164189763,77.5631320161429));
#130761=CARTESIAN_POINT('Ctrl Pts',(35.2980032775437,14.2274212809664,77.5542493220942));
#130762=CARTESIAN_POINT('Ctrl Pts',(35.2747285838988,14.2315248799444,77.5456430074866));
#130763=CARTESIAN_POINT('Ctrl Pts',(35.2513373519199,14.2355283160288,77.5373160290319));
#130764=CARTESIAN_POINT('Ctrl Pts',(35.2083795937033,14.2428805854393,77.5220236182921));
#130765=CARTESIAN_POINT('Ctrl Pts',(35.1650259012283,14.2498975030737,77.5076661870025));
#130766=CARTESIAN_POINT('Ctrl Pts',(35.1212771035081,14.2565914142495,77.4942454624149));
#130767=CARTESIAN_POINT('Ctrl Pts',(35.0993661923743,14.2599439565034,77.4875238993295));
#130768=CARTESIAN_POINT('Ctrl Pts',(35.077356146224,14.2632154521057,77.4810373778554));
#130769=CARTESIAN_POINT('Ctrl Pts',(35.0552470419858,14.2664069878756,77.4747869789205));
#130770=CARTESIAN_POINT('Ctrl Pts',(35.0221202281705,14.2711889731651,77.4654217961634));
#130771=CARTESIAN_POINT('Ctrl Pts',(34.988771045946,14.2757917356906,77.4565857932991));
#130772=CARTESIAN_POINT('Ctrl Pts',(34.9551997454641,14.280219626959,77.4482803889722));
#130773=CARTESIAN_POINT('Ctrl Pts',(34.9422709177221,14.2819248764622,77.4450818491382));
#130774=CARTESIAN_POINT('Ctrl Pts',(34.9293091485656,14.2836041887418,77.4419620088157));
#130775=CARTESIAN_POINT('Ctrl Pts',(34.9163144477114,14.2852578167427,77.4389209376207));
#130776=CARTESIAN_POINT('Ctrl Pts',(34.9124379744826,14.2857511135679,77.438013750052));
#130777=CARTESIAN_POINT('Ctrl Pts',(34.9085585705191,14.2862421246787,77.4371135724129));
#130778=CARTESIAN_POINT('Ctrl Pts',(34.9046762371865,14.2867308552347,77.4362204079851));
#130779=CARTESIAN_POINT('Ctrl Pts',(34.8962278979827,14.2877943809966,77.4342767943372));
#130780=CARTESIAN_POINT('Ctrl Pts',(34.8877656839372,14.2888471091787,77.4323663859133));
#130781=CARTESIAN_POINT('Ctrl Pts',(34.8792895983832,14.2898890981529,77.4304892016174));
#130782=CARTESIAN_POINT('Ctrl Pts',(34.8750515556062,14.2904100926399,77.4295506094695));
#130783=CARTESIAN_POINT('Ctrl Pts',(34.8708100449522,14.290928402325,77.4286203233538));
#130784=CARTESIAN_POINT('Ctrl Pts',(34.8665650668364,14.2914440345086,77.4276983456258));
#130785=CARTESIAN_POINT('Ctrl Pts',(34.8630614993612,14.2918696084689,77.426937396784));
#130786=CARTESIAN_POINT('Ctrl Pts',(34.8608359622675,14.292139014898,77.4264567387017));
#130787=CARTESIAN_POINT('Ctrl Pts',(34.8567182529457,14.2926345630268,77.4255759377945));
#130788=CARTESIAN_POINT('Ctrl Pts',(34.8558468801156,14.292739428898,77.4253895463037));
#130789=CARTESIAN_POINT('Ctrl Pts',(34.8548907417037,14.29285437067,77.425185390079));
#130790=CARTESIAN_POINT('Ctrl Pts',(34.8538197305188,14.2929829058584,77.4249573399584));
#130791=CARTESIAN_POINT('Ctrl Pts',(34.8050235101287,14.2988390831483,77.4145671740102));
#130792=CARTESIAN_POINT('Ctrl Pts',(34.7562088083104,14.30427527912,77.405416163315));
#130793=CARTESIAN_POINT('Ctrl Pts',(34.7073784381505,14.3093168215444,77.3974681360169));
#130794=CARTESIAN_POINT('Ctrl Pts',(34.6367845691646,14.3166053590719,77.3859777050425));
#130795=CARTESIAN_POINT('Ctrl Pts',(34.5661586592343,14.3230696569618,77.3769996824145));
#130796=CARTESIAN_POINT('Ctrl Pts',(34.4955002238291,14.3287650076083,77.370466012057));
#130797=CARTESIAN_POINT('Ctrl Pts',(34.4242963422592,14.3345043233829,77.3638819051815));
#130798=CARTESIAN_POINT('Ctrl Pts',(34.3530589739449,14.339462739832,77.3597798029414));
#130799=CARTESIAN_POINT('Ctrl Pts',(34.2817762337855,14.3436823305113,77.3581082693766));
#130800=CARTESIAN_POINT('Ctrl Pts',(34.2103212232019,14.3479121187599,77.3564326961832));
#130801=CARTESIAN_POINT('Ctrl Pts',(34.1388201014431,14.3513994978328,77.3571992693894));
#130802=CARTESIAN_POINT('Ctrl Pts',(34.0672795372947,14.3541443651951,77.360469723857));
#130803=CARTESIAN_POINT('Ctrl Pts',(33.995928686004,14.3568819536571,77.3637315056608));
#130804=CARTESIAN_POINT('Ctrl Pts',(33.924538247131,14.358880723838,77.3694846102313));
#130805=CARTESIAN_POINT('Ctrl Pts',(33.853048606998,14.3602097289537,77.3775449630649));
#130806=CARTESIAN_POINT('Ctrl Pts',(33.7930046121601,14.3613259574891,77.3843148360567));
#130807=CARTESIAN_POINT('Ctrl Pts',(33.7328896972954,14.3619703585475,77.3927103145005));
#130808=CARTESIAN_POINT('Ctrl Pts',(33.6728395094596,14.361977126785,77.4032750323744));
#130809=CARTESIAN_POINT('',(33.6728394518991,14.36197600861,77.403274705915));
#130810=CARTESIAN_POINT('Origin',(57.8121127436691,0.499074165591614,68.674471503788));
#130811=CARTESIAN_POINT('Ctrl Pts',(29.6420897207618,-14.3619786049856,
78.1139943677011));
#130812=CARTESIAN_POINT('Ctrl Pts',(29.4150088098653,-14.4336850553689,
77.9083573314674));
#130813=CARTESIAN_POINT('Ctrl Pts',(29.1961090381446,-14.5001071219915,
77.6973723716935));
#130814=CARTESIAN_POINT('Ctrl Pts',(28.988087795971,-14.5608976041789,77.4805442029342));
#130815=CARTESIAN_POINT('Ctrl Pts',(28.8137425456767,-14.6118468809053,
77.2988177553936));
#130816=CARTESIAN_POINT('Ctrl Pts',(28.6470387676822,-14.6588395856372,
77.1129870427136));
#130817=CARTESIAN_POINT('Ctrl Pts',(28.489566865647,-14.7016466499152,76.9227741006316));
#130818=CARTESIAN_POINT('Ctrl Pts',(28.328472849534,-14.7454383474399,76.7281859464236));
#130819=CARTESIAN_POINT('Ctrl Pts',(28.1771332810037,-14.784864646458,76.5288895083911));
#130820=CARTESIAN_POINT('Ctrl Pts',(28.037477697831,-14.8195994014424,76.3249565636834));
#130821=CARTESIAN_POINT('Ctrl Pts',(27.8986632578008,-14.8541249496032,
76.1222519035461));
#130822=CARTESIAN_POINT('Ctrl Pts',(27.7713925293067,-14.8840150929903,
75.9149666874586));
#130823=CARTESIAN_POINT('Ctrl Pts',(27.6575651521258,-14.9089932661783,
75.7031983825737));
#130824=CARTESIAN_POINT('Ctrl Pts',(27.6404658644236,-14.9127455178791,
75.6713862890237));
#130825=CARTESIAN_POINT('Ctrl Pts',(27.6236699529832,-14.916387008058,75.639473073654));
#130826=CARTESIAN_POINT('Ctrl Pts',(27.60718386578,-14.9199168893285,75.6074591138482));
#130827=CARTESIAN_POINT('',(36.6019507223326,-13.7800919958273,78.5369560490225));
#130828=CARTESIAN_POINT('Ctrl Pts',(33.6728409414565,-14.3619769299805,
77.4032752837662));
#130829=CARTESIAN_POINT('Ctrl Pts',(33.7272025377404,-14.361970498807,77.3937110128019));
#130830=CARTESIAN_POINT('Ctrl Pts',(33.7815742626743,-14.3615351034956,
77.3856122868006));
#130831=CARTESIAN_POINT('Ctrl Pts',(33.8359564067913,-14.3606723999005,
77.3789753427906));
#130832=CARTESIAN_POINT('Ctrl Pts',(33.9066462029422,-14.3595509961334,
77.3703481688026));
#130833=CARTESIAN_POINT('Ctrl Pts',(33.9773542073291,-14.3577080326573,
77.3641892993487));
#130834=CARTESIAN_POINT('Ctrl Pts',(34.04807857051,-14.355129255808,77.3605032924183));
#130835=CARTESIAN_POINT('Ctrl Pts',(34.0992590960304,-14.3532630933088,
77.3578358697187));
#130836=CARTESIAN_POINT('Ctrl Pts',(34.1504484442645,-14.3510120544897,
77.3564618530038));
#130837=CARTESIAN_POINT('Ctrl Pts',(34.2016464248871,-14.34837174654,77.3563790209224));
#130838=CARTESIAN_POINT('Ctrl Pts',(34.2130363325421,-14.3477843627534,
77.3563605934425));
#130839=CARTESIAN_POINT('Ctrl Pts',(34.2244266638507,-14.3471776973984,
77.3564061216377));
#130840=CARTESIAN_POINT('Ctrl Pts',(34.2358174143738,-14.3465516544306,
77.3565155763719));
#130841=CARTESIAN_POINT('Ctrl Pts',(34.2671136743056,-14.3448315918756,
77.3568163049152));
#130842=CARTESIAN_POINT('Ctrl Pts',(34.2984131089727,-14.3429653097249,
77.3575994149109));
#130843=CARTESIAN_POINT('Ctrl Pts',(34.3297156117792,-14.340950787442,77.3588643018472));
#130844=CARTESIAN_POINT('Ctrl Pts',(34.3453668631825,-14.3399435263006,
77.3594967453153));
#130845=CARTESIAN_POINT('Ctrl Pts',(34.3610188815834,-14.3388992044659,
77.3602496328084));
#130846=CARTESIAN_POINT('Ctrl Pts',(34.3766716533494,-14.3378175653105,
77.3611228870165));
#130847=CARTESIAN_POINT('Ctrl Pts',(34.3844980392324,-14.3372767457328,
77.3615595141205));
#130848=CARTESIAN_POINT('Ctrl Pts',(34.3923246134542,-14.3367265967795,
77.3620262328891));
#130849=CARTESIAN_POINT('Ctrl Pts',(34.4001513742904,-14.3361670861053,
77.3625230335429));
#130850=CARTESIAN_POINT('Ctrl Pts',(34.4066761933168,-14.3357006471825,
77.3629371939378));
#130851=CARTESIAN_POINT('Ctrl Pts',(34.4140182080303,-14.3351679045298,
77.3634285831324));
#130852=CARTESIAN_POINT('Ctrl Pts',(34.4201339208968,-14.3347182637942,
77.3638567490773));
#130853=CARTESIAN_POINT('Ctrl Pts',(34.4213542309539,-14.3346285438999,
77.3639421839596));
#130854=CARTESIAN_POINT('Ctrl Pts',(34.4225257326911,-14.3345421830295,
77.3640249374553));
#130855=CARTESIAN_POINT('Ctrl Pts',(34.4236322149063,-14.334460436391,77.3641036713141));
#130856=CARTESIAN_POINT('Ctrl Pts',(34.4597437123129,-14.3317925276942,
77.3666732539962));
#130857=CARTESIAN_POINT('Ctrl Pts',(34.4957326686996,-14.3289393393633,
77.3698560515037));
#130858=CARTESIAN_POINT('Ctrl Pts',(34.5315995951639,-14.3258983524844,
77.3736496133823));
#130859=CARTESIAN_POINT('Ctrl Pts',(34.6014396266313,-14.3199769468819,
77.3810364320224));
#130860=CARTESIAN_POINT('Ctrl Pts',(34.6708180602052,-14.313344326686,77.3907363531963));
#130861=CARTESIAN_POINT('Ctrl Pts',(34.7397301308635,-14.3059682544703,
77.4027474724843));
#130862=CARTESIAN_POINT('Ctrl Pts',(34.7687691767077,-14.3028600312349,
77.4078088708767));
#130863=CARTESIAN_POINT('Ctrl Pts',(34.7977255652342,-14.2996199103586,
77.4132802005972));
#130864=CARTESIAN_POINT('Ctrl Pts',(34.8265993196458,-14.2962456152313,
77.4191605433792));
#130865=CARTESIAN_POINT('Ctrl Pts',(34.8495799359604,-14.293560014303,77.4238407072175));
#130866=CARTESIAN_POINT('Ctrl Pts',(34.8725082027622,-14.2907894109111,
77.4287799916888));
#130867=CARTESIAN_POINT('Ctrl Pts',(34.8953839390617,-14.2879323808891,
77.4339780314365));
#130868=CARTESIAN_POINT('Ctrl Pts',(34.9211927967197,-14.2847090231709,
77.4398425625797));
#130869=CARTESIAN_POINT('Ctrl Pts',(34.9469348594218,-14.2813756705961,
77.4460363981471));
#130870=CARTESIAN_POINT('Ctrl Pts',(34.9726100094389,-14.2779302667008,
77.4525588704641));
#130871=CARTESIAN_POINT('Ctrl Pts',(34.9854475844475,-14.2762075647531,
77.4558201066226));
#130872=CARTESIAN_POINT('Ctrl Pts',(34.9982684312438,-14.2744568492298,
77.459163501736));
#130873=CARTESIAN_POINT('Ctrl Pts',(35.0110725347527,-14.2726778586205,
77.4625889703087));
#130874=CARTESIAN_POINT('Ctrl Pts',(35.0174745865072,-14.2717883633158,
77.4643017045951));
#130875=CARTESIAN_POINT('Ctrl Pts',(35.023872452437,-14.27089179919,77.4660349572307));
#130876=CARTESIAN_POINT('Ctrl Pts',(35.0302661306316,-14.2699881332691,
77.4677887173792));
#130877=CARTESIAN_POINT('Ctrl Pts',(35.0356931412296,-14.2692210936433,
77.4692773245037));
#130878=CARTESIAN_POINT('Ctrl Pts',(35.0420294242761,-14.2683183798507,
77.4710354852173));
#130879=CARTESIAN_POINT('Ctrl Pts',(35.0469517917309,-14.2676123183688,
77.4724147355838));
#130880=CARTESIAN_POINT('Ctrl Pts',(35.0478285715033,-14.2674865535958,
77.4726604098114));
#130881=CARTESIAN_POINT('Ctrl Pts',(35.0486605342653,-14.2673670708111,
77.4728939369763));
#130882=CARTESIAN_POINT('Ctrl Pts',(35.0494346000841,-14.2672557969472,
77.4731115094452));
#130883=CARTESIAN_POINT('Ctrl Pts',(35.0623241236228,-14.2654028962588,
77.4767344642254));
#130884=CARTESIAN_POINT('Ctrl Pts',(35.0753465740663,-14.2634907558366,
77.4805104914103));
#130885=CARTESIAN_POINT('Ctrl Pts',(35.0885017828721,-14.261518982626,77.484438676299));
#130886=CARTESIAN_POINT('Ctrl Pts',(35.1345547101024,-14.254616323039,77.4981902187866));
#130887=CARTESIAN_POINT('Ctrl Pts',(35.1822339451496,-14.2469843083068,
77.5138031645961));
#130888=CARTESIAN_POINT('Ctrl Pts',(35.2315364670706,-14.2385942411379,
77.5312608583579));
#130889=CARTESIAN_POINT('Ctrl Pts',(35.2576548507792,-14.2341495396273,
77.5405092036062));
#130890=CARTESIAN_POINT('Ctrl Pts',(35.2842289482715,-14.2294917892299,
77.550275976932));
#130891=CARTESIAN_POINT('Ctrl Pts',(35.3112593298257,-14.2246143399155,
77.5605641669722));
#130892=CARTESIAN_POINT('Ctrl Pts',(35.3140793555763,-14.2241054853647,
77.5616375133022));
#130893=CARTESIAN_POINT('Ctrl Pts',(35.3169043406836,-14.2235942515125,
77.562716497919));
#130894=CARTESIAN_POINT('Ctrl Pts',(35.3197342849219,-14.223080632316,77.5638011189002));
#130895=CARTESIAN_POINT('Ctrl Pts',(35.3285237742618,-14.2214853887098,
77.5671698299947));
#130896=CARTESIAN_POINT('Ctrl Pts',(35.3373611008867,-14.2198671364423,
77.5705929090628));
#130897=CARTESIAN_POINT('Ctrl Pts',(35.3462462540574,-14.2182256868004,
77.5740702954494));
#130898=CARTESIAN_POINT('Ctrl Pts',(35.3540296323547,-14.2167877798478,
77.5771164797089));
#130899=CARTESIAN_POINT('Ctrl Pts',(35.3599572575574,-14.2156825647817,
77.579461915545));
#130900=CARTESIAN_POINT('Ctrl Pts',(35.3656786235503,-14.2146112070245,
77.5817371358453));
#130901=CARTESIAN_POINT('Ctrl Pts',(35.3685913724629,-14.2140657785121,
77.5828954510909));
#130902=CARTESIAN_POINT('Ctrl Pts',(35.3714502843064,-14.2135288364717,
77.584036354385));
#130903=CARTESIAN_POINT('Ctrl Pts',(35.3744709742961,-14.2129594153419,
77.5852472046803));
#130904=CARTESIAN_POINT('Ctrl Pts',(35.3923791327044,-14.2095836025881,
77.5924257297757));
#130905=CARTESIAN_POINT('Ctrl Pts',(35.4099953379316,-14.2061959516237,
77.5996561073567));
#130906=CARTESIAN_POINT('Ctrl Pts',(35.4273195837607,-14.2027964278702,
77.6069383021139));
#130907=CARTESIAN_POINT('Ctrl Pts',(35.4607114505945,-14.1962439669093,
77.6209744731535));
#130908=CARTESIAN_POINT('Ctrl Pts',(35.4930186015498,-14.1896473791923,
77.6352031769755));
#130909=CARTESIAN_POINT('Ctrl Pts',(35.5242411510413,-14.183006578874,77.6496241184234));
#130910=CARTESIAN_POINT('Ctrl Pts',(35.5254161386802,-14.1827566678829,
77.6501668168327));
#130911=CARTESIAN_POINT('Ctrl Pts',(35.5265895893368,-14.1825066941666,
77.6507097880553));
#130912=CARTESIAN_POINT('Ctrl Pts',(35.527761502806,-14.1822566576985,77.6512530321797));
#130913=CARTESIAN_POINT('Ctrl Pts',(35.5600742768922,-14.1753624866553,
77.6662317188553));
#130914=CARTESIAN_POINT('Ctrl Pts',(35.5901199709455,-14.1686382498632,
77.6809571423816));
#130915=CARTESIAN_POINT('Ctrl Pts',(35.6178208546784,-14.1622409278501,
77.6950090128537));
#130916=CARTESIAN_POINT('Ctrl Pts',(35.6455217384113,-14.155843605837,77.7090608833258));
#130917=CARTESIAN_POINT('Ctrl Pts',(35.672869329356,-14.1493103821472,77.7234596228866));
#130918=CARTESIAN_POINT('Ctrl Pts',(35.6998633988907,-14.1426379035811,
77.7382039349708));
#130919=CARTESIAN_POINT('Ctrl Pts',(35.7012774602112,-14.1422883714796,
77.73897630319));
#130920=CARTESIAN_POINT('Ctrl Pts',(35.7026905508738,-14.1419384571469,
77.7397496200118));
#130921=CARTESIAN_POINT('Ctrl Pts',(35.7041026711878,-14.1415881600775,
77.7405238852301));
#130922=CARTESIAN_POINT('Ctrl Pts',(35.7296475670897,-14.1352513755382,
77.7545301453251));
#130923=CARTESIAN_POINT('Ctrl Pts',(35.7548750275898,-14.1287893912822,
77.7688466343453));
#130924=CARTESIAN_POINT('Ctrl Pts',(35.7797848051706,-14.1221992814675,
77.7834722384713));
#130925=CARTESIAN_POINT('Ctrl Pts',(35.7929281994666,-14.1187220761225,
77.7911892917939));
#130926=CARTESIAN_POINT('Ctrl Pts',(35.8059831537425,-14.1152091991775,
77.7989923998503));
#130927=CARTESIAN_POINT('Ctrl Pts',(35.8189496368222,-14.1116602102718,
77.8068813858294));
#130928=CARTESIAN_POINT('Ctrl Pts',(35.8276686349742,-14.1092737784598,
77.8121861437774));
#130929=CARTESIAN_POINT('Ctrl Pts',(35.8368584600997,-14.1067289489184,
77.8178457671225));
#130930=CARTESIAN_POINT('Ctrl Pts',(35.8454873274808,-14.1043115113263,
77.8232242220107));
#130931=CARTESIAN_POINT('Ctrl Pts',(35.8496909049451,-14.1031338496779,
77.8258443517175));
#130932=CARTESIAN_POINT('Ctrl Pts',(35.8537618658522,-14.1019866869613,
77.8283971315277));
#130933=CARTESIAN_POINT('Ctrl Pts',(35.8575836406485,-14.10090445785,77.8308057970622));
#130934=CARTESIAN_POINT('Ctrl Pts',(35.859161032695,-14.1004577806689,77.8317999450849));
#130935=CARTESIAN_POINT('Ctrl Pts',(35.8607397270648,-14.1000095030216,
77.8327979050927));
#130936=CARTESIAN_POINT('Ctrl Pts',(35.862319725231,-14.0995596222712,77.8337996742316));
#130937=CARTESIAN_POINT('Ctrl Pts',(35.8989675468846,-14.0891247054091,
77.8570355598966));
#130938=CARTESIAN_POINT('Ctrl Pts',(35.9363187501883,-14.0778289565087,
77.8823174887484));
#130939=CARTESIAN_POINT('Ctrl Pts',(35.9743728723604,-14.065631652356,77.9096255199391));
#130940=CARTESIAN_POINT('Ctrl Pts',(35.9831256240291,-14.0628261750994,
77.9159065849573));
#130941=CARTESIAN_POINT('Ctrl Pts',(35.9919154615997,-14.0599729189671,
77.9222950088109));
#130942=CARTESIAN_POINT('Ctrl Pts',(36.0007421893682,-14.0570712344685,
77.9287908690435));
#130943=CARTESIAN_POINT('Ctrl Pts',(36.0008339072921,-14.0570410832635,
77.9288583670824));
#130944=CARTESIAN_POINT('Ctrl Pts',(36.0009256291984,-14.0570109268291,
77.9289258767226));
#130945=CARTESIAN_POINT('Ctrl Pts',(36.0010173550866,-14.0569807651646,
77.928993397964));
#130946=CARTESIAN_POINT('Ctrl Pts',(36.0254938233812,-14.0489323173462,
77.9470110106164));
#130947=CARTESIAN_POINT('Ctrl Pts',(36.0502552108871,-14.0405123339591,
77.9658522623971));
#130948=CARTESIAN_POINT('Ctrl Pts',(36.0753006900738,-14.0317086757779,
77.9855124604623));
#130949=CARTESIAN_POINT('Ctrl Pts',(36.0878234296672,-14.0273068466874,
77.9953425594949));
#130950=CARTESIAN_POINT('Ctrl Pts',(36.1004171912915,-14.0228090849255,
78.0053773900386));
#130951=CARTESIAN_POINT('Ctrl Pts',(36.1130818628475,-14.0182137803284,
78.0156163166988));
#130952=CARTESIAN_POINT('Ctrl Pts',(36.1159381083572,-14.0171774077653,
78.0179254873842));
#130953=CARTESIAN_POINT('Ctrl Pts',(36.1187979572607,-14.0161360746697,
78.0202450365019));
#130954=CARTESIAN_POINT('Ctrl Pts',(36.1216614144598,-14.0150897599198,
78.0225749611393));
#130955=CARTESIAN_POINT('Ctrl Pts',(36.1251462814536,-14.0138163804056,
78.0254105116304));
#130956=CARTESIAN_POINT('Ctrl Pts',(36.1286364928932,-14.0125356224787,
78.028261429478));
#130957=CARTESIAN_POINT('Ctrl Pts',(36.1321320379128,-14.0112474556699,
78.0311276953339));
#130958=CARTESIAN_POINT('Ctrl Pts',(36.1369172510304,-14.0094840245952,
78.0350514591232));
#130959=CARTESIAN_POINT('Ctrl Pts',(36.1423402142178,-14.0074737274822,
78.0395217443241));
#130960=CARTESIAN_POINT('Ctrl Pts',(36.1469848824806,-14.0057413974127,
78.0433719312452));
#130961=CARTESIAN_POINT('Ctrl Pts',(36.1485209646206,-14.0051684821624,
78.0446452629516));
#130962=CARTESIAN_POINT('Ctrl Pts',(36.1499722687784,-14.00462610118,78.0458504981156));
#130963=CARTESIAN_POINT('Ctrl Pts',(36.1512884913628,-14.0041335817444,
78.0469447278));
#130964=CARTESIAN_POINT('Ctrl Pts',(36.1782330656311,-13.9940511483721,
78.0693448547607));
#130965=CARTESIAN_POINT('Ctrl Pts',(36.2037212320875,-13.9842162837019,
78.0911091994145));
#130966=CARTESIAN_POINT('Ctrl Pts',(36.2277600458757,-13.9746408618653,
78.1122449979267));
#130967=CARTESIAN_POINT('Ctrl Pts',(36.2415208838529,-13.9691594837233,
78.1243440266646));
#130968=CARTESIAN_POINT('Ctrl Pts',(36.2548065124784,-13.9637630862073,
78.1362371448907));
#130969=CARTESIAN_POINT('Ctrl Pts',(36.2676148158524,-13.9584547731634,
78.147923948464));
#130970=CARTESIAN_POINT('Ctrl Pts',(36.2852063828794,-13.9511640694703,
78.1639751913482));
#130971=CARTESIAN_POINT('Ctrl Pts',(36.3019001339735,-13.9440388550898,
78.1796385997256));
#130972=CARTESIAN_POINT('Ctrl Pts',(36.3176964474293,-13.9370850777245,
78.1949163196451));
#130973=CARTESIAN_POINT('Ctrl Pts',(36.3185529732293,-13.9367080220439,
78.1957447256724));
#130974=CARTESIAN_POINT('Ctrl Pts',(36.3194068612149,-13.9363314697869,
78.1965719988951));
#130975=CARTESIAN_POINT('Ctrl Pts',(36.3202581102729,-13.9359554225258,
78.1973981381346));
#130976=CARTESIAN_POINT('Ctrl Pts',(36.3272563602897,-13.9328638798961,
78.2041899564549));
#130977=CARTESIAN_POINT('Ctrl Pts',(36.3340762696947,-13.9298064677979,
78.2109051346778));
#130978=CARTESIAN_POINT('Ctrl Pts',(36.3407178844198,-13.9267836947292,
78.2175438886205));
#130979=CARTESIAN_POINT('Ctrl Pts',(36.3457493310117,-13.9244937514121,
78.2225731679873));
#130980=CARTESIAN_POINT('Ctrl Pts',(36.3511819022624,-13.9219895669129,
78.2280732250152));
#130981=CARTESIAN_POINT('Ctrl Pts',(36.3559936534691,-13.9197452641846,
78.2330022598293));
#130982=CARTESIAN_POINT('Ctrl Pts',(36.358306108191,-13.9186666862991,78.2353710792759));
#130983=CARTESIAN_POINT('Ctrl Pts',(36.3604759564432,-13.9176483357899,
78.2376076286151));
#130984=CARTESIAN_POINT('Ctrl Pts',(36.3623934414974,-13.9167437885408,
78.2395944935088));
#130985=CARTESIAN_POINT('Ctrl Pts',(36.3749919734724,-13.9108006040469,
78.2526488747348));
#130986=CARTESIAN_POINT('Ctrl Pts',(36.3873118234454,-13.9048459166144,
78.2657120018899));
#130987=CARTESIAN_POINT('Ctrl Pts',(36.3993672617985,-13.898875701994,78.2787923249773));
#130988=CARTESIAN_POINT('Ctrl Pts',(36.4229875655499,-13.8871782191928,
78.3044206924779));
#130989=CARTESIAN_POINT('Ctrl Pts',(36.4455937762913,-13.8754216409494,
78.330114080275));
#130990=CARTESIAN_POINT('Ctrl Pts',(36.4672289647874,-13.8635913786357,
78.3559045591743));
#130991=CARTESIAN_POINT('Ctrl Pts',(36.487490605428,-13.8525121812565,78.3800576843251));
#130992=CARTESIAN_POINT('Ctrl Pts',(36.5069006425037,-13.8413682226984,
78.4042962747751));
#130993=CARTESIAN_POINT('Ctrl Pts',(36.5254653006551,-13.8301512702905,
78.4286404423582));
#130994=CARTESIAN_POINT('Ctrl Pts',(36.5427401219216,-13.8197136502481,
78.4512932238126));
#130995=CARTESIAN_POINT('Ctrl Pts',(36.5592829741807,-13.809212717274,78.4740376470478));
#130996=CARTESIAN_POINT('Ctrl Pts',(36.5750485509559,-13.7986683824196,
78.4968346922204));
#130997=CARTESIAN_POINT('Ctrl Pts',(36.5842881569723,-13.7924887480714,
78.5101951749186));
#130998=CARTESIAN_POINT('Ctrl Pts',(36.5932605244772,-13.7862941512809,
78.5235738259073));
#130999=CARTESIAN_POINT('Ctrl Pts',(36.6019498638648,-13.7800926665008,
78.5369546240003));
#131000=CARTESIAN_POINT('',(36.732951463716,-13.66231606687,78.7896965370107));
#131001=CARTESIAN_POINT('Ctrl Pts',(36.6019526015505,-13.7800906846102,
78.5369587979563));
#131002=CARTESIAN_POINT('Ctrl Pts',(36.6186687600556,-13.7682869278469,
78.5623962793156));
#131003=CARTESIAN_POINT('Ctrl Pts',(36.6410689345548,-13.751533992336,78.598384532446));
#131004=CARTESIAN_POINT('Ctrl Pts',(36.6597206152858,-13.7363178480004,
78.6309989125395));
#131005=CARTESIAN_POINT('Ctrl Pts',(36.6713225306487,-13.7265215745043,
78.6519946927202));
#131006=CARTESIAN_POINT('Ctrl Pts',(36.6772545910443,-13.7212964464913,
78.6631933561585));
#131007=CARTESIAN_POINT('Ctrl Pts',(36.6993608981787,-13.701065109125,78.706581709443));
#131008=CARTESIAN_POINT('Ctrl Pts',(36.7163702000577,-13.6827870327493,
78.745902507885));
#131009=CARTESIAN_POINT('Ctrl Pts',(36.7329514516655,-13.6623159070804,
78.7896964668812));
#131010=CARTESIAN_POINT('',(36.7432202460569,-13.6362301419005,78.8470059772675));
#131011=CARTESIAN_POINT('Ctrl Pts',(36.732951638443,-13.6623156764858,78.7896969601932));
#131012=CARTESIAN_POINT('Ctrl Pts',(36.7358943168784,-13.6534550679484,
78.8093974025206));
#131013=CARTESIAN_POINT('Ctrl Pts',(36.7390843317269,-13.6445697336436,
78.8289974475113));
#131014=CARTESIAN_POINT('Ctrl Pts',(36.7385844993717,-13.6362413718505,
78.8476679968162));
#131015=CARTESIAN_POINT('',(37.505104684855,-10.7061845463452,83.1298573144579));
#131016=CARTESIAN_POINT('Origin',(35.6454492392491,0.499074165591614,72.5830523519042));
#131017=CARTESIAN_POINT('',(44.6819372453691,-0.790063546693886,86.67424130138));
#131018=CARTESIAN_POINT('Ctrl Pts',(44.6819372453691,-0.790063546693886,
86.67424130138));
#131019=CARTESIAN_POINT('Ctrl Pts',(44.6247705097188,-1.31120277256221,
86.6400071574514));
#131020=CARTESIAN_POINT('Ctrl Pts',(44.5244235625226,-1.8281974408512,86.5868803494066));
#131021=CARTESIAN_POINT('Ctrl Pts',(44.2439884476587,-2.84029710432558,
86.4453289128632));
#131022=CARTESIAN_POINT('Ctrl Pts',(44.0639901013491,-3.33552362347414,
86.3569370305293));
#131023=CARTESIAN_POINT('Ctrl Pts',(43.421984756127,-4.77832198714366,86.045504650961));
#131024=CARTESIAN_POINT('Ctrl Pts',(42.8581121434222,-5.68082820437495,
85.7763936738176));
#131025=CARTESIAN_POINT('Ctrl Pts',(41.5521349176424,-7.34586556449325,
85.1489543034165));
#131026=CARTESIAN_POINT('Ctrl Pts',(40.8103108900288,-8.10938402555221,
84.7907746159092));
#131027=CARTESIAN_POINT('Ctrl Pts',(39.2226854324597,-9.50361172924995,
84.0079690139411));
#131028=CARTESIAN_POINT('Ctrl Pts',(38.3764113480733,-10.134813445805,83.5832161340583));
#131029=CARTESIAN_POINT('Ctrl Pts',(37.5051065718069,-10.7061611690822,
83.129837958246));
#131030=CARTESIAN_POINT('',(66.1162021796967,-0.790200987013387,82.8948096729252));
#131031=CARTESIAN_POINT('',(44.6819400502385,-0.790064894780452,86.6742572085851));
#131032=CARTESIAN_POINT('',(63.7044145293691,-14.9224898553757,69.2168822194142));
#131033=CARTESIAN_POINT('Origin',(63.4339821949991,0.499074165591614,67.683184237498));
#131034=CARTESIAN_POINT('',(63.7242525775431,-14.9985986835124,67.8461529431334));
#131035=CARTESIAN_POINT('Ctrl Pts',(63.7242555858646,-14.9994907861995,
67.8461682206232));
#131036=CARTESIAN_POINT('Ctrl Pts',(63.6999435022481,-14.9979924635271,
67.9622549775836));
#131037=CARTESIAN_POINT('Ctrl Pts',(63.681735399389,-14.9952970619206,68.0786951824008));
#131038=CARTESIAN_POINT('Ctrl Pts',(63.6693017595057,-14.99134917377,68.1948747105009));
#131039=CARTESIAN_POINT('Ctrl Pts',(63.6570882649006,-14.9874711854189,
68.3089972082561));
#131040=CARTESIAN_POINT('Ctrl Pts',(63.6504465299545,-14.9823847045197,
68.4228679931466));
#131041=CARTESIAN_POINT('Ctrl Pts',(63.6490641819511,-14.9760888534598,
68.5359047043168));
#131042=CARTESIAN_POINT('Ctrl Pts',(63.6476444592164,-14.9696227806171,
68.6519976044444));
#131043=CARTESIAN_POINT('Ctrl Pts',(63.6517723278146,-14.9618807905353,
68.7672105049499));
#131044=CARTESIAN_POINT('Ctrl Pts',(63.6611098706025,-14.9529192231808,
68.8809152638675));
#131045=CARTESIAN_POINT('Ctrl Pts',(63.6704474133904,-14.9439576558262,
68.9946200227852));
#131046=CARTESIAN_POINT('Ctrl Pts',(63.6849945952704,-14.933776612024,69.1068164410672));
#131047=CARTESIAN_POINT('Ctrl Pts',(63.7044145293206,-14.9224898553757,
69.2168822194228));
#131048=CARTESIAN_POINT('Ctrl Pts',(27.2861973898773,-14.9986800996563,
74.271170552334));
#131049=CARTESIAN_POINT('Ctrl Pts',(39.4322141020864,-14.9978694362286,
72.1294879217807));
#131050=CARTESIAN_POINT('Ctrl Pts',(51.5782329298002,-14.9978694348211,
69.9878171992915));
#131051=CARTESIAN_POINT('Ctrl Pts',(63.7242533594791,-14.99854733863,67.846155561997));
#131052=CARTESIAN_POINT('Origin',(58.0356083261291,-9.5,68.77323523472));
#131053=CARTESIAN_POINT('',(65.9990597672842,-14.4574398737317,64.9541505386072));
#131054=CARTESIAN_POINT('Ctrl Pts',(65.9990597672842,-14.4574398737317,
64.9541505386072));
#131055=CARTESIAN_POINT('Ctrl Pts',(65.9270095132669,-14.457429104092,64.9668321465929));
#131056=CARTESIAN_POINT('Ctrl Pts',(65.8553939405631,-14.4591199027381,
64.9830287465842));
#131057=CARTESIAN_POINT('Ctrl Pts',(65.784532717612,-14.4625090986378,65.0027367719546));
#131058=CARTESIAN_POINT('Ctrl Pts',(65.7329671490077,-14.4649754096384,
65.0170782621515));
#131059=CARTESIAN_POINT('Ctrl Pts',(65.6818011220681,-14.4683401652805,
65.03327966161));
#131060=CARTESIAN_POINT('Ctrl Pts',(65.6311590992478,-14.4725863916555,
65.0513468480837));
#131061=CARTESIAN_POINT('Ctrl Pts',(65.5710420430455,-14.4776270795155,
65.0727943733634));
#131062=CARTESIAN_POINT('Ctrl Pts',(65.5116611670506,-14.4839081718085,
65.0968661895181));
#131063=CARTESIAN_POINT('Ctrl Pts',(65.4532016956852,-14.49136284998,65.123557551863));
#131064=CARTESIAN_POINT('Ctrl Pts',(65.4239719600025,-14.4950901890658,
65.1369032330354));
#131065=CARTESIAN_POINT('Ctrl Pts',(65.3949702682945,-14.4991102138833,
65.1509037399944));
#131066=CARTESIAN_POINT('Ctrl Pts',(65.3662323314153,-14.5034123711069,
65.1655579908485));
#131067=CARTESIAN_POINT('Ctrl Pts',(65.3518633629756,-14.5055634497187,
65.1728851162755));
#131068=CARTESIAN_POINT('Ctrl Pts',(65.3375603353684,-14.5077850356995,
65.1803756897286));
#131069=CARTESIAN_POINT('Ctrl Pts',(65.3233279147348,-14.5100756367114,
65.1880295723925));
#131070=CARTESIAN_POINT('Ctrl Pts',(65.3162117044181,-14.5112209372173,
65.1918565137245));
#131071=CARTESIAN_POINT('Ctrl Pts',(65.3091131459849,-14.5123834898947,
65.1957242831542));
#131072=CARTESIAN_POINT('Ctrl Pts',(65.3020327945485,-14.5135630957985,
65.199632866648));
#131073=CARTESIAN_POINT('Ctrl Pts',(65.294952443112,-14.5147427017023,65.2035414501419));
#131074=CARTESIAN_POINT('Ctrl Pts',(65.2861174085656,-14.5162448133906,
65.2084952227636));
#131075=CARTESIAN_POINT('Ctrl Pts',(65.2808469250696,-14.5171528679838,
65.2114810471074));
#131076=CARTESIAN_POINT('Ctrl Pts',(65.2471863459398,-14.5229522682689,
65.2305503747447));
#131077=CARTESIAN_POINT('Ctrl Pts',(65.2102793351576,-14.529835281351,65.2527723345158));
#131078=CARTESIAN_POINT('Ctrl Pts',(65.170514597363,-14.5379387602517,65.2786049054499));
#131079=CARTESIAN_POINT('Ctrl Pts',(65.1341288410832,-14.5453536515511,
65.3022423712606));
#131080=CARTESIAN_POINT('Ctrl Pts',(65.0953503875563,-14.5537906843503,
65.3289028868235));
#131081=CARTESIAN_POINT('Ctrl Pts',(65.0544797357755,-14.5633146115661,
65.3589526481561));
#131082=CARTESIAN_POINT('Ctrl Pts',(65.0281172728456,-14.5694577526034,
65.3783354004408));
#131083=CARTESIAN_POINT('Ctrl Pts',(65.0008843990089,-14.5760522986969,
65.3991285700309));
#131084=CARTESIAN_POINT('Ctrl Pts',(64.9728624378503,-14.5831045879113,
65.4214342907374));
#131085=CARTESIAN_POINT('Ctrl Pts',(64.934797171896,-14.5926844764499,65.4517345679446));
#131086=CARTESIAN_POINT('Ctrl Pts',(64.8952962752854,-14.6031201309233,
65.4848433642836));
#131087=CARTESIAN_POINT('Ctrl Pts',(64.854649312531,-14.6144275372323,65.5211013146095));
#131088=CARTESIAN_POINT('Ctrl Pts',(64.8317911295075,-14.6207863582958,
65.5414912972415));
#131089=CARTESIAN_POINT('Ctrl Pts',(64.8085705507282,-14.6274200722944,
65.5628774467885));
#131090=CARTESIAN_POINT('Ctrl Pts',(64.7850394363295,-14.634324440184,65.5853223999462));
#131091=CARTESIAN_POINT('Ctrl Pts',(64.7523520864935,-14.6439153794305,
65.6165009503322));
#131092=CARTESIAN_POINT('Ctrl Pts',(64.7190722998677,-14.6540298778063,
65.6497217557215));
#131093=CARTESIAN_POINT('Ctrl Pts',(64.6853904030749,-14.6646369600161,
65.6851483623767));
#131094=CARTESIAN_POINT('Ctrl Pts',(64.6685494546785,-14.6699405011211,
65.7028616657043));
#131095=CARTESIAN_POINT('Ctrl Pts',(64.6516084134835,-14.6753668640736,
65.7211265619829));
#131096=CARTESIAN_POINT('Ctrl Pts',(64.6345938415512,-14.6809100308888,
65.7399643525514));
#131097=CARTESIAN_POINT('Ctrl Pts',(64.626086555585,-14.6836816142964,65.7493832478357));
#131098=CARTESIAN_POINT('Ctrl Pts',(64.6175608885395,-14.686482372973,65.7589453757946));
#131099=CARTESIAN_POINT('Ctrl Pts',(64.6090203879065,-14.6893114063194,
65.7686534527022));
#131100=CARTESIAN_POINT('Ctrl Pts',(64.6011479460988,-14.6919191457656,
65.7776021401157));
#131101=CARTESIAN_POINT('Ctrl Pts',(64.5921868900647,-14.6949139227446,
65.7879309235735));
#131102=CARTESIAN_POINT('Ctrl Pts',(64.5851155508268,-14.6972910105629,
65.7961684881991));
#131103=CARTESIAN_POINT('Ctrl Pts',(64.5845154739129,-14.6974927312659,
65.7968675315051));
#131104=CARTESIAN_POINT('Ctrl Pts',(64.5839290036382,-14.6976900332066,
65.7975515053185));
#131105=CARTESIAN_POINT('Ctrl Pts',(64.5833579591697,-14.6978823175386,
65.7982182831661));
#131106=CARTESIAN_POINT('Ctrl Pts',(64.5249558489375,-14.717547705039,65.8664112795133));
#131107=CARTESIAN_POINT('Ctrl Pts',(64.4695712568179,-14.7373782766372,
65.9376452711858));
#131108=CARTESIAN_POINT('Ctrl Pts',(64.4175227606522,-14.7569885426821,
66.011790428281));
#131109=CARTESIAN_POINT('Ctrl Pts',(64.3914985125693,-14.7667936757046,
66.0488630068287));
#131110=CARTESIAN_POINT('Ctrl Pts',(64.3663083025939,-14.7765435299738,
66.0866634568049));
#131111=CARTESIAN_POINT('Ctrl Pts',(64.3419912851458,-14.7861886364692,
66.1251755013527));
#131112=CARTESIAN_POINT('Ctrl Pts',(64.3298327764217,-14.7910111897169,
66.1444315236266));
#131113=CARTESIAN_POINT('Ctrl Pts',(64.3178925663944,-14.7958075451137,
66.163865447748));
#131114=CARTESIAN_POINT('Ctrl Pts',(64.3061755059024,-14.8005714396201,
66.1834752027238));
#131115=CARTESIAN_POINT('Ctrl Pts',(64.3003169756564,-14.8029533868733,
66.1932800802117));
#131116=CARTESIAN_POINT('Ctrl Pts',(64.2945142328176,-14.8053272182757,
66.2031289155464));
#131117=CARTESIAN_POINT('Ctrl Pts',(64.2887678799285,-14.8076921461525,
66.2130214471302));
#131118=CARTESIAN_POINT('Ctrl Pts',(64.2830215270394,-14.8100570740294,
66.2229139787141));
#131119=CARTESIAN_POINT('Ctrl Pts',(64.2767774131408,-14.8126439219698,
66.2338319698607));
#131120=CARTESIAN_POINT('Ctrl Pts',(64.2716985922896,-14.8147594287093,
66.242829868022));
#131121=CARTESIAN_POINT('Ctrl Pts',(64.2455179843022,-14.8256645687533,
66.2892127689693));
#131122=CARTESIAN_POINT('Ctrl Pts',(64.2186897195521,-14.8367435952576,
66.3383173283336));
#131123=CARTESIAN_POINT('Ctrl Pts',(64.1915599660569,-14.8478672945918,
66.3903785105779));
#131124=CARTESIAN_POINT('Ctrl Pts',(64.1765861418789,-14.8540068386931,
66.4191128295079));
#131125=CARTESIAN_POINT('Ctrl Pts',(64.1615204845469,-14.860159138803,66.4487478811398));
#131126=CARTESIAN_POINT('Ctrl Pts',(64.146421231491,-14.8662955758726,66.479323365031));
#131127=CARTESIAN_POINT('Ctrl Pts',(64.1251931014459,-14.874922829396,66.5223096204327));
#131128=CARTESIAN_POINT('Ctrl Pts',(64.1039048702332,-14.8835197451949,
66.5671536303125));
#131129=CARTESIAN_POINT('Ctrl Pts',(64.0827596108614,-14.8919890457415,
66.6139619949472));
#131130=CARTESIAN_POINT('Ctrl Pts',(64.0721869811755,-14.8962236960148,
66.6373661772646));
#131131=CARTESIAN_POINT('Ctrl Pts',(64.0616505576379,-14.9004261006137,
66.6612614116885));
#131132=CARTESIAN_POINT('Ctrl Pts',(64.0511786752497,-14.9045819186505,
66.6856607382273));
#131133=CARTESIAN_POINT('Ctrl Pts',(64.0459427340556,-14.9066598276688,
66.6978604014967));
#131134=CARTESIAN_POINT('Ctrl Pts',(64.0407229289312,-14.9087260667076,
66.7101860922319));
#131135=CARTESIAN_POINT('Ctrl Pts',(64.0355230345318,-14.9107786956948,
66.7226394085536));
#131136=CARTESIAN_POINT('Ctrl Pts',(64.0329230873321,-14.9118050101884,
66.7288660667144));
#131137=CARTESIAN_POINT('Ctrl Pts',(64.0303281178679,-14.9128279206411,
66.7351246315797));
#131138=CARTESIAN_POINT('Ctrl Pts',(64.0277386058808,-14.9138471750793,
66.7414153025324));
#131139=CARTESIAN_POINT('Ctrl Pts',(64.0251490938937,-14.9148664295174,
66.7477059734851));
#131140=CARTESIAN_POINT('Ctrl Pts',(64.0219496993838,-14.9161234947288,
66.7555455694723));
#131141=CARTESIAN_POINT('Ctrl Pts',(64.0199869263796,-14.9168937119836,
66.7603838331213));
#131142=CARTESIAN_POINT('Ctrl Pts',(63.9930424016886,-14.9274670884227,
66.8268024735216));
#131143=CARTESIAN_POINT('Ctrl Pts',(63.9667351901692,-14.9373914127289,
66.8954367155941));
#131144=CARTESIAN_POINT('Ctrl Pts',(63.9414487228419,-14.9464636582685,
66.9664575673575));
#131145=CARTESIAN_POINT('Ctrl Pts',(63.9170190071715,-14.9552285195738,
67.0350721030613));
#131146=CARTESIAN_POINT('Ctrl Pts',(63.893542086014,-14.9631981366324,67.1059145343941));
#131147=CARTESIAN_POINT('Ctrl Pts',(63.8713619612557,-14.9701418134995,
67.1791290840267));
#131148=CARTESIAN_POINT('Ctrl Pts',(63.8629841166152,-14.9727645690818,
67.20678357781));
#131149=CARTESIAN_POINT('Ctrl Pts',(63.8547912654684,-14.9752404488901,
67.2347763792355));
#131150=CARTESIAN_POINT('Ctrl Pts',(63.8468018538309,-14.9775551290378,
67.2631147380346));
#131151=CARTESIAN_POINT('Ctrl Pts',(63.8212844927312,-14.9849479799559,
67.3536245486764));
#131152=CARTESIAN_POINT('Ctrl Pts',(63.7978340122759,-14.9906976585156,
67.4476669344656));
#131153=CARTESIAN_POINT('Ctrl Pts',(63.7771704812227,-14.994266115557,67.5449460559198));
#131154=CARTESIAN_POINT('Ctrl Pts',(63.7565069501695,-14.9978345725983,
67.642225177374));
#131155=CARTESIAN_POINT('Ctrl Pts',(63.7386304626905,-14.9992212736701,
67.7427415685702));
#131156=CARTESIAN_POINT('Ctrl Pts',(63.7242517575141,-14.9978694334135,
67.8461464768021));
#131157=CARTESIAN_POINT('',(82.7407915597954,-14.4574398738313,62.0021315200116));
#131158=CARTESIAN_POINT('',(83.2822162694133,-14.4574398738744,61.9066637357724));
#131159=CARTESIAN_POINT('',(82.3362806376591,-12.34366528766,59.70878371338));
#131160=CARTESIAN_POINT('Origin',(83.1537660643691,-9.5,64.344226319777));
#131161=CARTESIAN_POINT('',(62.6710204155491,-11.87440155793,62.91980324276));
#131162=CARTESIAN_POINT('Ctrl Pts',(82.3362806376591,-12.34366528766,59.70878371338));
#131163=CARTESIAN_POINT('Ctrl Pts',(81.5289715591157,-12.5189817352091,
59.9597488743679));
#131164=CARTESIAN_POINT('Ctrl Pts',(80.7191589758644,-12.6646044612898,
60.205268368155));
#131165=CARTESIAN_POINT('Ctrl Pts',(79.0922716340717,-12.9033042732495,
60.6726263401023));
#131166=CARTESIAN_POINT('Ctrl Pts',(78.2740835955906,-12.9965399890585,
60.8947778340494));
#131167=CARTESIAN_POINT('Ctrl Pts',(76.6333619159099,-13.1367557266633,
61.3054335510454));
#131168=CARTESIAN_POINT('Ctrl Pts',(75.8144583018363,-13.1835019769691,
61.4930702647479));
#131169=CARTESIAN_POINT('Ctrl Pts',(74.5876982409067,-13.2215047114112,
61.7446398483009));
#131170=CARTESIAN_POINT('Ctrl Pts',(74.1790500717552,-13.2287938444501,
61.8235492499852));
#131171=CARTESIAN_POINT('Ctrl Pts',(73.5664630342142,-13.2317789353712,
61.9343647160185));
#131172=CARTESIAN_POINT('Ctrl Pts',(73.3623319014373,-13.2314474053304,
61.9700470478659));
#131173=CARTESIAN_POINT('Ctrl Pts',(72.9541990694171,-13.2281294125987,
62.0389013302574));
#131174=CARTESIAN_POINT('Ctrl Pts',(72.7513086447414,-13.2251664982903,
62.0718993111952));
#131175=CARTESIAN_POINT('Ctrl Pts',(71.7260750308394,-13.2034383942672,
62.2323964648994));
#131176=CARTESIAN_POINT('Ctrl Pts',(70.901717929154,-13.1646760772142,62.3414667200486));
#131177=CARTESIAN_POINT('Ctrl Pts',(69.6594184975944,-13.0719790447237,
62.4788685448483));
#131178=CARTESIAN_POINT('Ctrl Pts',(69.2443638049454,-13.0352930516122,
62.5203344903412));
#131179=CARTESIAN_POINT('Ctrl Pts',(68.6204663969968,-12.9710473833339,
62.5766946947534));
#131180=CARTESIAN_POINT('Ctrl Pts',(68.3081894608378,-12.9366182519558,
62.6034185783192));
#131181=CARTESIAN_POINT('Ctrl Pts',(67.9433242738696,-12.8922774289481,
62.6322313077126));
#131182=CARTESIAN_POINT('Ctrl Pts',(67.7607607235711,-12.869045168763,62.646072288788));
#131183=CARTESIAN_POINT('Ctrl Pts',(67.6824916428283,-12.8588589471043,
62.6518858367753));
#131184=CARTESIAN_POINT('Ctrl Pts',(67.6303061887625,-12.8520168987905,
62.6557355716152));
#131185=CARTESIAN_POINT('Ctrl Pts',(67.605471099205,-12.848737986768,62.6575557243891));
#131186=CARTESIAN_POINT('Ctrl Pts',(65.8271077618809,-12.6121314762894,
62.7869577419132));
#131187=CARTESIAN_POINT('Ctrl Pts',(64.188516413027,-12.295603114885,62.8572957814988));
#131188=CARTESIAN_POINT('Ctrl Pts',(62.6710204155491,-11.87440155793,62.91980324276));
#131189=CARTESIAN_POINT('',(36.1590071618821,-11.8741528675302,67.5951619717139));
#131190=CARTESIAN_POINT('',(36.1589535195822,-11.8742995089298,67.5948528813764));
#131191=CARTESIAN_POINT('',(35.3959116334435,-12.2791716992138,67.9475259026238));
#131192=CARTESIAN_POINT('Ctrl Pts',(35.3959116334435,-12.2791716992137,
67.9475259026238));
#131193=CARTESIAN_POINT('Ctrl Pts',(35.500819870766,-12.228986514838,67.8990761283221));
#131194=CARTESIAN_POINT('Ctrl Pts',(35.5993587298791,-12.1799558327146,
67.8535278096658));
#131195=CARTESIAN_POINT('Ctrl Pts',(35.6918786734976,-12.1322701611091,
67.8107381519324));
#131196=CARTESIAN_POINT('Ctrl Pts',(35.786399164668,-12.0835533879935,67.7670232586047));
#131197=CARTESIAN_POINT('Ctrl Pts',(35.8746375695955,-12.0362405275576,
67.7261873566712));
#131198=CARTESIAN_POINT('Ctrl Pts',(35.9569194368958,-11.9905098620958,
67.6880679527576));
#131199=CARTESIAN_POINT('Ctrl Pts',(36.0287090291249,-11.9506105995537,
67.6548093922416));
#131200=CARTESIAN_POINT('Ctrl Pts',(36.0959635043088,-11.9119153534715,
67.6236184209543));
#131201=CARTESIAN_POINT('Ctrl Pts',(36.158870968792,-11.874526930468,67.5943834483743));
#131202=CARTESIAN_POINT('Ctrl Pts',(27.2015513459991,-14.9604546753208,
73.5554952088459));
#131203=CARTESIAN_POINT('Ctrl Pts',(27.2537025903662,-14.9462882647007,
73.4244569905557));
#131204=CARTESIAN_POINT('Ctrl Pts',(27.3252684746861,-14.9283662985821,
73.2922068281088));
#131205=CARTESIAN_POINT('Ctrl Pts',(27.412747118424,-14.9070793296614,73.1596515499058));
#131206=CARTESIAN_POINT('Ctrl Pts',(27.4999391612395,-14.8858621019332,
73.0275305544418));
#131207=CARTESIAN_POINT('Ctrl Pts',(27.6029398617996,-14.8613023293257,
72.8951064138094));
#131208=CARTESIAN_POINT('Ctrl Pts',(27.7182733036733,-14.8338054582636,
72.7632297613986));
#131209=CARTESIAN_POINT('Ctrl Pts',(27.8272278175409,-14.8078293998821,
72.6386470183496));
#131210=CARTESIAN_POINT('Ctrl Pts',(27.9470866107628,-14.7792198528575,
72.5144976463921));
#131211=CARTESIAN_POINT('Ctrl Pts',(28.0757305316629,-14.7482215091595,
72.3910614055773));
#131212=CARTESIAN_POINT('Ctrl Pts',(28.2074333096326,-14.7164860960213,
72.2646901343684));
#131213=CARTESIAN_POINT('Ctrl Pts',(28.3483438822667,-14.6822469401442,
72.1390658554838));
#131214=CARTESIAN_POINT('Ctrl Pts',(28.4961857531228,-14.6457145038354,
72.0144742663498));
#131215=CARTESIAN_POINT('Ctrl Pts',(28.5101650783585,-14.642260145433,72.002693393069));
#131216=CARTESIAN_POINT('Ctrl Pts',(28.5242063737892,-14.6387852456508,
71.9909217454062));
#131217=CARTESIAN_POINT('Ctrl Pts',(28.5383077140983,-14.6352899590774,
71.9791595606471));
#131218=CARTESIAN_POINT('Ctrl Pts',(28.6847794480744,-14.5989841417632,
71.8569848198595));
#131219=CARTESIAN_POINT('Ctrl Pts',(28.8377290347631,-14.5604732260721,
71.7358048516294));
#131220=CARTESIAN_POINT('Ctrl Pts',(28.9958806914247,-14.5198822842996,
71.6156910439134));
#131221=CARTESIAN_POINT('Ctrl Pts',(29.1567521931228,-14.4785932716132,
71.4935115547457));
#131222=CARTESIAN_POINT('Ctrl Pts',(29.3230061490674,-14.4351519447313,
71.3724347497099));
#131223=CARTESIAN_POINT('Ctrl Pts',(29.4933006217649,-14.3896366301522,
71.2525403307251));
#131224=CARTESIAN_POINT('Ctrl Pts',(29.5086621111986,-14.3855309007477,
71.2417252007844));
#131225=CARTESIAN_POINT('Ctrl Pts',(29.5240564794304,-14.381408260802,71.2309196977313));
#131226=CARTESIAN_POINT('Ctrl Pts',(29.5394827421391,-14.3772687475314,
71.2201238838441));
#131227=CARTESIAN_POINT('Ctrl Pts',(29.7221144459034,-14.3282610017378,
71.0923121175746));
#131228=CARTESIAN_POINT('Ctrl Pts',(29.9091906174023,-14.2768899174541,
70.9658567538731));
#131229=CARTESIAN_POINT('Ctrl Pts',(30.099730401364,-14.2232101873667,70.840797820168));
#131230=CARTESIAN_POINT('Ctrl Pts',(30.2791033513307,-14.1726764282798,
70.7230681293288));
#131231=CARTESIAN_POINT('Ctrl Pts',(30.4615457919628,-14.1200960307155,
70.6065757634804));
#131232=CARTESIAN_POINT('Ctrl Pts',(30.6462418466383,-14.0654748228539,
70.4913679270501));
#131233=CARTESIAN_POINT('Ctrl Pts',(30.860779879735,-14.0020282780938,70.3575455632291));
#131234=CARTESIAN_POINT('Ctrl Pts',(31.0782473012234,-13.9358160337048,
70.225457787358));
#131235=CARTESIAN_POINT('Ctrl Pts',(31.2978702818636,-13.8668363361836,
70.0951844910434));
#131236=CARTESIAN_POINT('Ctrl Pts',(31.517347052676,-13.7979025605858,69.9649979217014));
#131237=CARTESIAN_POINT('Ctrl Pts',(31.7389764286382,-13.7262046325469,
69.8366229352475));
#131238=CARTESIAN_POINT('Ctrl Pts',(31.9619915002813,-13.6516990359388,
69.710169748752));
#131239=CARTESIAN_POINT('Ctrl Pts',(32.1834412073867,-13.5777164013796,
69.584604149505));
#131240=CARTESIAN_POINT('Ctrl Pts',(32.4062571525262,-13.5009649386618,
69.4609330508715));
#131241=CARTESIAN_POINT('Ctrl Pts',(32.6296949326618,-13.4213670101209,
69.3393010612166));
#131242=CARTESIAN_POINT('Ctrl Pts',(32.7555951577233,-13.3765160582735,
69.2707652260371));
#131243=CARTESIAN_POINT('Ctrl Pts',(32.8816929368142,-13.330760762943,69.2028775008318));
#131244=CARTESIAN_POINT('Ctrl Pts',(33.0078561433856,-13.2840830912989,
69.1356696935853));
#131245=CARTESIAN_POINT('Ctrl Pts',(33.2327786922416,-13.2008665881188,
69.0158522624996));
#131246=CARTESIAN_POINT('Ctrl Pts',(33.4579869112649,-13.1147366014515,
68.8981960536854));
#131247=CARTESIAN_POINT('Ctrl Pts',(33.6828933077903,-13.0255928904122,
68.7829022808979));
#131248=CARTESIAN_POINT('Ctrl Pts',(33.904633708151,-12.9377040509621,68.6692314928191));
#131249=CARTESIAN_POINT('Ctrl Pts',(34.1260806762181,-12.8468852456101,
68.5578568279212));
#131250=CARTESIAN_POINT('Ctrl Pts',(34.3466794893567,-12.7530259357027,
68.4490182347965));
#131251=CARTESIAN_POINT('Ctrl Pts',(34.5618976776729,-12.6614559478706,
68.3428343233877));
#131252=CARTESIAN_POINT('Ctrl Pts',(34.7763085573311,-12.5669914708446,
68.239064142722));
#131253=CARTESIAN_POINT('Ctrl Pts',(34.9894054742867,-12.4695232535759,
68.1379784867459));
#131254=CARTESIAN_POINT('Ctrl Pts',(35.1254955837338,-12.4072771143768,
68.0734221422344));
#131255=CARTESIAN_POINT('Ctrl Pts',(35.2610499665858,-12.3438057886536,
68.0099616468521));
#131256=CARTESIAN_POINT('Ctrl Pts',(35.3959386020984,-12.2790808122887,
67.9476785607999));
#131257=CARTESIAN_POINT('Origin',(58.0359414686091,9.5,68.773176492713));
#131258=CARTESIAN_POINT('',(35.3959428302217,12.2790662096383,67.9477033388501));
#131259=CARTESIAN_POINT('Ctrl Pts',(35.3959384678484,12.2790809112017,67.9476786433073));
#131260=CARTESIAN_POINT('Ctrl Pts',(35.1846027686219,12.38049236243,68.0452626205346));
#131261=CARTESIAN_POINT('Ctrl Pts',(34.971630142807,12.4788242303402,68.1457335657174));
#131262=CARTESIAN_POINT('Ctrl Pts',(34.7575222122605,12.5741879244869,68.2487880787564));
#131263=CARTESIAN_POINT('Ctrl Pts',(34.5399879310559,12.6710777155668,68.3534917642369));
#131264=CARTESIAN_POINT('Ctrl Pts',(34.3212817528117,12.7649041083006,68.4608625658059));
#131265=CARTESIAN_POINT('Ctrl Pts',(34.1019392637244,12.8557816179673,68.5706361300887));
#131266=CARTESIAN_POINT('Ctrl Pts',(33.8777656711369,12.9486607400751,68.6828274997536));
#131267=CARTESIAN_POINT('Ctrl Pts',(33.6529274636052,13.0384601940759,68.7975288373825));
#131268=CARTESIAN_POINT('Ctrl Pts',(33.4280057224191,13.1252915128353,68.9145107933281));
#131269=CARTESIAN_POINT('Ctrl Pts',(33.2879527170998,13.1793591502455,68.9873524599982));
#131270=CARTESIAN_POINT('Ctrl Pts',(33.1478675064981,13.2322757250493,69.061079411678));
#131271=CARTESIAN_POINT('Ctrl Pts',(33.0078920406793,13.2840647581322,69.1356457047561));
#131272=CARTESIAN_POINT('Ctrl Pts',(32.7838505729871,13.3669570772566,69.2549947752798));
#131273=CARTESIAN_POINT('Ctrl Pts',(32.5600163098531,13.4469415289604,69.3764846407735));
#131274=CARTESIAN_POINT('Ctrl Pts',(32.3371306874339,13.5241132751291,69.4999469835736));
#131275=CARTESIAN_POINT('Ctrl Pts',(32.1131440080578,13.6016662504102,69.6240192314451));
#131276=CARTESIAN_POINT('Ctrl Pts',(31.8901154401888,13.6763791066002,69.7500839185269));
#131277=CARTESIAN_POINT('Ctrl Pts',(31.6688047376244,13.7483162091762,69.8780114798589));
#131278=CARTESIAN_POINT('Ctrl Pts',(31.4471601729343,13.8203618337246,70.0061320285479));
#131279=CARTESIAN_POINT('Ctrl Pts',(31.2272387427077,13.8896237244916,70.136121542552));
#131280=CARTESIAN_POINT('Ctrl Pts',(31.0098097350917,13.9561279803308,70.267884411958));
#131281=CARTESIAN_POINT('Ctrl Pts',(30.8877961052469,13.9934478657685,70.3418251715248));
#131282=CARTESIAN_POINT('Ctrl Pts',(30.7665674583,14.0298986263602,70.4163249544217));
#131283=CARTESIAN_POINT('Ctrl Pts',(30.6462604266937,14.0654788649446,70.4913707665092));
#131284=CARTESIAN_POINT('Ctrl Pts',(30.4507151912467,14.1233104483389,70.6133490980999));
#131285=CARTESIAN_POINT('Ctrl Pts',(30.2576886721935,14.1788533664209,70.7367664634594));
#131286=CARTESIAN_POINT('Ctrl Pts',(30.0681599843068,14.2321011530085,70.861568004652));
#131287=CARTESIAN_POINT('Ctrl Pts',(29.8885216001801,14.2825702743198,70.9798569425765));
#131288=CARTESIAN_POINT('Ctrl Pts',(29.7120256014514,14.3309774346097,71.0993898650131));
#131289=CARTESIAN_POINT('Ctrl Pts',(29.5395081699614,14.3772763216838,71.2201341766509));
#131290=CARTESIAN_POINT('Ctrl Pts',(29.3622416148093,14.4248497416456,71.3442023823584));
#131291=CARTESIAN_POINT('Ctrl Pts',(29.1891821649001,14.470197093175,71.4695456224595));
#131292=CARTESIAN_POINT('Ctrl Pts',(29.0218222185181,14.5132384215319,71.5960808254033));
#131293=CARTESIAN_POINT('Ctrl Pts',(28.8640265888147,14.5538200162215,71.7153847715375));
#131294=CARTESIAN_POINT('Ctrl Pts',(28.7112977339314,14.5923513952753,71.8357488452308));
#131295=CARTESIAN_POINT('Ctrl Pts',(28.5648874571433,14.6287141046279,71.9571086643009));
#131296=CARTESIAN_POINT('Ctrl Pts',(28.5560132300508,14.630918123004,71.9644645317848));
#131297=CARTESIAN_POINT('Ctrl Pts',(28.547162216342,14.6331141581006,71.9718240578045));
#131298=CARTESIAN_POINT('Ctrl Pts',(28.5383346947726,14.635302177299,71.9791872280613));
#131299=CARTESIAN_POINT('Ctrl Pts',(28.3838674613872,14.6735889455064,72.1080307012333));
#131300=CARTESIAN_POINT('Ctrl Pts',(28.2366363763939,14.7094295606917,72.2379913483665));
#131301=CARTESIAN_POINT('Ctrl Pts',(28.0991271518032,14.7426018475479,72.3687793402463));
#131302=CARTESIAN_POINT('Ctrl Pts',(27.9715295101533,14.7733830957412,72.4901402116327));
#131303=CARTESIAN_POINT('Ctrl Pts',(27.8523028105917,14.8018663841165,72.6122138209336));
#131304=CARTESIAN_POINT('Ctrl Pts',(27.743431052339,14.827824076867,72.7347571512724));
#131305=CARTESIAN_POINT('Ctrl Pts',(27.7349740663958,14.8298404293741,72.7442761233066));
#131306=CARTESIAN_POINT('Ctrl Pts',(27.7265795601537,14.8318415175968,72.753797921904));
#131307=CARTESIAN_POINT('Ctrl Pts',(27.7182484627975,14.833827222121,72.7633224290272));
#131308=CARTESIAN_POINT('Ctrl Pts',(27.6026668404061,14.8613759279739,72.8954608423381));
#131309=CARTESIAN_POINT('Ctrl Pts',(27.499559649583,14.8859752343313,73.0281296908167));
#131310=CARTESIAN_POINT('Ctrl Pts',(27.4123172044704,14.9072171780113,73.1604861524754));
#131311=CARTESIAN_POINT('Ctrl Pts',(27.3250747593577,14.9284591216913,73.2928426141342));
#131312=CARTESIAN_POINT('Ctrl Pts',(27.2536970570319,14.946343257526,73.4248866723926));
#131313=CARTESIAN_POINT('Ctrl Pts',(27.2015660065188,14.9604820182035,73.5557278374816));
#131314=CARTESIAN_POINT('',(36.1590567380064,11.8740010057512,67.5954592543057));
#131315=CARTESIAN_POINT('Ctrl Pts',(36.1588385012177,11.8746149117224,67.5942070353847));
#131316=CARTESIAN_POINT('Ctrl Pts',(36.0248459115227,11.9546473040868,67.6567966276318));
#131317=CARTESIAN_POINT('Ctrl Pts',(35.8850483327633,12.0328525721753,67.7221131308698));
#131318=CARTESIAN_POINT('Ctrl Pts',(35.7391385019241,12.1090378043059,67.7897526024016));
#131319=CARTESIAN_POINT('Ctrl Pts',(35.6283105785524,12.1669053997931,67.8411291417665));
#131320=CARTESIAN_POINT('Ctrl Pts',(35.5139562241468,12.2236075905504,67.8938446914323));
#131321=CARTESIAN_POINT('Ctrl Pts',(35.3959428302217,12.2790662096383,67.9477033388501));
#131322=CARTESIAN_POINT('',(62.6710208743191,11.87440113975,62.91980295862));
#131323=CARTESIAN_POINT('',(36.1589529072075,11.874300349392,67.5948533979391));
#131324=CARTESIAN_POINT('',(82.3364382228178,12.3433341995235,59.7089279795811));
#131325=CARTESIAN_POINT('Ctrl Pts',(62.6710208743191,11.87440113975,62.91980295862));
#131326=CARTESIAN_POINT('Ctrl Pts',(63.4281166754305,12.0846306344014,62.8888133082932));
#131327=CARTESIAN_POINT('Ctrl Pts',(64.2163274555045,12.2690616559132,62.8560593750203));
#131328=CARTESIAN_POINT('Ctrl Pts',(65.4435012996331,12.5103870064531,62.7939898400575));
#131329=CARTESIAN_POINT('Ctrl Pts',(65.8600410701228,12.584956407583,62.7711749943272));
#131330=CARTESIAN_POINT('Ctrl Pts',(66.4958864972862,12.6885240050038,62.7327049090558));
#131331=CARTESIAN_POINT('Ctrl Pts',(66.8165686353613,12.7382365709795,62.7124106437459));
#131332=CARTESIAN_POINT('Ctrl Pts',(67.195490824901,12.7927258737427,62.6866763968924));
#131333=CARTESIAN_POINT('Ctrl Pts',(67.3861460351238,12.8191077763637,62.6732713839456));
#131334=CARTESIAN_POINT('Ctrl Pts',(67.4681108568743,12.8302309673599,62.6674086440074));
#131335=CARTESIAN_POINT('Ctrl Pts',(67.5228107896359,12.8376058562909,62.6634737181123));
#131336=CARTESIAN_POINT('Ctrl Pts',(67.5514629683228,12.8414425243988,62.6614003567288));
#131337=CARTESIAN_POINT('Ctrl Pts',(68.4138456274695,12.9561983158044,62.5986558946661));
#131338=CARTESIAN_POINT('Ctrl Pts',(69.2465420140072,13.0411633210121,62.5245233792394));
#131339=CARTESIAN_POINT('Ctrl Pts',(70.4891530095295,13.1339297429258,62.3871328855657));
#131340=CARTESIAN_POINT('Ctrl Pts',(70.902291431658,13.1590527041346,62.337010585665));
#131341=CARTESIAN_POINT('Ctrl Pts',(71.726331983732,13.1982235913239,62.227514992348));
#131342=CARTESIAN_POINT('Ctrl Pts',(72.1385502864971,13.2122999760018,62.1679361496933));
#131343=CARTESIAN_POINT('Ctrl Pts',(74.1807440478251,13.2554807810021,61.8481459426687));
#131344=CARTESIAN_POINT('Ctrl Pts',(75.8173705513391,13.206865618323,61.5099893968683));
#131345=CARTESIAN_POINT('Ctrl Pts',(79.0977809214279,12.9263175231934,60.6887657913152));
#131346=CARTESIAN_POINT('Ctrl Pts',(80.7213342216137,12.694823500819,60.2100114146928));
#131347=CARTESIAN_POINT('Ctrl Pts',(82.3365243969791,12.34303336447,59.70941850923));
#131348=CARTESIAN_POINT('',(82.7407915597713,14.4574398737622,62.0021315198703));
#131349=CARTESIAN_POINT('Origin',(83.1537660643691,9.5,64.344226319776));
#131350=CARTESIAN_POINT('',(65.9990597676261,14.4574398737488,64.9541505385815));
#131351=CARTESIAN_POINT('',(65.617923889253,14.4574398737354,65.021355077224));
#131352=CARTESIAN_POINT('Ctrl Pts',(63.7242517378918,14.9978694345806,67.8461463931036));
#131353=CARTESIAN_POINT('Ctrl Pts',(63.7337825611654,14.998764850968,67.7776529607607));
#131354=CARTESIAN_POINT('Ctrl Pts',(63.7449416159549,14.9985039978351,67.7066972644362));
#131355=CARTESIAN_POINT('Ctrl Pts',(63.7581983113509,14.9968754692981,67.6336509130626));
#131356=CARTESIAN_POINT('Ctrl Pts',(63.771015396592,14.9953009449952,67.5630268786308));
#131357=CARTESIAN_POINT('Ctrl Pts',(63.7857933628015,14.9924477215874,67.4904488594246));
#131358=CARTESIAN_POINT('Ctrl Pts',(63.802958556956,14.9881719476635,67.4162646465039));
#131359=CARTESIAN_POINT('Ctrl Pts',(63.8117053466523,14.9859931610466,67.378462935474));
#131360=CARTESIAN_POINT('Ctrl Pts',(63.8210720260374,14.9834457896389,67.340244331803));
#131361=CARTESIAN_POINT('Ctrl Pts',(63.8311151525638,14.9805159890665,67.301655683593));
#131362=CARTESIAN_POINT('Ctrl Pts',(63.8436495338607,14.9768594347652,67.2534949012788));
#131363=CARTESIAN_POINT('Ctrl Pts',(63.8572423152196,14.9726097528716,67.2047923803538));
#131364=CARTESIAN_POINT('Ctrl Pts',(63.8719889212853,14.9677502820913,67.1556379765422));
#131365=CARTESIAN_POINT('Ctrl Pts',(63.8756755728017,14.9665354143963,67.1433493755893));
#131366=CARTESIAN_POINT('Ctrl Pts',(63.8794342263518,14.9652824508048,67.1310322852469));
#131367=CARTESIAN_POINT('Ctrl Pts',(63.8832662473991,14.9639911935129,67.1186879620414));
#131368=CARTESIAN_POINT('Ctrl Pts',(63.8851822579228,14.963345564867,67.1125158004387));
#131369=CARTESIAN_POINT('Ctrl Pts',(63.8871190274097,14.9626890327076,67.1063445400929));
#131370=CARTESIAN_POINT('Ctrl Pts',(63.8881246655709,14.9623466418033,67.1031452704268));
#131371=CARTESIAN_POINT('Ctrl Pts',(63.889130303732,14.962004250899,67.0999460007607));
#131372=CARTESIAN_POINT('Ctrl Pts',(63.8901472151135,14.9616562478876,67.0967169599364));
#131373=CARTESIAN_POINT('Ctrl Pts',(63.8911756672465,14.9613025150278,67.0934582802534));
#131374=CARTESIAN_POINT('Ctrl Pts',(63.8952894757787,14.9598875835887,67.0804235615214));
#131375=CARTESIAN_POINT('Ctrl Pts',(63.8995879358875,14.9583809988961,67.0669146185049));
#131376=CARTESIAN_POINT('Ctrl Pts',(63.9040893584918,14.9567751639957,67.0529409938371));
#131377=CARTESIAN_POINT('Ctrl Pts',(63.9220950489092,14.950351824394,66.9970464951659));
#131378=CARTESIAN_POINT('Ctrl Pts',(63.9433324465097,14.9423392673845,66.9336940725849));
#131379=CARTESIAN_POINT('Ctrl Pts',(63.9691124192012,14.9322462007947,66.8636663834272));
#131380=CARTESIAN_POINT('Ctrl Pts',(63.9892714061719,14.9243537953096,66.8089073155952));
#131381=CARTESIAN_POINT('Ctrl Pts',(64.0122117937822,14.9151735758559,66.7499932158726));
#131382=CARTESIAN_POINT('Ctrl Pts',(64.0386276242206,14.9045267344321,66.6875743978673));
#131383=CARTESIAN_POINT('Ctrl Pts',(64.0626328772686,14.8948514708384,66.6308516109511));
#131384=CARTESIAN_POINT('Ctrl Pts',(64.0895082802585,14.8839646264364,66.5712349562864));
#131385=CARTESIAN_POINT('Ctrl Pts',(64.1197755996161,14.8717745154457,66.5092176688769));
#131386=CARTESIAN_POINT('Ctrl Pts',(64.1413890174507,14.86306974846,66.4649320970391));
#131387=CARTESIAN_POINT('Ctrl Pts',(64.1647320513516,14.8537012799868,66.4194225295541));
#131388=CARTESIAN_POINT('Ctrl Pts',(64.1899947219018,14.8436522220047,66.3728687534608));
#131389=CARTESIAN_POINT('Ctrl Pts',(64.2208107999915,14.8313941135482,66.3160812180094));
#131390=CARTESIAN_POINT('Ctrl Pts',(64.2544746774233,14.8181382068145,66.2578139673371));
#131391=CARTESIAN_POINT('Ctrl Pts',(64.2913278249673,14.8039250787308,66.1984992639139));
#131392=CARTESIAN_POINT('Ctrl Pts',(64.3140132909143,14.7951759906709,66.1619872758115));
#131393=CARTESIAN_POINT('Ctrl Pts',(64.3379072085807,14.7860651649021,66.12507825814));
#131394=CARTESIAN_POINT('Ctrl Pts',(64.3630889037512,14.7766117776763,66.0878712102795));
#131395=CARTESIAN_POINT('Ctrl Pts',(64.3961339207526,14.764206443584,66.0390457630331));
#131396=CARTESIAN_POINT('Ctrl Pts',(64.4313982390898,14.7512094777188,65.989704540002));
#131397=CARTESIAN_POINT('Ctrl Pts',(64.4690558065301,14.7376915386291,65.9400894217365));
#131398=CARTESIAN_POINT('Ctrl Pts',(64.4878845902503,14.7309325690842,65.9152818626037));
#131399=CARTESIAN_POINT('Ctrl Pts',(64.5073115484353,14.7240438671898,65.8904061716917));
#131400=CARTESIAN_POINT('Ctrl Pts',(64.5273575133116,14.7170375583601,65.8654948206653));
#131401=CARTESIAN_POINT('Ctrl Pts',(64.5373804957498,14.7135344039452,65.8530391451521));
#131402=CARTESIAN_POINT('Ctrl Pts',(64.5475582283756,14.7100018734831,65.840574546187));
#131403=CARTESIAN_POINT('Ctrl Pts',(64.5578932426902,14.7064417183732,65.8281052748378));
#131404=CARTESIAN_POINT('Ctrl Pts',(64.5630607498474,14.7046616408183,65.8218706391632));
#131405=CARTESIAN_POINT('Ctrl Pts',(64.5682675773319,14.7028746588143,65.8156348348536));
#131406=CARTESIAN_POINT('Ctrl Pts',(64.5735140388626,14.701081004319,65.8093983984261));
#131407=CARTESIAN_POINT('Ctrl Pts',(64.5787605003933,14.6992873498238,65.8031619619987));
#131408=CARTESIAN_POINT('Ctrl Pts',(64.5850099785308,14.6971602131997,65.7957967052526));
#131409=CARTESIAN_POINT('Ctrl Pts',(64.5893726377915,14.695680263695,65.790687731514));
#131410=CARTESIAN_POINT('Ctrl Pts',(64.6293285984423,14.6821259609999,65.7438965563464));
#131411=CARTESIAN_POINT('Ctrl Pts',(64.6689335996178,14.6691901554928,65.7004189411246));
#131412=CARTESIAN_POINT('Ctrl Pts',(64.7079063914946,14.6569598950792,65.6599692986373));
#131413=CARTESIAN_POINT('Ctrl Pts',(64.7483012578738,14.6442833658546,65.6180436929858));
#131414=CARTESIAN_POINT('Ctrl Pts',(64.7880169175196,14.6323643974131,65.5793709618982));
#131415=CARTESIAN_POINT('Ctrl Pts',(64.826742420664,14.621243752578,65.5436457176895));
#131416=CARTESIAN_POINT('Ctrl Pts',(64.8678098352823,14.6094505905741,65.5057600016334));
#131417=CARTESIAN_POINT('Ctrl Pts',(64.9077636973584,14.5985549248645,65.4711889571079));
#131418=CARTESIAN_POINT('Ctrl Pts',(64.9462359138267,14.5885487374807,65.43958397432));
#131419=CARTESIAN_POINT('Ctrl Pts',(64.9587773526386,14.585286851415,65.4292811637681));
#131420=CARTESIAN_POINT('Ctrl Pts',(64.9711613623282,14.5821190820351,65.4192936715562));
#131421=CARTESIAN_POINT('Ctrl Pts',(64.983375252308,14.5790440470746,65.4096097661362));
#131422=CARTESIAN_POINT('Ctrl Pts',(65.0252691727882,14.5684966072071,65.3763937502495));
#131423=CARTESIAN_POINT('Ctrl Pts',(65.0652298005112,14.5590473736055,65.3467438621354));
#131424=CARTESIAN_POINT('Ctrl Pts',(65.1029270992231,14.5506453301593,65.3202694661502));
#131425=CARTESIAN_POINT('Ctrl Pts',(65.1188141328085,14.54710439882,65.3091121781603));
#131426=CARTESIAN_POINT('Ctrl Pts',(65.1342992176172,14.5437488222219,65.2985191076289));
#131427=CARTESIAN_POINT('Ctrl Pts',(65.1493578101058,14.5405722609322,65.2884619225297));
#131428=CARTESIAN_POINT('Ctrl Pts',(65.1747528789681,14.5352152534457,65.2715013129411));
#131429=CARTESIAN_POINT('Ctrl Pts',(65.1989388090877,14.5303694416143,65.2560677928051));
#131430=CARTESIAN_POINT('Ctrl Pts',(65.2218214051471,14.5260066845789,65.2420469573045));
#131431=CARTESIAN_POINT('Ctrl Pts',(65.2332627031767,14.5238253060612,65.2350365395543));
#131432=CARTESIAN_POINT('Ctrl Pts',(65.2443784165704,14.5217646555267,65.2283795358765));
#131433=CARTESIAN_POINT('Ctrl Pts',(65.2551582593996,14.5198210938599,65.2220630808855));
#131434=CARTESIAN_POINT('Ctrl Pts',(65.2605481808143,14.5188493130265,65.21890485339));
#131435=CARTESIAN_POINT('Ctrl Pts',(65.2658541351246,14.5179067975575,65.2158317661106));
#131436=CARTESIAN_POINT('Ctrl Pts',(65.2710749504499,14.5169931010738,65.2128423158431));
#131437=CARTESIAN_POINT('Ctrl Pts',(65.2762957657751,14.5160794045901,65.2098528655756));
#131438=CARTESIAN_POINT('Ctrl Pts',(65.2799085769594,14.5154528431045,65.2077986373233));
#131439=CARTESIAN_POINT('Ctrl Pts',(65.2864808157042,14.5143380012837,65.204123389393));
#131440=CARTESIAN_POINT('Ctrl Pts',(65.3567384846777,14.5024202681267,65.1648347447609));
#131441=CARTESIAN_POINT('Ctrl Pts',(65.4303996117143,14.4920729911742,65.1290510718699));
#131442=CARTESIAN_POINT('Ctrl Pts',(65.5070958740645,14.483608530346,65.0970873481068));
#131443=CARTESIAN_POINT('Ctrl Pts',(65.5795143800122,14.4756161772894,65.0669064103594));
#131444=CARTESIAN_POINT('Ctrl Pts',(65.6546388188878,14.4693028578232,65.0401307723377));
#131445=CARTESIAN_POINT('Ctrl Pts',(65.7321620506938,14.4648886760428,65.0170421886093));
#131446=CARTESIAN_POINT('Ctrl Pts',(65.8049708097341,14.4607429368867,64.9953577065501));
#131447=CARTESIAN_POINT('Ctrl Pts',(65.8798954386498,14.4582725686681,64.9769252656061));
#131448=CARTESIAN_POINT('Ctrl Pts',(65.9566848864551,14.4576170913444,64.9619975203067));
#131449=CARTESIAN_POINT('Ctrl Pts',(65.9707478015117,14.4574970498258,64.9592637122102));
#131450=CARTESIAN_POINT('Ctrl Pts',(65.9848732708248,14.4574377505937,64.9566475067169));
#131451=CARTESIAN_POINT('Ctrl Pts',(65.9990597670304,14.4574398737327,64.9541505386571));
#131452=CARTESIAN_POINT('Ctrl Pts',(25.8674011700191,-10.80158154637,60.29014909768));
#131453=CARTESIAN_POINT('Ctrl Pts',(25.9483639155891,-10.67317627998,60.2578289519001));
#131454=CARTESIAN_POINT('Ctrl Pts',(26.1402448136891,-10.34972776486,60.17641841982));
#131455=CARTESIAN_POINT('Ctrl Pts',(26.4133227121591,-9.809477103913,60.04060145495));
#131456=CARTESIAN_POINT('Ctrl Pts',(26.6746608848491,-9.173794293496,59.88240498685));
#131457=CARTESIAN_POINT('Ctrl Pts',(26.8930528742491,-8.50966725041199,
59.72121052569));
#131458=CARTESIAN_POINT('Ctrl Pts',(27.0742534024791,-7.80453902184299,
59.5573550630001));
#131459=CARTESIAN_POINT('Ctrl Pts',(27.2212200353591,-7.04916242399599,
59.39317676603));
#131460=CARTESIAN_POINT('Ctrl Pts',(27.3357604796091,-6.23957271011399,
59.23300930155));
#131461=CARTESIAN_POINT('Ctrl Pts',(27.4201508701391,-5.37834024197199,
59.08272261093));
#131462=CARTESIAN_POINT('Ctrl Pts',(27.4783655117691,-4.47147007015,58.94826811738));
#131463=CARTESIAN_POINT('Ctrl Pts',(27.5154691587491,-3.53139160346499,
58.8354266391701));
#131464=CARTESIAN_POINT('Ctrl Pts',(27.5369855402391,-2.57512600928299,
58.74841910647));
#131465=CARTESIAN_POINT('Ctrl Pts',(27.5481191645691,-1.62102984739999,
58.68926281351));
#131466=CARTESIAN_POINT('Ctrl Pts',(27.5529848278191,-0.692828865468586,
58.65792260557));
#131467=CARTESIAN_POINT('Ctrl Pts',(27.5536467947491,-0.0610093872017058,
58.65357386177));
#131468=CARTESIAN_POINT('Ctrl Pts',(27.5533212468091,0.257051205251114,
58.6558663386));
#131469=CARTESIAN_POINT('Ctrl Pts',(27.5532919224291,0.281757260524914,
58.65607129804));
#131470=CARTESIAN_POINT('Ctrl Pts',(27.8395702403391,-9.323660637594,64.630699852874));
#131471=CARTESIAN_POINT('Ctrl Pts',(27.9330797739191,-9.212845822649,64.59866767931));
#131472=CARTESIAN_POINT('Ctrl Pts',(28.1541305252591,-8.93370631904499,
64.518698253699));
#131473=CARTESIAN_POINT('Ctrl Pts',(28.4665607003691,-8.46745880057699,
64.388043824903));
#131474=CARTESIAN_POINT('Ctrl Pts',(28.7630789213891,-7.91883929150999,
64.23908399161));
#131475=CARTESIAN_POINT('Ctrl Pts',(29.0088575136291,-7.34565535370899,
64.0899266273461));
#131476=CARTESIAN_POINT('Ctrl Pts',(29.2112030172591,-6.737065109368,63.940452046196));
#131477=CARTESIAN_POINT('Ctrl Pts',(29.3742190560191,-6.08508333800299,
63.792406643038));
#131478=CARTESIAN_POINT('Ctrl Pts',(29.5006182945091,-5.386284106142,63.649329525158));
#131479=CARTESIAN_POINT('Ctrl Pts',(29.5935058932791,-4.64288310331099,
63.516088541777));
#131480=CARTESIAN_POINT('Ctrl Pts',(29.6576464719891,-3.86006210124599,
63.3975884347841));
#131481=CARTESIAN_POINT('Ctrl Pts',(29.6988058455691,-3.04855202192599,
63.298576769657));
#131482=CARTESIAN_POINT('Ctrl Pts',(29.7230108418491,-2.22304983625699,
63.222478230382));
#131483=CARTESIAN_POINT('Ctrl Pts',(29.7357938430891,-1.39940580633199,
63.170853244553));
#131484=CARTESIAN_POINT('Ctrl Pts',(29.7414883797391,-0.598107824388886,
63.143535409107));
#131485=CARTESIAN_POINT('Ctrl Pts',(29.7422638030691,-0.0526681594190058,
63.139745384407));
#131486=CARTESIAN_POINT('Ctrl Pts',(29.7418782228891,0.221908182666614,
63.1417428011591));
#131487=CARTESIAN_POINT('Ctrl Pts',(29.7418435361591,0.243236501092214,
63.141921385014));
#131488=CARTESIAN_POINT('Ctrl Pts',(31.8804542988291,-9.85977556851199,
67.511305247789));
#131489=CARTESIAN_POINT('Ctrl Pts',(32.0040134654391,-9.72150630571099,
67.442225131604));
#131490=CARTESIAN_POINT('Ctrl Pts',(32.2941843453491,-9.37393636982899,
67.27417511811));
#131491=CARTESIAN_POINT('Ctrl Pts',(32.6971211611091,-8.7987533155,67.018567541111));
#131492=CARTESIAN_POINT('Ctrl Pts',(33.0712071741991,-8.13380665328499,
66.752472039828));
#131493=CARTESIAN_POINT('Ctrl Pts',(33.3743008109591,-7.45473129633099,
66.508910810442));
#131494=CARTESIAN_POINT('Ctrl Pts',(33.6180362316491,-6.75303160889099,
66.285205978187));
#131495=CARTESIAN_POINT('Ctrl Pts',(33.8098260170691,-6.02348256075299,
66.081109857837));
#131496=CARTESIAN_POINT('Ctrl Pts',(33.9551252743891,-5.26605698609299,
65.898363870823));
#131497=CARTESIAN_POINT('Ctrl Pts',(34.0595863091591,-4.48602846810799,
65.739583721531));
#131498=CARTESIAN_POINT('Ctrl Pts',(34.1303183702891,-3.69048826277099,
65.60678565305));
#131499=CARTESIAN_POINT('Ctrl Pts',(34.1750618306191,-2.88866222149599,
65.501251127434));
#131500=CARTESIAN_POINT('Ctrl Pts',(34.2011679964491,-2.09146054688399,
65.423232491143));
#131501=CARTESIAN_POINT('Ctrl Pts',(34.2149297644291,-1.31041085152599,
65.371822179204));
#131502=CARTESIAN_POINT('Ctrl Pts',(34.2210737681691,-0.558921368337586,
65.3450673699811));
#131503=CARTESIAN_POINT('Ctrl Pts',(34.2219093654591,-0.0494594423831458,
65.341370578215));
#131504=CARTESIAN_POINT('Ctrl Pts',(34.2214919003791,0.207288115816814,
65.3433200745641));
#131505=CARTESIAN_POINT('Ctrl Pts',(34.2214543888891,0.227233674714814,
65.3434944532351));
#131506=CARTESIAN_POINT('Ctrl Pts',(36.2923205729991,-12.18468357669,67.721710765645));
#131507=CARTESIAN_POINT('Ctrl Pts',(36.4508071964791,-11.98544964953,67.593812075596));
#131508=CARTESIAN_POINT('Ctrl Pts',(36.8210084222691,-11.48546012732,67.285165865292));
#131509=CARTESIAN_POINT('Ctrl Pts',(37.3275808780091,-10.6641709201,66.8269871398981));
#131510=CARTESIAN_POINT('Ctrl Pts',(37.7890331764291,-9.72838021784798,
66.366596924014));
#131511=CARTESIAN_POINT('Ctrl Pts',(38.1552900169491,-8.79106802662099,
65.961853607951));
#131512=CARTESIAN_POINT('Ctrl Pts',(38.4432707802091,-7.84573037211999,
65.606494411466));
#131513=CARTESIAN_POINT('Ctrl Pts',(38.6644696814491,-6.89024097792099,
65.297713052213));
#131514=CARTESIAN_POINT('Ctrl Pts',(38.8277695481891,-5.92940344555999,
65.035205417231));
#131515=CARTESIAN_POINT('Ctrl Pts',(38.9420177955091,-4.97367707759999,
64.819031227146));
#131516=CARTESIAN_POINT('Ctrl Pts',(39.0172375459191,-4.03399312862899,
64.647689979609));
#131517=CARTESIAN_POINT('Ctrl Pts',(39.0635876386991,-3.11889813453199,
64.518020427672));
#131518=CARTESIAN_POINT('Ctrl Pts',(39.0900087734791,-2.23564392661399,
64.426059311459));
#131519=CARTESIAN_POINT('Ctrl Pts',(39.1036674799791,-1.39143522956399,
64.367456847303));
#131520=CARTESIAN_POINT('Ctrl Pts',(39.1096927058991,-0.591733253689086,
64.337569168795));
#131521=CARTESIAN_POINT('Ctrl Pts',(39.1105099132791,-0.0527313430901759,
64.333460953008));
#131522=CARTESIAN_POINT('Ctrl Pts',(39.1101021067291,0.219333464190314,
64.335629801855));
#131523=CARTESIAN_POINT('Ctrl Pts',(39.1100654948391,0.240472192012714,
64.335823912502));
#131524=CARTESIAN_POINT('',(28.7120116773549,-9.91584041054405,64.1367640219333));
#131525=CARTESIAN_POINT('Ctrl Pts',(30.8903812387966,-6.76809619335577,
63.752816963338));
#131526=CARTESIAN_POINT('Ctrl Pts',(30.605546535352,-7.34848963938884,63.8030410065974));
#131527=CARTESIAN_POINT('Ctrl Pts',(30.2797662869634,-7.90595274493995,
63.8604848541702));
#131528=CARTESIAN_POINT('Ctrl Pts',(29.5502034758413,-8.9598024251586,63.9891264618925));
#131529=CARTESIAN_POINT('Ctrl Pts',(29.1494368108939,-9.45399235856436,
64.0597924378913));
#131530=CARTESIAN_POINT('Ctrl Pts',(28.7116284843023,-9.91532477875859,
64.1369898582482));
#131531=CARTESIAN_POINT('Ctrl Pts',(29.6609510243113,-9.94007378487892,
64.9665024957973));
#131532=CARTESIAN_POINT('Ctrl Pts',(31.6715154505519,-10.0843062537526,
66.5643539924829));
#131533=CARTESIAN_POINT('Ctrl Pts',(33.9364614048553,-10.773624544685,67.4539976470912));
#131534=CARTESIAN_POINT('Ctrl Pts',(36.1591009162391,-11.87389313049,67.595688809357));
#131535=CARTESIAN_POINT('',(38.8135870865772,3.00384514409506E-5,64.3914459142308));
#131536=CARTESIAN_POINT('Ctrl Pts',(36.1592915186016,-11.873367524377,67.5967699365276));
#131537=CARTESIAN_POINT('Ctrl Pts',(36.2669689976408,-11.7330105239143,
67.5095497815776));
#131538=CARTESIAN_POINT('Ctrl Pts',(36.3709096198074,-11.5904287102527,
67.4233916251011));
#131539=CARTESIAN_POINT('Ctrl Pts',(36.4710609268351,-11.4457706775564,
67.338483268842));
#131540=CARTESIAN_POINT('Ctrl Pts',(36.6764809564459,-11.1490630434591,
67.1643280074219));
#131541=CARTESIAN_POINT('Ctrl Pts',(36.8659592292947,-10.8436207467023,
66.9954307180623));
#131542=CARTESIAN_POINT('Ctrl Pts',(37.0396680152484,-10.5307740965049,
66.833093734618));
#131543=CARTESIAN_POINT('Ctrl Pts',(37.2050431549548,-10.2329362053525,
66.6785448373402));
#131544=CARTESIAN_POINT('Ctrl Pts',(37.3561256133158,-9.92838738276226,
66.529941885612));
#131545=CARTESIAN_POINT('Ctrl Pts',(37.4934100494082,-9.61845064646555,
66.3882186911218));
#131546=CARTESIAN_POINT('Ctrl Pts',(37.5647540297729,-9.45738271292513,
66.3145679766437));
#131547=CARTESIAN_POINT('Ctrl Pts',(37.6323716366623,-9.29485967912372,
66.2427752450919));
#131548=CARTESIAN_POINT('Ctrl Pts',(37.6963876506001,-9.13107418210396,
66.1729346611957));
#131549=CARTESIAN_POINT('Ctrl Pts',(37.7517279747585,-8.98948550858375,
66.1125591345973));
#131550=CARTESIAN_POINT('Ctrl Pts',(37.8043764883067,-8.84695258256744,
66.0536422481846));
#131551=CARTESIAN_POINT('Ctrl Pts',(37.8544136268491,-8.70359951764846,
65.9962447764266));
#131552=CARTESIAN_POINT('Ctrl Pts',(37.9608898797757,-8.39855215397505,
65.8741061430377));
#131553=CARTESIAN_POINT('Ctrl Pts',(38.0555414402464,-8.08979107905725,
65.7588476438518));
#131554=CARTESIAN_POINT('Ctrl Pts',(38.1394401871514,-7.7784358182481,65.6508064746933));
#131555=CARTESIAN_POINT('Ctrl Pts',(38.2234081819392,-7.46682357275948,
65.5426761311135));
#131556=CARTESIAN_POINT('Ctrl Pts',(38.2966056056107,-7.15261285739073,
65.4417750367764));
#131557=CARTESIAN_POINT('Ctrl Pts',(38.3603322672021,-6.83683049605349,
65.3482233732188));
#131558=CARTESIAN_POINT('Ctrl Pts',(38.4239729235666,-6.52147431322542,
65.2547979665817));
#131559=CARTESIAN_POINT('Ctrl Pts',(38.4781683640289,-6.20455072395373,
65.1687021668385));
#131560=CARTESIAN_POINT('Ctrl Pts',(38.5243727106882,-5.88694167445974,
65.0898666901936));
#131561=CARTESIAN_POINT('Ctrl Pts',(38.5702075601737,-5.57187255150246,
65.011661662585));
#131562=CARTESIAN_POINT('Ctrl Pts',(38.6081786148033,-5.25612888799339,
64.9406013006287));
#131563=CARTESIAN_POINT('Ctrl Pts',(38.6398248347944,-4.94044272901774,
64.876470820854));
#131564=CARTESIAN_POINT('Ctrl Pts',(38.6710156948983,-4.62929900240211,
64.8132631194727));
#131565=CARTESIAN_POINT('Ctrl Pts',(38.6960624280192,-4.31821113828359,
64.7567873060298));
#131566=CARTESIAN_POINT('Ctrl Pts',(38.7164371727119,-4.00754868885774,
64.7067206894537));
#131567=CARTESIAN_POINT('Ctrl Pts',(38.7363728080012,-3.70358152837316,
64.6577330911655));
#131568=CARTESIAN_POINT('Ctrl Pts',(38.7518356631662,-3.40002164398495,
64.6148814090228));
#131569=CARTESIAN_POINT('Ctrl Pts',(38.7640695060587,-3.09700899262399,
64.5778465685617));
#131570=CARTESIAN_POINT('Ctrl Pts',(38.7759411598554,-2.80296718380441,
64.5419081632522));
#131571=CARTESIAN_POINT('Ctrl Pts',(38.7847721643487,-2.50944068763906,
64.5114472770169));
#131572=CARTESIAN_POINT('Ctrl Pts',(38.7915268784732,-2.21653862227863,
64.4862013713735));
#131573=CARTESIAN_POINT('Ctrl Pts',(38.7980203465799,-1.93496486730855,
64.4619318789721));
#131574=CARTESIAN_POINT('Ctrl Pts',(38.8025950242488,-1.6539681767044,64.4424817775391));
#131575=CARTESIAN_POINT('Ctrl Pts',(38.8059154064001,-1.37337909271983,
64.4276474507953));
#131576=CARTESIAN_POINT('Ctrl Pts',(38.8090729839858,-1.10654781789107,
64.41354047892));
#131577=CARTESIAN_POINT('Ctrl Pts',(38.8110962515457,-0.84008515838022,
64.4036077382365));
#131578=CARTESIAN_POINT('Ctrl Pts',(38.8122885340855,-0.573747525170082,
64.3977531549656));
#131579=CARTESIAN_POINT('Ctrl Pts',(38.8131448252488,-0.382465212306163,
64.3935484234921));
#131580=CARTESIAN_POINT('Ctrl Pts',(38.8135724911743,-0.191247388130586,
64.3914472211002));
#131581=CARTESIAN_POINT('Ctrl Pts',(38.8135869206495,-5.89859875857534E-6,
64.3914449648797));
#131582=CARTESIAN_POINT('',(29.3346501807501,-0.000166304983923139,61.2371511371894));
#131583=CARTESIAN_POINT('Origin',(36.9902838008291,9.11708457778009E-5,
54.05096298925));
#131584=CARTESIAN_POINT('',(26.0609428066925,-10.6024189297442,60.5235111130438));
#131585=CARTESIAN_POINT('Ctrl Pts',(26.0609458870592,-10.6024210452326,
60.5235102920714));
#131586=CARTESIAN_POINT('Ctrl Pts',(26.1340051539456,-10.4995374865864,
60.5325244292292));
#131587=CARTESIAN_POINT('Ctrl Pts',(26.205815570463,-10.3957845448575,60.5417420628761));
#131588=CARTESIAN_POINT('Ctrl Pts',(26.2763660096282,-10.2912186445723,
60.551115732591));
#131589=CARTESIAN_POINT('Ctrl Pts',(26.4066686286617,-10.0980914177259,
60.568428363501));
#131590=CARTESIAN_POINT('Ctrl Pts',(26.5326736501716,-9.90218734680289,
60.586274058075));
#131591=CARTESIAN_POINT('Ctrl Pts',(26.6543717528362,-9.70376604529024,
60.6044649137639));
#131592=CARTESIAN_POINT('Ctrl Pts',(26.6711113225576,-9.67647320227824,
60.6069670653212));
#131593=CARTESIAN_POINT('Ctrl Pts',(26.6877693949852,-9.64913281307989,
60.6094757416172));
#131594=CARTESIAN_POINT('Ctrl Pts',(26.7043459355548,-9.62174563018688,
60.6119904505528));
#131595=CARTESIAN_POINT('Ctrl Pts',(26.8150897230983,-9.43877860211641,
60.6287906020033));
#131596=CARTESIAN_POINT('Ctrl Pts',(26.9221952178138,-9.25371929193362,
60.6458619956123));
#131597=CARTESIAN_POINT('Ctrl Pts',(27.0256916473619,-9.06678321563396,
60.6631785262035));
#131598=CARTESIAN_POINT('Ctrl Pts',(27.0485406571303,-9.0255131519991,60.6670015138985));
#131599=CARTESIAN_POINT('Ctrl Pts',(27.0712137299627,-8.98415179397156,
60.6708363619945));
#131600=CARTESIAN_POINT('Ctrl Pts',(27.0937111268443,-8.94270176648723,
60.6746826491534));
#131601=CARTESIAN_POINT('Ctrl Pts',(27.1883240419292,-8.76838346862868,
60.6908582290334));
#131602=CARTESIAN_POINT('Ctrl Pts',(27.2798309733679,-8.59249358838892,
60.7072384651671));
#131603=CARTESIAN_POINT('Ctrl Pts',(27.3683076969092,-8.4152183524266,60.7238529822909));
#131604=CARTESIAN_POINT('Ctrl Pts',(27.3968229707421,-8.35808409502051,
60.7292076957842));
#131605=CARTESIAN_POINT('Ctrl Pts',(27.4250233906279,-8.3008062658783,60.7345865250659));
#131606=CARTESIAN_POINT('Ctrl Pts',(27.4529112094475,-8.24339203259607,
60.7399898601321));
#131607=CARTESIAN_POINT('Ctrl Pts',(27.465373696585,-8.21773480395399,60.7424044983725));
#131608=CARTESIAN_POINT('Ctrl Pts',(27.4777737553893,-8.19205034178118,
60.744824027499));
#131609=CARTESIAN_POINT('Ctrl Pts',(27.490111727036,-8.16633949305757,60.7472487306104));
#131610=CARTESIAN_POINT('Ctrl Pts',(27.5696717026261,-8.00054607454193,
60.7628841466965));
#131611=CARTESIAN_POINT('Ctrl Pts',(27.6466011738908,-7.83363559644287,
60.7786216795869));
#131612=CARTESIAN_POINT('Ctrl Pts',(27.7209360913992,-7.6656957373092,60.7943841121699));
#131613=CARTESIAN_POINT('Ctrl Pts',(27.7436866560245,-7.61429692304464,
60.7992082816605));
#131614=CARTESIAN_POINT('Ctrl Pts',(27.7661938877754,-7.56280159465106,
60.8040345841593));
#131615=CARTESIAN_POINT('Ctrl Pts',(27.7884580319085,-7.51121201955401,
60.8088603130104));
#131616=CARTESIAN_POINT('Ctrl Pts',(27.8605471700752,-7.34416998169749,
60.8244855547362));
#131617=CARTESIAN_POINT('Ctrl Pts',(27.9300912157483,-7.17614108287275,
60.8401067990999));
#131618=CARTESIAN_POINT('Ctrl Pts',(27.9971233774981,-7.00720542713339,
60.8556482213058));
#131619=CARTESIAN_POINT('Ctrl Pts',(28.03298344009,-6.91683025451935,60.8639623851121));
#131620=CARTESIAN_POINT('Ctrl Pts',(28.0681238540866,-6.82619530707491,
60.8722532523379));
#131621=CARTESIAN_POINT('Ctrl Pts',(28.1025446498989,-6.7353109499957,60.8805064763249));
#131622=CARTESIAN_POINT('Ctrl Pts',(28.1669247756048,-6.56532224998455,
60.8959431792026));
#131623=CARTESIAN_POINT('Ctrl Pts',(28.2287902220065,-6.39446245166542,
60.9112495188088));
#131624=CARTESIAN_POINT('Ctrl Pts',(28.2881562178294,-6.2228067422687,60.9263366729753));
#131625=CARTESIAN_POINT('Ctrl Pts',(28.3233436216813,-6.12106299677433,
60.9352791286567));
#131626=CARTESIAN_POINT('Ctrl Pts',(28.3576520525177,-6.01903922463956,
60.9441441547936));
#131627=CARTESIAN_POINT('Ctrl Pts',(28.3910776390518,-5.91674739756847,
60.9529100851415));
#131628=CARTESIAN_POINT('Ctrl Pts',(28.4312885744125,-5.79369046804852,
60.9634554874858));
#131629=CARTESIAN_POINT('Ctrl Pts',(28.4702222115227,-5.67024587282327,
60.9738575900759));
#131630=CARTESIAN_POINT('Ctrl Pts',(28.5078800904185,-5.54643685186405,
60.9840783438174));
#131631=CARTESIAN_POINT('Ctrl Pts',(28.5568725875443,-5.38536264159635,
60.9973754349703));
#131632=CARTESIAN_POINT('Ctrl Pts',(28.6036936117278,-5.22371262456759,
61.0103612983112));
#131633=CARTESIAN_POINT('Ctrl Pts',(28.6483637057455,-5.06146209877235,
61.0229802871025));
#131634=CARTESIAN_POINT('Ctrl Pts',(28.693312736543,-4.89819841998956,61.0356780735812));
#131635=CARTESIAN_POINT('Ctrl Pts',(28.7360838398638,-4.73432836280087,
61.0480044081514));
#131636=CARTESIAN_POINT('Ctrl Pts',(28.7766913856413,-4.56991859505214,
61.05991043261));
#131637=CARTESIAN_POINT('Ctrl Pts',(28.8089412496872,-4.43934698437749,
61.0693660070055));
#131638=CARTESIAN_POINT('Ctrl Pts',(28.8398258479387,-4.30843400606396,
61.0785562347327));
#131639=CARTESIAN_POINT('Ctrl Pts',(28.8693411221056,-4.17719291721427,
61.0874532897539));
#131640=CARTESIAN_POINT('Ctrl Pts',(28.9064349057422,-4.01225362081862,
61.098634803166));
#131641=CARTESIAN_POINT('Ctrl Pts',(28.941366418073,-3.8467981115552,61.1093531768065));
#131642=CARTESIAN_POINT('Ctrl Pts',(28.9741192877105,-3.68089353564549,
61.1195396968139));
#131643=CARTESIAN_POINT('Ctrl Pts',(29.0007130622788,-3.54618689954222,
61.1278106672574));
#131644=CARTESIAN_POINT('Ctrl Pts',(29.0258700307831,-3.41118314000499,
61.1357309106386));
#131645=CARTESIAN_POINT('Ctrl Pts',(29.0495730671724,-3.27589448461818,
61.1432629515434));
#131646=CARTESIAN_POINT('Ctrl Pts',(29.0767194006975,-3.12095269146694,
61.1518891583789));
#131647=CARTESIAN_POINT('Ctrl Pts',(29.101958714058,-2.96563784557567,61.1600059981815));
#131648=CARTESIAN_POINT('Ctrl Pts',(29.1252546356709,-2.80995284228324,
61.1675423561766));
#131649=CARTESIAN_POINT('Ctrl Pts',(29.1470495934849,-2.66429867433893,
61.1745931441773));
#131650=CARTESIAN_POINT('Ctrl Pts',(29.1671294652963,-2.51837247222515,
61.181126774727));
#131651=CARTESIAN_POINT('Ctrl Pts',(29.1855117296563,-2.37214187313919,
61.187140620576));
#131652=CARTESIAN_POINT('Ctrl Pts',(29.2080620413757,-2.19275452848295,
61.1945180630864));
#131653=CARTESIAN_POINT('Ctrl Pts',(29.228057371095,-2.01291121835345,61.2011129594027));
#131654=CARTESIAN_POINT('Ctrl Pts',(29.2455069431775,-1.83269989880674,
61.2069077148872));
#131655=CARTESIAN_POINT('Ctrl Pts',(29.2568340689288,-1.71571844684613,
61.2106692927505));
#131656=CARTESIAN_POINT('Ctrl Pts',(29.2670884527505,-1.59858067744723,
61.2140938214548));
#131657=CARTESIAN_POINT('Ctrl Pts',(29.2762732055751,-1.48129922084861,
61.2171779988336));
#131658=CARTESIAN_POINT('Ctrl Pts',(29.2919370185711,-1.28128569417749,
61.2224378004451));
#131659=CARTESIAN_POINT('Ctrl Pts',(29.30448893715,-1.08085703169033,61.226706770597));
#131660=CARTESIAN_POINT('Ctrl Pts',(29.3138822904479,-0.88013702625373,
61.2299282192372));
#131661=CARTESIAN_POINT('Ctrl Pts',(29.317922658066,-0.793801232787563,
61.2313138625061));
#131662=CARTESIAN_POINT('Ctrl Pts',(29.3213788304288,-0.707410859236777,
61.2325058918773));
#131663=CARTESIAN_POINT('Ctrl Pts',(29.3242480131973,-0.62097323986363,
61.2335006727539));
#131664=CARTESIAN_POINT('Ctrl Pts',(29.3311096570109,-0.414257877309318,
61.2358796888706));
#131665=CARTESIAN_POINT('Ctrl Pts',(29.3346124522058,-0.207273328511921,
61.2371293245613));
#131666=CARTESIAN_POINT('Ctrl Pts',(29.3346488664094,-0.000153350959778772,
61.2371523603219));
#131667=CARTESIAN_POINT('Ctrl Pts',(26.0609412665091,-10.602417872,60.52351152353));
#131668=CARTESIAN_POINT('Ctrl Pts',(26.6967356456957,-10.1833303319981,
61.8291376819548));
#131669=CARTESIAN_POINT('Ctrl Pts',(27.5872970382304,-9.94480591158098,
63.0575054451691));
#131670=CARTESIAN_POINT('Ctrl Pts',(28.712093773969,-9.9158440831149,64.1368357767385));
#131671=CARTESIAN_POINT('Ctrl Pts',(17.4667653729091,-22.5257212764,77.256905072711));
#131672=CARTESIAN_POINT('Ctrl Pts',(17.4522156153291,-22.52947690984,77.201794509167));
#131673=CARTESIAN_POINT('Ctrl Pts',(17.2326821287691,-22.58361462996,76.351112313277));
#131674=CARTESIAN_POINT('Ctrl Pts',(16.9332603507591,-22.57430986834,74.585159968858));
#131675=CARTESIAN_POINT('Ctrl Pts',(16.9282178457291,-22.22368100432,72.0018522533659));
#131676=CARTESIAN_POINT('Ctrl Pts',(17.3279784679891,-21.55585890438,69.568778249818));
#131677=CARTESIAN_POINT('Ctrl Pts',(18.0359271396891,-20.63613602496,67.425763312453));
#131678=CARTESIAN_POINT('Ctrl Pts',(18.9494515331591,-19.52905542686,65.598121631019));
#131679=CARTESIAN_POINT('Ctrl Pts',(20.0049202231791,-18.26930231769,64.050828430023));
#131680=CARTESIAN_POINT('Ctrl Pts',(21.1756845328891,-16.86079661466,62.74165530726));
#131681=CARTESIAN_POINT('Ctrl Pts',(22.4532806921391,-15.29024780344,61.65009812484));
#131682=CARTESIAN_POINT('Ctrl Pts',(23.8321876788191,-13.5386198194,60.78746444366));
#131683=CARTESIAN_POINT('Ctrl Pts',(24.9093942416691,-12.10874261238,60.35716873393));
#131684=CARTESIAN_POINT('Ctrl Pts',(25.5188775489791,-11.26992181782,60.2071336687));
#131685=CARTESIAN_POINT('Ctrl Pts',(25.6673509880891,-11.06368060085,60.17641247788));
#131686=CARTESIAN_POINT('Ctrl Pts',(18.7773649827691,-17.75527490826,76.717063290409));
#131687=CARTESIAN_POINT('Ctrl Pts',(18.7654556117691,-17.75828882524,76.674914380299));
#131688=CARTESIAN_POINT('Ctrl Pts',(18.5862635620091,-17.80174165801,76.0240512343981));
#131689=CARTESIAN_POINT('Ctrl Pts',(18.3577568645891,-17.79425534819,74.665378823862));
#131690=CARTESIAN_POINT('Ctrl Pts',(18.4246335003491,-17.51291935268,72.6770817004958));
#131691=CARTESIAN_POINT('Ctrl Pts',(18.8714641952291,-16.98119012651,70.822183427483));
#131692=CARTESIAN_POINT('Ctrl Pts',(19.6142963879091,-16.25801796827,69.218239633607));
#131693=CARTESIAN_POINT('Ctrl Pts',(20.5621683937491,-15.40160733776,67.8849620187121));
#131694=CARTESIAN_POINT('Ctrl Pts',(21.6579870981791,-14.44562122449,66.791899033372));
#131695=CARTESIAN_POINT('Ctrl Pts',(22.8780955574091,-13.40004445027,65.903735017982));
#131696=CARTESIAN_POINT('Ctrl Pts',(24.2153171433191,-12.26374841242,65.203217298719));
#131697=CARTESIAN_POINT('Ctrl Pts',(25.6646851711591,-11.03571934281,64.698047871997));
#131698=CARTESIAN_POINT('Ctrl Pts',(26.8015432713391,-10.07428690511,64.495800893793));
#131699=CARTESIAN_POINT('Ctrl Pts',(27.4463952672191,-9.53132694979998,
64.453831767256));
#131700=CARTESIAN_POINT('Ctrl Pts',(27.6035705906891,-9.399240458337,64.448068196782));
#131701=CARTESIAN_POINT('Ctrl Pts',(22.6527444970191,-14.84009533989,75.599270274124));
#131702=CARTESIAN_POINT('Ctrl Pts',(22.6450480694791,-14.8417831418,75.575183427031));
#131703=CARTESIAN_POINT('Ctrl Pts',(22.5298127564291,-14.866114563,75.203116801731));
#131704=CARTESIAN_POINT('Ctrl Pts',(22.4006621202491,-14.86192846848,74.422696506464));
#131705=CARTESIAN_POINT('Ctrl Pts',(22.5181198569391,-14.70436463479,73.2633823361753));
#131706=CARTESIAN_POINT('Ctrl Pts',(22.9377195244991,-14.4052238805,72.1556566073007));
#131707=CARTESIAN_POINT('Ctrl Pts',(23.6141508774891,-13.99538058674,71.163675788398));
#131708=CARTESIAN_POINT('Ctrl Pts',(24.4918032145691,-13.50533859052,70.299994638951));
#131709=CARTESIAN_POINT('Ctrl Pts',(25.5329266094991,-12.95204779512,69.5496905418731));
#131710=CARTESIAN_POINT('Ctrl Pts',(26.7219181594991,-12.33886835717,68.8939981611091));
#131711=CARTESIAN_POINT('Ctrl Pts',(28.0550484564891,-11.66205659809,68.32348737336));
#131712=CARTESIAN_POINT('Ctrl Pts',(29.5302626991891,-10.91639130965,67.842821810496));
#131713=CARTESIAN_POINT('Ctrl Pts',(30.7112123601191,-10.3172835446,67.571237827604));
#131714=CARTESIAN_POINT('Ctrl Pts',(31.3905930089891,-9.97074480891598,
67.457066442736));
#131715=CARTESIAN_POINT('Ctrl Pts',(31.5567731140791,-9.88587105497599,
67.431705971039));
#131716=CARTESIAN_POINT('Ctrl Pts',(27.4727097388691,-14.99894242272,74.370845864195));
#131717=CARTESIAN_POINT('Ctrl Pts',(27.4690374908891,-14.99927412475,74.362370216541));
#131718=CARTESIAN_POINT('Ctrl Pts',(27.4146355861491,-15.00404176909,74.231520094978));
#131719=CARTESIAN_POINT('Ctrl Pts',(27.3717438376491,-15.00325792021,73.9585721062895));
#131720=CARTESIAN_POINT('Ctrl Pts',(27.4972980083791,-14.97219965841,73.5156372957745));
#131721=CARTESIAN_POINT('Ctrl Pts',(27.8267501244891,-14.90490385564,73.0117077491551));
#131722=CARTESIAN_POINT('Ctrl Pts',(28.3632567205591,-14.79417301808,72.4487361234403));
#131723=CARTESIAN_POINT('Ctrl Pts',(29.0954791031191,-14.63302923949,71.833557915698));
#131724=CARTESIAN_POINT('Ctrl Pts',(30.0097285339691,-14.41300577028,71.171242909551));
#131725=CARTESIAN_POINT('Ctrl Pts',(31.1001512767791,-14.12091813026,70.4622944187711));
#131726=CARTESIAN_POINT('Ctrl Pts',(32.3671840294791,-13.73672387177,69.7064055545461));
#131727=CARTESIAN_POINT('Ctrl Pts',(33.8128240385791,-13.23052362994,68.90703904439));
#131728=CARTESIAN_POINT('Ctrl Pts',(35.0038717625891,-12.73614203142,68.297720297344));
#131729=CARTESIAN_POINT('Ctrl Pts',(35.7025055078291,-12.40446635354,67.961264321001));
#131730=CARTESIAN_POINT('Ctrl Pts',(35.8742286296091,-12.32012494619,67.879945375125));
#131731=CARTESIAN_POINT('Ctrl Pts',(29.4810590753118,-10.3417444512209,
65.2638123960938));
#131732=CARTESIAN_POINT('Ctrl Pts',(29.6345266860941,-10.3548479162145,
65.3858288214936));
#131733=CARTESIAN_POINT('Ctrl Pts',(29.7903387355854,-10.3717675925251,
65.5046171518437));
#131734=CARTESIAN_POINT('Ctrl Pts',(29.948127817785,-10.3924631647627,65.6198958223942));
#131735=CARTESIAN_POINT('Ctrl Pts',(30.1076455746656,-10.4133854694917,
65.736437440395));
#131736=CARTESIAN_POINT('Ctrl Pts',(30.26918353621,-10.438166853462,65.8493917336466));
#131737=CARTESIAN_POINT('Ctrl Pts',(30.4323438463269,-10.4667289049876,
65.9585030743414));
#131738=CARTESIAN_POINT('Ctrl Pts',(30.5955041564438,-10.4952909565132,
66.0676144150361));
#131739=CARTESIAN_POINT('Ctrl Pts',(30.7602863706003,-10.5276335464042,
66.1728825820115));
#131740=CARTESIAN_POINT('Ctrl Pts',(30.9262808011331,-10.5636428134725,
66.2740912134265));
#131741=CARTESIAN_POINT('Ctrl Pts',(31.0913257917805,-10.5994461180016,
66.3747209608927));
#131742=CARTESIAN_POINT('Ctrl Pts',(31.2575687584314,-10.6388740362011,
66.4713373530446));
#131743=CARTESIAN_POINT('Ctrl Pts',(31.4246015632957,-10.6817828365551,
66.5637694060554));
#131744=CARTESIAN_POINT('Ctrl Pts',(31.5924715009742,-10.7249066866702,
66.6566647088135));
#131745=CARTESIAN_POINT('Ctrl Pts',(31.7611387787817,-10.7715461974904,
66.7453335089057));
#131746=CARTESIAN_POINT('Ctrl Pts',(31.9301906162814,-10.8215255613416,
66.8296458007108));
#131747=CARTESIAN_POINT('Ctrl Pts',(32.0986259760348,-10.8713226665079,
66.9136506326717));
#131748=CARTESIAN_POINT('Ctrl Pts',(32.267442692503,-10.9244350361494,66.9933306894848));
#131749=CARTESIAN_POINT('Ctrl Pts',(32.4362402859212,-10.980662794166,67.0686011625235));
#131750=CARTESIAN_POINT('Ctrl Pts',(32.6071295117973,-11.0375872908111,
67.144804339408));
#131751=CARTESIAN_POINT('Ctrl Pts',(32.7779990938665,-11.0977046862795,
67.216488060209));
#131752=CARTESIAN_POINT('Ctrl Pts',(32.9484476739858,-11.1607845021936,
67.2836092914197));
#131753=CARTESIAN_POINT('Ctrl Pts',(33.1198528403072,-11.2242183326819,
67.3511072183095));
#131754=CARTESIAN_POINT('Ctrl Pts',(33.2908318931408,-11.2906476239985,
67.4139913896642));
#131755=CARTESIAN_POINT('Ctrl Pts',(33.4609969732177,-11.3598192426461,
67.472263038667));
#131756=CARTESIAN_POINT('Ctrl Pts',(33.6329763863426,-11.4297283824915,
67.5311559912798));
#131757=CARTESIAN_POINT('Ctrl Pts',(33.8041240204778,-11.5024383239172,
67.5853376584749));
#131758=CARTESIAN_POINT('Ctrl Pts',(33.9740657157468,-11.5776733361085,
67.6348536143392));
#131759=CARTESIAN_POINT('Ctrl Pts',(34.1450660047094,-11.6533769990881,
67.6846780129228));
#131760=CARTESIAN_POINT('Ctrl Pts',(34.3148449983275,-11.731636951271,67.7297786077743));
#131761=CARTESIAN_POINT('Ctrl Pts',(34.4830527710675,-11.8121627363735,
67.7702438497114));
#131762=CARTESIAN_POINT('Ctrl Pts',(34.653232272717,-11.8936324434831,67.8111834245884));
#131763=CARTESIAN_POINT('Ctrl Pts',(34.8218032405913,-11.9774210769124,
67.8473785768995));
#131764=CARTESIAN_POINT('Ctrl Pts',(34.9884394131694,-12.0632232380785,
67.8789603878941));
#131765=CARTESIAN_POINT('Ctrl Pts',(35.1256376224812,-12.13386758069,67.9049629529329));
#131766=CARTESIAN_POINT('Ctrl Pts',(35.2615248946371,-12.2058767063507,
67.9278390016601));
#131767=CARTESIAN_POINT('Ctrl Pts',(35.3959387673533,-12.2790802564028,
67.9476794933271));
#131768=CARTESIAN_POINT('Ctrl Pts',(25.3886736533591,-11.44208510792,60.2115109699));
#131769=CARTESIAN_POINT('Ctrl Pts',(25.5981770475491,-11.17175375805,60.22632667139));
#131770=CARTESIAN_POINT('Ctrl Pts',(25.8078177068491,-10.88204468039,60.24561988886));
#131771=CARTESIAN_POINT('Ctrl Pts',(26.0168787184791,-10.57129328633,60.270855635));
#131772=CARTESIAN_POINT('Ctrl Pts',(27.3087836696091,-9.624602273718,64.44463626086));
#131773=CARTESIAN_POINT('Ctrl Pts',(27.5425179224791,-9.479512324536,64.50183542974));
#131774=CARTESIAN_POINT('Ctrl Pts',(27.7759878147791,-9.32787789472698,
64.56281239081));
#131775=CARTESIAN_POINT('Ctrl Pts',(28.0092438744591,-9.16583693103399,
64.625382279757));
#131776=CARTESIAN_POINT('Ctrl Pts',(31.2407814247091,-10.04443147536,67.489770329979));
#131777=CARTESIAN_POINT('Ctrl Pts',(31.5318184331991,-9.93037722233698,
67.468249475135));
#131778=CARTESIAN_POINT('Ctrl Pts',(31.8153253258691,-9.81435677539199,
67.4542319002));
#131779=CARTESIAN_POINT('Ctrl Pts',(32.0927104552091,-9.69360679656099,
67.4456953393931));
#131780=CARTESIAN_POINT('Ctrl Pts',(35.5328635075091,-12.52520554518,68.067674694392));
#131781=CARTESIAN_POINT('Ctrl Pts',(35.8902027012991,-12.3349434155,67.879400029176));
#131782=CARTESIAN_POINT('Ctrl Pts',(36.2289341849091,-12.1371151135,67.705214293035));
#131783=CARTESIAN_POINT('Ctrl Pts',(36.5518441070791,-11.93289063421,67.547001987805));
#131784=CARTESIAN_POINT('Ctrl Pts',(36.2511910984291,-0.816951121684487,
99.13095237507));
#131785=CARTESIAN_POINT('Ctrl Pts',(36.2200982088991,-1.45683196280799,
99.1098451401801));
#131786=CARTESIAN_POINT('Ctrl Pts',(36.0778630790891,-2.85039942836099,
99.0419676728901));
#131787=CARTESIAN_POINT('Ctrl Pts',(35.6275483510391,-4.94247000735899,
98.84599903898));
#131788=CARTESIAN_POINT('Ctrl Pts',(34.9397597871691,-7.05113172994599,
98.51977184372));
#131789=CARTESIAN_POINT('Ctrl Pts',(34.0734741662491,-9.09163743804897,
98.0649602571899));
#131790=CARTESIAN_POINT('Ctrl Pts',(33.0099168483791,-11.12983443612,97.44906592845));
#131791=CARTESIAN_POINT('Ctrl Pts',(31.7699785170891,-13.12298748389,96.6589115129399));
#131792=CARTESIAN_POINT('Ctrl Pts',(30.4746258290591,-14.92251334854,95.75721789378));
#131793=CARTESIAN_POINT('Ctrl Pts',(29.1968815731991,-16.50069944243,94.7947864407199));
#131794=CARTESIAN_POINT('Ctrl Pts',(27.9225293421991,-17.92619343051,93.76208048801));
#131795=CARTESIAN_POINT('Ctrl Pts',(26.5896727465691,-19.28349187111,92.5956876894801));
#131796=CARTESIAN_POINT('Ctrl Pts',(25.1814694175691,-20.58838494568,91.25117303266));
#131797=CARTESIAN_POINT('Ctrl Pts',(23.7249591534991,-21.81419974781,89.71266771848));
#131798=CARTESIAN_POINT('Ctrl Pts',(22.2142909846591,-22.9637208008,87.91364117654));
#131799=CARTESIAN_POINT('Ctrl Pts',(20.6065395382091,-24.05476593901,85.68623624305));
#131800=CARTESIAN_POINT('Ctrl Pts',(18.9416778012191,-25.02348229969,82.825890425796));
#131801=CARTESIAN_POINT('Ctrl Pts',(17.5339994345191,-25.65356630387,79.417420667109));
#131802=CARTESIAN_POINT('Ctrl Pts',(16.9242179391691,-25.78353110717,76.926255793732));
#131803=CARTESIAN_POINT('Ctrl Pts',(16.7312453442491,-25.77964745785,75.805602355198));
#131804=CARTESIAN_POINT('Ctrl Pts',(34.9680768531591,-0.377262712455286,
92.83793248162));
#131805=CARTESIAN_POINT('Ctrl Pts',(34.9401900659091,-0.768818210978587,
92.83356221903));
#131806=CARTESIAN_POINT('Ctrl Pts',(34.8109275223991,-1.62812620872499,
92.8325719567701));
#131807=CARTESIAN_POINT('Ctrl Pts',(34.3972755661991,-2.97122279462399,
92.8255990532501));
#131808=CARTESIAN_POINT('Ctrl Pts',(33.7599966114291,-4.39375486831299,
92.76261787049));
#131809=CARTESIAN_POINT('Ctrl Pts',(32.9521573659891,-5.82931930270299,
92.61621541888));
#131810=CARTESIAN_POINT('Ctrl Pts',(31.9551618598791,-7.31697565127499,
92.35621163472));
#131811=CARTESIAN_POINT('Ctrl Pts',(30.7878189799691,-8.81951599642399,
91.9596113594201));
#131812=CARTESIAN_POINT('Ctrl Pts',(29.5643467643691,-10.21287137887,91.45281600972));
#131813=CARTESIAN_POINT('Ctrl Pts',(28.3547145027491,-11.46125770319,90.86912642514));
#131814=CARTESIAN_POINT('Ctrl Pts',(27.1462246720591,-12.60932492795,90.2068010813201));
#131815=CARTESIAN_POINT('Ctrl Pts',(25.8804633212691,-13.72121825748,89.42218714027));
#131816=CARTESIAN_POINT('Ctrl Pts',(24.5415426038291,-14.80846467629,88.4770655865801));
#131817=CARTESIAN_POINT('Ctrl Pts',(23.1553900553591,-15.84725088264,87.34998754959));
#131818=CARTESIAN_POINT('Ctrl Pts',(21.7169286490991,-16.83785256507,85.9795861337301));
#131819=CARTESIAN_POINT('Ctrl Pts',(20.1864646779891,-17.79411649535,84.2176273015201));
#131820=CARTESIAN_POINT('Ctrl Pts',(18.6056376920291,-18.65837811088,81.868380902977));
#131821=CARTESIAN_POINT('Ctrl Pts',(17.2833457609491,-19.22934869733,78.9739891356611));
#131822=CARTESIAN_POINT('Ctrl Pts',(16.7318898964791,-19.34793907064,76.820460370021));
#131823=CARTESIAN_POINT('Ctrl Pts',(16.5654152065891,-19.34439445674,75.849914932886));
#131824=CARTESIAN_POINT('Ctrl Pts',(38.6686947048191,-0.267618408180286,
87.57152762521));
#131825=CARTESIAN_POINT('Ctrl Pts',(38.6331457099391,-0.640502714598286,
87.56228047755));
#131826=CARTESIAN_POINT('Ctrl Pts',(38.4681697649291,-1.45257130791499,
87.5371031361401));
#131827=CARTESIAN_POINT('Ctrl Pts',(37.9543196144491,-2.67152049410099,
87.46697907679));
#131828=CARTESIAN_POINT('Ctrl Pts',(37.1964789572891,-3.89993484531899,
87.33954011223));
#131829=CARTESIAN_POINT('Ctrl Pts',(36.2722354399091,-5.08847143352099,
87.1482156939501));
#131830=CARTESIAN_POINT('Ctrl Pts',(35.1711071623791,-6.27550574943099,
86.8740206795701));
#131831=CARTESIAN_POINT('Ctrl Pts',(33.9234036585391,-7.436166673543,86.50611895787));
#131832=CARTESIAN_POINT('Ctrl Pts',(32.6526782149891,-8.48396598041999,
86.07171874038));
#131833=CARTESIAN_POINT('Ctrl Pts',(31.4266015655591,-9.40280963542199,
85.5959755830301));
#131834=CARTESIAN_POINT('Ctrl Pts',(30.2282183070691,-10.23269364386,85.07485106796));
#131835=CARTESIAN_POINT('Ctrl Pts',(29.0009821455491,-11.02282107056,84.4750277186701));
#131836=CARTESIAN_POINT('Ctrl Pts',(27.7349646372491,-11.7823880216,83.77066674245));
#131837=CARTESIAN_POINT('Ctrl Pts',(26.4611997445191,-12.49587308951,82.949856613029));
#131838=CARTESIAN_POINT('Ctrl Pts',(25.1820693516891,-13.16490311603,81.9728674396441));
#131839=CARTESIAN_POINT('Ctrl Pts',(23.8728795301391,-13.79985263807,80.741966022882));
#131840=CARTESIAN_POINT('Ctrl Pts',(22.5850112147791,-14.36356654138,79.133191069062));
#131841=CARTESIAN_POINT('Ctrl Pts',(21.5697113092491,-14.73019815096,77.183930116823));
#131842=CARTESIAN_POINT('Ctrl Pts',(21.1758003549191,-14.80581932552,75.7409655371681));
#131843=CARTESIAN_POINT('Ctrl Pts',(21.0646250899491,-14.8035595922,75.088550558094));
#131844=CARTESIAN_POINT('Ctrl Pts',(45.0312706731691,-0.556809233210386,
86.63588923546));
#131845=CARTESIAN_POINT('Ctrl Pts',(44.9819984429591,-1.15239083593299,
86.6032111113799));
#131846=CARTESIAN_POINT('Ctrl Pts',(44.7550297579291,-2.43387817146999,
86.47794742155));
#131847=CARTESIAN_POINT('Ctrl Pts',(44.0669849657891,-4.23139684260399,
86.1321464635101));
#131848=CARTESIAN_POINT('Ctrl Pts',(43.0931519133991,-5.87949518942999,
85.65298684557));
#131849=CARTESIAN_POINT('Ctrl Pts',(41.9506857162891,-7.33390305288999,
85.0915934778799));
#131850=CARTESIAN_POINT('Ctrl Pts',(40.6400631633491,-8.65884473130499,
84.44202906066));
#131851=CARTESIAN_POINT('Ctrl Pts',(39.2094613534091,-9.84085525044999,
83.71996478425));
#131852=CARTESIAN_POINT('Ctrl Pts',(37.8019957376891,-10.82051536224,82.99003573172));
#131853=CARTESIAN_POINT('Ctrl Pts',(36.4852355554891,-11.6168290835,82.283717786993));
#131854=CARTESIAN_POINT('Ctrl Pts',(35.2348621603691,-12.28740211764,81.586024678646));
#131855=CARTESIAN_POINT('Ctrl Pts',(33.9934103628291,-12.88127932846,80.858065721516));
#131856=CARTESIAN_POINT('Ctrl Pts',(32.7581770629291,-13.40872065919,80.08477919832));
#131857=CARTESIAN_POINT('Ctrl Pts',(31.5683175582891,-13.86272653758,79.272924596943));
#131858=CARTESIAN_POINT('Ctrl Pts',(30.4356778789491,-14.24928723071,78.407307267481));
#131859=CARTESIAN_POINT('Ctrl Pts',(29.3529211006491,-14.57798235441,77.439888248051));
#131860=CARTESIAN_POINT('Ctrl Pts',(28.3831326036191,-14.83361972799,76.336383711929));
#131861=CARTESIAN_POINT('Ctrl Pts',(27.7038229907891,-14.97888942575,75.170329705841));
#131862=CARTESIAN_POINT('Ctrl Pts',(27.4678322792991,-15.00690558171,74.365048202755));
#131863=CARTESIAN_POINT('Ctrl Pts',(27.4060630052191,-15.00607043787,73.999190543978));
#131864=CARTESIAN_POINT('Origin',(26.4624892479491,-5.,78.749546355382));
#131865=CARTESIAN_POINT('',(-5.14030444921783,-5.,85.3373981618386));
#131866=CARTESIAN_POINT('Ctrl Pts',(-5.03958561217558,-6.,84.3042121015221));
#131867=CARTESIAN_POINT('Ctrl Pts',(-5.01779961145864,-5.9999999999996,
84.4277666513109));
#131868=CARTESIAN_POINT('Ctrl Pts',(-5.00224861254975,-5.97492290499363,
84.560469325189));
#131869=CARTESIAN_POINT('Ctrl Pts',(-4.98975476340367,-5.87416764040792,
84.8064865857881));
#131870=CARTESIAN_POINT('Ctrl Pts',(-4.99272071568298,-5.798526343987,84.9198116323849));
#131871=CARTESIAN_POINT('Ctrl Pts',(-5.01199432837025,-5.62256919818321,
85.1045000068224));
#131872=CARTESIAN_POINT('Ctrl Pts',(-5.03011167864627,-5.50920575318542,
85.1870555783692));
#131873=CARTESIAN_POINT('Ctrl Pts',(-5.07864362193569,-5.26113860665341,
85.3007472862074));
#131874=CARTESIAN_POINT('Ctrl Pts',(-5.1089932976158,-5.12641933949878,
85.3318771610163));
#131875=CARTESIAN_POINT('Ctrl Pts',(-5.14030444921746,-5.,85.3373981618407));
#131876=CARTESIAN_POINT('',(-6.54682286628224,-5.,85.5854053076332));
#131877=CARTESIAN_POINT('Origin',(-6.72047103979891,-5.,84.60059755389));
#131878=CARTESIAN_POINT('',(-0.138906894980912,-5.,84.45551683178));
#131879=CARTESIAN_POINT('Origin',(-7.10051551200191,5.,84.66760964821));
#131880=CARTESIAN_POINT('',(-5.14030444921695,5.,85.3373981618436));
#131881=CARTESIAN_POINT('Ctrl Pts',(-5.14030444921696,5.,85.3373981618436));
#131882=CARTESIAN_POINT('Ctrl Pts',(-5.10929140005093,5.12521574553663,
85.3319297245216));
#131883=CARTESIAN_POINT('Ctrl Pts',(-5.07918376137443,5.2587323981861,85.301326613419));
#131884=CARTESIAN_POINT('Ctrl Pts',(-5.03087653636086,5.50495104913208,
85.1895150329288));
#131885=CARTESIAN_POINT('Ctrl Pts',(-5.01273977349526,5.61766789433613,
85.1083121247498));
#131886=CARTESIAN_POINT('Ctrl Pts',(-4.99292749239007,5.7948754580924,84.924877408976));
#131887=CARTESIAN_POINT('Ctrl Pts',(-4.98968965602442,5.87184753647394,
84.8108658563746));
#131888=CARTESIAN_POINT('Ctrl Pts',(-5.00197073577722,5.97442824468255,
84.5629279946691));
#131889=CARTESIAN_POINT('Ctrl Pts',(-5.01758370837151,6.,84.4289910985632));
#131890=CARTESIAN_POINT('Ctrl Pts',(-5.03958561217562,6.,84.3042121015219));
#131891=CARTESIAN_POINT('',(-6.54682286760695,5.,85.5854053078674));
#131892=CARTESIAN_POINT('',(-6.54682287186491,5.,85.58540530862));
#131893=CARTESIAN_POINT('Origin',(-6.72047103979891,5.,84.60059755389));
#131894=CARTESIAN_POINT('Ctrl Pts',(25.6728519466291,11.05620868577,60.1753393120401));
#131895=CARTESIAN_POINT('Ctrl Pts',(25.5908811595391,11.17010610055,60.1922130334301));
#131896=CARTESIAN_POINT('Ctrl Pts',(25.0176949940091,11.96220506401,60.3226366877));
#131897=CARTESIAN_POINT('Ctrl Pts',(23.9454509711491,13.3937300709,60.72216890038));
#131898=CARTESIAN_POINT('Ctrl Pts',(22.4585522519091,15.28518638036,61.63777386195));
#131899=CARTESIAN_POINT('Ctrl Pts',(21.0802507927691,16.97737598619,62.82703989993));
#131900=CARTESIAN_POINT('Ctrl Pts',(19.8267910571591,18.48224713566,64.271659173669));
#131901=CARTESIAN_POINT('Ctrl Pts',(18.7098146781291,19.81562337201,66.003616761918));
#131902=CARTESIAN_POINT('Ctrl Pts',(17.7716110472991,20.96488749236,68.078902873165));
#131903=CARTESIAN_POINT('Ctrl Pts',(17.1084342304291,21.8744622819,70.533431788808));
#131904=CARTESIAN_POINT('Ctrl Pts',(16.8638554479991,22.45052823568,73.2803532769174));
#131905=CARTESIAN_POINT('Ctrl Pts',(17.0786448222291,22.59937448267,75.596712572949));
#131906=CARTESIAN_POINT('Ctrl Pts',(17.3662061271091,22.55171003512,76.874515663416));
#131907=CARTESIAN_POINT('Ctrl Pts',(17.4669987734891,22.52571394401,77.2562285499651));
#131908=CARTESIAN_POINT('Ctrl Pts',(27.6093946371291,9.39445532140801,64.447920892227));
#131909=CARTESIAN_POINT('Ctrl Pts',(27.5226174428891,9.46737944809301,64.451034788112));
#131910=CARTESIAN_POINT('Ctrl Pts',(26.9160359092391,9.97752475953103,64.482341733254));
#131911=CARTESIAN_POINT('Ctrl Pts',(25.7838601800091,10.93479181558,64.661006837171));
#131912=CARTESIAN_POINT('Ctrl Pts',(24.2207011124691,12.25908842062,65.194134063823));
#131913=CARTESIAN_POINT('Ctrl Pts',(22.7783053134691,13.48485509378,65.959148542412));
#131914=CARTESIAN_POINT('Ctrl Pts',(21.4726982157391,14.6052048364,66.94431046259));
#131915=CARTESIAN_POINT('Ctrl Pts',(20.3137223160191,15.62131353079,68.176238741846));
#131916=CARTESIAN_POINT('Ctrl Pts',(19.3392518035291,16.51491733119,69.702089136366));
#131917=CARTESIAN_POINT('Ctrl Pts',(18.6353752499191,17.23396255898,71.553480602797));
#131918=CARTESIAN_POINT('Ctrl Pts',(18.3290383767791,17.69470562174,73.6596809561242));
#131919=CARTESIAN_POINT('Ctrl Pts',(18.4647369076291,17.81439079021,75.444726555105));
#131920=CARTESIAN_POINT('Ctrl Pts',(18.6950959018691,17.77610222599,76.424554931989));
#131921=CARTESIAN_POINT('Ctrl Pts',(18.7775986176291,17.7552396856,76.716506355083));
#131922=CARTESIAN_POINT('Ctrl Pts',(31.5629272267991,9.88281068194302,67.430842306303));
#131923=CARTESIAN_POINT('Ctrl Pts',(31.4711681472091,9.92967730101103,67.444807195928));
#131924=CARTESIAN_POINT('Ctrl Pts',(30.8310903628191,10.25631090589,67.5476759313801));
#131925=CARTESIAN_POINT('Ctrl Pts',(29.6521222456891,10.85487243909,67.805767900236));
#131926=CARTESIAN_POINT('Ctrl Pts',(28.0597002587091,11.65964394348,68.317830215232));
#131927=CARTESIAN_POINT('Ctrl Pts',(26.6228516811691,12.38921116325,68.938303098405));
#131928=CARTESIAN_POINT('Ctrl Pts',(25.3542093351291,13.0450930181,69.658831925755));
#131929=CARTESIAN_POINT('Ctrl Pts',(24.2590278301191,13.63170757615,70.4940295766521));
#131930=CARTESIAN_POINT('Ctrl Pts',(23.3629396071591,14.14148255666,71.468571308628));
#131931=CARTESIAN_POINT('Ctrl Pts',(22.7218359561591,14.5476997234,72.5973874861561));
#131932=CARTESIAN_POINT('Ctrl Pts',(22.4115473378591,14.8062209636,73.8396950223705));
#131933=CARTESIAN_POINT('Ctrl Pts',(22.4566140195691,14.87316749049,74.870971069554));
#131934=CARTESIAN_POINT('Ctrl Pts',(22.5996423578891,14.85173828971,75.432105059216));
#131935=CARTESIAN_POINT('Ctrl Pts',(22.6529499976691,14.84005551372,75.5989411619891));
#131936=CARTESIAN_POINT('Ctrl Pts',(35.8805628265291,12.31710390136,67.87700830848));
#131937=CARTESIAN_POINT('Ctrl Pts',(35.7857292024291,12.36372287642,67.921898444141));
#131938=CARTESIAN_POINT('Ctrl Pts',(35.1260583462191,12.68200901524,68.23708902494));
#131939=CARTESIAN_POINT('Ctrl Pts',(33.9330000499891,13.18738451274,68.8416951696051));
#131940=CARTESIAN_POINT('Ctrl Pts',(32.3705467692491,13.73746778379,69.702912182422));
#131941=CARTESIAN_POINT('Ctrl Pts',(31.0065678005891,14.14850934188,70.5189831644171));
#131942=CARTESIAN_POINT('Ctrl Pts',(29.8485481528991,14.4541608558,71.28034056044));
#131943=CARTESIAN_POINT('Ctrl Pts',(28.8962838945291,14.67861693811,71.987970801025));
#131944=CARTESIAN_POINT('Ctrl Pts',(28.1604571839791,14.83686516773,72.6398212113681));
#131945=CARTESIAN_POINT('Ctrl Pts',(27.6593550752991,14.93874245386,73.2287174375679));
#131946=CARTESIAN_POINT('Ctrl Pts',(27.4045731969891,14.99268753181,73.7451354687612));
#131947=CARTESIAN_POINT('Ctrl Pts',(27.3853582494091,15.0053667451,74.11532093663));
#131948=CARTESIAN_POINT('Ctrl Pts',(27.4474386542391,15.00123185086,74.312087977728));
#131949=CARTESIAN_POINT('Ctrl Pts',(27.4728519056491,14.99893719101,74.370762926049));
#131950=CARTESIAN_POINT('Origin',(33.8227660273614,17.5861371975626,59.0248880432778));
#131951=CARTESIAN_POINT('Ctrl Pts',(26.0076877261891,10.58495646334,60.26985796972));
#131952=CARTESIAN_POINT('Ctrl Pts',(25.7990037333791,10.89447975427,60.24482455385));
#131953=CARTESIAN_POINT('Ctrl Pts',(25.5896565743691,11.1831771459,60.22557462704));
#131954=CARTESIAN_POINT('Ctrl Pts',(25.3807021623791,11.45236674632,60.21090371374));
#131955=CARTESIAN_POINT('Ctrl Pts',(27.9987970739791,9.17295597816802,64.622590824873));
#131956=CARTESIAN_POINT('Ctrl Pts',(27.7660735618591,9.33426324017502,64.560255312909));
#131957=CARTESIAN_POINT('Ctrl Pts',(27.5333174178191,9.48524635017302,64.499674997551));
#131958=CARTESIAN_POINT('Ctrl Pts',(27.3000253208991,9.63004663000602,64.442635376589));
#131959=CARTESIAN_POINT('Ctrl Pts',(32.0801713998191,9.69904765178202,67.445984142724));
#131960=CARTESIAN_POINT('Ctrl Pts',(31.8033473372391,9.81925633458402,67.454791081483));
#131961=CARTESIAN_POINT('Ctrl Pts',(31.5208971300691,9.93468827936802,67.469340771313));
#131962=CARTESIAN_POINT('Ctrl Pts',(31.2300886277791,10.04875492352,67.490838049821));
#131963=CARTESIAN_POINT('Ctrl Pts',(36.5371673514891,11.94221289613,67.553890268911));
#131964=CARTESIAN_POINT('Ctrl Pts',(36.2147089752091,12.14570654659,67.712396250694));
#131965=CARTESIAN_POINT('Ctrl Pts',(35.8771568089191,12.34268599228,67.886973156649));
#131966=CARTESIAN_POINT('Ctrl Pts',(35.5198166400391,12.53258632276,68.07491847425));
#131967=CARTESIAN_POINT('Ctrl Pts',(29.6607179856746,9.94038469281037,64.9669467760166));
#131968=CARTESIAN_POINT('Ctrl Pts',(30.1590068583674,9.97665887137027,65.3620001554969));
#131969=CARTESIAN_POINT('Ctrl Pts',(30.6858019445019,10.0485591111603,65.7214144613769));
#131970=CARTESIAN_POINT('Ctrl Pts',(31.7706505757518,10.2607534512662,66.3509683676041));
#131971=CARTESIAN_POINT('Ctrl Pts',(32.3285497113111,10.4009981803986,66.6210514629286));
#131972=CARTESIAN_POINT('Ctrl Pts',(33.4471502167783,10.7395896426921,67.0635873838908));
#131973=CARTESIAN_POINT('Ctrl Pts',(34.0077151370051,10.9378504308792,67.2360632541964));
#131974=CARTESIAN_POINT('Ctrl Pts',(35.1057006193385,11.3778331546057,67.4848315470064));
#131975=CARTESIAN_POINT('Ctrl Pts',(35.6430402158663,11.6194638105209,67.5612071130097));
#131976=CARTESIAN_POINT('Ctrl Pts',(36.1590910689312,11.8739168214411,67.5956414534657));
#131977=CARTESIAN_POINT('Ctrl Pts',(29.1301066186391,-0.189325198801386,
61.01350638832));
#131978=CARTESIAN_POINT('Ctrl Pts',(29.1301171086491,-0.188219559987986,
61.01351029305));
#131979=CARTESIAN_POINT('Ctrl Pts',(29.1327100608491,0.0875421358441442,
61.0144753342501));
#131980=CARTESIAN_POINT('Ctrl Pts',(29.1259762223391,0.661869688765914,
61.01189519272));
#131981=CARTESIAN_POINT('Ctrl Pts',(29.0771717435891,1.54597290477701,60.99362463442));
#131982=CARTESIAN_POINT('Ctrl Pts',(28.9836009802591,2.46822553813401,60.95933878612));
#131983=CARTESIAN_POINT('Ctrl Pts',(28.8434009410291,3.40217169142201,60.90943180935));
#131984=CARTESIAN_POINT('Ctrl Pts',(28.6591089571391,4.32587075588902,60.84674448141));
#131985=CARTESIAN_POINT('Ctrl Pts',(28.4369612179591,5.21837798582801,60.77569210592));
#131986=CARTESIAN_POINT('Ctrl Pts',(28.1848437175191,6.06426036422701,60.7009064822));
#131987=CARTESIAN_POINT('Ctrl Pts',(27.9087860776491,6.86007287828601,60.6258067072));
#131988=CARTESIAN_POINT('Ctrl Pts',(27.6123385282491,7.60966710787701,60.55276423571));
#131989=CARTESIAN_POINT('Ctrl Pts',(27.2953631596791,8.32198182378201,60.48284598351));
#131990=CARTESIAN_POINT('Ctrl Pts',(26.9557511764191,9.005721841742,60.4165783700401));
#131991=CARTESIAN_POINT('Ctrl Pts',(26.5893525670591,9.66929542127001,60.35387730236));
#131992=CARTESIAN_POINT('Ctrl Pts',(26.2203209213991,10.27138042785,60.29879040396));
#131993=CARTESIAN_POINT('Ctrl Pts',(25.9689287341191,10.644849342,60.2655374623699));
#131994=CARTESIAN_POINT('Ctrl Pts',(25.8531256415191,10.80992702953,60.25094661876));
#131995=CARTESIAN_POINT('Ctrl Pts',(32.4394962150591,-0.167024129634686,
64.749778129328));
#131996=CARTESIAN_POINT('Ctrl Pts',(32.4395119001291,-0.166048254254086,
64.749778207149));
#131997=CARTESIAN_POINT('Ctrl Pts',(32.4433890940291,0.0773483601619742,
64.749797340987));
#131998=CARTESIAN_POINT('Ctrl Pts',(32.4333485056991,0.584125359624015,
64.749674192331));
#131999=CARTESIAN_POINT('Ctrl Pts',(32.3605007182391,1.36476629894001,64.749089885125));
#132000=CARTESIAN_POINT('Ctrl Pts',(32.2210472241191,2.18063018348501,64.747997284018));
#132001=CARTESIAN_POINT('Ctrl Pts',(32.0127791294291,3.00860637761601,64.7459906738651));
#132002=CARTESIAN_POINT('Ctrl Pts',(31.7401977260491,3.82775603881801,64.742789422125));
#132003=CARTESIAN_POINT('Ctrl Pts',(31.4134431009691,4.61757681790401,64.738144734598));
#132004=CARTESIAN_POINT('Ctrl Pts',(31.0452165535591,5.36205215158601,64.731695005533));
#132005=CARTESIAN_POINT('Ctrl Pts',(30.6455255091491,6.05580663071101,64.722864194901));
#132006=CARTESIAN_POINT('Ctrl Pts',(30.2207588970491,6.70093674850502,64.711266502485));
#132007=CARTESIAN_POINT('Ctrl Pts',(29.7720976663891,7.30453372749301,64.696364088189));
#132008=CARTESIAN_POINT('Ctrl Pts',(29.2980989030191,7.87385850082301,64.677553778107));
#132009=CARTESIAN_POINT('Ctrl Pts',(28.7946523707591,8.41600459963101,64.65389332063));
#132010=CARTESIAN_POINT('Ctrl Pts',(28.2960783560391,8.89829044039401,64.626420017414));
#132011=CARTESIAN_POINT('Ctrl Pts',(27.9617318331491,9.19221969143401,64.605290317917));
#132012=CARTESIAN_POINT('Ctrl Pts',(27.8087966595791,9.32115549717301,64.595039748394));
#132013=CARTESIAN_POINT('Ctrl Pts',(37.3447733550991,-0.163980749822586,
65.672020113937));
#132014=CARTESIAN_POINT('Ctrl Pts',(37.3447903319791,-0.163021244871686,
65.672013375157));
#132015=CARTESIAN_POINT('Ctrl Pts',(37.3489869127291,0.0762913557168342,
65.670347533373));
#132016=CARTESIAN_POINT('Ctrl Pts',(37.3381301106191,0.574047424134414,
65.6745698296091));
#132017=CARTESIAN_POINT('Ctrl Pts',(37.2592439496991,1.34342225796901,65.705562251813));
#132018=CARTESIAN_POINT('Ctrl Pts',(37.1076946494091,2.15544100000801,65.764984131401));
#132019=CARTESIAN_POINT('Ctrl Pts',(36.8799583449391,2.99224404832201,65.853458683805));
#132020=CARTESIAN_POINT('Ctrl Pts',(36.5791966436791,3.83427439653601,65.968635887493));
#132021=CARTESIAN_POINT('Ctrl Pts',(36.2143485134491,4.66159926833502,66.105852848797));
#132022=CARTESIAN_POINT('Ctrl Pts',(35.7971950983691,5.45638915732801,66.2592392798661));
#132023=CARTESIAN_POINT('Ctrl Pts',(35.3370171608391,6.20886237306701,66.423469431256));
#132024=CARTESIAN_POINT('Ctrl Pts',(34.8393757953291,6.91789819603101,66.595098260699));
#132025=CARTESIAN_POINT('Ctrl Pts',(34.3039881031491,7.58819161688801,66.772690714863));
#132026=CARTESIAN_POINT('Ctrl Pts',(33.7273674188191,8.22516768701401,66.955765342088));
#132027=CARTESIAN_POINT('Ctrl Pts',(33.1027247613091,8.83364473392301,67.144103602868));
#132028=CARTESIAN_POINT('Ctrl Pts',(32.4716469885691,9.37388448744801,67.323077248415));
#132029=CARTESIAN_POINT('Ctrl Pts',(32.0408207166291,9.70072437204801,67.43736279039));
#132030=CARTESIAN_POINT('Ctrl Pts',(31.8422612865091,9.84329152591,67.488269711376));
#132031=CARTESIAN_POINT('Ctrl Pts',(41.7851639409491,-0.181473624899186,
63.392785855529));
#132032=CARTESIAN_POINT('Ctrl Pts',(41.7851777637091,-0.180410219933086,
63.3927721742101));
#132033=CARTESIAN_POINT('Ctrl Pts',(41.7885946976491,0.0848151845503942,
63.389390169875));
#132034=CARTESIAN_POINT('Ctrl Pts',(41.7797551203791,0.635869761000514,
63.3980207821121));
#132035=CARTESIAN_POINT('Ctrl Pts',(41.7153723246291,1.49090770575301,63.461214595618));
#132036=CARTESIAN_POINT('Ctrl Pts',(41.5905957566191,2.40324030861401,63.5830492274001));
#132037=CARTESIAN_POINT('Ctrl Pts',(41.4001699495591,3.35995874213701,63.766573362888));
#132038=CARTESIAN_POINT('Ctrl Pts',(41.1431760010491,4.34268737770601,64.0092889910721));
#132039=CARTESIAN_POINT('Ctrl Pts',(40.8227513495791,5.33195090286801,64.304223540789));
#132040=CARTESIAN_POINT('Ctrl Pts',(40.4444080932191,6.30763911352001,64.6417970378541));
#132041=CARTESIAN_POINT('Ctrl Pts',(40.0123011460691,7.25493929209501,65.013174868938));
#132042=CARTESIAN_POINT('Ctrl Pts',(39.5278450183091,8.16940297534801,65.412835992148));
#132043=CARTESIAN_POINT('Ctrl Pts',(38.9871252392491,9.05378692831301,65.839532615121));
#132044=CARTESIAN_POINT('Ctrl Pts',(38.3827603673591,9.91205960048301,66.294105186865));
#132045=CARTESIAN_POINT('Ctrl Pts',(37.7036895340791,10.7467594847,66.778336709372));
#132046=CARTESIAN_POINT('Ctrl Pts',(36.9928132575991,11.49835899722,67.2558594670681));
#132047=CARTESIAN_POINT('Ctrl Pts',(36.4925142868991,11.95673360421,67.571962452628));
#132048=CARTESIAN_POINT('Ctrl Pts',(36.2590057995691,12.1569786201,67.715150981305));
#132049=CARTESIAN_POINT('',(28.7111341928544,9.91622892707765,64.1370768870198));
#132050=CARTESIAN_POINT('Ctrl Pts',(28.7109512875422,9.91605044034905,64.1371092663083));
#132051=CARTESIAN_POINT('Ctrl Pts',(29.148581955101,9.45497570515531,64.0599431720322));
#132052=CARTESIAN_POINT('Ctrl Pts',(29.5494667496106,8.96082664876228,63.9892563666044));
#132053=CARTESIAN_POINT('Ctrl Pts',(30.2796472512486,7.90616282799916,63.8605058433784));
#132054=CARTESIAN_POINT('Ctrl Pts',(30.6055849921346,7.34840822091101,63.803034225629));
#132055=CARTESIAN_POINT('Ctrl Pts',(30.8903745807655,6.76811552282497,63.7528181373285));
#132056=CARTESIAN_POINT('',(26.0609380919473,10.6024171740512,60.5235125955283));
#132057=CARTESIAN_POINT('Ctrl Pts',(26.0609344740391,10.60241468947,60.52351356035));
#132058=CARTESIAN_POINT('Ctrl Pts',(26.3648183022441,10.401891666185,61.146627197821));
#132059=CARTESIAN_POINT('Ctrl Pts',(26.7394129476864,10.2366073125495,61.7754982937505));
#132060=CARTESIAN_POINT('Ctrl Pts',(27.6275351327377,10.001078989055,62.9967881531343));
#132061=CARTESIAN_POINT('Ctrl Pts',(28.1411187061796,9.93108796101538,63.5888221040813));
#132062=CARTESIAN_POINT('Ctrl Pts',(28.7111243222551,9.91621952674004,64.1370786896818));
#132063=CARTESIAN_POINT('Ctrl Pts',(29.3346503782312,-0.000127443506814966,
61.2371509483293));
#132064=CARTESIAN_POINT('Ctrl Pts',(29.3346040565051,0.282953605848506,
61.2371193840476));
#132065=CARTESIAN_POINT('Ctrl Pts',(29.3281537463615,0.565553188024372,
61.2348664918606));
#132066=CARTESIAN_POINT('Ctrl Pts',(29.3154481518555,0.847407377566151,
61.2305057032888));
#132067=CARTESIAN_POINT('Ctrl Pts',(29.3021838212238,1.14165627384997,61.2259531464286));
#132068=CARTESIAN_POINT('Ctrl Pts',(29.2821023136189,1.43509359721723,61.2191030646222));
#132069=CARTESIAN_POINT('Ctrl Pts',(29.2553141053501,1.72742139194876,61.2100979542848));
#132070=CARTESIAN_POINT('Ctrl Pts',(29.2299254193272,2.00447682326973,61.2015633066271));
#132071=CARTESIAN_POINT('Ctrl Pts',(29.1985120692105,2.28053633570582,61.1910930274013));
#132072=CARTESIAN_POINT('Ctrl Pts',(29.1611184543843,2.55533716942498,61.1788202705036));
#132073=CARTESIAN_POINT('Ctrl Pts',(29.1590571741844,2.57048525072437,61.1781437488325));
#132074=CARTESIAN_POINT('Ctrl Pts',(29.1569777098301,2.58562950338368,61.1774617529707));
#132075=CARTESIAN_POINT('Ctrl Pts',(29.1548800644485,2.60076988187894,61.1767743062269));
#132076=CARTESIAN_POINT('Ctrl Pts',(29.1351359216109,2.74327909637595,61.1703036955026));
#132077=CARTESIAN_POINT('Ctrl Pts',(29.1137813215554,2.88544521608041,61.1633501010702));
#132078=CARTESIAN_POINT('Ctrl Pts',(29.0908380177679,3.02725396856825,61.1559509750705));
#132079=CARTESIAN_POINT('Ctrl Pts',(29.0484230490313,3.28941385012007,61.1422723130581));
#132080=CARTESIAN_POINT('Ctrl Pts',(29.0005809630906,3.55035400563275,61.1270704993233));
#132081=CARTESIAN_POINT('Ctrl Pts',(28.947416319256,3.80996623292663,61.1105886151822));
#132082=CARTESIAN_POINT('Ctrl Pts',(28.8951800522402,4.06504503431329,61.0943945426028));
#132083=CARTESIAN_POINT('Ctrl Pts',(28.8378053277324,4.31884238976034,61.0769648279692));
#132084=CARTESIAN_POINT('Ctrl Pts',(28.7753516804205,4.57122651109775,61.0585372022695));
#132085=CARTESIAN_POINT('Ctrl Pts',(28.7146812543561,4.81640438032536,61.0406357353308));
#132086=CARTESIAN_POINT('Ctrl Pts',(28.6492175358221,5.06024900272142,61.0217927282713));
#132087=CARTESIAN_POINT('Ctrl Pts',(28.5789805654299,5.30260498783434,61.0022306465424));
#132088=CARTESIAN_POINT('Ctrl Pts',(28.5507781664335,5.39991869816618,60.9943758425689));
#132089=CARTESIAN_POINT('Ctrl Pts',(28.5218058098204,5.49699196477918,60.9864051388434));
#132090=CARTESIAN_POINT('Ctrl Pts',(28.4920633168648,5.59381284229683,60.9783330220678));
#132091=CARTESIAN_POINT('Ctrl Pts',(28.4848734235303,5.61721813596013,60.9763816840045));
#132092=CARTESIAN_POINT('Ctrl Pts',(28.4776385217535,5.64060867527659,60.9744244196547));
#132093=CARTESIAN_POINT('Ctrl Pts',(28.4703586020432,5.66398428202551,60.9724614341921));
#132094=CARTESIAN_POINT('Ctrl Pts',(28.4590031072118,5.7004464398765,60.9693994950277));
#132095=CARTESIAN_POINT('Ctrl Pts',(28.4475380803588,5.73687226648814,60.966323635946));
#132096=CARTESIAN_POINT('Ctrl Pts',(28.4359635892217,5.77326141434145,60.9632347536892));
#132097=CARTESIAN_POINT('Ctrl Pts',(28.4264661853811,5.80312038857079,60.9607001833256));
#132098=CARTESIAN_POINT('Ctrl Pts',(28.416895075509,5.83295463521824,60.9581568278517));
#132099=CARTESIAN_POINT('Ctrl Pts',(28.4072502933072,5.86276398696542,60.9556052012388));
#132100=CARTESIAN_POINT('Ctrl Pts',(28.4024279022063,5.87766866283902,60.9543293879324));
#132101=CARTESIAN_POINT('Ctrl Pts',(28.3975870929037,5.8925671149521,60.9530515069221));
#132102=CARTESIAN_POINT('Ctrl Pts',(28.3927278679136,5.90745931329707,60.9517716181211));
#132103=CARTESIAN_POINT('Ctrl Pts',(28.3902982554186,5.91490541246956,60.9511316737206));
#132104=CARTESIAN_POINT('Ctrl Pts',(28.3878640389965,5.9223499481988,60.9504912273764));
#132105=CARTESIAN_POINT('Ctrl Pts',(28.3854252189674,5.92979291706548,60.949850286783));
#132106=CARTESIAN_POINT('Ctrl Pts',(28.3829863989383,5.93723588593217,60.9492093461897));
#132107=CARTESIAN_POINT('Ctrl Pts',(28.3801780333721,5.94578638788186,60.9484722163124));
#132108=CARTESIAN_POINT('Ctrl Pts',(28.3780949483526,5.95211711963359,60.947925989957));
#132109=CARTESIAN_POINT('Ctrl Pts',(28.3048789970587,6.17462870377922,60.9287273101853));
#132110=CARTESIAN_POINT('Ctrl Pts',(28.22739228315,6.39629757519428,60.9090858571923));
#132111=CARTESIAN_POINT('Ctrl Pts',(28.145553301647,6.61699125281535,60.8891871897609));
#132112=CARTESIAN_POINT('Ctrl Pts',(28.0652757589614,6.83347422706881,60.8696681770023));
#132113=CARTESIAN_POINT('Ctrl Pts',(27.9808100487485,7.04901915966549,60.8499020459908));
#132114=CARTESIAN_POINT('Ctrl Pts',(27.8920624579535,7.26345498945963,60.8300597329815));
#132115=CARTESIAN_POINT('Ctrl Pts',(27.805828513612,7.47181723620495,60.8107794246338));
#132116=CARTESIAN_POINT('Ctrl Pts',(27.7155513158858,7.67913243299848,60.7914275624999));
#132117=CARTESIAN_POINT('Ctrl Pts',(27.6211354006745,7.88519689102183,60.7721515041307));
#132118=CARTESIAN_POINT('Ctrl Pts',(27.5510318959288,8.03819906950659,60.7578390945508));
#132119=CARTESIAN_POINT('Ctrl Pts',(27.4786464523346,8.19051076703679,60.7435683264394));
#132120=CARTESIAN_POINT('Ctrl Pts',(27.4039391396142,8.3420307462116,60.7293940501294));
#132121=CARTESIAN_POINT('Ctrl Pts',(27.3367459515862,8.47831071774229,60.7166454345176));
#132122=CARTESIAN_POINT('Ctrl Pts',(27.2676743838534,8.6139500075147,60.7039748378232));
#132123=CARTESIAN_POINT('Ctrl Pts',(27.1966964811296,8.74886401607158,60.691417775478));
#132124=CARTESIAN_POINT('Ctrl Pts',(27.0948901072376,8.94237643995736,60.6734066912527));
#132125=CARTESIAN_POINT('Ctrl Pts',(26.9891610162539,9.13439839250478,60.6556304769479));
#132126=CARTESIAN_POINT('Ctrl Pts',(26.8794196045641,9.32469535356695,60.6381656550562));
#132127=CARTESIAN_POINT('Ctrl Pts',(26.7713769209198,9.51204663733419,60.6209711776253));
#132128=CARTESIAN_POINT('Ctrl Pts',(26.6594445193728,9.69772559687088,60.6040787935889));
#132129=CARTESIAN_POINT('Ctrl Pts',(26.5435554204452,9.88147066671254,60.5875343807167));
#132130=CARTESIAN_POINT('Ctrl Pts',(26.4299980517524,10.0615187198477,60.5713228473653));
#132131=CARTESIAN_POINT('Ctrl Pts',(26.312641021048,10.2397094160614,60.5554455552208));
#132132=CARTESIAN_POINT('Ctrl Pts',(26.1914483184166,10.4157662665093,60.5399165005658));
#132133=CARTESIAN_POINT('Ctrl Pts',(26.1484304803057,10.4782583549474,60.534404400046));
#132134=CARTESIAN_POINT('Ctrl Pts',(26.1049296699126,10.5404813492215,60.5289358943947));
#132135=CARTESIAN_POINT('Ctrl Pts',(26.0609453277637,10.6024221432137,60.5235106658849));
#132136=CARTESIAN_POINT('Ctrl Pts',(38.8135870908017,3.00384513004725E-5,
64.3914459355285));
#132137=CARTESIAN_POINT('Ctrl Pts',(38.8135820972561,0.192706244171883,
64.3914481968697));
#132138=CARTESIAN_POINT('Ctrl Pts',(38.8134083063988,0.387806629527274,
64.3935322941669));
#132139=CARTESIAN_POINT('Ctrl Pts',(38.8127385775239,0.585429506725301,
64.397923885268));
#132140=CARTESIAN_POINT('Ctrl Pts',(38.8121085403539,0.771340198272692,
64.4020552072595));
#132141=CARTESIAN_POINT('Ctrl Pts',(38.8110390230174,0.95948224467097,64.408229225816));
#132142=CARTESIAN_POINT('Ctrl Pts',(38.8093095217539,1.14994410220109,64.416628624266));
#132143=CARTESIAN_POINT('Ctrl Pts',(38.8086870405138,1.21849503983687,64.4196517316051));
#132144=CARTESIAN_POINT('Ctrl Pts',(38.8079791123787,1.2873467781357,64.4229634783117));
#132145=CARTESIAN_POINT('Ctrl Pts',(38.8071756217047,1.35650461339875,64.4265736374001));
#132146=CARTESIAN_POINT('Ctrl Pts',(38.8069873798435,1.37270691673054,64.4274194257681));
#132147=CARTESIAN_POINT('Ctrl Pts',(38.806793893207,1.38892602418888,64.4282815961541));
#132148=CARTESIAN_POINT('Ctrl Pts',(38.8065950324194,1.40516201022104,64.4291602798004));
#132149=CARTESIAN_POINT('Ctrl Pts',(38.8043449063288,1.58887352128373,64.4391026571894));
#132150=CARTESIAN_POINT('Ctrl Pts',(38.8014063278112,1.77474311766781,64.4511567002304));
#132151=CARTESIAN_POINT('Ctrl Pts',(38.7976161790703,1.96281884870537,64.4654920541126));
#132152=CARTESIAN_POINT('Ctrl Pts',(38.795522242117,2.06672472421815,64.4734118824058));
#132153=CARTESIAN_POINT('Ctrl Pts',(38.7931684751674,2.17130455486487,64.4820285567688));
#132154=CARTESIAN_POINT('Ctrl Pts',(38.7905278800185,2.27657201409169,64.4913748701255));
#132155=CARTESIAN_POINT('Ctrl Pts',(38.789267029482,2.32683588452887,64.4958376156603));
#132156=CARTESIAN_POINT('Ctrl Pts',(38.7879407867535,2.37725660874965,64.500466763006));
#132157=CARTESIAN_POINT('Ctrl Pts',(38.7865471193559,2.4278337674776,64.5052652859232));
#132158=CARTESIAN_POINT('Ctrl Pts',(38.7848700453846,2.48869594778754,64.51103960331));
#132159=CARTESIAN_POINT('Ctrl Pts',(38.7830953359685,2.54978464605298,64.517059179869));
#132160=CARTESIAN_POINT('Ctrl Pts',(38.781219494281,2.61109939041232,64.5233294322324));
#132161=CARTESIAN_POINT('Ctrl Pts',(38.7802815734372,2.64175676259198,64.5264645584142));
#132162=CARTESIAN_POINT('Ctrl Pts',(38.7793183701495,2.67247064594839,64.5296623570849));
#132163=CARTESIAN_POINT('Ctrl Pts',(38.7783294509264,2.7032410152705,64.5329235298439));
#132164=CARTESIAN_POINT('Ctrl Pts',(38.7778349913149,2.71862619993155,64.5345541162234));
#132165=CARTESIAN_POINT('Ctrl Pts',(38.7773341027581,2.7340255060635,64.536200546343));
#132166=CARTESIAN_POINT('Ctrl Pts',(38.7768267312168,2.74943893151487,64.5378629093229));
#132167=CARTESIAN_POINT('Ctrl Pts',(38.7765730454461,2.75714564424056,64.5386940908129));
#132168=CARTESIAN_POINT('Ctrl Pts',(38.7763177389317,2.76485588679473,64.5395292555312));
#132169=CARTESIAN_POINT('Ctrl Pts',(38.776060804929,2.77256965903347,64.5403684147119));
#132170=CARTESIAN_POINT('Ctrl Pts',(38.7758038709264,2.78028343127222,64.5412075738926));
#132171=CARTESIAN_POINT('Ctrl Pts',(38.7754963970519,2.7894521186308,64.5422099791408));
#132172=CARTESIAN_POINT('Ctrl Pts',(38.7752851137195,2.79572156469527,64.5428978869322));
#132173=CARTESIAN_POINT('Ctrl Pts',(38.7710886572831,2.92024372642544,64.5565609385614));
#132174=CARTESIAN_POINT('Ctrl Pts',(38.7665003779421,3.05057812754349,64.5717655398374));
#132175=CARTESIAN_POINT('Ctrl Pts',(38.7610604810182,3.18673981322833,64.5888571002793));
#132176=CARTESIAN_POINT('Ctrl Pts',(38.7549253313141,3.34030381220565,64.6081330688239));
#132177=CARTESIAN_POINT('Ctrl Pts',(38.7477065709253,3.50128046984096,64.6298086462359));
#132178=CARTESIAN_POINT('Ctrl Pts',(38.738733342239,3.66967113078567,64.654417207798));
#132179=CARTESIAN_POINT('Ctrl Pts',(38.7309997754733,3.81479842717775,64.6756260681205));
#132180=CARTESIAN_POINT('Ctrl Pts',(38.7219625628368,3.96543251726767,64.6990143256146));
#132181=CARTESIAN_POINT('Ctrl Pts',(38.711181534982,4.12156833073821,64.7249519486975));
#132182=CARTESIAN_POINT('Ctrl Pts',(38.6993179051263,4.29338288526685,64.7534941585625));
#132183=CARTESIAN_POINT('Ctrl Pts',(38.6853434491788,4.4718616116839,64.7851231239542));
#132184=CARTESIAN_POINT('Ctrl Pts',(38.6686427422749,4.65694578221642,64.8203651711238));
#132185=CARTESIAN_POINT('Ctrl Pts',(38.6566479590734,4.78987695167738,64.8456767173838));
#132186=CARTESIAN_POINT('Ctrl Pts',(38.643246518751,4.92621491879245,64.8728528240778));
#132187=CARTESIAN_POINT('Ctrl Pts',(38.6282032124862,5.0659271041141,64.9020988916168));
#132188=CARTESIAN_POINT('Ctrl Pts',(38.6144690008673,5.19348129234847,64.9287999155496));
#132189=CARTESIAN_POINT('Ctrl Pts',(38.5993665687579,5.32384849862264,64.9572264447523));
#132190=CARTESIAN_POINT('Ctrl Pts',(38.5826941727004,5.45698250875477,64.987540669278));
#132191=CARTESIAN_POINT('Ctrl Pts',(38.5731193768813,5.53344008325061,65.0049498352579));
#132192=CARTESIAN_POINT('Ctrl Pts',(38.563026619093,5.61080991664418,65.0229816761299));
#132193=CARTESIAN_POINT('Ctrl Pts',(38.5523761053502,5.6890808590101,65.0416675976743));
#132194=CARTESIAN_POINT('Ctrl Pts',(38.5470508484787,5.72821633019306,65.0510105584466));
#132195=CARTESIAN_POINT('Ctrl Pts',(38.5415861542849,5.76757707657575,65.0605170488365));
#132196=CARTESIAN_POINT('Ctrl Pts',(38.5359769028551,5.80716148728286,65.0701910325787));
#132197=CARTESIAN_POINT('Ctrl Pts',(38.5331722771402,5.82695369263642,65.0750280244498));
#132198=CARTESIAN_POINT('Ctrl Pts',(38.5303315122135,5.84680181395491,65.0799068902103));
#132199=CARTESIAN_POINT('Ctrl Pts',(38.5274539635382,5.86670564209971,65.0848281279772));
#132200=CARTESIAN_POINT('Ctrl Pts',(38.5260151892006,5.87665755617211,65.0872887468607));
#132201=CARTESIAN_POINT('Ctrl Pts',(38.5245672189318,5.88662339694342,65.0897599587801));
#132202=CARTESIAN_POINT('Ctrl Pts',(38.5231099716393,5.89660313747531,65.0922418261374));
#132203=CARTESIAN_POINT('Ctrl Pts',(38.5218348802584,5.90533541044071,65.094413460075));
#132204=CARTESIAN_POINT('Ctrl Pts',(38.5205526861564,5.91407832540984,65.0965932520843));
#132205=CARTESIAN_POINT('Ctrl Pts',(38.5192633348198,5.92283186404408,65.0987812440293));
#132206=CARTESIAN_POINT('Ctrl Pts',(38.5190791417718,5.92408236956326,65.0990938143072));
#132207=CARTESIAN_POINT('Ctrl Pts',(38.5187288748741,5.92645819778244,65.0996879815923));
#132208=CARTESIAN_POINT('Ctrl Pts',(38.518710317313,5.92658403096877,65.0997194570216));
#132209=CARTESIAN_POINT('Ctrl Pts',(38.5176144759863,5.93401459820143,65.101578110536));
#132210=CARTESIAN_POINT('Ctrl Pts',(38.515667100619,5.94740709121132,65.1049243388498));
#132211=CARTESIAN_POINT('Ctrl Pts',(38.5128218551399,5.96675695826927,65.1097938036597));
#132212=CARTESIAN_POINT('Ctrl Pts',(38.5112591083899,5.97738484330801,65.1124683497972));
#132213=CARTESIAN_POINT('Ctrl Pts',(38.5094247736796,5.98980984107125,65.1156029740003));
#132214=CARTESIAN_POINT('Ctrl Pts',(38.5073058910958,6.00403060254209,65.1192076456793));
#132215=CARTESIAN_POINT('Ctrl Pts',(38.5034388974516,6.0299837132257,65.1257862275123));
#132216=CARTESIAN_POINT('Ctrl Pts',(38.4986265569299,6.06191828979016,65.133928546497));
#132217=CARTESIAN_POINT('Ctrl Pts',(38.4927581848926,6.09982199600826,65.1437197725091));
#132218=CARTESIAN_POINT('Ctrl Pts',(38.4868802194934,6.13778766557277,65.1535270047958));
#132219=CARTESIAN_POINT('Ctrl Pts',(38.4799427498706,6.18174212272886,65.1649885645098));
#132220=CARTESIAN_POINT('Ctrl Pts',(38.4717934127655,6.23166615807523,65.1782216012355));
#132221=CARTESIAN_POINT('Ctrl Pts',(38.4636310427066,6.28167003521022,65.1914758011006));
#132222=CARTESIAN_POINT('Ctrl Pts',(38.4542529101786,6.3376627778107,65.2065071918731));
#132223=CARTESIAN_POINT('Ctrl Pts',(38.4434649420875,6.3996159803555,65.2234646158817));
#132224=CARTESIAN_POINT('Ctrl Pts',(38.4326805962475,6.46154838101719,65.2404163461353));
#132225=CARTESIAN_POINT('Ctrl Pts',(38.4204873439494,6.5294374749201,65.259292893285));
#132226=CARTESIAN_POINT('Ctrl Pts',(38.4066506692628,6.60324270730986,65.2802731239176));
#132227=CARTESIAN_POINT('Ctrl Pts',(38.39286939175,6.67675244953393,65.3011693570933));
#132228=CARTESIAN_POINT('Ctrl Pts',(38.3774578062107,6.75613134498252,65.3241525857494));
#132229=CARTESIAN_POINT('Ctrl Pts',(38.3601442014692,6.84132331852189,65.349427957903));
#132230=CARTESIAN_POINT('Ctrl Pts',(38.3547333605568,6.86794748042917,65.357327007221));
#132231=CARTESIAN_POINT('Ctrl Pts',(38.349136458325,6.89513926088066,65.3654501285514));
#132232=CARTESIAN_POINT('Ctrl Pts',(38.3433443968407,6.92289654971471,65.3738041241803));
#132233=CARTESIAN_POINT('Ctrl Pts',(38.3302782335287,6.98551350742247,65.3926496891818));
#132234=CARTESIAN_POINT('Ctrl Pts',(38.316219613751,7.05100866780108,65.4126697325342));
#132235=CARTESIAN_POINT('Ctrl Pts',(38.3010560936442,7.11935545607374,65.4339474345147));
#132236=CARTESIAN_POINT('Ctrl Pts',(38.2894153604296,7.17182392795556,65.4502819037164));
#132237=CARTESIAN_POINT('Ctrl Pts',(38.2771232685237,7.225972869957,65.4673576902076));
#132238=CARTESIAN_POINT('Ctrl Pts',(38.2641246953319,7.28178792485946,65.48521493203));
#132239=CARTESIAN_POINT('Ctrl Pts',(38.2576254087359,7.30969545231069,65.4941435529412));
#132240=CARTESIAN_POINT('Ctrl Pts',(38.2509495069607,7.33801949982202,65.5032675668473));
#132241=CARTESIAN_POINT('Ctrl Pts',(38.2440896730612,7.3667580259864,65.512592188913));
#132242=CARTESIAN_POINT('Ctrl Pts',(38.2406597561114,7.38112728906859,65.5172544999459));
#132243=CARTESIAN_POINT('Ctrl Pts',(38.2371838564442,7.39560017132269,65.5219669647981));
#132244=CARTESIAN_POINT('Ctrl Pts',(38.2336610480672,7.41017640708869,65.5267302462064));
#132245=CARTESIAN_POINT('Ctrl Pts',(38.2318996438786,7.41746452497169,65.5291118869106));
#132246=CARTESIAN_POINT('Ctrl Pts',(38.230126512532,7.42477848120126,65.5315062318641));
#132247=CARTESIAN_POINT('Ctrl Pts',(38.2283415368226,7.43211824162908,65.5339133646321));
#132248=CARTESIAN_POINT('Ctrl Pts',(38.2274490489679,7.43578812184299,65.535116931016));
#132249=CARTESIAN_POINT('Ctrl Pts',(38.2265536000237,7.43946445310452,65.5363236943605));
#132250=CARTESIAN_POINT('Ctrl Pts',(38.2256551752428,7.44314723108138,65.5375336651556));
#132251=CARTESIAN_POINT('Ctrl Pts',(38.2247567504619,7.44683000905825,65.5387436359507));
#132252=CARTESIAN_POINT('Ctrl Pts',(38.2235147663237,7.45191098024706,65.5404148952795));
#132253=CARTESIAN_POINT('Ctrl Pts',(38.2229509586165,7.4542149008017,65.5411732104112));
#132254=CARTESIAN_POINT('Ctrl Pts',(38.1916849363716,7.58197908420835,65.5832256645933));
#132255=CARTESIAN_POINT('Ctrl Pts',(38.1596549613227,7.70530747405823,65.6251569615781));
#132256=CARTESIAN_POINT('Ctrl Pts',(38.1271540676055,7.82421379407133,65.666726707534));
#132257=CARTESIAN_POINT('Ctrl Pts',(38.087141251882,7.9706028968584,65.7179044566469));
#132258=CARTESIAN_POINT('Ctrl Pts',(38.0464155863636,8.11028986157072,65.7685331157816));
#132259=CARTESIAN_POINT('Ctrl Pts',(38.0054821089969,8.24334003244639,65.8182073193746));
#132260=CARTESIAN_POINT('Ctrl Pts',(37.9645486316303,8.37639020332206,65.8678815229677));
#132261=CARTESIAN_POINT('Ctrl Pts',(37.9234072600134,8.50280361865002,65.9166012267983));
#132262=CARTESIAN_POINT('Ctrl Pts',(37.8825226040607,8.62265784585839,65.9640032148954));
#132263=CARTESIAN_POINT('Ctrl Pts',(37.8720105022222,8.65347429307648,65.9761910275263));
#132264=CARTESIAN_POINT('Ctrl Pts',(37.8615151664394,8.6838571813318,65.9882919458989));
#132265=CARTESIAN_POINT('Ctrl Pts',(37.8510440635881,8.71380795371077,66.0003002512402));
#132266=CARTESIAN_POINT('Ctrl Pts',(37.8424268442424,8.7384560140752,66.0101825150824));
#132267=CARTESIAN_POINT('Ctrl Pts',(37.8338260325903,8.7628114254635,66.0200020601993));
#132268=CARTESIAN_POINT('Ctrl Pts',(37.8252456323684,8.78687508443175,66.0297558031867));
#132269=CARTESIAN_POINT('Ctrl Pts',(37.8157422509733,8.813527236199,66.0405587421222));
#132270=CARTESIAN_POINT('Ctrl Pts',(37.8062639679525,8.83982145500476,66.051280935983));
#132271=CARTESIAN_POINT('Ctrl Pts',(37.7968160555023,8.86575901704537,66.061918341461));
#132272=CARTESIAN_POINT('Ctrl Pts',(37.7920920992772,8.87872779806568,66.0672370442));
#132273=CARTESIAN_POINT('Ctrl Pts',(37.7873757359399,8.89160741441799,66.0725345512341));
#132274=CARTESIAN_POINT('Ctrl Pts',(37.7826676268362,8.90439801829518,66.0778103637185));
#132275=CARTESIAN_POINT('Ctrl Pts',(37.7803135722843,8.91079332023378,66.0804482699607));
#132276=CARTESIAN_POINT('Ctrl Pts',(37.7779615813058,8.91716636902401,66.0830807526508));
#132277=CARTESIAN_POINT('Ctrl Pts',(37.7756117355492,8.92351718410612,66.0857077503478));
#132278=CARTESIAN_POINT('Ctrl Pts',(37.7732618897927,8.92986799918824,66.0883347480448));
#132279=CARTESIAN_POINT('Ctrl Pts',(37.7716146995104,8.93431309154039,66.0901749639149));
#132280=CARTESIAN_POINT('Ctrl Pts',(37.7685687154191,8.94250294763226,66.0935722274305));
#132281=CARTESIAN_POINT('Ctrl Pts',(37.6865595247574,9.16300425348457,66.1850391632491));
#132282=CARTESIAN_POINT('Ctrl Pts',(37.5981393895329,9.38096554045745,66.2799356242712));
#132283=CARTESIAN_POINT('Ctrl Pts',(37.5032569308291,9.5959827456451,66.377974791091));
#132284=CARTESIAN_POINT('Ctrl Pts',(37.4097025963978,9.80799023151144,66.4746416473817));
#132285=CARTESIAN_POINT('Ctrl Pts',(37.3098648312833,10.0171347851144,66.5743637156262));
#132286=CARTESIAN_POINT('Ctrl Pts',(37.2037041734696,10.2230579005808,66.6768286946188));
#132287=CARTESIAN_POINT('Ctrl Pts',(37.1603529916719,10.3071475303811,66.7186707293582));
#132288=CARTESIAN_POINT('Ctrl Pts',(37.1159475219664,10.3906995226895,66.760969733924));
#132289=CARTESIAN_POINT('Ctrl Pts',(37.0704854132497,10.4736876985386,66.8037027644647));
#132290=CARTESIAN_POINT('Ctrl Pts',(36.9539219146008,10.6864669205439,66.9132689875966));
#132291=CARTESIAN_POINT('Ctrl Pts',(36.8304107459624,10.8955419080915,67.0256912169882));
#132292=CARTESIAN_POINT('Ctrl Pts',(36.6999028887975,11.1005327456061,67.140552801349));
#132293=CARTESIAN_POINT('Ctrl Pts',(36.646808624253,11.1839287800875,67.1872817223393));
#132294=CARTESIAN_POINT('Ctrl Pts',(36.5925565519594,11.2666484735295,67.2344139344862));
#132295=CARTESIAN_POINT('Ctrl Pts',(36.5371442385606,11.3486648066635,67.2819196312367));
#132296=CARTESIAN_POINT('Ctrl Pts',(36.4166606394213,11.5269938169157,67.3852117873128));
#132297=CARTESIAN_POINT('Ctrl Pts',(36.2906906955439,11.7019983860824,67.4902710991956));
#132298=CARTESIAN_POINT('Ctrl Pts',(36.1592882551018,11.8733756711545,67.5967554170151));
#132299=CARTESIAN_POINT('Ctrl Pts',(29.9859214083691,12.46437431082,79.070188223874));
#132300=CARTESIAN_POINT('Ctrl Pts',(29.8857014163891,12.47044857532,79.090205232738));
#132301=CARTESIAN_POINT('Ctrl Pts',(29.6104280963791,12.4897806276,79.145015827581));
#132302=CARTESIAN_POINT('Ctrl Pts',(29.1457827926491,12.5346015555,79.236730680776));
#132303=CARTESIAN_POINT('Ctrl Pts',(28.5738695769491,12.60957457799,79.348292639236));
#132304=CARTESIAN_POINT('Ctrl Pts',(28.0282967728591,12.70185657079,79.453349622617));
#132305=CARTESIAN_POINT('Ctrl Pts',(27.6733467087591,12.77424630289,79.52093552273));
#132306=CARTESIAN_POINT('Ctrl Pts',(27.5249257075591,12.80670959195,79.549068580612));
#132307=CARTESIAN_POINT('Ctrl Pts',(30.0308651063291,13.45208857236,79.385705808435));
#132308=CARTESIAN_POINT('Ctrl Pts',(29.9359068375091,13.45982740229,79.399762458128));
#132309=CARTESIAN_POINT('Ctrl Pts',(29.6751805090291,13.4834545797,79.438192693413));
#132310=CARTESIAN_POINT('Ctrl Pts',(29.2355716482891,13.53421738821,79.502277776235));
#132311=CARTESIAN_POINT('Ctrl Pts',(28.6953648245591,13.61430233658,79.580029006533));
#132312=CARTESIAN_POINT('Ctrl Pts',(28.1810574803591,13.70908983217,79.653211426916));
#132313=CARTESIAN_POINT('Ctrl Pts',(27.8470766860091,13.78168016274,79.700369027776));
#132314=CARTESIAN_POINT('Ctrl Pts',(27.7075360699391,13.81397234352,79.720024504347));
#132315=CARTESIAN_POINT('Ctrl Pts',(29.9227251759491,14.31914031007,78.82563632132));
#132316=CARTESIAN_POINT('Ctrl Pts',(29.8324306026191,14.32407596873,78.834452846557));
#132317=CARTESIAN_POINT('Ctrl Pts',(29.5843934297591,14.33979311782,78.858607745173));
#132318=CARTESIAN_POINT('Ctrl Pts',(29.1656884915291,14.3762918562,78.899185618871));
#132319=CARTESIAN_POINT('Ctrl Pts',(28.6504842183591,14.4374986971,78.9490683359909));
#132320=CARTESIAN_POINT('Ctrl Pts',(28.1593784162991,14.51307015343,78.996867416962));
#132321=CARTESIAN_POINT('Ctrl Pts',(27.8401641858791,14.57254123544,79.028243803073));
#132322=CARTESIAN_POINT('Ctrl Pts',(27.7067467992491,14.59925012658,79.041431119251));
#132323=CARTESIAN_POINT('Ctrl Pts',(29.7422836619591,14.41782971493,77.8083595247319));
#132324=CARTESIAN_POINT('Ctrl Pts',(29.6525709105191,14.41758847387,77.816570606694));
#132325=CARTESIAN_POINT('Ctrl Pts',(29.4058860801291,14.41909934329,77.839219068241));
#132326=CARTESIAN_POINT('Ctrl Pts',(28.9883370206291,14.43178352124,77.877972508984));
#132327=CARTESIAN_POINT('Ctrl Pts',(28.4727542006591,14.46422443239,77.926747098128));
#132328=CARTESIAN_POINT('Ctrl Pts',(27.9794541455991,14.51321295826,77.974615773832));
#132329=CARTESIAN_POINT('Ctrl Pts',(27.6577729429091,14.55604520736,78.006646818456));
#132330=CARTESIAN_POINT('Ctrl Pts',(27.5231474917591,14.57592942316,78.020207201693));
#132331=CARTESIAN_POINT('Origin',(29.5680409582791,12.92381928297,77.694240492923));
#132332=CARTESIAN_POINT('Origin',(34.5835698427891,12.92381190166,76.809867428062));
#132333=CARTESIAN_POINT('Ctrl Pts',(33.859212171956,12.923698620032,78.460731142598));
#132334=CARTESIAN_POINT('Ctrl Pts',(33.8592330215353,12.9682330973519,78.4607308814309));
#132335=CARTESIAN_POINT('Ctrl Pts',(33.8589027995551,13.0134405826951,78.458775094831));
#132336=CARTESIAN_POINT('Ctrl Pts',(33.858195831669,13.0590476424942,78.4547074451838));
#132337=CARTESIAN_POINT('Ctrl Pts',(33.8574929818102,13.1043890450873,78.4506634892464));
#132338=CARTESIAN_POINT('Ctrl Pts',(33.8564177039448,13.1501248925192,78.4445318705706));
#132339=CARTESIAN_POINT('Ctrl Pts',(33.8549525564639,13.1959615089143,78.4362031281502));
#132340=CARTESIAN_POINT('Ctrl Pts',(33.8534967317702,13.2415064652354,78.4279273818239));
#132341=CARTESIAN_POINT('Ctrl Pts',(33.8516559441973,13.2871503581839,78.4174821624424));
#132342=CARTESIAN_POINT('Ctrl Pts',(33.8494215183369,13.3325881208068,78.4048079246059));
#132343=CARTESIAN_POINT('Ctrl Pts',(33.8485692243438,13.3499197910253,78.3999734939964));
#132344=CARTESIAN_POINT('Ctrl Pts',(33.8476597488197,13.3672213377937,78.3948152677034));
#132345=CARTESIAN_POINT('Ctrl Pts',(33.8466929517904,13.3844754437921,78.3893318777936));
#132346=CARTESIAN_POINT('Ctrl Pts',(33.8442933552275,13.4273002479616,78.3757220680998));
#132347=CARTESIAN_POINT('Ctrl Pts',(33.8415402198523,13.4698282902136,78.360106775778));
#132348=CARTESIAN_POINT('Ctrl Pts',(33.8384375007938,13.5117692111429,78.342508579162));
#132349=CARTESIAN_POINT('Ctrl Pts',(33.835341716617,13.553616389997,78.3249497162428));
#132350=CARTESIAN_POINT('Ctrl Pts',(33.8318979241246,13.5948784493562,78.3054168847981));
#132351=CARTESIAN_POINT('Ctrl Pts',(33.8281189268964,13.6352754672863,78.283982844231));
#132352=CARTESIAN_POINT('Ctrl Pts',(33.8243454303277,13.6756136838386,78.2625800027767));
#132353=CARTESIAN_POINT('Ctrl Pts',(33.8202377395313,13.7150887785906,78.2392816835676));
#132354=CARTESIAN_POINT('Ctrl Pts',(33.8158170891901,13.753439665697,78.2142084605291));
#132355=CARTESIAN_POINT('Ctrl Pts',(33.8131665113712,13.7764344747988,78.1991748062687));
#132356=CARTESIAN_POINT('Ctrl Pts',(33.810403583591,13.7990255042493,78.1835039757881));
#132357=CARTESIAN_POINT('Ctrl Pts',(33.8075342494431,13.821160836655,78.1672297083637));
#132358=CARTESIAN_POINT('Ctrl Pts',(33.8027477314033,13.8580861867245,78.1400815720378));
#132359=CARTESIAN_POINT('Ctrl Pts',(33.7976655387112,13.8937354478372,78.1112566664626));
#132360=CARTESIAN_POINT('Ctrl Pts',(33.7923212707233,13.9278946034537,78.0809456828264));
#132361=CARTESIAN_POINT('Ctrl Pts',(33.7869735948705,13.9620755412472,78.0506153708668));
#132362=CARTESIAN_POINT('Ctrl Pts',(33.7813635916826,13.9947640491257,78.0187975517465));
#132363=CARTESIAN_POINT('Ctrl Pts',(33.7755310657962,14.0257841675171,77.9857181088134));
#132364=CARTESIAN_POINT('Ctrl Pts',(33.7696813509459,14.0568957049104,77.9525411778689));
#132365=CARTESIAN_POINT('Ctrl Pts',(33.7636078935501,14.0863286700283,77.9180957071712));
#132366=CARTESIAN_POINT('Ctrl Pts',(33.7573557026574,14.1139499662343,77.8826370969955));
#132367=CARTESIAN_POINT('Ctrl Pts',(33.753619333804,14.1304567160449,77.8614466936765));
#132368=CARTESIAN_POINT('Ctrl Pts',(33.7498192191244,14.1463173315367,77.8398949514358));
#132369=CARTESIAN_POINT('Ctrl Pts',(33.7459655687823,14.1615115822075,77.8180398051419));
#132370=CARTESIAN_POINT('Ctrl Pts',(33.7391493068818,14.1883868777734,77.7793828467295));
#132371=CARTESIAN_POINT('Ctrl Pts',(33.7321663331587,14.2131715935981,77.7397810915173));
#132372=CARTESIAN_POINT('Ctrl Pts',(33.725070623432,14.2358167896528,77.6995388812372));
#132373=CARTESIAN_POINT('Ctrl Pts',(33.7179458023146,14.2585548915865,77.6591315702484));
#132374=CARTESIAN_POINT('Ctrl Pts',(33.7107074246475,14.2791359137209,77.6180791416206));
#132375=CARTESIAN_POINT('Ctrl Pts',(33.7034103001888,14.2975630174627,77.5766906447098));
#132376=CARTESIAN_POINT('Ctrl Pts',(33.6960537060775,14.3161402972723,77.5349648423925));
#132377=CARTESIAN_POINT('Ctrl Pts',(33.6886375073168,14.3325285302607,77.4928980591992));
#132378=CARTESIAN_POINT('Ctrl Pts',(33.6812164409681,14.3467833059797,77.4507988880263));
#132379=CARTESIAN_POINT('Ctrl Pts',(33.6784238764152,14.3521474112864,77.4349568718525));
#132380=CARTESIAN_POINT('Ctrl Pts',(33.6756306002789,14.3572099280516,77.4191101428676));
#132381=CARTESIAN_POINT('Ctrl Pts',(33.67283943295,14.3619756402683,77.4032745984495));
#132382=CARTESIAN_POINT('Origin',(33.9027788805691,-12.77732087006,79.976189078581));
#132383=CARTESIAN_POINT('',(35.3799890432589,11.6378875163018,79.715708490352));
#132384=CARTESIAN_POINT('Origin',(33.9027998622653,11.6379092722801,79.9761546590259));
#132385=CARTESIAN_POINT('',(35.3799958958808,-11.6378856606036,79.7157076007637));
#132386=CARTESIAN_POINT('',(35.3799907980991,-11.63788566034,79.715708499663));
#132387=CARTESIAN_POINT('Ctrl Pts',(35.3799880137154,-11.6378856588156,
79.7157026548483));
#132388=CARTESIAN_POINT('Ctrl Pts',(35.3695520560716,-11.6378709771185,
79.6565207146777));
#132389=CARTESIAN_POINT('Ctrl Pts',(35.3555553115347,-11.6378607889906,
79.5979668413592));
#132390=CARTESIAN_POINT('Ctrl Pts',(35.3380986507356,-11.637853719103,79.5404630667693));
#132391=CARTESIAN_POINT('Ctrl Pts',(35.3206441808791,-11.6378466501027,
79.4829665093374));
#132392=CARTESIAN_POINT('Ctrl Pts',(35.2997307855574,-11.63784269856,79.4265201864714));
#132393=CARTESIAN_POINT('Ctrl Pts',(35.2755091568529,-11.6378404896635,
79.3715308374448));
#132394=CARTESIAN_POINT('Ctrl Pts',(35.2512868264982,-11.637838280703,79.3165398954914));
#132395=CARTESIAN_POINT('Ctrl Pts',(35.2237562392352,-11.6378378144897,
79.2630063941493));
#132396=CARTESIAN_POINT('Ctrl Pts',(35.1931157868798,-11.6378377160928,
79.2113161033672));
#132397=CARTESIAN_POINT('Ctrl Pts',(35.1849189661822,-11.63783768977,79.1974881076041));
#132398=CARTESIAN_POINT('Ctrl Pts',(35.176499843879,-11.63783768977,79.1837918872206));
#132399=CARTESIAN_POINT('Ctrl Pts',(35.1678627706239,-11.63783768977,79.1702345196114));
#132400=CARTESIAN_POINT('Ctrl Pts',(35.1355720633058,-11.63783768977,79.1195487170784));
#132401=CARTESIAN_POINT('Ctrl Pts',(35.1002317032601,-11.63783768977,79.0708060227495));
#132402=CARTESIAN_POINT('Ctrl Pts',(35.0620964188945,-11.63783768977,79.024357767197));
#132403=CARTESIAN_POINT('Ctrl Pts',(35.0239637323516,-11.63783768977,78.977912675757));
#132404=CARTESIAN_POINT('Ctrl Pts',(34.9830367677872,-11.63783768977,78.9337620329779));
#132405=CARTESIAN_POINT('Ctrl Pts',(34.9396104809761,-11.63783768977,78.8922240273005));
#132406=CARTESIAN_POINT('Ctrl Pts',(34.8961866618653,-11.63783768977,78.8506883820219));
#132407=CARTESIAN_POINT('Ctrl Pts',(34.8502641066618,-11.63783768977,78.8117653652228));
#132408=CARTESIAN_POINT('Ctrl Pts',(34.8021737362379,-11.63783768977,78.7757354586537));
#132409=CARTESIAN_POINT('Ctrl Pts',(34.7540753816382,-11.63783768977,78.7396995702404));
#132410=CARTESIAN_POINT('Ctrl Pts',(34.7038088254441,-11.63783768977,78.7065580044565));
#132411=CARTESIAN_POINT('Ctrl Pts',(34.651736411703,-11.63783768977,78.6765496606816));
#132412=CARTESIAN_POINT('Ctrl Pts',(34.5996711332875,-11.63783768977,78.6465454288595));
#132413=CARTESIAN_POINT('Ctrl Pts',(34.5458008546994,-11.63783768977,78.6196737679673));
#132414=CARTESIAN_POINT('Ctrl Pts',(34.4905137910617,-11.63783768977,78.5961283281108));
#132415=CARTESIAN_POINT('Ctrl Pts',(34.4352229874562,-11.63783768977,78.5725812954914));
#132416=CARTESIAN_POINT('Ctrl Pts',(34.3785155912039,-11.63783768977,78.5523610981484));
#132417=CARTESIAN_POINT('Ctrl Pts',(34.3208003182326,-11.63783768977,78.535613472216));
#132418=CARTESIAN_POINT('Ctrl Pts',(34.2899453102775,-11.63783768977,78.5266600686408));
#132419=CARTESIAN_POINT('Ctrl Pts',(34.2588025590782,-11.63783768977,78.5186983117861));
#132420=CARTESIAN_POINT('Ctrl Pts',(34.2274363156242,-11.63783768977,78.5117446276497));
#132421=CARTESIAN_POINT('Ctrl Pts',(34.1687709160204,-11.63783768977,78.4987389051386));
#132422=CARTESIAN_POINT('Ctrl Pts',(34.1093232084526,-11.63783768977,78.4892626423694));
#132423=CARTESIAN_POINT('Ctrl Pts',(34.0495216251489,-11.6378376897611,
78.4833841459414));
#132424=CARTESIAN_POINT('Ctrl Pts',(33.9897275200442,-11.6378376897522,
78.4775063846205));
#132425=CARTESIAN_POINT('Ctrl Pts',(33.9295800437199,-11.6378376897345,
78.4752255297055));
#132426=CARTESIAN_POINT('Ctrl Pts',(33.8695125657921,-11.6378376896989,
78.4765580065166));
#132427=CARTESIAN_POINT('Ctrl Pts',(33.8094432159812,-11.6378376896634,
78.4778905248516));
#132428=CARTESIAN_POINT('Ctrl Pts',(33.7494542873367,-11.6378376896101,
78.4828365910624));
#132429=CARTESIAN_POINT('Ctrl Pts',(33.6899780297751,-11.6378376895301,
78.4913605369974));
#132430=CARTESIAN_POINT('Ctrl Pts',(33.6740480624911,-11.6378376895087,
78.4936435686716));
#132431=CARTESIAN_POINT('Ctrl Pts',(33.6581548467044,-11.6378376894854,
78.4961829780519));
#132432=CARTESIAN_POINT('Ctrl Pts',(33.6423066140169,-11.63783768946,78.4989774490718));
#132433=CARTESIAN_POINT('Ctrl Pts',(36.4624006913807,-13.6175309807164,
78.8714913648239));
#132434=CARTESIAN_POINT('Ctrl Pts',(36.4624006913807,-13.6175309807164,
78.8714913648239));
#132435=CARTESIAN_POINT('Ctrl Pts',(36.4624006913807,-13.6175309807164,
78.8714913648239));
#132436=CARTESIAN_POINT('Ctrl Pts',(36.4624006913807,-13.6175309807164,
78.8714913648239));
#132437=CARTESIAN_POINT('Ctrl Pts',(36.4624006913807,-13.6175309807164,
78.8714913648239));
#132438=CARTESIAN_POINT('Ctrl Pts',(36.4624006913807,-13.6175309807164,
78.8714913648239));
#132439=CARTESIAN_POINT('Ctrl Pts',(36.4624006913807,-13.6175309807164,
78.8714913648239));
#132440=CARTESIAN_POINT('Ctrl Pts',(36.4624006913807,-13.6175309807164,
78.8714913648239));
#132441=CARTESIAN_POINT('Ctrl Pts',(36.4624006913807,-13.6175309807164,
78.8714913648239));
#132442=CARTESIAN_POINT('Ctrl Pts',(36.5087707847954,-13.6295464641391,
78.8593182230073));
#132443=CARTESIAN_POINT('Ctrl Pts',(36.5147533430926,-13.621753782623,78.8765850066188));
#132444=CARTESIAN_POINT('Ctrl Pts',(36.5128106723893,-13.6240150405474,
78.8715208625787));
#132445=CARTESIAN_POINT('Ctrl Pts',(36.5203475397483,-13.605877824589,78.9100485185392));
#132446=CARTESIAN_POINT('Ctrl Pts',(36.5241109898786,-13.5968212093523,
78.9292868711512));
#132447=CARTESIAN_POINT('Ctrl Pts',(36.5278744400088,-13.5877645941156,
78.9485252237633));
#132448=CARTESIAN_POINT('Ctrl Pts',(36.539056905061,-13.5608543708176,79.0056887833431));
#132449=CARTESIAN_POINT('Ctrl Pts',(36.5502393701132,-13.5339441475196,
79.062852342923));
#132450=CARTESIAN_POINT('Ctrl Pts',(36.5614218351653,-13.5070339242215,
79.1200159025029));
#132451=CARTESIAN_POINT('Ctrl Pts',(36.554898911248,-13.6392407963244,78.8462285202114));
#132452=CARTESIAN_POINT('Ctrl Pts',(36.5644326177738,-13.6265498978342,
78.8733225560771));
#132453=CARTESIAN_POINT('Ctrl Pts',(36.5607337607929,-13.6312719831418,
78.8635158637679));
#132454=CARTESIAN_POINT('Ctrl Pts',(36.5755647018899,-13.598691414449,78.9332013525492));
#132455=CARTESIAN_POINT('Ctrl Pts',(36.5829703658806,-13.5824226731206,
78.9679980192992));
#132456=CARTESIAN_POINT('Ctrl Pts',(36.5903760298713,-13.5661539317922,
79.0027946860492));
#132457=CARTESIAN_POINT('Ctrl Pts',(36.6123807265986,-13.5178140773893,
79.1061871839961));
#132458=CARTESIAN_POINT('Ctrl Pts',(36.6343854233258,-13.4694742229864,
79.2095796819431));
#132459=CARTESIAN_POINT('Ctrl Pts',(36.6563901200531,-13.4211343685835,
79.31297217989));
#132460=CARTESIAN_POINT('Ctrl Pts',(36.646046826565,-13.6541488424738,78.8185742721227));
#132461=CARTESIAN_POINT('Ctrl Pts',(36.6560492376511,-13.6408860043036,
78.8469292136561));
#132462=CARTESIAN_POINT('Ctrl Pts',(36.6516381391679,-13.6466133680293,
78.8348889376155));
#132463=CARTESIAN_POINT('Ctrl Pts',(36.6698272747732,-13.6089261693074,
78.9158412543503));
#132464=CARTESIAN_POINT('Ctrl Pts',(36.678909815503,-13.590107489585,78.9562638851925));
#132465=CARTESIAN_POINT('Ctrl Pts',(36.6879923562327,-13.5712888098627,
78.9966865160346));
#132466=CARTESIAN_POINT('Ctrl Pts',(36.7149796128139,-13.5153722383551,
79.1167956289673));
#132467=CARTESIAN_POINT('Ctrl Pts',(36.7419668693951,-13.4594556668474,
79.2369047419));
#132468=CARTESIAN_POINT('Ctrl Pts',(36.7689541259764,-13.4035390953398,
79.3570138548327));
#132469=CARTESIAN_POINT('Ctrl Pts',(36.6910658924978,-13.6593662375177,
78.8040117096523));
#132470=CARTESIAN_POINT('Ctrl Pts',(36.6980086982724,-13.6500749817604,
78.8236273955465));
#132471=CARTESIAN_POINT('Ctrl Pts',(36.6946216542961,-13.6545438906777,
78.8142013835284));
#132472=CARTESIAN_POINT('Ctrl Pts',(36.7088642892985,-13.6262319890973,
78.8752406196854));
#132473=CARTESIAN_POINT('Ctrl Pts',(36.7159761892433,-13.6120947587846,
78.9057198772234));
#132474=CARTESIAN_POINT('Ctrl Pts',(36.7230880891881,-13.5979575284719,
78.9361991347614));
#132475=CARTESIAN_POINT('Ctrl Pts',(36.7442199149957,-13.5559511039319,
79.0267631705372));
#132476=CARTESIAN_POINT('Ctrl Pts',(36.7653517408033,-13.5139446793919,
79.1173272063129));
#132477=CARTESIAN_POINT('Ctrl Pts',(36.7864835666109,-13.4719382548519,
79.2078912420887));
#132478=CARTESIAN_POINT('Ctrl Pts',(36.735264603282,-13.662485738696,78.7888968893297));
#132479=CARTESIAN_POINT('Ctrl Pts',(36.735264603282,-13.662485738696,78.7888968893297));
#132480=CARTESIAN_POINT('Ctrl Pts',(36.735264603282,-13.662485738696,78.7888968893297));
#132481=CARTESIAN_POINT('Ctrl Pts',(36.735264603282,-13.662485738696,78.7888968893297));
#132482=CARTESIAN_POINT('Ctrl Pts',(36.735264603282,-13.662485738696,78.7888968893297));
#132483=CARTESIAN_POINT('Ctrl Pts',(36.735264603282,-13.662485738696,78.7888968893297));
#132484=CARTESIAN_POINT('Ctrl Pts',(36.735264603282,-13.662485738696,78.7888968893297));
#132485=CARTESIAN_POINT('Ctrl Pts',(36.735264603282,-13.662485738696,78.7888968893297));
#132486=CARTESIAN_POINT('Ctrl Pts',(36.735264603282,-13.662485738696,78.7888968893297));
#132487=CARTESIAN_POINT('',(36.4640508930212,-13.6179550204625,78.87106300086));
#132488=CARTESIAN_POINT('Origin',(36.6259767577074,-12.2926480245168,78.1865226505801));
#132489=CARTESIAN_POINT('',(36.646332255877,-13.6311708400759,78.8663936093756));
#132490=CARTESIAN_POINT('Ctrl Pts',(36.4640508930212,-13.6179550204625,
78.87106300086));
#132491=CARTESIAN_POINT('Ctrl Pts',(36.4641834917382,-13.6179473140954,
78.8711126536229));
#132492=CARTESIAN_POINT('Ctrl Pts',(36.4644911975365,-13.6179838279465,
78.8711182044604));
#132493=CARTESIAN_POINT('Ctrl Pts',(36.4649737737274,-13.6180415198724,
78.871125291467));
#132494=CARTESIAN_POINT('Ctrl Pts',(36.4655876503714,-13.6181149087518,
78.871134306723));
#132495=CARTESIAN_POINT('Ctrl Pts',(36.4664838602382,-13.6182233599688,
78.8711440605703));
#132496=CARTESIAN_POINT('Ctrl Pts',(36.4676360949594,-13.6183510738823,
78.8711764188561));
#132497=CARTESIAN_POINT('Ctrl Pts',(36.4690935083757,-13.6185126138598,
78.8712173474958));
#132498=CARTESIAN_POINT('Ctrl Pts',(36.4709596083455,-13.6187054886973,
78.8712931103674));
#132499=CARTESIAN_POINT('Ctrl Pts',(36.4731615799429,-13.6189260841508,
78.871383593139));
#132500=CARTESIAN_POINT('Ctrl Pts',(36.4745159257299,-13.6190617637042,
78.8714392455193));
#132501=CARTESIAN_POINT('Ctrl Pts',(36.4759971252191,-13.6192083478747,
78.8714995350199));
#132502=CARTESIAN_POINT('Ctrl Pts',(36.4775866615851,-13.6193689971118,
78.8715511966506));
#132503=CARTESIAN_POINT('Ctrl Pts',(36.481498301009,-13.6197643337036,78.8716783291124));
#132504=CARTESIAN_POINT('Ctrl Pts',(36.4860955308366,-13.6201950577805,
78.8718621100866));
#132505=CARTESIAN_POINT('Ctrl Pts',(36.4913605508575,-13.6206584093813,
78.872062869958));
#132506=CARTESIAN_POINT('Ctrl Pts',(36.4944173529083,-13.6209274252859,
78.8721794285245));
#132507=CARTESIAN_POINT('Ctrl Pts',(36.498427044011,-13.6212734725104,78.872318854442));
#132508=CARTESIAN_POINT('Ctrl Pts',(36.5021159668906,-13.6215799022322,
78.8724371945187));
#132509=CARTESIAN_POINT('Ctrl Pts',(36.5047808256736,-13.6218012654762,
78.8725226827773));
#132510=CARTESIAN_POINT('Ctrl Pts',(36.5072783975182,-13.6220034758983,
78.8725962439108));
#132511=CARTESIAN_POINT('Ctrl Pts',(36.5091329606862,-13.6221552057529,
78.8726410581783));
#132512=CARTESIAN_POINT('Ctrl Pts',(36.5113438638537,-13.6223360893281,
78.8726944831614));
#132513=CARTESIAN_POINT('Ctrl Pts',(36.513894066682,-13.6225288354596,78.8727781102579));
#132514=CARTESIAN_POINT('Ctrl Pts',(36.5167833448577,-13.6227214582233,
78.8729055097517));
#132515=CARTESIAN_POINT('Ctrl Pts',(36.5184740378156,-13.6228341735557,
78.8729800589692));
#132516=CARTESIAN_POINT('Ctrl Pts',(36.5197239075041,-13.6229146600396,
78.8730370241672));
#132517=CARTESIAN_POINT('Ctrl Pts',(36.5215109915733,-13.623017746904,78.8731367032908));
#132518=CARTESIAN_POINT('Ctrl Pts',(36.5227779114705,-13.6230908284125,
78.873207368945));
#132519=CARTESIAN_POINT('Ctrl Pts',(36.5243147509991,-13.6231754392616,
78.8732990990183));
#132520=CARTESIAN_POINT('Ctrl Pts',(36.5264694745122,-13.6232799356834,
78.8734448705763));
#132521=CARTESIAN_POINT('Ctrl Pts',(36.5316635946536,-13.6235318320244,
78.8737962636813));
#132522=CARTESIAN_POINT('Ctrl Pts',(36.5359073745668,-13.6236836049445,
78.8741393503315));
#132523=CARTESIAN_POINT('Ctrl Pts',(36.5392037712793,-13.6237853428906,
78.8744231137472));
#132524=CARTESIAN_POINT('Ctrl Pts',(36.5411147015973,-13.6238443206602,
78.8745876121863));
#132525=CARTESIAN_POINT('Ctrl Pts',(36.541964118272,-13.6238622908226,78.8746733276918));
#132526=CARTESIAN_POINT('Ctrl Pts',(36.5430437731837,-13.6238905992486,
78.87477082179));
#132527=CARTESIAN_POINT('Ctrl Pts',(36.5438265466757,-13.6239111234784,
78.8748415071497));
#132528=CARTESIAN_POINT('Ctrl Pts',(36.5447303543849,-13.6239366598944,
78.8749188999794));
#132529=CARTESIAN_POINT('Ctrl Pts',(36.5462476870491,-13.6239763351117,
78.8750492221757));
#132530=CARTESIAN_POINT('Ctrl Pts',(36.5525034608565,-13.6241399110965,
78.8755865243777));
#132531=CARTESIAN_POINT('Ctrl Pts',(36.5592164190559,-13.6243250047039,
78.8760561426797));
#132532=CARTESIAN_POINT('Ctrl Pts',(36.5659768361521,-13.6245795260801,
78.8762820986765));
#132533=CARTESIAN_POINT('Ctrl Pts',(36.5713532118987,-13.6247819400044,
78.8764617953317));
#132534=CARTESIAN_POINT('Ctrl Pts',(36.576758741326,-13.6250305635944,78.8764832172777));
#132535=CARTESIAN_POINT('Ctrl Pts',(36.5819898328604,-13.6253560057479,
78.8762639167306));
#132536=CARTESIAN_POINT('Ctrl Pts',(36.585364772629,-13.6255659710408,78.8761224307457));
#132537=CARTESIAN_POINT('Ctrl Pts',(36.5886671911254,-13.6258079351807,
78.8758810768004));
#132538=CARTESIAN_POINT('Ctrl Pts',(36.5918452765511,-13.6260865301216,
78.8755292468544));
#132539=CARTESIAN_POINT('Ctrl Pts',(36.5987888095358,-13.6266952089023,
78.8747605630377));
#132540=CARTESIAN_POINT('Ctrl Pts',(36.6053277000037,-13.6272886118807,
78.8738825820606));
#132541=CARTESIAN_POINT('Ctrl Pts',(36.6114802495672,-13.6278560793253,
78.8729530400328));
#132542=CARTESIAN_POINT('Ctrl Pts',(36.6176999701247,-13.628429742145,78.8720133496492));
#132543=CARTESIAN_POINT('Ctrl Pts',(36.6235248914239,-13.6289742806592,
78.8710195194918));
#132544=CARTESIAN_POINT('Ctrl Pts',(36.6289738469251,-13.6294787066028,
78.8700292146934));
#132545=CARTESIAN_POINT('Ctrl Pts',(36.7432179278938,-13.636198950746,78.846992041912));
#132546=CARTESIAN_POINT('Ctrl Pts',(36.7108115055979,-13.6358752288811,
78.8531074637301));
#132547=CARTESIAN_POINT('Ctrl Pts',(36.6784828947467,-13.6342021234484,
78.8595796977137));
#132548=CARTESIAN_POINT('Ctrl Pts',(36.646332255877,-13.6311708400759,78.8663936093756));
#132549=CARTESIAN_POINT('Ctrl Pts',(36.0413541965395,-13.5385524084063,
78.8219185637222));
#132550=CARTESIAN_POINT('Ctrl Pts',(36.0443390692377,-13.5362121365262,
78.8266178467828));
#132551=CARTESIAN_POINT('Ctrl Pts',(36.0545148270121,-13.5280801594399,
78.8429498748798));
#132552=CARTESIAN_POINT('Ctrl Pts',(36.0694283772597,-13.5152701077307,
78.8686972121326));
#132553=CARTESIAN_POINT('Ctrl Pts',(36.0839605510938,-13.5014873949538,
78.8964610094424));
#132554=CARTESIAN_POINT('Ctrl Pts',(36.0945588044003,-13.4901669739601,
78.9192863632301));
#132555=CARTESIAN_POINT('Ctrl Pts',(36.1008211011128,-13.4824751555828,
78.9346626965391));
#132556=CARTESIAN_POINT('Ctrl Pts',(36.1030740999561,-13.4787635377289,
78.9421913259183));
#132557=CARTESIAN_POINT('Ctrl Pts',(36.1031818402804,-13.4783683893573,
78.9428310903551));
#132558=CARTESIAN_POINT('Ctrl Pts',(36.0764411019647,-13.5628769378654,
78.8083910122847));
#132559=CARTESIAN_POINT('Ctrl Pts',(36.0795496624071,-13.5604610111995,
78.8132750854961));
#132560=CARTESIAN_POINT('Ctrl Pts',(36.0901598135502,-13.5520573333247,
78.8302669905896));
#132561=CARTESIAN_POINT('Ctrl Pts',(36.1057882041297,-13.5387628136805,
78.8571683985934));
#132562=CARTESIAN_POINT('Ctrl Pts',(36.1211176864259,-13.5243725536988,
78.8863481172406));
#132563=CARTESIAN_POINT('Ctrl Pts',(36.1324763252156,-13.5124084261907,
78.9106408618895));
#132564=CARTESIAN_POINT('Ctrl Pts',(36.1394869313789,-13.5039781844258,
78.9276665689722));
#132565=CARTESIAN_POINT('Ctrl Pts',(36.1421967665385,-13.4997783128599,
78.9362679756959));
#132566=CARTESIAN_POINT('Ctrl Pts',(36.1425452691223,-13.4990816441658,
78.9375681334444));
#132567=CARTESIAN_POINT('Ctrl Pts',(36.1120453547769,-13.5856109486442,
78.7937519683683));
#132568=CARTESIAN_POINT('Ctrl Pts',(36.1152797484648,-13.5831184353831,
78.7988231638101));
#132569=CARTESIAN_POINT('Ctrl Pts',(36.1263318291934,-13.5744396714938,
78.8164833502305));
#132570=CARTESIAN_POINT('Ctrl Pts',(36.1426874700359,-13.5606544072964,
78.8445540039736));
#132571=CARTESIAN_POINT('Ctrl Pts',(36.1588280835953,-13.545648404286,78.8751689131062));
#132572=CARTESIAN_POINT('Ctrl Pts',(36.1709603469915,-13.5330314196273,
78.9009499735806));
#132573=CARTESIAN_POINT('Ctrl Pts',(36.178732400364,-13.5238515041513,78.9196501725559));
#132574=CARTESIAN_POINT('Ctrl Pts',(36.1819071181667,-13.5191557445104,
78.9293410910961));
#132575=CARTESIAN_POINT('Ctrl Pts',(36.1825006715159,-13.5181525710206,
78.9313125421451));
#132576=CARTESIAN_POINT('Ctrl Pts',(36.1480898606898,-13.6067252227425,
78.7780424920219));
#132577=CARTESIAN_POINT('Ctrl Pts',(36.1514519573532,-13.6041553550248,
78.783302740626));
#132578=CARTESIAN_POINT('Ctrl Pts',(36.1629525353573,-13.5951987091683,
78.8016381792719));
#132579=CARTESIAN_POINT('Ctrl Pts',(36.1800462424778,-13.580917477517,78.8308907408642));
#132580=CARTESIAN_POINT('Ctrl Pts',(36.1970100325351,-13.5652888611044,
78.8629570185049));
#132581=CARTESIAN_POINT('Ctrl Pts',(36.2099274637118,-13.552011278801,78.8902441044039));
#132582=CARTESIAN_POINT('Ctrl Pts',(36.2184724316828,-13.5420720662877,
78.9106402793977));
#132583=CARTESIAN_POINT('Ctrl Pts',(36.2221190583888,-13.5368738624281,
78.9214350756853));
#132584=CARTESIAN_POINT('Ctrl Pts',(36.2229614128174,-13.5355598688766,
78.9240872545302));
#132585=CARTESIAN_POINT('',(36.1480898606898,-13.6067252227425,78.7780424920219));
#132586=CARTESIAN_POINT('',(36.1887546648804,-13.5728292529327,78.847489288857));
#132587=CARTESIAN_POINT('Origin',(36.1118745043311,-13.5960811534144,78.8009259388539));
#132588=CARTESIAN_POINT('',(36.0446752548501,-13.5408399095576,78.8206418568075));
#132589=CARTESIAN_POINT('Origin',(36.5006306047883,-12.3981418696704,77.9625345273951));
#132590=CARTESIAN_POINT('Ctrl Pts',(36.0446774732356,-13.5408384751336,
78.8206449445472));
#132591=CARTESIAN_POINT('Ctrl Pts',(36.0916850857421,-13.5518449805492,
78.8309651869554));
#132592=CARTESIAN_POINT('Ctrl Pts',(36.1397079808775,-13.562648531607,78.8400689323397));
#132593=CARTESIAN_POINT('Ctrl Pts',(36.1887545950258,-13.5728294813495,
78.8474894372116));
#132594=CARTESIAN_POINT('Ctrl Pts',(36.1480898606898,-13.6067252227425,
78.7780424920219));
#132595=CARTESIAN_POINT('Ctrl Pts',(36.1514519573532,-13.6041553550248,
78.783302740626));
#132596=CARTESIAN_POINT('Ctrl Pts',(36.1629525353573,-13.5951987091683,
78.8016381792719));
#132597=CARTESIAN_POINT('Ctrl Pts',(36.1800462424778,-13.580917477517,78.8308907408642));
#132598=CARTESIAN_POINT('Ctrl Pts',(36.1970100325351,-13.5652888611044,
78.8629570185049));
#132599=CARTESIAN_POINT('Ctrl Pts',(36.2099274637118,-13.552011278801,78.8902441044039));
#132600=CARTESIAN_POINT('Ctrl Pts',(36.2184724316828,-13.5420720662877,
78.9106402793977));
#132601=CARTESIAN_POINT('Ctrl Pts',(36.2221190583888,-13.5368738624281,
78.9214350756853));
#132602=CARTESIAN_POINT('Ctrl Pts',(36.2229614128174,-13.5355598688766,
78.9240872545302));
#132603=CARTESIAN_POINT('Ctrl Pts',(36.2992619131484,-13.6952793052796,
78.712156340383));
#132604=CARTESIAN_POINT('Ctrl Pts',(36.3031596010323,-13.692385009978,78.7182094852644));
#132605=CARTESIAN_POINT('Ctrl Pts',(36.3165411939635,-13.6822629163989,
78.7393769578717));
#132606=CARTESIAN_POINT('Ctrl Pts',(36.3367303796114,-13.6659015780555,
78.7735864867146));
#132607=CARTESIAN_POINT('Ctrl Pts',(36.357146603752,-13.6476616969434,78.8117398600354));
#132608=CARTESIAN_POINT('Ctrl Pts',(36.3733570589803,-13.6316135425576,
78.8453432748377));
#132609=CARTESIAN_POINT('Ctrl Pts',(36.3851436606838,-13.6184898088911,
78.8728524388754));
#132610=CARTESIAN_POINT('Ctrl Pts',(36.3907694915897,-13.611184334537,78.8882769411472));
#132611=CARTESIAN_POINT('Ctrl Pts',(36.3926553273718,-13.6085667496204,
78.8937841187074));
#132612=CARTESIAN_POINT('Ctrl Pts',(36.4537997192532,-13.7531348275884,
78.6295167031115));
#132613=CARTESIAN_POINT('Ctrl Pts',(36.4582503159403,-13.7499119605313,
78.6363738171947));
#132614=CARTESIAN_POINT('Ctrl Pts',(36.4735737634649,-13.7386088786915,
78.6604141624838));
#132615=CARTESIAN_POINT('Ctrl Pts',(36.4969586862089,-13.7201356487196,
78.6996601572554));
#132616=CARTESIAN_POINT('Ctrl Pts',(36.5209388506112,-13.6992391416549,
78.7440091958987));
#132617=CARTESIAN_POINT('Ctrl Pts',(36.5405496289052,-13.6803644397312,
78.784057646114));
#132618=CARTESIAN_POINT('Ctrl Pts',(36.555685304629,-13.6639792082828,78.8188515496762));
#132619=CARTESIAN_POINT('Ctrl Pts',(36.5633563690056,-13.6545122521614,
78.8390241994241));
#132620=CARTESIAN_POINT('Ctrl Pts',(36.5663212970924,-13.6505530241725,
78.8474694278411));
#132621=CARTESIAN_POINT('Ctrl Pts',(36.6061800233323,-13.7808703344089,
78.5343153943199));
#132622=CARTESIAN_POINT('Ctrl Pts',(36.6111806483402,-13.7773262453333,
78.5419593493064));
#132623=CARTESIAN_POINT('Ctrl Pts',(36.6284358515173,-13.7648680007667,
78.5688125275726));
#132624=CARTESIAN_POINT('Ctrl Pts',(36.6550000141886,-13.7443253975173,
78.6129969813538));
#132625=CARTESIAN_POINT('Ctrl Pts',(36.6825254422131,-13.7208208173866,
78.6634310023575));
#132626=CARTESIAN_POINT('Ctrl Pts',(36.7055195608249,-13.6991641521518,
78.7098238115797));
#132627=CARTESIAN_POINT('Ctrl Pts',(36.7239891966374,-13.6795575058957,
78.7518127609135));
#132628=CARTESIAN_POINT('Ctrl Pts',(36.7336966470516,-13.6679526999726,
78.7766810540519));
#132629=CARTESIAN_POINT('Ctrl Pts',(36.7377367084417,-13.6626624594582,
78.7880407996123));
#132630=CARTESIAN_POINT('Ctrl Pts',(36.1887545950258,-13.5728294813495,
78.8474894372116));
#132631=CARTESIAN_POINT('Ctrl Pts',(36.2103531003999,-13.5773124084669,
78.8507555351564));
#132632=CARTESIAN_POINT('Ctrl Pts',(36.2333779264413,-13.5820188593518,
78.8537513247424));
#132633=CARTESIAN_POINT('Ctrl Pts',(36.2700715262227,-13.5890837908734,
78.8578224956519));
#132634=CARTESIAN_POINT('Ctrl Pts',(36.2826588017725,-13.5914430098648,
78.8591009144093));
#132635=CARTESIAN_POINT('Ctrl Pts',(36.3020645457527,-13.594948564419,78.8608867383133));
#132636=CARTESIAN_POINT('Ctrl Pts',(36.3086204007986,-13.5961116785867,
78.8614596409308));
#132637=CARTESIAN_POINT('Ctrl Pts',(36.3219066323604,-13.5984171078203,
78.8625653497166));
#132638=CARTESIAN_POINT('Ctrl Pts',(36.3302025631481,-13.5998173492539,
78.8632181139596));
#132639=CARTESIAN_POINT('Ctrl Pts',(36.3774837518109,-13.607618724868,78.8668175026506));
#132640=CARTESIAN_POINT('Ctrl Pts',(36.4205818929086,-13.6132479681494,
78.8698470622943));
#132641=CARTESIAN_POINT('Ctrl Pts',(36.4640390336471,-13.6179681794182,
78.8710264250399));
#132642=CARTESIAN_POINT('Origin',(36.500517881468,-12.3982157262051,77.9623752096788));
#132643=CARTESIAN_POINT('Ctrl Pts',(33.8458695692469,-12.9128498070933,
78.4631124071519));
#132644=CARTESIAN_POINT('Ctrl Pts',(33.8804362530074,-12.9129747103335,
78.4567626655418));
#132645=CARTESIAN_POINT('Ctrl Pts',(33.9826122819526,-12.9119078622902,
78.4409210188779));
#132646=CARTESIAN_POINT('Ctrl Pts',(34.1471526591361,-12.9034887777877,
78.4290883853484));
#132647=CARTESIAN_POINT('Ctrl Pts',(34.3311801082618,-12.8847575734329,
78.4347345631763));
#132648=CARTESIAN_POINT('Ctrl Pts',(34.4943806698859,-12.8605115333373,
78.4549675889316));
#132649=CARTESIAN_POINT('Ctrl Pts',(34.6376087672186,-12.8328563598802,
78.4851552568926));
#132650=CARTESIAN_POINT('Ctrl Pts',(34.7622094291334,-12.8033920014129,
78.5216784145264));
#132651=CARTESIAN_POINT('Ctrl Pts',(34.8698019746813,-12.7733116204556,
78.5617757514179));
#132652=CARTESIAN_POINT('Ctrl Pts',(34.9620805957375,-12.7434939376387,
78.6033721543705));
#132653=CARTESIAN_POINT('Ctrl Pts',(35.0406096689484,-12.7145884065802,
78.6448937820371));
#132654=CARTESIAN_POINT('Ctrl Pts',(35.1067871905256,-12.6871002078555,
78.6851310414152));
#132655=CARTESIAN_POINT('Ctrl Pts',(35.1618042910709,-12.6614673796507,
78.7230847384953));
#132656=CARTESIAN_POINT('Ctrl Pts',(35.2067591673776,-12.638064763268,78.7579355717776));
#132657=CARTESIAN_POINT('Ctrl Pts',(35.2427975912993,-12.6171473317229,
78.7891118095416));
#132658=CARTESIAN_POINT('Ctrl Pts',(35.2711482263803,-12.5988148329409,
78.8163469814348));
#132659=CARTESIAN_POINT('Ctrl Pts',(35.2924658755658,-12.5832772605048,
78.8390556915725));
#132660=CARTESIAN_POINT('Ctrl Pts',(35.307594129335,-12.5706238579202,78.8569665984833));
#132661=CARTESIAN_POINT('Ctrl Pts',(35.3161484118183,-12.5620595878754,
78.868320030909));
#132662=CARTESIAN_POINT('Ctrl Pts',(35.3193543369156,-12.5580624372546,
78.8730441549028));
#132663=CARTESIAN_POINT('Ctrl Pts',(35.3202691478143,-12.5567666477221,
78.8744528479851));
#132664=CARTESIAN_POINT('Ctrl Pts',(33.8456503110567,-13.1996018417486,
78.4652773762441));
#132665=CARTESIAN_POINT('Ctrl Pts',(33.8817341482106,-13.1997300776071,
78.4586391357277));
#132666=CARTESIAN_POINT('Ctrl Pts',(33.9884075750797,-13.1986344466374,
78.442183999269));
#132667=CARTESIAN_POINT('Ctrl Pts',(34.1602613719234,-13.1899904211345,
78.4304739338996));
#132668=CARTESIAN_POINT('Ctrl Pts',(34.3526252622446,-13.1707383594976,
78.4377877021175));
#132669=CARTESIAN_POINT('Ctrl Pts',(34.5234134998431,-13.1457760760133,
78.4607551811517));
#132670=CARTESIAN_POINT('Ctrl Pts',(34.6735293868505,-13.117241205332,78.4944083592027));
#132671=CARTESIAN_POINT('Ctrl Pts',(34.8043784561376,-13.0867587194026,
78.5348810387088));
#132672=CARTESIAN_POINT('Ctrl Pts',(34.9176431493598,-13.0555426788163,
78.5792333474792));
#132673=CARTESIAN_POINT('Ctrl Pts',(35.0150809485904,-13.0244894070125,
78.6252639513317));
#132674=CARTESIAN_POINT('Ctrl Pts',(35.0983262747713,-12.9942599913201,
78.6713200250023));
#132675=CARTESIAN_POINT('Ctrl Pts',(35.1688308592319,-12.9653700241188,
78.7161364225069));
#132676=CARTESIAN_POINT('Ctrl Pts',(35.2278214704078,-12.9382698112071,
78.7586663017047));
#132677=CARTESIAN_POINT('Ctrl Pts',(35.2764170860985,-12.9133502711739,
78.798043119068));
#132678=CARTESIAN_POINT('Ctrl Pts',(35.3157809568853,-12.8908828291008,
78.8336565464687));
#132679=CARTESIAN_POINT('Ctrl Pts',(35.3471570245691,-12.8709847417339,
78.8652070156515));
#132680=CARTESIAN_POINT('Ctrl Pts',(35.3712663398007,-12.8538549257744,
78.8921474444993));
#132681=CARTESIAN_POINT('Ctrl Pts',(35.3889799319516,-12.8395820074481,
78.9142198800224));
#132682=CARTESIAN_POINT('Ctrl Pts',(35.3996646373259,-12.8295547046685,
78.9292177539998));
#132683=CARTESIAN_POINT('Ctrl Pts',(35.4041355774772,-12.8246203414302,
78.9362229220246));
#132684=CARTESIAN_POINT('Ctrl Pts',(35.4055167149387,-12.8229685286228,
78.9384907818235));
#132685=CARTESIAN_POINT('Ctrl Pts',(33.830959299843,-13.4811758603199,78.3886016868916));
#132686=CARTESIAN_POINT('Ctrl Pts',(33.8700008488003,-13.4813078297855,
78.3814104950211));
#132687=CARTESIAN_POINT('Ctrl Pts',(33.9854233930445,-13.4801797753416,
78.363681584177));
#132688=CARTESIAN_POINT('Ctrl Pts',(34.1714180492613,-13.4712835724188,
78.3515924091162));
#132689=CARTESIAN_POINT('Ctrl Pts',(34.379783168837,-13.451436218611,78.3607835554978));
#132690=CARTESIAN_POINT('Ctrl Pts',(34.5650427439325,-13.4256328239301,
78.3873046950815));
#132691=CARTESIAN_POINT('Ctrl Pts',(34.7282218355506,-13.3960332628245,
78.4256839226055));
#132692=CARTESIAN_POINT('Ctrl Pts',(34.8708633928763,-13.3642806825697,
78.471684431699));
#132693=CARTESIAN_POINT('Ctrl Pts',(34.9947868847451,-13.331606452154,78.5220980344836));
#132694=CARTESIAN_POINT('Ctrl Pts',(35.1018829476443,-13.2989233549325,
78.5745332487887));
#132695=CARTESIAN_POINT('Ctrl Pts',(35.1939288624648,-13.2669023334983,
78.6272195490899));
#132696=CARTESIAN_POINT('Ctrl Pts',(35.2724856408592,-13.2360689329893,
78.6788095232723));
#132697=CARTESIAN_POINT('Ctrl Pts',(35.3388534094284,-13.2068875266087,
78.7281857189888));
#132698=CARTESIAN_POINT('Ctrl Pts',(35.3941952422174,-13.1797704356727,
78.7744099921202));
#132699=CARTESIAN_POINT('Ctrl Pts',(35.4397110275899,-13.1550129019841,
78.8168114512847));
#132700=CARTESIAN_POINT('Ctrl Pts',(35.4766760070711,-13.1327600841396,
78.8550347205036));
#132701=CARTESIAN_POINT('Ctrl Pts',(35.5059391995938,-13.1131891801329,
78.8886010640387));
#132702=CARTESIAN_POINT('Ctrl Pts',(35.5284245683134,-13.0963864512112,
78.9172756129049));
#132703=CARTESIAN_POINT('Ctrl Pts',(35.5430419032332,-13.0840310911762,
78.938135949469));
#132704=CARTESIAN_POINT('Ctrl Pts',(35.5498485579447,-13.0775832102601,
78.9488534430825));
#132705=CARTESIAN_POINT('Ctrl Pts',(35.552090839722,-13.0753531353839,78.9525261362449));
#132706=CARTESIAN_POINT('Ctrl Pts',(33.8015018549743,-13.7317040852684,
78.231178210434));
#132707=CARTESIAN_POINT('Ctrl Pts',(33.8448367011614,-13.7318398987138,
78.2231897821826));
#132708=CARTESIAN_POINT('Ctrl Pts',(33.9729484993377,-13.7306782863685,
78.2035675708194));
#132709=CARTESIAN_POINT('Ctrl Pts',(34.1794028973399,-13.7215222815351,
78.1905757013909));
#132710=CARTESIAN_POINT('Ctrl Pts',(34.410851781839,-13.7010503656952,78.2017087925164));
#132711=CARTESIAN_POINT('Ctrl Pts',(34.6169343870141,-13.67434261052,78.2323749945655));
#132712=CARTESIAN_POINT('Ctrl Pts',(34.7988676057059,-13.6435683591641,
78.2764569312182));
#132713=CARTESIAN_POINT('Ctrl Pts',(34.9584049522099,-13.6103796896382,
78.3292431282214));
#132714=CARTESIAN_POINT('Ctrl Pts',(35.097572763067,-13.576019734666,78.3871814162859));
#132715=CARTESIAN_POINT('Ctrl Pts',(35.2184605265174,-13.5414149887607,
78.4476361863756));
#132716=CARTESIAN_POINT('Ctrl Pts',(35.3230564896596,-13.5072433877898,
78.5086867494384));
#132717=CARTESIAN_POINT('Ctrl Pts',(35.4130828699557,-13.4740390254729,
78.5688811234007));
#132718=CARTESIAN_POINT('Ctrl Pts',(35.4899484910174,-13.4422810794632,
78.6270120644502));
#132719=CARTESIAN_POINT('Ctrl Pts',(35.5548824783634,-13.412407270912,78.6820491833158));
#132720=CARTESIAN_POINT('Ctrl Pts',(35.609139363501,-13.3847427053007,78.7332420479501));
#132721=CARTESIAN_POINT('Ctrl Pts',(35.6540406849326,-13.3594694892852,
78.7801592442625));
#132722=CARTESIAN_POINT('Ctrl Pts',(35.6906205410342,-13.3367332240462,
78.8224176266727));
#132723=CARTESIAN_POINT('Ctrl Pts',(35.7198794129803,-13.3166160756286,
78.8598141138234));
#132724=CARTESIAN_POINT('Ctrl Pts',(35.7400793850874,-13.3011802483082,
78.8884757827741));
#132725=CARTESIAN_POINT('Ctrl Pts',(35.7502020927212,-13.2927142033317,
78.9041630984296));
#132726=CARTESIAN_POINT('Ctrl Pts',(35.7536670291066,-13.2897107768893,
78.9097209772309));
#132727=CARTESIAN_POINT('',(35.5596734607929,-13.4095846150427,78.6873016513911));
#132728=CARTESIAN_POINT('Ctrl Pts',(33.8182597453945,-13.731730151521,78.2281566277179));
#132729=CARTESIAN_POINT('Ctrl Pts',(33.8560618757607,-13.7317293665389,
78.221492864037));
#132730=CARTESIAN_POINT('Ctrl Pts',(33.8940274438895,-13.7313259452154,
78.2158292380679));
#132731=CARTESIAN_POINT('Ctrl Pts',(33.9320951477329,-13.7305213553383,
78.2111736280892));
#132732=CARTESIAN_POINT('Ctrl Pts',(34.0169064520391,-13.7287288039099,
78.2008013619744));
#132733=CARTESIAN_POINT('Ctrl Pts',(34.1022250961173,-13.7249450244162,
78.195432386092));
#132734=CARTESIAN_POINT('Ctrl Pts',(34.1873481686048,-13.7192029136075,
78.1950277686168));
#132735=CARTESIAN_POINT('Ctrl Pts',(34.2643490590768,-13.7140086973683,
78.1946617584977));
#132736=CARTESIAN_POINT('Ctrl Pts',(34.3411899190785,-13.7072120363153,
78.1983579365909));
#132737=CARTESIAN_POINT('Ctrl Pts',(34.417325725842,-13.6988484278996,78.206007871343));
#132738=CARTESIAN_POINT('Ctrl Pts',(34.4863484062467,-13.6912662048267,
78.2129430970136));
#132739=CARTESIAN_POINT('Ctrl Pts',(34.5547916210708,-13.6823961470003,
78.2231278161601));
#132740=CARTESIAN_POINT('Ctrl Pts',(34.6222345488869,-13.6722763786065,
78.2364239788855));
#132741=CARTESIAN_POINT('Ctrl Pts',(34.6834691079089,-13.6630881719989,
78.2484961810799));
#132742=CARTESIAN_POINT('Ctrl Pts',(34.7438790637868,-13.6528697458096,
78.2631333532651));
#132743=CARTESIAN_POINT('Ctrl Pts',(34.8031364780348,-13.6416615624858,
78.280190220379));
#132744=CARTESIAN_POINT('Ctrl Pts',(34.8570759116934,-13.6314592431896,
78.2957163408449));
#132745=CARTESIAN_POINT('Ctrl Pts',(34.9100603879659,-13.6204368442871,
78.3132473394726));
#132746=CARTESIAN_POINT('Ctrl Pts',(34.9618313520066,-13.6086372852596,
78.3326405258081));
#132747=CARTESIAN_POINT('Ctrl Pts',(35.0090686726923,-13.597871027299,78.3503354283277));
#132748=CARTESIAN_POINT('Ctrl Pts',(35.0552957124219,-13.586457763026,78.3695806512548));
#132749=CARTESIAN_POINT('Ctrl Pts',(35.1003030116186,-13.5744433217375,
78.3902385394434));
#132750=CARTESIAN_POINT('Ctrl Pts',(35.1414645456183,-13.5634554854884,
78.4091312608957));
#132751=CARTESIAN_POINT('Ctrl Pts',(35.1816058811802,-13.5519648211087,
78.429205544208));
#132752=CARTESIAN_POINT('Ctrl Pts',(35.2205439385965,-13.5400208429106,
78.4503268176181));
#132753=CARTESIAN_POINT('Ctrl Pts',(35.2562938277347,-13.52905481315,78.4697187244818));
#132754=CARTESIAN_POINT('Ctrl Pts',(35.2910294158456,-13.5177066633672,
78.4899931896598));
#132755=CARTESIAN_POINT('Ctrl Pts',(35.3245957725461,-13.5060284012021,
78.5110211295801));
#132756=CARTESIAN_POINT('Ctrl Pts',(35.3555447859984,-13.4952607538203,
78.5304094117601));
#132757=CARTESIAN_POINT('Ctrl Pts',(35.3854998010571,-13.484212468085,78.550438245226));
#132758=CARTESIAN_POINT('Ctrl Pts',(35.4143262731496,-13.4729390883247,
78.5709802880509));
#132759=CARTESIAN_POINT('Ctrl Pts',(35.4408701611854,-13.4625583754445,
78.5898957378159));
#132760=CARTESIAN_POINT('Ctrl Pts',(35.4664571544482,-13.4519868047037,
78.609246339248));
#132761=CARTESIAN_POINT('Ctrl Pts',(35.490971220126,-13.4412831820079,78.628905712652));
#132762=CARTESIAN_POINT('Ctrl Pts',(35.5134775053156,-13.4314562202905,
78.6469549204128));
#132763=CARTESIAN_POINT('Ctrl Pts',(35.5350794179883,-13.4215179517519,
78.6652643926028));
#132764=CARTESIAN_POINT('Ctrl Pts',(35.5556775566379,-13.4115300417887,
78.6837080606934));
#132765=CARTESIAN_POINT('Ctrl Pts',(35.5570141769009,-13.4108819228946,
78.6849048766248));
#132766=CARTESIAN_POINT('Ctrl Pts',(35.5583465680834,-13.4102335959948,
78.6861022557473));
#132767=CARTESIAN_POINT('Ctrl Pts',(35.5596745636201,-13.4095851513792,
78.687300028573));
#132768=CARTESIAN_POINT('Ctrl Pts',(33.8591397922934,-12.9236390706349,
78.4607429230119));
#132769=CARTESIAN_POINT('Ctrl Pts',(33.908472676192,-12.9380113427995,78.4520416150425));
#132770=CARTESIAN_POINT('Ctrl Pts',(33.9580236612373,-12.9521633117262,
78.4451171978411));
#132771=CARTESIAN_POINT('Ctrl Pts',(34.007638426583,-12.9661715905133,78.4398814384144));
#132772=CARTESIAN_POINT('Ctrl Pts',(34.0578196552616,-12.9803398050822,
78.4345859011027));
#132773=CARTESIAN_POINT('Ctrl Pts',(34.1080659159905,-12.9943612810097,
78.4310169990531));
#132774=CARTESIAN_POINT('Ctrl Pts',(34.1582623969643,-13.0082990936994,
78.4290584575211));
#132775=CARTESIAN_POINT('Ctrl Pts',(34.2095192959217,-13.0225313474922,
78.4270585411233));
#132776=CARTESIAN_POINT('Ctrl Pts',(34.2607242534686,-13.0366766097167,
78.4267369299929));
#132777=CARTESIAN_POINT('Ctrl Pts',(34.311803574672,-13.0507813956557,78.4279563167816));
#132778=CARTESIAN_POINT('Ctrl Pts',(34.333416528815,-13.0567494877233,78.4284722702071));
#132779=CARTESIAN_POINT('Ctrl Pts',(34.3550075773263,-13.0627100626087,
78.4292640252931));
#132780=CARTESIAN_POINT('Ctrl Pts',(34.3765736336232,-13.068665420362,78.4303210013202));
#132781=CARTESIAN_POINT('Ctrl Pts',(34.42801194318,-13.0828698502967,78.4328420491804));
#132782=CARTESIAN_POINT('Ctrl Pts',(34.4792917621374,-13.0970587752727,
78.4368698844851));
#132783=CARTESIAN_POINT('Ctrl Pts',(34.5303722969248,-13.1112753418308,
78.4422469157871));
#132784=CARTESIAN_POINT('Ctrl Pts',(34.564595068784,-13.1208001112164,78.445849401867));
#132785=CARTESIAN_POINT('Ctrl Pts',(34.5987293951249,-13.130336803972,78.4500572985107));
#132786=CARTESIAN_POINT('Ctrl Pts',(34.6327744137633,-13.1398920509902,
78.4548228733457));
#132787=CARTESIAN_POINT('Ctrl Pts',(34.6752045342199,-13.151800703069,78.4607621831884));
#132788=CARTESIAN_POINT('Ctrl Pts',(34.7174946114257,-13.1637388489874,
78.4675673950512));
#132789=CARTESIAN_POINT('Ctrl Pts',(34.7596551910158,-13.1757108017934,
78.4751458445683));
#132790=CARTESIAN_POINT('Ctrl Pts',(34.7807354808108,-13.1816967781963,
78.4789350693268));
#132791=CARTESIAN_POINT('Ctrl Pts',(34.8017834698038,-13.1876912266013,
78.4829175192826));
#132792=CARTESIAN_POINT('Ctrl Pts',(34.822802247122,-13.1936930008152,78.4870820527824));
#132793=CARTESIAN_POINT('Ctrl Pts',(34.8333116357811,-13.1966938879222,
78.4891643195323));
#132794=CARTESIAN_POINT('Ctrl Pts',(34.8438137228632,-13.1996966050832,
78.4912921044355));
#132795=CARTESIAN_POINT('Ctrl Pts',(34.8543090003529,-13.2027008853781,
78.493464063845));
#132796=CARTESIAN_POINT('Ctrl Pts',(34.8595566390978,-13.2042030255256,
78.4945500435497));
#132797=CARTESIAN_POINT('Ctrl Pts',(34.8648025755231,-13.2057055563589,
78.4956470670043));
#132798=CARTESIAN_POINT('Ctrl Pts',(34.87004683806,-13.2072084783804,78.4967549450849));
#132799=CARTESIAN_POINT('Ctrl Pts',(34.8741979733,-13.2083981275488,78.4976318942669));
#132800=CARTESIAN_POINT('Ctrl Pts',(34.8792571988079,-13.2098505351454,
78.4987096806394));
#132801=CARTESIAN_POINT('Ctrl Pts',(34.8830654949073,-13.2109417802667,
78.4995279518091));
#132802=CARTESIAN_POINT('Ctrl Pts',(34.884068341642,-13.211229140172,78.4997434289015));
#132803=CARTESIAN_POINT('Ctrl Pts',(34.8849845050134,-13.2114916755989,
78.4999406967177));
#132804=CARTESIAN_POINT('Ctrl Pts',(34.8857746690469,-13.2117183788852,
78.5001109749738));
#132805=CARTESIAN_POINT('Ctrl Pts',(34.9100945387471,-13.2186959103221,
78.5053518424715));
#132806=CARTESIAN_POINT('Ctrl Pts',(34.9342189656613,-13.2256313637476,
78.5107893280521));
#132807=CARTESIAN_POINT('Ctrl Pts',(34.9581484132018,-13.2325305233415,
78.5163921257357));
#132808=CARTESIAN_POINT('Ctrl Pts',(35.0048895547385,-13.2460065801755,
78.5273360123043));
#132809=CARTESIAN_POINT('Ctrl Pts',(35.0508840015399,-13.2593453448709,
78.5389095306765));
#132810=CARTESIAN_POINT('Ctrl Pts',(35.0961507179162,-13.2725609978667,
78.5508925589417));
#132811=CARTESIAN_POINT('Ctrl Pts',(35.1425714629307,-13.2861135704195,
78.563181082257));
#132812=CARTESIAN_POINT('Ctrl Pts',(35.1882273720385,-13.2995368995391,
78.57589963341));
#132813=CARTESIAN_POINT('Ctrl Pts',(35.233184133054,-13.3128242107358,78.5888332034734));
#132814=CARTESIAN_POINT('Ctrl Pts',(35.2787909991607,-13.3263036654158,
78.6019538016847));
#132815=CARTESIAN_POINT('Ctrl Pts',(35.3236790285745,-13.3396432619918,
78.6152952466246));
#132816=CARTESIAN_POINT('Ctrl Pts',(35.3679537683612,-13.3528108903353,
78.628663951463));
#132817=CARTESIAN_POINT('Ctrl Pts',(35.4131923761518,-13.3662651800055,
78.6423236950948));
#132818=CARTESIAN_POINT('Ctrl Pts',(35.4577914138216,-13.3795400306877,
78.6560115792164));
#132819=CARTESIAN_POINT('Ctrl Pts',(35.5018911194648,-13.3925735054304,
78.6695589811007));
#132820=CARTESIAN_POINT('Ctrl Pts',(35.5212430944352,-13.3982928968259,
78.6755038956609));
#132821=CARTESIAN_POINT('Ctrl Pts',(35.5404992028223,-13.4039654452126,
78.6814222703796));
#132822=CARTESIAN_POINT('Ctrl Pts',(35.5596723868115,-13.4095842301505,
78.6873022747948));
#132823=CARTESIAN_POINT('Ctrl Pts',(65.1557612162105,6.92938600905312,68.809717168058));
#132824=CARTESIAN_POINT('Ctrl Pts',(65.1557223413134,6.92884377002472,68.80949676108));
#132825=CARTESIAN_POINT('Ctrl Pts',(65.1547571448173,6.91548128803838,68.8040243621952));
#132826=CARTESIAN_POINT('Ctrl Pts',(65.1532329741082,6.89796927816452,68.7953802655176));
#132827=CARTESIAN_POINT('Ctrl Pts',(65.1516150584316,6.8802663389542,68.7862046028055));
#132828=CARTESIAN_POINT('Ctrl Pts',(65.1510483078126,6.87421650353521,68.7829904020141));
#132829=CARTESIAN_POINT('Ctrl Pts',(65.149557281728,6.94310530121973,68.7748362751515));
#132830=CARTESIAN_POINT('Ctrl Pts',(65.1495311999736,6.94271782251477,68.7746863566555));
#132831=CARTESIAN_POINT('Ctrl Pts',(65.1488690708498,6.93302369305127,68.7708838930986));
#132832=CARTESIAN_POINT('Ctrl Pts',(65.1473099992198,6.91515192374951,68.7620449531505));
#132833=CARTESIAN_POINT('Ctrl Pts',(65.1457440350422,6.8980165865314,68.7531641480283));
#132834=CARTESIAN_POINT('Ctrl Pts',(65.1452003608014,6.89221246259175,68.7500807649487));
#132835=CARTESIAN_POINT('Ctrl Pts',(65.1454741812578,6.95683738476643,68.7395472040424));
#132836=CARTESIAN_POINT('Ctrl Pts',(65.1454609074645,6.95660481341836,68.7394678612072));
#132837=CARTESIAN_POINT('Ctrl Pts',(65.1451021969836,6.9505825218207,68.7373374000129));
#132838=CARTESIAN_POINT('Ctrl Pts',(65.143508191757,6.93235065627285,68.7283034343758));
#132839=CARTESIAN_POINT('Ctrl Pts',(65.1419942277171,6.91578345245396,68.7197177628987));
#132840=CARTESIAN_POINT('Ctrl Pts',(65.1414736514594,6.91022527003653,68.7167653200066));
#132841=CARTESIAN_POINT('Ctrl Pts',(65.1435571535124,6.97053667058868,68.7039615141308));
#132842=CARTESIAN_POINT('Ctrl Pts',(65.1435566600202,6.97045863939525,68.7039526001507));
#132843=CARTESIAN_POINT('Ctrl Pts',(65.1435007131574,6.96809948185238,68.7034906650766));
#132844=CARTESIAN_POINT('Ctrl Pts',(65.1418718576327,6.949508378702,68.6942621387861));
#132845=CARTESIAN_POINT('Ctrl Pts',(65.1404097697371,6.93350795357761,68.6859708972127));
#132846=CARTESIAN_POINT('Ctrl Pts',(65.1399122363857,6.9281951262389,68.6831490822834));
#132847=CARTESIAN_POINT('',(65.150886598664,6.87471515335625,68.7820772040975));
#132848=CARTESIAN_POINT('',(65.1445501446421,6.89804540344547,68.7391944229629));
#132849=CARTESIAN_POINT('Origin',(66.1356794036644,6.87480345545517,68.6083476476019));
#132850=CARTESIAN_POINT('',(65.1554607867035,6.92820316509666,68.8079865227404));
#132851=CARTESIAN_POINT('Ctrl Pts',(65.1554552753629,6.92820316432873,68.8079874964246));
#132852=CARTESIAN_POINT('Ctrl Pts',(65.1551868768224,6.92440994225428,68.8064652897237));
#132853=CARTESIAN_POINT('Ctrl Pts',(65.1548906041493,6.92041985602695,68.8047850232824));
#132854=CARTESIAN_POINT('Ctrl Pts',(65.1545659556445,6.91628081087331,68.8029438300205));
#132855=CARTESIAN_POINT('Ctrl Pts',(65.1542481880873,6.91222949306833,68.8011416609773));
#132856=CARTESIAN_POINT('Ctrl Pts',(65.1539032520095,6.90803584356044,68.799185408462));
#132857=CARTESIAN_POINT('Ctrl Pts',(65.1535310020591,6.90369367510328,68.7970742510979));
#132858=CARTESIAN_POINT('Ctrl Pts',(65.1532244215364,6.90011751807833,68.7953355276207));
#132859=CARTESIAN_POINT('Ctrl Pts',(65.1528993120918,6.89643948335413,68.7934917232776));
#132860=CARTESIAN_POINT('Ctrl Pts',(65.1525557304649,6.89262942801718,68.7915431797103));
#132861=CARTESIAN_POINT('Ctrl Pts',(65.1520411631357,6.88692327307375,68.7886249303608));
#132862=CARTESIAN_POINT('Ctrl Pts',(65.1514851293121,6.88091493848609,68.7854715795498));
#132863=CARTESIAN_POINT('Ctrl Pts',(65.1508866467258,6.87471566536353,68.7820774766692));
#132864=CARTESIAN_POINT('Ctrl Pts',(65.1554552752064,6.92820316476403,68.8079874955378));
#132865=CARTESIAN_POINT('Ctrl Pts',(65.1550749035392,6.92721170906623,68.8058321165897));
#132866=CARTESIAN_POINT('Ctrl Pts',(65.1546285636395,6.92601568182351,68.803279705676));
#132867=CARTESIAN_POINT('Ctrl Pts',(65.1541213470041,6.9246723299939,68.8003307695755));
#132868=CARTESIAN_POINT('Ctrl Pts',(65.1536487850895,6.92342076041135,68.7975833145582));
#132869=CARTESIAN_POINT('Ctrl Pts',(65.1531233821133,6.92204216782181,68.7944915961647));
#132870=CARTESIAN_POINT('Ctrl Pts',(65.1525462541141,6.92053247120318,68.7910330627761));
#132871=CARTESIAN_POINT('Ctrl Pts',(65.1519056417045,6.91885670709223,68.7871940887348));
#132872=CARTESIAN_POINT('Ctrl Pts',(65.1512008572797,6.91701668953906,68.7829008645889));
#132873=CARTESIAN_POINT('Ctrl Pts',(65.1504321489964,6.91494662720502,68.7781066343339));
#132874=CARTESIAN_POINT('Ctrl Pts',(65.1499261574398,6.91358403740928,68.7749508988198));
#132875=CARTESIAN_POINT('Ctrl Pts',(65.1493923353321,6.9121192319998,68.7715771586181));
#132876=CARTESIAN_POINT('Ctrl Pts',(65.1488334069601,6.91054665220031,68.7679845589492));
#132877=CARTESIAN_POINT('Ctrl Pts',(65.1485432048206,6.9097301503992,68.7661192392362));
#132878=CARTESIAN_POINT('Ctrl Pts',(65.1482462915086,6.90888499198604,68.7641952058584));
#132879=CARTESIAN_POINT('Ctrl Pts',(65.1479436555084,6.90801551870994,68.7622155123594));
#132880=CARTESIAN_POINT('Ctrl Pts',(65.1468755595425,6.90494687883227,68.7552285622329));
#132881=CARTESIAN_POINT('Ctrl Pts',(65.1457368023009,6.90157963766923,68.7475533689889));
#132882=CARTESIAN_POINT('Ctrl Pts',(65.1445498748409,6.89804540979059,68.7391944585906));
#132883=CARTESIAN_POINT('Ctrl Pts',(65.1399122363857,6.9281951262389,68.6831490822834));
#132884=CARTESIAN_POINT('Ctrl Pts',(65.1393493185638,6.92218410168036,68.6799564321636));
#132885=CARTESIAN_POINT('Ctrl Pts',(65.1376171252306,6.90420410579108,68.6701305745004));
#132886=CARTESIAN_POINT('Ctrl Pts',(65.1342088860127,6.87246916263756,68.6508029263816));
#132887=CARTESIAN_POINT('Ctrl Pts',(65.1292353292282,6.83210489462999,68.6225959678029));
#132888=CARTESIAN_POINT('Ctrl Pts',(65.1240218446123,6.79503133510698,68.593028962644));
#132889=CARTESIAN_POINT('Ctrl Pts',(65.1203934945133,6.77172179746152,68.5724515663476));
#132890=CARTESIAN_POINT('Ctrl Pts',(65.1189319128645,6.76267723202094,68.5641625212446));
#132891=CARTESIAN_POINT('Ctrl Pts',(65.1389667820184,6.93907607603473,68.6627940727123));
#132892=CARTESIAN_POINT('Ctrl Pts',(65.1384196505658,6.93323314077171,68.6596909139631));
#132893=CARTESIAN_POINT('Ctrl Pts',(65.1367488206894,6.91589489164434,68.650212637829));
#132894=CARTESIAN_POINT('Ctrl Pts',(65.1334525332493,6.88519445031666,68.6315201924649));
#132895=CARTESIAN_POINT('Ctrl Pts',(65.128626463115,6.84602415585857,68.6041495670674));
#132896=CARTESIAN_POINT('Ctrl Pts',(65.1235483963183,6.80990900854383,68.5753505820931));
#132897=CARTESIAN_POINT('Ctrl Pts',(65.1200060341081,6.7871513123966,68.5552608472742));
#132898=CARTESIAN_POINT('Ctrl Pts',(65.118578006522,6.77831439876664,68.5471620959691));
#132899=CARTESIAN_POINT('Ctrl Pts',(65.1388177654475,6.94991825968818,68.6423717434951));
#132900=CARTESIAN_POINT('Ctrl Pts',(65.1382863641213,6.94424281485995,68.6393577572805));
#132901=CARTESIAN_POINT('Ctrl Pts',(65.1366766790788,6.92754402610895,68.6302258243284));
#132902=CARTESIAN_POINT('Ctrl Pts',(65.1334919445599,6.89787440093207,68.6121663186481));
#132903=CARTESIAN_POINT('Ctrl Pts',(65.1288128356172,6.85989382618996,68.5856290467829));
#132904=CARTESIAN_POINT('Ctrl Pts',(65.1238697041796,6.82473367649701,68.5575953457266));
#132905=CARTESIAN_POINT('Ctrl Pts',(65.1204130235043,6.80252585577276,68.5379915349674));
#132906=CARTESIAN_POINT('Ctrl Pts',(65.1190184304362,6.7938958541412,68.5300823994905));
#132907=CARTESIAN_POINT('Ctrl Pts',(65.1394699820383,6.96070828693927,68.6219065034142));
#132908=CARTESIAN_POINT('Ctrl Pts',(65.1389542351686,6.9551995268319,68.6189812607692));
#132909=CARTESIAN_POINT('Ctrl Pts',(65.1374054008223,6.93913712232853,68.6101940049127));
#132910=CARTESIAN_POINT('Ctrl Pts',(65.1343316825986,6.91049335455396,68.5927643941554));
#132911=CARTESIAN_POINT('Ctrl Pts',(65.1297988278895,6.8736967763726,68.5670564669691));
#132912=CARTESIAN_POINT('Ctrl Pts',(65.1249899827035,6.83948703027851,68.5397843684272));
#132913=CARTESIAN_POINT('Ctrl Pts',(65.1216185713916,6.81782643979757,68.5206641441865));
#132914=CARTESIAN_POINT('Ctrl Pts',(65.1202572520044,6.80940235481273,68.5129437123894));
#132915=CARTESIAN_POINT('',(65.1322122844213,6.85640303813197,68.6394073971386));
#132916=CARTESIAN_POINT('',(65.1189319128645,6.76267723202094,68.5641625212446));
#132917=CARTESIAN_POINT('Origin',(65.0612614902037,6.85286176575256,68.2371121691863));
#132918=CARTESIAN_POINT('',(65.1202119716011,6.80865446689099,68.5137529809028));
#132919=CARTESIAN_POINT('Ctrl Pts',(65.1322122597858,6.85640293841445,68.6394071751272));
#132920=CARTESIAN_POINT('Ctrl Pts',(65.1290955654378,6.84478572588336,68.6108421213684));
#132921=CARTESIAN_POINT('Ctrl Pts',(65.1265159645158,6.83473800066337,68.5838575775351));
#132922=CARTESIAN_POINT('Ctrl Pts',(65.1239761302869,6.82439218292853,68.5563457900104));
#132923=CARTESIAN_POINT('Ctrl Pts',(65.1232138928177,6.82125728420136,68.5479861954865));
#132924=CARTESIAN_POINT('Ctrl Pts',(65.1224504009973,6.81808207925492,68.5394643466061));
#132925=CARTESIAN_POINT('Ctrl Pts',(65.121941009263,6.81595673594787,68.5337465582695));
#132926=CARTESIAN_POINT('Ctrl Pts',(65.1215473922881,6.8143075610625,68.5292949851828));
#132927=CARTESIAN_POINT('Ctrl Pts',(65.1211981470453,6.8128417025367,68.5253313373399));
#132928=CARTESIAN_POINT('Ctrl Pts',(65.1207483588331,6.81094850659989,68.5201917259831));
#132929=CARTESIAN_POINT('Ctrl Pts',(65.1203129737665,6.80911846789646,68.5151650880062));
#132930=CARTESIAN_POINT('Ctrl Pts',(65.1202038189481,6.80866554628641,68.5138751223312));
#132931=CARTESIAN_POINT('Ctrl Pts',(65.1202119716011,6.80865446689099,68.5137529809029));
#132932=CARTESIAN_POINT('Origin',(66.1117715670066,6.68571538702879,68.4727063556212));
#132933=CARTESIAN_POINT('Ctrl Pts',(65.1510483078126,6.87421650353521,68.7829904020141));
#132934=CARTESIAN_POINT('Ctrl Pts',(65.1504070763793,6.86737161531276,68.7793537997567));
#132935=CARTESIAN_POINT('Ctrl Pts',(65.1483704689148,6.84620801808512,68.7678036466433));
#132936=CARTESIAN_POINT('Ctrl Pts',(65.1444068551304,6.80934107958273,68.7453248609419));
#132937=CARTESIAN_POINT('Ctrl Pts',(65.1387016410555,6.76305370293533,68.7129689894385));
#132938=CARTESIAN_POINT('Ctrl Pts',(65.1328163706566,6.72122561628415,68.6795919610231));
#132939=CARTESIAN_POINT('Ctrl Pts',(65.1287614486238,6.6951784826949,68.6565953554305));
#132940=CARTESIAN_POINT('Ctrl Pts',(65.1271334107255,6.68510379038588,68.6473622937371));
#132941=CARTESIAN_POINT('Ctrl Pts',(65.1452003608014,6.89221246259175,68.7500807649487));
#132942=CARTESIAN_POINT('Ctrl Pts',(65.1445852383808,6.88564557657838,68.7465921721086));
#132943=CARTESIAN_POINT('Ctrl Pts',(65.1426501196904,6.86554336173635,68.7356168826869));
#132944=CARTESIAN_POINT('Ctrl Pts',(65.1388716625005,6.83038738163843,68.714188656264));
#132945=CARTESIAN_POINT('Ctrl Pts',(65.1334103760025,6.78607471303712,68.6832159928414));
#132946=CARTESIAN_POINT('Ctrl Pts',(65.1277490725898,6.74583174047826,68.6511091899172));
#132947=CARTESIAN_POINT('Ctrl Pts',(65.1238363655798,6.72069729532103,68.6289191256786));
#132948=CARTESIAN_POINT('Ctrl Pts',(65.1222638226107,6.7109660375055,68.6200007901315));
#132949=CARTESIAN_POINT('Ctrl Pts',(65.1414736514594,6.91022527003653,68.7167653200066));
#132950=CARTESIAN_POINT('Ctrl Pts',(65.1408846624955,6.90393664650673,68.7134248751548));
#132951=CARTESIAN_POINT('Ctrl Pts',(65.1390511275962,6.88489680775021,68.7030249876305));
#132952=CARTESIAN_POINT('Ctrl Pts',(65.1354580003504,6.85145338791034,68.6826483040529));
#132953=CARTESIAN_POINT('Ctrl Pts',(65.1302408698022,6.80911727613949,68.6530601437148));
#132954=CARTESIAN_POINT('Ctrl Pts',(65.1248037430605,6.7704609017071,68.6222247555069));
#132955=CARTESIAN_POINT('Ctrl Pts',(65.1210333842194,6.74623999946976,68.600841987732));
#132956=CARTESIAN_POINT('Ctrl Pts',(65.1195163881358,6.73685249768201,68.5922386729879));
#132957=CARTESIAN_POINT('Ctrl Pts',(65.1399122363857,6.9281951262389,68.6831490822834));
#132958=CARTESIAN_POINT('Ctrl Pts',(65.1393493185638,6.92218410168036,68.6799564321636));
#132959=CARTESIAN_POINT('Ctrl Pts',(65.1376171252306,6.90420410579108,68.6701305745004));
#132960=CARTESIAN_POINT('Ctrl Pts',(65.1342088860127,6.87246916263756,68.6508029263816));
#132961=CARTESIAN_POINT('Ctrl Pts',(65.1292353292282,6.83210489462999,68.6225959678029));
#132962=CARTESIAN_POINT('Ctrl Pts',(65.1240218446123,6.79503133510698,68.593028962644));
#132963=CARTESIAN_POINT('Ctrl Pts',(65.1203934945133,6.77172179746152,68.5724515663476));
#132964=CARTESIAN_POINT('Ctrl Pts',(65.1189319128645,6.76267723202094,68.5641625212446));
#132965=CARTESIAN_POINT('',(65.1269899214714,6.68586921358489,68.6465524467399));
#132966=CARTESIAN_POINT('Ctrl Pts',(65.1508865027656,6.87471412864423,68.78207666023));
#132967=CARTESIAN_POINT('Ctrl Pts',(65.1502491988091,6.86802460506826,68.7784623662399));
#132968=CARTESIAN_POINT('Ctrl Pts',(65.1495817613522,6.86116856242663,68.7746771454042));
#132969=CARTESIAN_POINT('Ctrl Pts',(65.1488754684122,6.85416574004831,68.7706715562182));
#132970=CARTESIAN_POINT('Ctrl Pts',(65.1476733767521,6.8422471239859,68.7638541507448));
#132971=CARTESIAN_POINT('Ctrl Pts',(65.1463585261558,6.82990176790923,68.7563972389876));
#132972=CARTESIAN_POINT('Ctrl Pts',(65.1449099343834,6.81710107376072,68.7481818600873));
#132973=CARTESIAN_POINT('Ctrl Pts',(65.1447034677796,6.81527660126446,68.7470109288335));
#132974=CARTESIAN_POINT('Ctrl Pts',(65.1444942810936,6.8134429638408,68.7458245714453));
#132975=CARTESIAN_POINT('Ctrl Pts',(65.1442823110769,6.81160017130178,68.7446224292225));
#132976=CARTESIAN_POINT('Ctrl Pts',(65.1427531869705,6.79830650582067,68.7359503317226));
#132977=CARTESIAN_POINT('Ctrl Pts',(65.141079473815,6.78453266254534,68.7264582415822));
#132978=CARTESIAN_POINT('Ctrl Pts',(65.1392293302725,6.77023710148806,68.7159655663571));
#132979=CARTESIAN_POINT('Ctrl Pts',(65.1390293137508,6.7686916276736,68.7148312173981));
#132980=CARTESIAN_POINT('Ctrl Pts',(65.1388272326218,6.76714010483981,68.7136851594773));
#132981=CARTESIAN_POINT('Ctrl Pts',(65.1386230449928,6.76558251795905,68.712527154994));
#132982=CARTESIAN_POINT('Ctrl Pts',(65.1367344209749,6.75117569024202,68.7018162461568));
#132983=CARTESIAN_POINT('Ctrl Pts',(65.1346656938585,6.73624601825409,68.690083919913));
#132984=CARTESIAN_POINT('Ctrl Pts',(65.1323813143638,6.72077703545733,68.6771285607866));
#132985=CARTESIAN_POINT('Ctrl Pts',(65.1321721153332,6.71936041610313,68.6759421341986));
#132986=CARTESIAN_POINT('Ctrl Pts',(65.1319611071595,6.71793931029428,68.6747454473994));
#132987=CARTESIAN_POINT('Ctrl Pts',(65.1317482623707,6.71651372845993,68.6735383445911));
#132988=CARTESIAN_POINT('Ctrl Pts',(65.1302559977912,6.70651890881531,68.6650752914219));
#132989=CARTESIAN_POINT('Ctrl Pts',(65.1286734752311,6.69630338628556,68.6561003573301));
#132990=CARTESIAN_POINT('Ctrl Pts',(65.1269899309713,6.68586927237242,68.6465525006164));
#132991=CARTESIAN_POINT('Ctrl Pts',(65.1445506842445,6.89804539075522,68.7391943517073));
#132992=CARTESIAN_POINT('Ctrl Pts',(65.1388995878143,6.88121747909777,68.6994030493852));
#132993=CARTESIAN_POINT('Ctrl Pts',(65.1351670463109,6.86836305827018,68.6660352394652));
#132994=CARTESIAN_POINT('Ctrl Pts',(65.1322122844213,6.85640303813197,68.6394073971386));
#132995=CARTESIAN_POINT('Origin',(66.1117907052193,6.68589932942379,68.4728725765555));
#132996=CARTESIAN_POINT('Ctrl Pts',(65.1346705530482,6.8919798904543,68.4202960166216));
#132997=CARTESIAN_POINT('Ctrl Pts',(65.1338389881117,6.88683406911642,68.4155799705943));
#132998=CARTESIAN_POINT('Ctrl Pts',(65.1307272078985,6.86806865274327,68.3979321456351));
#132999=CARTESIAN_POINT('Ctrl Pts',(65.1247065901473,6.83491377283282,68.3637875588852));
#133000=CARTESIAN_POINT('Ctrl Pts',(65.1159503997162,6.79260266483268,68.3141287229154));
#133001=CARTESIAN_POINT('Ctrl Pts',(65.1056217526553,6.74903116432229,68.2555520583749));
#133002=CARTESIAN_POINT('Ctrl Pts',(65.0935877735642,6.70501820397611,68.187303970419));
#133003=CARTESIAN_POINT('Ctrl Pts',(65.0796903316755,6.66136171514741,68.1084876612219));
#133004=CARTESIAN_POINT('Ctrl Pts',(65.0637304459047,6.61886989600768,68.0179746511137));
#133005=CARTESIAN_POINT('Ctrl Pts',(65.0455161134506,6.57848378907752,67.9146760386274));
#133006=CARTESIAN_POINT('Ctrl Pts',(65.0248965098102,6.54163495336659,67.7977364553764));
#133007=CARTESIAN_POINT('Ctrl Pts',(65.0016762933978,6.5099268953333,67.6660480641928));
#133008=CARTESIAN_POINT('Ctrl Pts',(64.9756853622109,6.48522042825308,67.5186461686814));
#133009=CARTESIAN_POINT('Ctrl Pts',(64.9475375191463,6.46988450894962,67.3590118180421));
#133010=CARTESIAN_POINT('Ctrl Pts',(64.9279729835967,6.46669330688071,67.248055823275));
#133011=CARTESIAN_POINT('Ctrl Pts',(64.9181216456064,6.4668870503417,67.1921861092301));
#133012=CARTESIAN_POINT('Ctrl Pts',(65.1539262221606,6.9627202545652,68.3397108632764));
#133013=CARTESIAN_POINT('Ctrl Pts',(65.1532012561442,6.95823412856528,68.3355993673901));
#133014=CARTESIAN_POINT('Ctrl Pts',(65.1504777508534,6.94180854698276,68.320153544379));
#133015=CARTESIAN_POINT('Ctrl Pts',(65.1451443581134,6.91242436785244,68.2899064157574));
#133016=CARTESIAN_POINT('Ctrl Pts',(65.1372940192507,6.87447666454151,68.245384915083));
#133017=CARTESIAN_POINT('Ctrl Pts',(65.1279288955758,6.83495486124124,68.1922726644923));
#133018=CARTESIAN_POINT('Ctrl Pts',(65.116907777658,6.79463263891094,68.1297687973011));
#133019=CARTESIAN_POINT('Ctrl Pts',(65.1040642329972,6.75427238436194,68.0569294364098));
#133020=CARTESIAN_POINT('Ctrl Pts',(65.0891844235482,6.7146422157174,67.9725418434751));
#133021=CARTESIAN_POINT('Ctrl Pts',(65.0720761044474,6.67669704588737,67.8755157444185));
#133022=CARTESIAN_POINT('Ctrl Pts',(65.0526198386,6.64191840341569,67.7651737776444));
#133023=CARTESIAN_POINT('Ctrl Pts',(65.0306058055575,6.61184718228901,67.6403259922737));
#133024=CARTESIAN_POINT('Ctrl Pts',(65.0058555336308,6.58830632030332,67.4999602250676));
#133025=CARTESIAN_POINT('Ctrl Pts',(64.9789014271637,6.57360946623491,67.3470958910942));
#133026=CARTESIAN_POINT('Ctrl Pts',(64.9601115765747,6.57054055281461,67.2405333530598));
#133027=CARTESIAN_POINT('Ctrl Pts',(64.9506397889729,6.570726798958,67.1868161762322));
#133028=CARTESIAN_POINT('Ctrl Pts',(65.1900881115087,7.02858813577264,68.2614614009606));
#133029=CARTESIAN_POINT('Ctrl Pts',(65.1894624020497,7.02471626635308,68.2579128147706));
#133030=CARTESIAN_POINT('Ctrl Pts',(65.1871004279267,7.01046935549091,68.2445173233425));
#133031=CARTESIAN_POINT('Ctrl Pts',(65.1824069252406,6.98459615731431,68.2178992021798));
#133032=CARTESIAN_POINT('Ctrl Pts',(65.175400044342,6.9507113143709,68.1781611853795));
#133033=CARTESIAN_POINT('Ctrl Pts',(65.1669320781066,6.9149602716274,68.1301369686635));
#133034=CARTESIAN_POINT('Ctrl Pts',(65.1568540571083,6.87807457519367,68.0729816695171));
#133035=CARTESIAN_POINT('Ctrl Pts',(65.1449918189232,6.84078351559007,68.0057075743117));
#133036=CARTESIAN_POINT('Ctrl Pts',(65.1311176918693,6.80381789154104,67.9270234896327));
#133037=CARTESIAN_POINT('Ctrl Pts',(65.1150392056949,6.7681455309758,67.8358378633339));
#133038=CARTESIAN_POINT('Ctrl Pts',(65.096666148798,6.73529449015099,67.7316390797878));
#133039=CARTESIAN_POINT('Ctrl Pts',(65.0757752191479,6.70674736322814,67.6131607302648));
#133040=CARTESIAN_POINT('Ctrl Pts',(65.0521801518604,6.68429182132624,67.4793464541235));
#133041=CARTESIAN_POINT('Ctrl Pts',(65.0263375593267,6.67019001470368,67.3327858289185));
#133042=CARTESIAN_POINT('Ctrl Pts',(65.0082690346399,6.6672349668859,67.2303141333585));
#133043=CARTESIAN_POINT('Ctrl Pts',(64.9991506546043,6.66741423211489,67.1786012304346));
#133044=CARTESIAN_POINT('Ctrl Pts',(65.2417928776143,7.08799141016858,68.1875253039243));
#133045=CARTESIAN_POINT('Ctrl Pts',(65.2412566831725,7.08467351108365,68.1844843806276));
#133046=CARTESIAN_POINT('Ctrl Pts',(65.2392207577211,7.07239144518454,68.1729379908769));
#133047=CARTESIAN_POINT('Ctrl Pts',(65.2351043430444,7.04968464254353,68.149592708037));
#133048=CARTESIAN_POINT('Ctrl Pts',(65.2288581388817,7.0194639103142,68.1141686998238));
#133049=CARTESIAN_POINT('Ctrl Pts',(65.2211992785201,6.98711354662591,68.0707331516192));
#133050=CARTESIAN_POINT('Ctrl Pts',(65.2119717941427,6.95332709806631,68.0184014850135));
#133051=CARTESIAN_POINT('Ctrl Pts',(65.2009945520552,6.91880400710191,67.9561464521882));
#133052=CARTESIAN_POINT('Ctrl Pts',(65.1880274046423,6.88424141577304,67.8826061046348));
#133053=CARTESIAN_POINT('Ctrl Pts',(65.1728776783849,6.85061879948269,67.7966877375746));
#133054=CARTESIAN_POINT('Ctrl Pts',(65.155481518837,6.81950617573553,67.698029214202));
#133055=CARTESIAN_POINT('Ctrl Pts',(65.1356034655349,6.79233356070731,67.5852951718964));
#133056=CARTESIAN_POINT('Ctrl Pts',(65.1130502252646,6.77085682009007,67.4573893903701));
#133057=CARTESIAN_POINT('Ctrl Pts',(65.0882100570683,6.75729165994912,67.316513796091));
#133058=CARTESIAN_POINT('Ctrl Pts',(65.0707920637135,6.75443930238809,67.2177314470463));
#133059=CARTESIAN_POINT('Ctrl Pts',(65.061992406039,6.75461227184489,67.1678261084541));
#133060=CARTESIAN_POINT('',(65.0995369296605,6.72719442421048,68.2212878397353));
#133061=CARTESIAN_POINT('',(64.9199577054575,6.46687174464771,67.202598919663));
#133062=CARTESIAN_POINT('Ctrl Pts',(65.0995791195013,6.72720037365666,68.2212825822045));
#133063=CARTESIAN_POINT('Ctrl Pts',(65.0976822698379,6.72028556494202,68.2105250131428));
#133064=CARTESIAN_POINT('Ctrl Pts',(65.0957558389128,6.71350272843201,68.1995996803412));
#133065=CARTESIAN_POINT('Ctrl Pts',(65.0938019734153,6.70685605161901,68.1885187583979));
#133066=CARTESIAN_POINT('Ctrl Pts',(65.0893294910235,6.69164152173065,68.1631540501626));
#133067=CARTESIAN_POINT('Ctrl Pts',(65.0847132023982,6.67714022326058,68.1369737765162));
#133068=CARTESIAN_POINT('Ctrl Pts',(65.0799737924691,6.66336991240936,68.1100952471924));
#133069=CARTESIAN_POINT('Ctrl Pts',(65.0748169564677,6.64838677404176,68.0808493769774));
#133070=CARTESIAN_POINT('Ctrl Pts',(65.0695143561238,6.63426905803681,68.0507768360194));
#133071=CARTESIAN_POINT('Ctrl Pts',(65.0640933132977,6.62101769306386,68.0200325743827));
#133072=CARTESIAN_POINT('Ctrl Pts',(65.0581802097322,6.60656351958042,67.986497697619));
#133073=CARTESIAN_POINT('Ctrl Pts',(65.0521261861146,6.59314010997735,67.9521636235467));
#133074=CARTESIAN_POINT('Ctrl Pts',(65.0459645287121,6.58076937331775,67.9172191279448));
#133075=CARTESIAN_POINT('Ctrl Pts',(65.0392369363317,6.56726241110686,67.8790650555916));
#133076=CARTESIAN_POINT('Ctrl Pts',(65.0323810303017,6.55501037370809,67.8401832803673));
#133077=CARTESIAN_POINT('Ctrl Pts',(65.0254209754051,6.54399779743841,67.80071084757));
#133078=CARTESIAN_POINT('Ctrl Pts',(65.0178227566917,6.53197548377289,67.75761920792));
#133079=CARTESIAN_POINT('Ctrl Pts',(65.0101004148254,6.52143034243136,67.71382363089));
#133080=CARTESIAN_POINT('Ctrl Pts',(65.0022830167957,6.5123274224688,67.6694889635685));
#133081=CARTESIAN_POINT('Ctrl Pts',(64.9937552008312,6.50239726081085,67.6211253159296));
#133082=CARTESIAN_POINT('Ctrl Pts',(64.9851142669312,6.49418335930004,67.5721201445991));
#133083=CARTESIAN_POINT('Ctrl Pts',(64.9763867994217,6.48759887860092,67.522624216781));
#133084=CARTESIAN_POINT('Ctrl Pts',(64.9668634700515,6.48041395601466,67.468614732061));
#133085=CARTESIAN_POINT('Ctrl Pts',(64.9572371054031,6.47516917931563,67.4140209052397));
#133086=CARTESIAN_POINT('Ctrl Pts',(64.9475515457086,6.4717450887343,67.3590913666322));
#133087=CARTESIAN_POINT('Ctrl Pts',(64.9383987364529,6.46850933892178,67.3071832059018));
#133088=CARTESIAN_POINT('Ctrl Pts',(64.9291930728841,6.46689949148789,67.2549752934684));
#133089=CARTESIAN_POINT('Ctrl Pts',(64.9199577054575,6.4668717446477,67.202598919663));
#133090=CARTESIAN_POINT('',(65.0614282834239,6.75162228554997,67.1773189309182));
#133091=CARTESIAN_POINT('Ctrl Pts',(65.0995369296605,6.72719442421049,68.2212878397353));
#133092=CARTESIAN_POINT('Ctrl Pts',(65.0995675555563,6.72716010371951,68.221136173046));
#133093=CARTESIAN_POINT('Ctrl Pts',(65.0994719063417,6.72683619259612,68.2195356587124));
#133094=CARTESIAN_POINT('Ctrl Pts',(65.0991078651206,6.72561893193096,68.2132807572063));
#133095=CARTESIAN_POINT('Ctrl Pts',(65.0989280671564,6.72501418471105,68.210209911432));
#133096=CARTESIAN_POINT('Ctrl Pts',(65.0980260005293,6.72207473766137,68.1940983041802));
#133097=CARTESIAN_POINT('Ctrl Pts',(65.097360711155,6.71994808440332,68.1821554868447));
#133098=CARTESIAN_POINT('Ctrl Pts',(65.0967081062033,6.71792384189042,68.1704251071661));
#133099=CARTESIAN_POINT('Ctrl Pts',(65.0962753846899,6.71659547529839,68.1626520285289));
#133100=CARTESIAN_POINT('Ctrl Pts',(65.0959604444661,6.71564207815097,68.1570014255529));
#133101=CARTESIAN_POINT('Ctrl Pts',(65.0953880058314,6.71392179538477,68.1467429225592));
#133102=CARTESIAN_POINT('Ctrl Pts',(65.0945397680694,6.71136873889932,68.1324085686363));
#133103=CARTESIAN_POINT('Ctrl Pts',(65.0927881222842,6.70655433500724,68.1015604372104));
#133104=CARTESIAN_POINT('Ctrl Pts',(65.0921252586568,6.70479202834819,68.089718680223));
#133105=CARTESIAN_POINT('Ctrl Pts',(65.0910345580279,6.70206233773065,68.0695921665363));
#133106=CARTESIAN_POINT('Ctrl Pts',(65.0904652080591,6.70067637610273,68.0589379489014));
#133107=CARTESIAN_POINT('Ctrl Pts',(65.0898649673399,6.69929060171878,68.0473930398002));
#133108=CARTESIAN_POINT('Ctrl Pts',(65.0894585811012,6.69837057395887,68.0394980979976));
#133109=CARTESIAN_POINT('Ctrl Pts',(65.0891647052933,6.69772220656397,68.0337151425024));
#133110=CARTESIAN_POINT('Ctrl Pts',(65.0870987600182,6.69323358761507,67.9927505910103));
#133111=CARTESIAN_POINT('Ctrl Pts',(65.0852415502832,6.68999131681029,67.9537767255883));
#133112=CARTESIAN_POINT('Ctrl Pts',(65.0825675280683,6.68653839116838,67.8948244268623));
#133113=CARTESIAN_POINT('Ctrl Pts',(65.0816952976188,6.68562456629401,67.8750943663708));
#133114=CARTESIAN_POINT('Ctrl Pts',(65.0799871749233,6.68427009479148,67.8355045982994));
#133115=CARTESIAN_POINT('Ctrl Pts',(65.0792365216954,6.68385037915333,67.8177201330391));
#133116=CARTESIAN_POINT('Ctrl Pts',(65.0710677997279,6.68174643674947,67.6196579069018));
#133117=CARTESIAN_POINT('Ctrl Pts',(65.0645780549624,6.69992461595788,67.411398489151));
#133118=CARTESIAN_POINT('Ctrl Pts',(65.0614400430891,6.75161362534301,67.177316857372));
#133119=CARTESIAN_POINT('Ctrl Pts',(64.9199577054575,6.46687174464771,67.202598919663));
#133120=CARTESIAN_POINT('Ctrl Pts',(64.9333050247472,6.50957649447236,67.2002436743331));
#133121=CARTESIAN_POINT('Ctrl Pts',(64.9494820555029,6.55136533225673,67.1973921465925));
#133122=CARTESIAN_POINT('Ctrl Pts',(64.9683398996363,6.59186707079172,67.1940423684793));
#133123=CARTESIAN_POINT('Ctrl Pts',(64.9867017502843,6.63130354447895,67.1907806952475));
#133124=CARTESIAN_POINT('Ctrl Pts',(65.0076053315602,6.66951971007743,67.1870467099025));
#133125=CARTESIAN_POINT('Ctrl Pts',(65.0308682154119,6.70618765028569,67.1828511423827));
#133126=CARTESIAN_POINT('Ctrl Pts',(65.040651362678,6.72160826027071,67.1810867070198));
#133127=CARTESIAN_POINT('Ctrl Pts',(65.0508512121906,6.73675523607014,67.1792407850699));
#133128=CARTESIAN_POINT('Ctrl Pts',(65.0614516307786,6.75160508908749,67.1773148179911));
#133129=CARTESIAN_POINT('Ctrl Pts',(65.1432217654919,-6.97297506433017,
68.6973703391101));
#133130=CARTESIAN_POINT('Ctrl Pts',(65.1432243503256,-6.9729296867911,68.6973781401607));
#133131=CARTESIAN_POINT('Ctrl Pts',(65.1432367108929,-6.97136627551693,
68.6972928489378));
#133132=CARTESIAN_POINT('Ctrl Pts',(65.141532389107,-6.95194096119578,68.687637522311));
#133133=CARTESIAN_POINT('Ctrl Pts',(65.1400238117738,-6.93547409352959,
68.6790824101809));
#133134=CARTESIAN_POINT('Ctrl Pts',(65.1394727093545,-6.92962631050212,
68.6759566677395));
#133135=CARTESIAN_POINT('Ctrl Pts',(65.1449771131016,-6.95849924894636,
68.7351837598004));
#133136=CARTESIAN_POINT('Ctrl Pts',(65.1449653224239,-6.95827999915231,
68.7351123311065));
#133137=CARTESIAN_POINT('Ctrl Pts',(65.1446513814295,-6.95276757579234,
68.7332285542318));
#133138=CARTESIAN_POINT('Ctrl Pts',(65.1429860104,-6.93374364056231,68.7237906471918));
#133139=CARTESIAN_POINT('Ctrl Pts',(65.141417161647,-6.91661976904466,68.7148935659804));
#133140=CARTESIAN_POINT('Ctrl Pts',(65.1408375768619,-6.91047034785759,
68.7116063878611));
#133141=CARTESIAN_POINT('Ctrl Pts',(65.1491744576555,-6.94398141948418,
68.7726764498994));
#133142=CARTESIAN_POINT('Ctrl Pts',(65.1491482532267,-6.94358779616249,
68.7725255874527));
#133143=CARTESIAN_POINT('Ctrl Pts',(65.1485071429687,-6.93411497591497,
68.7688386960651));
#133144=CARTESIAN_POINT('Ctrl Pts',(65.1468808355773,-6.91549358299687,
68.7596188387069));
#133145=CARTESIAN_POINT('Ctrl Pts',(65.1452515407344,-6.89771080359099,
68.7503787973671));
#133146=CARTESIAN_POINT('Ctrl Pts',(65.1446433910398,-6.89125887007876,
68.7469297157195));
#133147=CARTESIAN_POINT('Ctrl Pts',(65.1557607443018,-6.92947588538437,
68.8097147522224));
#133148=CARTESIAN_POINT('Ctrl Pts',(65.155720141749,-6.92890803952096,68.8094845487692));
#133149=CARTESIAN_POINT('Ctrl Pts',(65.1547522172099,-6.91547825177383,
68.8039966501812));
#133150=CARTESIAN_POINT('Ctrl Pts',(65.1531649402084,-6.8972590585529,68.7949946569169));
#133151=CARTESIAN_POINT('Ctrl Pts',(65.1514752507228,-6.87881793207328,
68.7854119473515));
#133152=CARTESIAN_POINT('Ctrl Pts',(65.1508385604312,-6.87206374371237,
68.781801099976));
#133153=CARTESIAN_POINT('',(65.1441607442837,-6.89690667515947,68.7364336189164));
#133154=CARTESIAN_POINT('',(65.1506852045397,-6.87254041891262,68.7809350460487));
#133155=CARTESIAN_POINT('Origin',(66.1354906276427,-6.87281762818581,68.607288395026));
#133156=CARTESIAN_POINT('',(65.1554676900943,-6.9282418042031,68.808018444524));
#133157=CARTESIAN_POINT('Ctrl Pts',(65.1554654484591,-6.92824180453999,
68.808018841215));
#133158=CARTESIAN_POINT('Ctrl Pts',(65.1511823527249,-6.91706470348454,
68.7837161221291));
#133159=CARTESIAN_POINT('Ctrl Pts',(65.1474541412159,-6.90679031326606,
68.7598370684572));
#133160=CARTESIAN_POINT('Ctrl Pts',(65.14416106117,-6.89690666738156,68.7364335775926));
#133161=CARTESIAN_POINT('Ctrl Pts',(65.1554609455217,-6.92824180338472,
68.8080196357745));
#133162=CARTESIAN_POINT('Ctrl Pts',(65.1554598852463,-6.9282270379923,68.8080136226073));
#133163=CARTESIAN_POINT('Ctrl Pts',(65.1554588248862,-6.92821227449162,
68.8080076089597));
#133164=CARTESIAN_POINT('Ctrl Pts',(65.1554577644413,-6.92819751288013,
68.8080015948315));
#133165=CARTESIAN_POINT('Ctrl Pts',(65.1545901961715,-6.91612078396726,
68.8030813328399));
#133166=CARTESIAN_POINT('Ctrl Pts',(65.1536662468902,-6.9053125244734,68.7978413830879));
#133167=CARTESIAN_POINT('Ctrl Pts',(65.1526864112108,-6.89434361965686,
68.7922844405439));
#133168=CARTESIAN_POINT('Ctrl Pts',(65.1526345313573,-6.89376284352584,
68.7919902143066));
#133169=CARTESIAN_POINT('Ctrl Pts',(65.1525824938791,-6.89318160595316,
68.7916950941604));
#133170=CARTESIAN_POINT('Ctrl Pts',(65.1525302985756,-6.89259969156981,
68.7913990789963));
#133171=CARTESIAN_POINT('Ctrl Pts',(65.1519369363571,-6.88598442186751,
68.7880339445319));
#133172=CARTESIAN_POINT('Ctrl Pts',(65.1513231666928,-6.87928156135235,
68.7845530819381));
#133173=CARTESIAN_POINT('Ctrl Pts',(65.1506852076991,-6.87254041916445,
68.7809350467598));
#133174=CARTESIAN_POINT('Ctrl Pts',(65.1394962399547,-6.92987609657407,
68.6760901283112));
#133175=CARTESIAN_POINT('Ctrl Pts',(65.1389690427465,-6.92427743436571,
68.6730999838425));
#133176=CARTESIAN_POINT('Ctrl Pts',(65.1372553241028,-6.90657130252873,
68.6633787872026));
#133177=CARTESIAN_POINT('Ctrl Pts',(65.1338515053416,-6.87499181440707,
68.6440763568521));
#133178=CARTESIAN_POINT('Ctrl Pts',(65.1288246013982,-6.83442541808995,
68.615566793012));
#133179=CARTESIAN_POINT('Ctrl Pts',(65.1235003522383,-6.79680702773606,
68.5853716269996));
#133180=CARTESIAN_POINT('Ctrl Pts',(65.1197752963197,-6.7730817711464,68.5642457819742));
#133181=CARTESIAN_POINT('Ctrl Pts',(65.1182256999152,-6.7635933515749,68.5554575793337));
#133182=CARTESIAN_POINT('Ctrl Pts',(65.1408623196493,-6.91073297552592,
68.7117467190877));
#133183=CARTESIAN_POINT('Ctrl Pts',(65.1403080523265,-6.90484744757448,
68.7086031398901));
#133184=CARTESIAN_POINT('Ctrl Pts',(65.1384869336936,-6.88602316190435,
68.6982735918235));
#133185=CARTESIAN_POINT('Ctrl Pts',(65.134885933983,-6.85262897908219,68.6778523602412));
#133186=CARTESIAN_POINT('Ctrl Pts',(65.1295969110304,-6.80995270579319,
68.6478564387582));
#133187=CARTESIAN_POINT('Ctrl Pts',(65.1240299537541,-6.77062767825713,
68.616284755745));
#133188=CARTESIAN_POINT('Ctrl Pts',(65.1201503127629,-6.74591898706875,
68.5942822162525));
#133189=CARTESIAN_POINT('Ctrl Pts',(65.1185385200063,-6.73604970686306,
68.5851412821568));
#133190=CARTESIAN_POINT('Ctrl Pts',(65.1446693495273,-6.89153437655917,
68.7470769375128));
#133191=CARTESIAN_POINT('Ctrl Pts',(65.1440879336391,-6.88536115151044,
68.7437794789231));
#133192=CARTESIAN_POINT('Ctrl Pts',(65.1421591037656,-6.86541547152994,
68.7328398163906));
#133193=CARTESIAN_POINT('Ctrl Pts',(65.1383603516631,-6.83020133491268,
68.7112965412231));
#133194=CARTESIAN_POINT('Ctrl Pts',(65.1328084500647,-6.78540907010117,
68.6798099545433));
#133195=CARTESIAN_POINT('Ctrl Pts',(65.1269980812893,-6.74437245944551,
68.6468577653));
#133196=CARTESIAN_POINT('Ctrl Pts',(65.1229634072287,-6.71867748360566,
68.6239759906272));
#133197=CARTESIAN_POINT('Ctrl Pts',(65.121289237871,-6.70842623900873,68.614481302839));
#133198=CARTESIAN_POINT('Ctrl Pts',(65.150865733584,-6.87235211804336,68.7819552064712));
#133199=CARTESIAN_POINT('Ctrl Pts',(65.1502571922374,-6.86589144076419,
68.7785039994602));
#133200=CARTESIAN_POINT('Ctrl Pts',(65.1482207427991,-6.84482532092261,
68.766954741747));
#133201=CARTESIAN_POINT('Ctrl Pts',(65.1442244066172,-6.80779277952251,
68.7442903779965));
#133202=CARTESIAN_POINT('Ctrl Pts',(65.1384098501162,-6.76088632416654,
68.7113143948654));
#133203=CARTESIAN_POINT('Ctrl Pts',(65.1323562770159,-6.71813958716634,
68.6769828743784));
#133204=CARTESIAN_POINT('Ctrl Pts',(65.1281667018386,-6.69145916612878,
68.6532226128664));
#133205=CARTESIAN_POINT('Ctrl Pts',(65.1264302089705,-6.68082628224091,
68.6433744724751));
#133206=CARTESIAN_POINT('',(65.1309287612286,-6.85155002742103,68.6274185545369));
#133207=CARTESIAN_POINT('Ctrl Pts',(65.14416106117,-6.89690666738156,68.7364335775926));
#133208=CARTESIAN_POINT('Ctrl Pts',(65.139541879359,-6.88303685803668,68.7035889625114));
#133209=CARTESIAN_POINT('Ctrl Pts',(65.1351852092738,-6.86772274606561,
68.6676631553856));
#133210=CARTESIAN_POINT('Ctrl Pts',(65.1309287612286,-6.85155002742104,
68.6274185545369));
#133211=CARTESIAN_POINT('',(65.1263322567563,-6.68184571691787,68.6428226491504));
#133212=CARTESIAN_POINT('Origin',(65.0998354960377,-6.818067512662,68.4925520530996));
#133213=CARTESIAN_POINT('',(65.1182638051832,-6.76382675080627,68.5556736851631));
#133214=CARTESIAN_POINT('Origin',(66.1111353668526,-6.68186340008987,68.4691561841244));
#133215=CARTESIAN_POINT('Origin',(65.0627991145643,-6.85369791430341,68.2411322661509));
#133216=CARTESIAN_POINT('Ctrl Pts',(65.1393808590346,-6.96014231171326,
68.618798447603));
#133217=CARTESIAN_POINT('Ctrl Pts',(65.1389042098079,-6.95508367036459,
68.6160948227003));
#133218=CARTESIAN_POINT('Ctrl Pts',(65.1373676824532,-6.9392301048245,68.6073773797974));
#133219=CARTESIAN_POINT('Ctrl Pts',(65.1342860536698,-6.91061645632782,
68.5899030215337));
#133220=CARTESIAN_POINT('Ctrl Pts',(65.129676712871,-6.87341115490448,68.5637612683055));
#133221=CARTESIAN_POINT('Ctrl Pts',(65.1247496922159,-6.83858632048248,
68.5358189776352));
#133222=CARTESIAN_POINT('Ctrl Pts',(65.1212833835859,-6.81649988158678,
68.5161605602661));
#133223=CARTESIAN_POINT('Ctrl Pts',(65.1198454596578,-6.80768964317406,
68.508005681332));
#133224=CARTESIAN_POINT('Ctrl Pts',(65.1387132610527,-6.95001387475172,
68.6378926818026));
#133225=CARTESIAN_POINT('Ctrl Pts',(65.1382224181339,-6.94480491726722,
68.6351086082347));
#133226=CARTESIAN_POINT('Ctrl Pts',(65.1366293538061,-6.92836306631528,
68.6260709173592));
#133227=CARTESIAN_POINT('Ctrl Pts',(65.1334437409379,-6.89879243202413,
68.6080065552313));
#133228=CARTESIAN_POINT('Ctrl Pts',(65.1286958085209,-6.86047156380297,
68.5810789119924));
#133229=CARTESIAN_POINT('Ctrl Pts',(65.1236407346436,-6.82474630464972,
68.5524103685699));
#133230=CARTESIAN_POINT('Ctrl Pts',(65.1200929585004,-6.80214140449738,
68.5322899264659));
#133231=CARTESIAN_POINT('Ctrl Pts',(65.118622415774,-6.79313129599011,68.5239500579557));
#133232=CARTESIAN_POINT('Ctrl Pts',(65.1387451082755,-6.93983821679403,
68.6569520576361));
#133233=CARTESIAN_POINT('Ctrl Pts',(65.1382400054905,-6.93447824236689,
68.6540871603338));
#133234=CARTESIAN_POINT('Ctrl Pts',(65.1365901406018,-6.91744536328741,
68.6447277284193));
#133235=CARTESIAN_POINT('Ctrl Pts',(65.1333000588522,-6.88691328152396,
68.6260706116997));
#133236=CARTESIAN_POINT('Ctrl Pts',(65.1284128886725,-6.84747164548773,
68.5983534144583));
#133237=CARTESIAN_POINT('Ctrl Pts',(65.1232291645607,-6.81084176362548,
68.5689552323338));
#133238=CARTESIAN_POINT('Ctrl Pts',(65.1195995410848,-6.78771598503634,
68.5483706114342));
#133239=CARTESIAN_POINT('Ctrl Pts',(65.1180962274842,-6.77850507459625,
68.539844890886));
#133240=CARTESIAN_POINT('Ctrl Pts',(65.1394727093545,-6.92962631050212,
68.6759566677395));
#133241=CARTESIAN_POINT('Ctrl Pts',(65.1389532959058,-6.92411478117078,
68.6730106587876));
#133242=CARTESIAN_POINT('Ctrl Pts',(65.1372464281181,-6.90648876856817,
68.663328339709));
#133243=CARTESIAN_POINT('Ctrl Pts',(65.1338515053416,-6.87499181440707,
68.6440763568521));
#133244=CARTESIAN_POINT('Ctrl Pts',(65.1288246013981,-6.83442541808995,
68.615566793012));
#133245=CARTESIAN_POINT('Ctrl Pts',(65.1235117687664,-6.79688769101786,
68.5854363730231));
#133246=CARTESIAN_POINT('Ctrl Pts',(65.1198000063964,-6.77323917848776,
68.5643859198026));
#133247=CARTESIAN_POINT('Ctrl Pts',(65.1182638051832,-6.76382675080628,
68.5556736851632));
#133248=CARTESIAN_POINT('',(65.1197969390187,-6.80693156137258,68.5088219205847));
#133249=CARTESIAN_POINT('Ctrl Pts',(65.1309287467098,-6.85154997225577,
68.6274184172623));
#133250=CARTESIAN_POINT('Ctrl Pts',(65.1271634026351,-6.83714074568404,
68.5915609828876));
#133251=CARTESIAN_POINT('Ctrl Pts',(65.1234786475439,-6.82209332249245,
68.5522537135607));
#133252=CARTESIAN_POINT('Ctrl Pts',(65.1197969390187,-6.80693156137258,
68.5088219205847));
#133253=CARTESIAN_POINT('Origin',(66.1111167056211,-6.68168974877604,68.4689977647608));
#133254=CARTESIAN_POINT('Ctrl Pts',(65.1342438570207,-6.88922545630012,
68.4173762199009));
#133255=CARTESIAN_POINT('Ctrl Pts',(65.133486060561,-6.88458243975978,68.4130785355508));
#133256=CARTESIAN_POINT('Ctrl Pts',(65.1304933916005,-6.86666656489,68.3961062266279));
#133257=CARTESIAN_POINT('Ctrl Pts',(65.1246847728085,-6.83477575818617,
68.3631639449019));
#133258=CARTESIAN_POINT('Ctrl Pts',(65.1161582670608,-6.79355322048586,
68.3148077157122));
#133259=CARTESIAN_POINT('Ctrl Pts',(65.1060825958666,-6.75087779215306,
68.2576657485828));
#133260=CARTESIAN_POINT('Ctrl Pts',(65.0942790437781,-6.70741963316853,
68.1907244770599));
#133261=CARTESIAN_POINT('Ctrl Pts',(65.0806265551699,-6.66416928709678,
68.1132973669754));
#133262=CARTESIAN_POINT('Ctrl Pts',(65.0650730726838,-6.62230767446081,
68.0250891843942));
#133263=CARTESIAN_POINT('Ctrl Pts',(65.0475810184328,-6.58288451356995,
67.9258868152054));
#133264=CARTESIAN_POINT('Ctrl Pts',(65.0280726826782,-6.5470248949559,67.8152495452771));
#133265=CARTESIAN_POINT('Ctrl Pts',(65.0063045667778,-6.51580441028535,
67.6917964253113));
#133266=CARTESIAN_POINT('Ctrl Pts',(64.9820073764202,-6.49060466876522,
67.5540002113891));
#133267=CARTESIAN_POINT('Ctrl Pts',(64.9549113829709,-6.47312496298017,
67.4003311963398));
#133268=CARTESIAN_POINT('Ctrl Pts',(64.9332779206116,-6.46744580878183,
67.2776417345743));
#133269=CARTESIAN_POINT('Ctrl Pts',(64.9207216538056,-6.46711162774575,
67.2064316069159));
#133270=CARTESIAN_POINT('Ctrl Pts',(64.9182105185209,-6.46716137792081,
67.1921902510292));
#133271=CARTESIAN_POINT('Ctrl Pts',(65.1156612636186,-6.82092619803015,
68.4944428007781));
#133272=CARTESIAN_POINT('Ctrl Pts',(65.1148110828427,-6.81571710110071,
68.4896211812618));
#133273=CARTESIAN_POINT('Ctrl Pts',(65.1114622226625,-6.79567000857472,
68.4706288246759));
#133274=CARTESIAN_POINT('Ctrl Pts',(65.1050182325365,-6.76030288849035,
68.4340831623743));
#133275=CARTESIAN_POINT('Ctrl Pts',(65.095644169583,-6.71499492821166,68.3809202014195));
#133276=CARTESIAN_POINT('Ctrl Pts',(65.0846629933304,-6.66849766520989,
68.3186428586899));
#133277=CARTESIAN_POINT('Ctrl Pts',(65.0719005692391,-6.62152193749562,
68.2462635541871));
#133278=CARTESIAN_POINT('Ctrl Pts',(65.0572480016601,-6.57511671269435,
68.1631647143009));
#133279=CARTESIAN_POINT('Ctrl Pts',(65.0406747571108,-6.53052359359599,
68.0691731737046));
#133280=CARTESIAN_POINT('Ctrl Pts',(65.0221556399096,-6.48879599868487,
67.964146041071));
#133281=CARTESIAN_POINT('Ctrl Pts',(65.0015802797845,-6.4509822157624,67.847457375233));
#133282=CARTESIAN_POINT('Ctrl Pts',(64.9787112300804,-6.41819144706752,
67.7177605494007));
#133283=CARTESIAN_POINT('Ctrl Pts',(64.95327920567,-6.39182510624466,67.5735283717446));
#133284=CARTESIAN_POINT('Ctrl Pts',(64.9250419773436,-6.37362011926285,
67.4133870920872));
#133285=CARTESIAN_POINT('Ctrl Pts',(64.9025780060496,-6.36772926219258,
67.2859875800991));
#133286=CARTESIAN_POINT('Ctrl Pts',(64.8895541865461,-6.36738304863499,
67.2121258293271));
#133287=CARTESIAN_POINT('Ctrl Pts',(64.8869501391361,-6.36743465915249,
67.1973575425938));
#133288=CARTESIAN_POINT('Ctrl Pts',(65.1132982389247,-6.75037255747734,
68.5710850505295));
#133289=CARTESIAN_POINT('Ctrl Pts',(65.1123526244647,-6.74457869530585,
68.5657222020991));
#133290=CARTESIAN_POINT('Ctrl Pts',(65.1086358161119,-6.722330039128,68.5446431212891));
#133291=CARTESIAN_POINT('Ctrl Pts',(65.1015354826836,-6.68337186152832,
68.5043751401169));
#133292=CARTESIAN_POINT('Ctrl Pts',(65.0912858868476,-6.63384362941354,
68.4462467895843));
#133293=CARTESIAN_POINT('Ctrl Pts',(65.0793693171516,-6.58339838284189,
68.3786645657567));
#133294=CARTESIAN_POINT('Ctrl Pts',(65.0656163711664,-6.5327889805305,68.3006677328371));
#133295=CARTESIAN_POINT('Ctrl Pts',(65.0499307145907,-6.48312474259335,
68.2117099539833));
#133296=CARTESIAN_POINT('Ctrl Pts',(65.0323040482633,-6.43570995705239,
68.1117441616463));
#133297=CARTESIAN_POINT('Ctrl Pts',(65.0127239674143,-6.39160186470016,
68.0007000051564));
#133298=CARTESIAN_POINT('Ctrl Pts',(64.9910463631973,-6.35176941554781,
67.8777602024444));
#133299=CARTESIAN_POINT('Ctrl Pts',(64.9670400407054,-6.31735653180476,
67.7416135821254));
#133300=CARTESIAN_POINT('Ctrl Pts',(64.9404357242987,-6.28978508524634,
67.5907330061794));
#133301=CARTESIAN_POINT('Ctrl Pts',(64.9110195918763,-6.27083087740692,
67.4239058291597));
#133302=CARTESIAN_POINT('Ctrl Pts',(64.8876976986906,-6.26472132969921,
67.2916408003443));
#133303=CARTESIAN_POINT('Ctrl Pts',(64.8741908937815,-6.26436268645759,
67.2150399032216));
#133304=CARTESIAN_POINT('Ctrl Pts',(64.871490867457,-6.26441621872265,67.1997272930141));
#133305=CARTESIAN_POINT('Ctrl Pts',(65.1268063180921,-6.67931671571179,
68.6454713706));
#133306=CARTESIAN_POINT('Ctrl Pts',(65.1257645906506,-6.67293392593594,
68.6395634407853));
#133307=CARTESIAN_POINT('Ctrl Pts',(65.121677215068,-6.64846803536371,68.6163827824362));
#133308=CARTESIAN_POINT('Ctrl Pts',(65.113915866482,-6.60589323908104,68.5723659869065));
#133309=CARTESIAN_POINT('Ctrl Pts',(65.1027845057151,-6.55211469521134,
68.5092369031251));
#133310=CARTESIAN_POINT('Ctrl Pts',(65.0899258844404,-6.49769336330045,
68.4363120380258));
#133311=CARTESIAN_POINT('Ctrl Pts',(65.075175366021,-6.44342442187559,68.3526576910904));
#133312=CARTESIAN_POINT('Ctrl Pts',(65.0584492669151,-6.39047797312858,
68.2577992693084));
#133313=CARTESIAN_POINT('Ctrl Pts',(65.0397616805472,-6.34022143650729,
68.151816700473));
#133314=CARTESIAN_POINT('Ctrl Pts',(65.0191130841056,-6.2937159023197,68.0347126909168));
#133315=CARTESIAN_POINT('Ctrl Pts',(64.9963253900166,-6.25185041805988,
67.9054772557028));
#133316=CARTESIAN_POINT('Ctrl Pts',(64.9711736996225,-6.21580387304457,
67.7628349312237));
#133317=CARTESIAN_POINT('Ctrl Pts',(64.9433887468392,-6.18701874280112,
67.605258633651));
#133318=CARTESIAN_POINT('Ctrl Pts',(64.9127853188742,-6.16730998114583,
67.4316979690137));
#133319=CARTESIAN_POINT('Ctrl Pts',(64.8885993971038,-6.16098018615946,
67.2945327905948));
#133320=CARTESIAN_POINT('Ctrl Pts',(64.8746061688967,-6.16060902475923,
67.2151732498622));
#133321=CARTESIAN_POINT('Ctrl Pts',(64.8718094804788,-6.16066449245085,
67.199312441683));
#133322=CARTESIAN_POINT('',(65.0995136833054,-6.72702879152427,68.2205016222657));
#133323=CARTESIAN_POINT('Ctrl Pts',(65.1197964539582,-6.80692956382894,
68.5088161984767));
#133324=CARTESIAN_POINT('Ctrl Pts',(65.117970090298,-6.79929279591152,68.4870734254445));
#133325=CARTESIAN_POINT('Ctrl Pts',(65.1161906463661,-6.79193584047724,
68.4647514783563));
#133326=CARTESIAN_POINT('Ctrl Pts',(65.1135867664279,-6.78123706716053,
68.4304642096668));
#133327=CARTESIAN_POINT('Ctrl Pts',(65.1127294947203,-6.77772688537746,
68.4189006628725));
#133328=CARTESIAN_POINT('Ctrl Pts',(65.1110297678899,-6.770811996763,68.3955047967372));
#133329=CARTESIAN_POINT('Ctrl Pts',(65.1100610746099,-6.76690233978478,
68.3818714985991));
#133330=CARTESIAN_POINT('Ctrl Pts',(65.1064983128958,-6.75265152221011,
68.3310438611609));
#133331=CARTESIAN_POINT('Ctrl Pts',(65.103111422614,-6.73945547580017,68.2811679223586));
#133332=CARTESIAN_POINT('Ctrl Pts',(65.0994829680072,-6.72702809613026,
68.2205074846029));
#133333=CARTESIAN_POINT('',(64.8738238573791,-6.16438935871099,67.210776354606));
#133334=CARTESIAN_POINT('Ctrl Pts',(65.1263322567668,-6.68184571628219,
68.6428226485642));
#133335=CARTESIAN_POINT('Ctrl Pts',(65.1252939386827,-6.67548394330349,
68.6369340541028));
#133336=CARTESIAN_POINT('Ctrl Pts',(65.1242407634166,-6.66918005369973,
68.6309612003757));
#133337=CARTESIAN_POINT('Ctrl Pts',(65.1231735592988,-6.6629353884095,68.6249087850782));
#133338=CARTESIAN_POINT('Ctrl Pts',(65.1201122562707,-6.64502240208925,
68.607547272909));
#133339=CARTESIAN_POINT('Ctrl Pts',(65.1169355176638,-6.62759673969112,
68.5895310930464));
#133340=CARTESIAN_POINT('Ctrl Pts',(65.1136570498455,-6.61067539008644,
68.5709379781644));
#133341=CARTESIAN_POINT('Ctrl Pts',(65.1100927169032,-6.59227858793113,
68.5507236416057));
#133342=CARTESIAN_POINT('Ctrl Pts',(65.1064081408252,-6.57447787972176,
68.5298273723462));
#133343=CARTESIAN_POINT('Ctrl Pts',(65.1026212919839,-6.55729893056469,
68.5083510854263));
#133344=CARTESIAN_POINT('Ctrl Pts',(65.0984830630297,-6.53852595393328,
68.4848820228665));
#133345=CARTESIAN_POINT('Ctrl Pts',(65.094222701058,-6.5204954750822,68.4607203095474));
#133346=CARTESIAN_POINT('Ctrl Pts',(65.0898599033342,-6.50321292732108,
68.4359776542108));
#133347=CARTESIAN_POINT('Ctrl Pts',(65.0850814403227,-6.48428378587311,
68.4088776438919));
#133348=CARTESIAN_POINT('Ctrl Pts',(65.0801800926007,-6.46625188284986,
68.3810807197495));
#133349=CARTESIAN_POINT('Ctrl Pts',(65.0751779368011,-6.44910586247529,
68.3527120845897));
#133350=CARTESIAN_POINT('Ctrl Pts',(65.0697293007619,-6.43042943009645,
68.3218113341725));
#133351=CARTESIAN_POINT('Ctrl Pts',(65.0641610577563,-6.41280408151792,
68.2902322589422));
#133352=CARTESIAN_POINT('Ctrl Pts',(65.0584982023557,-6.39619966014369,
68.2581166101517));
#133353=CARTESIAN_POINT('Ctrl Pts',(65.0523870831185,-6.37828085563542,
68.2234587308216));
#133354=CARTESIAN_POINT('Ctrl Pts',(65.0461657798431,-6.36155100579428,
68.1881759667537));
#133355=CARTESIAN_POINT('Ctrl Pts',(65.0398590110274,-6.34594160392812,
68.152408503523));
#133356=CARTESIAN_POINT('Ctrl Pts',(65.0331037660103,-6.32922221286453,
68.1140976053711));
#133357=CARTESIAN_POINT('Ctrl Pts',(65.0262504682212,-6.31378828614223,
68.0752306223181));
#133358=CARTESIAN_POINT('Ctrl Pts',(65.019312337714,-6.29957015532149,68.0358825289906));
#133359=CARTESIAN_POINT('Ctrl Pts',(65.0118621859929,-6.28430275271249,
67.9936306190665));
#133360=CARTESIAN_POINT('Ctrl Pts',(65.0043142186634,-6.27043721470028,
67.9508239692352));
#133361=CARTESIAN_POINT('Ctrl Pts',(64.9966934743881,-6.25793178150374,
67.9076045808126));
#133362=CARTESIAN_POINT('Ctrl Pts',(64.988443653798,-6.24439405125804,67.8608175233269));
#133363=CARTESIAN_POINT('Ctrl Pts',(64.9801085451537,-6.23245024118954,
67.8135467732247));
#133364=CARTESIAN_POINT('Ctrl Pts',(64.9717130036401,-6.22202862475033,
67.7659332912632));
#133365=CARTESIAN_POINT('Ctrl Pts',(64.9625709513924,-6.21068034401822,
67.7140861365454));
#133366=CARTESIAN_POINT('Ctrl Pts',(64.9533572414561,-6.20113699118725,
67.6618325908494));
#133367=CARTESIAN_POINT('Ctrl Pts',(64.944105499176,-6.19329504774133,67.6093633529697));
#133368=CARTESIAN_POINT('Ctrl Pts',(64.9339962248679,-6.18472624469832,
67.5520308092821));
#133369=CARTESIAN_POINT('Ctrl Pts',(64.9238415409629,-6.17818887081409,
67.4944407349221));
#133370=CARTESIAN_POINT('Ctrl Pts',(64.9136642615231,-6.17349919156016,
67.4367225148641));
#133371=CARTESIAN_POINT('Ctrl Pts',(64.9025266470073,-6.16836699095177,
67.3735579639306));
#133372=CARTESIAN_POINT('Ctrl Pts',(64.8913619713804,-6.16544763621553,
67.3102399417465));
#133373=CARTESIAN_POINT('Ctrl Pts',(64.8801826595514,-6.16462907124658,
67.2468389134668));
#133374=CARTESIAN_POINT('Ctrl Pts',(64.8780635186918,-6.16447390476599,
67.2348206683706));
#133375=CARTESIAN_POINT('Ctrl Pts',(64.8759438519186,-6.16439422531526,
67.2227994406676));
#133376=CARTESIAN_POINT('Ctrl Pts',(64.8738238574643,-6.16438935871099,
67.210776354591));
#133377=CARTESIAN_POINT('',(64.9200365392845,-6.46714802416996,67.2025868445748));
#133378=CARTESIAN_POINT('Origin',(65.8588874291605,-6.16436606275721,67.0386110313669));
#133379=CARTESIAN_POINT('Ctrl Pts',(65.0995290409546,-6.72702913922128,
68.2204986910971));
#133380=CARTESIAN_POINT('Ctrl Pts',(65.0978779672016,-6.72101820418093,
68.2111349864784));
#133381=CARTESIAN_POINT('Ctrl Pts',(65.0962045410388,-6.71510725237692,
68.201644515001));
#133382=CARTESIAN_POINT('Ctrl Pts',(65.0945101637993,-6.70929906104744,
68.1920352241046));
#133383=CARTESIAN_POINT('Ctrl Pts',(65.0900972320726,-6.69417187968862,
68.1670082444693));
#133384=CARTESIAN_POINT('Ctrl Pts',(65.0855421738897,-6.67974170153992,
68.1411752259264));
#133385=CARTESIAN_POINT('Ctrl Pts',(65.080865553793,-6.66602823420956,68.1146527954373));
#133386=CARTESIAN_POINT('Ctrl Pts',(65.0758187507953,-6.65122926260156,
68.0860309533949));
#133387=CARTESIAN_POINT('Ctrl Pts',(65.070630379487,-6.6372649565294,68.0566062374781));
#133388=CARTESIAN_POINT('Ctrl Pts',(65.065325250278,-6.62413396216025,68.0265193546337));
#133389=CARTESIAN_POINT('Ctrl Pts',(65.0596428831358,-6.61006924704979,
67.9942930491558));
#133390=CARTESIAN_POINT('Ctrl Pts',(65.0538265628448,-6.59696056768424,
67.9613070576571));
#133391=CARTESIAN_POINT('Ctrl Pts',(65.0479081195714,-6.58482980871447,
67.9277418979278));
#133392=CARTESIAN_POINT('Ctrl Pts',(65.0415529158574,-6.57180384210533,
67.8916997466531));
#133393=CARTESIAN_POINT('Ctrl Pts',(65.0350799603681,-6.55990545579126,
67.8549897918566));
#133394=CARTESIAN_POINT('Ctrl Pts',(65.0285101932219,-6.54912373938078,
67.8177307908735));
#133395=CARTESIAN_POINT('Ctrl Pts',(65.021398112376,-6.53745202605182,67.7773961760644));
#133396=CARTESIAN_POINT('Ctrl Pts',(65.0141725772018,-6.5270889468045,67.7364181297901));
#133397=CARTESIAN_POINT('Ctrl Pts',(65.0068585115159,-6.51800755521313,
67.6949380020386));
#133398=CARTESIAN_POINT('Ctrl Pts',(64.9988940986838,-6.50811867058614,
67.6497695723414));
#133399=CARTESIAN_POINT('Ctrl Pts',(64.9908247115997,-6.49974953548232,
67.6040058040826));
#133400=CARTESIAN_POINT('Ctrl Pts',(64.9826739639034,-6.49283962908175,
67.5577806168571));
#133401=CARTESIAN_POINT('Ctrl Pts',(64.9737677268307,-6.48528924636276,
67.5072708364669));
#133402=CARTESIAN_POINT('Ctrl Pts',(64.9647643475857,-6.47948113969311,
67.4562101354345));
#133403=CARTESIAN_POINT('Ctrl Pts',(64.9556971386543,-6.47530096076753,
67.4047874382661));
#133404=CARTESIAN_POINT('Ctrl Pts',(64.945774321196,-6.47072632785289,67.3485123440143));
#133405=CARTESIAN_POINT('Ctrl Pts',(64.9357750593742,-6.46810135045388,
67.2918037122387));
#133406=CARTESIAN_POINT('Ctrl Pts',(64.9257374667552,-6.46736283728807,
67.2348776957069));
#133407=CARTESIAN_POINT('Ctrl Pts',(64.9238407956026,-6.4672232902203,67.224121139082));
#133408=CARTESIAN_POINT('Ctrl Pts',(64.9219427574521,-6.4671510987288,67.2133568298243));
#133409=CARTESIAN_POINT('Ctrl Pts',(64.9200435026063,-6.46714577790044,
67.2025856178632));
#133410=CARTESIAN_POINT('Origin',(27.4324635166691,-5.,72.98888938658));
#133411=CARTESIAN_POINT('Origin',(-6.16760765460691,-5.,58.73107688658));
#133412=CARTESIAN_POINT('Origin',(-7.28284733203891,-5.,84.2626284592));
#133413=CARTESIAN_POINT('Origin',(1.07038457110909,-5.,122.41156512159));
#133414=CARTESIAN_POINT('',(22.0949841886482,-5.0000000038066,58.2694426477661));
#133415=CARTESIAN_POINT('Ctrl Pts',(21.7837562285525,-5.99999999944872,
59.2197092315316));
#133416=CARTESIAN_POINT('Ctrl Pts',(21.7975260636522,-5.9999985274307,59.1775705921136));
#133417=CARTESIAN_POINT('Ctrl Pts',(21.8113023518639,-5.99704480733659,
59.1354341304315));
#133418=CARTESIAN_POINT('Ctrl Pts',(21.8249621981295,-5.99116480402708,
59.0936711320751));
#133419=CARTESIAN_POINT('Ctrl Pts',(21.8386209201063,-5.98528528467776,
59.0519115710685));
#133420=CARTESIAN_POINT('Ctrl Pts',(21.8521630766078,-5.97648002554931,
59.0105258475984));
#133421=CARTESIAN_POINT('Ctrl Pts',(21.8654679408015,-5.96482663022172,
58.9698786061037));
#133422=CARTESIAN_POINT('Ctrl Pts',(21.878776121166,-5.95317033034366,58.9292212334874));
#133423=CARTESIAN_POINT('Ctrl Pts',(21.891846751647,-5.9386645937448,58.8893031360823));
#133424=CARTESIAN_POINT('Ctrl Pts',(21.9045632718707,-5.92143739888266,
58.8504762134119));
#133425=CARTESIAN_POINT('Ctrl Pts',(21.9172773736486,-5.90421348031269,
58.8116566749002));
#133426=CARTESIAN_POINT('Ctrl Pts',(21.929637367193,-5.88426931977393,58.7739283008067));
#133427=CARTESIAN_POINT('Ctrl Pts',(21.9415330544524,-5.86178085100885,
58.7376235503012));
#133428=CARTESIAN_POINT('Ctrl Pts',(21.9534307647554,-5.83928855773558,
58.7013126256175));
#133429=CARTESIAN_POINT('Ctrl Pts',(21.9648638862721,-5.81425132436283,
58.6664261886119));
#133430=CARTESIAN_POINT('Ctrl Pts',(21.9757303953022,-5.78689011291116,
58.6332717274391));
#133431=CARTESIAN_POINT('Ctrl Pts',(21.9855638438665,-5.76213008513021,
58.6032692042997));
#133432=CARTESIAN_POINT('Ctrl Pts',(21.9949333352515,-5.73546765831612,
58.5746848681192));
#133433=CARTESIAN_POINT('Ctrl Pts',(22.0037703020811,-5.70709562702803,
58.5477250946227));
#133434=CARTESIAN_POINT('Ctrl Pts',(22.0135389068795,-5.67573247196329,
58.5179230847457));
#133435=CARTESIAN_POINT('Ctrl Pts',(22.0226565265249,-5.64228005043222,
58.4901071089335));
#133436=CARTESIAN_POINT('Ctrl Pts',(22.0310426905364,-5.60703366985993,
58.4645226233129));
#133437=CARTESIAN_POINT('Ctrl Pts',(22.0394282631326,-5.57178977495957,
58.4389399419808));
#133438=CARTESIAN_POINT('Ctrl Pts',(22.0470823961994,-5.53475254125243,
58.4155887017076));
#133439=CARTESIAN_POINT('Ctrl Pts',(22.0539375354772,-5.49624883268982,
58.3946749534964));
#133440=CARTESIAN_POINT('Ctrl Pts',(22.060794398555,-5.4577354419469,58.3737559462936));
#133441=CARTESIAN_POINT('Ctrl Pts',(22.0668517939827,-5.41775523860441,
58.3552758767621));
#133442=CARTESIAN_POINT('Ctrl Pts',(22.0720562180904,-5.37666121128741,
58.3393979301013));
#133443=CARTESIAN_POINT('Ctrl Pts',(22.0772596369718,-5.33557512121761,
58.3235230502412));
#133444=CARTESIAN_POINT('Ctrl Pts',(22.0816103602574,-5.29337606565423,
58.3102494521123));
#133445=CARTESIAN_POINT('Ctrl Pts',(22.0850699519827,-5.25043647287593,
58.299694352261));
#133446=CARTESIAN_POINT('Ctrl Pts',(22.088530064537,-5.20749041569762,58.2891376633777));
#133447=CARTESIAN_POINT('Ctrl Pts',(22.0910987406586,-5.16380404500724,
58.2813004028194));
#133448=CARTESIAN_POINT('Ctrl Pts',(22.0927532489339,-5.11976304124748,
58.276251875659));
#133449=CARTESIAN_POINT('Ctrl Pts',(22.0942457554333,-5.08003432829404,
58.2716976768609));
#133450=CARTESIAN_POINT('Ctrl Pts',(22.0949945426852,-5.04001743309234,
58.2694122459578));
#133451=CARTESIAN_POINT('Ctrl Pts',(22.0949941775792,-5.00000000409752,
58.2694121261103));
#133452=CARTESIAN_POINT('',(-2.29973550255637,-5.,54.9957487971611));
#133453=CARTESIAN_POINT('Origin',(1.07038457110909,-5.,122.41156512159));
#133454=CARTESIAN_POINT('Origin',(-2.24980779825091,-5.,55.99450163162));
#133455=CARTESIAN_POINT('Origin',(-2.02513312664091,-5.,60.48888938658));
#133456=CARTESIAN_POINT('Origin',(-2.02513312664091,-5.,60.48888938658));
#133457=CARTESIAN_POINT('Origin',(-2.02513312664091,25.,60.48888938658));
#133458=CARTESIAN_POINT('',(-2.29973550255644,5.,54.9957487971611));
#133459=CARTESIAN_POINT('',(-2.29973550107091,-5.,54.99574879709));
#133460=CARTESIAN_POINT('Origin',(-2.02513312664091,5.,60.48888938658));
#133461=CARTESIAN_POINT('Origin',(-2.02513312664091,5.,60.48888938658));
#133462=CARTESIAN_POINT('Origin',(-6.16760765460691,5.,58.73107688658));
#133463=CARTESIAN_POINT('Origin',(-2.24980779825091,5.,55.99450163162));
#133464=CARTESIAN_POINT('Origin',(-8.75366715310791,111.0724296188,85.97453149762));
#133465=CARTESIAN_POINT('Origin',(14.4385554303262,1.4210854715202E-14,
81.8851169135651));
#133466=CARTESIAN_POINT('',(-6.54682287186491,5.,85.58540530862));
#133467=CARTESIAN_POINT('Origin',(26.6903689106391,-17.,82.263358164095));
#133468=CARTESIAN_POINT('',(23.6515258014716,7.5,65.0292224863863));
#133469=CARTESIAN_POINT('',(23.6515258014821,10.9472980747274,65.0292224863845));
#133470=CARTESIAN_POINT('',(23.6515258014693,-17.,65.0292224863868));
#133471=CARTESIAN_POINT('',(22.9296816314691,7.5,60.93544076844));
#133472=CARTESIAN_POINT('',(22.9296816314691,7.5,60.93544076844));
#133473=CARTESIAN_POINT('',(22.9296816314691,7.5,60.93544076844));
#133474=CARTESIAN_POINT('',(22.9354959621264,10.3319876690517,60.9684154762107));
#133475=CARTESIAN_POINT('',(22.9296818159191,10.33198965144,60.93544181454));
#133476=CARTESIAN_POINT('Ctrl Pts',(22.9354959621287,10.3319876695089,60.9684154762103));
#133477=CARTESIAN_POINT('Ctrl Pts',(22.9457594205585,10.3319918659453,61.0266224414067));
#133478=CARTESIAN_POINT('Ctrl Pts',(22.9561975687024,10.3325157444919,61.0858201212103));
#133479=CARTESIAN_POINT('Ctrl Pts',(22.9668129917587,10.3335903239921,61.1460231769825));
#133480=CARTESIAN_POINT('Ctrl Pts',(22.9892670680594,10.3358633083056,61.2733665716517));
#133481=CARTESIAN_POINT('Ctrl Pts',(23.0125146365289,10.3406023501125,61.4052100839497));
#133482=CARTESIAN_POINT('Ctrl Pts',(23.0365857422537,10.3481011670225,61.5417241083182));
#133483=CARTESIAN_POINT('Ctrl Pts',(23.0416535630085,10.3496799337151,61.5704651480497));
#133484=CARTESIAN_POINT('Ctrl Pts',(23.0467578645404,10.3513809019802,61.5994130805518));
#133485=CARTESIAN_POINT('Ctrl Pts',(23.0518988894436,10.3532065840058,61.62856928162));
#133486=CARTESIAN_POINT('Ctrl Pts',(23.0639202065515,10.3574755970881,61.696745558782));
#133487=CARTESIAN_POINT('Ctrl Pts',(23.0761427749971,10.3624230092554,61.7660631888724));
#133488=CARTESIAN_POINT('Ctrl Pts',(23.0885557652515,10.3680698206311,61.8364607547481));
#133489=CARTESIAN_POINT('Ctrl Pts',(23.1081071729758,10.3769639798374,61.9473422977947));
#133490=CARTESIAN_POINT('Ctrl Pts',(23.1281309847519,10.3875956593929,62.0609029775064));
#133491=CARTESIAN_POINT('Ctrl Pts',(23.1485877002943,10.4000241324366,62.176918776601));
#133492=CARTESIAN_POINT('Ctrl Pts',(23.1595523603548,10.4066857092528,62.2391024539405));
#133493=CARTESIAN_POINT('Ctrl Pts',(23.1706413774056,10.4138626166885,62.301991394839));
#133494=CARTESIAN_POINT('Ctrl Pts',(23.1818485931706,10.4215577992017,62.3655506738587));
#133495=CARTESIAN_POINT('Ctrl Pts',(23.1956058466466,10.4310039077265,62.4435719353888));
#133496=CARTESIAN_POINT('Ctrl Pts',(23.2095416513106,10.4412362594231,62.5226058109224));
#133497=CARTESIAN_POINT('Ctrl Pts',(23.2236490156693,10.4522538270402,62.6026126499251));
#133498=CARTESIAN_POINT('Ctrl Pts',(23.2464420503796,10.4700547283803,62.7318783732788));
#133499=CARTESIAN_POINT('Ctrl Pts',(23.2696828767045,10.4899077486182,62.8636836491963));
#133500=CARTESIAN_POINT('Ctrl Pts',(23.2933466050056,10.5118045940982,62.9978873213132));
#133501=CARTESIAN_POINT('Ctrl Pts',(23.30336140994,10.521071630694,63.0546841024722));
#133502=CARTESIAN_POINT('Ctrl Pts',(23.3134519635772,10.5307041071535,63.1119104758642));
#133503=CARTESIAN_POINT('Ctrl Pts',(23.3236163926547,10.5406985620617,63.1695558176983));
#133504=CARTESIAN_POINT('Ctrl Pts',(23.339000040912,10.5558249580115,63.2568008223788));
#133505=CARTESIAN_POINT('Ctrl Pts',(23.3545532509111,10.571784067664,63.3450074594824));
#133506=CARTESIAN_POINT('Ctrl Pts',(23.3702657805519,10.5885526295178,63.4341176431629));
#133507=CARTESIAN_POINT('Ctrl Pts',(23.3946901195582,10.6146185176166,63.5726349529082));
#133508=CARTESIAN_POINT('Ctrl Pts',(23.4194993251193,10.6426424725186,63.7133349493283));
#133509=CARTESIAN_POINT('Ctrl Pts',(23.4446595190143,10.6725366399531,63.8560254995665));
#133510=CARTESIAN_POINT('Ctrl Pts',(23.4549180172403,10.6847253084854,63.9142043340614));
#133511=CARTESIAN_POINT('Ctrl Pts',(23.4652348809764,10.6972242889174,63.9727141758234));
#133512=CARTESIAN_POINT('Ctrl Pts',(23.4756078830168,10.7100251716415,64.0315423937084));
#133513=CARTESIAN_POINT('Ctrl Pts',(23.4925128798764,10.7308869126697,64.1274153950565));
#133514=CARTESIAN_POINT('Ctrl Pts',(23.5095672887138,10.7525581219184,64.2241357538275));
#133515=CARTESIAN_POINT('Ctrl Pts',(23.5267450050852,10.7749698010488,64.3215554243934));
#133516=CARTESIAN_POINT('Ctrl Pts',(23.5524968689719,10.8085681268073,64.4676015018837));
#133517=CARTESIAN_POINT('Ctrl Pts',(23.5785257124883,10.8438323226742,64.6152184088107));
#133518=CARTESIAN_POINT('Ctrl Pts',(23.6047484448564,10.8805589711191,64.7639349141785));
#133519=CARTESIAN_POINT('Ctrl Pts',(23.6150258236674,10.894953111029,64.8222208257935));
#133520=CARTESIAN_POINT('Ctrl Pts',(23.6253330169625,10.9095713396704,64.8806758237816));
#133521=CARTESIAN_POINT('Ctrl Pts',(23.6356651406205,10.9243993782852,64.939272208841));
#133522=CARTESIAN_POINT('Ctrl Pts',(23.6409456318988,10.9319776198134,64.9692193630264));
#133523=CARTESIAN_POINT('Ctrl Pts',(23.6462325813711,10.9396109140533,64.9992031434345));
#133524=CARTESIAN_POINT('Ctrl Pts',(23.6515258014821,10.9472980747274,65.0292224863845));
#133525=CARTESIAN_POINT('Origin',(21.3942017988391,7.5,60.86545763396));
#133526=CARTESIAN_POINT('Origin',(22.1743141719575,7.5,65.289694752886));
#133527=CARTESIAN_POINT('Origin',(21.4524700019691,7.5,61.19591303503));
#133528=CARTESIAN_POINT('Ctrl Pts',(16.7315271092291,25.77957474242,75.8056538642681));
#133529=CARTESIAN_POINT('Ctrl Pts',(16.8902739491491,25.78276104928,76.726755143248));
#133530=CARTESIAN_POINT('Ctrl Pts',(17.4170423638691,25.68741378017,79.011155596728));
#133531=CARTESIAN_POINT('Ctrl Pts',(18.6971928491291,25.1486541372,82.327981456666));
#133532=CARTESIAN_POINT('Ctrl Pts',(20.3541926191191,24.21296098443,85.29757061493));
#133533=CARTESIAN_POINT('Ctrl Pts',(21.9876235905991,23.12636897321,87.62326197554));
#133534=CARTESIAN_POINT('Ctrl Pts',(23.5303110581191,21.96974605327,89.49482082956));
#133535=CARTESIAN_POINT('Ctrl Pts',(25.0147293345491,20.73535636643,91.08394632963));
#133536=CARTESIAN_POINT('Ctrl Pts',(26.4477039632491,19.42122041898,92.4661164628101));
#133537=CARTESIAN_POINT('Ctrl Pts',(27.8040593501691,18.0525443245,93.66246634875));
#133538=CARTESIAN_POINT('Ctrl Pts',(29.0976297887891,16.61722673478,94.7173081814599));
#133539=CARTESIAN_POINT('Ctrl Pts',(30.3859883571291,15.03805899871,95.692928827));
#133540=CARTESIAN_POINT('Ctrl Pts',(31.6846191544191,13.2490375268,96.6017522016999));
#133541=CARTESIAN_POINT('Ctrl Pts',(32.9283641549091,11.27078505501,97.39922069443));
#133542=CARTESIAN_POINT('Ctrl Pts',(34.0024905191591,9.24026551673301,98.0256740975701));
#133543=CARTESIAN_POINT('Ctrl Pts',(34.8835248980591,7.19980133487202,98.4916705583199));
#133544=CARTESIAN_POINT('Ctrl Pts',(35.5865206621291,5.09129120886101,98.8275149094299));
#133545=CARTESIAN_POINT('Ctrl Pts',(36.0644764908891,2.94897602587201,99.0360923986901));
#133546=CARTESIAN_POINT('Ctrl Pts',(36.2175390832591,1.50759720120401,99.1082321058299));
#133547=CARTESIAN_POINT('Ctrl Pts',(36.2511547877691,0.817200229439614,
99.1309346670101));
#133548=CARTESIAN_POINT('Ctrl Pts',(16.5657307648391,19.34436604072,75.8499470296021));
#133549=CARTESIAN_POINT('Ctrl Pts',(16.7027032210391,19.34727467235,76.647687526976));
#133550=CARTESIAN_POINT('Ctrl Pts',(17.1758927443291,19.26031994756,78.623309386718));
#133551=CARTESIAN_POINT('Ctrl Pts',(18.3744374416091,18.77127275203,81.451029832546));
#133552=CARTESIAN_POINT('Ctrl Pts',(19.9464727370091,17.9342387447,83.90371085737));
#133553=CARTESIAN_POINT('Ctrl Pts',(21.5011129654591,16.97934371574,85.75395997948));
#133554=CARTESIAN_POINT('Ctrl Pts',(22.9701058542891,15.98027083986,87.18714704112));
#133555=CARTESIAN_POINT('Ctrl Pts',(24.3829496628191,14.93205005415,88.35697360021));
#133556=CARTESIAN_POINT('Ctrl Pts',(25.7455828440791,13.83506997747,89.33304121868));
#133557=CARTESIAN_POINT('Ctrl Pts',(27.0338235509591,12.71200151814,90.14134599812));
#133558=CARTESIAN_POINT('Ctrl Pts',(28.2606989614091,11.55431815225,90.82076231519));
#133559=CARTESIAN_POINT('Ctrl Pts',(29.4805515038791,10.30341122855,91.41513380966));
#133560=CARTESIAN_POINT('Ctrl Pts',(30.7073346580191,8.91606547149402,91.92891446662));
#133561=CARTESIAN_POINT('Ctrl Pts',(31.8785519228191,7.42186252822301,92.33283454608));
#133562=CARTESIAN_POINT('Ctrl Pts',(32.8858034194691,5.93611159812901,92.60136415471));
#133563=CARTESIAN_POINT('Ctrl Pts',(33.7077479385191,4.49637949617201,92.75525280737));
#133564=CARTESIAN_POINT('Ctrl Pts',(34.3594477230791,3.06936714330901,92.82352537927));
#133565=CARTESIAN_POINT('Ctrl Pts',(34.7987841186091,1.68933111557601,92.83289655037));
#133566=CARTESIAN_POINT('Ctrl Pts',(34.9379185776691,0.799874261541514,
92.83329103801));
#133567=CARTESIAN_POINT('Ctrl Pts',(34.9680789093591,0.377412282680914,
92.8379453280101));
#133568=CARTESIAN_POINT('Ctrl Pts',(21.0648245475691,14.80356751578,75.088574197736));
#133569=CARTESIAN_POINT('Ctrl Pts',(21.1562893009191,14.80542149402,75.624814594272));
#133570=CARTESIAN_POINT('Ctrl Pts',(21.4915191590391,14.74994267437,76.949273101324));
#133571=CARTESIAN_POINT('Ctrl Pts',(22.4029329257891,14.43645292234,78.850401178621));
#133572=CARTESIAN_POINT('Ctrl Pts',(23.6728411634791,13.89196197301,80.525093828825));
#133573=CARTESIAN_POINT('Ctrl Pts',(24.9938756020691,13.25961078348,81.813737319686));
#133574=CARTESIAN_POINT('Ctrl Pts',(26.2936708744891,12.5864534242,82.832583999374));
#133575=CARTESIAN_POINT('Ctrl Pts',(27.5870975206191,11.86798256843,83.68225710374));
#133576=CARTESIAN_POINT('Ctrl Pts',(28.8717832775691,11.10303997034,84.4077907698501));
#133577=CARTESIAN_POINT('Ctrl Pts',(30.1179515221891,10.306293006,85.0241310085501));
#133578=CARTESIAN_POINT('Ctrl Pts',(31.3323143284891,9.47069299188402,85.55730149859));
#133579=CARTESIAN_POINT('Ctrl Pts',(32.5667384548491,8.55128051724301,86.04034306038));
#133580=CARTESIAN_POINT('Ctrl Pts',(33.8387497469191,7.50960072681501,86.47900335892));
#133581=CARTESIAN_POINT('Ctrl Pts',(35.0880429676691,6.35762147075602,86.85127259704));
#133582=CARTESIAN_POINT('Ctrl Pts',(36.1977391360291,5.17506491544101,87.13119140558));
#133583=CARTESIAN_POINT('Ctrl Pts',(37.1355508905091,3.98655984369701,87.32815521361));
#133584=CARTESIAN_POINT('Ctrl Pts',(37.9083300473991,2.75824145710901,87.46012871543));
#133585=CARTESIAN_POINT('Ctrl Pts',(38.4524854874891,1.51002426311401,87.5351100622101));
#133586=CARTESIAN_POINT('Ctrl Pts',(38.6303209632591,0.670091817760814,
87.56162468684));
#133587=CARTESIAN_POINT('Ctrl Pts',(38.6686985395891,0.267767345835414,
87.57156379687));
#133588=CARTESIAN_POINT('Ctrl Pts',(27.4060955579191,15.00605745049,73.9992175459301));
#133589=CARTESIAN_POINT('Ctrl Pts',(27.4568706345291,15.00674148237,74.299882608077));
#133590=CARTESIAN_POINT('Ctrl Pts',(27.6563153791591,14.98607407549,75.03933020766));
#133591=CARTESIAN_POINT('Ctrl Pts',(28.2552178354491,14.86384274642,76.157719195735));
#133592=CARTESIAN_POINT('Ctrl Pts',(29.1953897033191,14.62223845856,77.28144993045));
#133593=CARTESIAN_POINT('Ctrl Pts',(30.2745666151391,14.3009152899,78.274673456111));
#133594=CARTESIAN_POINT('Ctrl Pts',(31.4158151207291,13.9175608677,79.163166612491));
#133595=CARTESIAN_POINT('Ctrl Pts',(32.6169037455491,13.46553722345,79.992694706598));
#133596=CARTESIAN_POINT('Ctrl Pts',(33.8649399941491,12.93919476597,80.780446952018));
#133597=CARTESIAN_POINT('Ctrl Pts',(35.1214740837291,12.3447503952,81.5213409775531));
#133598=CARTESIAN_POINT('Ctrl Pts',(36.3853570661891,11.67360909312,82.229199358404));
#133599=CARTESIAN_POINT('Ctrl Pts',(37.7082882345091,10.88094645291,82.940678146904));
#133600=CARTESIAN_POINT('Ctrl Pts',(39.1142274982291,9.91205347783502,83.67127064968));
#133601=CARTESIAN_POINT('Ctrl Pts',(40.5432158335391,8.74576233655301,84.3936442258099));
#133602=CARTESIAN_POINT('Ctrl Pts',(41.8604028480391,7.43460302127903,85.0471196915701));
#133603=CARTESIAN_POINT('Ctrl Pts',(43.0163443071791,5.99020112655302,85.6153164434601));
#133604=CARTESIAN_POINT('Ctrl Pts',(44.0066134889891,4.35311312370201,86.1022978834));
#133605=CARTESIAN_POINT('Ctrl Pts',(44.7332634147991,2.52355184883601,86.4665423458501));
#133606=CARTESIAN_POINT('Ctrl Pts',(44.9781481988991,1.19967484028401,86.60065479763));
#133607=CARTESIAN_POINT('Ctrl Pts',(45.0312601718991,0.557056200456914,
86.6358961446099));
#133608=CARTESIAN_POINT('',(39.4126121040966,0.605802323126824,89.303174770965));
#133609=CARTESIAN_POINT('Origin',(46.4992391344146,1.66064392498492,96.9794802088298));
#133610=CARTESIAN_POINT('Ctrl Pts',(37.5050940990142,10.7061722565098,83.1298152725198));
#133611=CARTESIAN_POINT('Ctrl Pts',(37.552217423979,10.5471910708906,83.2904075500772));
#133612=CARTESIAN_POINT('Ctrl Pts',(37.599378677488,10.3862893955955,83.4509114661969));
#133613=CARTESIAN_POINT('Ctrl Pts',(37.6466151200992,10.2232847373308,83.6111957660706));
#133614=CARTESIAN_POINT('Ctrl Pts',(37.6923853029459,10.0653398837131,83.766504703559));
#133615=CARTESIAN_POINT('Ctrl Pts',(37.7382264410281,9.90542034687216,83.9216073065561));
#133616=CARTESIAN_POINT('Ctrl Pts',(37.7841362342735,9.74333882261691,84.0763598865346));
#133617=CARTESIAN_POINT('Ctrl Pts',(37.8126492894712,9.64267534493789,84.1724715991559));
#133618=CARTESIAN_POINT('Ctrl Pts',(37.8411880929764,9.54117752683905,84.2684478260362));
#133619=CARTESIAN_POINT('Ctrl Pts',(37.86974377233,9.43879676405171,84.3642495668624));
#133620=CARTESIAN_POINT('Ctrl Pts',(37.9139822359765,9.28018846772753,84.5126656411683));
#133621=CARTESIAN_POINT('Ctrl Pts',(37.9582636609881,9.11946131063388,84.6606639083057));
#133622=CARTESIAN_POINT('Ctrl Pts',(38.002495868906,8.95642861022755,84.8080614815933));
#133623=CARTESIAN_POINT('Ctrl Pts',(38.045356649548,8.79845076696536,84.950888967564));
#133624=CARTESIAN_POINT('Ctrl Pts',(38.0881714412079,8.63830788130787,85.093152305827));
#133625=CARTESIAN_POINT('Ctrl Pts',(38.1308108615095,8.47582372812318,85.2346675575267));
#133626=CARTESIAN_POINT('Ctrl Pts',(38.1419845864,8.43324450884893,85.2717518442998));
#133627=CARTESIAN_POINT('Ctrl Pts',(38.1531460090944,8.39050448870853,85.3087846687433));
#133628=CARTESIAN_POINT('Ctrl Pts',(38.1642922319669,8.34760045463328,85.3457625296133));
#133629=CARTESIAN_POINT('Ctrl Pts',(38.2000540816169,8.20994596543751,85.4644033208424));
#133630=CARTESIAN_POINT('Ctrl Pts',(38.2356900159584,8.07059403849077,85.5824775687261));
#133631=CARTESIAN_POINT('Ctrl Pts',(38.2712115945426,7.92939023146871,85.6998388074438));
#133632=CARTESIAN_POINT('Ctrl Pts',(38.3077375849418,7.78419373105429,85.8205185646365));
#133633=CARTESIAN_POINT('Ctrl Pts',(38.3441432944549,7.63703875702918,85.9404442433346));
#133634=CARTESIAN_POINT('Ctrl Pts',(38.3803739820712,7.48776076653468,86.0594246406868));
#133635=CARTESIAN_POINT('Ctrl Pts',(38.4166046696875,7.33848277604017,86.1784050380389));
#133636=CARTESIAN_POINT('Ctrl Pts',(38.4526608349029,7.18708149166657,86.2964401025204));
#133637=CARTESIAN_POINT('Ctrl Pts',(38.4884369449348,7.03338765491548,86.4133197013914));
#133638=CARTESIAN_POINT('Ctrl Pts',(38.5205640696361,6.89536982528776,86.5182781623482));
#133639=CARTESIAN_POINT('Ctrl Pts',(38.5524923683579,6.75549952963279,86.6222935863113));
#133640=CARTESIAN_POINT('Ctrl Pts',(38.5841939839849,6.61362336899418,86.7251659839855));
#133641=CARTESIAN_POINT('Ctrl Pts',(38.5988420549672,6.54806796966731,86.7726992769566));
#133642=CARTESIAN_POINT('Ctrl Pts',(38.6134410812288,6.48208423576418,86.8199882613318));
#133643=CARTESIAN_POINT('Ctrl Pts',(38.6279847854992,6.41565671969214,86.8670118300703));
#133644=CARTESIAN_POINT('Ctrl Pts',(38.6340595331057,6.38791066636475,86.8866530649533));
#133645=CARTESIAN_POINT('Ctrl Pts',(38.6401246006179,6.36008718736758,86.9062479834196));
#133646=CARTESIAN_POINT('Ctrl Pts',(38.646179288585,6.33218524996709,86.9257950052816));
#133647=CARTESIAN_POINT('Ctrl Pts',(38.6721403751459,6.21254826520258,87.0096080653973));
#133648=CARTESIAN_POINT('Ctrl Pts',(38.6979186362708,6.09146585004635,87.092540259136));
#133649=CARTESIAN_POINT('Ctrl Pts',(38.7234769891415,5.96883836752666,87.1744532102944));
#133650=CARTESIAN_POINT('Ctrl Pts',(38.7362561655769,5.90752462626682,87.2154096858736));
#133651=CARTESIAN_POINT('Ctrl Pts',(38.7489802003326,5.8458244661527,87.2561111365291));
#133652=CARTESIAN_POINT('Ctrl Pts',(38.7616433871205,5.78372476399081,87.2965386867928));
#133653=CARTESIAN_POINT('Ctrl Pts',(38.7679749805145,5.75267491290986,87.3167524619246));
#133654=CARTESIAN_POINT('Ctrl Pts',(38.7742913485755,5.72152516801141,87.3368977468268));
#133655=CARTESIAN_POINT('Ctrl Pts',(38.7805917707051,5.69027391197471,87.3569719794879));
#133656=CARTESIAN_POINT('Ctrl Pts',(38.7837419817699,5.67464828395636,87.3670090958184));
#133657=CARTESIAN_POINT('Ctrl Pts',(38.7868882053342,5.6589972777635,87.3770284480717));
#133658=CARTESIAN_POINT('Ctrl Pts',(38.7900304108563,5.64332074742208,87.387029619085));
#133659=CARTESIAN_POINT('Ctrl Pts',(38.7916015136173,5.63548248225137,87.3920302045916));
#133660=CARTESIAN_POINT('Ctrl Pts',(38.793171611861,5.62763783596085,87.3970262447299));
#133661=CARTESIAN_POINT('Ctrl Pts',(38.7947406975676,5.61978678615472,87.4020176927));
#133662=CARTESIAN_POINT('Ctrl Pts',(38.7963097832741,5.61193573634858,87.4070091406701));
#133663=CARTESIAN_POINT('Ctrl Pts',(38.7976672957473,5.60513493051777,87.4113265501283));
#133664=CARTESIAN_POINT('Ctrl Pts',(38.7994449103682,5.59621440491363,87.4169782110083));
#133665=CARTESIAN_POINT('Ctrl Pts',(38.8268161624268,5.4588584493859,87.5040010294981));
#133666=CARTESIAN_POINT('Ctrl Pts',(38.8527567462118,5.32506777322639,87.5861152448737));
#133667=CARTESIAN_POINT('Ctrl Pts',(38.8772743032886,5.19511788675176,87.6635181014004));
#133668=CARTESIAN_POINT('Ctrl Pts',(38.8897280675518,5.12910946482259,87.7028351069842));
#133669=CARTESIAN_POINT('Ctrl Pts',(38.9018154030616,5.06409193786023,87.7409370043211));
#133670=CARTESIAN_POINT('Ctrl Pts',(38.9135415606847,5.00010079004935,87.7778523004227));
#133671=CARTESIAN_POINT('Ctrl Pts',(38.9380151229955,4.86654541806606,87.8548978961243));
#133672=CARTESIAN_POINT('Ctrl Pts',(38.9609123280281,4.73746215436914,87.9267734403203));
#133673=CARTESIAN_POINT('Ctrl Pts',(38.9823131061757,4.61317397417699,87.9937636561146));
#133674=CARTESIAN_POINT('Ctrl Pts',(39.0061356217478,4.4748211961784,88.0683345641409));
#133675=CARTESIAN_POINT('Ctrl Pts',(39.0281041862561,4.34241024754061,88.1368526571142));
#133676=CARTESIAN_POINT('Ctrl Pts',(39.0483876372309,4.21636440778313,88.1997316609947));
#133677=CARTESIAN_POINT('Ctrl Pts',(39.0554044509918,4.17276037886256,88.2214838894616));
#133678=CARTESIAN_POINT('Ctrl Pts',(39.0622200434846,4.12991789653019,88.2425613851375));
#133679=CARTESIAN_POINT('Ctrl Pts',(39.0688426197856,4.08785393259761,88.2629815187296));
#133680=CARTESIAN_POINT('Ctrl Pts',(39.0918493621927,3.94172427869416,88.3339207925283));
#133681=CARTESIAN_POINT('Ctrl Pts',(39.1124319604812,3.80500972636446,88.3969883469281));
#133682=CARTESIAN_POINT('Ctrl Pts',(39.1307949414565,3.67849151113324,88.4530154364568));
#133683=CARTESIAN_POINT('Ctrl Pts',(39.1384490160761,3.6257560722948,88.4763686994453));
#133684=CARTESIAN_POINT('Ctrl Pts',(39.1457180528506,3.57479184947902,88.4984987120231));
#133685=CARTESIAN_POINT('Ctrl Pts',(39.1526181182454,3.52565431267108,88.519464946207));
#133686=CARTESIAN_POINT('Ctrl Pts',(39.153421600476,3.51993246288875,88.5219063718521));
#133687=CARTESIAN_POINT('Ctrl Pts',(39.1542200793681,3.51423538159438,88.5243320162628));
#133688=CARTESIAN_POINT('Ctrl Pts',(39.1550135811842,3.50856315513645,88.5267419732416));
#133689=CARTESIAN_POINT('Ctrl Pts',(39.1669917121232,3.42293931679378,88.563120945114));
#133690=CARTESIAN_POINT('Ctrl Pts',(39.1778340435463,3.34297408472003,88.5959321303305));
#133691=CARTESIAN_POINT('Ctrl Pts',(39.1876199347076,3.26891537418542,88.6255169987751));
#133692=CARTESIAN_POINT('Ctrl Pts',(39.1925128802883,3.23188601891811,88.6403094329974));
#133693=CARTESIAN_POINT('Ctrl Pts',(39.1971416061376,3.19633263902273,88.6542952132579));
#133694=CARTESIAN_POINT('Ctrl Pts',(39.2015152946873,3.16228236620596,88.6675157076164));
#133695=CARTESIAN_POINT('Ctrl Pts',(39.2037021389622,3.14525722979757,88.6741259547957));
#133696=CARTESIAN_POINT('Ctrl Pts',(39.2058252034364,3.1286078582077,88.680544856444));
#133697=CARTESIAN_POINT('Ctrl Pts',(39.2078855970158,3.11233737620093,88.686777438232));
#133698=CARTESIAN_POINT('Ctrl Pts',(39.2089157938054,3.10420213519754,88.6898937291259));
#133699=CARTESIAN_POINT('Ctrl Pts',(39.2099303213754,3.09616161571765,88.6929634382969));
#133700=CARTESIAN_POINT('Ctrl Pts',(39.2109293128743,3.08821619883033,88.6959871818242));
#133701=CARTESIAN_POINT('Ctrl Pts',(39.2114288086237,3.08424349038668,88.6974990535879));
#133702=CARTESIAN_POINT('Ctrl Pts',(39.2119244202558,3.08029455753482,88.6989994338242));
#133703=CARTESIAN_POINT('Ctrl Pts',(39.2124161641733,3.07636944696151,88.7004883988127));
#133704=CARTESIAN_POINT('Ctrl Pts',(39.2126620361321,3.07440689167485,88.7012328813069));
#133705=CARTESIAN_POINT('Ctrl Pts',(39.2129069411559,3.07245029195421,88.7019745099817));
#133706=CARTESIAN_POINT('Ctrl Pts',(39.2131508812819,3.07049965357541,88.7027132943232));
#133707=CARTESIAN_POINT('Ctrl Pts',(39.2133948214078,3.0685490151966,88.7034520786646));
#133708=CARTESIAN_POINT('Ctrl Pts',(39.2134400757702,3.0681882383282,88.7035890815634));
#133709=CARTESIAN_POINT('Ctrl Pts',(39.2138798089855,3.06466562821442,88.7049211238016));
#133710=CARTESIAN_POINT('Ctrl Pts',(39.2310447207238,2.9271611377798,88.756917167442));
#133711=CARTESIAN_POINT('Ctrl Pts',(39.247089602519,2.79108612147949,88.8053255292509));
#133712=CARTESIAN_POINT('Ctrl Pts',(39.2619938081742,2.65665221882818,88.8502537192043));
#133713=CARTESIAN_POINT('Ctrl Pts',(39.2771796828001,2.51967770046989,88.8960309901025));
#133714=CARTESIAN_POINT('Ctrl Pts',(39.2911813148946,2.38440688037919,88.9381956585786));
#133715=CARTESIAN_POINT('Ctrl Pts',(39.3040289835558,2.25105544495463,88.9768759642758));
#133716=CARTESIAN_POINT('Ctrl Pts',(39.3154345014117,2.13267270813758,89.011214405664));
#133717=CARTESIAN_POINT('Ctrl Pts',(39.3259313823954,2.01580250615974,89.0428071815956));
#133718=CARTESIAN_POINT('Ctrl Pts',(39.335574287149,1.90059075916109,89.0717500576461));
#133719=CARTESIAN_POINT('Ctrl Pts',(39.3393662685198,1.85528482599282,89.0831315707487));
#133720=CARTESIAN_POINT('Ctrl Pts',(39.3430265391906,1.81023531083248,89.0941033538999));
#133721=CARTESIAN_POINT('Ctrl Pts',(39.3465613453223,1.76545096114672,89.1046710760339));
#133722=CARTESIAN_POINT('Ctrl Pts',(39.3572631219915,1.62986442803529,89.1366653065426));
#133723=CARTESIAN_POINT('Ctrl Pts',(39.366770729011,1.49685015350463,89.1649482792311));
#133724=CARTESIAN_POINT('Ctrl Pts',(39.3751201764905,1.36667079983074,89.1898546186758));
#133725=CARTESIAN_POINT('Ctrl Pts',(39.3837779490806,1.2316842342166,89.2156806896215));
#133726=CARTESIAN_POINT('Ctrl Pts',(39.3911904902059,1.0997455921959,89.2378764788459));
#133727=CARTESIAN_POINT('Ctrl Pts',(39.3974554150243,0.971144094561306,
89.2568175177896));
#133728=CARTESIAN_POINT('Ctrl Pts',(39.4035460066799,0.846121172323219,
89.2752314871642));
#133729=CARTESIAN_POINT('Ctrl Pts',(39.4085526120063,0.724252072113412,
89.2905695595766));
#133730=CARTESIAN_POINT('Ctrl Pts',(39.4126121040966,0.605802323126824,
89.303174770965));
#133731=CARTESIAN_POINT('Ctrl Pts',(38.4618783725391,10.5104216086,82.548487971909));
#133732=CARTESIAN_POINT('Ctrl Pts',(38.5526802105791,10.01289241835,83.06345078517));
#133733=CARTESIAN_POINT('Ctrl Pts',(38.7398454136791,8.95695275023301,84.12491739878));
#133734=CARTESIAN_POINT('Ctrl Pts',(39.0045880266591,7.31849282792101,85.62634736661));
#133735=CARTESIAN_POINT('Ctrl Pts',(39.2417436224691,5.61044727625601,86.9713235856));
#133736=CARTESIAN_POINT('Ctrl Pts',(39.4296302152491,3.90871748337901,88.0368814033801));
#133737=CARTESIAN_POINT('Ctrl Pts',(39.5601688728291,2.20504120005801,88.77720291884));
#133738=CARTESIAN_POINT('Ctrl Pts',(39.6063198374691,1.00828919109001,89.0389380455399));
#133739=CARTESIAN_POINT('Ctrl Pts',(39.6165263283691,0.422474636108614,
89.0968219318599));
#133740=CARTESIAN_POINT('Ctrl Pts',(39.6168726794091,0.401711040790814,
89.09878618618));
#133741=CARTESIAN_POINT('Ctrl Pts',(37.3374165872391,11.41764504428,83.62342900089));
#133742=CARTESIAN_POINT('Ctrl Pts',(37.4297627814791,10.91166281239,84.1471502934));
#133743=CARTESIAN_POINT('Ctrl Pts',(37.6207808413991,9.83411841866803,85.2304675438201));
#133744=CARTESIAN_POINT('Ctrl Pts',(37.8940999251891,8.14335594153101,86.7805370947));
#133745=CARTESIAN_POINT('Ctrl Pts',(38.1435439664991,6.34856195272902,88.1952045512));
#133746=CARTESIAN_POINT('Ctrl Pts',(38.3465988703891,4.51349428134101,89.3467861359801));
#133747=CARTESIAN_POINT('Ctrl Pts',(38.4930032378491,2.61111516505002,90.1770865634601));
#133748=CARTESIAN_POINT('Ctrl Pts',(38.5466699117291,1.22869486492401,90.48144539536));
#133749=CARTESIAN_POINT('Ctrl Pts',(38.5585559689691,0.546009918402814,
90.54885457573));
#133750=CARTESIAN_POINT('Ctrl Pts',(38.5589593261391,0.521805644301214,
90.5511421279301));
#133751=CARTESIAN_POINT('Ctrl Pts',(35.6787452111791,10.79042214836,83.3097995382401));
#133752=CARTESIAN_POINT('Ctrl Pts',(35.7700236909691,10.29028405701,83.82746552121));
#133753=CARTESIAN_POINT('Ctrl Pts',(35.9583780189791,9.22767642310003,84.8956759973201));
#133754=CARTESIAN_POINT('Ctrl Pts',(36.2257676275791,7.57307412284002,86.41211782328));
#133755=CARTESIAN_POINT('Ctrl Pts',(36.4667158628191,5.83825500221001,87.77860316929));
#133756=CARTESIAN_POINT('Ctrl Pts',(36.6592839211891,4.09537252689102,88.8707108977601));
#133757=CARTESIAN_POINT('Ctrl Pts',(36.7947192857491,2.33036967472801,89.6388030185));
#133758=CARTESIAN_POINT('Ctrl Pts',(36.8431898582791,1.07631400748201,89.91369329529));
#133759=CARTESIAN_POINT('Ctrl Pts',(36.8539147214691,0.460601898215214,
89.9745170169101));
#133760=CARTESIAN_POINT('Ctrl Pts',(36.8542786665691,0.438776390386414,
89.9765810521401));
#133761=CARTESIAN_POINT('Ctrl Pts',(35.8222578729191,9.51225498089002,82.0493759893619));
#133762=CARTESIAN_POINT('Ctrl Pts',(35.9113605431891,9.02402619420501,82.554702343344));
#133763=CARTESIAN_POINT('Ctrl Pts',(36.0942866658791,7.99185698356001,83.59212793729));
#133764=CARTESIAN_POINT('Ctrl Pts',(36.3495930731491,6.41094260374401,85.04004252327));
#133765=CARTESIAN_POINT('Ctrl Pts',(36.5732283875091,4.79834145039201,86.30834141581));
#133766=CARTESIAN_POINT('Ctrl Pts',(36.7444261455991,3.24331578276701,87.2792521488301));
#133767=CARTESIAN_POINT('Ctrl Pts',(36.8575086600591,1.75826098661201,87.9205749571999));
#133768=CARTESIAN_POINT('Ctrl Pts',(36.8953905149491,0.765789295776714,
88.13541363216));
#133769=CARTESIAN_POINT('Ctrl Pts',(36.9037490740191,0.286555752975114,
88.1828173762601));
#133770=CARTESIAN_POINT('Ctrl Pts',(36.9040327044291,0.269577741895514,
88.1844259242101));
#133771=CARTESIAN_POINT('',(36.9231015705691,0.454612543733214,88.46713451361));
#133772=CARTESIAN_POINT('Ctrl Pts',(39.4126046545741,0.605801203662559,
89.3031667019448));
#133773=CARTESIAN_POINT('Ctrl Pts',(39.3831045186586,0.60835665082592,89.3300482189441));
#133774=CARTESIAN_POINT('Ctrl Pts',(39.3518228481273,0.610817150309038,
89.3563993223594));
#133775=CARTESIAN_POINT('Ctrl Pts',(39.3187170774961,0.613149296867715,
89.3819539330426));
#133776=CARTESIAN_POINT('Ctrl Pts',(39.286414762165,0.61542484376182,89.406888350116));
#133777=CARTESIAN_POINT('Ctrl Pts',(39.2523752998365,0.617578123298112,
89.4310639775319));
#133778=CARTESIAN_POINT('Ctrl Pts',(39.216600896201,0.619575784801966,89.4542071436158));
#133779=CARTESIAN_POINT('Ctrl Pts',(39.181989572322,0.621508499320843,89.476597890505));
#133780=CARTESIAN_POINT('Ctrl Pts',(39.1457539831398,0.623295470029379,
89.4980216010856));
#133781=CARTESIAN_POINT('Ctrl Pts',(39.1079414762182,0.62490538503978,89.5182134310987));
#133782=CARTESIAN_POINT('Ctrl Pts',(39.0707821876153,0.626487488459201,
89.5380564433706));
#133783=CARTESIAN_POINT('Ctrl Pts',(39.0320997293332,0.627898515182738,
89.5567091000904));
#133784=CARTESIAN_POINT('Ctrl Pts',(38.9919878848528,0.62910886732803,89.573912709109));
#133785=CARTESIAN_POINT('Ctrl Pts',(38.9528180544733,0.630290794732382,
89.5907122967595));
#133786=CARTESIAN_POINT('Ctrl Pts',(38.9122851561905,0.631281276339598,
89.6061293842026));
#133787=CARTESIAN_POINT('Ctrl Pts',(38.8705255806283,0.632054124925481,
89.6199261912394));
#133788=CARTESIAN_POINT('Ctrl Pts',(38.8369824924627,0.632674910168289,
89.6310083803806));
#133789=CARTESIAN_POINT('Ctrl Pts',(38.8026488932324,0.633155284016311,
89.6410450494364));
#133790=CARTESIAN_POINT('Ctrl Pts',(38.7676190350803,0.633482926508632,
89.6499194058903));
#133791=CARTESIAN_POINT('Ctrl Pts',(38.7252106504547,0.633879582092383,
89.6606630155324));
#133792=CARTESIAN_POINT('Ctrl Pts',(38.6817806079962,0.634052293748719,
89.6697019627361));
#133793=CARTESIAN_POINT('Ctrl Pts',(38.6375365916026,0.633983196901231,
89.6768494372612));
#133794=CARTESIAN_POINT('Ctrl Pts',(38.5938457079763,0.633914963893276,
89.6839075550171));
#133795=CARTESIAN_POINT('Ctrl Pts',(38.5493614881786,0.633610864087447,
89.6891205653363));
#133796=CARTESIAN_POINT('Ctrl Pts',(38.504323097568,0.633058259373022,89.6923400995111));
#133797=CARTESIAN_POINT('Ctrl Pts',(38.4597464968879,0.632511320653523,
89.6955266229935));
#133798=CARTESIAN_POINT('Ctrl Pts',(38.4146275926837,0.631720896463281,
89.6967598172212));
#133799=CARTESIAN_POINT('Ctrl Pts',(38.3692296616835,0.630680106018952,
89.6959355169049));
#133800=CARTESIAN_POINT('Ctrl Pts',(38.3241942624029,0.629647626956688,
89.6951177991576));
#133801=CARTESIAN_POINT('Ctrl Pts',(38.278884954633,0.628368733852932,89.6922749404782));
#133802=CARTESIAN_POINT('Ctrl Pts',(38.2335805705822,0.626842630152893,
89.6873512332037));
#133803=CARTESIAN_POINT('Ctrl Pts',(38.1885345620774,0.625325229978679,
89.6824556063364));
#133804=CARTESIAN_POINT('Ctrl Pts',(38.1434941789864,0.623563422769541,
89.6755025961845));
#133805=CARTESIAN_POINT('Ctrl Pts',(38.0987444207698,0.621562594626665,
89.6664874308702));
#133806=CARTESIAN_POINT('Ctrl Pts',(38.0541334199269,0.619567970532022,
89.6575002192412));
#133807=CARTESIAN_POINT('Ctrl Pts',(38.0098120340049,0.617335820360408,
89.6464636073945));
#133808=CARTESIAN_POINT('Ctrl Pts',(37.9660618899869,0.614877582249971,
89.6334243368702));
#133809=CARTESIAN_POINT('Ctrl Pts',(37.9223233221598,0.61241999458387,89.620388516508));
#133810=CARTESIAN_POINT('Ctrl Pts',(37.8791564685519,0.609736475757642,
89.6053512735637));
#133811=CARTESIAN_POINT('Ctrl Pts',(37.8368302231893,0.606844175965338,
89.5884096475916));
#133812=CARTESIAN_POINT('Ctrl Pts',(37.7944288784365,0.60394674437009,89.5714379621194));
#133813=CARTESIAN_POINT('Ctrl Pts',(37.7528718357621,0.600839848338323,
89.5525554938259));
#133814=CARTESIAN_POINT('Ctrl Pts',(37.7124056615877,0.597545755861513,
89.5319062665894));
#133815=CARTESIAN_POINT('Ctrl Pts',(37.6717851806981,0.594239102261745,
89.5111782991584));
#133816=CARTESIAN_POINT('Ctrl Pts',(37.6322644978623,0.590743897019806,
89.4886706010158));
#133817=CARTESIAN_POINT('Ctrl Pts',(37.5940592138503,0.587086718114105,
89.4645689017616));
#133818=CARTESIAN_POINT('Ctrl Pts',(37.5554338119455,0.583389323663991,
89.44020217228));
#133819=CARTESIAN_POINT('Ctrl Pts',(37.5181533823027,0.579526460037029,
89.4142068334793));
#133820=CARTESIAN_POINT('Ctrl Pts',(37.4823979404021,0.575528505140439,
89.3868068410641));
#133821=CARTESIAN_POINT('Ctrl Pts',(37.4463906011989,0.571502384627633,
89.3592138155382));
#133822=CARTESIAN_POINT('Ctrl Pts',(37.4119300728137,0.567339358331094,
89.3301970339475));
#133823=CARTESIAN_POINT('Ctrl Pts',(37.3791514117944,0.563071999857544,
89.3000068278654));
#133824=CARTESIAN_POINT('Ctrl Pts',(37.3458646911807,0.558738498584144,
89.2693486824783));
#133825=CARTESIAN_POINT('Ctrl Pts',(37.3143124981168,0.554297502710505,
89.2374812493819));
#133826=CARTESIAN_POINT('Ctrl Pts',(37.2845831075364,0.549783244820651,
89.2046770404806));
#133827=CARTESIAN_POINT('Ctrl Pts',(37.2627034046058,0.54646092237631,89.1805343879869));
#133828=CARTESIAN_POINT('Ctrl Pts',(37.24180985427,0.543098924907988,89.1558845980402));
#133829=CARTESIAN_POINT('Ctrl Pts',(37.2219196441713,0.539710495501798,
89.1308360746835));
#133830=CARTESIAN_POINT('Ctrl Pts',(37.1941781887475,0.534984554304494,
89.0959001694978));
#133831=CARTESIAN_POINT('Ctrl Pts',(37.1683903997965,0.530207421110298,
89.0601895405553));
#133832=CARTESIAN_POINT('Ctrl Pts',(37.14455706585,0.52541249504094,89.0239885723349));
#133833=CARTESIAN_POINT('Ctrl Pts',(37.1203265038489,0.520537652365768,
88.9871842458008));
#133834=CARTESIAN_POINT('Ctrl Pts',(37.0981156574704,0.515644488939498,
88.9498737657369));
#133835=CARTESIAN_POINT('Ctrl Pts',(37.0778757845561,0.510764523307869,
88.912334325911));
#133836=CARTESIAN_POINT('Ctrl Pts',(37.0570110825334,0.505733907294808,
88.8736359986347));
#133837=CARTESIAN_POINT('Ctrl Pts',(37.0382404193393,0.500717379709185,
88.8346949775485));
#133838=CARTESIAN_POINT('Ctrl Pts',(37.0214652583305,0.495744645027273,
88.7957820015511));
#133839=CARTESIAN_POINT('Ctrl Pts',(37.0043895620494,0.490682821354183,
88.756171880422));
#133840=CARTESIAN_POINT('Ctrl Pts',(36.9893807934452,0.485666403661524,
88.7165911940317));
#133841=CARTESIAN_POINT('Ctrl Pts',(36.9762985638914,0.480721090680712,
88.6772842583823));
#133842=CARTESIAN_POINT('Ctrl Pts',(36.9627909027976,0.475614957091374,
88.6366990688923));
#133843=CARTESIAN_POINT('Ctrl Pts',(36.9513363870551,0.470584648266651,
88.5964060215216));
#133844=CARTESIAN_POINT('Ctrl Pts',(36.9417531125328,0.465652089719945,
88.5566250685652));
#133845=CARTESIAN_POINT('Ctrl Pts',(36.934490203723,0.461913834821746,88.5264761426404));
#133846=CARTESIAN_POINT('Ctrl Pts',(36.9283014467381,0.458231586758951,
88.4966202929128));
#133847=CARTESIAN_POINT('Ctrl Pts',(36.9231015707506,0.454612543733214,
88.467134513578));
#133848=CARTESIAN_POINT('',(35.848006166586,9.6214649594803,82.3699654947659));
#133849=CARTESIAN_POINT('Ctrl Pts',(35.8480061888895,9.62146509318402,82.3699656206012));
#133850=CARTESIAN_POINT('Ctrl Pts',(35.8840711939915,9.42298356395101,82.574500428362));
#133851=CARTESIAN_POINT('Ctrl Pts',(35.9193837200317,9.22621999154996,82.774767717099));
#133852=CARTESIAN_POINT('Ctrl Pts',(35.9539203620774,9.03104931189124,82.9706347473929));
#133853=CARTESIAN_POINT('Ctrl Pts',(35.9894216077162,8.83042754238368,83.1719723165117));
#133854=CARTESIAN_POINT('Ctrl Pts',(36.0241030425718,8.63148893673031,83.3686605057258));
#133855=CARTESIAN_POINT('Ctrl Pts',(36.0579470929178,8.43412917023835,83.5605996528873));
#133856=CARTESIAN_POINT('Ctrl Pts',(36.0693471268102,8.36765048331987,83.625252457754));
#133857=CARTESIAN_POINT('Ctrl Pts',(36.0806522129673,8.30135118823686,83.6893667874641));
#133858=CARTESIAN_POINT('Ctrl Pts',(36.0918618660515,8.23522805483293,83.7529398895296));
#133859=CARTESIAN_POINT('Ctrl Pts',(36.1080946788707,8.13947447178146,83.8450007462238));
#133860=CARTESIAN_POINT('Ctrl Pts',(36.1241273207524,8.04409016349334,83.9359263777126));
#133861=CARTESIAN_POINT('Ctrl Pts',(36.1399548504375,7.94905716829722,84.0256887590647));
#133862=CARTESIAN_POINT('Ctrl Pts',(36.1699269360555,7.76909623154801,84.1956689033256));
#133863=CARTESIAN_POINT('Ctrl Pts',(36.1991722019866,7.59041721187683,84.361527047438));
#133864=CARTESIAN_POINT('Ctrl Pts',(36.2276690111892,7.41287080158735,84.5231404839857));
#133865=CARTESIAN_POINT('Ctrl Pts',(36.2573201523836,7.22813244570188,84.6913004625973));
#133866=CARTESIAN_POINT('Ctrl Pts',(36.2861609991746,7.04462034885526,84.8548650311814));
#133867=CARTESIAN_POINT('Ctrl Pts',(36.3141757533437,6.86219513928813,85.0137445959195));
#133868=CARTESIAN_POINT('Ctrl Pts',(36.3306688043748,6.75479643528424,85.1072813356391));
#133869=CARTESIAN_POINT('Ctrl Pts',(36.3468756902773,6.647774982912,85.1991951530901));
#133870=CARTESIAN_POINT('Ctrl Pts',(36.3627944292351,6.54110664613089,85.2894748091241));
#133871=CARTESIAN_POINT('Ctrl Pts',(36.3725512678293,6.47572799096003,85.3448085911901));
#133872=CARTESIAN_POINT('Ctrl Pts',(36.3821998662822,6.41048203844461,85.3995285133107));
#133873=CARTESIAN_POINT('Ctrl Pts',(36.3917380100775,6.34536180651616,85.4536220148097));
#133874=CARTESIAN_POINT('Ctrl Pts',(36.4151586647637,6.1854608343972,85.5864471479344));
#133875=CARTESIAN_POINT('Ctrl Pts',(36.4379238621124,6.02632755772767,85.7155549932985));
#133876=CARTESIAN_POINT('Ctrl Pts',(36.4600028935504,5.86790369704439,85.8407714030872));
#133877=CARTESIAN_POINT('Ctrl Pts',(36.4827582420661,5.70462705272387,85.9698233976288));
#133878=CARTESIAN_POINT('Ctrl Pts',(36.5047847585164,5.54210395707846,86.0947419824114));
#133879=CARTESIAN_POINT('Ctrl Pts',(36.5260579787218,5.38029126230337,86.2153884103457));
#133880=CARTESIAN_POINT('Ctrl Pts',(36.5469684503834,5.22123777929047,86.3339775890421));
#133881=CARTESIAN_POINT('Ctrl Pts',(36.5671511750975,5.06287082270039,86.4484395084244));
#133882=CARTESIAN_POINT('Ctrl Pts',(36.5865908243859,4.90516767849405,86.5586872380554));
#133883=CARTESIAN_POINT('Ctrl Pts',(36.5912217730954,4.86759934784603,86.5849506532892));
#133884=CARTESIAN_POINT('Ctrl Pts',(36.5958105837709,4.83006876709066,86.6109750918747));
#133885=CARTESIAN_POINT('Ctrl Pts',(36.6003566184185,4.79257619115534,86.6367569355226));
#133886=CARTESIAN_POINT('Ctrl Pts',(36.6182300293975,4.64516855564193,86.7381220862625));
#133887=CARTESIAN_POINT('Ctrl Pts',(36.6354503671782,4.49833567642529,86.8357834752628));
#133888=CARTESIAN_POINT('Ctrl Pts',(36.6519849745124,4.35208529549298,86.9295558923853));
#133889=CARTESIAN_POINT('Ctrl Pts',(36.6688419771116,4.20298329375253,87.0251567038968));
#133890=CARTESIAN_POINT('Ctrl Pts',(36.6849862825463,4.05448672669592,87.1167156064538));
#133891=CARTESIAN_POINT('Ctrl Pts',(36.7003927145458,3.90661167622958,87.204089821805));
#133892=CARTESIAN_POINT('Ctrl Pts',(36.7162531253124,3.75437921626744,87.294038678615));
#133893=CARTESIAN_POINT('Ctrl Pts',(36.7313315593775,3.6028054167375,87.3795527288836));
#133894=CARTESIAN_POINT('Ctrl Pts',(36.7456100178923,3.45191629917935,87.4605298956186));
#133895=CARTESIAN_POINT('Ctrl Pts',(36.7498735780939,3.40686067669738,87.4847097484345));
#133896=CARTESIAN_POINT('Ctrl Pts',(36.7540658716536,3.36186615950828,87.5084854281124));
#133897=CARTESIAN_POINT('Ctrl Pts',(36.7581865714518,3.31693358625967,87.5318550785251));
#133898=CARTESIAN_POINT('Ctrl Pts',(36.7592349768714,3.30550165585511,87.5378008812641));
#133899=CARTESIAN_POINT('Ctrl Pts',(36.7602787482342,3.29407373556857,87.5437204029012));
#133900=CARTESIAN_POINT('Ctrl Pts',(36.7613178686119,3.28264988434538,87.5496135474077));
#133901=CARTESIAN_POINT('Ctrl Pts',(36.7730845101796,3.15329012435176,87.616345487808));
#133902=CARTESIAN_POINT('Ctrl Pts',(36.7842599602964,3.0244358430859,87.6797246024727));
#133903=CARTESIAN_POINT('Ctrl Pts',(36.7948211288705,2.89624577466549,87.7396199479668));
#133904=CARTESIAN_POINT('Ctrl Pts',(36.805436243692,2.76740091382348,87.7998212377418));
#133905=CARTESIAN_POINT('Ctrl Pts',(36.815430793198,2.63922710560392,87.8565031226065));
#133906=CARTESIAN_POINT('Ctrl Pts',(36.8247905074935,2.51188131067207,87.9095846926443));
#133907=CARTESIAN_POINT('Ctrl Pts',(36.8342534255052,2.38313135329914,87.9632515599587));
#133908=CARTESIAN_POINT('Ctrl Pts',(36.8430674352554,2.25522781027107,88.0132383038302));
#133909=CARTESIAN_POINT('Ctrl Pts',(36.8512270697234,2.12832799735421,88.0595139153293));
#133910=CARTESIAN_POINT('Ctrl Pts',(36.8577570806654,2.02677232471509,88.0965474675826));
#133911=CARTESIAN_POINT('Ctrl Pts',(36.8638681804114,1.92585940324179,88.1312052663135));
#133912=CARTESIAN_POINT('Ctrl Pts',(36.8695617213592,1.82566739860244,88.1634949415812));
#133913=CARTESIAN_POINT('Ctrl Pts',(36.8702935771886,1.81278857620878,88.1676455022413));
#133914=CARTESIAN_POINT('Ctrl Pts',(36.8710183827158,1.79992141933469,88.1717560780887));
#133915=CARTESIAN_POINT('Ctrl Pts',(36.871736162201,1.78706580880341,88.175826806872));
#133916=CARTESIAN_POINT('Ctrl Pts',(36.8790227325904,1.65656150634758,88.2171509912854));
#133917=CARTESIAN_POINT('Ctrl Pts',(36.8855855249633,1.52725131520177,88.254370399929));
#133918=CARTESIAN_POINT('Ctrl Pts',(36.8914577225618,1.39914210405543,88.2876732807));
#133919=CARTESIAN_POINT('Ctrl Pts',(36.8974061744229,1.26936931240779,88.3214086207968));
#133920=CARTESIAN_POINT('Ctrl Pts',(36.9026460801669,1.14082839355656,88.351125616774));
#133921=CARTESIAN_POINT('Ctrl Pts',(36.9072075243119,1.01347890114135,88.3769948657369));
#133922=CARTESIAN_POINT('Ctrl Pts',(36.9117999441885,0.885264607236343,
88.4030397868963));
#133923=CARTESIAN_POINT('Ctrl Pts',(36.9157047485802,0.758257457362063,
88.4251850441213));
#133924=CARTESIAN_POINT('Ctrl Pts',(36.9189467463333,0.632376055362981,
88.443571330873));
#133925=CARTESIAN_POINT('Ctrl Pts',(36.9204791775988,0.572874287978069,
88.4522621822617));
#133926=CARTESIAN_POINT('Ctrl Pts',(36.9218634261454,0.513623514599076,
88.4601126465874));
#133927=CARTESIAN_POINT('Ctrl Pts',(36.9231015707506,0.454612543733215,
88.467134513578));
#133928=CARTESIAN_POINT('Ctrl Pts',(37.5050981553872,10.7062004821443,83.1298391922139));
#133929=CARTESIAN_POINT('Ctrl Pts',(37.4486493927448,10.7060934330738,83.1399044895495));
#133930=CARTESIAN_POINT('Ctrl Pts',(37.3917867645175,10.7036375396935,83.1477000261519));
#133931=CARTESIAN_POINT('Ctrl Pts',(37.334903968502,10.6988391558546,83.1531809198935));
#133932=CARTESIAN_POINT('Ctrl Pts',(37.2762089392287,10.6938878999457,83.1588364298394));
#133933=CARTESIAN_POINT('Ctrl Pts',(37.2174927205558,10.6864428650605,83.1620277542348));
#133934=CARTESIAN_POINT('Ctrl Pts',(37.1591691607311,10.676547766656,83.1627445914778));
#133935=CARTESIAN_POINT('Ctrl Pts',(37.098160489066,10.6661971157104,83.1634944306187));
#133936=CARTESIAN_POINT('Ctrl Pts',(37.0375814842102,10.6531658024788,83.1615368786296));
#133937=CARTESIAN_POINT('Ctrl Pts',(36.9778831345637,10.6375391372142,83.1568983825099));
#133938=CARTESIAN_POINT('Ctrl Pts',(36.9605629018404,10.6330053857676,83.1555526194737));
#133939=CARTESIAN_POINT('Ctrl Pts',(36.9433166599605,10.6282533801909,83.1539814155578));
#133940=CARTESIAN_POINT('Ctrl Pts',(36.9261551025346,10.6232857040459,83.1521859576523));
#133941=CARTESIAN_POINT('Ctrl Pts',(36.8683516997991,10.6065536221176,83.1461385125501));
#133942=CARTESIAN_POINT('Ctrl Pts',(36.8115253014697,10.5873765401978,83.1375457685393));
#133943=CARTESIAN_POINT('Ctrl Pts',(36.7560879726994,10.5658938613993,83.1264703670938));
#133944=CARTESIAN_POINT('Ctrl Pts',(36.7008470163571,10.5444872794454,83.1154341973992));
#133945=CARTESIAN_POINT('Ctrl Pts',(36.6469852670891,10.5207913936621,83.1019329227223));
#133946=CARTESIAN_POINT('Ctrl Pts',(36.5948915091628,10.4949767860708,83.0860635508859));
#133947=CARTESIAN_POINT('Ctrl Pts',(36.5439322613576,10.4697243750796,83.0705397859644));
#133948=CARTESIAN_POINT('Ctrl Pts',(36.494664911665,10.4424444925548,83.0527499052946));
#133949=CARTESIAN_POINT('Ctrl Pts',(36.4474351482632,10.4133283745433,83.0328185619169));
#133950=CARTESIAN_POINT('Ctrl Pts',(36.4340930536825,10.4051032645205,83.0271880897461));
#133951=CARTESIAN_POINT('Ctrl Pts',(36.4209134439883,10.3967318172069,83.0213869376233));
#133952=CARTESIAN_POINT('Ctrl Pts',(36.4079038136097,10.3882188220656,83.0154184325699));
#133953=CARTESIAN_POINT('Ctrl Pts',(36.3598710697787,10.3567880663133,82.99338216667));
#133954=CARTESIAN_POINT('Ctrl Pts',(36.314170375116,10.3234347915396,82.9690687730562));
#133955=CARTESIAN_POINT('Ctrl Pts',(36.2711213983952,10.2883947419835,82.9426506901393));
#133956=CARTESIAN_POINT('Ctrl Pts',(36.2302742105267,10.2551468555955,82.9175837901053));
#133957=CARTESIAN_POINT('Ctrl Pts',(36.1918148357754,10.2203800814043,82.890621679067));
#133958=CARTESIAN_POINT('Ctrl Pts',(36.1560043315853,10.1843264971648,82.8619435718565));
#133959=CARTESIAN_POINT('Ctrl Pts',(36.122171073087,10.1502635800696,82.834848901272));
#133960=CARTESIAN_POINT('Ctrl Pts',(36.0907028358421,10.1150520863725,82.8062224489253));
#133961=CARTESIAN_POINT('Ctrl Pts',(36.0618014956011,10.078917047279,82.7762470260351));
#133962=CARTESIAN_POINT('Ctrl Pts',(36.0505806496355,10.0648877426083,82.7646091711743));
#133963=CARTESIAN_POINT('Ctrl Pts',(36.0397464753727,10.0507195466556,82.7527683331707));
#133964=CARTESIAN_POINT('Ctrl Pts',(36.0293096587076,10.0364268503567,82.7407365951547));
#133965=CARTESIAN_POINT('Ctrl Pts',(36.0019553020889,9.99896643266913,82.7092020321751));
#133966=CARTESIAN_POINT('Ctrl Pts',(35.97734245913,9.9606666476471,82.6763694076741));
#133967=CARTESIAN_POINT('Ctrl Pts',(35.9555939932428,9.92172709202522,82.6424109829633));
#133968=CARTESIAN_POINT('Ctrl Pts',(35.9348937405076,9.88466431035839,82.6100892561048));
#133969=CARTESIAN_POINT('Ctrl Pts',(35.9167897165306,9.84702175446862,82.5767472218424));
#133970=CARTESIAN_POINT('Ctrl Pts',(35.9013866724505,9.80900396939047,82.5425651082853));
#133971=CARTESIAN_POINT('Ctrl Pts',(35.8867598368852,9.77290202174963,82.5101055404448));
#133972=CARTESIAN_POINT('Ctrl Pts',(35.8745697086462,9.73646199232484,82.4768885102196));
#133973=CARTESIAN_POINT('Ctrl Pts',(35.8648878244567,9.69988801776518,82.4430996797116));
#133974=CARTESIAN_POINT('Ctrl Pts',(35.85797840509,9.67378721721952,82.4189864807394));
#133975=CARTESIAN_POINT('Ctrl Pts',(35.8523460717753,9.64761884945182,82.3945827596681));
#133976=CARTESIAN_POINT('Ctrl Pts',(35.8480061888895,9.62146509318402,82.3699656206012));
#133977=CARTESIAN_POINT('Origin',(35.6454492392491,-0.499074165591586,72.5830523519042));
#133978=CARTESIAN_POINT('Origin',(34.1682376097291,-0.499074165591586,72.8435246184046));
#133979=CARTESIAN_POINT('',(36.4721616570127,13.601148584803,78.9068347604569));
#133980=CARTESIAN_POINT('Ctrl Pts',(35.3799890432589,11.6378875163018,79.715708490352));
#133981=CARTESIAN_POINT('Ctrl Pts',(35.3749324082523,11.7220490369113,79.6870221410859));
#133982=CARTESIAN_POINT('Ctrl Pts',(35.373425518673,11.8046126959294,79.6587776786043));
#133983=CARTESIAN_POINT('Ctrl Pts',(35.3753115536373,11.8852617928397,79.6309665278877));
#133984=CARTESIAN_POINT('Ctrl Pts',(35.3772248952026,11.9670785524741,79.6027527186759));
#133985=CARTESIAN_POINT('Ctrl Pts',(35.3826298212747,12.0469244565627,79.5749851036809));
#133986=CARTESIAN_POINT('Ctrl Pts',(35.3913271476137,12.1244920829818,79.5476888454789));
#133987=CARTESIAN_POINT('Ctrl Pts',(35.400215773304,12.2037658241355,79.5197922008726));
#133988=CARTESIAN_POINT('Ctrl Pts',(35.4125429179075,12.2806595160899,79.4923881468149));
#133989=CARTESIAN_POINT('Ctrl Pts',(35.4280637952047,12.3548760684726,79.4655350257877));
#133990=CARTESIAN_POINT('Ctrl Pts',(35.4366246988836,12.3958119475572,79.4507235574545));
#133991=CARTESIAN_POINT('Ctrl Pts',(35.4461567062305,12.4359339381909,79.4360802289885));
#133992=CARTESIAN_POINT('Ctrl Pts',(35.456615237334,12.475196785861,79.4216183015939));
#133993=CARTESIAN_POINT('Ctrl Pts',(35.4761345726474,12.5484752110474,79.3946272062575));
#133994=CARTESIAN_POINT('Ctrl Pts',(35.4988824621292,12.6187583521234,79.3682667391691));
#133995=CARTESIAN_POINT('Ctrl Pts',(35.5245504448773,12.6857847818072,79.3426417792656));
#133996=CARTESIAN_POINT('Ctrl Pts',(35.5424494187773,12.7325241117848,79.3247728063509));
#133997=CARTESIAN_POINT('Ctrl Pts',(35.5617678012447,12.7776807092336,79.3072620146635));
#133998=CARTESIAN_POINT('Ctrl Pts',(35.5823956077124,12.8211787476974,79.2901504470772));
#133999=CARTESIAN_POINT('Ctrl Pts',(35.6005139328016,12.8593850205195,79.2751205918768));
#134000=CARTESIAN_POINT('Ctrl Pts',(35.6197240475077,12.8964574372431,79.2603561273214));
#134001=CARTESIAN_POINT('Ctrl Pts',(35.6398698334597,12.9321867415071,79.2459266087515));
#134002=CARTESIAN_POINT('Ctrl Pts',(35.6601964451968,12.9682367470587,79.231367572821));
#134003=CARTESIAN_POINT('Ctrl Pts',(35.6814752036809,13.0029190103381,79.2171495440437));
#134004=CARTESIAN_POINT('Ctrl Pts',(35.7035123966813,13.0360515929857,79.2033694579059));
#134005=CARTESIAN_POINT('Ctrl Pts',(35.7201597213545,13.0610805910339,79.1929597125289));
#134006=CARTESIAN_POINT('Ctrl Pts',(35.737239108389,13.0852259193827,79.1828004280045));
#134007=CARTESIAN_POINT('Ctrl Pts',(35.7546569098908,13.1084233171307,79.1729425959568));
#134008=CARTESIAN_POINT('Ctrl Pts',(35.7954313567611,13.1627275909456,79.149865765678));
#134009=CARTESIAN_POINT('Ctrl Pts',(35.8389976528179,13.213328348537,79.1275471673048));
#134010=CARTESIAN_POINT('Ctrl Pts',(35.8850246599171,13.2599453121747,79.1060565522116));
#134011=CARTESIAN_POINT('Ctrl Pts',(35.9310021019971,13.3065120754877,79.0845890796781));
#134012=CARTESIAN_POINT('Ctrl Pts',(35.9794346537849,13.3491032713937,79.0639480256613));
#134013=CARTESIAN_POINT('Ctrl Pts',(36.0299562710254,13.387476333018,79.044210147366));
#134014=CARTESIAN_POINT('Ctrl Pts',(36.0803829479537,13.4257772839172,79.0245093605263));
#134015=CARTESIAN_POINT('Ctrl Pts',(36.132890498998,13.4598756486123,79.0057085595006));
#134016=CARTESIAN_POINT('Ctrl Pts',(36.1870839697266,13.4895716938935,78.987888132682));
#134017=CARTESIAN_POINT('Ctrl Pts',(36.1930758446128,13.4928550227806,78.9859178258077));
#134018=CARTESIAN_POINT('Ctrl Pts',(36.1990883010099,13.4960845797666,78.9839595058598));
#134019=CARTESIAN_POINT('Ctrl Pts',(36.2051207847567,13.4992601283539,78.9820132829396));
#134020=CARTESIAN_POINT('Ctrl Pts',(36.259550749436,13.5279125051692,78.9644528800851));
#134021=CARTESIAN_POINT('Ctrl Pts',(36.3156128403408,13.5521640749948,78.9478773243603));
#134022=CARTESIAN_POINT('Ctrl Pts',(36.3728872414993,13.5718670326191,78.9323676256727));
#134023=CARTESIAN_POINT('Ctrl Pts',(36.4056097441414,13.5831238955435,78.9235064914483));
#134024=CARTESIAN_POINT('Ctrl Pts',(36.4387275411762,13.59289687207,78.9149932713656));
#134025=CARTESIAN_POINT('Ctrl Pts',(36.4721594611798,13.6011654789238,78.9068428925862));
#134026=CARTESIAN_POINT('Ctrl Pts',(36.7497137917856,13.6349227617825,78.8487558990981));
#134027=CARTESIAN_POINT('Ctrl Pts',(36.7468847875822,13.6349194461349,78.8492624067619));
#134028=CARTESIAN_POINT('Ctrl Pts',(36.7426787151625,13.6349315419734,78.8499636260781));
#134029=CARTESIAN_POINT('Ctrl Pts',(36.736873947881,13.6349239250663,78.8508794246839));
#134030=CARTESIAN_POINT('Ctrl Pts',(36.733483665418,13.6349194764011,78.8514142981426));
#134031=CARTESIAN_POINT('Ctrl Pts',(36.7288578444576,13.6349071712433,78.8521225574776));
#134032=CARTESIAN_POINT('Ctrl Pts',(36.7241942792919,13.6348695191711,78.8528303166485));
#134033=CARTESIAN_POINT('Ctrl Pts',(36.7207774203749,13.6348419325899,78.8533488712624));
#134034=CARTESIAN_POINT('Ctrl Pts',(36.717340287326,13.6348016235124,78.8538669156717));
#134035=CARTESIAN_POINT('Ctrl Pts',(36.7143532752961,13.6347596533172,78.854311252123));
#134036=CARTESIAN_POINT('Ctrl Pts',(36.7056794312614,13.6346377780373,78.8556015398887));
#134037=CARTESIAN_POINT('Ctrl Pts',(36.6982661745955,13.6344046896701,78.8568142260074));
#134038=CARTESIAN_POINT('Ctrl Pts',(36.6915576979266,13.6340792668169,78.8580703235985));
#134039=CARTESIAN_POINT('Ctrl Pts',(36.6873395410126,13.633874647389,78.8588601328205));
#134040=CARTESIAN_POINT('Ctrl Pts',(36.6834000513446,13.6336322545447,78.8596674527749));
#134041=CARTESIAN_POINT('Ctrl Pts',(36.6796015271321,13.6333469994752,78.8605250079955));
#134042=CARTESIAN_POINT('Ctrl Pts',(36.6697619021318,13.6326080801591,78.8627464027573));
#134043=CARTESIAN_POINT('Ctrl Pts',(36.6594157298214,13.6313826480724,78.8658247010245));
#134044=CARTESIAN_POINT('Ctrl Pts',(36.6485285247017,13.6296454571002,78.8697212645982));
#134045=CARTESIAN_POINT('Ctrl Pts',(36.6430849221418,13.6287768616141,78.871669546385));
#134046=CARTESIAN_POINT('Ctrl Pts',(36.6375059082805,13.627780369151,78.8738222161859));
#134047=CARTESIAN_POINT('Ctrl Pts',(36.6317862300815,13.6266529083236,78.8761732365801));
#134048=CARTESIAN_POINT('Ctrl Pts',(36.6303073109073,13.6263613843291,78.8767811325175));
#134049=CARTESIAN_POINT('Ctrl Pts',(36.6289104049784,13.6260808457358,78.877361111239));
#134050=CARTESIAN_POINT('Ctrl Pts',(36.6275243140171,13.6257965115786,78.8779448496941));
#134051=CARTESIAN_POINT('Ctrl Pts',(36.62412449698,13.6250990940651,78.879376648905));
#134052=CARTESIAN_POINT('Ctrl Pts',(36.6207887373414,13.6243818440834,78.880830319144));
#134053=CARTESIAN_POINT('Ctrl Pts',(36.6164755445211,13.6233980448365,78.8827804225888));
#134054=CARTESIAN_POINT('Ctrl Pts',(36.615746373096,13.6232317276026,78.8831100994122));
#134055=CARTESIAN_POINT('Ctrl Pts',(36.6149893036036,13.6230576833706,78.8834539914887));
#134056=CARTESIAN_POINT('Ctrl Pts',(36.6141993559312,13.6228745694473,78.8838144294026));
#134057=CARTESIAN_POINT('Ctrl Pts',(36.5994639910949,13.6194588362783,78.8905378926753));
#134058=CARTESIAN_POINT('Ctrl Pts',(36.5865212063194,13.6165129372762,78.895752371069));
#134059=CARTESIAN_POINT('Ctrl Pts',(36.5754711213109,13.6141643825912,78.8995604732951));
#134060=CARTESIAN_POINT('Ctrl Pts',(36.5699460788067,13.6129901052487,78.9014645244082));
#134061=CARTESIAN_POINT('Ctrl Pts',(36.5648934069248,13.6119650049175,78.9030165200554));
#134062=CARTESIAN_POINT('Ctrl Pts',(36.5603209149633,13.6111033595531,78.9042259614167));
#134063=CARTESIAN_POINT('Ctrl Pts',(36.5569937647847,13.6104763877504,78.9051060051816));
#134064=CARTESIAN_POINT('Ctrl Pts',(36.5532155524438,13.6098369441149,78.905907742029));
#134065=CARTESIAN_POINT('Ctrl Pts',(36.5505279016848,13.6094049524859,78.9064091210418));
#134066=CARTESIAN_POINT('Ctrl Pts',(36.5495219225108,13.6092432593862,78.9065967856197));
#134067=CARTESIAN_POINT('Ctrl Pts',(36.5486686510362,13.6091111684528,78.906742236496));
#134068=CARTESIAN_POINT('Ctrl Pts',(36.5480487784383,13.6090214533071,78.9068335184581));
#134069=CARTESIAN_POINT('Ctrl Pts',(36.5448171192864,13.6085537301448,78.9073094100999));
#134070=CARTESIAN_POINT('Ctrl Pts',(36.5395942224044,13.6080020236394,78.9076128636903));
#134071=CARTESIAN_POINT('Ctrl Pts',(36.5323984940512,13.6073025311191,78.9077469719079));
#134072=CARTESIAN_POINT('Ctrl Pts',(36.5294587023756,13.6070167556997,78.9078017613889));
#134073=CARTESIAN_POINT('Ctrl Pts',(36.5261895964218,13.6067057282038,78.9078284516419));
#134074=CARTESIAN_POINT('Ctrl Pts',(36.5225923495154,13.6063626979722,78.9078279197424));
#134075=CARTESIAN_POINT('Ctrl Pts',(36.5163912352713,13.6057713652917,78.9078270028275));
#134076=CARTESIAN_POINT('Ctrl Pts',(36.5092160916144,13.6050858528307,78.9077445915112));
#134077=CARTESIAN_POINT('Ctrl Pts',(36.5010800577092,13.6042641038228,78.9075853796198));
#134078=CARTESIAN_POINT('Ctrl Pts',(36.4970120407567,13.6038532293188,78.9075057736741));
#134079=CARTESIAN_POINT('Ctrl Pts',(36.4927038226765,13.6034081692886,78.9074069052325));
#134080=CARTESIAN_POINT('Ctrl Pts',(36.4881576515518,13.602922681148,78.9072896469837));
#134081=CARTESIAN_POINT('Ctrl Pts',(36.4851625366389,13.6026028311621,78.9072123947377));
#134082=CARTESIAN_POINT('Ctrl Pts',(36.4810938518181,13.6021605085673,78.9070959579087));
#134083=CARTESIAN_POINT('Ctrl Pts',(36.4778700682971,13.601798676173,78.9070028584328));
#134084=CARTESIAN_POINT('Ctrl Pts',(36.4762005933016,13.6016112969241,78.9069546457517));
#134085=CARTESIAN_POINT('Ctrl Pts',(36.4747576873657,13.6014466821658,78.9069123781233));
#134086=CARTESIAN_POINT('Ctrl Pts',(36.4738076969342,13.6013382249055,78.9068833613598));
#134087=CARTESIAN_POINT('Ctrl Pts',(36.4732593742324,13.6012756247192,78.9068666132436));
#134088=CARTESIAN_POINT('Ctrl Pts',(36.4727106942741,13.6012124119033,78.9068504133483));
#134089=CARTESIAN_POINT('Ctrl Pts',(36.4721616570127,13.601148584803,78.906834760457));
#134090=CARTESIAN_POINT('Ctrl Pts',(35.4047464453691,11.47699078912,80.070829087246));
#134091=CARTESIAN_POINT('Ctrl Pts',(35.4010430938991,11.56996412073,80.039824743627));
#134092=CARTESIAN_POINT('Ctrl Pts',(35.4016895299391,11.88007018329,79.9341244321319));
#134093=CARTESIAN_POINT('Ctrl Pts',(35.4766108372791,12.36407360515,79.7569593010479));
#134094=CARTESIAN_POINT('Ctrl Pts',(35.6840194032591,12.85992909088,79.553941580112));
#134095=CARTESIAN_POINT('Ctrl Pts',(35.9715431495691,13.22233503903,79.382321605689));
#134096=CARTESIAN_POINT('Ctrl Pts',(36.3111476474691,13.4522667151,79.2458202724909));
#134097=CARTESIAN_POINT('Ctrl Pts',(36.6410702301991,13.54317413932,79.1573907935629));
#134098=CARTESIAN_POINT('Ctrl Pts',(36.8519924730991,13.54113934177,79.1207853593));
#134099=CARTESIAN_POINT('Ctrl Pts',(36.9359089029591,13.53124995019,79.109308518752));
#134100=CARTESIAN_POINT('Ctrl Pts',(35.4799873971691,11.49461145088,78.883043833973));
#134101=CARTESIAN_POINT('Ctrl Pts',(35.4515476021091,11.57600382921,78.85030473176));
#134102=CARTESIAN_POINT('Ctrl Pts',(35.3679195444291,11.85551262843,78.742056216998));
#134103=CARTESIAN_POINT('Ctrl Pts',(35.3086113826091,12.33697706548,78.5757610906141));
#134104=CARTESIAN_POINT('Ctrl Pts',(35.4013575593891,12.89860219014,78.396444849156));
#134105=CARTESIAN_POINT('Ctrl Pts',(35.6470520231591,13.35737986134,78.24380932435));
#134106=CARTESIAN_POINT('Ctrl Pts',(36.0126298069591,13.67448865407,78.114215280491));
#134107=CARTESIAN_POINT('Ctrl Pts',(36.4059824524991,13.80651913688,78.019865391245));
#134108=CARTESIAN_POINT('Ctrl Pts',(36.6613386460491,13.80349217816,77.97561025295));
#134109=CARTESIAN_POINT('Ctrl Pts',(36.7618041096891,13.78918487375,77.960551786597));
#134110=CARTESIAN_POINT('Ctrl Pts',(34.5323713981891,11.4437981521,78.16457618897));
#134111=CARTESIAN_POINT('Ctrl Pts',(34.4868146111391,11.55294239059,78.152451057442));
#134112=CARTESIAN_POINT('Ctrl Pts',(34.3532969408491,11.9344083525,78.1132993532569));
#134113=CARTESIAN_POINT('Ctrl Pts',(34.2636399697991,12.62703032885,78.0538368049579));
#134114=CARTESIAN_POINT('Ctrl Pts',(34.4346417170091,13.47889013285,77.9728297289189));
#134115=CARTESIAN_POINT('Ctrl Pts',(34.8683475554791,14.19947679409,77.873493505207));
#134116=CARTESIAN_POINT('Ctrl Pts',(35.5086014344991,14.70855335123,77.752522500601));
#134117=CARTESIAN_POINT('Ctrl Pts',(36.1932838806191,14.92297019512,77.629734621697));
#134118=CARTESIAN_POINT('Ctrl Pts',(36.6339629540391,14.91801708291,77.552516340959));
#134119=CARTESIAN_POINT('Ctrl Pts',(36.8064748222491,14.89480530408,77.522190509913));
#134120=CARTESIAN_POINT('Ctrl Pts',(33.4121724780091,11.37014449647,78.5600906369051));
#134121=CARTESIAN_POINT('Ctrl Pts',(33.3724768335991,11.52147230307,78.572431763808));
#134122=CARTESIAN_POINT('Ctrl Pts',(33.2682192331391,12.04596603781,78.612022905951));
#134123=CARTESIAN_POINT('Ctrl Pts',(33.2793254009391,12.97397527668,78.6594970952119));
#134124=CARTESIAN_POINT('Ctrl Pts',(33.6512837556791,14.08011390146,78.663196318665));
#134125=CARTESIAN_POINT('Ctrl Pts',(34.3341433460291,14.99303163765,78.603650011164));
#134126=CARTESIAN_POINT('Ctrl Pts',(35.2513155901291,15.62661834944,78.485280541034));
#134127=CARTESIAN_POINT('Ctrl Pts',(36.1938240485491,15.89076147096,78.337053846843));
#134128=CARTESIAN_POINT('Ctrl Pts',(36.7944289755491,15.88467650615,78.231136054428));
#134129=CARTESIAN_POINT('Ctrl Pts',(37.0298390382191,15.8560634713,78.187556174812));
#134130=CARTESIAN_POINT('Ctrl Pts',(36.4721616570127,13.601148584803,78.906834760457));
#134131=CARTESIAN_POINT('Ctrl Pts',(36.4504061654935,13.598619448735,78.9062145177738));
#134132=CARTESIAN_POINT('Ctrl Pts',(36.428088693382,13.59512625113,78.9064529546472));
#134133=CARTESIAN_POINT('Ctrl Pts',(36.4052122412434,13.5905635514609,78.9074754761355));
#134134=CARTESIAN_POINT('Ctrl Pts',(36.3934853518584,13.5882246278379,78.9079996394243));
#134135=CARTESIAN_POINT('Ctrl Pts',(36.3816115827963,13.5856047262905,78.908729525301));
#134136=CARTESIAN_POINT('Ctrl Pts',(36.3695915648287,13.5826898772137,78.9096530208533));
#134137=CARTESIAN_POINT('Ctrl Pts',(36.3635815558449,13.5812324526753,78.9101147686295));
#134138=CARTESIAN_POINT('Ctrl Pts',(36.3575349823577,13.5797012811641,78.9106249156237));
#134139=CARTESIAN_POINT('Ctrl Pts',(36.3514519583453,13.5780946372335,78.9111817763396));
#134140=CARTESIAN_POINT('Ctrl Pts',(36.3472346223365,13.5769807574777,78.9115678456275));
#134141=CARTESIAN_POINT('Ctrl Pts',(36.3435292244632,13.5759772404352,78.9119216633451));
#134142=CARTESIAN_POINT('Ctrl Pts',(36.3392342676222,13.5747801330311,78.9123560774501));
#134143=CARTESIAN_POINT('Ctrl Pts',(36.3373342412936,13.5742505501575,78.9125482559207));
#134144=CARTESIAN_POINT('Ctrl Pts',(36.3353189419999,13.5736825169018,78.9127563333781));
#134145=CARTESIAN_POINT('Ctrl Pts',(36.3330936499266,13.5730465216947,78.9129907842902));
#134146=CARTESIAN_POINT('Ctrl Pts',(36.3122587859171,13.5670918545255,78.9151858906899));
#134147=CARTESIAN_POINT('Ctrl Pts',(36.2931857227023,13.5612738711274,78.9169194038706));
#134148=CARTESIAN_POINT('Ctrl Pts',(36.2758412379195,13.5558046431333,78.9182299553678));
#134149=CARTESIAN_POINT('Ctrl Pts',(36.2690256488441,13.553655486728,78.9187449421534));
#134150=CARTESIAN_POINT('Ctrl Pts',(36.2624770389035,13.5515596390135,78.9191947814029));
#134151=CARTESIAN_POINT('Ctrl Pts',(36.2561937050724,13.5495278851669,78.9195824250782));
#134152=CARTESIAN_POINT('Ctrl Pts',(36.2450570441208,13.5459267787583,78.9202694896681));
#134153=CARTESIAN_POINT('Ctrl Pts',(36.2347522538573,13.5425280212809,78.9207596890134));
#134154=CARTESIAN_POINT('Ctrl Pts',(36.2252649480616,13.5393851503123,78.9210638349686));
#134155=CARTESIAN_POINT('Ctrl Pts',(36.2239299671903,13.5389429096262,78.9211066320536));
#134156=CARTESIAN_POINT('Ctrl Pts',(36.2226111757268,13.5385057219258,78.9211457408626));
#134157=CARTESIAN_POINT('Ctrl Pts',(36.2213085307405,13.5380737218633,78.9211811859676));
#134158=CARTESIAN_POINT('Ctrl Pts',(36.2179824235124,13.5369706749508,78.9212716896898));
#134159=CARTESIAN_POINT('Ctrl Pts',(36.2147615805659,13.5359014635584,78.9213383042534));
#134160=CARTESIAN_POINT('Ctrl Pts',(36.2116452961703,13.5348682206978,78.9213814728402));
#134161=CARTESIAN_POINT('Ctrl Pts',(36.2087853143723,13.533919958152,78.921421090974));
#134162=CARTESIAN_POINT('Ctrl Pts',(36.2068846778224,13.5332829968046,78.9214485990927));
#134163=CARTESIAN_POINT('Ctrl Pts',(36.2042187359777,13.5324049186788,78.9214487403883));
#134164=CARTESIAN_POINT('Ctrl Pts',(36.2028421578516,13.5319515167625,78.9214488133474));
#134165=CARTESIAN_POINT('Ctrl Pts',(36.2012616263255,13.5314333037895,78.9214416966704));
#134166=CARTESIAN_POINT('Ctrl Pts',(36.1992406519875,13.5307688878843,78.9214263749526));
#134167=CARTESIAN_POINT('Ctrl Pts',(36.1670570918207,13.520188214563,78.9211823800541));
#134168=CARTESIAN_POINT('Ctrl Pts',(36.1351752345258,13.5094888143299,78.9192661055963));
#134169=CARTESIAN_POINT('Ctrl Pts',(36.10375519299,13.4988266822702,78.9159806720018));
#134170=CARTESIAN_POINT('Ctrl Pts',(36.0888225633727,13.4937594175182,78.9144192430348));
#134171=CARTESIAN_POINT('Ctrl Pts',(36.0739945375956,13.4887013497456,78.91254856096));
#134172=CARTESIAN_POINT('Ctrl Pts',(36.0592901050985,13.4836727766471,78.9104013418097));
#134173=CARTESIAN_POINT('Ctrl Pts',(36.0364679451207,13.475868130005,78.9070687290777));
#134174=CARTESIAN_POINT('Ctrl Pts',(36.0139347499633,13.4681316932326,78.9030690828645));
#134175=CARTESIAN_POINT('Ctrl Pts',(35.9917231242992,13.4605285167546,78.8985167430992));
#134176=CARTESIAN_POINT('Ctrl Pts',(35.9806173114672,13.4567269285156,78.8962405732166));
#134177=CARTESIAN_POINT('Ctrl Pts',(35.9695915956965,13.452958566235,78.8938261252443));
#134178=CARTESIAN_POINT('Ctrl Pts',(35.9586484977955,13.4492308986411,78.8912869754962));
#134179=CARTESIAN_POINT('Ctrl Pts',(35.9521332283931,13.4470115308866,78.8897752239967));
#134180=CARTESIAN_POINT('Ctrl Pts',(35.946232804495,13.4449969559354,78.888371918885));
#134181=CARTESIAN_POINT('Ctrl Pts',(35.9399018577183,13.4428519618481,78.8868063897854));
#134182=CARTESIAN_POINT('Ctrl Pts',(35.9355992963306,13.4413942069399,78.8857424438556));
#134183=CARTESIAN_POINT('Ctrl Pts',(35.9310978609088,13.4398753672442,78.88460376303));
#134184=CARTESIAN_POINT('Ctrl Pts',(35.9260687135604,13.4381769231713,78.8833084515107));
#134185=CARTESIAN_POINT('Ctrl Pts',(35.899945135366,13.4293544661078,78.8765800402282));
#134186=CARTESIAN_POINT('Ctrl Pts',(35.8741882104117,13.4206854200628,78.8692741996048));
#134187=CARTESIAN_POINT('Ctrl Pts',(35.8485408966571,13.4121822154005,78.8614124658743));
#134188=CARTESIAN_POINT('Ctrl Pts',(35.82250526924,13.4035502677994,78.8534317014084));
#134189=CARTESIAN_POINT('Ctrl Pts',(35.7965825163458,13.3950891138958,78.844878072982));
#134190=CARTESIAN_POINT('Ctrl Pts',(35.7705075977699,13.3867622396569,78.8357933863257));
#134191=CARTESIAN_POINT('Ctrl Pts',(35.7640936161502,13.3847139717721,78.8335587096166));
#134192=CARTESIAN_POINT('Ctrl Pts',(35.7576704489817,13.382673600299,78.8312919907959));
#134193=CARTESIAN_POINT('Ctrl Pts',(35.7512341970586,13.380640136617,78.8289940301167));
#134194=CARTESIAN_POINT('Ctrl Pts',(35.7253016081509,13.3724470176477,78.8197352145307));
#134195=CARTESIAN_POINT('Ctrl Pts',(35.699156188398,13.364369732452,78.8099677195824));
#134196=CARTESIAN_POINT('Ctrl Pts',(35.6725345118184,13.3563152336591,78.7997573802145));
#134197=CARTESIAN_POINT('Ctrl Pts',(35.6583696149245,13.3520295852855,78.7943246493357));
#134198=CARTESIAN_POINT('Ctrl Pts',(35.644069970644,13.347749596578,78.7887668669451));
#134199=CARTESIAN_POINT('Ctrl Pts',(35.6295965665019,13.3434556875699,78.7830962085536));
#134200=CARTESIAN_POINT('Ctrl Pts',(35.5957491463823,13.3334139765305,78.7698348392829));
#134201=CARTESIAN_POINT('Ctrl Pts',(35.5610961675901,13.3234052337112,78.7559509003528));
#134202=CARTESIAN_POINT('Ctrl Pts',(35.5254411255284,13.3134447719003,78.7415837844168));
#134203=CARTESIAN_POINT('Ctrl Pts',(35.4890666251392,13.303283324849,78.7269267644277));
#134204=CARTESIAN_POINT('Ctrl Pts',(35.4516484315061,13.2931726331318,78.7117663479471));
#134205=CARTESIAN_POINT('Ctrl Pts',(35.4129822688164,13.2830990650404,78.6963000244749));
#134206=CARTESIAN_POINT('Ctrl Pts',(35.3774872942956,13.2738516761643,78.6821021646567));
#134207=CARTESIAN_POINT('Ctrl Pts',(35.3409400501456,13.2646354930113,78.6676469707998));
#134208=CARTESIAN_POINT('Ctrl Pts',(35.3031958978858,13.2554129208036,78.6531274388204));
#134209=CARTESIAN_POINT('Ctrl Pts',(35.2998237639228,13.2545889587563,78.651830236367));
#134210=CARTESIAN_POINT('Ctrl Pts',(35.2964420893669,13.253764926886,78.6505325463469));
#134211=CARTESIAN_POINT('Ctrl Pts',(35.2930507794226,13.2529407870952,78.6492345216881));
#134212=CARTESIAN_POINT('Ctrl Pts',(35.2565394350175,13.244067976224,78.6352597962448));
#134213=CARTESIAN_POINT('Ctrl Pts',(35.2189214988429,13.2351963570681,78.6212427822176));
#134214=CARTESIAN_POINT('Ctrl Pts',(35.1800835948419,13.2262912408389,78.6073783241714));
#134215=CARTESIAN_POINT('Ctrl Pts',(35.1533790067126,13.2201681642399,78.597845249427));
#134216=CARTESIAN_POINT('Ctrl Pts',(35.1260979765889,13.2140287947895,78.5883851016776));
#134217=CARTESIAN_POINT('Ctrl Pts',(35.0982113352202,13.207855117831,78.579071407501));
#134218=CARTESIAN_POINT('Ctrl Pts',(35.0763291035399,13.2030107255737,78.5717630905517));
#134219=CARTESIAN_POINT('Ctrl Pts',(35.0540757775653,13.1981444782573,78.5645460778694));
#134220=CARTESIAN_POINT('Ctrl Pts',(35.0314390924283,13.193246632164,78.5574578386157));
#134221=CARTESIAN_POINT('Ctrl Pts',(35.0186740463358,13.1904846892931,78.5534607118174));
#134222=CARTESIAN_POINT('Ctrl Pts',(35.0057871537928,13.187712659575,78.5495045921738));
#134223=CARTESIAN_POINT('Ctrl Pts',(34.9927763607437,13.1849282282858,78.5455966860617));
#134224=CARTESIAN_POINT('Ctrl Pts',(34.9743582771188,13.180986586286,78.5400646526723));
#134225=CARTESIAN_POINT('Ctrl Pts',(34.9554131454896,13.1769677477061,78.5345457685357));
#134226=CARTESIAN_POINT('Ctrl Pts',(34.9363618770901,13.1729421492203,78.5291938283296));
#134227=CARTESIAN_POINT('Ctrl Pts',(34.9180893898604,13.169081109872,78.524060665696));
#134228=CARTESIAN_POINT('Ctrl Pts',(34.8997196252843,13.1652138258829,78.5190810386885));
#134229=CARTESIAN_POINT('Ctrl Pts',(34.8816401240329,13.1614272575593,78.5143564196021));
#134230=CARTESIAN_POINT('Ctrl Pts',(34.8391099224564,13.1525197378306,78.5032422301495));
#134231=CARTESIAN_POINT('Ctrl Pts',(34.7955882146145,13.1434492907672,78.4928655648522));
#134232=CARTESIAN_POINT('Ctrl Pts',(34.7510398756842,13.1341533320885,78.4834200768374));
#134233=CARTESIAN_POINT('Ctrl Pts',(34.7074698710593,13.1250615236765,78.4741820229307));
#134234=CARTESIAN_POINT('Ctrl Pts',(34.6629172741695,13.1157539344517,78.4658352247198));
#134235=CARTESIAN_POINT('Ctrl Pts',(34.6173892125664,13.1061531878966,78.4585819459816));
#134236=CARTESIAN_POINT('Ctrl Pts',(34.5732100030488,13.0968368810158,78.4515435588907));
#134237=CARTESIAN_POINT('Ctrl Pts',(34.5281119258475,13.0872443608496,78.445535517776));
#134238=CARTESIAN_POINT('Ctrl Pts',(34.4821460687883,13.0772887589311,78.4407539859881));
#134239=CARTESIAN_POINT('Ctrl Pts',(34.4556942684274,13.0715596458183,78.4380023757199));
#134240=CARTESIAN_POINT('Ctrl Pts',(34.4289559538174,13.0657100025855,78.4356571048377));
#134241=CARTESIAN_POINT('Ctrl Pts',(34.4019484562768,13.0597211322695,78.4337559236378));
#134242=CARTESIAN_POINT('Ctrl Pts',(34.3575430466552,13.0498743021752,78.4306300238828));
#134243=CARTESIAN_POINT('Ctrl Pts',(34.3124132438406,13.0396630086552,78.4287031985923));
#134244=CARTESIAN_POINT('Ctrl Pts',(34.2666189774245,13.0290012971378,78.4281398834861));
#134245=CARTESIAN_POINT('Ctrl Pts',(34.2216993254271,13.0185432112564,78.4275873270088));
#134246=CARTESIAN_POINT('Ctrl Pts',(34.1761401095282,13.0076515539986,78.4283474448037));
#134247=CARTESIAN_POINT('Ctrl Pts',(34.1300448615253,12.9962314458899,78.4305751618034));
#134248=CARTESIAN_POINT('Ctrl Pts',(34.0851465644316,12.9851078826394,78.4327450318882));
#134249=CARTESIAN_POINT('Ctrl Pts',(34.0397397518139,12.9734826841811,78.4363080260802));
#134250=CARTESIAN_POINT('Ctrl Pts',(33.9939664444587,12.9612584436044,78.4413960448565));
#134251=CARTESIAN_POINT('Ctrl Pts',(33.9493383893727,12.9493400546271,78.4463567609451));
#134252=CARTESIAN_POINT('Ctrl Pts',(33.9043622022559,12.9368519188894,78.4527678284234));
#134253=CARTESIAN_POINT('Ctrl Pts',(33.8592119939158,12.9236986194734,78.4607301343571));
#134254=CARTESIAN_POINT('Ctrl Pts',(35.28916359171,12.25029619447,78.8322534413786));
#134255=CARTESIAN_POINT('Ctrl Pts',(35.2779279497709,12.2624028118831,78.8186638264655));
#134256=CARTESIAN_POINT('Ctrl Pts',(35.2666923078319,12.2745094292961,78.8050742115524));
#134257=CARTESIAN_POINT('Ctrl Pts',(35.2554566658928,12.2866160467092,78.7914845966393));
#134258=CARTESIAN_POINT('Ctrl Pts',(35.2498393249075,12.2926688382236,78.7846903697282));
#134259=CARTESIAN_POINT('Ctrl Pts',(35.2378447957871,12.3055931709764,78.7701828736105));
#134260=CARTESIAN_POINT('Ctrl Pts',(35.1977745566455,12.3335999215784,78.7309978424039));
#134261=CARTESIAN_POINT('Ctrl Pts',(35.1455449414878,12.3640756612257,78.6882977707834));
#134262=CARTESIAN_POINT('Ctrl Pts',(35.0806760308514,12.3962322793046,78.6430241955527));
#134263=CARTESIAN_POINT('Ctrl Pts',(35.0054940744708,12.4283335028473,78.5983814367481));
#134264=CARTESIAN_POINT('Ctrl Pts',(34.9213590600735,12.4595076387769,78.5559499882088));
#134265=CARTESIAN_POINT('Ctrl Pts',(34.8297226352172,12.4890184640333,78.5171196827213));
#134266=CARTESIAN_POINT('Ctrl Pts',(34.7318182707934,12.5163508899825,78.4828709295655));
#134267=CARTESIAN_POINT('Ctrl Pts',(34.6286945809858,12.5411170357543,78.4539359247313));
#134268=CARTESIAN_POINT('Ctrl Pts',(34.521309326854,12.5630211819863,78.4308698615195));
#134269=CARTESIAN_POINT('Ctrl Pts',(34.410582224273,12.5818286325215,78.4141056081173));
#134270=CARTESIAN_POINT('Ctrl Pts',(34.2973831835532,12.5973569512455,78.4039606649909));
#134271=CARTESIAN_POINT('Ctrl Pts',(34.182550136185,12.6094541243224,78.4006770615684));
#134272=CARTESIAN_POINT('Ctrl Pts',(34.0668631558752,12.6180352212567,78.4043475217904));
#134273=CARTESIAN_POINT('Ctrl Pts',(33.9511293651193,12.6229294807815,78.4152033744343));
#134274=CARTESIAN_POINT('Ctrl Pts',(33.8358811094663,12.6244155387313,78.4326287066328));
#134275=CARTESIAN_POINT('Ctrl Pts',(33.7603444272674,12.6222852452232,78.4500993196882));
#134276=CARTESIAN_POINT('Ctrl Pts',(33.7225560295391,12.62121953283,78.458839265043));
#134277=CARTESIAN_POINT('Ctrl Pts',(35.4366085353606,13.1319050302734,79.1874339641305));
#134278=CARTESIAN_POINT('Ctrl Pts',(35.4207517619085,13.1486721140446,79.1625108794446));
#134279=CARTESIAN_POINT('Ctrl Pts',(35.4048949884563,13.1654391978158,79.1375877947585));
#134280=CARTESIAN_POINT('Ctrl Pts',(35.3890382150042,13.1822062815871,79.1126647100726));
#134281=CARTESIAN_POINT('Ctrl Pts',(35.3811105056762,13.1905891071864,79.1002042324384));
#134282=CARTESIAN_POINT('Ctrl Pts',(35.3641827206898,13.2084886874374,79.0735977717966));
#134283=CARTESIAN_POINT('Ctrl Pts',(35.3177304804994,13.2419830464803,79.0201443411684));
#134284=CARTESIAN_POINT('Ctrl Pts',(35.2588716100858,13.2776620254717,78.9634162208831));
#134285=CARTESIAN_POINT('Ctrl Pts',(35.1873965239757,13.3144101862539,78.9051574459597));
#134286=CARTESIAN_POINT('Ctrl Pts',(35.1056278786597,13.350605956571,78.8484493715112));
#134287=CARTESIAN_POINT('Ctrl Pts',(35.0149498370101,13.3853905016559,78.7949465547076));
#134288=CARTESIAN_POINT('Ctrl Pts',(34.9168131164966,13.4180705017977,78.7460465944024));
#134289=CARTESIAN_POINT('Ctrl Pts',(34.8124542051494,13.4481598270206,78.7027629943066));
#134290=CARTESIAN_POINT('Ctrl Pts',(34.7029353862565,13.4752955310091,78.6658669209103));
#134291=CARTESIAN_POINT('Ctrl Pts',(34.5892300455026,13.4992036211595,78.6359530878952));
#134292=CARTESIAN_POINT('Ctrl Pts',(34.4722724330095,13.5196689246599,78.6134911795104));
#134293=CARTESIAN_POINT('Ctrl Pts',(34.3529487854807,13.536525360577,78.5988334811408));
#134294=CARTESIAN_POINT('Ctrl Pts',(34.2321151716127,13.5496335413214,78.5922569555576));
#134295=CARTESIAN_POINT('Ctrl Pts',(34.1105699318438,13.5589198993391,78.5938744656302));
#134296=CARTESIAN_POINT('Ctrl Pts',(33.9891475214067,13.5642122072015,78.6039717921799));
#134297=CARTESIAN_POINT('Ctrl Pts',(33.8683813111162,13.5658193574116,78.621834011338));
#134298=CARTESIAN_POINT('Ctrl Pts',(33.7893531292966,13.5635153199518,78.6406889999889));
#134299=CARTESIAN_POINT('Ctrl Pts',(33.7498180546891,13.56236268945,78.650121500723));
#134300=CARTESIAN_POINT('Ctrl Pts',(36.2117870627125,13.731466576071,79.1317548552529));
#134301=CARTESIAN_POINT('Ctrl Pts',(36.1637348888923,13.7660243550344,79.0619065056057));
#134302=CARTESIAN_POINT('Ctrl Pts',(36.1156827150721,13.8005821339978,78.9920581559585));
#134303=CARTESIAN_POINT('Ctrl Pts',(36.067630541252,13.8351399129612,78.9222098063113));
#134304=CARTESIAN_POINT('Ctrl Pts',(36.0436065071205,13.852417326142,78.8872886153943));
#134305=CARTESIAN_POINT('Ctrl Pts',(35.9923087529454,13.8893092356887,78.8127225097455));
#134306=CARTESIAN_POINT('Ctrl Pts',(35.9013880959124,13.9401153189454,78.7100025341022));
#134307=CARTESIAN_POINT('Ctrl Pts',(35.7958684940579,13.9911722275058,78.606777171674));
#134308=CARTESIAN_POINT('Ctrl Pts',(35.6773128854183,14.0400985472753,78.5080807209751));
#134309=CARTESIAN_POINT('Ctrl Pts',(35.5479476310375,14.0862484994258,78.415498960707));
#134310=CARTESIAN_POINT('Ctrl Pts',(35.4092346850833,14.1290516801646,78.330544171871));
#134311=CARTESIAN_POINT('Ctrl Pts',(35.2625355537129,14.16820270898,78.254228706184));
#134312=CARTESIAN_POINT('Ctrl Pts',(35.1090331574187,14.2034821063204,78.1874101995993));
#134313=CARTESIAN_POINT('Ctrl Pts',(34.9498411966155,14.2347418113983,78.1307946248619));
#134314=CARTESIAN_POINT('Ctrl Pts',(34.786010574763,14.2618838966983,78.0849619730775));
#134315=CARTESIAN_POINT('Ctrl Pts',(34.6185511567095,14.2848431924266,78.0503886163853));
#134316=CARTESIAN_POINT('Ctrl Pts',(34.4484483884156,14.3035755304223,78.0274544727356));
#134317=CARTESIAN_POINT('Ctrl Pts',(34.2766775950479,14.3180385947544,78.0164841582442));
#134318=CARTESIAN_POINT('Ctrl Pts',(34.1041767867636,14.3282324593606,78.017610234519));
#134319=CARTESIAN_POINT('Ctrl Pts',(33.9319683359579,14.3340234493632,78.031253517041));
#134320=CARTESIAN_POINT('Ctrl Pts',(33.7606990047544,14.3357830595542,78.0563719770334));
#134321=CARTESIAN_POINT('Ctrl Pts',(33.6485441033515,14.3332597659042,78.0834328777287));
#134322=CARTESIAN_POINT('Ctrl Pts',(33.5924368730891,14.33199744909,78.096970513333));
#134323=CARTESIAN_POINT('Ctrl Pts',(37.0959814013386,13.6477787622855,78.702474297618));
#134324=CARTESIAN_POINT('Ctrl Pts',(37.0097034037152,13.7013526595415,78.5841710380778));
#134325=CARTESIAN_POINT('Ctrl Pts',(36.9234254060918,13.7549265567976,78.4658677785376));
#134326=CARTESIAN_POINT('Ctrl Pts',(36.8371474084684,13.8085004540536,78.3475645189974));
#134327=CARTESIAN_POINT('Ctrl Pts',(36.7940120954343,13.8352851140162,78.2884179431172));
#134328=CARTESIAN_POINT('Ctrl Pts',(36.7019066367019,13.8924775445173,78.1621241452819));
#134329=CARTESIAN_POINT('Ctrl Pts',(36.5581875931855,13.9608351698212,78.0081066363786));
#134330=CARTESIAN_POINT('Ctrl Pts',(36.3971992371637,14.0271544164863,77.8570288914372));
#134331=CARTESIAN_POINT('Ctrl Pts',(36.222593119429,14.0876963855601,77.7175015279586));
#134332=CARTESIAN_POINT('Ctrl Pts',(36.0364710403563,14.142999223141,77.5892429153225));
#134333=CARTESIAN_POINT('Ctrl Pts',(35.8403743068097,14.192863522938,77.4735019242573));
#134334=CARTESIAN_POINT('Ctrl Pts',(35.6355466289455,14.2374572864306,77.3707704377697));
#134335=CARTESIAN_POINT('Ctrl Pts',(35.4230966202696,14.276886944725,77.2816655621943));
#134336=CARTESIAN_POINT('Ctrl Pts',(35.2041927400843,14.311265480877,77.2067675372761));
#134337=CARTESIAN_POINT('Ctrl Pts',(34.9799734310699,14.3407075552358,77.1465972403352));
#134338=CARTESIAN_POINT('Ctrl Pts',(34.7515346550071,14.3653281048325,77.1016031279655));
#134339=CARTESIAN_POINT('Ctrl Pts',(34.5199775631649,14.3852288528339,77.0721671077446));
#134340=CARTESIAN_POINT('Ctrl Pts',(34.2864180549368,14.4004840439715,77.0586422814665));
#134341=CARTESIAN_POINT('Ctrl Pts',(34.0519617518984,14.4111803943695,77.061167287698));
#134342=CARTESIAN_POINT('Ctrl Pts',(33.8178537815412,14.4172370026292,77.080288199522));
#134343=CARTESIAN_POINT('Ctrl Pts',(33.5848907865268,14.4190784205302,77.1146266745727));
#134344=CARTESIAN_POINT('Ctrl Pts',(33.4321409917259,14.416437075733,77.1512239629719));
#134345=CARTESIAN_POINT('Ctrl Pts',(33.3557255359391,14.415115702,77.169532324546));
#134346=CARTESIAN_POINT('Origin',(58.0152958556891,-0.499074165591486,68.638644839116));
#134347=CARTESIAN_POINT('',(69.9613704439522,11.9506555274059,75.9079901281648));
#134348=CARTESIAN_POINT('',(70.5465864373914,11.5358766795373,76.3475297110445));
#134349=CARTESIAN_POINT('Ctrl Pts',(69.9613704417151,11.95065551084,75.9079901160842));
#134350=CARTESIAN_POINT('Ctrl Pts',(69.9615209599404,11.9500108384424,75.9088462703833));
#134351=CARTESIAN_POINT('Ctrl Pts',(69.9616732757947,11.9493665883909,75.909701329011));
#134352=CARTESIAN_POINT('Ctrl Pts',(69.9618273824786,11.9487227594097,75.9105552952276));
#134353=CARTESIAN_POINT('Ctrl Pts',(69.9652026681753,11.9346214453371,75.9292590910818));
#134354=CARTESIAN_POINT('Ctrl Pts',(69.9694325138086,11.9207229649935,75.9474390034307));
#134355=CARTESIAN_POINT('Ctrl Pts',(69.9744552735693,11.907002133724,75.965153413181));
#134356=CARTESIAN_POINT('Ctrl Pts',(69.9796461127933,11.892822154483,75.9834606102881));
#134357=CARTESIAN_POINT('Ctrl Pts',(69.9856840690767,11.8788312841992,76.0012713858033));
#134358=CARTESIAN_POINT('Ctrl Pts',(69.9925567342574,11.8649965119743,76.0186414871835));
#134359=CARTESIAN_POINT('Ctrl Pts',(69.999429399438,11.8511617397494,76.0360115885636));
#134360=CARTESIAN_POINT('Ctrl Pts',(70.007137210894,11.837482415808,76.0529417523489));
#134361=CARTESIAN_POINT('Ctrl Pts',(70.0157168351401,11.8239301149553,76.0694679524188));
#134362=CARTESIAN_POINT('Ctrl Pts',(70.0203011593225,11.8166887558067,76.078298345971));
#134363=CARTESIAN_POINT('Ctrl Pts',(70.0251185502922,11.8094823846021,76.0870177768771));
#134364=CARTESIAN_POINT('Ctrl Pts',(70.0301626360558,11.8023273164306,76.0956060680119));
#134365=CARTESIAN_POINT('Ctrl Pts',(70.041856427489,11.7857395979006,76.1155164521738));
#134366=CARTESIAN_POINT('Ctrl Pts',(70.0547716746612,11.7694286456886,76.1347198592858));
#134367=CARTESIAN_POINT('Ctrl Pts',(70.0687605648971,11.7536201996829,76.1529698102241));
#134368=CARTESIAN_POINT('Ctrl Pts',(70.0819348412068,11.738732325649,76.1701570132291));
#134369=CARTESIAN_POINT('Ctrl Pts',(70.0960605979567,11.7242907164731,76.1864980767739));
#134370=CARTESIAN_POINT('Ctrl Pts',(70.1109807244523,11.7104662987638,76.2018184769042));
#134371=CARTESIAN_POINT('Ctrl Pts',(70.1119032907124,11.7096114842053,76.2027657935543));
#134372=CARTESIAN_POINT('Ctrl Pts',(70.1128288849219,11.708759021985,76.2037092195967));
#134373=CARTESIAN_POINT('Ctrl Pts',(70.1137574663665,11.707908949425,76.2046487185943));
#134374=CARTESIAN_POINT('Ctrl Pts',(70.1269673712688,11.6958159039061,76.2180139354918));
#134375=CARTESIAN_POINT('Ctrl Pts',(70.1407853915092,11.6842152396375,76.2305725267381));
#134376=CARTESIAN_POINT('Ctrl Pts',(70.1551548756988,11.6731568727412,76.2422830906839));
#134377=CARTESIAN_POINT('Ctrl Pts',(70.1770158002945,11.6563332956608,76.2600988836529));
#134378=CARTESIAN_POINT('Ctrl Pts',(70.2001503279608,11.6407646475148,76.275953100659));
#134379=CARTESIAN_POINT('Ctrl Pts',(70.2242568536363,11.6266454419759,76.2897076010034));
#134380=CARTESIAN_POINT('Ctrl Pts',(70.2308104620605,11.6228069898651,76.2934469042335));
#134381=CARTESIAN_POINT('Ctrl Pts',(70.2374361978791,11.6190756679541,76.2970309202755));
#134382=CARTESIAN_POINT('Ctrl Pts',(70.2441285749294,11.6154554353968,76.3004566166471));
#134383=CARTESIAN_POINT('Ctrl Pts',(70.2636026522798,11.6049209588846,76.3104250143655));
#134384=CARTESIAN_POINT('Ctrl Pts',(70.2836308477456,11.5952996211569,76.3190897115059));
#134385=CARTESIAN_POINT('Ctrl Pts',(70.3039992462445,11.5867074310029,76.3263646979402));
#134386=CARTESIAN_POINT('Ctrl Pts',(70.3087115952567,11.5847195771819,76.3280478089192));
#134387=CARTESIAN_POINT('Ctrl Pts',(70.3134421864876,11.5827866695546,76.329656700523));
#134388=CARTESIAN_POINT('Ctrl Pts',(70.3181884448014,11.5809098859167,76.3311906113044));
#134389=CARTESIAN_POINT('Ctrl Pts',(70.3385421726943,11.5728615368899,76.3377685934946));
#134390=CARTESIAN_POINT('Ctrl Pts',(70.3591820291187,11.5658477224918,76.3429650876769));
#134391=CARTESIAN_POINT('Ctrl Pts',(70.3798508972394,11.5598993598248,76.3468012621473));
#134392=CARTESIAN_POINT('Ctrl Pts',(70.3843330575984,11.558609423908,76.347633158168));
#134393=CARTESIAN_POINT('Ctrl Pts',(70.3888166800923,11.5573694772226,76.3484012058652));
#134394=CARTESIAN_POINT('Ctrl Pts',(70.3932993148755,11.5561796438526,76.3491058224419));
#134395=CARTESIAN_POINT('Ctrl Pts',(70.4086833100591,11.5520962438616,76.3515240024957));
#134396=CARTESIAN_POINT('Ctrl Pts',(70.4240634684271,11.5486366102045,76.3531516559179));
#134397=CARTESIAN_POINT('Ctrl Pts',(70.4394636545303,11.5457823417567,76.3540132419426));
#134398=CARTESIAN_POINT('Ctrl Pts',(70.4545216765585,11.542991489953,76.3548556850957));
#134399=CARTESIAN_POINT('Ctrl Pts',(70.4695994969117,11.5407791919864,76.3549658203571));
#134400=CARTESIAN_POINT('Ctrl Pts',(70.4847292631062,11.5391574455067,76.3543277140276));
#134401=CARTESIAN_POINT('Ctrl Pts',(70.4887566369168,11.5387257548106,76.3541578572905));
#134402=CARTESIAN_POINT('Ctrl Pts',(70.492787717123,11.5383360820643,76.3539347604712));
#134403=CARTESIAN_POINT('Ctrl Pts',(70.4968231425723,11.537989046077,76.3536576266829));
#134404=CARTESIAN_POINT('Ctrl Pts',(70.5119504136597,11.5366881405039,76.3526187577966));
#134405=CARTESIAN_POINT('Ctrl Pts',(70.5271393428903,11.5359838640424,76.3508236001816));
#134406=CARTESIAN_POINT('Ctrl Pts',(70.5424074352129,11.5358880698067,76.3482528518716));
#134407=CARTESIAN_POINT('Ctrl Pts',(70.5437998025831,11.535879333891,76.3480184135418));
#134408=CARTESIAN_POINT('Ctrl Pts',(70.5451928217474,11.5358756809335,76.3477774978885));
#134409=CARTESIAN_POINT('Ctrl Pts',(70.5465865013678,11.5358771335693,76.3475300739397));
#134410=CARTESIAN_POINT('',(69.083187826262,14.427762175719,70.9275690136187));
#134411=CARTESIAN_POINT('Origin',(68.3580209600691,-0.499074165591386,66.814943349163));
#134412=CARTESIAN_POINT('',(69.4827796255522,14.56707483593,70.3143821819286));
#134413=CARTESIAN_POINT('Ctrl Pts',(69.4827796254708,14.5670748341177,70.314382181467));
#134414=CARTESIAN_POINT('Ctrl Pts',(69.4361546598912,14.5670801487892,70.3225810935552));
#134415=CARTESIAN_POINT('Ctrl Pts',(69.3929252775548,14.5654384467918,70.3371198467491));
#134416=CARTESIAN_POINT('Ctrl Pts',(69.3523201741882,14.5622038470913,70.357789469697));
#134417=CARTESIAN_POINT('Ctrl Pts',(69.3464431011719,14.561735679865,70.3607811351088));
#134418=CARTESIAN_POINT('Ctrl Pts',(69.3406210002134,14.5612340569392,70.3639012146385));
#134419=CARTESIAN_POINT('Ctrl Pts',(69.3348515290093,14.5606990571707,70.3671490540045));
#134420=CARTESIAN_POINT('Ctrl Pts',(69.2892203485125,14.5564677038735,70.3928364591566));
#134421=CARTESIAN_POINT('Ctrl Pts',(69.2468815147492,14.5501525445106,70.4265166668452));
#134422=CARTESIAN_POINT('Ctrl Pts',(69.2107930600392,14.5419632084295,70.466287573233));
#134423=CARTESIAN_POINT('Ctrl Pts',(69.1747046053292,14.5337738723484,70.5060584796207));
#134424=CARTESIAN_POINT('Ctrl Pts',(69.1448663859906,14.5237071471177,70.5519192698477));
#134425=CARTESIAN_POINT('Ctrl Pts',(69.1225129952057,14.5120087061897,70.6020288875747));
#134426=CARTESIAN_POINT('Ctrl Pts',(69.1048716394728,14.5027762653526,70.6415755317713));
#134427=CARTESIAN_POINT('Ctrl Pts',(69.0918919799643,14.492523915542,70.6837676073393));
#134428=CARTESIAN_POINT('Ctrl Pts',(69.0838883173712,14.4816669226518,70.7266921111021));
#134429=CARTESIAN_POINT('Ctrl Pts',(69.0817505259648,14.4787670020429,70.738157316463));
#134430=CARTESIAN_POINT('Ctrl Pts',(69.0799677501241,14.4758242191456,70.7496748414087));
#134431=CARTESIAN_POINT('Ctrl Pts',(69.0785460067399,14.472847127587,70.7612083884841));
#134432=CARTESIAN_POINT('Ctrl Pts',(69.0718014080478,14.4587241233547,70.815922303375));
#134433=CARTESIAN_POINT('Ctrl Pts',(69.0731819728056,14.4438345223755,70.8709984930405));
#134434=CARTESIAN_POINT('Ctrl Pts',(69.0831878262661,14.4277621757181,70.9275690136177));
#134435=CARTESIAN_POINT('',(86.2245113351368,14.5670697090797,67.3623619192218));
#134436=CARTESIAN_POINT('',(86.2245112270591,14.56706714654,67.362361309341));
#134437=CARTESIAN_POINT('',(88.2224712053084,14.9706018766884,64.2964292184508));
#134438=CARTESIAN_POINT('Ctrl Pts',(88.2224711443474,14.9705962804753,64.2964288732062));
#134439=CARTESIAN_POINT('Ctrl Pts',(88.2354174097173,14.9659270873237,64.3698241832643));
#134440=CARTESIAN_POINT('Ctrl Pts',(88.2440702868443,14.9611459120881,64.4370977395704));
#134441=CARTESIAN_POINT('Ctrl Pts',(88.2498443108715,14.9565213241849,64.4979844054106));
#134442=CARTESIAN_POINT('Ctrl Pts',(88.2556032614391,14.9519088090647,64.55871212271));
#134443=CARTESIAN_POINT('Ctrl Pts',(88.2584984067044,14.9474520828081,64.6130864601102));
#134444=CARTESIAN_POINT('Ctrl Pts',(88.2599335408691,14.9433657903529,64.660846100787));
#134445=CARTESIAN_POINT('Ctrl Pts',(88.260279627699,14.9423803688941,64.6723634787769));
#134446=CARTESIAN_POINT('Ctrl Pts',(88.2605408080041,14.9414162521163,64.6834961810361));
#134447=CARTESIAN_POINT('Ctrl Pts',(88.2607367681307,14.940475995797,64.6942405386883));
#134448=CARTESIAN_POINT('Ctrl Pts',(88.2615381757232,14.9366306800897,64.73818116041));
#134449=CARTESIAN_POINT('Ctrl Pts',(88.2612428319285,14.9331827046254,64.7756951912911));
#134450=CARTESIAN_POINT('Ctrl Pts',(88.2605168109006,14.9302585107549,64.8068121861044));
#134451=CARTESIAN_POINT('Ctrl Pts',(88.2597778818599,14.9272823272991,64.8384824136122));
#134452=CARTESIAN_POINT('Ctrl Pts',(88.2585928411687,14.9248486301795,64.863526205497));
#134453=CARTESIAN_POINT('Ctrl Pts',(88.2576632884832,14.9230369568775,64.8819711113012));
#134454=CARTESIAN_POINT('Ctrl Pts',(88.2574282754275,14.9225789227226,64.8866344227448));
#134455=CARTESIAN_POINT('Ctrl Pts',(88.2572095893997,14.9221603881518,64.8908759129916));
#134456=CARTESIAN_POINT('Ctrl Pts',(88.2570185607416,14.9217821181808,64.8946959828093));
#134457=CARTESIAN_POINT('Ctrl Pts',(88.2565963132184,14.9209459946378,64.9031398206904));
#134458=CARTESIAN_POINT('Ctrl Pts',(88.2562712022575,14.9203072488869,64.9095280000816));
#134459=CARTESIAN_POINT('Ctrl Pts',(88.2560899903014,14.9198719047267,64.9138655813363));
#134460=CARTESIAN_POINT('Ctrl Pts',(88.2560673388069,14.9198174867067,64.9144077789932));
#134461=CARTESIAN_POINT('Ctrl Pts',(88.2560468972339,14.9197662418315,64.9149179318388));
#134462=CARTESIAN_POINT('Ctrl Pts',(88.256028723928,14.9197181776152,64.9153960459549));
#134463=CARTESIAN_POINT('Ctrl Pts',(88.256010550622,14.919670113399,64.9158741600709));
#134464=CARTESIAN_POINT('Ctrl Pts',(88.2558562461538,14.9192592168772,64.9199572610432));
#134465=CARTESIAN_POINT('Ctrl Pts',(88.2557457474718,14.9189792843175,64.9227300865272));
#134466=CARTESIAN_POINT('Ctrl Pts',(88.2555247501079,14.918419419198,64.9282757374953));
#134467=CARTESIAN_POINT('Ctrl Pts',(88.2552877605797,14.9178571301713,64.9338196072238));
#134468=CARTESIAN_POINT('Ctrl Pts',(88.2550348046356,14.9172924397025,64.9393616051558));
#134469=CARTESIAN_POINT('Ctrl Pts',(88.2545288927474,14.9161630587648,64.95044560102));
#134470=CARTESIAN_POINT('Ctrl Pts',(88.2539591151671,14.915024071526,64.9615221095362));
#134471=CARTESIAN_POINT('Ctrl Pts',(88.2533253068796,14.9138756948231,64.9725901620931));
#134472=CARTESIAN_POINT('Ctrl Pts',(88.2507900737295,14.9092821880115,65.0168623723205));
#134473=CARTESIAN_POINT('Ctrl Pts',(88.2472303467211,14.9045383476269,65.0609992727766));
#134474=CARTESIAN_POINT('Ctrl Pts',(88.2426573629239,14.8996570010548,65.1049540329731));
#134475=CARTESIAN_POINT('Ctrl Pts',(88.2335113953295,14.8898943079108,65.1928635533662));
#134476=CARTESIAN_POINT('Ctrl Pts',(88.2203306558311,14.8795792338678,65.2800557341386));
#134477=CARTESIAN_POINT('Ctrl Pts',(88.2033243438967,14.868814256945,65.3662407316185));
#134478=CARTESIAN_POINT('Ctrl Pts',(88.1863180319623,14.8580492800221,65.4524257290985));
#134479=CARTESIAN_POINT('Ctrl Pts',(88.1652121891123,14.8467374872076,65.538371625361));
#134480=CARTESIAN_POINT('Ctrl Pts',(88.1397815886332,14.8350748453393,65.6231584256026));
#134481=CARTESIAN_POINT('Ctrl Pts',(88.1143509881541,14.823412203471,65.7079452258441));
#134482=CARTESIAN_POINT('Ctrl Pts',(88.0845956189412,14.8113991791083,65.7915728670862));
#134483=CARTESIAN_POINT('Ctrl Pts',(88.0502920910252,14.7992858156939,65.8731317712184));
#134484=CARTESIAN_POINT('Ctrl Pts',(88.0159885631092,14.7871724522795,65.9546906753507));
#134485=CARTESIAN_POINT('Ctrl Pts',(87.9773977777193,14.7749447602975,66.034244508071));
#134486=CARTESIAN_POINT('Ctrl Pts',(87.934822257459,14.7627705061534,66.1114563460231));
#134487=CARTESIAN_POINT('Ctrl Pts',(87.9135344973288,14.7566833790813,66.1500622649992));
#134488=CARTESIAN_POINT('Ctrl Pts',(87.8912508018819,14.7506097358628,66.1880826405594));
#134489=CARTESIAN_POINT('Ctrl Pts',(87.8680103019539,14.744571231414,66.2254747634526));
#134490=CARTESIAN_POINT('Ctrl Pts',(87.8563900519898,14.7415519791896,66.2441708248993));
#134491=CARTESIAN_POINT('Ctrl Pts',(87.8445306010193,14.7385415169717,66.2627098238248));
#134492=CARTESIAN_POINT('Ctrl Pts',(87.8324369300872,14.7355425866634,66.2810863695465));
#134493=CARTESIAN_POINT('Ctrl Pts',(87.8263900946211,14.7340431215092,66.2902746424073));
#134494=CARTESIAN_POINT('Ctrl Pts',(87.8202847041712,14.732546539589,66.2994223020043));
#134495=CARTESIAN_POINT('Ctrl Pts',(87.8141213836461,14.731053185234,66.3085286732507));
#134496=CARTESIAN_POINT('Ctrl Pts',(87.8094988932523,14.7299331694678,66.3153584516855));
#134497=CARTESIAN_POINT('Ctrl Pts',(87.8048438171917,14.728814969226,66.3221650054258));
#134498=CARTESIAN_POINT('Ctrl Pts',(87.8001564201215,14.7276987301555,66.3289480490743));
#134499=CARTESIAN_POINT('Ctrl Pts',(87.7985939544314,14.7273266504653,66.3312090636238));
#134500=CARTESIAN_POINT('Ctrl Pts',(87.7958048109861,14.7266652022143,66.3352252043825));
#134501=CARTESIAN_POINT('Ctrl Pts',(87.7954582592733,14.7265831502223,66.3357232454002));
#134502=CARTESIAN_POINT('Ctrl Pts',(87.7892255990741,14.7251074622792,66.3446804091176));
#134503=CARTESIAN_POINT('Ctrl Pts',(87.7771203691377,14.7220802144287,66.3629316915066));
#134504=CARTESIAN_POINT('Ctrl Pts',(87.7582190801493,14.7175870837742,66.3897974811068));
#134505=CARTESIAN_POINT('Ctrl Pts',(87.7434896619196,14.7140856717483,66.4107334845367));
#134506=CARTESIAN_POINT('Ctrl Pts',(87.7246330858878,14.7096923853249,66.4369005971158));
#134507=CARTESIAN_POINT('Ctrl Pts',(87.7012115473724,14.7044267669997,66.4679728232031));
#134508=CARTESIAN_POINT('Ctrl Pts',(87.674473121858,14.6984154478336,66.5034454033777));
#134509=CARTESIAN_POINT('Ctrl Pts',(87.6416817796703,14.6912835176468,66.5452343893276));
#134510=CARTESIAN_POINT('Ctrl Pts',(87.6016632841941,14.6831867054477,66.5922686344081));
#134511=CARTESIAN_POINT('Ctrl Pts',(87.581654036456,14.6791382993481,66.6157857569484));
#134512=CARTESIAN_POINT('Ctrl Pts',(87.5598333021963,14.6748502795821,66.6406073953481));
#134513=CARTESIAN_POINT('Ctrl Pts',(87.5360298823028,14.6703529806913,66.666560780772));
#134514=CARTESIAN_POINT('Ctrl Pts',(87.5241281723561,14.6681043312459,66.6795374734839));
#134515=CARTESIAN_POINT('Ctrl Pts',(87.5117305795691,14.6658034992355,66.6927966415966));
#134516=CARTESIAN_POINT('Ctrl Pts',(87.4988146086698,14.6634551870718,66.7063137579672));
#134517=CARTESIAN_POINT('Ctrl Pts',(87.4923566232201,14.6622810309899,66.7130723161525));
#134518=CARTESIAN_POINT('Ctrl Pts',(87.4857690433586,14.6610950078844,66.7198953620615));
#134519=CARTESIAN_POINT('Ctrl Pts',(87.4790489920845,14.6598977774674,66.7267795971394));
#134520=CARTESIAN_POINT('Ctrl Pts',(87.4756889664475,14.6592991622588,66.7302217146783));
#134521=CARTESIAN_POINT('Ctrl Pts',(87.4722958229659,14.6586977454466,66.7336791295583));
#134522=CARTESIAN_POINT('Ctrl Pts',(87.468869200926,14.6580936125992,66.7371514217866));
#134523=CARTESIAN_POINT('Ctrl Pts',(87.465442578886,14.6574894797517,66.7406237140148));
#134524=CARTESIAN_POINT('Ctrl Pts',(87.4605108792611,14.6566259272614,66.7455857192466));
#134525=CARTESIAN_POINT('Ctrl Pts',(87.4584885375708,14.6562731534097,66.7476125064636));
#134526=CARTESIAN_POINT('Ctrl Pts',(87.4054627353892,14.647023422484,66.8007548703619));
#134527=CARTESIAN_POINT('Ctrl Pts',(87.3528925759193,14.6387686224732,66.8482170400251));
#134528=CARTESIAN_POINT('Ctrl Pts',(87.3017326677347,14.6314687994132,66.890577180893));
#134529=CARTESIAN_POINT('Ctrl Pts',(87.2904548578659,14.6298596093371,66.8999151494641));
#134530=CARTESIAN_POINT('Ctrl Pts',(87.2792455724829,14.6282966269739,66.9090051493782));
#134531=CARTESIAN_POINT('Ctrl Pts',(87.2681150271531,14.6267791040544,66.9178533143707));
#134532=CARTESIAN_POINT('Ctrl Pts',(87.2373038209364,14.6225783474673,66.9423465110782));
#134533=CARTESIAN_POINT('Ctrl Pts',(87.2070887730209,14.6187264164645,66.9649875047977));
#134534=CARTESIAN_POINT('Ctrl Pts',(87.1776452324069,14.6152048017754,66.9859073994173));
#134535=CARTESIAN_POINT('Ctrl Pts',(87.1629234620999,14.6134439944308,66.9963673467271));
#134536=CARTESIAN_POINT('Ctrl Pts',(87.1483941537617,14.611765699395,67.0063969940054));
#134537=CARTESIAN_POINT('Ctrl Pts',(87.1340767958401,14.61016726836,67.0160124828669));
#134538=CARTESIAN_POINT('Ctrl Pts',(87.1269181168793,14.6093680528425,67.0208202272977));
#134539=CARTESIAN_POINT('Ctrl Pts',(87.1198124253448,14.608588798866,67.0255244311162));
#134540=CARTESIAN_POINT('Ctrl Pts',(87.1127619828297,14.6078291613001,67.0301270865025));
#134541=CARTESIAN_POINT('Ctrl Pts',(87.1092367615721,14.6074493425172,67.0324284141957));
#134542=CARTESIAN_POINT('Ctrl Pts',(87.1057253525592,14.6070744275826,67.034704354724));
#134543=CARTESIAN_POINT('Ctrl Pts',(87.1022280339322,14.6067043722668,67.036955155796));
#134544=CARTESIAN_POINT('Ctrl Pts',(87.1004793746187,14.6065193446089,67.0380805563319));
#134545=CARTESIAN_POINT('Ctrl Pts',(87.098734237901,14.6063355318405,67.0391996720004));
#134546=CARTESIAN_POINT('Ctrl Pts',(87.0969926579404,14.6061529283869,67.0403125336566));
#134547=CARTESIAN_POINT('Ctrl Pts',(87.0952510779798,14.6059703249333,67.0414253953128));
#134548=CARTESIAN_POINT('Ctrl Pts',(87.092477517043,14.6056813486228,67.0431889842275));
#134549=CARTESIAN_POINT('Ctrl Pts',(87.09177862231,14.6056087403507,67.0436323873999));
#134550=CARTESIAN_POINT('Ctrl Pts',(87.0639156806064,14.6027140554189,67.0613096085345));
#134551=CARTESIAN_POINT('Ctrl Pts',(87.0183425494523,14.5983355081594,67.0885690084124));
#134552=CARTESIAN_POINT('Ctrl Pts',(86.9535310488286,14.5933892370839,67.1214652454699));
#134553=CARTESIAN_POINT('Ctrl Pts',(86.9142985945187,14.5903951025228,67.1413783797887));
#134554=CARTESIAN_POINT('Ctrl Pts',(86.8680167117813,14.5871934479021,67.1633571067526));
#134555=CARTESIAN_POINT('Ctrl Pts',(86.8143468322071,14.5839974444716,67.186528560568));
#134556=CARTESIAN_POINT('Ctrl Pts',(86.7417455207952,14.5796740876432,67.2178734778228));
#134557=CARTESIAN_POINT('Ctrl Pts',(86.6554329600215,14.5753575824665,67.2514350519375));
#134558=CARTESIAN_POINT('Ctrl Pts',(86.5547790289479,14.5721621883357,67.2826899772011));
#134559=CARTESIAN_POINT('Ctrl Pts',(86.4581051615004,14.5690931466663,67.3127090183829));
#134560=CARTESIAN_POINT('Ctrl Pts',(86.3482018854432,14.567063355292,67.3406014193676));
#134561=CARTESIAN_POINT('Ctrl Pts',(86.2245115502461,14.5670748341591,67.3623631391674));
#134562=CARTESIAN_POINT('',(88.0908006755043,14.9994907909963,63.5496885367596));
#134563=CARTESIAN_POINT('Origin',(88.0541760202691,-0.499074165591386,63.341979795825));
#134564=CARTESIAN_POINT('',(91.9155428748487,14.9991665202061,62.8752788267285));
#134565=CARTESIAN_POINT('Ctrl Pts',(91.9155428714327,14.9991665204673,62.8752788073534));
#134566=CARTESIAN_POINT('Ctrl Pts',(90.6406264262798,14.9978694380589,63.1000630531378));
#134567=CARTESIAN_POINT('Ctrl Pts',(89.3657116351699,14.9978694380387,63.3248649304237));
#134568=CARTESIAN_POINT('Ctrl Pts',(88.0907987597691,14.99868011451,63.549677672236));
#134569=CARTESIAN_POINT('',(94.5611372758984,0.791525290730867,77.8791831282366));
#134570=CARTESIAN_POINT('Ctrl Pts',(94.5611183165859,0.791951999546357,
77.8790756181347));
#134571=CARTESIAN_POINT('Ctrl Pts',(94.5585207580642,0.993626479914886,
77.8644747740234));
#134572=CARTESIAN_POINT('Ctrl Pts',(94.5463339987654,1.68049538207119,77.7953921430714));
#134573=CARTESIAN_POINT('Ctrl Pts',(94.5098935016048,2.87766921816737,77.5886537952174));
#134574=CARTESIAN_POINT('Ctrl Pts',(94.4423986509273,4.30232735919002,77.2059804831616));
#134575=CARTESIAN_POINT('Ctrl Pts',(94.3207402637469,6.15219286716509,76.5155669569138));
#134576=CARTESIAN_POINT('Ctrl Pts',(94.1113738053345,8.32212312656844,75.3288542270853));
#134577=CARTESIAN_POINT('Ctrl Pts',(93.6699846192174,11.3677656920828,72.8250722276183));
#134578=CARTESIAN_POINT('Ctrl Pts',(93.087946136268,13.5971623798519,69.524355250224));
#134579=CARTESIAN_POINT('Ctrl Pts',(92.4297040189939,14.7677508337306,65.7913701368731));
#134580=CARTESIAN_POINT('Ctrl Pts',(92.0866907650382,14.9860768541558,63.8460104975704));
#134581=CARTESIAN_POINT('Ctrl Pts',(91.9155428748487,14.9991665202061,62.8752788267284));
#134582=CARTESIAN_POINT('',(88.0594949212713,0.791921988601748,79.0254659908079));
#134583=CARTESIAN_POINT('',(91.3065552302825,0.793741304715882,78.4527675754261));
#134584=CARTESIAN_POINT('',(80.8776257882291,11.5357844058001,74.5260054838839));
#134585=CARTESIAN_POINT('Ctrl Pts',(88.0594324394305,0.791351947310389,
79.025455896363));
#134586=CARTESIAN_POINT('Ctrl Pts',(88.0477203701159,0.973879312121693,
79.0119992383338));
#134587=CARTESIAN_POINT('Ctrl Pts',(88.0320804261398,1.15611822191438,78.9959592578232));
#134588=CARTESIAN_POINT('Ctrl Pts',(88.0125470385509,1.33793703208646,78.9773660909821));
#134589=CARTESIAN_POINT('Ctrl Pts',(87.9931417220772,1.51856374295249,78.9588948306769));
#134590=CARTESIAN_POINT('Ctrl Pts',(87.9698935769308,1.69877638732119,78.9379035863993));
#134591=CARTESIAN_POINT('Ctrl Pts',(87.9427961451028,1.87842090265091,78.9144027844327));
#134592=CARTESIAN_POINT('Ctrl Pts',(87.9211783458309,2.02173777110342,78.8956543058732));
#134593=CARTESIAN_POINT('Ctrl Pts',(87.8971098401237,2.16469267454061,78.8753082141352));
#134594=CARTESIAN_POINT('Ctrl Pts',(87.8705704964911,2.30719242424511,78.853362054785));
#134595=CARTESIAN_POINT('Ctrl Pts',(87.8361333749774,2.49209832335759,78.824884991947));
#134596=CARTESIAN_POINT('Ctrl Pts',(87.7975366690727,2.67623903058067,78.7937140384208));
#134597=CARTESIAN_POINT('Ctrl Pts',(87.7548208470993,2.85957500628548,78.7599011198712));
#134598=CARTESIAN_POINT('Ctrl Pts',(87.7122905662646,3.04211464086624,78.7262350716643));
#134599=CARTESIAN_POINT('Ctrl Pts',(87.6656764501589,3.22385684472079,78.6899496925974));
#134600=CARTESIAN_POINT('Ctrl Pts',(87.6149908274805,3.4047205988487,78.6510856509235));
#134601=CARTESIAN_POINT('Ctrl Pts',(87.5721441382589,3.55761233924866,78.6182322414653));
#134602=CARTESIAN_POINT('Ctrl Pts',(87.5263873425785,3.709875733188,78.5835358498526));
#134603=CARTESIAN_POINT('Ctrl Pts',(87.4777157295167,3.86143569573502,78.5470172182685));
#134604=CARTESIAN_POINT('Ctrl Pts',(87.4198385260649,4.04166121602626,78.5035915716335));
#134605=CARTESIAN_POINT('Ctrl Pts',(87.3578374371053,4.220915970472,78.4575823211593));
#134606=CARTESIAN_POINT('Ctrl Pts',(87.2917265304253,4.39898836359106,78.4090258963552));
#134607=CARTESIAN_POINT('Ctrl Pts',(87.2195795766543,4.59331909295807,78.3560361808672));
#134608=CARTESIAN_POINT('Ctrl Pts',(87.1425377435868,4.78624112568613,78.3000124822576));
#134609=CARTESIAN_POINT('Ctrl Pts',(87.0606094891262,4.9776696797924,78.2410222443041));
#134610=CARTESIAN_POINT('Ctrl Pts',(87.0095176912571,5.09704765332733,78.2042349682465));
#134611=CARTESIAN_POINT('Ctrl Pts',(86.9565254694602,5.21584382961004,78.1662941261412));
#134612=CARTESIAN_POINT('Ctrl Pts',(86.9016348008891,5.33402749986044,78.1272179048115));
#134613=CARTESIAN_POINT('Ctrl Pts',(86.8162754043854,5.51781259542876,78.0664512434249));
#134614=CARTESIAN_POINT('Ctrl Pts',(86.7263296708448,5.70009605369247,78.0029471940521));
#134615=CARTESIAN_POINT('Ctrl Pts',(86.6318090499446,5.88075710407649,77.9367702818263));
#134616=CARTESIAN_POINT('Ctrl Pts',(86.6025492456507,5.9366825405306,77.9162845562559));
#134617=CARTESIAN_POINT('Ctrl Pts',(86.5728510453442,5.99245213998999,77.8955427711251));
#134618=CARTESIAN_POINT('Ctrl Pts',(86.5427148301024,6.0480613217974,77.8745470633363));
#134619=CARTESIAN_POINT('Ctrl Pts',(86.4789708368259,6.16568562474364,77.8301370322362));
#134620=CARTESIAN_POINT('Ctrl Pts',(86.4132669540331,6.28259506106173,77.7845898555511));
#134621=CARTESIAN_POINT('Ctrl Pts',(86.3456058938825,6.39875192413486,77.7379209342159));
#134622=CARTESIAN_POINT('Ctrl Pts',(86.3168914034263,6.44804741446146,77.7181152395771));
#134623=CARTESIAN_POINT('Ctrl Pts',(86.2878243493149,6.49720740280034,77.6981074633652));
#134624=CARTESIAN_POINT('Ctrl Pts',(86.2584050800181,6.54622874504472,77.6778986926338));
#134625=CARTESIAN_POINT('Ctrl Pts',(86.253163470472,6.55496284149277,77.6742981108344));
#134626=CARTESIAN_POINT('Ctrl Pts',(86.2479106800764,6.56369253576868,77.6706911487874));
#134627=CARTESIAN_POINT('Ctrl Pts',(86.2426466960718,6.57241782802459,77.6670778101688));
#134628=CARTESIAN_POINT('Ctrl Pts',(86.2252422795267,6.60126643789267,77.6551309557747));
#134629=CARTESIAN_POINT('Ctrl Pts',(86.2077156177023,6.63006680114151,77.6431144372659));
#134630=CARTESIAN_POINT('Ctrl Pts',(86.1900667695632,6.65881836985443,77.6310285888921));
#134631=CARTESIAN_POINT('Ctrl Pts',(86.1812423454936,6.67319415421089,77.6249856647052));
#134632=CARTESIAN_POINT('Ctrl Pts',(86.1723873748607,6.68755773998491,77.6189254081387));
#134633=CARTESIAN_POINT('Ctrl Pts',(86.1635018651202,6.70190905903075,77.6128478614586));
#134634=CARTESIAN_POINT('Ctrl Pts',(86.1555510918172,6.71475065030288,77.6074096595655));
#134635=CARTESIAN_POINT('Ctrl Pts',(86.1481823015576,6.72660935050173,77.602372145213));
#134636=CARTESIAN_POINT('Ctrl Pts',(86.1397676972441,6.7400973297256,77.5966226230958));
#134637=CARTESIAN_POINT('Ctrl Pts',(86.1387784302936,6.74168305040569,77.5959466777989));
#134638=CARTESIAN_POINT('Ctrl Pts',(86.1377746666064,6.74329125227717,77.5952608751832));
#134639=CARTESIAN_POINT('Ctrl Pts',(86.1367537260879,6.74492614805065,77.5945633936618));
#134640=CARTESIAN_POINT('Ctrl Pts',(86.00881390989,6.94980416100596,77.5071580492268));
#134641=CARTESIAN_POINT('Ctrl Pts',(85.8747726359394,7.15144056709324,77.4165864361061));
#134642=CARTESIAN_POINT('Ctrl Pts',(85.7346650950376,7.34973594036529,77.3230461454545));
#134643=CARTESIAN_POINT('Ctrl Pts',(85.5980353985829,7.54310909133311,77.2318277753671));
#134644=CARTESIAN_POINT('Ctrl Pts',(85.4556365520976,7.73330486201888,77.1377859535212));
#134645=CARTESIAN_POINT('Ctrl Pts',(85.3075056162184,7.92019078118287,77.0411321728384));
#134646=CARTESIAN_POINT('Ctrl Pts',(85.2388152472846,8.00685237323805,76.9963124745454));
#134647=CARTESIAN_POINT('Ctrl Pts',(85.1688923952485,8.09280168547449,76.9509315582908));
#134648=CARTESIAN_POINT('Ctrl Pts',(85.0977413507567,8.17802259737751,76.9050129474954));
#134649=CARTESIAN_POINT('Ctrl Pts',(84.9969947592835,8.29869147100831,76.839994316274));
#134650=CARTESIAN_POINT('Ctrl Pts',(84.8937705370257,8.41791117900397,76.7738927940239));
#134651=CARTESIAN_POINT('Ctrl Pts',(84.7881066860137,8.53565033322103,76.7067595560638));
#134652=CARTESIAN_POINT('Ctrl Pts',(84.693484094356,8.6410864289615,76.646641351954));
#134653=CARTESIAN_POINT('Ctrl Pts',(84.596905332987,8.74533506168276,76.5856957563942));
#134654=CARTESIAN_POINT('Ctrl Pts',(84.498353570467,8.84837818683794,76.5239687584006));
#134655=CARTESIAN_POINT('Ctrl Pts',(84.3940519360044,8.95743322653478,76.4586403805354));
#134656=CARTESIAN_POINT('Ctrl Pts',(84.2875543154507,9.06513757121163,76.3924346762747));
#134657=CARTESIAN_POINT('Ctrl Pts',(84.1788694032987,9.17147009623087,76.3254009623234));
#134658=CARTESIAN_POINT('Ctrl Pts',(84.1245269472227,9.22463635874049,76.2918841053477));
#134659=CARTESIAN_POINT('Ctrl Pts',(84.0696376676571,9.27745966607002,76.2581602424503));
#134660=CARTESIAN_POINT('Ctrl Pts',(84.0142026276105,9.32993746418419,76.2242354005939));
#134661=CARTESIAN_POINT('Ctrl Pts',(83.9864851075872,9.35617636324127,76.2072729796657));
#134662=CARTESIAN_POINT('Ctrl Pts',(83.958631147334,9.3823288843911,76.1902603133487));
#134663=CARTESIAN_POINT('Ctrl Pts',(83.9306408784229,9.4083947073915,76.1731981474495));
#134664=CARTESIAN_POINT('Ctrl Pts',(83.9091818797392,9.42837831180883,76.160117280069));
#134665=CARTESIAN_POINT('Ctrl Pts',(83.8882122260337,9.44778514997001,76.1473541205618));
#134666=CARTESIAN_POINT('Ctrl Pts',(83.8664227891014,9.46782515105231,76.1341113943047));
#134667=CARTESIAN_POINT('Ctrl Pts',(83.859790946544,9.473924534549,76.1300808323476));
#134668=CARTESIAN_POINT('Ctrl Pts',(83.8530829427933,9.48008228762863,76.1260058335305));
#134669=CARTESIAN_POINT('Ctrl Pts',(83.8462612763603,9.48633175977909,76.1218638914719));
#134670=CARTESIAN_POINT('Ctrl Pts',(83.6909822796265,9.62858611583186,76.0275824407875));
#134671=CARTESIAN_POINT('Ctrl Pts',(83.5339563944129,9.76553363640028,75.9337084657981));
#134672=CARTESIAN_POINT('Ctrl Pts',(83.3753719479445,9.89746523305497,75.8405159414567));
#134673=CARTESIAN_POINT('Ctrl Pts',(83.2891838353113,9.96916794770057,75.7898672936014));
#134674=CARTESIAN_POINT('Ctrl Pts',(83.2025346840625,10.0393887572179,75.7394193684984));
#134675=CARTESIAN_POINT('Ctrl Pts',(83.1154500868582,10.1081720505422,75.6892123862321));
#134676=CARTESIAN_POINT('Ctrl Pts',(82.9579334742314,10.2325856864502,75.5983991536893));
#134677=CARTESIAN_POINT('Ctrl Pts',(82.7989946428256,10.3522969956233,75.5083764411655));
#134678=CARTESIAN_POINT('Ctrl Pts',(82.6387110277812,10.4675211445887,75.419473812973));
#134679=CARTESIAN_POINT('Ctrl Pts',(82.4753962995857,10.5849242900358,75.3288899528878));
#134680=CARTESIAN_POINT('Ctrl Pts',(82.3106853535623,10.6976690143454,75.2394687192886));
#134681=CARTESIAN_POINT('Ctrl Pts',(82.1446200741637,10.8059675085606,75.1515243932705));
#134682=CARTESIAN_POINT('Ctrl Pts',(81.9734552235275,10.9175916581335,75.0608794524273));
#134683=CARTESIAN_POINT('Ctrl Pts',(81.8008515311353,11.0244924141495,74.9718033227587));
#134684=CARTESIAN_POINT('Ctrl Pts',(81.6268137343084,11.1268846371928,74.8846071328486));
#134685=CARTESIAN_POINT('Ctrl Pts',(81.5572992342724,11.1677823290862,74.8497790687317));
#134686=CARTESIAN_POINT('Ctrl Pts',(81.4875554957942,11.2079605398945,74.8152505821908));
#134687=CARTESIAN_POINT('Ctrl Pts',(81.4175811060443,11.247432161209,74.7810402061456));
#134688=CARTESIAN_POINT('Ctrl Pts',(81.256957695813,11.3380376876818,74.7025116575534));
#134689=CARTESIAN_POINT('Ctrl Pts',(81.0951223899492,11.4249207260478,74.6256609860501));
#134690=CARTESIAN_POINT('Ctrl Pts',(80.9320695380522,11.5081527096928,74.5508783706375));
#134691=CARTESIAN_POINT('Ctrl Pts',(80.9139367883308,11.5174087558808,74.5425619601423));
#134692=CARTESIAN_POINT('Ctrl Pts',(80.8957889348062,11.5266196385521,74.5342711021844));
#134693=CARTESIAN_POINT('Ctrl Pts',(80.8776259354588,11.5357854481567,74.5260063163204));
#134694=CARTESIAN_POINT('',(70.5465863094891,11.53587577156,76.347528985137));
#134695=CARTESIAN_POINT('Origin',(63.4339821949991,-0.499074165591486,67.683184237498));
#134696=CARTESIAN_POINT('',(65.1554518235812,13.43008177675,68.8079679196157));
#134697=CARTESIAN_POINT('Origin',(63.6783172724722,13.4301641189394,69.0684179803352));
#134698=CARTESIAN_POINT('',(67.333842554444,0.665543397954793,81.1622356683442));
#134699=CARTESIAN_POINT('Origin',(64.9111938245191,-0.499074165591386,67.422711970998));
#134700=CARTESIAN_POINT('Origin',(65.8566295019347,0.665611037261871,81.4226998345101));
#134701=CARTESIAN_POINT('Origin',(64.4693974219391,1.4210854715202E-14,
73.5553157898091));
#134702=CARTESIAN_POINT('',(67.3338425586293,-0.665543403176102,81.1622356920742));
#134703=CARTESIAN_POINT('Origin',(65.9466090514591,1.4210854715202E-14,
73.2948435233078));
#134704=CARTESIAN_POINT('Origin',(65.8566323754803,-0.665476912000534,81.4227161320649));
#134705=CARTESIAN_POINT('Origin',(64.4693974219391,1.4210854715202E-14,
73.5553157898091));
#134706=CARTESIAN_POINT('Origin',(62.8196722231591,1.4210854715202E-14,
73.84620685311));
#134707=CARTESIAN_POINT('',(94.5668566070113,1.85499763697787E-13,77.9116179430035));
#134708=CARTESIAN_POINT('Origin',(94.1728845515327,3.42614080963416,75.6787268466269));
#134709=CARTESIAN_POINT('',(94.5611364251491,-0.79152367744104,77.8791780069701));
#134710=CARTESIAN_POINT('Origin',(94.1728845250001,-3.42614191077933,75.6787266825563));
#134711=CARTESIAN_POINT('',(88.0594917515577,-0.791960232028162,79.0254638190457));
#134712=CARTESIAN_POINT('',(91.3040130871753,-0.793741771912361,78.4532214918126));
#134713=CARTESIAN_POINT('Origin',(82.8491886620102,-4.65600993454496E-7,
72.5661599447829));
#134714=CARTESIAN_POINT('Origin',(62.8196722231591,1.4210854715202E-14,
73.84620685311));
#134715=CARTESIAN_POINT('',(44.7346267930369,9.30978071375613E-8,86.6983316276));
#134716=CARTESIAN_POINT('Origin',(37.4857771329516,-0.268313559242106,83.3762268319904));
#134717=CARTESIAN_POINT('Origin',(37.5708463135294,0.26765030096014,83.4145770345828));
#134718=CARTESIAN_POINT('Ctrl Pts',(88.3300732516691,1.02797677064201,78.929837570272));
#134719=CARTESIAN_POINT('Ctrl Pts',(88.3504557367691,0.829610805066913,
78.9472771505469));
#134720=CARTESIAN_POINT('Ctrl Pts',(88.3844025449691,0.364027776906714,
78.976250751736));
#134721=CARTESIAN_POINT('Ctrl Pts',(88.3864239591691,-0.325044243107086,
78.977972504701));
#134722=CARTESIAN_POINT('Ctrl Pts',(88.3524181702692,-0.810557832525686,
78.948954580408));
#134723=CARTESIAN_POINT('Ctrl Pts',(88.3300322943691,-1.02835836804799,
78.9298017468989));
#134724=CARTESIAN_POINT('Ctrl Pts',(87.0482634675391,0.955316939249614,
79.392387743809));
#134725=CARTESIAN_POINT('Ctrl Pts',(87.0680695837392,0.771048317590214,
79.410443610716));
#134726=CARTESIAN_POINT('Ctrl Pts',(87.1010648505991,0.338398308666014,
79.440446636557));
#134727=CARTESIAN_POINT('Ctrl Pts',(87.1030300333491,-0.302162842145186,
79.442229937658));
#134728=CARTESIAN_POINT('Ctrl Pts',(87.0699766830691,-0.753349368884286,
79.412180128005));
#134729=CARTESIAN_POINT('Ctrl Pts',(87.0482237482091,-0.955671368820286,
79.392350572629));
#134730=CARTESIAN_POINT('Ctrl Pts',(85.9392714052091,0.783680110261714,
78.615892494063));
#134731=CARTESIAN_POINT('Ctrl Pts',(85.9549454524891,0.632390227145814,
78.632561950362));
#134732=CARTESIAN_POINT('Ctrl Pts',(85.9810378503591,0.277431166609014,
78.660241182834));
#134733=CARTESIAN_POINT('Ctrl Pts',(85.982590889989,-0.247718294763486,
78.6618849678071));
#134734=CARTESIAN_POINT('Ctrl Pts',(85.9564544208491,-0.617858911184986,
78.6341659430299));
#134735=CARTESIAN_POINT('Ctrl Pts',(85.9392398380891,-0.783971188810686,
78.615858527218));
#134736=CARTESIAN_POINT('Ctrl Pts',(85.9409580116291,0.658217438893014,
77.257024303179));
#134737=CARTESIAN_POINT('Ctrl Pts',(85.9524387298491,0.530897975386414,
77.271477122028));
#134738=CARTESIAN_POINT('Ctrl Pts',(85.9715146025091,0.232685512903214,
77.295444546582));
#134739=CARTESIAN_POINT('Ctrl Pts',(85.9726481316892,-0.207753685037586,
77.296865738237));
#134740=CARTESIAN_POINT('Ctrl Pts',(85.9535434649091,-0.518669073028486,
77.272869052471));
#134741=CARTESIAN_POINT('Ctrl Pts',(85.9409346167292,-0.658462558413086,
77.256995382944));
#134742=CARTESIAN_POINT('Ctrl Pts',(88.0595159253563,-0.790233462113526,
79.0256009152192));
#134743=CARTESIAN_POINT('Ctrl Pts',(88.0115976870962,-0.787497376323707,
79.0342820975747));
#134744=CARTESIAN_POINT('Ctrl Pts',(87.962523231512,-0.784546129529816,
79.0411633131422));
#134745=CARTESIAN_POINT('Ctrl Pts',(87.9124786883384,-0.781377432771924,
79.0460185829796));
#134746=CARTESIAN_POINT('Ctrl Pts',(87.8636188139199,-0.778283746310966,
79.0507589174792));
#134747=CARTESIAN_POINT('Ctrl Pts',(87.8138344699327,-0.774982752994071,
79.0535674336194));
#134748=CARTESIAN_POINT('Ctrl Pts',(87.7633439937735,-0.771476934775263,
79.0542538663812));
#134749=CARTESIAN_POINT('Ctrl Pts',(87.7134935528966,-0.768015557558482,
79.0549315976764));
#134750=CARTESIAN_POINT('Ctrl Pts',(87.6629550882688,-0.764354492275542,
79.0535400629856));
#134751=CARTESIAN_POINT('Ctrl Pts',(87.611979293738,-0.76050108358359,79.0499255435374));
#134752=CARTESIAN_POINT('Ctrl Pts',(87.5618006799654,-0.756707936105629,
79.0463675494535));
#134753=CARTESIAN_POINT('Ctrl Pts',(87.5111987980573,-0.752728411193017,
79.0406550275279));
#134754=CARTESIAN_POINT('Ctrl Pts',(87.4604462803083,-0.748574534984207,
79.0326786585723));
#134755=CARTESIAN_POINT('Ctrl Pts',(87.4352918048017,-0.746515748898587,
79.0287253300199));
#134756=CARTESIAN_POINT('Ctrl Pts',(87.41010080336,-0.744414212157575,79.0242165199435));
#134757=CARTESIAN_POINT('Ctrl Pts',(87.3849089575827,-0.742271852738476,
79.0191429675415));
#134758=CARTESIAN_POINT('Ctrl Pts',(87.3348606636315,-0.738015656709632,
79.0090634106785));
#134759=CARTESIAN_POINT('Ctrl Pts',(87.2848081894561,-0.733598098828918,
78.9967517500166));
#134760=CARTESIAN_POINT('Ctrl Pts',(87.2350455907678,-0.729037222401108,
78.9821710322096));
#134761=CARTESIAN_POINT('Ctrl Pts',(87.1832191844151,-0.724287192432773,
78.9669856072942));
#134762=CARTESIAN_POINT('Ctrl Pts',(87.1317079557453,-0.719381712102373,
78.9493383050321));
#134763=CARTESIAN_POINT('Ctrl Pts',(87.080855677245,-0.714346282895627,
78.9292470049815));
#134764=CARTESIAN_POINT('Ctrl Pts',(87.0328008475358,-0.709587859081028,
78.9102609530083));
#134765=CARTESIAN_POINT('Ctrl Pts',(86.9853352518275,-0.704713477305003,
78.8890928356417));
#134766=CARTESIAN_POINT('Ctrl Pts',(86.938747481068,-0.699748338979591,
78.8658102316267));
#134767=CARTESIAN_POINT('Ctrl Pts',(86.892300276527,-0.694798181639693,
78.8425978766823));
#134768=CARTESIAN_POINT('Ctrl Pts',(86.8467263411344,-0.689757877297502,
78.8172839288121));
#134769=CARTESIAN_POINT('Ctrl Pts',(86.8022989455266,-0.684655114927824,
78.7899853926447));
#134770=CARTESIAN_POINT('Ctrl Pts',(86.7579230677471,-0.679558269700754,
78.7627185117495));
#134771=CARTESIAN_POINT('Ctrl Pts',(86.7146917516815,-0.674399182542361,
78.7334719678742));
#134772=CARTESIAN_POINT('Ctrl Pts',(86.6728539796854,-0.669207152221488,
78.7024087800593));
#134773=CARTESIAN_POINT('Ctrl Pts',(86.6309867960358,-0.664011471940562,
78.6713237550463));
#134774=CARTESIAN_POINT('Ctrl Pts',(86.590515699779,-0.658782877845103,
78.6384200104976));
#134775=CARTESIAN_POINT('Ctrl Pts',(86.5516572818512,-0.653551332452891,
78.603901378124));
#134776=CARTESIAN_POINT('Ctrl Pts',(86.5125912920345,-0.648291841461844,
78.5691983559037));
#134777=CARTESIAN_POINT('Ctrl Pts',(86.4751557303154,-0.643029443972041,
78.5328637427483));
#134778=CARTESIAN_POINT('Ctrl Pts',(86.4395293635135,-0.637794042230455,
78.4951374517933));
#134779=CARTESIAN_POINT('Ctrl Pts',(86.4037592935678,-0.632537522879708,
78.4572589874031));
#134780=CARTESIAN_POINT('Ctrl Pts',(86.3698133364644,-0.627308288868703,
78.4179782984031));
#134781=CARTESIAN_POINT('Ctrl Pts',(86.337825082915,-0.62213493953996,78.3775613343045));
#134782=CARTESIAN_POINT('Ctrl Pts',(86.3055413922718,-0.616913810194435,
78.3367710872319));
#134783=CARTESIAN_POINT('Ctrl Pts',(86.2752518803994,-0.611749666848358,
78.2948242271959));
#134784=CARTESIAN_POINT('Ctrl Pts',(86.2470423321364,-0.606669180465398,
78.252006638812));
#134785=CARTESIAN_POINT('Ctrl Pts',(86.2360595918244,-0.604691209670451,
78.2353365932791));
#134786=CARTESIAN_POINT('Ctrl Pts',(86.2253915644109,-0.602725885089282,
78.2185346388739));
#134787=CARTESIAN_POINT('Ctrl Pts',(86.2150411923762,-0.600774640746418,
78.2016177766988));
#134788=CARTESIAN_POINT('Ctrl Pts',(86.1880884478564,-0.59569352964312,
78.1575656534754));
#134789=CARTESIAN_POINT('Ctrl Pts',(86.1632933633963,-0.590708158946545,
78.1127349228115));
#134790=CARTESIAN_POINT('Ctrl Pts',(86.1406714482072,-0.585841286813566,
78.0674221018018));
#134791=CARTESIAN_POINT('Ctrl Pts',(86.1176168671584,-0.580881331075714,
78.0212426295609));
#134792=CARTESIAN_POINT('Ctrl Pts',(86.096819142508,-0.576044486020728,
77.9745631808592));
#134793=CARTESIAN_POINT('Ctrl Pts',(86.0782425606724,-0.571350078325953,
77.9276828680263));
#134794=CARTESIAN_POINT('Ctrl Pts',(86.0594470512591,-0.566600346389369,
77.8802500642441));
#134795=CARTESIAN_POINT('Ctrl Pts',(86.0429248803045,-0.561996439892889,
77.8326122452984));
#134796=CARTESIAN_POINT('Ctrl Pts',(86.0285916654781,-0.557553194866169,
77.785053992061));
#134797=CARTESIAN_POINT('Ctrl Pts',(86.0139578015265,-0.55301674969237,
77.7364981714669));
#134798=CARTESIAN_POINT('Ctrl Pts',(86.0016051422168,-0.548647776129665,
77.6880258181732));
#134799=CARTESIAN_POINT('Ctrl Pts',(85.9914024393367,-0.544456599778991,
77.6399048044329));
#134800=CARTESIAN_POINT('Ctrl Pts',(85.9865247883617,-0.542452905693841,
77.6168993800519));
#134801=CARTESIAN_POINT('Ctrl Pts',(85.9821379714158,-0.540489768759733,
77.5939736968655));
#134802=CARTESIAN_POINT('Ctrl Pts',(85.9782249940484,-0.538567898256704,
77.5711538245528));
#134803=CARTESIAN_POINT('Ctrl Pts',(88.0595203094199,0.790170290888587,
79.0256099738597));
#134804=CARTESIAN_POINT('Ctrl Pts',(88.0092098807286,0.78727734973052,79.0347261560292));
#134805=CARTESIAN_POINT('Ctrl Pts',(87.9580761965518,0.784180082109564,
79.0417740492722));
#134806=CARTESIAN_POINT('Ctrl Pts',(87.9063804748335,0.780885940482608,
79.0466121389104));
#134807=CARTESIAN_POINT('Ctrl Pts',(87.8551739204214,0.777622969450282,
79.0514044484494));
#134808=CARTESIAN_POINT('Ctrl Pts',(87.8034165227893,0.77416684437289,79.0540281564928));
#134809=CARTESIAN_POINT('Ctrl Pts',(87.7513891315324,0.770529824401712,
79.0543887488271));
#134810=CARTESIAN_POINT('Ctrl Pts',(87.6995895365358,0.766908728725948,
79.054747762347));
#134811=CARTESIAN_POINT('Ctrl Pts',(87.6475229935954,0.763108345196423,
79.0528631405066));
#134812=CARTESIAN_POINT('Ctrl Pts',(87.5954838982341,0.759145489286064,
79.0486898505836));
#134813=CARTESIAN_POINT('Ctrl Pts',(87.5435877275265,0.7551935173045,79.0445280225435));
#134814=CARTESIAN_POINT('Ctrl Pts',(87.4917195966933,0.751080007056776,
79.0380899585497));
#134815=CARTESIAN_POINT('Ctrl Pts',(87.4401779206803,0.746825818483686,
79.0293822268949));
#134816=CARTESIAN_POINT('Ctrl Pts',(87.3920138591992,0.742850414192706,
79.0212451278476));
#134817=CARTESIAN_POINT('Ctrl Pts',(87.344135423887,0.738752241542805,79.0111266002128));
#134818=CARTESIAN_POINT('Ctrl Pts',(87.2967824789059,0.734551054033569,
78.9990729707082));
#134819=CARTESIAN_POINT('Ctrl Pts',(87.2462388709382,0.730066788597694,
78.986207162161));
#134820=CARTESIAN_POINT('Ctrl Pts',(87.1962945801456,0.725465121249223,
78.9711363065946));
#134821=CARTESIAN_POINT('Ctrl Pts',(87.147228031733,0.720773238356931,78.9539651191248));
#134822=CARTESIAN_POINT('Ctrl Pts',(87.0978467927006,0.716051263852679,
78.9366838034352));
#134823=CARTESIAN_POINT('Ctrl Pts',(87.049355265712,0.711237986875821,78.9172754944996));
#134824=CARTESIAN_POINT('Ctrl Pts',(87.0020113270475,0.70636262969103,78.8958931161929));
#134825=CARTESIAN_POINT('Ctrl Pts',(86.9544627578656,0.701466200181208,
78.8744183187242));
#134826=CARTESIAN_POINT('Ctrl Pts',(86.9080722619709,0.696507230134741,
78.8509528929625));
#134827=CARTESIAN_POINT('Ctrl Pts',(86.863065762847,0.691515690155872,78.8256912702073));
#134828=CARTESIAN_POINT('Ctrl Pts',(86.8175405624627,0.686466622528131,
78.8001385064876));
#134829=CARTESIAN_POINT('Ctrl Pts',(86.7734318832503,0.681384306791206,
78.7727485405377));
#134830=CARTESIAN_POINT('Ctrl Pts',(86.7309299367083,0.676298961111208,
78.7437540428812));
#134831=CARTESIAN_POINT('Ctrl Pts',(86.6920888218353,0.671651632887533,
78.7172569361417));
#134832=CARTESIAN_POINT('Ctrl Pts',(86.6545891480054,0.667001800965946,
78.6894205862759));
#134833=CARTESIAN_POINT('Ctrl Pts',(86.6185412289497,0.662371180898521,
78.6604379072944));
#134834=CARTESIAN_POINT('Ctrl Pts',(86.5784683109295,0.657223520140154,
78.628219112167));
#134835=CARTESIAN_POINT('Ctrl Pts',(86.54019037328,0.652099710092061,78.5945842386416));
#134836=CARTESIAN_POINT('Ctrl Pts',(86.5038107624633,0.647027058822199,
78.5598100226415));
#134837=CARTESIAN_POINT('Ctrl Pts',(86.4666557946016,0.641846294358978,
78.5242946653055));
#134838=CARTESIAN_POINT('Ctrl Pts',(86.4314809103927,0.636718946712025,
78.4875916542119));
#134839=CARTESIAN_POINT('Ctrl Pts',(86.3983415904109,0.631670280497705,
78.4499961141552));
#134840=CARTESIAN_POINT('Ctrl Pts',(86.3647782353993,0.626557013943672,
78.411919519389));
#134841=CARTESIAN_POINT('Ctrl Pts',(86.3333025802584,0.621524486678621,
78.372928126645));
#134842=CARTESIAN_POINT('Ctrl Pts',(86.3039193424151,0.616594410867282,
78.3333173997979));
#134843=CARTESIAN_POINT('Ctrl Pts',(86.2738463955409,0.611548612009062,
78.2927768953621));
#134844=CARTESIAN_POINT('Ctrl Pts',(86.2459648711422,0.606610152131991,
78.2515883055234));
#134845=CARTESIAN_POINT('Ctrl Pts',(86.2202297511519,0.601797167259691,
78.2100460870321));
#134846=CARTESIAN_POINT('Ctrl Pts',(86.2038362292661,0.598731249056467,
78.1835832895677));
#134847=CARTESIAN_POINT('Ctrl Pts',(86.1883126817497,0.595716140142255,
78.1569764994874));
#134848=CARTESIAN_POINT('Ctrl Pts',(86.1736384964732,0.592755446686942,
78.130295614134));
#134849=CARTESIAN_POINT('Ctrl Pts',(86.1499235582225,0.587970672530877,
78.0871766581775));
#134850=CARTESIAN_POINT('Ctrl Pts',(86.1284286765579,0.58332836379019,78.0438664796944));
#134851=CARTESIAN_POINT('Ctrl Pts',(86.1090365218737,0.578839063866426,
78.0006310467195));
#134852=CARTESIAN_POINT('Ctrl Pts',(86.0889994335244,0.574200461263284,
77.9559577133822));
#134853=CARTESIAN_POINT('Ctrl Pts',(86.0712066149924,0.569725195969271,
77.9113645546615));
#134854=CARTESIAN_POINT('Ctrl Pts',(86.055496550876,0.565419402890934,77.8670996202735));
#134855=CARTESIAN_POINT('Ctrl Pts',(86.0394673054545,0.561026129033146,
77.821935355404));
#134856=CARTESIAN_POINT('Ctrl Pts',(86.0256055582469,0.556809238688697,
77.7771128860643));
#134857=CARTESIAN_POINT('Ctrl Pts',(86.0137178036998,0.552770126362036,
77.7328456993623));
#134858=CARTESIAN_POINT('Ctrl Pts',(86.0014595910415,0.548605143172438,
77.6871990142608));
#134859=CARTESIAN_POINT('Ctrl Pts',(85.9912995970003,0.54462914126965,77.6421427707851));
#134860=CARTESIAN_POINT('Ctrl Pts',(85.9830139446466,0.540838980814236,
77.5978574237659));
#134861=CARTESIAN_POINT('Ctrl Pts',(85.9813426232461,0.540074457272821,
77.5889245063513));
#134862=CARTESIAN_POINT('Ctrl Pts',(85.9797475481615,0.539317481949964,
77.5800227864653));
#134863=CARTESIAN_POINT('Ctrl Pts',(85.9782268654482,0.53856800990077,77.5711534942689));
#134864=CARTESIAN_POINT('Ctrl Pts',(80.848502459919,11.73661091945,74.241762346478));
#134865=CARTESIAN_POINT('Ctrl Pts',(81.1081094445191,11.633752433,74.322364138331));
#134866=CARTESIAN_POINT('Ctrl Pts',(82.0306236000289,11.23751074128,74.627356027073));
#134867=CARTESIAN_POINT('Ctrl Pts',(83.6166033891791,10.35667619639,75.2431312468769));
#134868=CARTESIAN_POINT('Ctrl Pts',(85.5127588197891,8.86506960620401,76.080446752923));
#134869=CARTESIAN_POINT('Ctrl Pts',(87.190145346969,6.95063939189201,76.8836477281941));
#134870=CARTESIAN_POINT('Ctrl Pts',(88.4365047595691,4.76169476788001,77.517745773655));
#134871=CARTESIAN_POINT('Ctrl Pts',(89.1412933993689,2.60934775846201,77.904463418106));
#134872=CARTESIAN_POINT('Ctrl Pts',(89.333960700069,1.21084850319901,78.032284899087));
#134873=CARTESIAN_POINT('Ctrl Pts',(89.368876214269,0.592587120183914,78.065563981149));
#134874=CARTESIAN_POINT('Ctrl Pts',(79.7312718086691,10.84772626501,76.16889230891));
#134875=CARTESIAN_POINT('Ctrl Pts',(79.9583593560691,10.78136985098,76.2474763667561));
#134876=CARTESIAN_POINT('Ctrl Pts',(80.780761401509,10.51543876535,76.547621989527));
#134877=CARTESIAN_POINT('Ctrl Pts',(82.2712335217692,9.85918473546302,77.171744493571));
#134878=CARTESIAN_POINT('Ctrl Pts',(84.1515576035891,8.62511070427802,78.045485899963));
#134879=CARTESIAN_POINT('Ctrl Pts',(85.8953437067791,6.91340464913602,78.905155887249));
#134880=CARTESIAN_POINT('Ctrl Pts',(87.2468356366392,4.83565870565902,79.600172027965));
#134881=CARTESIAN_POINT('Ctrl Pts',(88.0377922459692,2.70714470495302,80.031932373865));
#134882=CARTESIAN_POINT('Ctrl Pts',(88.2608915130691,1.29568079722601,80.175396060954));
#134883=CARTESIAN_POINT('Ctrl Pts',(88.3030331051691,0.670012739913314,
80.2125795690181));
#134884=CARTESIAN_POINT('Ctrl Pts',(79.0494024224791,8.66262403025101,75.453156756963));
#134885=CARTESIAN_POINT('Ctrl Pts',(79.2376340536491,8.60492377676502,75.5423376805901));
#134886=CARTESIAN_POINT('Ctrl Pts',(79.9168939222491,8.37610563642901,75.8785940986931));
#134887=CARTESIAN_POINT('Ctrl Pts',(81.1360155378491,7.82614458542902,76.554666819415));
#134888=CARTESIAN_POINT('Ctrl Pts',(82.6587891246792,6.81693899330302,77.47520250753));
#134889=CARTESIAN_POINT('Ctrl Pts',(84.0584024217591,5.44055771549901,78.36261756888));
#134890=CARTESIAN_POINT('Ctrl Pts',(85.1345531405991,3.79029526869902,79.067792236814));
#134891=CARTESIAN_POINT('Ctrl Pts',(85.7607667741192,2.11336906824801,79.499496090843));
#134892=CARTESIAN_POINT('Ctrl Pts',(85.9370342427891,1.00572501746301,79.641066725641));
#134893=CARTESIAN_POINT('Ctrl Pts',(85.9704058165791,0.514984673010614,
79.677294432062));
#134894=CARTESIAN_POINT('Ctrl Pts',(79.8524902757991,8.54481423012501,73.1962815772969));
#134895=CARTESIAN_POINT('Ctrl Pts',(80.055340106059,8.45459986811801,73.2923622975862));
#134896=CARTESIAN_POINT('Ctrl Pts',(80.7687653141991,8.11256935884601,73.6501015201404));
#134897=CARTESIAN_POINT('Ctrl Pts',(81.9583812039191,7.38699783676102,74.341760845944));
#134898=CARTESIAN_POINT('Ctrl Pts',(83.332259704859,6.22385841296701,75.247429141669));
#134899=CARTESIAN_POINT('Ctrl Pts',(84.5069102018391,4.79923984093301,76.091157573338));
#134900=CARTESIAN_POINT('Ctrl Pts',(85.3510764575991,3.23472385359101,76.740094262514));
#134901=CARTESIAN_POINT('Ctrl Pts',(85.815223686549,1.74201483404001,77.126729388828));
#134902=CARTESIAN_POINT('Ctrl Pts',(85.939483396599,0.787307726399214,77.2517856728581));
#134903=CARTESIAN_POINT('Ctrl Pts',(85.9615884733991,0.366136356086714,
77.283668607651));
#134904=CARTESIAN_POINT('',(80.3938476406748,10.4339876816843,75.1766107359184));
#134905=CARTESIAN_POINT('Ctrl Pts',(80.3938505465934,10.4339853760665,75.1766007796959));
#134906=CARTESIAN_POINT('Ctrl Pts',(80.3794956831756,10.4043236969974,75.1792779571772));
#134907=CARTESIAN_POINT('Ctrl Pts',(80.3681799513873,10.3731852311496,75.1822081054656));
#134908=CARTESIAN_POINT('Ctrl Pts',(80.3598138015333,10.3408757778269,75.185327398614));
#134909=CARTESIAN_POINT('Ctrl Pts',(80.3514342490384,10.3085145644937,75.1884516888957));
#134910=CARTESIAN_POINT('Ctrl Pts',(80.3460138121778,10.2749790675551,75.1917657423984));
#134911=CARTESIAN_POINT('Ctrl Pts',(80.3434557634103,10.2405725763164,75.1952574190916));
#134912=CARTESIAN_POINT('Ctrl Pts',(80.3419194802506,10.2199091262095,75.1973544096461));
#134913=CARTESIAN_POINT('Ctrl Pts',(80.3414154746935,10.1989314150935,75.1995164760688));
#134914=CARTESIAN_POINT('Ctrl Pts',(80.3419214521968,10.1777033896151,75.2017497411212));
#134915=CARTESIAN_POINT('Ctrl Pts',(80.3430222180311,10.1315213261305,75.2066082612192));
#134916=CARTESIAN_POINT('Ctrl Pts',(80.3488943629579,10.0841513673407,75.2118020083656));
#134917=CARTESIAN_POINT('Ctrl Pts',(80.3587399708604,10.0360620573974,75.2172498509544));
#134918=CARTESIAN_POINT('Ctrl Pts',(80.3684790861479,9.98849289373798,75.2226387682835));
#134919=CARTESIAN_POINT('Ctrl Pts',(80.3821062313102,9.94021889979879,75.2282775112244));
#134920=CARTESIAN_POINT('Ctrl Pts',(80.3988649310452,9.89164931798805,75.2341048459053));
#134921=CARTESIAN_POINT('Ctrl Pts',(80.4159555526203,9.84211776984164,75.2400475964407));
#134922=CARTESIAN_POINT('Ctrl Pts',(80.4361874576856,9.79236538991005,75.2461429831938));
#134923=CARTESIAN_POINT('Ctrl Pts',(80.4590421234356,9.74250323912191,75.2524219427782));
#134924=CARTESIAN_POINT('Ctrl Pts',(80.4828593033625,9.69054116582547,75.2589653379786));
#134925=CARTESIAN_POINT('Ctrl Pts',(80.5095245260965,9.63845899488816,75.265708498635));
#134926=CARTESIAN_POINT('Ctrl Pts',(80.5384695241847,9.58635298852964,75.2726459446336));
#134927=CARTESIAN_POINT('Ctrl Pts',(80.5677742386363,9.53359943045728,75.2796696063174));
#134928=CARTESIAN_POINT('Ctrl Pts',(80.5994156032385,9.48082042202425,75.286892562903));
#134929=CARTESIAN_POINT('Ctrl Pts',(80.6328241879231,9.42810235486638,75.2942615131889));
#134930=CARTESIAN_POINT('Ctrl Pts',(80.6596310629284,9.38580165131496,75.3001743206634));
#134931=CARTESIAN_POINT('Ctrl Pts',(80.6875761077926,9.34353977947596,75.3061801571795));
#134932=CARTESIAN_POINT('Ctrl Pts',(80.7163753358332,9.30136134543792,75.3122294516991));
#134933=CARTESIAN_POINT('Ctrl Pts',(80.7580602573791,9.24031093424897,75.3209853935981));
#134934=CARTESIAN_POINT('Ctrl Pts',(80.8016277183823,9.17937597468941,75.3298715087046));
#134935=CARTESIAN_POINT('Ctrl Pts',(80.8467191242501,9.11852787641061,75.3389213826274));
#134936=CARTESIAN_POINT('Ctrl Pts',(80.89237086256,9.05692364372325,75.3480837156287));
#134937=CARTESIAN_POINT('Ctrl Pts',(80.9395844286924,8.99540768739869,75.3574136933392));
#134938=CARTESIAN_POINT('Ctrl Pts',(80.9880017803453,8.93395060728147,75.3668943788865));
#134939=CARTESIAN_POINT('Ctrl Pts',(81.037189216702,8.87151604376801,75.3765258560544));
#134940=CARTESIAN_POINT('Ctrl Pts',(81.087618799575,8.8091415919427,75.3863125557427));
#134941=CARTESIAN_POINT('Ctrl Pts',(81.138933129947,8.74680748229801,75.396187602513));
#134942=CARTESIAN_POINT('Ctrl Pts',(81.1477877166934,8.73605136841898,75.3978915993813));
#134943=CARTESIAN_POINT('Ctrl Pts',(81.1566686948946,8.72529649517431,75.3995981175479));
#134944=CARTESIAN_POINT('Ctrl Pts',(81.1655742892056,8.71454281415756,75.4013066804546));
#134945=CARTESIAN_POINT('Ctrl Pts',(81.2271636357191,8.64017246184747,75.4131227669758));
#134946=CARTESIAN_POINT('Ctrl Pts',(81.2899742554949,8.56584216025802,75.4250668983327));
#134947=CARTESIAN_POINT('Ctrl Pts',(81.3537329467453,8.4914766887375,75.4371557885758));
#134948=CARTESIAN_POINT('Ctrl Pts',(81.4191635386663,8.41516118218237,75.4495616775417));
#134949=CARTESIAN_POINT('Ctrl Pts',(81.4855922124784,8.33880799469124,75.462119659779));
#134950=CARTESIAN_POINT('Ctrl Pts',(81.552738473848,8.26234763978692,75.4747959347963));
#134951=CARTESIAN_POINT('Ctrl Pts',(81.5917296022156,8.21794791518118,75.4821569144897));
#134952=CARTESIAN_POINT('Ctrl Pts',(81.6309630061373,8.17351233078151,75.4895568478986));
#134953=CARTESIAN_POINT('Ctrl Pts',(81.6703866518846,8.12903021326751,75.4969822402694));
#134954=CARTESIAN_POINT('Ctrl Pts',(81.6950453081994,8.1012075898865,75.5016266660956));
#134955=CARTESIAN_POINT('Ctrl Pts',(81.7197802155452,8.07336477096924,75.506281210966));
#134956=CARTESIAN_POINT('Ctrl Pts',(81.7445850781898,8.04549809771702,75.5109468154525));
#134957=CARTESIAN_POINT('Ctrl Pts',(81.8289357622139,7.95073551088164,75.5268125324072));
#134958=CARTESIAN_POINT('Ctrl Pts',(81.9140949701358,7.85569637818219,75.5428103106627));
#134959=CARTESIAN_POINT('Ctrl Pts',(81.9998081566341,7.76023375751805,75.5589691434916));
#134960=CARTESIAN_POINT('Ctrl Pts',(82.0877991469408,7.66223424457641,75.5755573927553));
#134961=CARTESIAN_POINT('Ctrl Pts',(82.1763735768846,7.56378785292534,75.5923148302763));
#134962=CARTESIAN_POINT('Ctrl Pts',(82.2652659129091,7.46475040757157,75.6092188800251));
#134963=CARTESIAN_POINT('Ctrl Pts',(82.3579357872776,7.36150430077359,75.6268412784972));
#134964=CARTESIAN_POINT('Ctrl Pts',(82.4509507670458,7.25761530954014,75.6446224383545));
#134965=CARTESIAN_POINT('Ctrl Pts',(82.5440266443157,7.15294479678162,75.6624874827657));
#134966=CARTESIAN_POINT('Ctrl Pts',(82.6089620675702,7.07992024683802,75.6749512301333));
#134967=CARTESIAN_POINT('Ctrl Pts',(82.673927494531,7.0065158574105,75.6874547530637));
#134968=CARTESIAN_POINT('Ctrl Pts',(82.7388322903256,6.93269290689744,75.6999617663264));
#134969=CARTESIAN_POINT('Ctrl Pts',(82.8448503955217,6.81210752892094,75.7203912250671));
#134970=CARTESIAN_POINT('Ctrl Pts',(82.9507217184122,6.69040801412927,75.7408568289677));
#134971=CARTESIAN_POINT('Ctrl Pts',(83.0562164481922,6.56736387199933,75.7613649477384));
#134972=CARTESIAN_POINT('Ctrl Pts',(83.0971173405337,6.51965897507221,75.7693160592273));
#134973=CARTESIAN_POINT('Ctrl Pts',(83.1379615312657,6.47175183804246,75.7772730197448));
#134974=CARTESIAN_POINT('Ctrl Pts',(83.1787353184465,6.42362861819271,75.7852341770899));
#134975=CARTESIAN_POINT('Ctrl Pts',(83.2876169880677,6.29512114103467,75.8064935244249));
#134976=CARTESIAN_POINT('Ctrl Pts',(83.3959975402901,6.1650728848407,75.8277865031236));
#134977=CARTESIAN_POINT('Ctrl Pts',(83.5035391676682,6.03323799801862,75.8490553375103));
#134978=CARTESIAN_POINT('Ctrl Pts',(83.6042434339213,5.90978500713803,75.8689719262136));
#134979=CARTESIAN_POINT('Ctrl Pts',(83.7042119487058,5.78476517016213,75.888866746447));
#134980=CARTESIAN_POINT('Ctrl Pts',(83.8031578769549,5.65797623157721,75.9086520659686));
#134981=CARTESIAN_POINT('Ctrl Pts',(80.8776258353147,11.5357847450604,74.5260057583377));
#134982=CARTESIAN_POINT('Ctrl Pts',(80.8241739589715,11.4290971482,74.6680655050188));
#134983=CARTESIAN_POINT('Ctrl Pts',(80.7695837405888,11.3036362609338,74.7920292317203));
#134984=CARTESIAN_POINT('Ctrl Pts',(80.7104997231134,11.1628322965241,74.8935242557125));
#134985=CARTESIAN_POINT('Ctrl Pts',(80.6942685092337,11.124151459318,74.9214063719351));
#134986=CARTESIAN_POINT('Ctrl Pts',(80.6776981555813,11.0843127079775,74.9475928168453));
#134987=CARTESIAN_POINT('Ctrl Pts',(80.6607375632814,11.0435148107972,74.9719321664642));
#134988=CARTESIAN_POINT('Ctrl Pts',(80.6194446553415,10.9441866869546,75.0311896797254));
#134989=CARTESIAN_POINT('Ctrl Pts',(80.5758387607439,10.8391735670981,75.0794984832658));
#134990=CARTESIAN_POINT('Ctrl Pts',(80.5291823535934,10.731343510345,75.1146733552099));
#134991=CARTESIAN_POINT('Ctrl Pts',(80.4869168772856,10.6336615629484,75.146537847304));
#134992=CARTESIAN_POINT('Ctrl Pts',(80.4421480523026,10.5336679203548,75.1676242054091));
#134993=CARTESIAN_POINT('Ctrl Pts',(80.3938476406443,10.4339876816213,75.1766107359241));
#134994=CARTESIAN_POINT('Ctrl Pts',(89.3691702808691,-0.592509543609686,
78.06499762776));
#134995=CARTESIAN_POINT('Ctrl Pts',(89.333364493069,-1.22675245987899,78.0308677484269));
#134996=CARTESIAN_POINT('Ctrl Pts',(89.1350209057691,-2.64413304960699,
77.899881169114));
#134997=CARTESIAN_POINT('Ctrl Pts',(88.4141708296692,-4.81338885261599,
77.50526087718));
#134998=CARTESIAN_POINT('Ctrl Pts',(87.1543010728991,-7.00151860831499,
76.865195019139));
#134999=CARTESIAN_POINT('Ctrl Pts',(85.4673513115891,-8.90801815554399,
76.05874833561));
#135000=CARTESIAN_POINT('Ctrl Pts',(83.5693396104491,-10.38775332569,75.222772426747));
#135001=CARTESIAN_POINT('Ctrl Pts',(81.9994121956191,-11.2524563877,74.615701488007));
#135002=CARTESIAN_POINT('Ctrl Pts',(81.0940117744891,-11.63968033551,74.317387098816));
#135003=CARTESIAN_POINT('Ctrl Pts',(80.848841500759,-11.73682984029,74.24126399703));
#135004=CARTESIAN_POINT('Ctrl Pts',(88.3037963433691,-0.670020240532286,
80.212989738538));
#135005=CARTESIAN_POINT('Ctrl Pts',(88.2605722655691,-1.31191574234599,
80.17485818836));
#135006=CARTESIAN_POINT('Ctrl Pts',(88.0309623922691,-2.74242877837699,
80.027804792461));
#135007=CARTESIAN_POINT('Ctrl Pts',(87.2224252329291,-4.88633006170198,
79.587339822944));
#135008=CARTESIAN_POINT('Ctrl Pts',(85.8573754622091,-6.96092439909799,
78.8861235752561));
#135009=CARTESIAN_POINT('Ctrl Pts',(84.1054574799991,-8.66266365324199,
78.023501439213));
#135010=CARTESIAN_POINT('Ctrl Pts',(82.2255471495491,-9.884161731605,77.151746893156));
#135011=CARTESIAN_POINT('Ctrl Pts',(80.7522513198091,-10.52642329792,76.536966540696));
#135012=CARTESIAN_POINT('Ctrl Pts',(79.9459230821792,-10.78575655111,76.243563881432));
#135013=CARTESIAN_POINT('Ctrl Pts',(79.7314542668592,-10.84842834365,76.16935458938));
#135014=CARTESIAN_POINT('Ctrl Pts',(85.9704220108091,-0.514982056589186,
79.677973373886));
#135015=CARTESIAN_POINT('Ctrl Pts',(85.9361932564492,-1.01843012321199,
79.640819503283));
#135016=CARTESIAN_POINT('Ctrl Pts',(85.7547895194892,-2.14099621798999,
79.495685929435));
#135017=CARTESIAN_POINT('Ctrl Pts',(85.1146074343491,-3.83019701732299,
79.055137172574));
#135018=CARTESIAN_POINT('Ctrl Pts',(84.0275042605191,-5.47826347261898,
78.343392903102));
#135019=CARTESIAN_POINT('Ctrl Pts',(82.6211065505191,-6.84703129507799,
77.452501919721));
#135020=CARTESIAN_POINT('Ctrl Pts',(81.0983702081792,-7.84636772488399,
76.53350254654));
#135021=CARTESIAN_POINT('Ctrl Pts',(79.8930386155091,-8.38493617109999,
75.866968193567));
#135022=CARTESIAN_POINT('Ctrl Pts',(79.2269700371691,-8.60816371974399,
75.5380273818501));
#135023=CARTESIAN_POINT('Ctrl Pts',(79.0492114403891,-8.66265061663799,
75.4538070962019));
#135024=CARTESIAN_POINT('Ctrl Pts',(85.961594855169,-0.366097390925386,
77.2836790921491));
#135025=CARTESIAN_POINT('Ctrl Pts',(85.9389255120391,-0.798156683534387,
77.250976980684));
#135026=CARTESIAN_POINT('Ctrl Pts',(85.8109804217291,-1.76582270548099,
77.1227940400109));
#135027=CARTESIAN_POINT('Ctrl Pts',(85.3359900028191,-3.27105037820099,
76.7280513880721));
#135028=CARTESIAN_POINT('Ctrl Pts',(84.4820233966991,-4.83629425178999,
76.072610788049));
#135029=CARTESIAN_POINT('Ctrl Pts',(83.2996589358591,-6.25653437109799,
75.224881302974));
#135030=CARTESIAN_POINT('Ctrl Pts',(81.9232512000892,-7.41183271016798,
74.319910758465));
#135031=CARTESIAN_POINT('Ctrl Pts',(80.7446490589091,-8.12510609244499,
73.6372601504587));
#135032=CARTESIAN_POINT('Ctrl Pts',(80.0440787679191,-8.45960257608299,
73.2870471296229));
#135033=CARTESIAN_POINT('Ctrl Pts',(79.852518768739,-8.54479915548399,73.1963043351081));
#135034=CARTESIAN_POINT('',(80.8778404067288,-11.5358771726413,74.525851299618));
#135035=CARTESIAN_POINT('Ctrl Pts',(80.8778403488691,-11.53587675694,74.525850965447));
#135036=CARTESIAN_POINT('Ctrl Pts',(81.3969169389546,-11.2739281687296,
74.7620470766188));
#135037=CARTESIAN_POINT('Ctrl Pts',(81.9044940104665,-10.9762832390086,
75.0181676961644));
#135038=CARTESIAN_POINT('Ctrl Pts',(82.6466403385913,-10.4673809179007,
75.4210629555873));
#135039=CARTESIAN_POINT('Ctrl Pts',(82.8908135114496,-10.2873411024514,
75.5584479718167));
#135040=CARTESIAN_POINT('Ctrl Pts',(83.2519588597215,-10.0006051938715,
75.7674482995734));
#135041=CARTESIAN_POINT('Ctrl Pts',(83.4312523337386,-9.85306899184976,
75.8726757764798));
#135042=CARTESIAN_POINT('Ctrl Pts',(83.6381171526523,-9.67342660579858,
75.9963039271245));
#135043=CARTESIAN_POINT('Ctrl Pts',(83.7262701415434,-9.59480336358862,
76.0494259686177));
#135044=CARTESIAN_POINT('Ctrl Pts',(83.7849260230865,-9.54202232590022,
76.0848662368444));
#135045=CARTESIAN_POINT('Ctrl Pts',(83.8150378412129,-9.51467944670708,
76.1031094855966));
#135046=CARTESIAN_POINT('Ctrl Pts',(84.2974032165774,-9.07288821655665,
76.3960663128352));
#135047=CARTESIAN_POINT('Ctrl Pts',(84.7160086697936,-8.63505965462778,
76.6588486116176));
#135048=CARTESIAN_POINT('Ctrl Pts',(85.2900464084644,-7.94763758112796,
77.0291165601318));
#135049=CARTESIAN_POINT('Ctrl Pts',(85.4724140397087,-7.7133904318713,77.1485556698116));
#135050=CARTESIAN_POINT('Ctrl Pts',(85.732400814426,-7.35471642757629,77.3211874942504));
#135051=CARTESIAN_POINT('Ctrl Pts',(85.8590030575354,-7.17355425421414,
77.4058718313578));
#135052=CARTESIAN_POINT('Ctrl Pts',(86.0007501877189,-6.95908918789543,
77.5016959600908));
#135053=CARTESIAN_POINT('Ctrl Pts',(86.0701322830086,-6.85109047841624,
77.5488497237172));
#135054=CARTESIAN_POINT('Ctrl Pts',(86.0995475883965,-6.80464234068808,
77.5688944119908));
#135055=CARTESIAN_POINT('Ctrl Pts',(86.1190866771446,-6.77364083372217,
77.58222090351));
#135056=CARTESIAN_POINT('Ctrl Pts',(86.129581954462,-6.7569024593158,77.5893859904182));
#135057=CARTESIAN_POINT('Ctrl Pts',(86.7104950006951,-5.82628527351812,
77.986299807247));
#135058=CARTESIAN_POINT('Ctrl Pts',(87.1575629529062,-4.85933241118305,
78.3065330622175));
#135059=CARTESIAN_POINT('Ctrl Pts',(87.7986061785262,-2.86235283752183,
78.7878566954693));
#135060=CARTESIAN_POINT('Ctrl Pts',(87.9926711462578,-1.8324008091606,78.9489796710299));
#135061=CARTESIAN_POINT('Ctrl Pts',(88.059439280893,-0.791398763418655,
79.0255044521198));
#135062=CARTESIAN_POINT('',(80.3938333635145,-10.4339884044026,75.1766012116704));
#135063=CARTESIAN_POINT('Ctrl Pts',(80.3938307448211,-10.4339904821502,
75.1766101838327));
#135064=CARTESIAN_POINT('Ctrl Pts',(80.4421453858671,-10.5336704769535,
75.1676281080308));
#135065=CARTESIAN_POINT('Ctrl Pts',(80.4869279350663,-10.633663298453,75.1465444690012));
#135066=CARTESIAN_POINT('Ctrl Pts',(80.5292078186286,-10.7313459535512,
75.1146810599036));
#135067=CARTESIAN_POINT('Ctrl Pts',(80.5758916995727,-10.8392035221319,
75.0794986641292));
#135068=CARTESIAN_POINT('Ctrl Pts',(80.6195243861941,-10.9442446065244,
75.0311738317282));
#135069=CARTESIAN_POINT('Ctrl Pts',(80.6608418244781,-11.0435938413397,
74.9718949947255));
#135070=CARTESIAN_POINT('Ctrl Pts',(80.6777947163431,-11.0843576666066,
74.9475723901468));
#135071=CARTESIAN_POINT('Ctrl Pts',(80.6943577989013,-11.1241631896455,
74.9214056769664));
#135072=CARTESIAN_POINT('Ctrl Pts',(80.7105818981162,-11.162811763929,74.893546047618));
#135073=CARTESIAN_POINT('Ctrl Pts',(80.769710077265,-11.3036651816639,74.7920125736594));
#135074=CARTESIAN_POINT('Ctrl Pts',(80.8243358251592,-11.4291518569876,
74.6679935591501));
#135075=CARTESIAN_POINT('Ctrl Pts',(80.8778405813924,-11.5358784198398,
74.525852301822));
#135076=CARTESIAN_POINT('Ctrl Pts',(83.8031819186192,-5.65795202609479,
75.9086537965711));
#135077=CARTESIAN_POINT('Ctrl Pts',(83.6949583155237,-5.79663127872643,
75.8870127524824));
#135078=CARTESIAN_POINT('Ctrl Pts',(83.5855117972911,-5.93319230169319,
75.8652409078052));
#135079=CARTESIAN_POINT('Ctrl Pts',(83.4752159873789,-6.06790048259671,
75.8434516164506));
#135080=CARTESIAN_POINT('Ctrl Pts',(83.3649201774668,-6.20260866350022,
75.821662325096));
#135081=CARTESIAN_POINT('Ctrl Pts',(83.2537750899658,-6.33546424712983,
75.7998557959442));
#135082=CARTESIAN_POINT('Ctrl Pts',(83.142141371957,-6.46673210215424,75.7780894655796));
#135083=CARTESIAN_POINT('Ctrl Pts',(83.0369680456649,-6.5904033118424,75.7575827816989));
#135084=CARTESIAN_POINT('Ctrl Pts',(82.9313605871511,-6.71266582993158,
75.7371116414454));
#135085=CARTESIAN_POINT('Ctrl Pts',(82.8255497425663,-6.83375266287503,
75.7166853181176));
#135086=CARTESIAN_POINT('Ctrl Pts',(82.7966651662695,-6.8668073263967,75.7111092762956));
#135087=CARTESIAN_POINT('Ctrl Pts',(82.7677653913127,-6.89977431904788,
75.7055362855964));
#135088=CARTESIAN_POINT('Ctrl Pts',(82.7388550041916,-6.93265823475957,
75.6999658762941));
#135089=CARTESIAN_POINT('Ctrl Pts',(82.6462278702881,-7.03801631423271,
75.6821186213894));
#135090=CARTESIAN_POINT('Ctrl Pts',(82.5534717057814,-7.14252558161222,
75.6642760957885));
#135091=CARTESIAN_POINT('Ctrl Pts',(82.4608543677029,-7.24630029078847,
75.6465407625238));
#135092=CARTESIAN_POINT('Ctrl Pts',(82.3706833984402,-7.3473339234269,75.6292738854589));
#135093=CARTESIAN_POINT('Ctrl Pts',(82.280644304359,-7.4476715982538,75.6121092748401));
#135094=CARTESIAN_POINT('Ctrl Pts',(82.1910024291584,-7.54744439154357,
75.5951053605184));
#135095=CARTESIAN_POINT('Ctrl Pts',(82.1051550617223,-7.64299383901446,
75.5788212156659));
#135096=CARTESIAN_POINT('Ctrl Pts',(82.0196723344532,-7.73802568404422,
75.5626848734953));
#135097=CARTESIAN_POINT('Ctrl Pts',(81.9347996244226,-7.8326731617615,75.5467064736755));
#135098=CARTESIAN_POINT('Ctrl Pts',(81.8590240022107,-7.91717584244927,
75.5324407198442));
#135099=CARTESIAN_POINT('Ctrl Pts',(81.7837349587665,-8.0013726371851,75.5183006467202));
#135100=CARTESIAN_POINT('Ctrl Pts',(81.7091125429145,-8.08536627130556,
75.5042595553665));
#135101=CARTESIAN_POINT('Ctrl Pts',(81.696182828616,-8.09991972256654,75.5018266764847));
#135102=CARTESIAN_POINT('Ctrl Pts',(81.6832731355542,-8.1144670855565,75.4993966830922));
#135103=CARTESIAN_POINT('Ctrl Pts',(81.6703843730783,-8.1290088775968,75.4969694336617));
#135104=CARTESIAN_POINT('Ctrl Pts',(81.6022415642135,-8.20589124372036,
75.4841365806772));
#135105=CARTESIAN_POINT('Ctrl Pts',(81.5346702893315,-8.28263226615724,
75.4713835484874));
#135106=CARTESIAN_POINT('Ctrl Pts',(81.4679410651791,-8.35929276064737,
75.458769962743));
#135107=CARTESIAN_POINT('Ctrl Pts',(81.4029018398334,-8.43401173482386,
75.4464758314075));
#135108=CARTESIAN_POINT('Ctrl Pts',(81.3386628796318,-8.50865474452786,
75.4343145697313));
#135109=CARTESIAN_POINT('Ctrl Pts',(81.2754907693696,-8.58329344530985,
75.4222975957938));
#135110=CARTESIAN_POINT('Ctrl Pts',(81.2384771239911,-8.62702556682338,
75.4152566403785));
#135111=CARTESIAN_POINT('Ctrl Pts',(81.2018300096906,-8.67075646661488,
75.4082643596455));
#135112=CARTESIAN_POINT('Ctrl Pts',(81.1656050134525,-8.71450187273681,
75.4013150054122));
#135113=CARTESIAN_POINT('Ctrl Pts',(81.1141320169016,-8.77666080640869,
75.391440495443));
#135114=CARTESIAN_POINT('Ctrl Pts',(81.063478630063,-8.8388587546476,75.381636850763));
#135115=CARTESIAN_POINT('Ctrl Pts',(81.0139956332105,-8.90111247007968,
75.3719783385541));
#135116=CARTESIAN_POINT('Ctrl Pts',(80.9650931467855,-8.96263585523153,
75.3624331353079));
#135117=CARTESIAN_POINT('Ctrl Pts',(80.9173339662622,-9.02421430425923,
75.3530300340532));
#135118=CARTESIAN_POINT('Ctrl Pts',(80.8710743650251,-9.08587610974556,
75.3437948427317));
#135119=CARTESIAN_POINT('Ctrl Pts',(80.8256376474274,-9.14644105123925,
75.3347239305575));
#135120=CARTESIAN_POINT('Ctrl Pts',(80.7816478632713,-9.20708711251621,
75.3258151868051));
#135121=CARTESIAN_POINT('Ctrl Pts',(80.739456477262,-9.26784327404333,75.3170446753161));
#135122=CARTESIAN_POINT('Ctrl Pts',(80.7317068667288,-9.27900281711263,
75.3154337292286));
#135123=CARTESIAN_POINT('Ctrl Pts',(80.724017962384,-9.29016606341629,75.3138273094398));
#135124=CARTESIAN_POINT('Ctrl Pts',(80.7163919846255,-9.30133316972677,
75.3122250801437));
#135125=CARTESIAN_POINT('Ctrl Pts',(80.6805114603629,-9.353874842625,75.3046865285043));
#135126=CARTESIAN_POINT('Ctrl Pts',(80.6459531886258,-9.40654633460277,
75.2972159848387));
#135127=CARTESIAN_POINT('Ctrl Pts',(80.6132706656793,-9.45926088566441,
75.2899059484022));
#135128=CARTESIAN_POINT('Ctrl Pts',(80.5807729794489,-9.5116773084414,75.282637254035));
#135129=CARTESIAN_POINT('Ctrl Pts',(80.5501300103034,-9.5641371706498,75.2755273211528));
#135130=CARTESIAN_POINT('Ctrl Pts',(80.5219072198447,-9.61655348817482,
75.2686204065309));
#135131=CARTESIAN_POINT('Ctrl Pts',(80.4941261501928,-9.66814942693174,
75.2618215934769));
#135132=CARTESIAN_POINT('Ctrl Pts',(80.4686902370224,-9.71970415366564,
75.255219285462));
#135133=CARTESIAN_POINT('Ctrl Pts',(80.446157482063,-9.77111939827723,75.2488114990542));
#135134=CARTESIAN_POINT('Ctrl Pts',(80.4430015386915,-9.77832063047093,
75.2479140228655));
#135135=CARTESIAN_POINT('Ctrl Pts',(80.4399025746111,-9.78551908723602,
75.247020294269));
#135136=CARTESIAN_POINT('Ctrl Pts',(80.4368621503838,-9.79271445619721,
75.246130241967));
#135137=CARTESIAN_POINT('Ctrl Pts',(80.4228985573425,-9.82576024074726,
75.2420425465659));
#135138=CARTESIAN_POINT('Ctrl Pts',(80.4101694983428,-9.85874141842604,
75.2380329443838));
#135139=CARTESIAN_POINT('Ctrl Pts',(80.3988281371886,-9.89162371531827,
75.2340908897384));
#135140=CARTESIAN_POINT('Ctrl Pts',(80.3819749010759,-9.94048673148717,
75.2282330057678));
#135141=CARTESIAN_POINT('Ctrl Pts',(80.3682876237009,-9.98907031929511,
75.2225640783406));
#135142=CARTESIAN_POINT('Ctrl Pts',(80.3585351980045,-10.0369369490896,
75.2171447714278));
#135143=CARTESIAN_POINT('Ctrl Pts',(80.3487958809904,-10.0847392391529,
75.2117327488538));
#135144=CARTESIAN_POINT('Ctrl Pts',(80.342980808203,-10.1318272875854,75.206568468694));
#135145=CARTESIAN_POINT('Ctrl Pts',(80.3418707948709,-10.1777210736054,
75.2017347817589));
#135146=CARTESIAN_POINT('Ctrl Pts',(80.3410240003497,-10.2127320103516,
75.1980473128833));
#135147=CARTESIAN_POINT('Ctrl Pts',(80.3429534869955,-10.2470637310563,
75.1945611852141));
#135148=CARTESIAN_POINT('Ctrl Pts',(80.3477336040891,-10.2804270866782,
75.191248594403));
#135149=CARTESIAN_POINT('Ctrl Pts',(80.3525057999656,-10.3137351552889,
75.1879414929452));
#135150=CARTESIAN_POINT('Ctrl Pts',(80.3601191070685,-10.3460775732638,
75.1848072246402));
#135151=CARTESIAN_POINT('Ctrl Pts',(80.370639260543,-10.3771592615142,75.1818691173166));
#135152=CARTESIAN_POINT('Ctrl Pts',(80.3772263692291,-10.3966208082636,
75.1800294452701));
#135153=CARTESIAN_POINT('Ctrl Pts',(80.3849529585172,-10.4155879636399,
75.178267714747));
#135154=CARTESIAN_POINT('Ctrl Pts',(80.393833729897,-10.4339881123427,75.1765999544888));
#135155=CARTESIAN_POINT('Ctrl Pts',(82.2802684813891,-4.44949575811698,
74.675770956836));
#135156=CARTESIAN_POINT('Ctrl Pts',(82.2515547398691,-4.47459854592499,
74.682359802912));
#135157=CARTESIAN_POINT('Ctrl Pts',(81.9823906719391,-4.70957506713498,
74.744877050762));
#135158=CARTESIAN_POINT('Ctrl Pts',(81.4784721044692,-5.14545068164199,
74.875238035718));
#135159=CARTESIAN_POINT('Ctrl Pts',(80.7929408853791,-5.76164297262998,
75.086564528771));
#135160=CARTESIAN_POINT('Ctrl Pts',(80.1708842271991,-6.36930087556499,
75.310730256588));
#135161=CARTESIAN_POINT('Ctrl Pts',(79.627849910789,-6.97242199968299,75.535523321951));
#135162=CARTESIAN_POINT('Ctrl Pts',(79.1658598934692,-7.58148319945498,
75.754792199969));
#135163=CARTESIAN_POINT('Ctrl Pts',(78.7839122270891,-8.21774497486598,
75.963729042074));
#135164=CARTESIAN_POINT('Ctrl Pts',(78.4905471606791,-8.91099832424997,
76.154488077099));
#135165=CARTESIAN_POINT('Ctrl Pts',(78.3164477158992,-9.69317749973099,
76.310267280487));
#135166=CARTESIAN_POINT('Ctrl Pts',(78.3332530958491,-10.5751191833,76.397661386524));
#135167=CARTESIAN_POINT('Ctrl Pts',(78.552159943209,-11.24208048039,76.382057866807));
#135168=CARTESIAN_POINT('Ctrl Pts',(78.7265238604091,-11.55499571287,76.348377280967));
#135169=CARTESIAN_POINT('Ctrl Pts',(78.7578974474891,-11.60737125339,76.341975098692));
#135170=CARTESIAN_POINT('Ctrl Pts',(83.1759968014491,-5.145175158979,74.314617629455));
#135171=CARTESIAN_POINT('Ctrl Pts',(83.1446436833991,-5.170233981977,74.314575250006));
#135172=CARTESIAN_POINT('Ctrl Pts',(82.8506132385191,-5.403970611904,74.315005581851));
#135173=CARTESIAN_POINT('Ctrl Pts',(82.2978958470191,-5.823239271777,74.330549238132));
#135174=CARTESIAN_POINT('Ctrl Pts',(81.5377842120691,-6.38454221490099,
74.390669473468));
#135175=CARTESIAN_POINT('Ctrl Pts',(80.8370587913791,-6.91472737682399,
74.483185378663));
#135176=CARTESIAN_POINT('Ctrl Pts',(80.2140754539491,-7.42515657005799,
74.599258127461));
#135177=CARTESIAN_POINT('Ctrl Pts',(79.6697283221492,-7.93290551323299,
74.731448452699));
#135178=CARTESIAN_POINT('Ctrl Pts',(79.2030231249391,-8.462495291134,74.8734975621001));
#135179=CARTESIAN_POINT('Ctrl Pts',(78.8228979343391,-9.04669161529399,
75.016582905033));
#135180=CARTESIAN_POINT('Ctrl Pts',(78.5624521075091,-9.721849384846,75.143445470533));
#135181=CARTESIAN_POINT('Ctrl Pts',(78.5012064800991,-10.50497709738,75.219507140925));
#135182=CARTESIAN_POINT('Ctrl Pts',(78.6770469362391,-11.10230153997,75.205989286091));
#135183=CARTESIAN_POINT('Ctrl Pts',(78.8330573272891,-11.37723786725,75.176271341392));
#135184=CARTESIAN_POINT('Ctrl Pts',(78.8613872357791,-11.42306524829,75.170636169063));
#135185=CARTESIAN_POINT('Ctrl Pts',(83.9722471046291,-5.62773758024599,
75.056136835834));
#135186=CARTESIAN_POINT('Ctrl Pts',(83.9438214655291,-5.65632355297999,
75.050655356093));
#135187=CARTESIAN_POINT('Ctrl Pts',(83.6770236031091,-5.92266876826999,
74.9996667050681));
#135188=CARTESIAN_POINT('Ctrl Pts',(83.1717502749291,-6.39475408463199,
74.9113173165371));
#135189=CARTESIAN_POINT('Ctrl Pts',(82.4700265622691,-7.00227131693099,
74.81064511086));
#135190=CARTESIAN_POINT('Ctrl Pts',(81.8180959209991,-7.54608119591799,
74.738536463235));
#135191=CARTESIAN_POINT('Ctrl Pts',(81.2363061342691,-8.034963233551,74.694203501958));
#135192=CARTESIAN_POINT('Ctrl Pts',(80.7264020875791,-8.48630143485999,
74.673073572076));
#135193=CARTESIAN_POINT('Ctrl Pts',(80.2885564578391,-8.91928079144999,
74.671182615835));
#135194=CARTESIAN_POINT('Ctrl Pts',(79.9302124268591,-9.35507338522099,
74.68366879445));
#135195=CARTESIAN_POINT('Ctrl Pts',(79.6752781953791,-9.81353295040099,
74.702418045188));
#135196=CARTESIAN_POINT('Ctrl Pts',(79.5756251446291,-10.30108863856,74.711599114768));
#135197=CARTESIAN_POINT('Ctrl Pts',(79.6608402008991,-10.64975679698,74.695800898555));
#135198=CARTESIAN_POINT('Ctrl Pts',(79.7520930242391,-10.80610135726,74.6798452933831));
#135199=CARTESIAN_POINT('Ctrl Pts',(79.7689255810191,-10.83203863183,74.676940461329));
#135200=CARTESIAN_POINT('Ctrl Pts',(83.9545624191291,-5.46419092780999,
76.234980550845));
#135201=CARTESIAN_POINT('Ctrl Pts',(83.9320043553292,-5.49671033498799,
76.230132474877));
#135202=CARTESIAN_POINT('Ctrl Pts',(83.7201028686891,-5.80025368320099,
76.184529837611));
#135203=CARTESIAN_POINT('Ctrl Pts',(83.3159460310292,-6.34718810348699,
76.0964325131561));
#135204=CARTESIAN_POINT('Ctrl Pts',(82.7531884472392,-7.06055624972298,
75.969657019754));
#135205=CARTESIAN_POINT('Ctrl Pts',(82.2337337008491,-7.69686316050198,
75.847662890942));
#135206=CARTESIAN_POINT('Ctrl Pts',(81.7773180167191,-8.25467658193697,
75.735167157942));
#135207=CARTESIAN_POINT('Ctrl Pts',(81.3877522714791,-8.74512160944298,
75.632045987688));
#135208=CARTESIAN_POINT('Ctrl Pts',(81.0664882854092,-9.17823841639897,
75.538316722994));
#135209=CARTESIAN_POINT('Ctrl Pts',(80.8189229673591,-9.55943980782899,
75.454461873142));
#135210=CARTESIAN_POINT('Ctrl Pts',(80.6564128816691,-9.88596265458298,
75.382908707838));
#135211=CARTESIAN_POINT('Ctrl Pts',(80.5924580838091,-10.14639820296,75.329671426931));
#135212=CARTESIAN_POINT('Ctrl Pts',(80.6208048058091,-10.2905041774,75.309272938575));
#135213=CARTESIAN_POINT('Ctrl Pts',(80.6590014868791,-10.35405375722,75.304530742518));
#135214=CARTESIAN_POINT('Ctrl Pts',(80.6661993264591,-10.3646059106,75.30386970992));
#135215=CARTESIAN_POINT('',(82.3561757813562,-4.7644135527838,74.6407035195125));
#135216=CARTESIAN_POINT('Ctrl Pts',(82.3561756416491,-4.76441355133499,
74.640702721084));
#135217=CARTESIAN_POINT('Ctrl Pts',(83.0512807828209,-5.28772211312453,
74.5181259705316));
#135218=CARTESIAN_POINT('Ctrl Pts',(83.6506984183361,-5.657776597521,75.0433097570123));
#135219=CARTESIAN_POINT('Ctrl Pts',(83.8031649527491,-5.65793925324699,
75.908656789893));
#135220=CARTESIAN_POINT('',(79.7232095658691,-10.75961935955,75.104974613695));
#135221=CARTESIAN_POINT('Ctrl Pts',(79.7232075621687,-10.7596193609995,
75.1049632444806));
#135222=CARTESIAN_POINT('Ctrl Pts',(79.7630725189922,-10.7392515715418,
75.0979348824883));
#135223=CARTESIAN_POINT('Ctrl Pts',(79.8035264705227,-10.7187747365093,
75.0928921008376));
#135224=CARTESIAN_POINT('Ctrl Pts',(79.8443296875199,-10.6983123783093,
75.0899236141334));
#135225=CARTESIAN_POINT('Ctrl Pts',(79.8849266519198,-10.6779534534863,
75.086970132572));
#135226=CARTESIAN_POINT('Ctrl Pts',(79.9258687109959,-10.6576092029207,
75.0860703188784));
#135227=CARTESIAN_POINT('Ctrl Pts',(79.9669032426091,-10.637405650997,75.0872629107693));
#135228=CARTESIAN_POINT('Ctrl Pts',(80.0078270615794,-10.6172566089834,
75.0884522850042));
#135229=CARTESIAN_POINT('Ctrl Pts',(80.048842150844,-10.5972478633285,75.0917228906908));
#135230=CARTESIAN_POINT('Ctrl Pts',(80.0896916129765,-10.5775035253354,
75.0970616829426));
#135231=CARTESIAN_POINT('Ctrl Pts',(80.1305204886073,-10.5577691377022,
75.1023977846557));
#135232=CARTESIAN_POINT('Ctrl Pts',(80.1711831903889,-10.5382992363802,
75.1097998906766));
#135233=CARTESIAN_POINT('Ctrl Pts',(80.2114275641653,-10.5192115693662,
75.1192034346234));
#135234=CARTESIAN_POINT('Ctrl Pts',(80.2518036430065,-10.5000614354236,
75.1286377529182));
#135235=CARTESIAN_POINT('Ctrl Pts',(80.2917579677754,-10.4812963575788,
75.140086349217));
#135236=CARTESIAN_POINT('Ctrl Pts',(80.3310508541424,-10.4630240216372,
75.1534349448914));
#135237=CARTESIAN_POINT('Ctrl Pts',(80.3521815758161,-10.4531976209625,
75.1606134824336));
#135238=CARTESIAN_POINT('Ctrl Pts',(80.3731213285904,-10.4435134999413,
75.1683406847968));
#135239=CARTESIAN_POINT('Ctrl Pts',(80.3938356163,-10.4339866196942,75.1765934966013));
#135240=CARTESIAN_POINT('Ctrl Pts',(82.3561757813562,-4.7644135527838,74.6407035195124));
#135241=CARTESIAN_POINT('Ctrl Pts',(82.3221239964285,-4.81104613577596,
74.6467080292841));
#135242=CARTESIAN_POINT('Ctrl Pts',(82.2819510045132,-4.86594979744543,
74.6537921579147));
#135243=CARTESIAN_POINT('Ctrl Pts',(82.2353302578256,-4.92949163792966,
74.6620132425268));
#135244=CARTESIAN_POINT('Ctrl Pts',(82.1963898194681,-4.98256558672512,
74.6688799845101));
#135245=CARTESIAN_POINT('Ctrl Pts',(82.1529502963756,-5.04166596062972,
74.6765400536491));
#135246=CARTESIAN_POINT('Ctrl Pts',(82.1048406200159,-5.10703723698665,
74.6850232781176));
#135247=CARTESIAN_POINT('Ctrl Pts',(82.0744718091815,-5.14830228127526,
74.6903782390868));
#135248=CARTESIAN_POINT('Ctrl Pts',(82.0422424927113,-5.19206666016719,
74.6960611264546));
#135249=CARTESIAN_POINT('Ctrl Pts',(82.0081167610943,-5.2384002206557,74.7020781786132));
#135250=CARTESIAN_POINT('Ctrl Pts',(81.9530318251687,-5.31319074058829,
74.7117907596162));
#135251=CARTESIAN_POINT('Ctrl Pts',(81.9029879776772,-5.38115981935113,
74.7206139398688));
#135252=CARTESIAN_POINT('Ctrl Pts',(81.8580159512924,-5.44231213731585,
74.728542600352));
#135253=CARTESIAN_POINT('Ctrl Pts',(81.8545255151115,-5.44705838248937,
74.7291579714091));
#135254=CARTESIAN_POINT('Ctrl Pts',(81.8510656072557,-5.45176355720081,
74.7297679581739));
#135255=CARTESIAN_POINT('Ctrl Pts',(81.8476362310092,-5.45642766055757,
74.7303725602019));
#135256=CARTESIAN_POINT('Ctrl Pts',(81.7897173888807,-5.5351998472664,74.7405837026627));
#135257=CARTESIAN_POINT('Ctrl Pts',(81.7405128536315,-5.60225686290772,
74.7492581479741));
#135258=CARTESIAN_POINT('Ctrl Pts',(81.6999946187848,-5.6575950026414,74.7564016288351));
#135259=CARTESIAN_POINT('Ctrl Pts',(81.6893579677409,-5.67212210343909,
74.758276900881));
#135260=CARTESIAN_POINT('Ctrl Pts',(81.6793196375855,-5.68584165827859,
74.7600467078884));
#135261=CARTESIAN_POINT('Ctrl Pts',(81.6698786644967,-5.69875383118292,
74.7617112172398));
#135262=CARTESIAN_POINT('Ctrl Pts',(81.6686886663476,-5.70038136064545,
74.7619210222068));
#135263=CARTESIAN_POINT('Ctrl Pts',(81.6683273437372,-5.7008754568627,74.7619847257784));
#135264=CARTESIAN_POINT('Ctrl Pts',(81.6663372235841,-5.70359793366945,
74.7623355989125));
#135265=CARTESIAN_POINT('Ctrl Pts',(81.5948817180262,-5.801348793734,74.7749337413662));
#135266=CARTESIAN_POINT('Ctrl Pts',(81.5267190804947,-5.89510372642465,
74.7869527340684));
#135267=CARTESIAN_POINT('Ctrl Pts',(81.4618889464816,-5.98487156474155,
74.7983854107181));
#135268=CARTESIAN_POINT('Ctrl Pts',(81.4078304522936,-6.0597243201739,74.8079185282048));
#135269=CARTESIAN_POINT('Ctrl Pts',(81.3560877708969,-6.13180382130643,
74.8170441209648));
#135270=CARTESIAN_POINT('Ctrl Pts',(81.306661090005,-6.20110051149391,74.8257610770255));
#135271=CARTESIAN_POINT('Ctrl Pts',(81.2481693983869,-6.28310643540894,
74.8360767505959));
#135272=CARTESIAN_POINT('Ctrl Pts',(81.1929221026482,-6.36121851360164,
74.8458198412785));
#135273=CARTESIAN_POINT('Ctrl Pts',(81.1409094522912,-6.43545153318075,
74.8549918064151));
#135274=CARTESIAN_POINT('Ctrl Pts',(81.1046125165828,-6.48725491410077,
74.8613924460018));
#135275=CARTESIAN_POINT('Ctrl Pts',(81.0698899954668,-6.53716790196466,
74.8675151243425));
#135276=CARTESIAN_POINT('Ctrl Pts',(81.0367299620014,-6.58518392843638,
74.8733620037368));
#135277=CARTESIAN_POINT('Ctrl Pts',(81.0340476590933,-6.58906792715362,
74.8738349556601));
#135278=CARTESIAN_POINT('Ctrl Pts',(81.032028582115,-6.59199285596816,74.8741909645567));
#135279=CARTESIAN_POINT('Ctrl Pts',(81.0287139553208,-6.5967987589946,74.8747754050657));
#135280=CARTESIAN_POINT('Ctrl Pts',(80.9667110097929,-6.68669730928631,
74.8857078675397));
#135281=CARTESIAN_POINT('Ctrl Pts',(80.9076641870499,-6.77336666141212,
74.8961180734007));
#135282=CARTESIAN_POINT('Ctrl Pts',(80.851588657655,-6.85680944092805,74.9060037059959));
#135283=CARTESIAN_POINT('Ctrl Pts',(80.8423562546751,-6.8705476503496,74.90763129908));
#135284=CARTESIAN_POINT('Ctrl Pts',(80.8332043271957,-6.8841983055889,74.9092446841864));
#135285=CARTESIAN_POINT('Ctrl Pts',(80.8241328663999,-6.89776131979979,
74.9108438639246));
#135286=CARTESIAN_POINT('Ctrl Pts',(80.77311800239,-6.97403517922627,74.9198371163572));
#135287=CARTESIAN_POINT('Ctrl Pts',(80.7246506285624,-7.04754099513986,
74.928380878209));
#135288=CARTESIAN_POINT('Ctrl Pts',(80.6787380567842,-7.11829359512274,
74.9364755325432));
#135289=CARTESIAN_POINT('Ctrl Pts',(80.626784219497,-7.19835595984763,74.9456352972413));
#135290=CARTESIAN_POINT('Ctrl Pts',(80.5781015087018,-7.27489212079903,
74.9542199644315));
#135291=CARTESIAN_POINT('Ctrl Pts',(80.532660148748,-7.34787246637765,74.9622340772334));
#135292=CARTESIAN_POINT('Ctrl Pts',(80.5296548706722,-7.35269904359167,
74.9627640930059));
#135293=CARTESIAN_POINT('Ctrl Pts',(80.5266637578906,-7.35751005453043,
74.9632916146101));
#135294=CARTESIAN_POINT('Ctrl Pts',(80.5236867969952,-7.36230548535573,
74.9638166439294));
#135295=CARTESIAN_POINT('Ctrl Pts',(80.5150756114505,-7.37617679440315,
74.9653353487574));
#135296=CARTESIAN_POINT('Ctrl Pts',(80.5073241553266,-7.38871501544494,
74.9667024535959));
#135297=CARTESIAN_POINT('Ctrl Pts',(80.4983501549054,-7.40330432530424,
74.9682851937703));
#135298=CARTESIAN_POINT('Ctrl Pts',(80.4977500467791,-7.40427993963376,
74.9683910345543));
#135299=CARTESIAN_POINT('Ctrl Pts',(80.4971444854725,-7.40526473955174,
74.9684978372034));
#135300=CARTESIAN_POINT('Ctrl Pts',(80.4965328545644,-7.40625974310928,
74.9686057104389));
#135301=CARTESIAN_POINT('Ctrl Pts',(80.46837446561,-7.45206792057731,74.9735720005396));
#135302=CARTESIAN_POINT('Ctrl Pts',(80.440705411131,-7.4978088530134,74.9784521857506));
#135303=CARTESIAN_POINT('Ctrl Pts',(80.4135176054478,-7.54347000097511,
74.9832471695868));
#135304=CARTESIAN_POINT('Ctrl Pts',(80.3685775476264,-7.61894555253318,
74.9911730336069));
#135305=CARTESIAN_POINT('Ctrl Pts',(80.3249538825194,-7.69420657960239,
74.9988656263258));
#135306=CARTESIAN_POINT('Ctrl Pts',(80.2826641860576,-7.76928408816456,
75.0063220008348));
#135307=CARTESIAN_POINT('Ctrl Pts',(80.2376597238191,-7.84918115959677,
75.0142570335521));
#135308=CARTESIAN_POINT('Ctrl Pts',(80.1941661592217,-7.92887004618887,
75.0219245605863));
#135309=CARTESIAN_POINT('Ctrl Pts',(80.1521764989142,-8.00833548164509,
75.029327703204));
#135310=CARTESIAN_POINT('Ctrl Pts',(80.1334129141781,-8.04384556724371,
75.0326358865235));
#135311=CARTESIAN_POINT('Ctrl Pts',(80.1149492620323,-8.07931039451579,
75.0358913599496));
#135312=CARTESIAN_POINT('Ctrl Pts',(80.0967831423889,-8.11472588878158,
75.0390947913165));
#135313=CARTESIAN_POINT('Ctrl Pts',(80.0906365109561,-8.12670896466862,
75.0401786943359));
#135314=CARTESIAN_POINT('Ctrl Pts',(80.0848331226111,-8.13808014782504,
75.0412021145088));
#135315=CARTESIAN_POINT('Ctrl Pts',(80.0786613749382,-8.15023621169719,
75.0422905554439));
#135316=CARTESIAN_POINT('Ctrl Pts',(80.0767917592039,-8.15391866429993,
75.0426202783046));
#135317=CARTESIAN_POINT('Ctrl Pts',(80.0748884873749,-8.15767325589699,
75.0429559423772));
#135318=CARTESIAN_POINT('Ctrl Pts',(80.072932208086,-8.16153915038168,75.0433009601853));
#135319=CARTESIAN_POINT('Ctrl Pts',(80.043613191896,-8.21947782183391,75.0484717876623));
#135320=CARTESIAN_POINT('Ctrl Pts',(80.0156502083981,-8.27609885371883,
75.0534042929127));
#135321=CARTESIAN_POINT('Ctrl Pts',(79.9890818078875,-8.33144904932179,
75.0580896385779));
#135322=CARTESIAN_POINT('Ctrl Pts',(79.9608350316895,-8.39029582058631,
75.0630709663158));
#135323=CARTESIAN_POINT('Ctrl Pts',(79.9341643577204,-8.4477054531432,75.0677730730202));
#135324=CARTESIAN_POINT('Ctrl Pts',(79.9090774098314,-8.50368695604994,
75.0721954540087));
#135325=CARTESIAN_POINT('Ctrl Pts',(79.8812033453984,-8.56588790715731,
75.0771091538802));
#135326=CARTESIAN_POINT('Ctrl Pts',(79.8552843213017,-8.6263251588515,75.0816776561257));
#135327=CARTESIAN_POINT('Ctrl Pts',(79.8312871038823,-8.68496473123229,
75.085910083439));
#135328=CARTESIAN_POINT('Ctrl Pts',(79.8254713788145,-8.69917603019671,
75.0869358120971));
#135329=CARTESIAN_POINT('Ctrl Pts',(79.8197683525908,-8.71328157761121,
75.0879418373131));
#135330=CARTESIAN_POINT('Ctrl Pts',(79.8141772391394,-8.72728060331489,
75.0889283496757));
#135331=CARTESIAN_POINT('Ctrl Pts',(79.8046653956645,-8.75109634993732,
75.0906066470777));
#135332=CARTESIAN_POINT('Ctrl Pts',(79.795477694382,-8.77460396542405,75.0922283974265));
#135333=CARTESIAN_POINT('Ctrl Pts',(79.7866194227751,-8.79780470966671,
75.0937919953709));
#135334=CARTESIAN_POINT('Ctrl Pts',(79.7802486673301,-8.81449038767148,
75.0949165149792));
#135335=CARTESIAN_POINT('Ctrl Pts',(79.7742737074603,-8.83041144080335,
75.0959711805973));
#135336=CARTESIAN_POINT('Ctrl Pts',(79.7682783263875,-8.8466781920646,75.0970293115271));
#135337=CARTESIAN_POINT('Ctrl Pts',(79.7644494819658,-8.8570666659696,75.0977050681902));
#135338=CARTESIAN_POINT('Ctrl Pts',(79.7606130668678,-8.86759659475772,
75.0983821064623));
#135339=CARTESIAN_POINT('Ctrl Pts',(79.7566703009177,-8.87856264167374,
75.0990778206578));
#135340=CARTESIAN_POINT('Ctrl Pts',(79.7351734430435,-8.93835202683703,
75.1028710128913));
#135341=CARTESIAN_POINT('Ctrl Pts',(79.7152579742709,-8.99804003517536,
75.1063816931034));
#135342=CARTESIAN_POINT('Ctrl Pts',(79.6969295737615,-9.05763451574551,
75.1096098269183));
#135343=CARTESIAN_POINT('Ctrl Pts',(79.6769678574295,-9.12253969475887,
75.113125632428));
#135344=CARTESIAN_POINT('Ctrl Pts',(79.6588885374546,-9.18733260356596,
75.1163064075041));
#135345=CARTESIAN_POINT('Ctrl Pts',(79.6426434504958,-9.25200807264128,
75.11917148176));
#135346=CARTESIAN_POINT('Ctrl Pts',(79.639742788396,-9.26355628302679,75.1196830587266));
#135347=CARTESIAN_POINT('Ctrl Pts',(79.6369004788179,-9.27510074573733,
75.120184613422));
#135348=CARTESIAN_POINT('Ctrl Pts',(79.6341160902083,-9.2866414416212,75.120676308863));
#135349=CARTESIAN_POINT('Ctrl Pts',(79.6263836928899,-9.31869057642894,
75.1220417736176));
#135350=CARTESIAN_POINT('Ctrl Pts',(79.61909868291,-9.35071065533344,75.1233309327924));
#135351=CARTESIAN_POINT('Ctrl Pts',(79.6123009130382,-9.38270283214319,
75.1245337281322));
#135352=CARTESIAN_POINT('Ctrl Pts',(79.6070714399134,-9.4073141726246,75.1254590295212));
#135353=CARTESIAN_POINT('Ctrl Pts',(79.6021955212803,-9.43153028046108,
75.1263217229009));
#135354=CARTESIAN_POINT('Ctrl Pts',(79.5975563075042,-9.4558487462413,75.1271417835214));
#135355=CARTESIAN_POINT('Ctrl Pts',(79.5932086114474,-9.47863909453801,
75.127910313384));
#135356=CARTESIAN_POINT('Ctrl Pts',(79.5890685290809,-9.50151949673387,
75.128641461581));
#135357=CARTESIAN_POINT('Ctrl Pts',(79.5850822443732,-9.52491545505902,
75.1293444826069));
#135358=CARTESIAN_POINT('Ctrl Pts',(79.5836856738333,-9.53311208639536,
75.1295907817365));
#135359=CARTESIAN_POINT('Ctrl Pts',(79.5823084003387,-9.541372138301,75.1298335565016));
#135360=CARTESIAN_POINT('Ctrl Pts',(79.5809495788261,-9.54971437395797,
75.1300729528898));
#135361=CARTESIAN_POINT('Ctrl Pts',(79.5721197715963,-9.60392335728163,
75.1316285832214));
#135362=CARTESIAN_POINT('Ctrl Pts',(79.5650408348773,-9.65723474203919,
75.132869710263));
#135363=CARTESIAN_POINT('Ctrl Pts',(79.5596463435658,-9.7097450737704,75.1338145482961));
#135364=CARTESIAN_POINT('Ctrl Pts',(79.5554914375936,-9.75018920062338,
75.134542274593));
#135365=CARTESIAN_POINT('Ctrl Pts',(79.5523341231431,-9.79015859311037,
75.1350947484855));
#135366=CARTESIAN_POINT('Ctrl Pts',(79.5501298052424,-9.82971155303763,
75.1354849314204));
#135367=CARTESIAN_POINT('Ctrl Pts',(79.5479574546926,-9.8686909099715,75.1358694558635));
#135368=CARTESIAN_POINT('Ctrl Pts',(79.5467119299754,-9.90726279713684,
75.1360958039005));
#135369=CARTESIAN_POINT('Ctrl Pts',(79.5464278727914,-9.94536583373473,
75.1361518654945));
#135370=CARTESIAN_POINT('Ctrl Pts',(79.5461164371936,-9.98714137275784,
75.1362133304988));
#135371=CARTESIAN_POINT('Ctrl Pts',(79.5469598782716,-10.0283533260274,
75.1360703538199));
#135372=CARTESIAN_POINT('Ctrl Pts',(79.5489855899427,-10.0689808890031,
75.1357154900053));
#135373=CARTESIAN_POINT('Ctrl Pts',(79.5511059017912,-10.1115057479858,
75.1353440541481));
#135374=CARTESIAN_POINT('Ctrl Pts',(79.5545202284435,-10.1533908886193,
75.13474085066));
#135375=CARTESIAN_POINT('Ctrl Pts',(79.5592581195504,-10.1946704171859,
75.1339011255562));
#135376=CARTESIAN_POINT('Ctrl Pts',(79.5641087126388,-10.2369318772835,
75.1330414255984));
#135377=CARTESIAN_POINT('Ctrl Pts',(79.5703452491432,-10.278559263329,75.1319342008308));
#135378=CARTESIAN_POINT('Ctrl Pts',(79.5780177252569,-10.3196387049876,
75.1305723363191));
#135379=CARTESIAN_POINT('Ctrl Pts',(79.5793401065986,-10.3267189078285,
75.1303376136307));
#135380=CARTESIAN_POINT('Ctrl Pts',(79.5807052148809,-10.3337829357129,
75.1300953139451));
#135381=CARTESIAN_POINT('Ctrl Pts',(79.5821134039448,-10.3408313516033,
75.1298453823846));
#135382=CARTESIAN_POINT('Ctrl Pts',(79.5890482516137,-10.375542379944,75.1286145552577));
#135383=CARTESIAN_POINT('Ctrl Pts',(79.5970246912381,-10.4098719194339,
75.1271993692909));
#135384=CARTESIAN_POINT('Ctrl Pts',(79.6059698498263,-10.4437654138459,
75.1256157332226));
#135385=CARTESIAN_POINT('Ctrl Pts',(79.6154126888406,-10.4795446354452,
75.1239439886356));
#135386=CARTESIAN_POINT('Ctrl Pts',(79.625934712514,-10.5148388029595,75.1220846122702));
#135387=CARTESIAN_POINT('Ctrl Pts',(79.6374969220201,-10.5496153933239,
75.1200456353118));
#135388=CARTESIAN_POINT('Ctrl Pts',(79.6495130050908,-10.5857571358272,
75.1179266184839));
#135389=CARTESIAN_POINT('Ctrl Pts',(79.6626522281328,-10.6213410362105,
75.1156137189209));
#135390=CARTESIAN_POINT('Ctrl Pts',(79.6769247672827,-10.6563478055494,
75.1131033722144));
#135391=CARTESIAN_POINT('Ctrl Pts',(79.6911973064326,-10.6913545748884,
75.110593025508));
#135392=CARTESIAN_POINT('Ctrl Pts',(79.7066031008277,-10.7257855013312,
75.1078852865875));
#135393=CARTESIAN_POINT('Ctrl Pts',(79.7232075620335,-10.759619360724,75.1049632445044));
#135394=CARTESIAN_POINT('Origin',(76.0272472665391,1.4210854715202E-14,
75.756664172774));
#135395=CARTESIAN_POINT('',(70.6107670387343,10.7594267271077,76.7115217636943));
#135396=CARTESIAN_POINT('',(70.610804188022,15.19124921296,76.7117292269897));
#135397=CARTESIAN_POINT('',(79.7231084232435,10.7594837524526,75.1049862577436));
#135398=CARTESIAN_POINT('',(70.6108041880485,10.75942685431,76.7117292269834));
#135399=CARTESIAN_POINT('',(82.3561326928982,4.76438284010808,74.6407108908467));
#135400=CARTESIAN_POINT('Ctrl Pts',(79.7231078884045,10.7594837533888,75.1049832214982));
#135401=CARTESIAN_POINT('Ctrl Pts',(79.7070082779656,10.726820962897,75.1078091201574));
#135402=CARTESIAN_POINT('Ctrl Pts',(79.6920518177104,10.6931496567333,75.1104327299098));
#135403=CARTESIAN_POINT('Ctrl Pts',(79.6781973871937,10.658469790198,75.1128661223029));
#135404=CARTESIAN_POINT('Ctrl Pts',(79.6648230633814,10.6249917079157,75.1152151887468));
#135405=CARTESIAN_POINT('Ctrl Pts',(79.6524756942354,10.5905725491408,75.1173869962559));
#135406=CARTESIAN_POINT('Ctrl Pts',(79.6411639813269,10.5552105178972,75.1193817573135));
#135407=CARTESIAN_POINT('Ctrl Pts',(79.633830050797,10.5322836028813,75.1206750573767));
#135408=CARTESIAN_POINT('Ctrl Pts',(79.6269323777341,10.5089603238528,75.1218937225791));
#135409=CARTESIAN_POINT('Ctrl Pts',(79.620484386902,10.4852436765249,75.1230352328094));
#135410=CARTESIAN_POINT('Ctrl Pts',(79.6114627338706,10.4520607256136,75.124632367405));
#135411=CARTESIAN_POINT('Ctrl Pts',(79.6032995916269,10.4180937995382,75.1260824053101));
#135412=CARTESIAN_POINT('Ctrl Pts',(79.5959883440864,10.3833556959088,75.1273839093862));
#135413=CARTESIAN_POINT('Ctrl Pts',(79.5912317856939,10.3607557473439,75.1282306431483));
#135414=CARTESIAN_POINT('Ctrl Pts',(79.5868366108061,10.3378294547095,75.1290143143681));
#135415=CARTESIAN_POINT('Ctrl Pts',(79.5828116799533,10.3145854786651,75.1297320293526));
#135416=CARTESIAN_POINT('Ctrl Pts',(79.5792932827944,10.2942667347497,75.1303594205936));
#135417=CARTESIAN_POINT('Ctrl Pts',(79.5760582626127,10.2737056656046,75.1309363036806));
#135418=CARTESIAN_POINT('Ctrl Pts',(79.5730919731977,10.2528807038193,75.131464874312));
#135419=CARTESIAN_POINT('Ctrl Pts',(79.5713315872362,10.2405218388381,75.1317785619496));
#135420=CARTESIAN_POINT('Ctrl Pts',(79.5696194381391,10.2277538194173,75.1320834751498));
#135421=CARTESIAN_POINT('Ctrl Pts',(79.5680312437019,10.2150153947845,75.1323661160601));
#135422=CARTESIAN_POINT('Ctrl Pts',(79.566395837817,10.2018983014856,75.1326571588929));
#135423=CARTESIAN_POINT('Ctrl Pts',(79.5648917760965,10.1888127234786,75.132924598392));
#135424=CARTESIAN_POINT('Ctrl Pts',(79.5635468212511,10.1762414066899,75.1331634348129));
#135425=CARTESIAN_POINT('Ctrl Pts',(79.563335072354,10.1742621859944,75.133201037078));
#135426=CARTESIAN_POINT('Ctrl Pts',(79.5631271639158,10.1722957169947,75.1332379487389));
#135427=CARTESIAN_POINT('Ctrl Pts',(79.5629230928202,10.1703438878504,75.1332741701308));
#135428=CARTESIAN_POINT('Ctrl Pts',(79.5589306391852,10.1321582381965,75.1339828066339));
#135429=CARTESIAN_POINT('Ctrl Pts',(79.555918953989,10.0939607728326,75.1345142386359));
#135430=CARTESIAN_POINT('Ctrl Pts',(79.5538527889503,10.0556979012006,75.1348750924712));
#135431=CARTESIAN_POINT('Ctrl Pts',(79.551752688671,10.0168065900539,75.1352418730652));
#135432=CARTESIAN_POINT('Ctrl Pts',(79.5506303572892,9.97784751617017,75.1354321980372));
#135433=CARTESIAN_POINT('Ctrl Pts',(79.5504708272491,9.93881356657663,75.1354515644425));
#135434=CARTESIAN_POINT('Ctrl Pts',(79.550311178441,9.89975055670353,75.135470945266));
#135435=CARTESIAN_POINT('Ctrl Pts',(79.5511167030462,9.86061244466846,75.1353188680087));
#135436=CARTESIAN_POINT('Ctrl Pts',(79.552880091036,9.82144305966724,75.1350029516353));
#135437=CARTESIAN_POINT('Ctrl Pts',(79.5530813947466,9.81697158623648,75.1349668874574));
#135438=CARTESIAN_POINT('Ctrl Pts',(79.5532951806317,9.81249976102359,75.1349286927825));
#135439=CARTESIAN_POINT('Ctrl Pts',(79.5535214357738,9.80802769258847,75.1348883829843));
#135440=CARTESIAN_POINT('Ctrl Pts',(79.5554633733376,9.76964413322029,75.1345424058251));
#135441=CARTESIAN_POINT('Ctrl Pts',(79.5583236194021,9.73124042997169,75.1340405635673));
#135442=CARTESIAN_POINT('Ctrl Pts',(79.5621872529113,9.69276973148076,75.1333629948776));
#135443=CARTESIAN_POINT('Ctrl Pts',(79.5643905906368,9.67083081281542,75.1329765936694));
#135444=CARTESIAN_POINT('Ctrl Pts',(79.5669372443528,9.64853832588428,75.1325300942824));
#135445=CARTESIAN_POINT('Ctrl Pts',(79.5697919943059,9.62631094002634,75.1320290018005));
#135446=CARTESIAN_POINT('Ctrl Pts',(79.5727801100865,9.60304515369211,75.131504499698));
#135447=CARTESIAN_POINT('Ctrl Pts',(79.5761056023998,9.57985087973573,75.1309201955627));
#135448=CARTESIAN_POINT('Ctrl Pts',(79.5796725514381,9.55719464793694,75.1302925377443));
#135449=CARTESIAN_POINT('Ctrl Pts',(79.5809847096477,9.54886019733674,75.1300616439608));
#135450=CARTESIAN_POINT('Ctrl Pts',(79.5823290394124,9.54059841602428,75.1298249768127));
#135451=CARTESIAN_POINT('Ctrl Pts',(79.5836991450315,9.53243203649979,75.1295836577841));
#135452=CARTESIAN_POINT('Ctrl Pts',(79.5912973542496,9.48714365922797,75.128245372296));
#135453=CARTESIAN_POINT('Ctrl Pts',(79.6001170930243,9.44123006425086,75.1266880721847));
#135454=CARTESIAN_POINT('Ctrl Pts',(79.6101544028514,9.3946257529472,75.1249135801248));
#135455=CARTESIAN_POINT('Ctrl Pts',(79.6190959753332,9.35310906823115,75.1233328030395));
#135456=CARTESIAN_POINT('Ctrl Pts',(79.6290041575734,9.31104459616811,75.1215795440022));
#135457=CARTESIAN_POINT('Ctrl Pts',(79.6398429807233,9.26838909153277,75.1196660781351));
#135458=CARTESIAN_POINT('Ctrl Pts',(79.6560516620485,9.20460084885738,75.1168046274003));
#135459=CARTESIAN_POINT('Ctrl Pts',(79.6743381454125,9.13949070888761,75.1135862443996));
#135460=CARTESIAN_POINT('Ctrl Pts',(79.6949050531781,9.07293568106988,75.109963852423));
#135461=CARTESIAN_POINT('Ctrl Pts',(79.7117269136601,9.01849971990908,75.1070010651563));
#135462=CARTESIAN_POINT('Ctrl Pts',(79.7300746113099,8.96309822499194,75.1037678757341));
#135463=CARTESIAN_POINT('Ctrl Pts',(79.7500221789991,8.90665503474601,75.1002492468614));
#135464=CARTESIAN_POINT('Ctrl Pts',(79.754463101825,8.89408909909735,75.0994658952508));
#135465=CARTESIAN_POINT('Ctrl Pts',(79.7589831423494,8.88147146004617,75.0986684496512));
#135466=CARTESIAN_POINT('Ctrl Pts',(79.7635827824328,8.86880112587223,75.0978568459067));
#135467=CARTESIAN_POINT('Ctrl Pts',(79.7773044742438,8.83100285958951,75.0954356615852));
#135468=CARTESIAN_POINT('Ctrl Pts',(79.7918795735844,8.79239252981469,75.092862743707));
#135469=CARTESIAN_POINT('Ctrl Pts',(79.8071842401293,8.75324530252362,75.0901616548501));
#135470=CARTESIAN_POINT('Ctrl Pts',(79.8125917316084,8.7394136847366,75.0892072978939));
#135471=CARTESIAN_POINT('Ctrl Pts',(79.8180899015046,8.72551478939534,75.0882370294827));
#135472=CARTESIAN_POINT('Ctrl Pts',(79.8236720223815,8.71155991451721,75.087252177119));
#135473=CARTESIAN_POINT('Ctrl Pts',(79.8415668027282,8.6668243335047,75.0840950049416));
#135474=CARTESIAN_POINT('Ctrl Pts',(79.8603273193853,8.62151576697663,75.0807874286856));
#135475=CARTESIAN_POINT('Ctrl Pts',(79.879771670602,8.57602561894005,75.0773597580627));
#135476=CARTESIAN_POINT('Ctrl Pts',(79.8911250151272,8.54946441782781,75.075358378584));
#135477=CARTESIAN_POINT('Ctrl Pts',(79.902710683486,8.52284070338079,75.0733162053902));
#135478=CARTESIAN_POINT('Ctrl Pts',(79.9144862264433,8.49622725323734,75.0712404748654));
#135479=CARTESIAN_POINT('Ctrl Pts',(79.948623841926,8.41907414607641,75.065222876292));
#135480=CARTESIAN_POINT('Ctrl Pts',(79.9840849050885,8.34254582030358,75.0589706569375));
#135481=CARTESIAN_POINT('Ctrl Pts',(80.020876997391,8.26665047317756,75.0524819528386));
#135482=CARTESIAN_POINT('Ctrl Pts',(80.0369322254888,8.23353147848552,75.0496504306868));
#135483=CARTESIAN_POINT('Ctrl Pts',(80.0532404759853,8.20053259600165,75.046774052383));
#135484=CARTESIAN_POINT('Ctrl Pts',(80.0698003682878,8.16765215996091,75.0438534924458));
#135485=CARTESIAN_POINT('Ctrl Pts',(80.075115914082,8.15709789666547,75.0429160243871));
#135486=CARTESIAN_POINT('Ctrl Pts',(80.08070748445,8.1460649251352,75.041929900323));
#135487=CARTESIAN_POINT('Ctrl Pts',(80.0860636261943,8.13555918782317,75.0409853404909));
#135488=CARTESIAN_POINT('Ctrl Pts',(80.0885538792637,8.13067471205022,75.040546182393));
#135489=CARTESIAN_POINT('Ctrl Pts',(80.0909930374926,8.12590404984408,75.040116044511));
#135490=CARTESIAN_POINT('Ctrl Pts',(80.0933287711423,8.12134760111213,75.0397041525492));
#135491=CARTESIAN_POINT('Ctrl Pts',(80.1259859114226,8.05764145660503,75.0339452709327));
#135492=CARTESIAN_POINT('Ctrl Pts',(80.1614580645366,7.99078064940021,75.0276914898257));
#135493=CARTESIAN_POINT('Ctrl Pts',(80.1997498623677,7.9207730884256,75.0209405741994));
#135494=CARTESIAN_POINT('Ctrl Pts',(80.2132341063598,7.89612031454328,75.0185632767459));
#135495=CARTESIAN_POINT('Ctrl Pts',(80.2270677787215,7.87107697126626,75.0161243674933));
#135496=CARTESIAN_POINT('Ctrl Pts',(80.2412502141385,7.84564198354711,75.0136238965939));
#135497=CARTESIAN_POINT('Ctrl Pts',(80.2537627413835,7.82320183363941,75.011417843167));
#135498=CARTESIAN_POINT('Ctrl Pts',(80.2669903513467,7.79967091032429,75.0090856555643));
#135499=CARTESIAN_POINT('Ctrl Pts',(80.2800178675766,7.77667701216853,75.0067886517101));
#135500=CARTESIAN_POINT('Ctrl Pts',(80.2858897676175,7.76631295894936,75.005753321814));
#135501=CARTESIAN_POINT('Ctrl Pts',(80.291720465817,7.75605752068295,75.0047252376859));
#135502=CARTESIAN_POINT('Ctrl Pts',(80.2974236300149,7.74605749375833,75.0037196216616));
#135503=CARTESIAN_POINT('Ctrl Pts',(80.3341362693609,7.68168491580153,74.997246229499));
#135504=CARTESIAN_POINT('Ctrl Pts',(80.3713257017052,7.61779994526875,74.9906878882944));
#135505=CARTESIAN_POINT('Ctrl Pts',(80.4089919611734,7.55440258182021,74.9840447954842));
#135506=CARTESIAN_POINT('Ctrl Pts',(80.4123996965283,7.54866690644703,74.9834437827329));
#135507=CARTESIAN_POINT('Ctrl Pts',(80.4158207173055,7.54291963320371,74.9828404221964));
#135508=CARTESIAN_POINT('Ctrl Pts',(80.4192525011407,7.53716499829019,74.9822351592188));
#135509=CARTESIAN_POINT('Ctrl Pts',(80.4421807333016,7.49871747023126,74.9781913118393));
#135510=CARTESIAN_POINT('Ctrl Pts',(80.4655926542994,7.4599444154685,74.9740619850969));
#135511=CARTESIAN_POINT('Ctrl Pts',(80.4887216130273,7.42210259000131,74.9699827347123));
#135512=CARTESIAN_POINT('Ctrl Pts',(80.5003949765524,7.40300352936788,74.9679239056396));
#135513=CARTESIAN_POINT('Ctrl Pts',(80.5119956206347,7.38414107161203,74.9658779424929));
#135514=CARTESIAN_POINT('Ctrl Pts',(80.5234215035191,7.36567331268513,74.9638628633655));
#135515=CARTESIAN_POINT('Ctrl Pts',(80.5691421296126,7.29177464689076,74.9557995320446));
#135516=CARTESIAN_POINT('Ctrl Pts',(80.6171836659155,7.21567229807172,74.9473280496147));
#135517=CARTESIAN_POINT('Ctrl Pts',(80.6675700432805,7.13739027779629,74.9384446819144));
#135518=CARTESIAN_POINT('Ctrl Pts',(80.7145949842145,7.06433070153476,74.9301539520933));
#135519=CARTESIAN_POINT('Ctrl Pts',(80.7636625121015,6.98937310146812,74.9215044753442));
#135520=CARTESIAN_POINT('Ctrl Pts',(80.8147666497352,6.91250481183277,74.9124953349109));
#135521=CARTESIAN_POINT('Ctrl Pts',(80.8709348331921,6.8280194375719,74.9025934546313));
#135522=CARTESIAN_POINT('Ctrl Pts',(80.9295626386359,6.74122532433875,74.8922569264201));
#135523=CARTESIAN_POINT('Ctrl Pts',(80.990643650238,6.65212799426251,74.8814869623144));
#135524=CARTESIAN_POINT('Ctrl Pts',(81.0034595898712,6.6334337065651,74.8792272222379));
#135525=CARTESIAN_POINT('Ctrl Pts',(81.0163834300284,6.61463787203028,74.8769484178491));
#135526=CARTESIAN_POINT('Ctrl Pts',(81.0294149479476,6.59574028291107,74.8746505893709));
#135527=CARTESIAN_POINT('Ctrl Pts',(81.0356148525333,6.58674952295774,74.8735573692712));
#135528=CARTESIAN_POINT('Ctrl Pts',(81.0429569835255,6.57611940119855,74.8722627305951));
#135529=CARTESIAN_POINT('Ctrl Pts',(81.0480881216829,6.56869910851812,74.8713579507368));
#135530=CARTESIAN_POINT('Ctrl Pts',(81.0952901848121,6.50043879028162,74.8630347532938));
#135531=CARTESIAN_POINT('Ctrl Pts',(81.1458682724802,6.42805597799933,74.8541157555898));
#135532=CARTESIAN_POINT('Ctrl Pts',(81.1998509741463,6.35155770879548,74.8445960348589));
#135533=CARTESIAN_POINT('Ctrl Pts',(81.2211447097429,6.32138259958922,74.8408409353559));
#135534=CARTESIAN_POINT('Ctrl Pts',(81.2429678750177,6.29056675285114,74.8369924256807));
#135535=CARTESIAN_POINT('Ctrl Pts',(81.2653208450812,6.25910868413534,74.8330504750036));
#135536=CARTESIAN_POINT('Ctrl Pts',(81.3236026068405,6.17708684716751,74.8227724748285));
#135537=CARTESIAN_POINT('Ctrl Pts',(81.3854886357688,6.09070017487662,74.811858887219));
#135538=CARTESIAN_POINT('Ctrl Pts',(81.4509817974625,5.99996393598028,74.8003102486381));
#135539=CARTESIAN_POINT('Ctrl Pts',(81.5116542981529,5.91590638898266,74.7896116540955));
#135540=CARTESIAN_POINT('Ctrl Pts',(81.5754228369729,5.82811668083589,74.7783680252541));
#135541=CARTESIAN_POINT('Ctrl Pts',(81.6422547371113,5.73658116761233,74.766584770311));
#135542=CARTESIAN_POINT('Ctrl Pts',(81.6475647858335,5.72930832284767,74.7656485458773));
#135543=CARTESIAN_POINT('Ctrl Pts',(81.6528941518874,5.72201181362249,74.7647089177965));
#135544=CARTESIAN_POINT('Ctrl Pts',(81.658242807361,5.71469162347861,74.7637658903752));
#135545=CARTESIAN_POINT('Ctrl Pts',(81.6601629436174,5.71206371772394,74.763427349007));
#135546=CARTESIAN_POINT('Ctrl Pts',(81.66326315078,5.70782163301846,74.7628807484576));
#135547=CARTESIAN_POINT('Ctrl Pts',(81.6640107439547,5.70679877827081,74.7627489396177));
#135548=CARTESIAN_POINT('Ctrl Pts',(81.6820712998922,5.68208837960556,74.7595646663972));
#135549=CARTESIAN_POINT('Ctrl Pts',(81.709573624922,5.64457759598908,74.7547157559832));
#135550=CARTESIAN_POINT('Ctrl Pts',(81.7465266716699,5.5942442761862,74.7482004881556));
#135551=CARTESIAN_POINT('Ctrl Pts',(81.7561074991364,5.58119434132866,74.7465112727201));
#135552=CARTESIAN_POINT('Ctrl Pts',(81.7663236195077,5.56728275206466,74.7447100391271));
#135553=CARTESIAN_POINT('Ctrl Pts',(81.7771750774218,5.5525096269153,74.7427967681625));
#135554=CARTESIAN_POINT('Ctrl Pts',(81.8076290683302,5.51104970304621,74.7374272835254));
#135555=CARTESIAN_POINT('Ctrl Pts',(81.8430884180969,5.4628038378542,74.7311751286016));
#135556=CARTESIAN_POINT('Ctrl Pts',(81.8835443613486,5.40778106533438,74.7240418188966));
#135557=CARTESIAN_POINT('Ctrl Pts',(81.9180946272034,5.36079040671102,74.7179498154251));
#135558=CARTESIAN_POINT('Ctrl Pts',(81.9571909747051,5.307630835837,74.7110561303366));
#135559=CARTESIAN_POINT('Ctrl Pts',(81.9983050426644,5.25174170406474,74.7038065921594));
#135560=CARTESIAN_POINT('Ctrl Pts',(82.0010104014637,5.2480641269742,74.7033295631795));
#135561=CARTESIAN_POINT('Ctrl Pts',(82.0037244899494,5.2443747138067,74.7028509946115));
#135562=CARTESIAN_POINT('Ctrl Pts',(82.0064465853113,5.24067443695834,74.7023710139139));
#135563=CARTESIAN_POINT('Ctrl Pts',(82.0581749918029,5.17035749375995,74.6932498651909));
#135564=CARTESIAN_POINT('Ctrl Pts',(82.1047779125546,5.10703436772081,74.6850323825771));
#135565=CARTESIAN_POINT('Ctrl Pts',(82.1462269620154,5.05066588751002,74.6777236571409));
#135566=CARTESIAN_POINT('Ctrl Pts',(82.1926906200799,4.98747780903283,74.6695307040099));
#135567=CARTESIAN_POINT('Ctrl Pts',(82.2326792188266,4.93302931311516,74.6624794640148));
#135568=CARTESIAN_POINT('Ctrl Pts',(82.2661944956993,4.88731790017762,74.6565696842625));
#135569=CARTESIAN_POINT('Ctrl Pts',(82.2922097950288,4.85183569023323,74.6519823824833));
#135570=CARTESIAN_POINT('Ctrl Pts',(82.3143258827971,4.82161901374268,74.648082639237));
#135571=CARTESIAN_POINT('Ctrl Pts',(82.3325496921101,4.79668191808424,74.6448692347889));
#135572=CARTESIAN_POINT('Ctrl Pts',(82.3413098557611,4.78469468560195,74.6433245550593));
#135573=CARTESIAN_POINT('Ctrl Pts',(82.349170640157,4.77392756708913,74.6419384647133));
#135574=CARTESIAN_POINT('Ctrl Pts',(82.3561326848172,4.76438284010716,74.6407108450246));
#135575=CARTESIAN_POINT('Origin',(76.0272472665991,1.4210854715202E-14,
75.756664173113));
#135576=CARTESIAN_POINT('',(70.6107884237591,-10.75942680297,76.71163854688));
#135577=CARTESIAN_POINT('',(79.7232081440958,-10.75961935955,75.1049665504179));
#135578=CARTESIAN_POINT('',(70.6108046249791,15.19124921296,76.7117291499424));
#135579=CARTESIAN_POINT('Origin',(76.6422369709091,1.4210854715202E-14,
79.244444102405));
#135580=CARTESIAN_POINT('Origin',(76.9027092374091,1.4210854715202E-14,
80.721655731923));
#135581=CARTESIAN_POINT('Ctrl Pts',(84.761279993589,1.01916108789501,82.134994479025));
#135582=CARTESIAN_POINT('Ctrl Pts',(84.7732730139091,0.938468758587613,
82.139847664892));
#135583=CARTESIAN_POINT('Ctrl Pts',(84.8096488123091,0.660239861587714,
82.154593658101));
#135584=CARTESIAN_POINT('Ctrl Pts',(84.8337698688191,0.312978103185414,
82.164415977497));
#135585=CARTESIAN_POINT('Ctrl Pts',(84.836850135019,0.0467873211332242,
82.165668020133));
#135586=CARTESIAN_POINT('Ctrl Pts',(84.8366553313491,-0.0200748059259058,
82.165588413034));
#135587=CARTESIAN_POINT('Ctrl Pts',(84.5809173493991,0.995359843725814,
82.174776982057));
#135588=CARTESIAN_POINT('Ctrl Pts',(84.5926714924792,0.916555418610414,
82.1796767163611));
#135589=CARTESIAN_POINT('Ctrl Pts',(84.6283234134691,0.644831872479714,
82.194563930964));
#135590=CARTESIAN_POINT('Ctrl Pts',(84.6519656862891,0.305675624410314,
82.204479935355));
#135591=CARTESIAN_POINT('Ctrl Pts',(84.6549847954192,0.0456956593620242,
82.2057439237761));
#135592=CARTESIAN_POINT('Ctrl Pts',(84.6547938588891,-0.0196064101613658,
82.2056635572961));
#135593=CARTESIAN_POINT('Ctrl Pts',(84.4304376221692,0.967037811556315,
82.068788726581));
#135594=CARTESIAN_POINT('Ctrl Pts',(84.4417750514292,0.890447491682914,
82.073688402416));
#135595=CARTESIAN_POINT('Ctrl Pts',(84.4761583942091,0.626392695906014,
82.0885737356621));
#135596=CARTESIAN_POINT('Ctrl Pts',(84.4989506696391,0.296922598800314,
82.0984857915431));
#135597=CARTESIAN_POINT('Ctrl Pts',(84.5018613118091,0.0443872372795342,
82.099749605468));
#135598=CARTESIAN_POINT('Ctrl Pts',(84.5016772295791,-0.0190450268719158,
82.0996693174671));
#135599=CARTESIAN_POINT('Ctrl Pts',(84.4060067611391,0.952294539800014,
81.884762831103));
#135600=CARTESIAN_POINT('Ctrl Pts',(84.417015946189,0.876829574608914,81.889615878929));
#135601=CARTESIAN_POINT('Ctrl Pts',(84.450396710689,0.616706117970314,81.904357430372));
#135602=CARTESIAN_POINT('Ctrl Pts',(84.4725109764891,0.292312756701114,
81.914170427584));
#135603=CARTESIAN_POINT('Ctrl Pts',(84.4753351589791,0.0436982183603942,
81.915422058245));
#135604=CARTESIAN_POINT('Ctrl Pts',(84.4751565378891,-0.0187494150606258,
81.91534263643));
#135605=CARTESIAN_POINT('',(84.7549733371667,0.998148603023009,82.1380581359606));
#135606=CARTESIAN_POINT('Origin',(84.7030401686601,0.973190333485317,81.8436101836762));
#135607=CARTESIAN_POINT('',(84.8242224574765,-4.37596713747203E-12,82.1680724930567));
#135608=CARTESIAN_POINT('Origin',(84.7721268038191,1.61954280611347E-8,
81.872630608394));
#135609=CARTESIAN_POINT('Origin',(78.7905139183666,0.196679718677362,79.5581506211462));
#135610=CARTESIAN_POINT('Origin',(60.0158221861891,1.4210854715202E-14,
74.357344709869));
#135611=CARTESIAN_POINT('',(84.7549627479325,-0.99814350218451,82.1379981311978));
#135612=CARTESIAN_POINT('Origin',(68.4696192519035,0.303986406784001,75.1006252905782));
#135613=CARTESIAN_POINT('',(94.9937559642379,-0.99814863954275,80.3326845061067));
#135614=CARTESIAN_POINT('',(62.0923792317741,-0.998148599370046,86.1340849298962));
#135615=CARTESIAN_POINT('',(95.0009770511691,1.4210854715202E-14,80.37363732553));
#135616=CARTESIAN_POINT('Origin',(92.9168980472373,7.21782711207708E-5,
68.5542381272426));
#135617=CARTESIAN_POINT('',(94.9937559642119,0.998148641326583,80.3326845059602));
#135618=CARTESIAN_POINT('Origin',(92.9168981020881,-7.21782753166342E-5,
68.554238117227));
#135619=CARTESIAN_POINT('',(62.0923792317078,0.998148602984376,86.1340849296003));
#135620=CARTESIAN_POINT('Origin',(60.0158221861891,1.4210854715202E-14,
74.357344709869));
#135621=CARTESIAN_POINT('',(69.9536255526515,4.5030342410532E-9,84.7901609152031));
#135622=CARTESIAN_POINT('',(70.0084327588244,0.998148594771459,84.7382711127335));
#135623=CARTESIAN_POINT('Origin',(82.9054078707814,-0.300965714281284,72.554181695039));
#135624=CARTESIAN_POINT('',(45.1145255780036,0.998148899244916,89.1277385792758));
#135625=CARTESIAN_POINT('',(62.092379227415,0.998148899153649,86.1340849052551));
#135626=CARTESIAN_POINT('',(45.1145147830591,-0.998148588064286,89.12774050813));
#135627=CARTESIAN_POINT('Origin',(33.434640608385,-0.00348829429348399,
82.0882160785412));
#135628=CARTESIAN_POINT('',(70.0084221937706,-0.998143435151018,84.7382111936731));
#135629=CARTESIAN_POINT('',(62.0923792319381,-0.998148588051504,86.1340849308266));
#135630=CARTESIAN_POINT('Origin',(82.9047265017384,0.317497967067761,72.554660600933));
#135631=CARTESIAN_POINT('Origin',(58.9775436614391,-0.499074165591686,68.468974588834));
#135632=CARTESIAN_POINT('',(91.9214587222691,17.49925882517,62.90882101338));
#135633=CARTESIAN_POINT('Ctrl Pts',(94.9937559636691,0.998148678733514,
80.332684502887));
#135634=CARTESIAN_POINT('Ctrl Pts',(94.9618224451266,3.20135410881214,80.1515805199092));
#135635=CARTESIAN_POINT('Ctrl Pts',(94.8586253251175,5.36962766443818,79.5663205693643));
#135636=CARTESIAN_POINT('Ctrl Pts',(94.5234359225885,9.34778727496904,77.665367004673));
#135637=CARTESIAN_POINT('Ctrl Pts',(94.2915459635635,11.156458914409,76.3502536959021));
#135638=CARTESIAN_POINT('Ctrl Pts',(93.7300322273922,14.1723129419968,73.1657510524878));
#135639=CARTESIAN_POINT('Ctrl Pts',(93.4005798639225,15.3785746783534,71.297333853112));
#135640=CARTESIAN_POINT('Ctrl Pts',(92.6881230943526,17.0272550257457,67.2567907285858));
#135641=CARTESIAN_POINT('Ctrl Pts',(92.3053361804104,17.4691703430208,65.0858982627576));
#135642=CARTESIAN_POINT('Ctrl Pts',(91.9214587222691,17.49925882517,62.90882101338));
#135643=CARTESIAN_POINT('',(27.1339043807878,17.4992593331729,74.3325770047843));
#135644=CARTESIAN_POINT('',(91.9214587222691,17.49925882517,62.90882101338));
#135645=CARTESIAN_POINT('Ctrl Pts',(45.1145255783225,0.998148899398187,
89.1277385810842));
#135646=CARTESIAN_POINT('Ctrl Pts',(44.9976684612899,2.21249084100214,89.0454209483036));
#135647=CARTESIAN_POINT('Ctrl Pts',(44.7078984407656,3.38431261135296,88.8727869361181));
#135648=CARTESIAN_POINT('Ctrl Pts',(44.2680522680653,4.5092437997717,88.6185778110664));
#135649=CARTESIAN_POINT('Ctrl Pts',(43.828206164389,5.63417481165772,88.364368725907));
#135650=CARTESIAN_POINT('Ctrl Pts',(43.2382839566064,6.71221526059232,88.0285845542609));
#135651=CARTESIAN_POINT('Ctrl Pts',(42.5452098960251,7.71206894624626,87.6315673683517));
#135652=CARTESIAN_POINT('Ctrl Pts',(41.8521358354439,8.7119226319002,87.2345501824426));
#135653=CARTESIAN_POINT('Ctrl Pts',(41.0559099194567,9.63358955770964,86.776299979814));
#135654=CARTESIAN_POINT('Ctrl Pts',(40.183589985931,10.4852190692797,86.2627573696543));
#135655=CARTESIAN_POINT('Ctrl Pts',(39.3112700524052,11.3368485808498,85.7492147594946));
#135656=CARTESIAN_POINT('Ctrl Pts',(38.3628561006925,12.1184406783657,85.1803797401492));
#135657=CARTESIAN_POINT('Ctrl Pts',(37.3872637706894,12.8188260449958,84.57196131843));
#135658=CARTESIAN_POINT('Ctrl Pts',(36.4116714406863,13.519211411626,83.9635428967109));
#135659=CARTESIAN_POINT('Ctrl Pts',(35.4089007309014,14.1383900461859,83.3155410718192));
#135660=CARTESIAN_POINT('Ctrl Pts',(34.3926908331965,14.6910771465553,82.6100092150662));
#135661=CARTESIAN_POINT('Ctrl Pts',(33.3764809354915,15.2437642469246,81.9044773583132));
#135662=CARTESIAN_POINT('Ctrl Pts',(32.3468318509836,15.7299598132973,81.1414154690442));
#135663=CARTESIAN_POINT('Ctrl Pts',(31.3767033281954,16.1355562382722,80.3185366650299));
#135664=CARTESIAN_POINT('Ctrl Pts',(30.8916390668014,16.3383544507596,79.9070972630227));
#135665=CARTESIAN_POINT('Ctrl Pts',(30.4214549456321,16.5210028773661,79.4807036324811));
#135666=CARTESIAN_POINT('Ctrl Pts',(29.9750215051742,16.6834373562275,79.030614851117));
#135667=CARTESIAN_POINT('Ctrl Pts',(29.5285880647162,16.8458718350889,78.5805260697528));
#135668=CARTESIAN_POINT('Ctrl Pts',(29.1059053050508,16.9880923662971,78.1067421374872));
#135669=CARTESIAN_POINT('Ctrl Pts',(28.7262323167119,17.1065284396786,77.6082728149804));
#135670=CARTESIAN_POINT('Ctrl Pts',(28.3465593283731,17.2249645130601,77.1098034924735));
#135671=CARTESIAN_POINT('Ctrl Pts',(28.009896111389,17.3196161285739,76.5866487795488));
#135672=CARTESIAN_POINT('Ctrl Pts',(27.7386129171228,17.3861177803941,76.0413307805799));
#135673=CARTESIAN_POINT('Ctrl Pts',(27.4673297244896,17.452619431814,75.4960127848936));
#135674=CARTESIAN_POINT('Ctrl Pts',(27.2614265536846,17.4909711198445,74.9285315036144));
#135675=CARTESIAN_POINT('Ctrl Pts',(27.1339043807867,17.4992593326678,74.3325770047782));
#135676=CARTESIAN_POINT('Ctrl Pts',(70.0084327588244,0.99814859477146,84.7382711127335));
#135677=CARTESIAN_POINT('Ctrl Pts',(70.0408249552918,1.28828368766016,84.7079688264717));
#135678=CARTESIAN_POINT('Ctrl Pts',(70.0873703993869,1.5739891510914,84.6683487276227));
#135679=CARTESIAN_POINT('Ctrl Pts',(70.1481706976984,1.85499710789222,84.6199870557848));
#135680=CARTESIAN_POINT('Ctrl Pts',(70.1839312559019,2.02027592516656,84.5915424522448));
#135681=CARTESIAN_POINT('Ctrl Pts',(70.2246230843227,2.183930710078,84.5600737409244));
#135682=CARTESIAN_POINT('Ctrl Pts',(70.2702666820332,2.34591528311728,84.5256971778405));
#135683=CARTESIAN_POINT('Ctrl Pts',(70.3318902336131,2.56461111763809,84.4792852818769));
#135684=CARTESIAN_POINT('Ctrl Pts',(70.4025397942232,2.78026172095382,84.4275732130301));
#135685=CARTESIAN_POINT('Ctrl Pts',(70.4822652821103,2.99277020937439,84.3708440717458));
#135686=CARTESIAN_POINT('Ctrl Pts',(70.5221280260539,3.09902445358468,84.3424795011036));
#135687=CARTESIAN_POINT('Ctrl Pts',(70.5642597412934,3.20449346788007,84.3128606026717));
#135688=CARTESIAN_POINT('Ctrl Pts',(70.6086665968864,3.30916689917204,84.2820223629132));
#135689=CARTESIAN_POINT('Ctrl Pts',(70.6308700246829,3.36150361481803,84.2666032430339));
#135690=CARTESIAN_POINT('Ctrl Pts',(70.6536422374628,3.41364143458008,84.2508792872282));
#135691=CARTESIAN_POINT('Ctrl Pts',(70.6769840006127,3.46557919132123,84.2348548362182));
#135692=CARTESIAN_POINT('Ctrl Pts',(70.6886548821876,3.4915480696918,84.2268426107132));
#135693=CARTESIAN_POINT('Ctrl Pts',(70.7004681513421,3.5174669322909,84.2187552613336));
#135694=CARTESIAN_POINT('Ctrl Pts',(70.7124239035289,3.54333563686625,84.2105933294197));
#135695=CARTESIAN_POINT('Ctrl Pts',(70.7243796557158,3.5692043414416,84.2024313975057));
#135696=CARTESIAN_POINT('Ctrl Pts',(70.7359459374217,3.59390306696996,84.1945560381431));
#135697=CARTESIAN_POINT('Ctrl Pts',(70.7487187045076,3.62079113635154,84.1858843266664));
#135698=CARTESIAN_POINT('Ctrl Pts',(70.8461589156814,3.82591342042526,84.1197300319982));
#135699=CARTESIAN_POINT('Ctrl Pts',(70.9508954747235,4.02431467555368,84.0500370558852));
#135700=CARTESIAN_POINT('Ctrl Pts',(71.0630373621699,4.21603094905015,83.97742345766));
#135701=CARTESIAN_POINT('Ctrl Pts',(71.1764589010252,4.40993489750997,83.9039812654509));
#135702=CARTESIAN_POINT('Ctrl Pts',(71.2974557581051,4.5970008058511,83.8275515361351));
#135703=CARTESIAN_POINT('Ctrl Pts',(71.426133100678,4.77729687882636,83.7487307029305));
#135704=CARTESIAN_POINT('Ctrl Pts',(71.5567245337391,4.96027487692887,83.6687374006331));
#135705=CARTESIAN_POINT('Ctrl Pts',(71.695226669071,5.1362805086737,83.5862814490635));
#135706=CARTESIAN_POINT('Ctrl Pts',(71.8417413389003,5.3054110421532,83.5019403674784));
#135707=CARTESIAN_POINT('Ctrl Pts',(71.8571753661282,5.32322745099356,83.4930557789855));
#135708=CARTESIAN_POINT('Ctrl Pts',(71.8726982990893,5.34096758888549,83.4841502293356));
#135709=CARTESIAN_POINT('Ctrl Pts',(71.8883102515518,5.35863158337501,83.4752243637404));
#135710=CARTESIAN_POINT('Ctrl Pts',(71.964015424898,5.44428747862736,83.4319412315525));
#135711=CARTESIAN_POINT('Ctrl Pts',(72.0418138959197,5.52815279928536,83.3881806293742));
#135712=CARTESIAN_POINT('Ctrl Pts',(72.1217183024344,5.61024285765931,83.3440142298299));
#135713=CARTESIAN_POINT('Ctrl Pts',(72.1616705056917,5.65128788684629,83.3219310300577));
#135714=CARTESIAN_POINT('Ctrl Pts',(72.2021491862545,5.69188908667612,83.2997463436959));
#135715=CARTESIAN_POINT('Ctrl Pts',(72.2431558690364,5.73204852559375,83.2774688189602));
#135716=CARTESIAN_POINT('Ctrl Pts',(72.2776528574498,5.76583276769884,83.2587277879732));
#135717=CARTESIAN_POINT('Ctrl Pts',(72.3134065669243,5.80012927619304,83.2394514719083));
#135718=CARTESIAN_POINT('Ctrl Pts',(72.3481892195389,5.83285725628534,83.2208296824366));
#135719=CARTESIAN_POINT('Ctrl Pts',(72.354752819675,5.83903313300668,83.2173156899512));
#135720=CARTESIAN_POINT('Ctrl Pts',(72.3612818659429,5.84515320903061,83.2138251429461));
#135721=CARTESIAN_POINT('Ctrl Pts',(72.3677614219254,5.85120357486777,83.2103662245637));
#135722=CARTESIAN_POINT('Ctrl Pts',(72.5080057922845,5.98215849671336,83.1355009356496));
#135723=CARTESIAN_POINT('Ctrl Pts',(72.651975851741,6.10597780332322,83.0609436593224));
#135724=CARTESIAN_POINT('Ctrl Pts',(72.7997490509113,6.22280030375475,82.9871336398563));
#135725=CARTESIAN_POINT('Ctrl Pts',(72.9481295964232,6.34010294347164,82.9130202619629));
#135726=CARTESIAN_POINT('Ctrl Pts',(73.1003445984089,6.450351485015,82.8396602437358));
#135727=CARTESIAN_POINT('Ctrl Pts',(73.2564633129398,6.55368553317688,82.7674463558738));
#135728=CARTESIAN_POINT('Ctrl Pts',(73.4132970739346,6.65749286633834,82.6949017178815));
#135729=CARTESIAN_POINT('Ctrl Pts',(73.5740703789479,6.75432253000789,82.6235136789544));
#135730=CARTESIAN_POINT('Ctrl Pts',(73.7388443628456,6.8443102417177,82.5536289521462));
#135731=CARTESIAN_POINT('Ctrl Pts',(73.8171991831552,6.8871020151172,82.5203967325815));
#135732=CARTESIAN_POINT('Ctrl Pts',(73.8964585374665,6.92834651867607,82.4875037102065));
#135733=CARTESIAN_POINT('Ctrl Pts',(73.9766282944521,6.96805759472821,82.4549831679167));
#135734=CARTESIAN_POINT('Ctrl Pts',(74.0739145429824,7.01624710857323,82.4155193890741));
#135735=CARTESIAN_POINT('Ctrl Pts',(74.1725414662957,7.06217856006159,82.3766042630444));
#135736=CARTESIAN_POINT('Ctrl Pts',(74.2725186684865,7.10587547603901,82.3382922573529));
#135737=CARTESIAN_POINT('Ctrl Pts',(74.3225072695819,7.12772393402772,82.3191362545071));
#135738=CARTESIAN_POINT('Ctrl Pts',(74.3728334265893,7.14901372090103,82.3001309534408));
#135739=CARTESIAN_POINT('Ctrl Pts',(74.4234982485887,7.16974765838724,82.2812826440585));
#135740=CARTESIAN_POINT('Ctrl Pts',(74.4741630705881,7.19048159587344,82.2624343346763));
#135741=CARTESIAN_POINT('Ctrl Pts',(74.5265056732342,7.21117152426198,82.2432597716744));
#135742=CARTESIAN_POINT('Ctrl Pts',(74.5765097637604,7.23028458917864,82.2252146696162));
#135743=CARTESIAN_POINT('Ctrl Pts',(74.7417299164944,7.29343669276685,82.1655912570758));
#135744=CARTESIAN_POINT('Ctrl Pts',(74.907909297554,7.34990495573201,82.1085724539664));
#135745=CARTESIAN_POINT('Ctrl Pts',(75.0750870566551,7.39978443221359,82.0543596574019));
#135746=CARTESIAN_POINT('Ctrl Pts',(75.2423672067323,7.44969445826296,82.0001136572511));
#135747=CARTESIAN_POINT('Ctrl Pts',(75.41064694741,7.49300777252423,81.9486770408288));
#135748=CARTESIAN_POINT('Ctrl Pts',(75.5799570925337,7.52980013287031,81.900203892247));
#135749=CARTESIAN_POINT('Ctrl Pts',(75.7492864642117,7.56659667129038,81.851725239142));
#135750=CARTESIAN_POINT('Ctrl Pts',(75.9196464655635,7.59687088235073,81.8062106770198));
#135751=CARTESIAN_POINT('Ctrl Pts',(76.0910596620054,7.62067716530175,81.7637675037834));
#135752=CARTESIAN_POINT('Ctrl Pts',(76.2624810430379,7.64448458494867,81.7213223039819));
#135753=CARTESIAN_POINT('Ctrl Pts',(76.4349557138269,7.66182352815182,81.6819487528516));
#135754=CARTESIAN_POINT('Ctrl Pts',(76.608498094561,7.67272569012792,81.6457079514525));
#135755=CARTESIAN_POINT('Ctrl Pts',(76.7542143825673,7.68187978014144,81.6152780643441));
#135756=CARTESIAN_POINT('Ctrl Pts',(76.900683292054,7.68649538445319,81.5870560432818));
#135757=CARTESIAN_POINT('Ctrl Pts',(77.0479089573794,7.68657849705202,81.5610530932745));
#135758=CARTESIAN_POINT('Ctrl Pts',(77.223218355197,7.68667746362568,81.5300900034003));
#135759=CARTESIAN_POINT('Ctrl Pts',(77.3986015539164,7.68034817596246,81.5024518303399));
#135760=CARTESIAN_POINT('Ctrl Pts',(77.5740545830778,7.66757898161181,81.4781160564969));
#135761=CARTESIAN_POINT('Ctrl Pts',(77.7495048183896,7.65480999059312,81.4537806701678));
#135762=CARTESIAN_POINT('Ctrl Pts',(77.9250248851518,7.6356012608945,81.432747596216));
#135763=CARTESIAN_POINT('Ctrl Pts',(78.1006027241673,7.60991774884212,81.4149484435362));
#135764=CARTESIAN_POINT('Ctrl Pts',(78.2761579227927,7.58423754862415,81.3971515860195));
#135765=CARTESIAN_POINT('Ctrl Pts',(78.451770885019,7.5520841606714,81.3825878512363));
#135766=CARTESIAN_POINT('Ctrl Pts',(78.6274213983951,7.51340001043409,81.3711426086793));
#135767=CARTESIAN_POINT('Ctrl Pts',(78.7380622968593,7.48903316369782,81.3639333390033));
#135768=CARTESIAN_POINT('Ctrl Pts',(78.848717931472,7.46207469518769,81.3579604522603));
#135769=CARTESIAN_POINT('Ctrl Pts',(78.9593815684807,7.43250587062521,81.3531857594439));
#135770=CARTESIAN_POINT('Ctrl Pts',(79.0656768329959,7.4041042554856,81.3485995444087));
#135771=CARTESIAN_POINT('Ctrl Pts',(79.1719794737027,7.37329427042475,81.3451187554495));
#135772=CARTESIAN_POINT('Ctrl Pts',(79.2782823783977,7.34005658147724,81.3427030572568));
#135773=CARTESIAN_POINT('Ctrl Pts',(79.3314338307452,7.32343773700349,81.3414952081604));
#135774=CARTESIAN_POINT('Ctrl Pts',(79.3845853320286,7.30621191919041,81.3405535349978));
#135775=CARTESIAN_POINT('Ctrl Pts',(79.4377358860987,7.28837648441645,81.3398723883246));
#135776=CARTESIAN_POINT('Ctrl Pts',(79.4908864401688,7.2705410496425,81.3391912416514));
#135777=CARTESIAN_POINT('Ctrl Pts',(79.5425882552996,7.25261513739578,81.3387751495482));
#135778=CARTESIAN_POINT('Ctrl Pts',(79.5971836411002,7.233038511023,81.3386044846345));
#135779=CARTESIAN_POINT('Ctrl Pts',(79.7857856516985,7.16541024829538,81.3380149156554));
#135780=CARTESIAN_POINT('Ctrl Pts',(79.9713248235223,7.09110427453467,81.3406701687274));
#135781=CARTESIAN_POINT('Ctrl Pts',(80.1537542859587,7.01000292279281,81.3463044273957));
#135782=CARTESIAN_POINT('Ctrl Pts',(80.3358408968339,6.9290539900993,81.351928097235));
#135783=CARTESIAN_POINT('Ctrl Pts',(80.5148294890063,6.84133495666976,81.3605196602627));
#135784=CARTESIAN_POINT('Ctrl Pts',(80.6906647240559,6.74671618626887,81.3717652767044));
#135785=CARTESIAN_POINT('Ctrl Pts',(80.8657827511281,6.6524833529467,81.3829650238081));
#135786=CARTESIAN_POINT('Ctrl Pts',(81.037773103144,6.55140667405553,81.3967972758552));
#135787=CARTESIAN_POINT('Ctrl Pts',(81.2065722766861,6.4433494501232,81.4129018870683));
#135788=CARTESIAN_POINT('Ctrl Pts',(81.288338740854,6.3910064383457,81.4207029745267));
#135789=CARTESIAN_POINT('Ctrl Pts',(81.3693562799857,6.33702537853851,81.4290365004588));
#135790=CARTESIAN_POINT('Ctrl Pts',(81.4496169145499,6.28139031486415,81.4378572106945));
#135791=CARTESIAN_POINT('Ctrl Pts',(81.5461173604788,6.21449813935357,81.4484626896542));
#135792=CARTESIAN_POINT('Ctrl Pts',(81.6415236397101,6.14521489446578,81.4597726094186));
#135793=CARTESIAN_POINT('Ctrl Pts',(81.7358209135696,6.07351267745926,81.471702815685));
#135794=CARTESIAN_POINT('Ctrl Pts',(81.7829695504994,6.037661568956,81.4776679188183));
#135795=CARTESIAN_POINT('Ctrl Pts',(81.8298409215836,6.00120568493967,81.4837880113286));
#135796=CARTESIAN_POINT('Ctrl Pts',(81.8764330685024,5.96414159187196,81.4900519870319));
#135797=CARTESIAN_POINT('Ctrl Pts',(81.9177073832813,5.93130783885908,81.4956010188334));
#135798=CARTESIAN_POINT('Ctrl Pts',(81.9578519764763,5.89875352494833,81.501132511256));
#135799=CARTESIAN_POINT('Ctrl Pts',(81.9992854773298,5.86446517396627,81.5069853745834));
#135800=CARTESIAN_POINT('Ctrl Pts',(82.0046238191941,5.86004742176729,81.5077394645029));
#135801=CARTESIAN_POINT('Ctrl Pts',(82.0099835454754,5.8556008594935,81.5084988238638));
#135802=CARTESIAN_POINT('Ctrl Pts',(82.0153698185917,5.85112115822791,81.509264118107));
#135803=CARTESIAN_POINT('Ctrl Pts',(82.2015453597434,5.69628110661652,81.535716373087));
#135804=CARTESIAN_POINT('Ctrl Pts',(82.3795555066486,5.53455025116332,81.5637737486441));
#135805=CARTESIAN_POINT('Ctrl Pts',(82.5493047637065,5.36580530934802,81.5928946623141));
#135806=CARTESIAN_POINT('Ctrl Pts',(82.7225984719925,5.19353688692007,81.6226236355422));
#135807=CARTESIAN_POINT('Ctrl Pts',(82.8872827416686,5.01395787070318,81.6534612300521));
#135808=CARTESIAN_POINT('Ctrl Pts',(83.0432468258943,4.82695827935064,81.684779369301));
#135809=CARTESIAN_POINT('Ctrl Pts',(83.1992109101201,4.6399586879981,81.7160975085499));
#135810=CARTESIAN_POINT('Ctrl Pts',(83.3464548080814,4.44553800507966,81.7478961879203));
#135811=CARTESIAN_POINT('Ctrl Pts',(83.484858501528,4.24361505436675,81.7794947500919));
#135812=CARTESIAN_POINT('Ctrl Pts',(83.5535885431426,4.14334191526296,81.795186314666));
#135813=CARTESIAN_POINT('Ctrl Pts',(83.6201384227432,4.04121919074353,81.8108277155241));
#135814=CARTESIAN_POINT('Ctrl Pts',(83.6844925963318,3.93724022648501,81.8263307982717));
#135815=CARTESIAN_POINT('Ctrl Pts',(83.7166696831261,3.88525074435576,81.8340823396455));
#135816=CARTESIAN_POINT('Ctrl Pts',(83.7482978367049,3.83279719257951,81.841799263423));
#135817=CARTESIAN_POINT('Ctrl Pts',(83.7793750594448,3.77987902508754,81.8494702405201));
#135818=CARTESIAN_POINT('Ctrl Pts',(83.7949136708148,3.75341994134156,81.8533057290687));
#135819=CARTESIAN_POINT('Ctrl Pts',(83.810314549073,3.72684470306123,81.857129728667));
#135820=CARTESIAN_POINT('Ctrl Pts',(83.8255774415903,3.70015325027683,81.8609408065833));
#135821=CARTESIAN_POINT('Ctrl Pts',(83.8399802554224,3.67496588654937,81.8645371265904));
#135822=CARTESIAN_POINT('Ctrl Pts',(83.8548412394187,3.64863145971816,81.8682691271197));
#135823=CARTESIAN_POINT('Ctrl Pts',(83.8685152708665,3.62410422449756,81.8717188749887));
#135824=CARTESIAN_POINT('Ctrl Pts',(83.8693318295698,3.62263955568618,81.8719248801934));
#135825=CARTESIAN_POINT('Ctrl Pts',(83.8701441581997,3.62118133485766,81.8721298936447));
#135826=CARTESIAN_POINT('Ctrl Pts',(83.8709519074023,3.61973019242326,81.872333831851));
#135827=CARTESIAN_POINT('Ctrl Pts',(84.0183892479838,3.35485517844943,81.9095583895194));
#135828=CARTESIAN_POINT('Ctrl Pts',(84.1489902741974,3.08463837448672,81.9445913018005));
#135829=CARTESIAN_POINT('Ctrl Pts',(84.2626499120171,2.80925089465851,81.9768366642815));
#135830=CARTESIAN_POINT('Ctrl Pts',(84.3751137249479,2.53676079519157,82.0087427699451));
#135831=CARTESIAN_POINT('Ctrl Pts',(84.4709907163675,2.25920809161474,82.0379194350411));
#135832=CARTESIAN_POINT('Ctrl Pts',(84.5501771425858,1.9768081545852,82.063778299866));
#135833=CARTESIAN_POINT('Ctrl Pts',(84.6282424776673,1.69840632785724,82.0892710647727));
#135834=CARTESIAN_POINT('Ctrl Pts',(84.6900864546966,1.41529344313058,82.1115390551691));
#135835=CARTESIAN_POINT('Ctrl Pts',(84.7356084100877,1.1277261993533,82.13001137949));
#135836=CARTESIAN_POINT('Ctrl Pts',(84.7424300286744,1.08463327774595,82.1327795196071));
#135837=CARTESIAN_POINT('Ctrl Pts',(84.7488851177831,1.04144042388919,82.1354624149764));
#135838=CARTESIAN_POINT('Ctrl Pts',(84.7549733371667,0.99814860302301,82.1380581359606));
#135839=CARTESIAN_POINT('Ctrl Pts',(69.6467142128891,0.785419361948713,
84.5431073525001));
#135840=CARTESIAN_POINT('Ctrl Pts',(69.6932298573291,1.31770282807001,84.49792214893));
#135841=CARTESIAN_POINT('Ctrl Pts',(69.9015994638491,2.45488886695201,84.33269026631));
#135842=CARTESIAN_POINT('Ctrl Pts',(70.5657769153691,4.08265548317301,83.88089933277));
#135843=CARTESIAN_POINT('Ctrl Pts',(71.6147694030391,5.55740671721501,83.25266276915));
#135844=CARTESIAN_POINT('Ctrl Pts',(72.9604189620991,6.71218455213701,82.569190226542));
#135845=CARTESIAN_POINT('Ctrl Pts',(74.5029817396891,7.48371999717802,81.9471764438769));
#135846=CARTESIAN_POINT('Ctrl Pts',(76.1535633017791,7.86342804363901,81.4678565067189));
#135847=CARTESIAN_POINT('Ctrl Pts',(77.8566888949492,7.86401665948,81.167249222321));
#135848=CARTESIAN_POINT('Ctrl Pts',(79.5728282472391,7.48520878558501,81.052512962104));
#135849=CARTESIAN_POINT('Ctrl Pts',(81.2376327103791,6.71339956417001,81.1092150367));
#135850=CARTESIAN_POINT('Ctrl Pts',(82.7377717224591,5.55727078208801,81.291474417738));
#135851=CARTESIAN_POINT('Ctrl Pts',(83.9388845251391,4.08125982842501,81.523214938505));
#135852=CARTESIAN_POINT('Ctrl Pts',(84.7169256774691,2.45387688843001,81.7204854573311));
#135853=CARTESIAN_POINT('Ctrl Pts',(84.9689920528791,1.31732416127501,81.80441443773));
#135854=CARTESIAN_POINT('Ctrl Pts',(85.0281079295492,0.785594937471314,
81.830940382969));
#135855=CARTESIAN_POINT('Ctrl Pts',(69.7131001219592,0.800479551205414,
84.78138913421));
#135856=CARTESIAN_POINT('Ctrl Pts',(69.7612232582491,1.33806790374101,84.73541059712));
#135857=CARTESIAN_POINT('Ctrl Pts',(69.9756538400191,2.48539832882801,84.56741528251));
#135858=CARTESIAN_POINT('Ctrl Pts',(70.6537549411791,4.11873126524301,84.10990240609));
#135859=CARTESIAN_POINT('Ctrl Pts',(71.7147266250591,5.58568200595701,83.47782034655));
#135860=CARTESIAN_POINT('Ctrl Pts',(73.0616884062191,6.72241378017701,82.795461872428));
#135861=CARTESIAN_POINT('Ctrl Pts',(74.5902699815791,7.47385793838302,82.179480822702));
#135862=CARTESIAN_POINT('Ctrl Pts',(76.2132276098791,7.84057298012902,81.708053004936));
#135863=CARTESIAN_POINT('Ctrl Pts',(77.8828743052091,7.84113956683401,81.413354483289));
#135864=CARTESIAN_POINT('Ctrl Pts',(79.5703075102091,7.47530120987402,81.300662572887));
#135865=CARTESIAN_POINT('Ctrl Pts',(81.2198565698392,6.72360904533501,81.356479029792));
#135866=CARTESIAN_POINT('Ctrl Pts',(82.7208490445491,5.58555316282103,81.537239976425));
#135867=CARTESIAN_POINT('Ctrl Pts',(83.9345496642491,4.11733640075101,81.76849788775));
#135868=CARTESIAN_POINT('Ctrl Pts',(84.7276253707291,2.48437788623201,81.966383439229));
#135869=CARTESIAN_POINT('Ctrl Pts',(84.9863259944791,1.33768534536301,82.050835901607));
#135870=CARTESIAN_POINT('Ctrl Pts',(85.0472221659491,0.800656874293014,
82.0775572867141));
#135871=CARTESIAN_POINT('Ctrl Pts',(69.9501060829392,0.786177546583314,
84.852354313));
#135872=CARTESIAN_POINT('Ctrl Pts',(69.9975371008791,1.31184806627701,84.80626783169));
#135873=CARTESIAN_POINT('Ctrl Pts',(70.2085206123191,2.43317701879001,84.63811593324));
#135874=CARTESIAN_POINT('Ctrl Pts',(70.873528140399,4.02522621269901,84.18143831868));
#135875=CARTESIAN_POINT('Ctrl Pts',(71.9096656973891,5.44894304416801,83.55295341525));
#135876=CARTESIAN_POINT('Ctrl Pts',(73.2189510831691,6.54640141231401,82.8778451648939));
#135877=CARTESIAN_POINT('Ctrl Pts',(74.6980547553291,7.26795848633102,82.272197496043));
#135878=CARTESIAN_POINT('Ctrl Pts',(76.2631781069791,7.61855497908201,81.812330154294));
#135879=CARTESIAN_POINT('Ctrl Pts',(77.8717848917391,7.61909572214601,81.528397109963));
#135880=CARTESIAN_POINT('Ctrl Pts',(79.5008623467592,7.26934102286101,81.4246339445011));
#135881=CARTESIAN_POINT('Ctrl Pts',(81.1002916501491,6.54755501071102,81.487675127427));
#135882=CARTESIAN_POINT('Ctrl Pts',(82.5633528474692,5.44882107944701,81.67451639658));
#135883=CARTESIAN_POINT('Ctrl Pts',(83.7524812891091,4.02386927061101,81.910890495113));
#135884=CARTESIAN_POINT('Ctrl Pts',(84.5329796997091,2.43217997060401,82.112466891796));
#135885=CARTESIAN_POINT('Ctrl Pts',(84.7884979941891,1.31147393282401,82.198244230732));
#135886=CARTESIAN_POINT('Ctrl Pts',(84.8487811433091,0.786350937502314,
82.225303450051));
#135887=CARTESIAN_POINT('Ctrl Pts',(70.1340181617991,0.756013252073015,
84.68901765668));
#135888=CARTESIAN_POINT('Ctrl Pts',(70.1791107533991,1.26379266360201,84.64361051084));
#135889=CARTESIAN_POINT('Ctrl Pts',(70.3803928968891,2.34751751437501,84.4780566788099));
#135890=CARTESIAN_POINT('Ctrl Pts',(71.0176488742091,3.89040132568301,84.0279831130701));
#135891=CARTESIAN_POINT('Ctrl Pts',(72.0155803335091,5.27626004995501,83.40714260132));
#135892=CARTESIAN_POINT('Ctrl Pts',(73.283764093069,6.35028849871101,82.7385771211889));
#135893=CARTESIAN_POINT('Ctrl Pts',(74.7245961904991,7.06037361530101,82.1378096282151));
#135894=CARTESIAN_POINT('Ctrl Pts',(76.2562656742691,7.40694058571701,81.6822589903259));
#135895=CARTESIAN_POINT('Ctrl Pts',(77.833888139419,7.40747606488501,81.4037864218081));
#135896=CARTESIAN_POINT('Ctrl Pts',(79.4300432208991,7.06173752758101,81.3074084030879));
#135897=CARTESIAN_POINT('Ctrl Pts',(80.9917973006791,6.35141784042201,81.3789651146941));
#135898=CARTESIAN_POINT('Ctrl Pts',(82.413946454709,5.27613825742201,81.5737261440561));
#135899=CARTESIAN_POINT('Ctrl Pts',(83.5645368175391,3.88908364255101,81.815985970834));
#135900=CARTESIAN_POINT('Ctrl Pts',(84.3167180044791,2.34655363670601,82.020845174075));
#135901=CARTESIAN_POINT('Ctrl Pts',(84.5622412464891,1.26343131915301,82.107498210764));
#135902=CARTESIAN_POINT('Ctrl Pts',(84.6200966982691,0.756180742730514,
82.134718771215));
#135903=CARTESIAN_POINT('Ctrl Pts',(70.3179302406591,0.725848957562814,
84.52568100036));
#135904=CARTESIAN_POINT('Ctrl Pts',(70.3606844059291,1.21573726092701,84.4809531899901));
#135905=CARTESIAN_POINT('Ctrl Pts',(70.5522651814691,2.26185800996101,84.31799742439));
#135906=CARTESIAN_POINT('Ctrl Pts',(71.1617696080291,3.75557643866701,83.87452790746));
#135907=CARTESIAN_POINT('Ctrl Pts',(72.1214949696291,5.10357705574302,83.26133178739));
#135908=CARTESIAN_POINT('Ctrl Pts',(73.3485771029692,6.15417558510801,82.599309077484));
#135909=CARTESIAN_POINT('Ctrl Pts',(74.7511376256591,6.85278874427201,82.0034217603881));
#135910=CARTESIAN_POINT('Ctrl Pts',(76.2493532415691,7.19532619235201,81.552187826359));
#135911=CARTESIAN_POINT('Ctrl Pts',(77.7959913870991,7.19585640762402,81.279175733652));
#135912=CARTESIAN_POINT('Ctrl Pts',(79.3592240950391,6.85413403230101,81.1901828616749));
#135913=CARTESIAN_POINT('Ctrl Pts',(80.8833029512191,6.15528067013201,81.27025510196));
#135914=CARTESIAN_POINT('Ctrl Pts',(82.2645400619392,5.10345543539701,81.472935891533));
#135915=CARTESIAN_POINT('Ctrl Pts',(83.3765923459791,3.75429801449001,81.721081446555));
#135916=CARTESIAN_POINT('Ctrl Pts',(84.1004563092491,2.26092730280701,81.929223456353));
#135917=CARTESIAN_POINT('Ctrl Pts',(84.3359844987991,1.21538870548301,82.016752190797));
#135918=CARTESIAN_POINT('Ctrl Pts',(84.3914122532191,0.726010547958614,
82.044134092379));
#135919=CARTESIAN_POINT('Ctrl Pts',(70.2751507164491,0.708294960791114,
84.2822187406399));
#135920=CARTESIAN_POINT('Ctrl Pts',(70.3161274275591,1.19120660018001,84.23831630919));
#135921=CARTESIAN_POINT('Ctrl Pts',(70.5009098227891,2.22361576577601,84.07826090145));
#135922=CARTESIAN_POINT('Ctrl Pts',(71.0941998788891,3.70669520774501,83.6409305469399));
#135923=CARTESIAN_POINT('Ctrl Pts',(72.0384105536192,5.057948427186,83.03221038356));
#135924=CARTESIAN_POINT('Ctrl Pts',(73.2597623498791,6.12307642092401,82.369847158899));
#135925=CARTESIAN_POINT('Ctrl Pts',(74.6713828128091,6.83946132401601,81.768780332156));
#135926=CARTESIAN_POINT('Ctrl Pts',(76.192102641159,7.19386181068701,81.310544720065));
#135927=CARTESIAN_POINT('Ctrl Pts',(77.7670586812291,7.19441231048701,81.032533866219));
#135928=CARTESIAN_POINT('Ctrl Pts',(79.3538783771191,6.84084767825001,80.942411577904));
#135929=CARTESIAN_POINT('Ctrl Pts',(80.8882888229391,6.12419755563401,81.024252198021));
#135930=CARTESIAN_POINT('Ctrl Pts',(82.2642506938791,5.05782011026801,81.2292165899171));
#135931=CARTESIAN_POINT('Ctrl Pts',(83.3601757425891,3.70542032188201,81.47846177581));
#135932=CARTESIAN_POINT('Ctrl Pts',(84.0667116606391,2.22269669503301,81.686379856903));
#135933=CARTESIAN_POINT('Ctrl Pts',(84.2948665735391,1.19086312606301,81.773508524379));
#135934=CARTESIAN_POINT('Ctrl Pts',(84.3483435002091,0.708454252188914,
81.80072298139));
#135935=CARTESIAN_POINT('Ctrl Pts',(70.0460599054191,0.719920776125714,
84.18843902109));
#135936=CARTESIAN_POINT('Ctrl Pts',(70.0874979035891,1.21335558682101,84.1447289228899));
#135937=CARTESIAN_POINT('Ctrl Pts',(70.2748020122591,2.26888828273301,83.98513846763));
#135938=CARTESIAN_POINT('Ctrl Pts',(70.8787198966591,3.78989745330101,83.5476875299399));
#135939=CARTESIAN_POINT('Ctrl Pts',(71.8447518705991,5.18244379829901,82.936049957039));
#135940=CARTESIAN_POINT('Ctrl Pts',(73.1011535809691,6.28634603308001,82.266784350285));
#135941=CARTESIAN_POINT('Ctrl Pts',(74.5606136683391,7.03297133186201,81.655367355105));
#135942=CARTESIAN_POINT('Ctrl Pts',(76.1385536828191,7.40392969533601,81.1854206853431));
#135943=CARTESIAN_POINT('Ctrl Pts',(77.774400092089,7.40450688118101,80.8966702485669));
#135944=CARTESIAN_POINT('Ctrl Pts',(79.419051980679,7.03441967967101,80.797970056011));
#135945=CARTESIAN_POINT('Ctrl Pts',(81.0020486672191,6.28750837427602,80.873162703487));
#135946=CARTESIAN_POINT('Ctrl Pts',(82.4133514899292,5.18230823705901,81.0726190089751));
#135947=CARTESIAN_POINT('Ctrl Pts',(83.530782916899,3.78858704523601,81.3171397681949));
#135948=CARTESIAN_POINT('Ctrl Pts',(84.247336203049,2.26794833049001,81.5215385554099));
#135949=CARTESIAN_POINT('Ctrl Pts',(84.477699375629,1.21300469000201,81.6073690211719));
#135950=CARTESIAN_POINT('Ctrl Pts',(84.5315437634291,0.720083539852114,
81.6342453016709));
#135951=CARTESIAN_POINT('Origin',(69.9560096372196,0.973231869956287,84.4436697031834));
#135952=CARTESIAN_POINT('Ctrl Pts',(69.9410902066692,-0.0200749179659658,
84.7920798508299));
#135953=CARTESIAN_POINT('Ctrl Pts',(69.9410243575191,0.00807640976446622,
84.7921397125799));
#135954=CARTESIAN_POINT('Ctrl Pts',(69.9416531080391,0.254907774005214,
84.7915720445599));
#135955=CARTESIAN_POINT('Ctrl Pts',(69.9574697196891,0.602587781192914,
84.7772449914899));
#135956=CARTESIAN_POINT('Ctrl Pts',(69.9895755752191,0.919382073654714,
84.7482586599001));
#135957=CARTESIAN_POINT('Ctrl Pts',(70.0014582496291,1.01916091177701,84.7375477247));
#135958=CARTESIAN_POINT('Ctrl Pts',(70.1256916253091,-0.0196065190321158,
84.7675386824));
#135959=CARTESIAN_POINT('Ctrl Pts',(70.1256274227291,0.00788796798874821,
84.7675982874601));
#135960=CARTESIAN_POINT('Ctrl Pts',(70.1262404858491,0.248960167223414,
84.76703309691));
#135961=CARTESIAN_POINT('Ctrl Pts',(70.1416623917691,0.588526916119514,
84.75276801805));
#135962=CARTESIAN_POINT('Ctrl Pts',(70.1729656463091,0.897915264457314,
84.72390818689));
#135963=CARTESIAN_POINT('Ctrl Pts',(70.1845510765691,0.995359642174814,
84.71324418904));
#135964=CARTESIAN_POINT('Ctrl Pts',(70.2333228313691,-0.0190451304001758,
84.6155670875601));
#135965=CARTESIAN_POINT('Ctrl Pts',(70.2332613314891,0.00766210207465321,
84.61562565729));
#135966=CARTESIAN_POINT('Ctrl Pts',(70.2338484032691,0.241831420262514,
84.61506984276));
#135967=CARTESIAN_POINT('Ctrl Pts',(70.2486158835091,0.571683637382613,
84.60104674069));
#135968=CARTESIAN_POINT('Ctrl Pts',(70.2786051836591,0.872330962898515,
84.57266800438));
#135969=CARTESIAN_POINT('Ctrl Pts',(70.2897064325991,0.967037502858313,
84.56218029236));
#135970=CARTESIAN_POINT('Ctrl Pts',(70.1952002761691,-0.0187495170019758,
84.43328509289));
#135971=CARTESIAN_POINT('Ctrl Pts',(70.1951408079091,0.00754315546745622,
84.4333425102999));
#135972=CARTESIAN_POINT('Ctrl Pts',(70.1957081946091,0.238077279840414,
84.4327969784399));
#135973=CARTESIAN_POINT('Ctrl Pts',(70.2099797510591,0.562821928084014,
84.4190412163801));
#135974=CARTESIAN_POINT('Ctrl Pts',(70.2389834482391,0.858979251046915,
84.39119071749));
#135975=CARTESIAN_POINT('Ctrl Pts',(70.2497230029891,0.952294237575714,
84.3808959813399));
#135976=CARTESIAN_POINT('Origin',(69.9015319855191,-1.31377662151953E-8,
84.4947179233));
#135977=CARTESIAN_POINT('Ctrl Pts',(69.7564804663291,-1.18130795621199,
84.6242643184));
#135978=CARTESIAN_POINT('Ctrl Pts',(69.7401068344391,-1.05954295648899,
84.63874639282));
#135979=CARTESIAN_POINT('Ctrl Pts',(69.7030507545791,-0.732436278044086,
84.67159393454));
#135980=CARTESIAN_POINT('Ctrl Pts',(69.6774028986991,-0.282494314856486,
84.69441260833));
#135981=CARTESIAN_POINT('Ctrl Pts',(69.6768465603291,0.0447208421045242,
84.6949039456));
#135982=CARTESIAN_POINT('Ctrl Pts',(69.6790678296691,0.164690824891014,
84.6929285177001));
#135983=CARTESIAN_POINT('Ctrl Pts',(69.8967461732791,-1.18166250822699,
84.77938870072));
#135984=CARTESIAN_POINT('Ctrl Pts',(69.8801437431891,-1.05993924015199,
84.79407745808));
#135985=CARTESIAN_POINT('Ctrl Pts',(69.8425571861291,-0.732848144525486,
84.8274028272));
#135986=CARTESIAN_POINT('Ctrl Pts',(69.8165254859392,-0.282676461232986,
84.85056404238));
#135987=CARTESIAN_POINT('Ctrl Pts',(69.8159607204191,0.0447499039312942,
84.85106211981));
#135988=CARTESIAN_POINT('Ctrl Pts',(69.8182151861391,0.164792365768414,
84.84905716968));
#135989=CARTESIAN_POINT('Ctrl Pts',(70.1035892209992,-1.15296456351699,
84.76796001164));
#135990=CARTESIAN_POINT('Ctrl Pts',(70.0873962121891,-1.03421196443699,
84.78259973814));
#135991=CARTESIAN_POINT('Ctrl Pts',(70.0507344739592,-0.715085683656586,
84.81581554535));
#135992=CARTESIAN_POINT('Ctrl Pts',(70.0253405075491,-0.275829379908586,
84.8389025823201));
#135993=CARTESIAN_POINT('Ctrl Pts',(70.0247895466191,0.0436659991401842,
84.8393989572201));
#135994=CARTESIAN_POINT('Ctrl Pts',(70.0269887758291,0.160799851340314,
84.8374004511201));
#135995=CARTESIAN_POINT('Ctrl Pts',(70.2208705491191,-1.11687726314599,
84.5986053952399));
#135996=CARTESIAN_POINT('Ctrl Pts',(70.2054161223391,-1.00178180941899,
84.6129773888799));
#135997=CARTESIAN_POINT('Ctrl Pts',(70.1704363834391,-0.692557196949986,
84.64557894957));
#135998=CARTESIAN_POINT('Ctrl Pts',(70.1462203244891,-0.267121708920386,
84.66823108342));
#135999=CARTESIAN_POINT('Ctrl Pts',(70.1456949792692,0.0422873320530842,
84.6687185983001));
#136000=CARTESIAN_POINT('Ctrl Pts',(70.1477922353091,0.155727100336014,
84.66675763812));
#136001=CARTESIAN_POINT('Ctrl Pts',(70.3381518772391,-1.08078996277499,
84.42925077884));
#136002=CARTESIAN_POINT('Ctrl Pts',(70.3234360324891,-0.969351654400286,
84.4433550396201));
#136003=CARTESIAN_POINT('Ctrl Pts',(70.2901382929191,-0.670028710243386,
84.47534235379));
#136004=CARTESIAN_POINT('Ctrl Pts',(70.2671001414291,-0.258414037932286,
84.49755958453));
#136005=CARTESIAN_POINT('Ctrl Pts',(70.2666004119091,0.0409086649659842,
84.49803823939));
#136006=CARTESIAN_POINT('Ctrl Pts',(70.2685956947891,0.150654349331714,
84.49611482512));
#136007=CARTESIAN_POINT('Ctrl Pts',(70.2773396420792,-1.06455443102999,
84.2298105032));
#136008=CARTESIAN_POINT('Ctrl Pts',(70.2631340086391,-0.954699084796287,
84.24363043191));
#136009=CARTESIAN_POINT('Ctrl Pts',(70.2310057625491,-0.659740216438386,
84.27496248958));
#136010=CARTESIAN_POINT('Ctrl Pts',(70.2087965283391,-0.254418913679886,
84.29671238647));
#136011=CARTESIAN_POINT('Ctrl Pts',(70.2083148891791,0.0402759463338542,
84.29718171195));
#136012=CARTESIAN_POINT('Ctrl Pts',(70.2102384384591,0.148330615786914,
84.29529860328));
#136013=CARTESIAN_POINT('Ctrl Pts',(70.0843390135691,-1.08042634050399,
84.15083551784));
#136014=CARTESIAN_POINT('Ctrl Pts',(70.0700300788791,-0.968884846785787,
84.16456914826));
#136015=CARTESIAN_POINT('Ctrl Pts',(70.0376760079891,-0.669458163442587,
84.19569957119));
#136016=CARTESIAN_POINT('Ctrl Pts',(70.0153209782991,-0.258152124963886,
84.21730247854));
#136017=CARTESIAN_POINT('Ctrl Pts',(70.0148362483192,0.0408667947848142,
84.2177690477299));
#136018=CARTESIAN_POINT('Ctrl Pts',(70.0167724529091,0.150510010251614,
84.21589857897));
#136019=CARTESIAN_POINT('Origin',(69.9565232205078,-0.973190806778888,84.4438203202395));
#136020=CARTESIAN_POINT('Ctrl Pts',(84.8366580532091,0.0200750409221942,
82.165589037612));
#136021=CARTESIAN_POINT('Ctrl Pts',(84.836751259439,-0.0117694511617658,
82.165627235365));
#136022=CARTESIAN_POINT('Ctrl Pts',(84.8357393583291,-0.266091686437686,
82.165216682068));
#136023=CARTESIAN_POINT('Ctrl Pts',(84.8151322061391,-0.613726406334186,
82.156819280891));
#136024=CARTESIAN_POINT('Ctrl Pts',(84.775011662459,-0.926769367276586,
82.140549742704));
#136025=CARTESIAN_POINT('Ctrl Pts',(84.7612796644692,-1.01916123813399,
82.134992792959));
#136026=CARTESIAN_POINT('Ctrl Pts',(84.6547958874591,0.0196066388531642,
82.205665345244));
#136027=CARTESIAN_POINT('Ctrl Pts',(84.6548872431291,-0.0114948418582758,
82.2057039075881));
#136028=CARTESIAN_POINT('Ctrl Pts',(84.6538954366891,-0.259883136404086,
82.205289437392));
#136029=CARTESIAN_POINT('Ctrl Pts',(84.6336971379591,-0.599405443717186,
82.1968119957));
#136030=CARTESIAN_POINT('Ctrl Pts',(84.5943748685691,-0.905129725272486,
82.1803866832581));
#136031=CARTESIAN_POINT('Ctrl Pts',(84.5809163839991,-0.995359963007886,
82.174776434602));
#136032=CARTESIAN_POINT('Ctrl Pts',(84.5016782566291,0.0190452493532842,
82.099670842561));
#136033=CARTESIAN_POINT('Ctrl Pts',(84.5017663374991,-0.0111656970980658,
82.099709346569));
#136034=CARTESIAN_POINT('Ctrl Pts',(84.5008101478991,-0.252441591377686,
82.099294800995));
#136035=CARTESIAN_POINT('Ctrl Pts',(84.4813393368691,-0.582252377763186,
82.090821072537));
#136036=CARTESIAN_POINT('Ctrl Pts',(84.4434170859791,-0.879342716401286,
82.074398259715));
#136037=CARTESIAN_POINT('Ctrl Pts',(84.4304357389791,-0.967037815738486,
82.0687880860861));
#136038=CARTESIAN_POINT('Ctrl Pts',(84.4751575973991,0.0187496379689842,
81.915343126508));
#136039=CARTESIAN_POINT('Ctrl Pts',(84.475243072029,-0.0109923624607558,
81.915381186535));
#136040=CARTESIAN_POINT('Ctrl Pts',(84.474315259909,-0.248522697782586,
81.914970455274));
#136041=CARTESIAN_POINT('Ctrl Pts',(84.4554256573791,-0.573229168182786,
81.906581820792));
#136042=CARTESIAN_POINT('Ctrl Pts',(84.418610463479,-0.865887969031586,
81.89031818404));
#136043=CARTESIAN_POINT('Ctrl Pts',(84.4060049552891,-0.952294548179087,
81.884761411431));
#136044=CARTESIAN_POINT('Origin',(84.703419321545,-0.973227037640828,81.8433412100757));
#136045=CARTESIAN_POINT('Ctrl Pts',(85.0281338392691,-0.785442429272785,
81.830954919499));
#136046=CARTESIAN_POINT('Ctrl Pts',(84.9678505702292,-1.32789691945799,
81.803904430336));
#136047=CARTESIAN_POINT('Ctrl Pts',(84.7111038549791,-2.47360497699299,
81.718691486301));
#136048=CARTESIAN_POINT('Ctrl Pts',(83.9232885536391,-4.10503857870399,
81.519756430079));
#136049=CARTESIAN_POINT('Ctrl Pts',(82.7216600039292,-5.57202437394999,
81.2890121320651));
#136050=CARTESIAN_POINT('Ctrl Pts',(81.226056711349,-6.71948616520598,81.108544375771));
#136051=CARTESIAN_POINT('Ctrl Pts',(79.569064807179,-7.48586908240599,81.052830407459));
#136052=CARTESIAN_POINT('Ctrl Pts',(77.8597106364491,-7.86330763548499,
81.1670786168599));
#136053=CARTESIAN_POINT('Ctrl Pts',(76.1616397228791,-7.86398436055798,
81.46614911781));
#136054=CARTESIAN_POINT('Ctrl Pts',(74.5148178179191,-7.48758304592898,
81.9432097462369));
#136055=CARTESIAN_POINT('Ctrl Pts',(72.9741081702291,-6.72095167631398,
82.5630023793679));
#136056=CARTESIAN_POINT('Ctrl Pts',(71.6285374682991,-5.57206334237799,
83.2450686800099));
#136057=CARTESIAN_POINT('Ctrl Pts',(70.5777712225591,-4.10373939010499,
83.8732652363599));
#136058=CARTESIAN_POINT('Ctrl Pts',(69.9060018891791,-2.47264156110999,
84.3293618700599));
#136059=CARTESIAN_POINT('Ctrl Pts',(69.6940862081691,-1.32753454776999,
84.49710121691));
#136060=CARTESIAN_POINT('Ctrl Pts',(69.6467257282991,-0.785616277860386,
84.5431000349299));
#136061=CARTESIAN_POINT('Ctrl Pts',(85.0472461895191,-0.800502691495985,
82.0775712267681));
#136062=CARTESIAN_POINT('Ctrl Pts',(84.9851471753292,-1.34836358114699,
82.050322866006));
#136063=CARTESIAN_POINT('Ctrl Pts',(84.7216504272292,-2.50426266210099,
81.964575828032));
#136064=CARTESIAN_POINT('Ctrl Pts',(83.9187195090792,-4.14108424026399,
81.7650369409531));
#136065=CARTESIAN_POINT('Ctrl Pts',(82.7046613300891,-5.60012874920398,
81.534791048907));
#136066=CARTESIAN_POINT('Ctrl Pts',(81.2083600665691,-6.72954445694999,
81.355816937138));
#136067=CARTESIAN_POINT('Ctrl Pts',(79.5666132765091,-7.47593236707499,
81.300973241494));
#136068=CARTESIAN_POINT('Ctrl Pts',(77.8858425823791,-7.84045426776599,
81.413185255052));
#136069=CARTESIAN_POINT('Ctrl Pts',(76.2211447682492,-7.84110567342098,
81.706377531878));
#136070=CARTESIAN_POINT('Ctrl Pts',(74.6019362569691,-7.47759387726698,
82.1755699227481));
#136071=CARTESIAN_POINT('Ctrl Pts',(73.0753129150491,-6.73098529397899,
82.7893114006941));
#136072=CARTESIAN_POINT('Ctrl Pts',(71.7285752976792,-5.60017339364298,
83.4702096729801));
#136073=CARTESIAN_POINT('Ctrl Pts',(70.6659436097491,-4.13978608838599,
84.1021953465));
#136074=CARTESIAN_POINT('Ctrl Pts',(69.9801822737691,-2.50329122298799,
84.5640276126));
#136075=CARTESIAN_POINT('Ctrl Pts',(69.7621119598991,-1.34799747674499,
84.73457509318));
#136076=CARTESIAN_POINT('Ctrl Pts',(69.7131142654991,-0.800678270688187,
84.7813801232101));
#136077=CARTESIAN_POINT('Ctrl Pts',(84.8488051384291,-0.786200190774086,
82.225315821893));
#136078=CARTESIAN_POINT('Ctrl Pts',(84.7873311119291,-1.32191566921299,
82.1977236032581));
#136079=CARTESIAN_POINT('Ctrl Pts',(84.5270803868991,-2.45160526767999,
82.1106264707551));
#136080=CARTESIAN_POINT('Ctrl Pts',(83.7369373580592,-4.04696374136098,
81.907358225748));
#136081=CARTESIAN_POINT('Ctrl Pts',(82.5475410294591,-5.46291975204299,
81.672000048526));
#136082=CARTESIAN_POINT('Ctrl Pts',(81.0891311949791,-6.55325925884998,
81.486962840279));
#136083=CARTESIAN_POINT('Ctrl Pts',(79.4972997300592,-7.26994271334799,
81.424922709271));
#136084=CARTESIAN_POINT('Ctrl Pts',(77.8746492819691,-7.61844194255998,
81.528241411345));
#136085=CARTESIAN_POINT('Ctrl Pts',(76.2708038416291,-7.619063639597,81.810706638627));
#136086=CARTESIAN_POINT('Ctrl Pts',(74.7093158197091,-7.27153427949499,
82.268368564623));
#136087=CARTESIAN_POINT('Ctrl Pts',(73.2321591228391,-6.55464945045899,
82.87177871305));
#136088=CARTESIAN_POINT('Ctrl Pts',(71.9231550752991,-5.46296592454899,
83.54540390462));
#136089=CARTESIAN_POINT('Ctrl Pts',(70.8854551199492,-4.04570102716299,
84.1737588213101));
#136090=CARTESIAN_POINT('Ctrl Pts',(70.2129742283391,-2.45065611591499,
84.63472359839));
#136091=CARTESIAN_POINT('Ctrl Pts',(69.9984125344692,-1.32155762322899,
84.8054295158));
#136092=CARTESIAN_POINT('Ctrl Pts',(69.9501192544392,-0.786371876604886,
84.8523437644201));
#136093=CARTESIAN_POINT('Ctrl Pts',(84.6201212081591,-0.756035202698286,
82.134731082037));
#136094=CARTESIAN_POINT('Ctrl Pts',(84.5611229699591,-1.27351763615699,
82.1069735901909));
#136095=CARTESIAN_POINT('Ctrl Pts',(84.3110503697891,-2.36533664275899,
82.018984730497));
#136096=CARTESIAN_POINT('Ctrl Pts',(83.5495281178791,-3.91151837616499,
81.8123817792899));
#136097=CARTESIAN_POINT('Ctrl Pts',(82.398606548459,-5.28991034745799,81.5711261636109));
#136098=CARTESIAN_POINT('Ctrl Pts',(80.980911438569,-6.35702795855899,81.378192136185));
#136099=CARTESIAN_POINT('Ctrl Pts',(79.4265499277991,-7.06233584602099,
81.30768165016));
#136100=CARTESIAN_POINT('Ctrl Pts',(77.8366962050891,-7.40683034689099,
81.403644412078));
#136101=CARTESIAN_POINT('Ctrl Pts',(76.2637432396491,-7.40744598837599,
81.6806591353349));
#136102=CARTESIAN_POINT('Ctrl Pts',(74.7355998470391,-7.06390599830199,
82.1340120919569));
#136103=CARTESIAN_POINT('Ctrl Pts',(73.2965980661991,-6.35838933813399,
82.732562583319));
#136104=CARTESIAN_POINT('Ctrl Pts',(72.0286109742291,-5.28995245772899,
83.3996747765199));
#136105=CARTESIAN_POINT('Ctrl Pts',(71.0291066107991,-3.91029205061899,
84.0204061706));
#136106=CARTESIAN_POINT('Ctrl Pts',(70.3846430642991,-2.36441905166499,
84.47471916893));
#136107=CARTESIAN_POINT('Ctrl Pts',(70.1799414212691,-1.27317183330099,
84.6427842761299));
#136108=CARTESIAN_POINT('Ctrl Pts',(70.1340292806191,-0.756201046184986,
84.6890076573999));
#136109=CARTESIAN_POINT('Ctrl Pts',(84.3914372778792,-0.725870214622486,
82.044146342181));
#136110=CARTESIAN_POINT('Ctrl Pts',(84.3349148279891,-1.22511960310099,
82.016223577123));
#136111=CARTESIAN_POINT('Ctrl Pts',(84.0950203526892,-2.27906801783799,
81.92734299024));
#136112=CARTESIAN_POINT('Ctrl Pts',(83.3621188776991,-3.77607301096799,
81.717405332832));
#136113=CARTESIAN_POINT('Ctrl Pts',(82.2496720674591,-5.11690094287299,
81.470252278697));
#136114=CARTESIAN_POINT('Ctrl Pts',(80.8726916821591,-6.16079665826698,
81.26942143209));
#136115=CARTESIAN_POINT('Ctrl Pts',(79.3558001255291,-6.85472897869398,
81.1904405910481));
#136116=CARTESIAN_POINT('Ctrl Pts',(77.7987431282091,-7.19521875122099,
81.2790474128101));
#136117=CARTESIAN_POINT('Ctrl Pts',(76.2566826376691,-7.19582833715499,
81.5506116320421));
#136118=CARTESIAN_POINT('Ctrl Pts',(74.7618838743691,-6.85627771710999,
81.999655619291));
#136119=CARTESIAN_POINT('Ctrl Pts',(73.361037009559,-6.162129225809,82.5933464535881));
#136120=CARTESIAN_POINT('Ctrl Pts',(72.1340668731491,-5.11693899090998,
83.2539456484301));
#136121=CARTESIAN_POINT('Ctrl Pts',(71.1727581016391,-3.77488307407499,
83.86705351989));
#136122=CARTESIAN_POINT('Ctrl Pts',(70.5563119002591,-2.27818198741599,
84.31471473947));
#136123=CARTESIAN_POINT('Ctrl Pts',(70.3614703080691,-1.22478604337199,
84.48013903646));
#136124=CARTESIAN_POINT('Ctrl Pts',(70.3179393067991,-0.726030215765186,
84.52567155037));
#136125=CARTESIAN_POINT('Ctrl Pts',(84.3483675511692,-0.708315777590186,
81.800736122662));
#136126=CARTESIAN_POINT('Ctrl Pts',(84.2938347685092,-1.20045484352899,
81.772982672117));
#136127=CARTESIAN_POINT('Ctrl Pts',(84.0614432845091,-2.24061799304199,
81.6845104357261));
#136128=CARTESIAN_POINT('Ctrl Pts',(83.3459800322391,-3.72715103435799,
81.474780386873));
#136129=CARTESIAN_POINT('Ctrl Pts',(82.2495041742791,-5.07139646376999,
81.2265113930151));
#136130=CARTESIAN_POINT('Ctrl Pts',(80.8776307673491,-6.12984397173298,
81.0234038922981));
#136131=CARTESIAN_POINT('Ctrl Pts',(79.3503955238792,-6.84146712689498,
80.942674030654));
#136132=CARTESIAN_POINT('Ctrl Pts',(77.7698545693192,-7.193750217943,81.032405630159));
#136133=CARTESIAN_POINT('Ctrl Pts',(76.1995669341991,-7.19438311728998,
81.3089406769521));
#136134=CARTESIAN_POINT('Ctrl Pts',(74.6822626061291,-6.84306319438998,
81.764964470253));
#136135=CARTESIAN_POINT('Ctrl Pts',(73.2722441158392,-6.13119675659699,
82.363854399566));
#136136=CARTESIAN_POINT('Ctrl Pts',(72.0508580000791,-5.07142869365499,
83.0248483636501));
#136137=CARTESIAN_POINT('Ctrl Pts',(71.1049554729691,-3.72596408947099,
83.63353586708));
#136138=CARTESIAN_POINT('Ctrl Pts',(70.5048176610391,-2.23974300617899,
84.0750396996601));
#136139=CARTESIAN_POINT('Ctrl Pts',(70.3168805484591,-1.20012615522599,
84.23751662696));
#136140=CARTESIAN_POINT('Ctrl Pts',(70.2751598299691,-0.708473502053986,
84.28221030427));
#136141=CARTESIAN_POINT('Ctrl Pts',(84.531565980199,-0.719941702880786,
81.6342578001199));
#136142=CARTESIAN_POINT('Ctrl Pts',(84.4766586765791,-1.22280467433099,
81.6068484341241));
#136143=CARTESIAN_POINT('Ctrl Pts',(84.2420129006891,-2.28627993701699,
81.519699179736));
#136144=CARTESIAN_POINT('Ctrl Pts',(83.5163452015191,-3.81093039657899,
81.31352309037));
#136145=CARTESIAN_POINT('Ctrl Pts',(82.398261345009,-5.19634904981199,81.0699730023531));
#136146=CARTESIAN_POINT('Ctrl Pts',(80.9910666415091,-6.29338645392199,
80.872357969515));
#136147=CARTESIAN_POINT('Ctrl Pts',(79.4154375811891,-7.03506828713499,
80.7982513399819));
#136148=CARTESIAN_POINT('Ctrl Pts',(77.7772987323591,-7.40381091052299,
80.896526746002));
#136149=CARTESIAN_POINT('Ctrl Pts',(76.1463082214191,-7.40447448647799,
81.183761937356));
#136150=CARTESIAN_POINT('Ctrl Pts',(74.5718913655091,-7.03673575225599,
81.6514660023639));
#136151=CARTESIAN_POINT('Ctrl Pts',(73.1140318986091,-6.29478940213099,
82.2607063002199));
#136152=CARTESIAN_POINT('Ctrl Pts',(71.8575260548191,-5.19637919744099,
82.928630174457));
#136153=CARTESIAN_POINT('Ctrl Pts',(70.8896983141291,-3.80971022286699,
83.5402728946901));
#136154=CARTESIAN_POINT('Ctrl Pts',(70.2787662816691,-2.28538505246999,
83.9819257520999));
#136155=CARTESIAN_POINT('Ctrl Pts',(70.0882608690891,-1.22246888756199,
84.1439308024));
#136156=CARTESIAN_POINT('Ctrl Pts',(70.0460708324691,-0.720102865311186,
84.1884294602499));
#136157=CARTESIAN_POINT('Ctrl Pts',(84.7549627479325,-0.99814350218451,
82.1379981311978));
#136158=CARTESIAN_POINT('Ctrl Pts',(84.7360744487648,-1.13241223971952,
82.1299177820536));
#136159=CARTESIAN_POINT('Ctrl Pts',(84.7136170682954,-1.26571601940023,
82.1210096891642));
#136160=CARTESIAN_POINT('Ctrl Pts',(84.6876572285705,-1.39804856021889,
82.1113348976728));
#136161=CARTESIAN_POINT('Ctrl Pts',(84.6614814584809,-1.53148182485237,
82.1015796326007));
#136162=CARTESIAN_POINT('Ctrl Pts',(84.6317445010843,-1.66392813449533,
82.0910446876825));
#136163=CARTESIAN_POINT('Ctrl Pts',(84.5984643610126,-1.79536714138599,
82.0797821861936));
#136164=CARTESIAN_POINT('Ctrl Pts',(84.5650886283709,-1.92718368852826,
82.0684873347368));
#136165=CARTESIAN_POINT('Ctrl Pts',(84.5281490881766,-2.05798764684406,
82.0564605808227));
#136166=CARTESIAN_POINT('Ctrl Pts',(84.4876170667267,-2.18773691933232,
82.0437465570486));
#136167=CARTESIAN_POINT('Ctrl Pts',(84.4724313855847,-2.23634863446342,
82.0389831353351));
#136168=CARTESIAN_POINT('Ctrl Pts',(84.4567409789409,-2.28481204838324,
82.0341231745087));
#136169=CARTESIAN_POINT('Ctrl Pts',(84.4405427555362,-2.33312394443514,
82.0291688025217));
#136170=CARTESIAN_POINT('Ctrl Pts',(84.4390468242843,-2.33758562355486,
82.0287112585242));
#136171=CARTESIAN_POINT('Ctrl Pts',(84.4375465613714,-2.34204600997798,
82.0282529092394));
#136172=CARTESIAN_POINT('Ctrl Pts',(84.4360419658959,-2.34650510524211,
82.0277937580412));
#136173=CARTESIAN_POINT('Ctrl Pts',(84.3879187107657,-2.48912561855823,
82.0131081826739));
#136174=CARTESIAN_POINT('Ctrl Pts',(84.3354085581316,-2.63044179820462,
81.9975928703134));
#136175=CARTESIAN_POINT('Ctrl Pts',(84.2785407679911,-2.7704378407857,81.9813486682572));
#136176=CARTESIAN_POINT('Ctrl Pts',(84.2481717672931,-2.84519966825197,
81.9726738071034));
#136177=CARTESIAN_POINT('Ctrl Pts',(84.2165592642238,-2.91958456298685,
81.9637910023635));
#136178=CARTESIAN_POINT('Ctrl Pts',(84.1837027095352,-2.99358666842466,
81.9547153285447));
#136179=CARTESIAN_POINT('Ctrl Pts',(84.1365114894892,-3.09987442971577,
81.9416801176313));
#136180=CARTESIAN_POINT('Ctrl Pts',(84.0867580073447,-3.2053758055543,81.9282459220336));
#136181=CARTESIAN_POINT('Ctrl Pts',(84.034448766139,-3.31008109859886,81.9144497094881));
#136182=CARTESIAN_POINT('Ctrl Pts',(84.0082941455361,-3.36243374512114,
81.9075516032154));
#136183=CARTESIAN_POINT('Ctrl Pts',(83.9815005706135,-3.41458735658898,
81.9005629111546));
#136184=CARTESIAN_POINT('Ctrl Pts',(83.9540687613753,-3.46654073992166,
81.8934877212652));
#136185=CARTESIAN_POINT('Ctrl Pts',(83.9403528567561,-3.49251743158801,
81.8899501263205));
#136186=CARTESIAN_POINT('Ctrl Pts',(83.9264773926352,-3.51844406489059,
81.886390901512));
#136187=CARTESIAN_POINT('Ctrl Pts',(83.9124424531876,-3.5443204855787,81.8828105236135));
#136188=CARTESIAN_POINT('Ctrl Pts',(83.9021601880128,-3.56327804647741,
81.8801874702604));
#136189=CARTESIAN_POINT('Ctrl Pts',(83.8921228909752,-3.58160738984613,
81.877636985306));
#136190=CARTESIAN_POINT('Ctrl Pts',(83.8816051507227,-3.60063058216534,
81.874974903863));
#136191=CARTESIAN_POINT('Ctrl Pts',(83.8777665361195,-3.60757339517311,
81.8740033354028));
#136192=CARTESIAN_POINT('Ctrl Pts',(83.8738635042219,-3.61460838629155,
81.8730168606676));
#136193=CARTESIAN_POINT('Ctrl Pts',(83.8698592890158,-3.62179895102489,
81.8720063837862));
#136194=CARTESIAN_POINT('Ctrl Pts',(83.8055567097488,-3.73727023189799,
81.8557794163486));
#136195=CARTESIAN_POINT('Ctrl Pts',(83.7386745311195,-3.85060309564398,
81.8392979899471));
#136196=CARTESIAN_POINT('Ctrl Pts',(83.6692606961145,-3.96180672417764,
81.822653964058));
#136197=CARTESIAN_POINT('Ctrl Pts',(83.5909232222349,-4.08730636477421,
81.8038702310565));
#136198=CARTESIAN_POINT('Ctrl Pts',(83.5093615914043,-4.21009506539025,
81.784879210787));
#136199=CARTESIAN_POINT('Ctrl Pts',(83.4246113298914,-4.33020869538295,
81.7658426068169));
#136200=CARTESIAN_POINT('Ctrl Pts',(83.3385057774693,-4.45224313255535,
81.7465015773991));
#136201=CARTESIAN_POINT('Ctrl Pts',(83.2491083602584,-4.57151647204202,
81.7271131680751));
#136202=CARTESIAN_POINT('Ctrl Pts',(83.1564231635584,-4.68802431461752,
81.707849683635));
#136203=CARTESIAN_POINT('Ctrl Pts',(83.1199550191273,-4.73386577562394,
81.700270225881));
#136204=CARTESIAN_POINT('Ctrl Pts',(83.0829775630784,-4.77927863195264,
81.69271016344));
#136205=CARTESIAN_POINT('Ctrl Pts',(83.0454898973026,-4.82426075402366,
81.6851802546591));
#136206=CARTESIAN_POINT('Ctrl Pts',(82.9501617902535,-4.93864665827622,
81.6660323046475));
#136207=CARTESIAN_POINT('Ctrl Pts',(82.8515564168775,-5.05027360440036,
81.6470681875175));
#136208=CARTESIAN_POINT('Ctrl Pts',(82.7497100436443,-5.15917427335519,
81.6284219468575));
#136209=CARTESIAN_POINT('Ctrl Pts',(82.6861528954071,-5.22713364922855,
81.6167857751994));
#136210=CARTESIAN_POINT('Ctrl Pts',(82.6213327335815,-5.29403071669238,
81.6052733983345));
#136211=CARTESIAN_POINT('Ctrl Pts',(82.5552505652913,-5.35986676314358,
81.5939182192025));
#136212=CARTESIAN_POINT('Ctrl Pts',(82.5384537895867,-5.37660097956119,
81.5910319580234));
#136213=CARTESIAN_POINT('Ctrl Pts',(82.5215755786135,-5.39326681014543,
81.5881557678984));
#136214=CARTESIAN_POINT('Ctrl Pts',(82.5046160985963,-5.40986432477732,
81.5852901326943));
#136215=CARTESIAN_POINT('Ctrl Pts',(82.4347552855232,-5.47823410179861,
81.5734857846171));
#136216=CARTESIAN_POINT('Ctrl Pts',(82.3635160576312,-5.54544506882284,
81.5618604322946));
#136217=CARTESIAN_POINT('Ctrl Pts',(82.2909042280843,-5.61150565977019,
81.550453444742));
#136218=CARTESIAN_POINT('Ctrl Pts',(82.2457846535634,-5.65255442241319,
81.5433653651804));
#136219=CARTESIAN_POINT('Ctrl Pts',(82.2001352523272,-5.69315901295719,
81.5363615340839));
#136220=CARTESIAN_POINT('Ctrl Pts',(82.15395761102,-5.73332162022948,81.5294509463107));
#136221=CARTESIAN_POINT('Ctrl Pts',(82.1279475844843,-5.75594361761455,
81.5255584874005));
#136222=CARTESIAN_POINT('Ctrl Pts',(82.1013153617168,-5.77881549905558,
81.5216285233666));
#136223=CARTESIAN_POINT('Ctrl Pts',(82.0748265419983,-5.80127511088066,
81.5177767301801));
#136224=CARTESIAN_POINT('Ctrl Pts',(82.0542876812979,-5.81868981049962,
81.5147901326441));
#136225=CARTESIAN_POINT('Ctrl Pts',(82.0338357770383,-5.83585745707664,
81.5118503788618));
#136226=CARTESIAN_POINT('Ctrl Pts',(82.0138415095347,-5.85248560413429,
81.5090076667125));
#136227=CARTESIAN_POINT('Ctrl Pts',(81.8986996425497,-5.9482428453725,81.4926372153268));
#136228=CARTESIAN_POINT('Ctrl Pts',(81.7817255834563,-6.04015142672838,
81.4771184995858));
#136229=CARTESIAN_POINT('Ctrl Pts',(81.662976231238,-6.12830999999474,81.462606173832));
#136230=CARTESIAN_POINT('Ctrl Pts',(81.5421023396451,-6.21804581437126,
81.447834208704));
#136231=CARTESIAN_POINT('Ctrl Pts',(81.4193886010348,-6.30389644475892,
81.4341046199841));
#136232=CARTESIAN_POINT('Ctrl Pts',(81.2948623372305,-6.38592298340322,
81.4215837817183));
#136233=CARTESIAN_POINT('Ctrl Pts',(81.2160303171265,-6.43785032423818,
81.4136573978075));
#136234=CARTESIAN_POINT('Ctrl Pts',(81.1364712807916,-6.4882442571981,81.4062155196424));
#136235=CARTESIAN_POINT('Ctrl Pts',(81.0561868626913,-6.53711103817155,
81.3993019051947));
#136236=CARTESIAN_POINT('Ctrl Pts',(80.9915799369693,-6.5764353873208,81.3937383427295));
#136237=CARTESIAN_POINT('Ctrl Pts',(80.9265031831495,-6.61477064596132,
81.3885168921367));
#136238=CARTESIAN_POINT('Ctrl Pts',(80.8609607459812,-6.65211621421108,
81.3836595627514));
#136239=CARTESIAN_POINT('Ctrl Pts',(80.7366263364312,-6.72296098865415,
81.3744451788009));
#136240=CARTESIAN_POINT('Ctrl Pts',(80.6106167089957,-6.79027164309577,
81.3665297512573));
#136241=CARTESIAN_POINT('Ctrl Pts',(80.4829624543209,-6.85410722446704,
81.3600260293172));
#136242=CARTESIAN_POINT('Ctrl Pts',(80.4042283439736,-6.89347949388779,
81.3560146881973));
#136243=CARTESIAN_POINT('Ctrl Pts',(80.3248678990058,-6.93152908843398,
81.3525405705145));
#136244=CARTESIAN_POINT('Ctrl Pts',(80.244882277825,-6.96826245974566,81.3496327876378));
#136245=CARTESIAN_POINT('Ctrl Pts',(80.1400477816455,-7.01640766906684,
81.3458216532317));
#136246=CARTESIAN_POINT('Ctrl Pts',(80.0341430047996,-7.06229648467652,
81.342980692216));
#136247=CARTESIAN_POINT('Ctrl Pts',(79.9271780363573,-7.10595372188797,
81.3411672326213));
#136248=CARTESIAN_POINT('Ctrl Pts',(79.8736955521362,-7.12778234049369,
81.340260502824));
#136249=CARTESIAN_POINT('Ctrl Pts',(79.8199480149917,-7.14905305259735,
81.3396106217187));
#136250=CARTESIAN_POINT('Ctrl Pts',(79.7659366481784,-7.16976899764375,
81.3392245662652));
#136251=CARTESIAN_POINT('Ctrl Pts',(79.7337719231639,-7.18210570962021,
81.3389946634089));
#136252=CARTESIAN_POINT('Ctrl Pts',(79.7010237910141,-7.19442951282771,
81.3388564533094));
#136253=CARTESIAN_POINT('Ctrl Pts',(79.6685665191181,-7.20640952989372,
81.3388161853128));
#136254=CARTESIAN_POINT('Ctrl Pts',(79.6465211761977,-7.21454649178191,
81.338788834838));
#136255=CARTESIAN_POINT('Ctrl Pts',(79.6246103822755,-7.22252580680398,
81.3388062332073));
#136256=CARTESIAN_POINT('Ctrl Pts',(79.6031122661378,-7.2302556298964,81.3388647593018));
#136257=CARTESIAN_POINT('Ctrl Pts',(79.5584502322042,-7.24631422866124,
81.3389863464401));
#136258=CARTESIAN_POINT('Ctrl Pts',(79.5137873203361,-7.26192891990934,
81.3392941039157));
#136259=CARTESIAN_POINT('Ctrl Pts',(79.4691233092725,-7.27710452603065,
81.3397909651462));
#136260=CARTESIAN_POINT('Ctrl Pts',(79.3345029844086,-7.32284482067527,
81.3412885382182));
#136261=CARTESIAN_POINT('Ctrl Pts',(79.1998747063359,-7.3645999865306,81.344502458572));
#136262=CARTESIAN_POINT('Ctrl Pts',(79.0652674206663,-7.40249677718022,
81.3494555717584));
#136263=CARTESIAN_POINT('Ctrl Pts',(78.933472145338,-7.43960188581444,81.35430521205));
#136264=CARTESIAN_POINT('Ctrl Pts',(78.8016963053603,-7.47300794763936,
81.3608221119125));
#136265=CARTESIAN_POINT('Ctrl Pts',(78.6699471663124,-7.50278713154373,
81.3690474907127));
#136266=CARTESIAN_POINT('Ctrl Pts',(78.533981488312,-7.5335193773794,81.3775361170026));
#136267=CARTESIAN_POINT('Ctrl Pts',(78.3980437019746,-7.56038914233644,
81.3878441265407));
#136268=CARTESIAN_POINT('Ctrl Pts',(78.2621295209197,-7.58342428445968,
81.4000401022841));
#136269=CARTESIAN_POINT('Ctrl Pts',(78.1262153398648,-7.60645942658291,
81.4122360780274));
#136270=CARTESIAN_POINT('Ctrl Pts',(77.9903241708066,-7.62565997343611,
81.4263199514631));
#136271=CARTESIAN_POINT('Ctrl Pts',(77.8544483957737,-7.6410013238083,81.4423850973286));
#136272=CARTESIAN_POINT('Ctrl Pts',(77.7209526142816,-7.65607395582517,
81.4581688468717));
#136273=CARTESIAN_POINT('Ctrl Pts',(77.5874711687472,-7.66742130973048,
81.4758650585326));
#136274=CARTESIAN_POINT('Ctrl Pts',(77.4540138689537,-7.67503337615444,
81.4954788561316));
#136275=CARTESIAN_POINT('Ctrl Pts',(77.3205565691602,-7.6826454425784,81.5150926537307));
#136276=CARTESIAN_POINT('Ctrl Pts',(77.1871229045546,-7.68652218089232,
81.5366242464878));
#136277=CARTESIAN_POINT('Ctrl Pts',(77.0537354665173,-7.68660419195478,
81.5601015030313));
#136278=CARTESIAN_POINT('Ctrl Pts',(76.9202673858979,-7.68668625259899,
81.5835929533145));
#136279=CARTESIAN_POINT('Ctrl Pts',(76.7874208243268,-7.68303005328711,
81.6088991951285));
#136280=CARTESIAN_POINT('Ctrl Pts',(76.6551998873563,-7.67566113397853,
81.6360063004115));
#136281=CARTESIAN_POINT('Ctrl Pts',(76.5229789503857,-7.66829221466995,
81.6631134056944));
#136282=CARTESIAN_POINT('Ctrl Pts',(76.3913831051237,-7.65721057010139,
81.6920214619695));
#136283=CARTESIAN_POINT('Ctrl Pts',(76.2604215554106,-7.64239141385766,
81.7227409989038));
#136284=CARTESIAN_POINT('Ctrl Pts',(76.1309714136242,-7.62774328331012,
81.7531060061938));
#136285=CARTESIAN_POINT('Ctrl Pts',(76.0021406178159,-7.60944320485009,
81.7852412915906));
#136286=CARTESIAN_POINT('Ctrl Pts',(75.8739036080351,-7.58748086647297,
81.8190837299511));
#136287=CARTESIAN_POINT('Ctrl Pts',(75.8490812052546,-7.58322969116773,
81.8256344958921));
#136288=CARTESIAN_POINT('Ctrl Pts',(75.824281097167,-7.57884115868288,81.8322492794074));
#136289=CARTESIAN_POINT('Ctrl Pts',(75.7995031705135,-7.57431499439249,
81.8389276969693));
#136290=CARTESIAN_POINT('Ctrl Pts',(75.6703568634415,-7.55072394048887,
81.8737366209468));
#136291=CARTESIAN_POINT('Ctrl Pts',(75.5418227299606,-7.52338594290897,
81.9102768687294));
#136292=CARTESIAN_POINT('Ctrl Pts',(75.4138856636451,-7.49228417086409,
81.9484803963819));
#136293=CARTESIAN_POINT('Ctrl Pts',(75.3378562073981,-7.47380124886977,
81.9711836951037));
#136294=CARTESIAN_POINT('Ctrl Pts',(75.2620377881377,-7.45398821726154,
81.9944747601753));
#136295=CARTESIAN_POINT('Ctrl Pts',(75.186429615227,-7.43283364015822,82.0183421750203));
#136296=CARTESIAN_POINT('Ctrl Pts',(75.0850114487219,-7.40445762814239,
82.0503570929796));
#136297=CARTESIAN_POINT('Ctrl Pts',(74.9839698448508,-7.37367323551073,
82.0834066995368));
#136298=CARTESIAN_POINT('Ctrl Pts',(74.8832988954068,-7.34046442508238,
82.1174574003437));
#136299=CARTESIAN_POINT('Ctrl Pts',(74.8329634206847,-7.32386001986821,
82.1344827507471));
#136300=CARTESIAN_POINT('Ctrl Pts',(74.782720607907,-7.30664950030032,82.1517583620035));
#136301=CARTESIAN_POINT('Ctrl Pts',(74.7325697048827,-7.28883083654385,
82.1692799170975));
#136302=CARTESIAN_POINT('Ctrl Pts',(74.7240302608494,-7.2857967639206,82.1722633995491));
#136303=CARTESIAN_POINT('Ctrl Pts',(74.7155330656988,-7.28275913879809,
82.1752401765379));
#136304=CARTESIAN_POINT('Ctrl Pts',(74.7070577589877,-7.27971106113057,
82.1782171902271));
#136305=CARTESIAN_POINT('Ctrl Pts',(74.6776617970466,-7.26913903369103,
82.188542737619));
#136306=CARTESIAN_POINT('Ctrl Pts',(74.6485275155047,-7.25844464497075,
82.1988700083502));
#136307=CARTESIAN_POINT('Ctrl Pts',(74.6188180851307,-7.24731174775921,
82.2094977507359));
#136308=CARTESIAN_POINT('Ctrl Pts',(74.6067881907205,-7.24280383305841,
82.2138011189631));
#136309=CARTESIAN_POINT('Ctrl Pts',(74.5946642400973,-7.23822351646149,
82.2181539192958));
#136310=CARTESIAN_POINT('Ctrl Pts',(74.5823917165411,-7.23354770312353,
82.2225766637255));
#136311=CARTESIAN_POINT('Ctrl Pts',(74.4580746745002,-7.18618309382779,
82.2673777596604));
#136312=CARTESIAN_POINT('Ctrl Pts',(74.3357407315584,-7.13550734464184,
82.3131825148036));
#136313=CARTESIAN_POINT('Ctrl Pts',(74.2153309053991,-7.0815174423743,82.3598796338195));
#136314=CARTESIAN_POINT('Ctrl Pts',(74.0935049939706,-7.02689258939118,
82.40712593644));
#136315=CARTESIAN_POINT('Ctrl Pts',(73.973648537563,-6.96887488323718,82.4552861201515));
#136316=CARTESIAN_POINT('Ctrl Pts',(73.8557364363267,-6.90742206970627,
82.5042519222903));
#136317=CARTESIAN_POINT('Ctrl Pts',(73.7369227152364,-6.84549935464542,
82.5535921435));
#136318=CARTESIAN_POINT('Ctrl Pts',(73.6200830207485,-6.78008853136454,
82.6037508515811));
#136319=CARTESIAN_POINT('Ctrl Pts',(73.50523071568,-6.71111110896202,82.654617501447));
#136320=CARTESIAN_POINT('Ctrl Pts',(73.474673851995,-6.69275942074431,82.6681507543072));
#136321=CARTESIAN_POINT('Ctrl Pts',(73.4442578854804,-6.67415509260198,
82.6817340957715));
#136322=CARTESIAN_POINT('Ctrl Pts',(73.4139835532656,-6.65529626560641,
82.6953653726223));
#136323=CARTESIAN_POINT('Ctrl Pts',(73.3532577660512,-6.61746827630128,
82.7227076773718));
#136324=CARTESIAN_POINT('Ctrl Pts',(73.2930910845494,-6.57862296025367,
82.7502418956387));
#136325=CARTESIAN_POINT('Ctrl Pts',(73.233481559248,-6.53875599409344,82.7779467051893));
#136326=CARTESIAN_POINT('Ctrl Pts',(73.1187118027947,-6.46199775833156,
82.8312884190953));
#136327=CARTESIAN_POINT('Ctrl Pts',(73.006005545972,-6.38145478231525,82.8852628427268));
#136328=CARTESIAN_POINT('Ctrl Pts',(72.8953331151939,-6.29706100314168,
82.9397174782743));
#136329=CARTESIAN_POINT('Ctrl Pts',(72.8890306839395,-6.29225505474236,
82.9428184908265));
#136330=CARTESIAN_POINT('Ctrl Pts',(72.8827348566264,-6.28743660724246,
82.9459210592896));
#136331=CARTESIAN_POINT('Ctrl Pts',(72.876445630877,-6.28260564440167,82.9490251549171));
#136332=CARTESIAN_POINT('Ctrl Pts',(72.7894002484549,-6.21574319984927,
82.9919870713344));
#136333=CARTESIAN_POINT('Ctrl Pts',(72.7036179244276,-6.14648865782259,
83.03524015749));
#136334=CARTESIAN_POINT('Ctrl Pts',(72.6190838017302,-6.0748140055321,83.0787001451335));
#136335=CARTESIAN_POINT('Ctrl Pts',(72.5768167403815,-6.03897667938686,
83.1004301389553));
#136336=CARTESIAN_POINT('Ctrl Pts',(72.534861713998,-6.00253429108223,83.1222117709614));
#136337=CARTESIAN_POINT('Ctrl Pts',(72.4932167522304,-5.96548337269157,
83.1440338661608));
#136338=CARTESIAN_POINT('Ctrl Pts',(72.4684716255418,-5.94346799242492,
83.1570003929002));
#136339=CARTESIAN_POINT('Ctrl Pts',(72.4442122146909,-5.92157790891612,
83.1697828502902));
#136340=CARTESIAN_POINT('Ctrl Pts',(72.4197650747079,-5.89920874176838,
83.1827325478749));
#136341=CARTESIAN_POINT('Ctrl Pts',(72.4030687514654,-5.8839315827378,83.1915766227612));
#136342=CARTESIAN_POINT('Ctrl Pts',(72.3862855263746,-5.86843017263442,
83.2004986849878));
#136343=CARTESIAN_POINT('Ctrl Pts',(72.36921001917,-5.85250144408564,83.209609964908));
#136344=CARTESIAN_POINT('Ctrl Pts',(72.2664577427722,-5.75664993590502,
83.2644373115564));
#136345=CARTESIAN_POINT('Ctrl Pts',(72.1668936099123,-5.65813854884049,
83.3187729618543));
#136346=CARTESIAN_POINT('Ctrl Pts',(72.0704444321277,-5.55696396556987,
83.3724839663531));
#136347=CARTESIAN_POINT('Ctrl Pts',(72.0239516868539,-5.50819336704083,
83.3983750325906));
#136348=CARTESIAN_POINT('Ctrl Pts',(71.9781833304177,-5.45880339191821,
83.4241209393293));
#136349=CARTESIAN_POINT('Ctrl Pts',(71.9331344087398,-5.40879086198571,
83.4497065171101));
#136350=CARTESIAN_POINT('Ctrl Pts',(71.8384680863801,-5.3036939561272,83.5034723446536));
#136351=CARTESIAN_POINT('Ctrl Pts',(71.7469760400854,-5.19584976202539,
83.5565309520128));
#136352=CARTESIAN_POINT('Ctrl Pts',(71.6586524489669,-5.08522986784536,
83.6087501663433));
#136353=CARTESIAN_POINT('Ctrl Pts',(71.5905511639268,-4.99993717481426,
83.6490134250567));
#136354=CARTESIAN_POINT('Ctrl Pts',(71.5243343689076,-4.91299360910555,
83.6887775636091));
#136355=CARTESIAN_POINT('Ctrl Pts',(71.4600165668395,-4.82437529006003,
83.7279761120231));
#136356=CARTESIAN_POINT('Ctrl Pts',(71.3770393817778,-4.71004771009223,
83.7785466399534));
#136357=CARTESIAN_POINT('Ctrl Pts',(71.2971899486146,-4.59294591585182,
83.8281775698261));
#136358=CARTESIAN_POINT('Ctrl Pts',(71.2204294110572,-4.47306146190551,
83.8767110777767));
#136359=CARTESIAN_POINT('Ctrl Pts',(71.1724066958443,-4.39805968138773,
83.9070744767935));
#136360=CARTESIAN_POINT('Ctrl Pts',(71.1255935713537,-4.32196797949701,
83.9370082301691));
#136361=CARTESIAN_POINT('Ctrl Pts',(71.0799873234695,-4.2447766950706,83.9664715749255));
#136362=CARTESIAN_POINT('Ctrl Pts',(71.0249406041176,-4.15160685174068,
84.0020338179343));
#136363=CARTESIAN_POINT('Ctrl Pts',(70.9716483317067,-4.05683928399666,
84.0369103266833));
#136364=CARTESIAN_POINT('Ctrl Pts',(70.9200963792618,-3.96046726874635,
84.0710235032939));
#136365=CARTESIAN_POINT('Ctrl Pts',(70.9161579623552,-3.95310473141867,
84.0736296492327));
#136366=CARTESIAN_POINT('Ctrl Pts',(70.9122297077862,-3.94573282279201,
84.076231338417));
#136367=CARTESIAN_POINT('Ctrl Pts',(70.9083116133528,-3.93835154817217,
84.0788285415872));
#136368=CARTESIAN_POINT('Ctrl Pts',(70.8807095955352,-3.88635227223872,
84.0971252032424));
#136369=CARTESIAN_POINT('Ctrl Pts',(70.8536115023071,-3.8338881617024,84.1151993319809));
#136370=CARTESIAN_POINT('Ctrl Pts',(70.8270155955156,-3.78095909067874,
84.1330410827773));
#136371=CARTESIAN_POINT('Ctrl Pts',(70.8137176421198,-3.75449455516691,
84.1419619581755));
#136372=CARTESIAN_POINT('Ctrl Pts',(70.8005452341496,-3.72791377663219,
84.15082473169));
#136373=CARTESIAN_POINT('Ctrl Pts',(70.7874981462678,-3.70121673421146,
84.1596281235744));
#136374=CARTESIAN_POINT('Ctrl Pts',(70.7780962506347,-3.68197850964915,
84.1659719584948));
#136375=CARTESIAN_POINT('Ctrl Pts',(70.7684676576691,-3.66207455726415,
84.1724822999379));
#136376=CARTESIAN_POINT('Ctrl Pts',(70.7592441592484,-3.64281282634221,
84.1787315082593));
#136377=CARTESIAN_POINT('Ctrl Pts',(70.7556681330659,-3.63534489487485,
84.1811543777127));
#136378=CARTESIAN_POINT('Ctrl Pts',(70.7521525557527,-3.62797378993837,
84.1835382034184));
#136379=CARTESIAN_POINT('Ctrl Pts',(70.74873261181,-3.62077678971988,84.1858588405169));
#136380=CARTESIAN_POINT('Ctrl Pts',(70.688329356344,-3.49366293929857,84.2268460724291));
#136381=CARTESIAN_POINT('Ctrl Pts',(70.6315071694851,-3.36531292644329,
84.2660184693106));
#136382=CARTESIAN_POINT('Ctrl Pts',(70.5781646283892,-3.23577268923496,
84.3033262527094));
#136383=CARTESIAN_POINT('Ctrl Pts',(70.5245696607706,-3.10561944426687,
84.3408105832663));
#136384=CARTESIAN_POINT('Ctrl Pts',(70.474487159193,-2.97426429595224,84.3764129514617));
#136385=CARTESIAN_POINT('Ctrl Pts',(70.4278502244862,-2.84171706529408,
84.4100715443734));
#136386=CARTESIAN_POINT('Ctrl Pts',(70.3812679668711,-2.70932523286541,
84.4436906759872));
#136387=CARTESIAN_POINT('Ctrl Pts',(70.3381230335348,-2.5757437198833,84.4753709110724));
#136388=CARTESIAN_POINT('Ctrl Pts',(70.2983871952725,-2.44095161278315,
84.5050344211557));
#136389=CARTESIAN_POINT('Ctrl Pts',(70.2876629873508,-2.4045729016259,84.5130402331313));
#136390=CARTESIAN_POINT('Ctrl Pts',(70.2771873200981,-2.36810585696577,
84.5208990415673));
#136391=CARTESIAN_POINT('Ctrl Pts',(70.2669601445328,-2.33154973971516,
84.5286090662555));
#136392=CARTESIAN_POINT('Ctrl Pts',(70.229543400307,-2.19780695996857,84.556816660805));
#136393=CARTESIAN_POINT('Ctrl Pts',(70.1954495382031,-2.0628735825815,84.5830346153964));
#136394=CARTESIAN_POINT('Ctrl Pts',(70.1646701972361,-1.92681521965721,
84.6072227704094));
#136395=CARTESIAN_POINT('Ctrl Pts',(70.1339904801362,-1.79119723848968,
84.6313326353271));
#136396=CARTESIAN_POINT('Ctrl Pts',(70.10660374315,-1.65446098223881,84.6534259993471));
#136397=CARTESIAN_POINT('Ctrl Pts',(70.0825437781818,-1.51665518632324,
84.6734379987387));
#136398=CARTESIAN_POINT('Ctrl Pts',(70.058800614693,-1.3806639017788,84.6931864968732));
#136399=CARTESIAN_POINT('Ctrl Pts',(70.0382971263697,-1.2436305189225,84.7109082196508));
#136400=CARTESIAN_POINT('Ctrl Pts',(70.021108087152,-1.10559420119456,84.7265140592814));
#136401=CARTESIAN_POINT('Ctrl Pts',(70.0166563193025,-1.06984434725915,
84.7305557962425));
#136402=CARTESIAN_POINT('Ctrl Pts',(70.0124270949701,-1.03402720429941,
84.7344554625199));
#136403=CARTESIAN_POINT('Ctrl Pts',(70.0084221937706,-0.998143435151018,
84.7382111936731));
#136404=CARTESIAN_POINT('Origin',(58.9775436614391,0.499074165591714,68.468974588834));
#136405=CARTESIAN_POINT('',(27.1339039101791,-17.49925933285,74.332577093855));
#136406=CARTESIAN_POINT('Ctrl Pts',(27.1339039101784,-17.4992593325406,
74.3325770938509));
#136407=CARTESIAN_POINT('Ctrl Pts',(27.1982913289528,-17.4950745137893,
74.6334817214542));
#136408=CARTESIAN_POINT('Ctrl Pts',(27.2828755029589,-17.4830576398145,
74.9272738053655));
#136409=CARTESIAN_POINT('Ctrl Pts',(27.3853788653411,-17.4637140526782,
75.2141944686376));
#136410=CARTESIAN_POINT('Ctrl Pts',(27.4863721644485,-17.4446554321992,
75.4968882622118));
#136411=CARTESIAN_POINT('Ctrl Pts',(27.6047606718065,-17.4184843758367,
75.7729121468281));
#136412=CARTESIAN_POINT('Ctrl Pts',(27.7383735353809,-17.3856492136401,
76.0425394622034));
#136413=CARTESIAN_POINT('Ctrl Pts',(27.8752459130299,-17.352013030715,76.3187443929808));
#136414=CARTESIAN_POINT('Ctrl Pts',(28.0280945594496,-17.3113838307385,
76.5882371363484));
#136415=CARTESIAN_POINT('Ctrl Pts',(28.1945927667414,-17.2642047518374,
76.8513508114181));
#136416=CARTESIAN_POINT('Ctrl Pts',(28.3604515551069,-17.2172068592474,
77.1134540259771));
#136417=CARTESIAN_POINT('Ctrl Pts',(28.5398553429514,-17.1637092839206,
77.3692275095003));
#136418=CARTESIAN_POINT('Ctrl Pts',(28.730509915084,-17.1041109159427,77.61903338945));
#136419=CARTESIAN_POINT('Ctrl Pts',(28.9399583222007,-17.0386376199178,
77.8934639633333));
#136420=CARTESIAN_POINT('Ctrl Pts',(29.1629774015092,-16.9658061284426,
78.1606496886631));
#136421=CARTESIAN_POINT('Ctrl Pts',(29.3963622189773,-16.8861931968548,
78.4208392935282));
#136422=CARTESIAN_POINT('Ctrl Pts',(29.5855699599087,-16.8216500826194,
78.6317779821903));
#136423=CARTESIAN_POINT('Ctrl Pts',(29.7815907945949,-16.7526500206384,
78.838119475292));
#136424=CARTESIAN_POINT('Ctrl Pts',(29.9827213544611,-16.6795013769138,
79.0400210135803));
#136425=CARTESIAN_POINT('Ctrl Pts',(30.1852441501547,-16.605846394607,79.2433201244473));
#136426=CARTESIAN_POINT('Ctrl Pts',(30.3929478467462,-16.5279897126078,
79.4421186857153));
#136427=CARTESIAN_POINT('Ctrl Pts',(30.6044386189885,-16.4461190354791,
79.6368566889028));
#136428=CARTESIAN_POINT('Ctrl Pts',(30.8188237598271,-16.3631279126954,
79.834259789744));
#136429=CARTESIAN_POINT('Ctrl Pts',(31.0371004033291,-16.2760121129733,
80.0274907773708));
#136430=CARTESIAN_POINT('Ctrl Pts',(31.257816792588,-16.1849137907709,80.2170084150241));
#136431=CARTESIAN_POINT('Ctrl Pts',(31.3023319280142,-16.1665406461052,
80.2552312372355));
#136432=CARTESIAN_POINT('Ctrl Pts',(31.3469463029,-16.148005335896,80.2933030041325));
#136433=CARTESIAN_POINT('Ctrl Pts',(31.391648004194,-16.1293087719458,80.3312274622805));
#136434=CARTESIAN_POINT('Ctrl Pts',(31.5979455906182,-16.0430244492983,
80.5062481875747));
#136435=CARTESIAN_POINT('Ctrl Pts',(31.8061017853515,-15.9533132910267,
80.6781242881749));
#136436=CARTESIAN_POINT('Ctrl Pts',(32.0158754047086,-15.8601965732316,
80.8471509506169));
#136437=CARTESIAN_POINT('Ctrl Pts',(32.2270784857348,-15.7664453296117,
81.017329412488));
#136438=CARTESIAN_POINT('Ctrl Pts',(32.4399211648802,-15.6692418259999,
81.1846197827002));
#136439=CARTESIAN_POINT('Ctrl Pts',(32.6541546846915,-15.56855720567,81.3493085237292));
#136440=CARTESIAN_POINT('Ctrl Pts',(32.7273779099949,-15.5341440445293,
81.4055977580186));
#136441=CARTESIAN_POINT('Ctrl Pts',(32.800763589346,-15.4993237904429,81.4615829181366));
#136442=CARTESIAN_POINT('Ctrl Pts',(32.8743017032979,-15.4640939912119,
81.5172749492701));
#136443=CARTESIAN_POINT('Ctrl Pts',(33.2821956378359,-15.2686848265071,
81.8261819973396));
#136444=CARTESIAN_POINT('Ctrl Pts',(33.6947782118764,-15.0606809876076,
82.1260641652557));
#136445=CARTESIAN_POINT('Ctrl Pts',(34.1084197158662,-14.8406064781875,
82.4171159496633));
#136446=CARTESIAN_POINT('Ctrl Pts',(34.2042488545752,-14.7896213848491,
82.4845444875409));
#136447=CARTESIAN_POINT('Ctrl Pts',(34.3001348340015,-14.7379882161778,
82.5514991156476));
#136448=CARTESIAN_POINT('Ctrl Pts',(34.3960325283857,-14.6857130992848,
82.6179822923526));
#136449=CARTESIAN_POINT('Ctrl Pts',(34.7537904431313,-14.4906944710184,
82.8660058013264));
#136450=CARTESIAN_POINT('Ctrl Pts',(35.1117127901067,-14.2867413796121,
83.1074757483565));
#136451=CARTESIAN_POINT('Ctrl Pts',(35.4674621532407,-14.0740785882671,
83.3426103575327));
#136452=CARTESIAN_POINT('Ctrl Pts',(35.6186855505316,-13.983679017341,83.4425623408814));
#136453=CARTESIAN_POINT('Ctrl Pts',(35.7695162523914,-13.8917050394001,
83.5413692964044));
#136454=CARTESIAN_POINT('Ctrl Pts',(35.9197744880949,-13.7981714029223,
83.6390466762019));
#136455=CARTESIAN_POINT('Ctrl Pts',(36.1573782913382,-13.6502663802506,
83.7935042127361));
#136456=CARTESIAN_POINT('Ctrl Pts',(36.3935505923242,-13.4984665969623,
83.9451369988048));
#136457=CARTESIAN_POINT('Ctrl Pts',(36.627934024532,-13.3426521202487,84.0941320905792));
#136458=CARTESIAN_POINT('Ctrl Pts',(36.8616537748734,-13.1872788489639,
84.2427052867458));
#136459=CARTESIAN_POINT('Ctrl Pts',(37.0935948225531,-13.0279133343153,
84.3886559872256));
#136460=CARTESIAN_POINT('Ctrl Pts',(37.3233966571362,-12.8643989719943,
84.5321346656806));
#136461=CARTESIAN_POINT('Ctrl Pts',(37.3517202451919,-12.8442454625675,
84.5498187324362));
#136462=CARTESIAN_POINT('Ctrl Pts',(37.3800113279564,-12.8240288832378,
84.5674651995495));
#136463=CARTESIAN_POINT('Ctrl Pts',(37.4082692233398,-12.8037489039716,
84.5850743085344));
#136464=CARTESIAN_POINT('Ctrl Pts',(37.6721007149409,-12.6144036924174,
84.7494827836253));
#136465=CARTESIAN_POINT('Ctrl Pts',(37.9330389136035,-12.4195387807628,
84.910632971492));
#136466=CARTESIAN_POINT('Ctrl Pts',(38.1907510642886,-12.2190247507161,
85.0684847317907));
#136467=CARTESIAN_POINT('Ctrl Pts',(38.4091796349929,-12.0490754764082,
85.2022748316891));
#136468=CARTESIAN_POINT('Ctrl Pts',(38.6252906002273,-11.8750674671407,
85.3336948424002));
#136469=CARTESIAN_POINT('Ctrl Pts',(38.8388767635722,-11.6969091604009,
85.4626942795363));
#136470=CARTESIAN_POINT('Ctrl Pts',(39.1270776544536,-11.4565125826627,
85.6367587045141));
#136471=CARTESIAN_POINT('Ctrl Pts',(39.4106809652526,-11.2085529188707,
85.8064124729285));
#136472=CARTESIAN_POINT('Ctrl Pts',(39.6883537137141,-10.9532280783211,
85.9712624875313));
#136473=CARTESIAN_POINT('Ctrl Pts',(39.8592578972352,-10.7960787590286,
86.0727256570546));
#136474=CARTESIAN_POINT('Ctrl Pts',(40.0279154407973,-10.6361403353735,
86.1723690806801));
#136475=CARTESIAN_POINT('Ctrl Pts',(40.1940157028205,-10.4734687442745,
86.2701020081475));
#136476=CARTESIAN_POINT('Ctrl Pts',(40.4577034541812,-10.2152240820163,
86.4252551401406));
#136477=CARTESIAN_POINT('Ctrl Pts',(40.7149464230308,-9.95008648200096,
86.575594196585));
#136478=CARTESIAN_POINT('Ctrl Pts',(40.9645956540344,-9.67833462016586,
86.720735668409));
#136479=CARTESIAN_POINT('Ctrl Pts',(41.1277037924083,-9.50078574446779,
86.81556374048));
#136480=CARTESIAN_POINT('Ctrl Pts',(41.2875704671745,-9.32041449813221,
86.9081733664075));
#136481=CARTESIAN_POINT('Ctrl Pts',(41.4438758282522,-9.13731015598172,
86.9984609032528));
#136482=CARTESIAN_POINT('Ctrl Pts',(41.6201794994561,-8.93077873881247,
87.1003001754316));
#136483=CARTESIAN_POINT('Ctrl Pts',(41.7919523874227,-8.72077832621035,
87.199185857265));
#136484=CARTESIAN_POINT('Ctrl Pts',(41.9588973073281,-8.50711064257257,
87.2951279169551));
#136485=CARTESIAN_POINT('Ctrl Pts',(42.1240576117314,-8.29572703359078,
87.390044370792));
#136486=CARTESIAN_POINT('Ctrl Pts',(42.2844926409153,-8.0807538024963,87.482079936388));
#136487=CARTESIAN_POINT('Ctrl Pts',(42.4399061015799,-7.86198528229721,
87.571195846887));
#136488=CARTESIAN_POINT('Ctrl Pts',(42.4798420701361,-7.80576922027538,
87.5940956020583));
#136489=CARTESIAN_POINT('Ctrl Pts',(42.5194464116305,-7.74930249330274,
87.6168023108442));
#136490=CARTESIAN_POINT('Ctrl Pts',(42.5587140031694,-7.69258150586829,
87.6393147742221));
#136491=CARTESIAN_POINT('Ctrl Pts',(42.7077371246306,-7.47732158620972,
87.7247510699781));
#136492=CARTESIAN_POINT('Ctrl Pts',(42.8519095415155,-7.25839729428666,
87.8073860353505));
#136493=CARTESIAN_POINT('Ctrl Pts',(42.9907582766186,-7.03615374217394,
87.8869286456913));
#136494=CARTESIAN_POINT('Ctrl Pts',(43.1288681098162,-6.81509288851389,
87.9660479595122));
#136495=CARTESIAN_POINT('Ctrl Pts',(43.2617107345816,-6.59074824536283,
88.0421075322903));
#136496=CARTESIAN_POINT('Ctrl Pts',(43.3888275786924,-6.36349230427373,
88.1148600590489));
#136497=CARTESIAN_POINT('Ctrl Pts',(43.5156337971883,-6.13679169097714,
88.1874348060764));
#136498=CARTESIAN_POINT('Ctrl Pts',(43.6367421491539,-5.9071942407316,88.2567184512936));
#136499=CARTESIAN_POINT('Ctrl Pts',(43.751704839413,-5.67509888870081,88.3225075991413));
#136500=CARTESIAN_POINT('Ctrl Pts',(43.8663745942534,-5.44359493679249,
88.3881291102408));
#136501=CARTESIAN_POINT('Ctrl Pts',(43.974929938052,-5.20960607161433,88.4502737462847));
#136502=CARTESIAN_POINT('Ctrl Pts',(44.0769343622043,-4.97355330867935,
88.5087843081332));
#136503=CARTESIAN_POINT('Ctrl Pts',(44.1464226989862,-4.81274740221558,
88.5486433795491));
#136504=CARTESIAN_POINT('Ctrl Pts',(44.2128710981111,-4.65098421905349,
88.5868169065546));
#136505=CARTESIAN_POINT('Ctrl Pts',(44.2761437580013,-4.48840253804638,
88.6232676465585));
#136506=CARTESIAN_POINT('Ctrl Pts',(44.3762043421766,-4.23129278470233,
88.6809115380077));
#136507=CARTESIAN_POINT('Ctrl Pts',(44.4683241866109,-3.97213157424582,
88.7342549993688));
#136508=CARTESIAN_POINT('Ctrl Pts',(44.5522953596013,-3.71081561019567,
88.7832791000227));
#136509=CARTESIAN_POINT('Ctrl Pts',(44.6354995476277,-3.45188648210521,
88.8318554190541));
#136510=CARTESIAN_POINT('Ctrl Pts',(44.7107032491022,-3.19084136186465,
88.8761909579907));
#136511=CARTESIAN_POINT('Ctrl Pts',(44.7776953346401,-2.92757671872878,
88.9162171463247));
#136512=CARTESIAN_POINT('Ctrl Pts',(44.8441968372951,-2.66623996194838,
88.9559502229767));
#136513=CARTESIAN_POINT('Ctrl Pts',(44.9026065573288,-2.40271565605888,
88.9914368688759));
#136514=CARTESIAN_POINT('Ctrl Pts',(44.952709117092,-2.13690571923174,89.0225598028839));
#136515=CARTESIAN_POINT('Ctrl Pts',(45.0021618408937,-1.87454336785105,
89.0532790688589));
#136516=CARTESIAN_POINT('Ctrl Pts',(45.0435214918964,-1.60995389394597,
89.0797470578205));
#136517=CARTESIAN_POINT('Ctrl Pts',(45.0765723089672,-1.34305209460568,
89.1018019043616));
#136518=CARTESIAN_POINT('Ctrl Pts',(45.0907559739345,-1.22851193988243,
89.1112666795765));
#136519=CARTESIAN_POINT('Ctrl Pts',(45.1034093144603,-1.11354608029957,
89.1199180806114));
#136520=CARTESIAN_POINT('Ctrl Pts',(45.1145147830323,-0.998148588051396,
89.1277405079779));
#136521=CARTESIAN_POINT('',(91.9214475326691,-17.49925970194,62.90875755409));
#136522=CARTESIAN_POINT('',(27.1339039101791,-17.49925933285,74.332577093855));
#136523=CARTESIAN_POINT('Ctrl Pts',(91.9214475326691,-17.49925970194,62.90875755409));
#136524=CARTESIAN_POINT('Ctrl Pts',(92.3053259419944,-17.4691790615711,
65.0858401978147));
#136525=CARTESIAN_POINT('Ctrl Pts',(92.6881140569403,-17.0272695410026,
67.2567394748733));
#136526=CARTESIAN_POINT('Ctrl Pts',(93.400573325857,-15.3785962058232,71.2972967738997));
#136527=CARTESIAN_POINT('Ctrl Pts',(93.7300269848005,-14.1723356877064,
73.1657213202724));
#136528=CARTESIAN_POINT('Ctrl Pts',(94.2915430224096,-11.1564801229904,
76.3502370157891));
#136529=CARTESIAN_POINT('Ctrl Pts',(94.523433985036,-9.34780573756797,77.6653560162659));
#136530=CARTESIAN_POINT('Ctrl Pts',(94.8586248200716,-5.36963819152602,
79.5663177051065));
#136531=CARTESIAN_POINT('Ctrl Pts',(94.9618223675578,-3.20135946055536,
80.1515800799944));
#136532=CARTESIAN_POINT('Ctrl Pts',(94.9937559636691,-0.998148678735586,
80.332684502886));
#136533=CARTESIAN_POINT('Ctrl Pts',(94.5010653292691,0.271395986764614,
80.458308728496));
#136534=CARTESIAN_POINT('Ctrl Pts',(96.7480709862691,0.273309186559814,
80.062047303158));
#136535=CARTESIAN_POINT('Ctrl Pts',(101.075637772369,0.277199406335714,
79.298871480375));
#136536=CARTESIAN_POINT('Ctrl Pts',(106.443694708969,0.282511544310714,
78.353143604676));
#136537=CARTESIAN_POINT('Ctrl Pts',(110.084319043969,0.286361092968914,
77.709147420917));
#136538=CARTESIAN_POINT('Ctrl Pts',(111.775396016869,0.288211127596014,
77.413751883086));
#136539=CARTESIAN_POINT('Ctrl Pts',(112.489943251869,0.289007101963614,
77.28503103697));
#136540=CARTESIAN_POINT('Ctrl Pts',(112.751175106569,0.289282890086814,
77.242567650816));
#136541=CARTESIAN_POINT('Ctrl Pts',(113.006167906869,0.289653838855314,
77.183975946042));
#136542=CARTESIAN_POINT('Ctrl Pts',(113.328591681969,0.289983672853814,
77.111221001818));
#136543=CARTESIAN_POINT('Ctrl Pts',(114.612842666369,0.291414265154114,
76.810397989321));
#136544=CARTESIAN_POINT('Ctrl Pts',(116.776314331769,0.293771628264714,
76.212440481214));
#136545=CARTESIAN_POINT('Ctrl Pts',(120.750299755769,0.297915106635414,
74.787245381488));
#136546=CARTESIAN_POINT('Ctrl Pts',(124.528351856069,0.301393775126614,
72.86985978332));
#136547=CARTESIAN_POINT('Ctrl Pts',(127.965747787169,0.304277195172014,
70.412480183491));
#136548=CARTESIAN_POINT('Ctrl Pts',(130.333310528569,0.306311939856314,
68.306131684901));
#136549=CARTESIAN_POINT('Ctrl Pts',(132.447053549369,0.308402827782414,
65.942396934738));
#136550=CARTESIAN_POINT('Ctrl Pts',(134.292447465669,0.310751914886114,
63.363026900454));
#136551=CARTESIAN_POINT('Ctrl Pts',(135.902727419669,0.313393793906214,
60.63324875935));
#136552=CARTESIAN_POINT('Ctrl Pts',(136.924148492969,0.315444210411514,
58.59002833958));
#136553=CARTESIAN_POINT('Ctrl Pts',(137.445518530069,0.316570291628914,
57.48076137169));
#136554=CARTESIAN_POINT('Ctrl Pts',(137.517690719469,0.316725377312314,
57.32787172523));
#136555=CARTESIAN_POINT('Ctrl Pts',(94.5045898659691,-0.391944427092286,
80.474860038171));
#136556=CARTESIAN_POINT('Ctrl Pts',(96.7489959251691,-0.394461845619086,
80.079326957343));
#136557=CARTESIAN_POINT('Ctrl Pts',(101.071548853969,-0.399670518957686,
79.317433953307));
#136558=CARTESIAN_POINT('Ctrl Pts',(106.433267535669,-0.406985840309386,
78.373020946999));
#136559=CARTESIAN_POINT('Ctrl Pts',(110.069594033769,-0.412377925771286,
77.729798875547));
#136560=CARTESIAN_POINT('Ctrl Pts',(111.758480158269,-0.414989404441086,
77.434719128118));
#136561=CARTESIAN_POINT('Ctrl Pts',(112.472526008569,-0.416116539930086,
77.30617199322));
#136562=CARTESIAN_POINT('Ctrl Pts',(112.732216228169,-0.416506671346586,
77.263625252347));
#136563=CARTESIAN_POINT('Ctrl Pts',(112.993369304269,-0.417036659726086,
77.205783041926));
#136564=CARTESIAN_POINT('Ctrl Pts',(113.314294777669,-0.417503094204386,
77.132922464813));
#136565=CARTESIAN_POINT('Ctrl Pts',(114.600497973669,-0.419534148736686,
76.832518581053));
#136566=CARTESIAN_POINT('Ctrl Pts',(116.767017756869,-0.422893026034286,
76.234797701647));
#136567=CARTESIAN_POINT('Ctrl Pts',(120.749908756769,-0.428836605210586,
74.808474794112));
#136568=CARTESIAN_POINT('Ctrl Pts',(124.539140129969,-0.433883045948486,
72.8865424998045));
#136569=CARTESIAN_POINT('Ctrl Pts',(127.985466074869,-0.438134496061686,
70.422019976291));
#136570=CARTESIAN_POINT('Ctrl Pts',(130.357485033669,-0.441174799508086,
68.310135147826));
#136571=CARTESIAN_POINT('Ctrl Pts',(132.472991956769,-0.444336740905886,
65.941867636944));
#136572=CARTESIAN_POINT('Ctrl Pts',(134.317626905469,-0.447916848216786,
63.36094910574));
#136573=CARTESIAN_POINT('Ctrl Pts',(135.926029587169,-0.451965219963786,
60.63261837717));
#136574=CARTESIAN_POINT('Ctrl Pts',(136.945697916469,-0.455126418189086,
58.59256372079));
#136575=CARTESIAN_POINT('Ctrl Pts',(137.466114009069,-0.456868308193486,
57.48538563185));
#136576=CARTESIAN_POINT('Ctrl Pts',(137.538154739269,-0.457108150346786,
57.33278041094));
#136577=CARTESIAN_POINT('Ctrl Pts',(94.4917696614691,-1.62653903695399,
80.388080157788));
#136578=CARTESIAN_POINT('Ctrl Pts',(96.7251100426691,-1.64079859934899,
79.993118959704));
#136579=CARTESIAN_POINT('Ctrl Pts',(101.026458471769,-1.66878149008799,
79.2329765847));
#136580=CARTESIAN_POINT('Ctrl Pts',(106.361947261869,-1.70470855576399,
78.292262003841));
#136581=CARTESIAN_POINT('Ctrl Pts',(109.980616118269,-1.72972033570599,
77.652304985682));
#136582=CARTESIAN_POINT('Ctrl Pts',(111.660992166569,-1.74151397354599,
77.358869004343));
#136583=CARTESIAN_POINT('Ctrl Pts',(112.372181585169,-1.74654816345699,
77.231135964501));
#136584=CARTESIAN_POINT('Ctrl Pts',(112.628477516769,-1.74829694560499,
77.188621965177));
#136585=CARTESIAN_POINT('Ctrl Pts',(112.899581170269,-1.75058962364099,
77.132307511686));
#136586=CARTESIAN_POINT('Ctrl Pts',(113.217019764069,-1.75268289638599,
77.059556568771));
#136587=CARTESIAN_POINT('Ctrl Pts',(114.503042211069,-1.76167159692399,
76.761105443198));
#136588=CARTESIAN_POINT('Ctrl Pts',(116.668876258069,-1.77634825257999,
76.166361663691));
#136589=CARTESIAN_POINT('Ctrl Pts',(120.656347418569,-1.80169977690999,
74.744518803754));
#136590=CARTESIAN_POINT('Ctrl Pts',(124.454818894169,-1.82235294021599,
72.8236298001459));
#136591=CARTESIAN_POINT('Ctrl Pts',(127.907560783969,-1.83870632291999,
70.35800518595));
#136592=CARTESIAN_POINT('Ctrl Pts',(130.281095772069,-1.84979591424999,
68.246000480916));
#136593=CARTESIAN_POINT('Ctrl Pts',(132.394030826169,-1.86076654056799,
65.880166190254));
#136594=CARTESIAN_POINT('Ctrl Pts',(134.232064870669,-1.87277787282499,
63.307347157382));
#136595=CARTESIAN_POINT('Ctrl Pts',(135.831863833569,-1.88603586839099,
60.592619078));
#136596=CARTESIAN_POINT('Ctrl Pts',(136.844484227669,-1.89610879742999,
58.56638963221));
#136597=CARTESIAN_POINT('Ctrl Pts',(137.361072184969,-1.90157570216799,
57.46742495816));
#136598=CARTESIAN_POINT('Ctrl Pts',(137.432585302369,-1.90232921860299,
57.31594512813));
#136599=CARTESIAN_POINT('Ctrl Pts',(94.4309652584691,-3.97364311980699,
79.989330260271));
#136600=CARTESIAN_POINT('Ctrl Pts',(96.6215442512691,-4.01169264542499,
79.594451364535));
#136601=CARTESIAN_POINT('Ctrl Pts',(100.840786175369,-4.08465026300699,
78.836243627137));
#136602=CARTESIAN_POINT('Ctrl Pts',(106.074691078369,-4.17431672897299,
77.901971576044));
#136603=CARTESIAN_POINT('Ctrl Pts',(109.624729243069,-4.23483510476799,
77.268298018584));
#136604=CARTESIAN_POINT('Ctrl Pts',(111.272721866769,-4.26293361266799,
76.978069056252));
#136605=CARTESIAN_POINT('Ctrl Pts',(111.971449487369,-4.27484978147099,
76.851954396361));
#136606=CARTESIAN_POINT('Ctrl Pts',(112.219310861169,-4.27899269673599,
76.809543041334));
#136607=CARTESIAN_POINT('Ctrl Pts',(112.504070747669,-4.28434331979599,
76.75599781504));
#136608=CARTESIAN_POINT('Ctrl Pts',(112.812264044869,-4.28929908170699,
76.683735558641));
#136609=CARTESIAN_POINT('Ctrl Pts',(114.084082260069,-4.31044323461999,
76.389871123831));
#136610=CARTESIAN_POINT('Ctrl Pts',(116.225387968569,-4.34464562068499,
75.803524995651));
#136611=CARTESIAN_POINT('Ctrl Pts',(120.177534500969,-4.40262868470399,
74.399493491444));
#136612=CARTESIAN_POINT('Ctrl Pts',(123.950655853569,-4.44814620623399,
72.496847968071));
#136613=CARTESIAN_POINT('Ctrl Pts',(127.376994494769,-4.48208320683399,
70.051519337007));
#136614=CARTESIAN_POINT('Ctrl Pts',(129.727278560469,-4.50391800270399,
67.958092508844));
#136615=CARTESIAN_POINT('Ctrl Pts',(131.812162782869,-4.52449284930599,
65.616466683786));
#136616=CARTESIAN_POINT('Ctrl Pts',(133.616536214469,-4.54639756885499,
63.077404462912));
#136617=CARTESIAN_POINT('Ctrl Pts',(135.178848514569,-4.57011609389099,
60.40502284092));
#136618=CARTESIAN_POINT('Ctrl Pts',(136.162260621769,-4.58765299989899,
58.41602012162));
#136619=CARTESIAN_POINT('Ctrl Pts',(136.662957925869,-4.59700952188599,
57.33845516432));
#136620=CARTESIAN_POINT('Ctrl Pts',(136.732281158069,-4.59830067204899,
57.18991365398));
#136621=CARTESIAN_POINT('Ctrl Pts',(94.2946923201691,-6.70804124817899,
79.112010850242));
#136622=CARTESIAN_POINT('Ctrl Pts',(96.4018922775691,-6.77081804645399,
78.714410710852));
#136623=CARTESIAN_POINT('Ctrl Pts',(100.461102932469,-6.88895937391199,
77.954609507465));
#136624=CARTESIAN_POINT('Ctrl Pts',(105.497454600769,-7.02880980603999,
77.026576208225));
#136625=CARTESIAN_POINT('Ctrl Pts',(108.914058256569,-7.12055052930399,
76.400938200377));
#136626=CARTESIAN_POINT('Ctrl Pts',(110.499660565269,-7.16252676436099,
76.115032764168));
#136627=CARTESIAN_POINT('Ctrl Pts',(111.173165327269,-7.18021962643399,
75.991147187523));
#136628=CARTESIAN_POINT('Ctrl Pts',(111.408225108969,-7.18635419350799,
75.949001332739));
#136629=CARTESIAN_POINT('Ctrl Pts',(111.700693228269,-7.19430470928699,
75.898572630968));
#136630=CARTESIAN_POINT('Ctrl Pts',(111.994181897569,-7.20161151815999,
75.827463650124));
#136631=CARTESIAN_POINT('Ctrl Pts',(113.228310289369,-7.23275451518899,
75.540921750577));
#136632=CARTESIAN_POINT('Ctrl Pts',(115.305714966569,-7.28245852194699,
74.970021382884));
#136633=CARTESIAN_POINT('Ctrl Pts',(119.150002336769,-7.36432237457899,
73.6050086640061));
#136634=CARTESIAN_POINT('Ctrl Pts',(122.829165031769,-7.42430540347799,
71.754540381793));
#136635=CARTESIAN_POINT('Ctrl Pts',(126.167856447969,-7.46373591418299,
69.375045120244));
#136636=CARTESIAN_POINT('Ctrl Pts',(128.453230587369,-7.48631180618699,
67.33878584061));
#136637=CARTESIAN_POINT('Ctrl Pts',(130.472696968569,-7.50545576601199,
65.062710327142));
#136638=CARTESIAN_POINT('Ctrl Pts',(132.208627615269,-7.52508893813999,
62.59881514699));
#136639=CARTESIAN_POINT('Ctrl Pts',(133.698071052769,-7.54598850132699,
60.00898250641));
#136640=CARTESIAN_POINT('Ctrl Pts',(134.625480995269,-7.56064429820999,
58.0861089762));
#136641=CARTESIAN_POINT('Ctrl Pts',(135.095677359169,-7.56813519765099,
57.04564624104));
#136642=CARTESIAN_POINT('Ctrl Pts',(135.160797579369,-7.56917204693599,
56.90220721139));
#136643=CARTESIAN_POINT('Ctrl Pts',(94.0331412950691,-9.72819839798099,
77.461391565822));
#136644=CARTESIAN_POINT('Ctrl Pts',(96.0072255155691,-9.80312259694499,
77.061683166786));
#136645=CARTESIAN_POINT('Ctrl Pts',(99.8110683163691,-9.94225626317999,
76.303613526659));
#136646=CARTESIAN_POINT('Ctrl Pts',(104.532674733669,-10.10237277876,75.390554672224));
#136647=CARTESIAN_POINT('Ctrl Pts',(107.736774407169,-10.20506710756,74.780870036665));
#136648=CARTESIAN_POINT('Ctrl Pts',(109.223468801269,-10.25150545695,74.503201540156));
#136649=CARTESIAN_POINT('Ctrl Pts',(109.856025930669,-10.2709864892,74.383369290596));
#136650=CARTESIAN_POINT('Ctrl Pts',(110.073541803969,-10.27768940791,74.342100727107));
#136651=CARTESIAN_POINT('Ctrl Pts',(110.363390117669,-10.2866439161,74.29539812619));
#136652=CARTESIAN_POINT('Ctrl Pts',(110.636083672869,-10.29455426583,74.226981390702));
#136653=CARTESIAN_POINT('Ctrl Pts',(111.802366463169,-10.32851663231,73.9536960572392));
#136654=CARTESIAN_POINT('Ctrl Pts',(113.765631696269,-10.38176050765,73.4123027455414));
#136655=CARTESIAN_POINT('Ctrl Pts',(117.408936777569,-10.46588100582,72.1259277537728));
#136656=CARTESIAN_POINT('Ctrl Pts',(120.906767485869,-10.52044842901,70.388769104978));
#136657=CARTESIAN_POINT('Ctrl Pts',(124.083745239269,-10.54709619697,68.155531276342));
#136658=CARTESIAN_POINT('Ctrl Pts',(126.256740506469,-10.55719661026,66.243657042203));
#136659=CARTESIAN_POINT('Ctrl Pts',(128.171601052569,-10.56185077472,64.103935177044));
#136660=CARTESIAN_POINT('Ctrl Pts',(129.805209314969,-10.56596145084,61.7842775069));
#136661=CARTESIAN_POINT('Ctrl Pts',(131.187259144569,-10.57057132432,59.34216081812));
#136662=CARTESIAN_POINT('Ctrl Pts',(132.031680827369,-10.57263717675,57.53092481926));
#136663=CARTESIAN_POINT('Ctrl Pts',(132.456503474169,-10.57307296402,56.55202285407));
#136664=CARTESIAN_POINT('Ctrl Pts',(132.515372864869,-10.57313948151,56.4170597467));
#136665=CARTESIAN_POINT('Ctrl Pts',(93.6821615622691,-12.38223409115,75.27715826278));
#136666=CARTESIAN_POINT('Ctrl Pts',(95.5036033007691,-12.45177258484,74.883599759386));
#136667=CARTESIAN_POINT('Ctrl Pts',(99.0144766641691,-12.5802692937,74.142647600746));
#136668=CARTESIAN_POINT('Ctrl Pts',(103.374764814069,-12.72653556026,73.2619966330297));
#136669=CARTESIAN_POINT('Ctrl Pts',(106.334684719569,-12.81951619743,72.6790624888142));
#136670=CARTESIAN_POINT('Ctrl Pts',(107.707954093569,-12.86137745058,72.4142380691917));
#136671=CARTESIAN_POINT('Ctrl Pts',(108.292895990869,-12.87891347918,72.3004044412196));
#136672=CARTESIAN_POINT('Ctrl Pts',(108.492143327769,-12.88488451512,72.2607679061845));
#136673=CARTESIAN_POINT('Ctrl Pts',(108.768958348269,-12.89325414546,72.2179669987607));
#136674=CARTESIAN_POINT('Ctrl Pts',(109.019525278469,-12.90021960472,72.1537748655661));
#136675=CARTESIAN_POINT('Ctrl Pts',(110.102605128169,-12.93055535856,71.899044541544));
#136676=CARTESIAN_POINT('Ctrl Pts',(111.926525841569,-12.9773529257,71.399025133737));
#136677=CARTESIAN_POINT('Ctrl Pts',(115.320061967569,-13.04832119269,70.223065623371));
#136678=CARTESIAN_POINT('Ctrl Pts',(118.590293578969,-13.08784543436,68.64729371565));
#136679=CARTESIAN_POINT('Ctrl Pts',(121.570885042369,-13.09763726794,66.622368575163));
#136680=CARTESIAN_POINT('Ctrl Pts',(123.613187646469,-13.09445150359,64.885470371931));
#136681=CARTESIAN_POINT('Ctrl Pts',(125.413286174969,-13.08547415731,62.93331204737));
#136682=CARTESIAN_POINT('Ctrl Pts',(126.940103658769,-13.07597683247,60.80415135462));
#136683=CARTESIAN_POINT('Ctrl Pts',(128.210308454669,-13.06716939491,58.54935029097));
#136684=CARTESIAN_POINT('Ctrl Pts',(128.966948564269,-13.05967497397,56.8745529502));
#136685=CARTESIAN_POINT('Ctrl Pts',(129.343483874869,-13.05498314335,55.96997774857));
#136686=CARTESIAN_POINT('Ctrl Pts',(129.395703783069,-13.05434233444,55.84525666692));
#136687=CARTESIAN_POINT('Ctrl Pts',(93.2525522503691,-14.56494720251,72.6292784804675));
#136688=CARTESIAN_POINT('Ctrl Pts',(94.9099069943691,-14.61582723887,72.2566981640195));
#136689=CARTESIAN_POINT('Ctrl Pts',(98.1053359090691,-14.71078585591,71.558752332215));
#136690=CARTESIAN_POINT('Ctrl Pts',(102.075446269569,-14.8211612689,70.735832604723));
#136691=CARTESIAN_POINT('Ctrl Pts',(104.771012343469,-14.89256300333,70.193284594267));
#136692=CARTESIAN_POINT('Ctrl Pts',(106.021560527069,-14.92503651236,69.946645860606));
#136693=CARTESIAN_POINT('Ctrl Pts',(106.554407446069,-14.93870838161,69.840964041424));
#136694=CARTESIAN_POINT('Ctrl Pts',(106.735454910169,-14.9433096718,69.803778649846));
#136695=CARTESIAN_POINT('Ctrl Pts',(106.989614914069,-14.95016974445,69.765111926735));
#136696=CARTESIAN_POINT('Ctrl Pts',(107.217710549069,-14.95547553046,69.70673385112));
#136697=CARTESIAN_POINT('Ctrl Pts',(108.206162207169,-14.97909147355,69.476010576657));
#136698=CARTESIAN_POINT('Ctrl Pts',(109.872101016469,-15.01529544008,69.028920839883));
#136699=CARTESIAN_POINT('Ctrl Pts',(112.979053178569,-15.06915909587,67.992654212769));
#136700=CARTESIAN_POINT('Ctrl Pts',(115.986803650169,-15.09616756986,66.620973578397));
#136701=CARTESIAN_POINT('Ctrl Pts',(118.747134698169,-15.0978837308,64.858171703176));
#136702=CARTESIAN_POINT('Ctrl Pts',(120.648236384269,-15.09059048003,63.339220675778));
#136703=CARTESIAN_POINT('Ctrl Pts',(122.330929139869,-15.07917832172,61.61678074719));
#136704=CARTESIAN_POINT('Ctrl Pts',(123.753705899769,-15.06867596534,59.71388200454));
#136705=CARTESIAN_POINT('Ctrl Pts',(124.914541955869,-15.0603582609,57.67407819686));
#136706=CARTESIAN_POINT('Ctrl Pts',(125.583377083969,-15.05453785733,56.15087193636));
#136707=CARTESIAN_POINT('Ctrl Pts',(125.911215285669,-15.05112088214,55.32792490375));
#136708=CARTESIAN_POINT('Ctrl Pts',(125.956732969069,-15.05065234144,55.21446089957));
#136709=CARTESIAN_POINT('Ctrl Pts',(92.7615318988691,-16.20464967702,69.620536734241));
#136710=CARTESIAN_POINT('Ctrl Pts',(94.2482285258691,-16.23101253952,69.28827995804));
#136711=CARTESIAN_POINT('Ctrl Pts',(97.1146507180691,-16.28269288864,68.665777442556));
#136712=CARTESIAN_POINT('Ctrl Pts',(100.675648889369,-16.34879084479,67.928895074072));
#136713=CARTESIAN_POINT('Ctrl Pts',(103.092866435569,-16.39470354547,67.439878040069));
#136714=CARTESIAN_POINT('Ctrl Pts',(104.214137922869,-16.41636882877,67.215955123965));
#136715=CARTESIAN_POINT('Ctrl Pts',(104.691547007069,-16.42563822416,67.120132104085));
#136716=CARTESIAN_POINT('Ctrl Pts',(104.854874208569,-16.42872819769,67.086043494429));
#136717=CARTESIAN_POINT('Ctrl Pts',(105.077166774169,-16.43364643686,67.051562487782));
#136718=CARTESIAN_POINT('Ctrl Pts',(105.282954985669,-16.43718598195,67.000347697702));
#136719=CARTESIAN_POINT('Ctrl Pts',(106.167370916869,-16.4533828966,66.798047782311));
#136720=CARTESIAN_POINT('Ctrl Pts',(107.659994694069,-16.47861830463,66.413110357911));
#136721=CARTESIAN_POINT('Ctrl Pts',(110.449346482569,-16.51753051004,65.539506830122));
#136722=CARTESIAN_POINT('Ctrl Pts',(113.164900595469,-16.5391631641,64.405441646321));
#136723=CARTESIAN_POINT('Ctrl Pts',(115.685632177769,-16.54470350357,62.94652020938));
#136724=CARTESIAN_POINT('Ctrl Pts',(117.438110061369,-16.54407453157,61.67801064453));
#136725=CARTESIAN_POINT('Ctrl Pts',(119.003522973169,-16.54227130612,60.2155314398));
#136726=CARTESIAN_POINT('Ctrl Pts',(120.327462124369,-16.54346569086,58.56130716037));
#136727=CARTESIAN_POINT('Ctrl Pts',(121.383545670869,-16.54890359416,56.7494057631));
#136728=CARTESIAN_POINT('Ctrl Pts',(121.965858310969,-16.55497485232,55.38123587483));
#136729=CARTESIAN_POINT('Ctrl Pts',(122.245228728369,-16.55854218877,54.6406482838));
#136730=CARTESIAN_POINT('Ctrl Pts',(122.284080188769,-16.55903132032,54.53855286788));
#136731=CARTESIAN_POINT('Ctrl Pts',(92.3160179092691,-17.05845633753,66.898897397011));
#136732=CARTESIAN_POINT('Ctrl Pts',(93.6568424647691,-17.06736861268,66.616905163633));
#136733=CARTESIAN_POINT('Ctrl Pts',(96.2410780501691,-17.08777775176,66.084296328605));
#136734=CARTESIAN_POINT('Ctrl Pts',(99.4489334442691,-17.12067117079,65.440189739954));
#136735=CARTESIAN_POINT('Ctrl Pts',(101.624696234569,-17.14672195508,65.003809046661));
#136736=CARTESIAN_POINT('Ctrl Pts',(102.633720717169,-17.15974422671,64.800948051197));
#136737=CARTESIAN_POINT('Ctrl Pts',(103.062536021769,-17.16544430497,64.714017968606));
#136738=CARTESIAN_POINT('Ctrl Pts',(103.211636753469,-17.16734450314,64.682771588846));
#136739=CARTESIAN_POINT('Ctrl Pts',(103.399836092569,-17.17046418614,64.651541526049));
#136740=CARTESIAN_POINT('Ctrl Pts',(103.587344926369,-17.17265333749,64.60706354595));
#136741=CARTESIAN_POINT('Ctrl Pts',(104.377911634569,-17.18284853984,64.430665787025));
#136742=CARTESIAN_POINT('Ctrl Pts',(105.714438850969,-17.19933510361,64.102439610754));
#136743=CARTESIAN_POINT('Ctrl Pts',(108.215174535469,-17.22692014645,63.377387806248));
#136744=CARTESIAN_POINT('Ctrl Pts',(110.664078907169,-17.24638005472,62.4617307178));
#136745=CARTESIAN_POINT('Ctrl Pts',(112.970350336469,-17.25840009369,61.2819001994));
#136746=CARTESIAN_POINT('Ctrl Pts',(114.593636762369,-17.26584272015,60.24176555596));
#136747=CARTESIAN_POINT('Ctrl Pts',(116.062124964169,-17.27413543879,59.01301835956));
#136748=CARTESIAN_POINT('Ctrl Pts',(117.308594600169,-17.28622002581,57.57589495172));
#136749=CARTESIAN_POINT('Ctrl Pts',(118.281647748769,-17.30325651225,55.95516825802));
#136750=CARTESIAN_POINT('Ctrl Pts',(118.793119890869,-17.31878215848,54.71170764927));
#136751=CARTESIAN_POINT('Ctrl Pts',(119.032366787569,-17.32781681205,54.03627261275));
#136752=CARTESIAN_POINT('Ctrl Pts',(119.065703705269,-17.329056353,53.94318115434));
#136753=CARTESIAN_POINT('Ctrl Pts',(91.9339282292691,-17.4341963447,64.566704269957));
#136754=CARTESIAN_POINT('Ctrl Pts',(93.1521736193691,-17.43521999266,64.333201342115));
#136755=CARTESIAN_POINT('Ctrl Pts',(95.4987864019691,-17.43932140529,63.88538165894));
#136756=CARTESIAN_POINT('Ctrl Pts',(98.4081188271691,-17.4493281509,63.323852177671));
#136757=CARTESIAN_POINT('Ctrl Pts',(100.379158684869,-17.45848054895,62.93137508751));
#136758=CARTESIAN_POINT('Ctrl Pts',(101.292974475169,-17.46329630395,62.7451797869));
#136759=CARTESIAN_POINT('Ctrl Pts',(101.680293297669,-17.46544498611,62.66516022947));
#136760=CARTESIAN_POINT('Ctrl Pts',(101.818048062769,-17.46615169702,62.63611238732));
#136761=CARTESIAN_POINT('Ctrl Pts',(101.973349896169,-17.46740733325,62.60711074564));
#136762=CARTESIAN_POINT('Ctrl Pts',(102.146036955169,-17.46821299911,62.56830582003));
#136763=CARTESIAN_POINT('Ctrl Pts',(102.854852085869,-17.47209930056,62.41320992242));
#136764=CARTESIAN_POINT('Ctrl Pts',(104.055600475469,-17.47846541605,62.1325348399));
#136765=CARTESIAN_POINT('Ctrl Pts',(106.303934729469,-17.4893232793,61.53434726652));
#136766=CARTESIAN_POINT('Ctrl Pts',(108.519326841369,-17.49710260775,60.80864805725));
#136767=CARTESIAN_POINT('Ctrl Pts',(110.640815547969,-17.50195369933,59.87303699715));
#136768=CARTESIAN_POINT('Ctrl Pts',(112.155484622169,-17.50507153116,59.03228889222));
#136769=CARTESIAN_POINT('Ctrl Pts',(113.546077712669,-17.50880752966,58.00598025268));
#136770=CARTESIAN_POINT('Ctrl Pts',(114.733439685769,-17.51475423024,56.75316932502));
#136771=CARTESIAN_POINT('Ctrl Pts',(115.642433562169,-17.52398002372,55.29003282689));
#136772=CARTESIAN_POINT('Ctrl Pts',(116.097511363769,-17.53322921597,54.14607296181));
#136773=CARTESIAN_POINT('Ctrl Pts',(116.304500203969,-17.53882514575,53.52193271673));
#136774=CARTESIAN_POINT('Ctrl Pts',(116.333406458469,-17.53959102319,53.43593682679));
#136775=CARTESIAN_POINT('Ctrl Pts',(91.7332982817691,-17.50195372971,63.342887103518));
#136776=CARTESIAN_POINT('Ctrl Pts',(92.8878681996691,-17.50179983727,63.135222319627));
#136777=CARTESIAN_POINT('Ctrl Pts',(95.1109254058691,-17.50192227436,62.73200794642));
#136778=CARTESIAN_POINT('Ctrl Pts',(97.8647643030691,-17.50290970614,62.21234046008));
#136779=CARTESIAN_POINT('Ctrl Pts',(99.7290153100691,-17.50390275863,61.84108070543));
#136780=CARTESIAN_POINT('Ctrl Pts',(100.593172064669,-17.50443116352,61.66256696193));
#136781=CARTESIAN_POINT('Ctrl Pts',(100.958742773169,-17.50466844116,61.585695238));
#136782=CARTESIAN_POINT('Ctrl Pts',(101.090860291969,-17.50473393574,61.55763501945));
#136783=CARTESIAN_POINT('Ctrl Pts',(101.227465085569,-17.50493912834,61.52952220183));
#136784=CARTESIAN_POINT('Ctrl Pts',(101.392690067069,-17.50499758326,61.49357700272));
#136785=CARTESIAN_POINT('Ctrl Pts',(102.058053275069,-17.50539027309,61.3490168858));
#136786=CARTESIAN_POINT('Ctrl Pts',(103.186735740569,-17.50590773878,61.09253083144));
#136787=CARTESIAN_POINT('Ctrl Pts',(105.300699706669,-17.50624097075,60.56055645071));
#136788=CARTESIAN_POINT('Ctrl Pts',(107.391848487069,-17.50516827901,59.93616891045));
#136789=CARTESIAN_POINT('Ctrl Pts',(109.416461786669,-17.50251851211,59.13193578514));
#136790=CARTESIAN_POINT('Ctrl Pts',(110.875433230569,-17.49995815976,58.39852460632));
#136791=CARTESIAN_POINT('Ctrl Pts',(112.227768617769,-17.49718667402,57.48085879437));
#136792=CARTESIAN_POINT('Ctrl Pts',(113.387641718569,-17.4949747375,56.32592812353));
#136793=CARTESIAN_POINT('Ctrl Pts',(114.266500764269,-17.4943355846,54.94512241615));
#136794=CARTESIAN_POINT('Ctrl Pts',(114.694184237269,-17.49556162849,53.8521807202));
#136795=CARTESIAN_POINT('Ctrl Pts',(114.885356344869,-17.49666826989,53.25414284847));
#136796=CARTESIAN_POINT('Ctrl Pts',(114.912091474169,-17.49681664757,53.17175964758));
#136797=CARTESIAN_POINT('Ctrl Pts',(91.6256651679691,-17.50087323455,62.6865987037));
#136798=CARTESIAN_POINT('Ctrl Pts',(92.7462347895691,-17.50094842656,62.49253283427));
#136799=CARTESIAN_POINT('Ctrl Pts',(94.9032917810691,-17.50020019636,62.11262574012));
#136800=CARTESIAN_POINT('Ctrl Pts',(97.5740108379691,-17.49697626082,61.61434289845));
#136801=CARTESIAN_POINT('Ctrl Pts',(99.3811417969691,-17.49355583457,61.25357815157));
#136802=CARTESIAN_POINT('Ctrl Pts',(100.218740387169,-17.49165921143,61.07872701066));
#136803=CARTESIAN_POINT('Ctrl Pts',(100.572648403969,-17.49079874116,61.0033456655));
#136804=CARTESIAN_POINT('Ctrl Pts',(100.701837613969,-17.49049444435,60.97574535699));
#136805=CARTESIAN_POINT('Ctrl Pts',(100.827969879369,-17.49009249956,60.94800687329));
#136806=CARTESIAN_POINT('Ctrl Pts',(100.989287633669,-17.48971654682,60.91354003403));
#136807=CARTESIAN_POINT('Ctrl Pts',(101.631166208969,-17.48806898008,60.77435960452));
#136808=CARTESIAN_POINT('Ctrl Pts',(102.720935232469,-17.48508413693,60.5305219036));
#136809=CARTESIAN_POINT('Ctrl Pts',(104.762242093969,-17.47881650364,60.03389490008));
#136810=CARTESIAN_POINT('Ctrl Pts',(106.786272863569,-17.47167663677,59.46446863206));
#136811=CARTESIAN_POINT('Ctrl Pts',(108.759059563469,-17.46330836921,58.73198247683));
#136812=CARTESIAN_POINT('Ctrl Pts',(110.188668690969,-17.45621320481,58.05726949414));
#136813=CARTESIAN_POINT('Ctrl Pts',(111.521433399769,-17.44821259642,57.19897765626));
#136814=CARTESIAN_POINT('Ctrl Pts',(112.667811977369,-17.43960128686,56.09731370129));
#136815=CARTESIAN_POINT('Ctrl Pts',(113.531742275669,-17.43136124665,54.76100557254));
#136816=CARTESIAN_POINT('Ctrl Pts',(113.945520944869,-17.42641977624,53.69542143466));
#136817=CARTESIAN_POINT('Ctrl Pts',(114.128610933769,-17.42406662281,53.11133790473));
#136818=CARTESIAN_POINT('Ctrl Pts',(114.154237126469,-17.42373918761,53.03088647436));
#136819=CARTESIAN_POINT('',(114.384013244638,-17.4511073706868,53.3319431971496));
#136820=CARTESIAN_POINT('Ctrl Pts',(114.384012850693,-17.4511074291882,
53.3319430705208));
#136821=CARTESIAN_POINT('Ctrl Pts',(114.220888472494,-17.4519988842083,
53.8398358110967));
#136822=CARTESIAN_POINT('Ctrl Pts',(113.829481233474,-17.4543725662864,
54.8352104074227));
#136823=CARTESIAN_POINT('Ctrl Pts',(112.960679338991,-17.4596410224806,
56.1902373905027));
#136824=CARTESIAN_POINT('Ctrl Pts',(111.808327125295,-17.4657668375024,
57.3134151931793));
#136825=CARTESIAN_POINT('Ctrl Pts',(110.467194168512,-17.4717374796403,
58.1951861692835));
#136826=CARTESIAN_POINT('Ctrl Pts',(109.028402063985,-17.4770568190849,
58.8957505557642));
#136827=CARTESIAN_POINT('Ctrl Pts',(107.031015069744,-17.4832149765507,
59.6550380994632));
#136828=CARTESIAN_POINT('Ctrl Pts',(104.468739305416,-17.4891377436966,
60.3958819176082));
#136829=CARTESIAN_POINT('Ctrl Pts',(101.35178149711,-17.4940454558258,61.1211273764285));
#136830=CARTESIAN_POINT('Ctrl Pts',(98.2162369710537,-17.4971942144887,
61.7585815172283));
#136831=CARTESIAN_POINT('Ctrl Pts',(95.071694526759,-17.4989202182121,62.3491703657761));
#136832=CARTESIAN_POINT('Ctrl Pts',(92.9717518845374,-17.4992596243613,
62.7235663753691));
#136833=CARTESIAN_POINT('Ctrl Pts',(91.9214475326691,-17.49925970194,62.90875755409));
#136834=CARTESIAN_POINT('',(137.305407436204,-9.29834912769915E-12,57.7874348564604));
#136835=CARTESIAN_POINT('Ctrl Pts',(137.305407436201,-9.29561982943028E-12,
57.7874348564612));
#136836=CARTESIAN_POINT('Ctrl Pts',(137.305407495695,-1.34472964465863,
57.7874347379193));
#136837=CARTESIAN_POINT('Ctrl Pts',(137.075117022675,-2.66554501472644,
57.7426704534051));
#136838=CARTESIAN_POINT('Ctrl Pts',(136.207322767474,-5.20088375491933,
57.5739872507397));
#136839=CARTESIAN_POINT('Ctrl Pts',(135.580897995914,-6.39181951377924,
57.4522218871268));
#136840=CARTESIAN_POINT('Ctrl Pts',(133.336328816589,-9.6643571443166,57.0159193422835));
#136841=CARTESIAN_POINT('Ctrl Pts',(131.322433877513,-11.5113308194662,
56.624455689254));
#136842=CARTESIAN_POINT('Ctrl Pts',(127.008689974315,-14.4665207294624,
55.7859443455056));
#136843=CARTESIAN_POINT('Ctrl Pts',(124.584096632227,-15.6695033005887,
55.314648673862));
#136844=CARTESIAN_POINT('Ctrl Pts',(118.850738143645,-17.5212377256219,
54.2001909378701));
#136845=CARTESIAN_POINT('Ctrl Pts',(116.347111372697,-17.6025946223322,
53.7135327557499));
#136846=CARTESIAN_POINT('Ctrl Pts',(114.384013344373,-17.4511059084411,
53.3319432645659));
#136847=CARTESIAN_POINT('Ctrl Pts',(95.0009770511696,1.41900380334903E-14,
80.3736373255327));
#136848=CARTESIAN_POINT('Ctrl Pts',(97.0803868675694,1.61737654382892E-12,
80.0069812709578));
#136849=CARTESIAN_POINT('Ctrl Pts',(99.1597966839195,1.75226639535239E-10,
79.6403252163851));
#136850=CARTESIAN_POINT('Ctrl Pts',(101.239237748174,2.37870695363185E-10,
79.2738274979082));
#136851=CARTESIAN_POINT('Ctrl Pts',(103.318678812429,3.00514713466124E-10,
78.9073297794313));
#136852=CARTESIAN_POINT('Ctrl Pts',(105.398151124589,2.52193602934045E-10,
78.5409903970502));
#136853=CARTESIAN_POINT('Ctrl Pts',(107.477432973366,2.43303190095023E-10,
78.1736859184611));
#136854=CARTESIAN_POINT('Ctrl Pts',(108.517073897755,2.38858067986138E-10,
77.9900336791664));
#136855=CARTESIAN_POINT('Ctrl Pts',(109.556667206299,2.44270592801756E-10,
77.8061401658197));
#136856=CARTESIAN_POINT('Ctrl Pts',(110.596551246173,2.46179396312662E-10,
77.6237198161581));
#136857=CARTESIAN_POINT('Ctrl Pts',(111.116493266109,2.4713382950139E-10,
77.5325096413276));
#136858=CARTESIAN_POINT('Ctrl Pts',(111.636507968877,2.47212066916387E-10,
77.4416677574185));
#136859=CARTESIAN_POINT('Ctrl Pts',(112.156094597342,2.47661648133946E-10,
77.3486567797055));
#136860=CARTESIAN_POINT('Ctrl Pts',(112.285991254459,2.4777404800645E-10,
77.3254040352771));
#136861=CARTESIAN_POINT('Ctrl Pts',(112.415861156932,2.47909381658537E-10,
77.3020157224859));
#136862=CARTESIAN_POINT('Ctrl Pts',(112.54601291089,2.48033642236134E-10,
77.2800555834686));
#136863=CARTESIAN_POINT('Ctrl Pts',(112.611088787869,2.48095820884867E-10,
77.2690755139599));
#136864=CARTESIAN_POINT('Ctrl Pts',(112.67623512772,2.48153283270535E-10,
77.2584524878953));
#136865=CARTESIAN_POINT('Ctrl Pts',(112.740991784632,2.48221304621765E-10,
77.2458558104383));
#136866=CARTESIAN_POINT('Ctrl Pts',(112.805748441545,2.4828932697814E-10,
77.2332591329813));
#136867=CARTESIAN_POINT('Ctrl Pts',(112.870115415519,2.48376480234793E-10,
77.2186888041303));
#136868=CARTESIAN_POINT('Ctrl Pts',(112.934479385948,2.48448171757953E-10,
77.2041226313424));
#136869=CARTESIAN_POINT('Ctrl Pts',(113.063207326806,2.48591558390765E-10,
77.1749902857666));
#136870=CARTESIAN_POINT('Ctrl Pts',(113.191923253486,2.4870328328373E-10,
77.1458745644437));
#136871=CARTESIAN_POINT('Ctrl Pts',(113.320527988354,2.48823461834746E-10,
77.1162858196239));
#136872=CARTESIAN_POINT('Ctrl Pts',(113.44913272322,2.48943552136221E-10,
77.0866970748045));
#136873=CARTESIAN_POINT('Ctrl Pts',(113.577626266275,2.49064188873619E-10,
77.0566353064879));
#136874=CARTESIAN_POINT('Ctrl Pts',(113.705989992107,2.49189731349464E-10,
77.0260066290821));
#136875=CARTESIAN_POINT('Ctrl Pts',(114.732899798777,2.50194018712686E-10,
76.7809772098333));
#136876=CARTESIAN_POINT('Ctrl Pts',(115.751501303018,2.51147685891077E-10,
76.4996656091634));
#136877=CARTESIAN_POINT('Ctrl Pts',(116.75796074466,2.52056604754802E-10,
76.1808266875528));
#136878=CARTESIAN_POINT('Ctrl Pts',(117.7644201863,2.52965460192699E-10,
75.8619877659428));
#136879=CARTESIAN_POINT('Ctrl Pts',(118.758737566024,2.53960974327935E-10,
75.5056215220171));
#136880=CARTESIAN_POINT('Ctrl Pts',(119.736805721593,2.54712154146297E-10,
75.1081300375498));
#136881=CARTESIAN_POINT('Ctrl Pts',(121.692942032732,2.56214528961853E-10,
74.3131470686145));
#136882=CARTESIAN_POINT('Ctrl Pts',(123.58408144016,2.56831564688639E-10,
73.3536631749867));
#136883=CARTESIAN_POINT('Ctrl Pts',(125.361375841541,2.59188642770525E-10,
72.2138533985717));
#136884=CARTESIAN_POINT('Ctrl Pts',(126.250023042232,2.60367181450065E-10,
71.6439485103637));
#136885=CARTESIAN_POINT('Ctrl Pts',(127.110208988119,2.6077903821463E-10,
71.0289621207599));
#136886=CARTESIAN_POINT('Ctrl Pts',(127.935165389,2.61042402971423E-10,
70.3700832646172));
#136887=CARTESIAN_POINT('Ctrl Pts',(128.760121789881,2.6130574685733E-10,
69.7112044084745));
#136888=CARTESIAN_POINT('Ctrl Pts',(129.549848682753,2.59856007144552E-10,
69.0084331956421));
#136889=CARTESIAN_POINT('Ctrl Pts',(130.2970945887,2.6277636316907E-10,
68.262834677594));
#136890=CARTESIAN_POINT('Ctrl Pts',(131.044340494645,2.65696716392728E-10,
67.5172361595471));
#136891=CARTESIAN_POINT('Ctrl Pts',(131.749105184572,2.65887614767794E-10,
66.728809956919));
#136892=CARTESIAN_POINT('Ctrl Pts',(132.408971868912,2.64547238282287E-10,
65.9046542110124));
#136893=CARTESIAN_POINT('Ctrl Pts',(133.068838553253,2.6320681047808E-10,
65.0804984651044));
#136894=CARTESIAN_POINT('Ctrl Pts',(133.683808222283,2.53115900951374E-10,
64.2206142302005));
#136895=CARTESIAN_POINT('Ctrl Pts',(134.259531000955,2.6650029405495E-10,
63.3358425354513));
#136896=CARTESIAN_POINT('Ctrl Pts',(134.835253779626,2.79884673425092E-10,
62.4510708407035));
#136897=CARTESIAN_POINT('Ctrl Pts',(135.371726233848,3.59572997301272E-10,
61.5414091247388));
#136898=CARTESIAN_POINT('Ctrl Pts',(135.876171533849,2.68671404568543E-10,
60.6140360578227));
#136899=CARTESIAN_POINT('Ctrl Pts',(136.380640904218,1.77765306356043E-10,
59.6866187399019));
#136900=CARTESIAN_POINT('Ctrl Pts',(136.853086992978,-1.4415087307438E-11,
58.7414924351101));
#136901=CARTESIAN_POINT('Ctrl Pts',(137.305407436203,-9.30262811227323E-12,
57.7874348564578));
#136902=CARTESIAN_POINT('Ctrl Pts',(94.5010623932691,-0.271390781348986,
80.458309380968));
#136903=CARTESIAN_POINT('Ctrl Pts',(96.7480690176691,-0.273303947139986,
80.062047787126));
#136904=CARTESIAN_POINT('Ctrl Pts',(101.075636752369,-0.277194096347286,
79.29887180002));
#136905=CARTESIAN_POINT('Ctrl Pts',(106.443694627169,-0.282506136256786,
78.353143760582));
#136906=CARTESIAN_POINT('Ctrl Pts',(110.084318928469,-0.286355612428486,
77.709147582895));
#136907=CARTESIAN_POINT('Ctrl Pts',(111.775395884169,-0.288205612061686,
77.413752047541));
#136908=CARTESIAN_POINT('Ctrl Pts',(112.489943115269,-0.289001571345486,
77.285031202788));
#136909=CARTESIAN_POINT('Ctrl Pts',(112.751174957869,-0.289277354245586,
77.24256781598));
#136910=CARTESIAN_POINT('Ctrl Pts',(113.006167806469,-0.289648295947586,
77.183976117084));
#136911=CARTESIAN_POINT('Ctrl Pts',(113.328591569869,-0.289978123700586,
77.111221172032));
#136912=CARTESIAN_POINT('Ctrl Pts',(114.612842569469,-0.291408688849486,
76.810398162822));
#136913=CARTESIAN_POINT('Ctrl Pts',(116.776314258869,-0.293766007124886,
76.212440656571));
#136914=CARTESIAN_POINT('Ctrl Pts',(120.750299752669,-0.297909406378086,
74.787245547999));
#136915=CARTESIAN_POINT('Ctrl Pts',(124.528351940669,-0.301388008002886,
72.8698599141694));
#136916=CARTESIAN_POINT('Ctrl Pts',(127.965747941769,-0.304271372086086,
70.412480258316));
#136917=CARTESIAN_POINT('Ctrl Pts',(130.333310718269,-0.306306076964386,
68.306131716301));
#136918=CARTESIAN_POINT('Ctrl Pts',(132.447053752769,-0.308396923690086,
65.942396930586));
#136919=CARTESIAN_POINT('Ctrl Pts',(134.292447663169,-0.310745964288386,
63.363026884157));
#136920=CARTESIAN_POINT('Ctrl Pts',(135.902727602469,-0.313387790833686,
60.63324875441));
#136921=CARTESIAN_POINT('Ctrl Pts',(136.924194019969,-0.315438257512286,
58.58993762679));
#136922=CARTESIAN_POINT('Ctrl Pts',(137.445604913769,-0.316564411408386,
57.48057796111));
#136923=CARTESIAN_POINT('Ctrl Pts',(137.517820678669,-0.316719586679086,
57.32759679869));
#136924=CARTESIAN_POINT('Ctrl Pts',(94.5045868697691,0.391947887872814,
80.474860316371));
#136925=CARTESIAN_POINT('Ctrl Pts',(96.7489938846691,0.394465340288714,
80.079327063307));
#136926=CARTESIAN_POINT('Ctrl Pts',(101.071547740669,0.399674078560414,
79.317433890141));
#136927=CARTESIAN_POINT('Ctrl Pts',(106.433267335469,0.406989481539114,
78.3730207204));
#136928=CARTESIAN_POINT('Ctrl Pts',(110.069593784169,0.412381622051114,
77.729798658109));
#136929=CARTESIAN_POINT('Ctrl Pts',(111.758479884769,0.414993126484714,
77.434718915293));
#136930=CARTESIAN_POINT('Ctrl Pts',(112.472525726969,0.416120272936414,
77.306171782679));
#136931=CARTESIAN_POINT('Ctrl Pts',(112.732215937069,0.416510408165114,
77.263625041898));
#136932=CARTESIAN_POINT('Ctrl Pts',(112.993369041169,0.417040401490514,
77.205782835764));
#136933=CARTESIAN_POINT('Ctrl Pts',(113.314294504769,0.417506840533414,
77.132922258958));
#136934=CARTESIAN_POINT('Ctrl Pts',(114.600497700269,0.419537914587914,
76.832518380677));
#136935=CARTESIAN_POINT('Ctrl Pts',(116.767017481569,0.422896823641614,
76.234797509625));
#136936=CARTESIAN_POINT('Ctrl Pts',(120.749908494269,0.428840457273914,
74.808474614661));
#136937=CARTESIAN_POINT('Ctrl Pts',(124.539139893469,0.433886941802114,
72.88654232328));
#136938=CARTESIAN_POINT('Ctrl Pts',(127.985465856269,0.438138425871614,
70.422019796674));
#136939=CARTESIAN_POINT('Ctrl Pts',(130.357484819269,0.441178751903214,
68.310134967873));
#136940=CARTESIAN_POINT('Ctrl Pts',(132.472991735269,0.444340715211014,
65.941867463818));
#136941=CARTESIAN_POINT('Ctrl Pts',(134.317626665369,0.447920846178814,
63.360948955341));
#136942=CARTESIAN_POINT('Ctrl Pts',(135.926029322969,0.451969243766714,
60.63261826494));
#136943=CARTESIAN_POINT('Ctrl Pts',(136.945742912569,0.455130601764614,
58.59247305525));
#136944=CARTESIAN_POINT('Ctrl Pts',(137.466199778869,0.456872649911514,
57.48520248006));
#136945=CARTESIAN_POINT('Ctrl Pts',(137.538284005369,0.457112636783714,
57.33250591017));
#136946=CARTESIAN_POINT('Ctrl Pts',(94.4917666714691,1.62654072710201,80.388080388391));
#136947=CARTESIAN_POINT('Ctrl Pts',(96.7251080033691,1.64080031285201,79.993119016481));
#136948=CARTESIAN_POINT('Ctrl Pts',(101.026457354669,1.66878324250101,79.232976468964));
#136949=CARTESIAN_POINT('Ctrl Pts',(106.361947052669,1.70471035391701,78.292261719665));
#136950=CARTESIAN_POINT('Ctrl Pts',(109.980615859169,1.72972215971201,77.652304706081));
#136951=CARTESIAN_POINT('Ctrl Pts',(111.660991883869,1.74151580942401,77.358868727078));
#136952=CARTESIAN_POINT('Ctrl Pts',(112.372181293369,1.74655000434601,77.231135688414));
#136953=CARTESIAN_POINT('Ctrl Pts',(112.628477218869,1.74829878823701,77.188621689165));
#136954=CARTESIAN_POINT('Ctrl Pts',(112.899580882369,1.75059146850001,77.13230723769));
#136955=CARTESIAN_POINT('Ctrl Pts',(113.217019469369,1.75268474332801,77.059556295131));
#136956=CARTESIAN_POINT('Ctrl Pts',(114.503041906069,1.76167345271701,76.761105172898));
#136957=CARTESIAN_POINT('Ctrl Pts',(116.668875935169,1.77635012259001,76.166361399505));
#136958=CARTESIAN_POINT('Ctrl Pts',(120.656347069869,1.80170167067901,74.744518552537));
#136959=CARTESIAN_POINT('Ctrl Pts',(124.454818527069,1.82235485208901,72.8236295622119));
#136960=CARTESIAN_POINT('Ctrl Pts',(127.907560397669,1.83870824759601,70.358004962794));
#136961=CARTESIAN_POINT('Ctrl Pts',(130.281095368769,1.84979784675001,68.246000271287));
#136962=CARTESIAN_POINT('Ctrl Pts',(132.394030402469,1.86076848006101,65.880165998251));
#136963=CARTESIAN_POINT('Ctrl Pts',(134.232064422569,1.87277981952201,63.307346989957));
#136964=CARTESIAN_POINT('Ctrl Pts',(135.831863358169,1.88603782270401,60.59261894141));
#136965=CARTESIAN_POINT('Ctrl Pts',(136.844528698069,1.89611120448401,58.56629954457));
#136966=CARTESIAN_POINT('Ctrl Pts',(137.361157107969,1.90157856884701,57.46724312117));
#136967=CARTESIAN_POINT('Ctrl Pts',(137.432713405869,1.90233253674001,57.3156726068));
#136968=CARTESIAN_POINT('Ctrl Pts',(94.4309623691691,3.97364306962101,79.989330781101));
#136969=CARTESIAN_POINT('Ctrl Pts',(96.6215423249691,4.01169261211601,79.594451710704));
#136970=CARTESIAN_POINT('Ctrl Pts',(100.840785212069,4.08465024650501,78.836243799081));
#136971=CARTESIAN_POINT('Ctrl Pts',(106.074691078369,4.17431672897301,77.901971576044));
#136972=CARTESIAN_POINT('Ctrl Pts',(109.624729243069,4.23483510476801,77.268298018584));
#136973=CARTESIAN_POINT('Ctrl Pts',(111.272721866769,4.26293361266801,76.978069056252));
#136974=CARTESIAN_POINT('Ctrl Pts',(111.971449487369,4.27484978147101,76.851954396361));
#136975=CARTESIAN_POINT('Ctrl Pts',(112.219310861169,4.27899269673601,76.809543041334));
#136976=CARTESIAN_POINT('Ctrl Pts',(112.504070747669,4.28434331979601,76.75599781504));
#136977=CARTESIAN_POINT('Ctrl Pts',(112.812264044869,4.28929908170701,76.683735558641));
#136978=CARTESIAN_POINT('Ctrl Pts',(114.084082260069,4.31044323462001,76.389871123831));
#136979=CARTESIAN_POINT('Ctrl Pts',(116.225387968569,4.34464562068501,75.803524995651));
#136980=CARTESIAN_POINT('Ctrl Pts',(120.177534500969,4.40262868470401,74.399493491444));
#136981=CARTESIAN_POINT('Ctrl Pts',(123.950655853569,4.44814620623401,72.496847968071));
#136982=CARTESIAN_POINT('Ctrl Pts',(127.376994494769,4.48208320683401,70.051519337007));
#136983=CARTESIAN_POINT('Ctrl Pts',(129.727278560469,4.50391800270401,67.958092508844));
#136984=CARTESIAN_POINT('Ctrl Pts',(131.812162782869,4.52449284930601,65.616466683786));
#136985=CARTESIAN_POINT('Ctrl Pts',(133.616536214469,4.54639756885501,63.077404462912));
#136986=CARTESIAN_POINT('Ctrl Pts',(135.178848514569,4.57011609389101,60.40502284092));
#136987=CARTESIAN_POINT('Ctrl Pts',(136.162304291869,4.58765377865501,58.41593179657));
#136988=CARTESIAN_POINT('Ctrl Pts',(136.663040729269,4.59701106923501,57.33827696026));
#136989=CARTESIAN_POINT('Ctrl Pts',(136.732405833069,4.59830299412501,57.18964650883));
#136990=CARTESIAN_POINT('Ctrl Pts',(94.2946895408691,6.70804116537901,79.112011374661));
#136991=CARTESIAN_POINT('Ctrl Pts',(96.4018904242691,6.77081799251501,78.714411057748));
#136992=CARTESIAN_POINT('Ctrl Pts',(100.461102005569,6.88895934817401,77.954609678261));
#136993=CARTESIAN_POINT('Ctrl Pts',(105.497454600769,7.02880980604001,77.026576208225));
#136994=CARTESIAN_POINT('Ctrl Pts',(108.914058256569,7.12055052930401,76.400938200377));
#136995=CARTESIAN_POINT('Ctrl Pts',(110.499660565269,7.16252676436101,76.115032764168));
#136996=CARTESIAN_POINT('Ctrl Pts',(111.173165327269,7.18021962643401,75.991147187523));
#136997=CARTESIAN_POINT('Ctrl Pts',(111.408225108969,7.18635419350801,75.949001332739));
#136998=CARTESIAN_POINT('Ctrl Pts',(111.700693228269,7.19430470928701,75.898572630968));
#136999=CARTESIAN_POINT('Ctrl Pts',(111.994181897569,7.20161151816001,75.827463650124));
#137000=CARTESIAN_POINT('Ctrl Pts',(113.228310289369,7.23275451518901,75.540921750577));
#137001=CARTESIAN_POINT('Ctrl Pts',(115.305714966569,7.28245852194701,74.970021382884));
#137002=CARTESIAN_POINT('Ctrl Pts',(119.150002336769,7.36432237457901,73.6050086640061));
#137003=CARTESIAN_POINT('Ctrl Pts',(122.829165031769,7.42430540347801,71.754540381793));
#137004=CARTESIAN_POINT('Ctrl Pts',(126.167856447969,7.46373591418301,69.375045120244));
#137005=CARTESIAN_POINT('Ctrl Pts',(128.453230587369,7.48631180618701,67.33878584061));
#137006=CARTESIAN_POINT('Ctrl Pts',(130.472696968569,7.50545576601201,65.062710327142));
#137007=CARTESIAN_POINT('Ctrl Pts',(132.208627615269,7.52508893814001,62.59881514699));
#137008=CARTESIAN_POINT('Ctrl Pts',(133.698071052769,7.54598850132701,60.00898250641));
#137009=CARTESIAN_POINT('Ctrl Pts',(134.625522178469,7.56064494902501,58.08602358773));
#137010=CARTESIAN_POINT('Ctrl Pts',(135.095755118369,7.56813643646701,57.04547417283));
#137011=CARTESIAN_POINT('Ctrl Pts',(135.160914695369,7.56917391166701,56.9019492428));
#137012=CARTESIAN_POINT('Ctrl Pts',(94.0331386912691,9.72819829915901,77.461392093022));
#137013=CARTESIAN_POINT('Ctrl Pts',(96.0072237788691,9.80312253342201,77.061683512892));
#137014=CARTESIAN_POINT('Ctrl Pts',(99.8110674473691,9.94225623371201,76.303613694699));
#137015=CARTESIAN_POINT('Ctrl Pts',(104.532674733669,10.10237277876,75.390554672224));
#137016=CARTESIAN_POINT('Ctrl Pts',(107.736774407169,10.20506710756,74.780870036665));
#137017=CARTESIAN_POINT('Ctrl Pts',(109.223468801269,10.25150545695,74.503201540156));
#137018=CARTESIAN_POINT('Ctrl Pts',(109.856025930669,10.2709864892,74.383369290596));
#137019=CARTESIAN_POINT('Ctrl Pts',(110.073541803969,10.27768940791,74.342100727107));
#137020=CARTESIAN_POINT('Ctrl Pts',(110.363390117669,10.2866439161,74.29539812619));
#137021=CARTESIAN_POINT('Ctrl Pts',(110.636083672869,10.29455426583,74.226981390702));
#137022=CARTESIAN_POINT('Ctrl Pts',(111.802366463169,10.32851663231,73.9536960572392));
#137023=CARTESIAN_POINT('Ctrl Pts',(113.765631696269,10.38176050765,73.4123027455414));
#137024=CARTESIAN_POINT('Ctrl Pts',(117.408936777569,10.46588100582,72.1259277537728));
#137025=CARTESIAN_POINT('Ctrl Pts',(120.906767485869,10.52044842901,70.388769104978));
#137026=CARTESIAN_POINT('Ctrl Pts',(124.083745239269,10.54709619697,68.155531276342));
#137027=CARTESIAN_POINT('Ctrl Pts',(126.256740506469,10.55719661026,66.243657042203));
#137028=CARTESIAN_POINT('Ctrl Pts',(128.171601052569,10.56185077472,64.103935177044));
#137029=CARTESIAN_POINT('Ctrl Pts',(129.805209314969,10.56596145084,61.7842775069));
#137030=CARTESIAN_POINT('Ctrl Pts',(131.187259144569,10.57057132432,59.34216081812));
#137031=CARTESIAN_POINT('Ctrl Pts',(132.031718325369,10.57263726849,57.53084438825));
#137032=CARTESIAN_POINT('Ctrl Pts',(132.456573729769,10.57307303608,56.55186096657));
#137033=CARTESIAN_POINT('Ctrl Pts',(132.515478739069,10.57313960115,56.41681702166));
#137034=CARTESIAN_POINT('Ctrl Pts',(93.6821591598691,12.38223399943,75.277158781868));
#137035=CARTESIAN_POINT('Ctrl Pts',(95.5036016978691,12.45177252617,74.883600097677));
#137036=CARTESIAN_POINT('Ctrl Pts',(99.0144758616691,12.58026926678,74.142647762821));
#137037=CARTESIAN_POINT('Ctrl Pts',(103.374764814069,12.72653556026,73.2619966330297));
#137038=CARTESIAN_POINT('Ctrl Pts',(106.334684719569,12.81951619743,72.6790624888142));
#137039=CARTESIAN_POINT('Ctrl Pts',(107.707954093569,12.86137745058,72.4142380691917));
#137040=CARTESIAN_POINT('Ctrl Pts',(108.292895990869,12.87891347918,72.3004044412196));
#137041=CARTESIAN_POINT('Ctrl Pts',(108.492143327769,12.88488451512,72.2607679061845));
#137042=CARTESIAN_POINT('Ctrl Pts',(108.768958348269,12.89325414546,72.2179669987607));
#137043=CARTESIAN_POINT('Ctrl Pts',(109.019525278469,12.90021960472,72.1537748655661));
#137044=CARTESIAN_POINT('Ctrl Pts',(110.102605128169,12.93055535856,71.899044541544));
#137045=CARTESIAN_POINT('Ctrl Pts',(111.926525841569,12.9773529257,71.399025133737));
#137046=CARTESIAN_POINT('Ctrl Pts',(115.320061967569,13.04832119269,70.223065623371));
#137047=CARTESIAN_POINT('Ctrl Pts',(118.590293578969,13.08784543436,68.64729371565));
#137048=CARTESIAN_POINT('Ctrl Pts',(121.570885042369,13.09763726794,66.622368575163));
#137049=CARTESIAN_POINT('Ctrl Pts',(123.613187646469,13.09445150359,64.885470371931));
#137050=CARTESIAN_POINT('Ctrl Pts',(125.413286174969,13.08547415731,62.93331204737));
#137051=CARTESIAN_POINT('Ctrl Pts',(126.940103658769,13.07597683247,60.80415135462));
#137052=CARTESIAN_POINT('Ctrl Pts',(128.210308454669,13.06716939491,58.54935029097));
#137053=CARTESIAN_POINT('Ctrl Pts',(128.966982164169,13.05967464117,56.87447857797));
#137054=CARTESIAN_POINT('Ctrl Pts',(129.343546144769,13.05498236743,55.96982815299));
#137055=CARTESIAN_POINT('Ctrl Pts',(129.395797698569,13.05434118198,55.8450323617));
#137056=CARTESIAN_POINT('Ctrl Pts',(93.2525500644691,14.5649471354,72.6292789718861));
#137057=CARTESIAN_POINT('Ctrl Pts',(94.9099055354691,14.61582719551,72.2566984826754));
#137058=CARTESIAN_POINT('Ctrl Pts',(98.1053351783691,14.7107858356,71.558752483666));
#137059=CARTESIAN_POINT('Ctrl Pts',(102.075446269569,14.8211612689,70.735832604723));
#137060=CARTESIAN_POINT('Ctrl Pts',(104.771012343469,14.89256300333,70.193284594267));
#137061=CARTESIAN_POINT('Ctrl Pts',(106.021560527069,14.92503651236,69.946645860606));
#137062=CARTESIAN_POINT('Ctrl Pts',(106.554407446069,14.93870838161,69.840964041424));
#137063=CARTESIAN_POINT('Ctrl Pts',(106.735454910169,14.9433096718,69.803778649846));
#137064=CARTESIAN_POINT('Ctrl Pts',(106.989614914069,14.95016974445,69.765111926735));
#137065=CARTESIAN_POINT('Ctrl Pts',(107.217710549069,14.95547553046,69.70673385112));
#137066=CARTESIAN_POINT('Ctrl Pts',(108.206162207169,14.97909147355,69.476010576657));
#137067=CARTESIAN_POINT('Ctrl Pts',(109.872101016469,15.01529544008,69.028920839883));
#137068=CARTESIAN_POINT('Ctrl Pts',(112.979053178569,15.06915909587,67.992654212769));
#137069=CARTESIAN_POINT('Ctrl Pts',(115.986803650169,15.09616756986,66.620973578397));
#137070=CARTESIAN_POINT('Ctrl Pts',(118.747134698169,15.0978837308,64.858171703176));
#137071=CARTESIAN_POINT('Ctrl Pts',(120.648236384269,15.09059048003,63.339220675778));
#137072=CARTESIAN_POINT('Ctrl Pts',(122.330929139869,15.07917832172,61.61678074719));
#137073=CARTESIAN_POINT('Ctrl Pts',(123.753705899769,15.06867596534,59.71388200454));
#137074=CARTESIAN_POINT('Ctrl Pts',(124.914541955869,15.0603582609,57.67407819686));
#137075=CARTESIAN_POINT('Ctrl Pts',(125.583406784669,15.05453759886,56.1508042958));
#137076=CARTESIAN_POINT('Ctrl Pts',(125.911269502169,15.05112031705,55.32778880756));
#137077=CARTESIAN_POINT('Ctrl Pts',(125.956814830969,15.05065149879,55.2142568397));
#137078=CARTESIAN_POINT('Ctrl Pts',(92.7615299379691,16.20464964225,69.620537172474));
#137079=CARTESIAN_POINT('Ctrl Pts',(94.2482272171691,16.23101251592,69.288280242251));
#137080=CARTESIAN_POINT('Ctrl Pts',(97.1146500626691,16.28269287648,68.665777578172));
#137081=CARTESIAN_POINT('Ctrl Pts',(100.675648889369,16.34879084479,67.928895074072));
#137082=CARTESIAN_POINT('Ctrl Pts',(103.092866435569,16.39470354547,67.439878040069));
#137083=CARTESIAN_POINT('Ctrl Pts',(104.214137922869,16.41636882877,67.215955123965));
#137084=CARTESIAN_POINT('Ctrl Pts',(104.691547007069,16.42563822416,67.120132104085));
#137085=CARTESIAN_POINT('Ctrl Pts',(104.854874208569,16.42872819769,67.086043494429));
#137086=CARTESIAN_POINT('Ctrl Pts',(105.077166774169,16.43364643686,67.051562487782));
#137087=CARTESIAN_POINT('Ctrl Pts',(105.282954985669,16.43718598195,67.000347697702));
#137088=CARTESIAN_POINT('Ctrl Pts',(106.167370916869,16.4533828966,66.798047782311));
#137089=CARTESIAN_POINT('Ctrl Pts',(107.659994694069,16.47861830463,66.413110357911));
#137090=CARTESIAN_POINT('Ctrl Pts',(110.449346482569,16.51753051004,65.539506830122));
#137091=CARTESIAN_POINT('Ctrl Pts',(113.164900595469,16.5391631641,64.405441646321));
#137092=CARTESIAN_POINT('Ctrl Pts',(115.685632177769,16.54470350357,62.94652020938));
#137093=CARTESIAN_POINT('Ctrl Pts',(117.438110061369,16.54407453157,61.67801064453));
#137094=CARTESIAN_POINT('Ctrl Pts',(119.003522973169,16.54227130612,60.2155314398));
#137095=CARTESIAN_POINT('Ctrl Pts',(120.327462124369,16.54346569086,58.56130716037));
#137096=CARTESIAN_POINT('Ctrl Pts',(121.383545670869,16.54890359416,56.7494057631));
#137097=CARTESIAN_POINT('Ctrl Pts',(121.965884169569,16.55497512192,55.38117511892));
#137098=CARTESIAN_POINT('Ctrl Pts',(122.245274929469,16.55854277873,54.64052580792));
#137099=CARTESIAN_POINT('Ctrl Pts',(122.284150061769,16.5590322,54.53836925391));
#137100=CARTESIAN_POINT('Ctrl Pts',(92.3160161407691,17.05845632578,66.898897768948));
#137101=CARTESIAN_POINT('Ctrl Pts',(93.6568412849691,17.06736860337,66.616905406802));
#137102=CARTESIAN_POINT('Ctrl Pts',(96.2410774598691,17.08777774571,66.084296447147));
#137103=CARTESIAN_POINT('Ctrl Pts',(99.4489334442691,17.12067117079,65.440189739954));
#137104=CARTESIAN_POINT('Ctrl Pts',(101.624696234569,17.14672195508,65.003809046661));
#137105=CARTESIAN_POINT('Ctrl Pts',(102.633720717169,17.15974422671,64.800948051197));
#137106=CARTESIAN_POINT('Ctrl Pts',(103.062536021769,17.16544430497,64.714017968606));
#137107=CARTESIAN_POINT('Ctrl Pts',(103.211636753469,17.16734450314,64.682771588846));
#137108=CARTESIAN_POINT('Ctrl Pts',(103.399836092569,17.17046418614,64.651541526049));
#137109=CARTESIAN_POINT('Ctrl Pts',(103.587344926369,17.17265333749,64.60706354595));
#137110=CARTESIAN_POINT('Ctrl Pts',(104.377911634569,17.18284853984,64.430665787025));
#137111=CARTESIAN_POINT('Ctrl Pts',(105.714438850969,17.19933510361,64.102439610754));
#137112=CARTESIAN_POINT('Ctrl Pts',(108.215174535469,17.22692014645,63.377387806248));
#137113=CARTESIAN_POINT('Ctrl Pts',(110.664078907169,17.24638005472,62.4617307178));
#137114=CARTESIAN_POINT('Ctrl Pts',(112.970350336469,17.25840009369,61.2819001994));
#137115=CARTESIAN_POINT('Ctrl Pts',(114.593636762369,17.26584272015,60.24176555596));
#137116=CARTESIAN_POINT('Ctrl Pts',(116.062124964169,17.27413543879,59.01301835956));
#137117=CARTESIAN_POINT('Ctrl Pts',(117.308594600169,17.28622002581,57.57589495172));
#137118=CARTESIAN_POINT('Ctrl Pts',(118.281647748769,17.30325651225,55.95516825802));
#137119=CARTESIAN_POINT('Ctrl Pts',(118.793142603669,17.31878284792,54.71165243129));
#137120=CARTESIAN_POINT('Ctrl Pts',(119.032406353169,17.32781830618,54.03616091157));
#137121=CARTESIAN_POINT('Ctrl Pts',(119.065763660669,17.32905858225,53.9430137336));
#137122=CARTESIAN_POINT('Ctrl Pts',(91.9339550857691,17.43416835301,64.566878312127));
#137123=CARTESIAN_POINT('Ctrl Pts',(93.1522101427691,17.4351925881,64.333371668602));
#137124=CARTESIAN_POINT('Ctrl Pts',(95.4988411627691,17.43929521558,63.885545568036));
#137125=CARTESIAN_POINT('Ctrl Pts',(98.4081963615691,17.44930366796,63.32400983193));
#137126=CARTESIAN_POINT('Ctrl Pts',(100.379251469769,17.45845732483,62.93152947122));
#137127=CARTESIAN_POINT('Ctrl Pts',(101.293074352569,17.46327369117,62.74533292911));
#137128=CARTESIAN_POINT('Ctrl Pts',(101.680396266369,17.46542263789,62.66531285689));
#137129=CARTESIAN_POINT('Ctrl Pts',(101.818151876569,17.46612943771,62.63626485097));
#137130=CARTESIAN_POINT('Ctrl Pts',(101.973456160669,17.46738521279,62.60726304328));
#137131=CARTESIAN_POINT('Ctrl Pts',(102.146144323769,17.46819098171,62.56845769507));
#137132=CARTESIAN_POINT('Ctrl Pts',(102.854965544569,17.47207775314,62.41336021059));
#137133=CARTESIAN_POINT('Ctrl Pts',(104.055724048769,17.47844462254,62.13268158581));
#137134=CARTESIAN_POINT('Ctrl Pts',(106.304077105169,17.48930373187,61.53448456181));
#137135=CARTESIAN_POINT('Ctrl Pts',(108.519486612369,17.49708393044,60.80877120184));
#137136=CARTESIAN_POINT('Ctrl Pts',(110.640989084169,17.50193555607,59.87314194888));
#137137=CARTESIAN_POINT('Ctrl Pts',(112.155666249669,17.50505371007,59.03237899087));
#137138=CARTESIAN_POINT('Ctrl Pts',(113.546265142869,17.50879004802,58.00605527088));
#137139=CARTESIAN_POINT('Ctrl Pts',(114.733631519169,17.51473720583,56.75323061307));
#137140=CARTESIAN_POINT('Ctrl Pts',(115.642630167569,17.52396358116,55.29008237542));
#137141=CARTESIAN_POINT('Ctrl Pts',(116.097732378869,17.53321365172,54.14606429834));
#137142=CARTESIAN_POINT('Ctrl Pts',(116.304737644669,17.5388103524,53.52186781304));
#137143=CARTESIAN_POINT('Ctrl Pts',(116.333661985569,17.53957671709,53.4358199528));
#137144=CARTESIAN_POINT('Ctrl Pts',(91.7333543710691,17.50193427032,63.343238804133));
#137145=CARTESIAN_POINT('Ctrl Pts',(92.8879430816691,17.50178071582,63.135566510854));
#137146=CARTESIAN_POINT('Ctrl Pts',(95.1110362757691,17.50190429546,62.7323392405));
#137147=CARTESIAN_POINT('Ctrl Pts',(97.8649203306691,17.50289431744,62.21265963756));
#137148=CARTESIAN_POINT('Ctrl Pts',(99.7292020028691,17.50388971296,61.84139379018));
#137149=CARTESIAN_POINT('Ctrl Pts',(100.593373017269,17.50441934898,61.66287784085));
#137150=CARTESIAN_POINT('Ctrl Pts',(100.958949970969,17.50465717549,61.58600521299));
#137151=CARTESIAN_POINT('Ctrl Pts',(101.091069108469,17.5047228542,61.55794471084));
#137152=CARTESIAN_POINT('Ctrl Pts',(101.227679271069,17.50492834844,61.52983163798));
#137153=CARTESIAN_POINT('Ctrl Pts',(101.392906395369,17.50498701793,61.49388561767));
#137154=CARTESIAN_POINT('Ctrl Pts',(102.058282080869,17.50538071097,61.34932247533));
#137155=CARTESIAN_POINT('Ctrl Pts',(103.186985240469,17.50589985612,61.09282947493));
#137156=CARTESIAN_POINT('Ctrl Pts',(105.300987791769,17.50623611027,60.56083608065));
#137157=CARTESIAN_POINT('Ctrl Pts',(107.392172249469,17.50516596038,59.93641944816));
#137158=CARTESIAN_POINT('Ctrl Pts',(109.416813367469,17.50251834733,59.13214859692));
#137159=CARTESIAN_POINT('Ctrl Pts',(110.875800805269,17.49995962543,58.39870659569));
#137160=CARTESIAN_POINT('Ctrl Pts',(112.228147178369,17.49719000828,57.48100958633));
#137161=CARTESIAN_POINT('Ctrl Pts',(113.388028172869,17.49498041446,56.32605080859));
#137162=CARTESIAN_POINT('Ctrl Pts',(114.266895872169,17.49434409422,54.9452214594));
#137163=CARTESIAN_POINT('Ctrl Pts',(114.694606203969,17.49557249646,53.85221657865));
#137164=CARTESIAN_POINT('Ctrl Pts',(114.885795476969,17.49668055561,53.25412084327));
#137165=CARTESIAN_POINT('Ctrl Pts',(114.912547697369,17.49682919454,53.1716873435));
#137166=CARTESIAN_POINT('Ctrl Pts',(91.6257501351691,17.5008740942,62.68712605541));
#137167=CARTESIAN_POINT('Ctrl Pts',(92.7463475571691,17.50094910285,62.49304918148));
#137168=CARTESIAN_POINT('Ctrl Pts',(94.9034580498691,17.50020157244,62.11312328629));
#137169=CARTESIAN_POINT('Ctrl Pts',(97.5742443556691,17.49698101879,61.61482317768));
#137170=CARTESIAN_POINT('Ctrl Pts',(99.3814211904691,17.4935641372,61.25405000158));
#137171=CARTESIAN_POINT('Ctrl Pts',(100.219041110869,17.49166946169,61.07919591897));
#137172=CARTESIAN_POINT('Ctrl Pts',(100.572958494569,17.49080987306,61.00381337677));
#137173=CARTESIAN_POINT('Ctrl Pts',(100.702150056369,17.49050587323,60.97621269887));
#137174=CARTESIAN_POINT('Ctrl Pts',(100.828290732669,17.49010441605,60.9484739145));
#137175=CARTESIAN_POINT('Ctrl Pts',(100.989611625069,17.4897288122,60.91400588789));
#137176=CARTESIAN_POINT('Ctrl Pts',(101.631509061969,17.48808288405,60.77482113764));
#137177=CARTESIAN_POINT('Ctrl Pts',(102.721309338569,17.48510085369,60.53097327818));
#137178=CARTESIAN_POINT('Ctrl Pts',(104.762674554169,17.47883852165,60.0343178855));
#137179=CARTESIAN_POINT('Ctrl Pts',(106.786759229369,17.47170352733,59.46484747566));
#137180=CARTESIAN_POINT('Ctrl Pts',(108.759587553569,17.4633398522,58.73230369738));
#137181=CARTESIAN_POINT('Ctrl Pts',(110.189220263469,17.4562483296,58.05754357168));
#137182=CARTESIAN_POINT('Ctrl Pts',(111.522000690569,17.44825192058,57.19920404805));
#137183=CARTESIAN_POINT('Ctrl Pts',(112.668390106469,17.43964575023,56.09749731227));
#137184=CARTESIAN_POINT('Ctrl Pts',(113.532332395069,17.43141181414,54.76115344552));
#137185=CARTESIAN_POINT('Ctrl Pts',(113.946140607069,17.42647507754,53.69550001546));
#137186=CARTESIAN_POINT('Ctrl Pts',(114.129248991669,17.42412453312,53.11135600252));
#137187=CARTESIAN_POINT('Ctrl Pts',(114.154891885069,17.42379728054,53.03085492537));
#137188=CARTESIAN_POINT('',(114.384105937906,17.4511140883104,53.3319645993539));
#137189=CARTESIAN_POINT('Ctrl Pts',(114.384106000532,17.4511131438857,53.3319646520768));
#137190=CARTESIAN_POINT('Ctrl Pts',(116.347347433182,17.6026023327896,53.7135820476909));
#137191=CARTESIAN_POINT('Ctrl Pts',(118.851091663061,17.5211983263482,54.200263045881));
#137192=CARTESIAN_POINT('Ctrl Pts',(124.584741871326,15.6692377812452,55.3147771283751));
#137193=CARTESIAN_POINT('Ctrl Pts',(127.009446406625,14.4661198773037,55.7860941811001));
#137194=CARTESIAN_POINT('Ctrl Pts',(131.323096521923,11.5107569636489,56.6245867223739));
#137195=CARTESIAN_POINT('Ctrl Pts',(133.336771014781,9.66385111634966,57.0160071673924));
#137196=CARTESIAN_POINT('Ctrl Pts',(135.581104357009,6.39144737287628,57.4522632366775));
#137197=CARTESIAN_POINT('Ctrl Pts',(136.207456627177,5.20057247572336,57.5740142769302));
#137198=CARTESIAN_POINT('Ctrl Pts',(137.075144789367,2.66538159270485,57.7426763665124));
#137199=CARTESIAN_POINT('Ctrl Pts',(137.305407382829,1.3446443670393,57.7874349761847));
#137200=CARTESIAN_POINT('Ctrl Pts',(137.305407436207,-9.29645249669875E-12,
57.7874348564623));
#137201=CARTESIAN_POINT('Ctrl Pts',(114.384105646626,17.4511131146219,53.3319645061305));
#137202=CARTESIAN_POINT('Ctrl Pts',(114.371589774419,17.4511819034599,53.3703524107852));
#137203=CARTESIAN_POINT('Ctrl Pts',(114.357320213996,17.4512575190875,53.4134407155842));
#137204=CARTESIAN_POINT('Ctrl Pts',(114.341143340837,17.45134138163,53.4611755752132));
#137205=CARTESIAN_POINT('Ctrl Pts',(114.325809473745,17.4514208739441,53.5064228851237));
#137206=CARTESIAN_POINT('Ctrl Pts',(114.308762036051,17.4515077781385,53.5558453044607));
#137207=CARTESIAN_POINT('Ctrl Pts',(114.289827745447,17.4516035983617,53.6093757289036));
#137208=CARTESIAN_POINT('Ctrl Pts',(114.285716357714,17.4516244047441,53.6209993135934));
#137209=CARTESIAN_POINT('Ctrl Pts',(114.281515834125,17.4516456326073,53.6328164989034));
#137210=CARTESIAN_POINT('Ctrl Pts',(114.277224105706,17.4516672991808,53.6448264394875));
#137211=CARTESIAN_POINT('Ctrl Pts',(114.258540385167,17.4517616229974,53.6971108227662));
#137212=CARTESIAN_POINT('Ctrl Pts',(114.238131584234,17.4518642423489,53.7530503429297));
#137213=CARTESIAN_POINT('Ctrl Pts',(114.215800873513,17.4519767262012,53.8125605070917));
#137214=CARTESIAN_POINT('Ctrl Pts',(114.211283543716,17.4519994808132,53.8245989523145));
#137215=CARTESIAN_POINT('Ctrl Pts',(114.206687418172,17.4520226398948,53.8367834311851));
#137216=CARTESIAN_POINT('Ctrl Pts',(114.202010636999,17.452046217648,53.849113109929));
#137217=CARTESIAN_POINT('Ctrl Pts',(114.186407098532,17.4521248820898,53.8902496543791));
#137218=CARTESIAN_POINT('Ctrl Pts',(114.169654599657,17.4522094553237,53.9336529273905));
#137219=CARTESIAN_POINT('Ctrl Pts',(114.152096554589,17.4522984297842,53.9781912391146));
#137220=CARTESIAN_POINT('Ctrl Pts',(114.138377180561,17.4523679519832,54.0129922522513));
#137221=CARTESIAN_POINT('Ctrl Pts',(114.12416655042,17.4524401550677,54.0484863843268));
#137222=CARTESIAN_POINT('Ctrl Pts',(114.109649605634,17.4525141353038,54.0841415616067));
#137223=CARTESIAN_POINT('Ctrl Pts',(114.067083963232,17.4527310553459,54.1886873560771));
#137224=CARTESIAN_POINT('Ctrl Pts',(114.026117877619,17.4529477408174,54.2844675121801));
#137225=CARTESIAN_POINT('Ctrl Pts',(113.987376113768,17.4531583366583,54.371707940627));
#137226=CARTESIAN_POINT('Ctrl Pts',(113.947900494458,17.4533729216544,54.4606008974683));
#137227=CARTESIAN_POINT('Ctrl Pts',(113.91073816483,17.4535811767367,54.5406304621533));
#137228=CARTESIAN_POINT('Ctrl Pts',(113.876535028894,17.4537778853062,54.6120707171014));
#137229=CARTESIAN_POINT('Ctrl Pts',(113.866007534157,17.4538384308783,54.6340595461213));
#137230=CARTESIAN_POINT('Ctrl Pts',(113.855760052481,17.4538978898741,54.6552347304349));
#137231=CARTESIAN_POINT('Ctrl Pts',(113.845810293893,17.4539561299282,54.6756042812164));
#137232=CARTESIAN_POINT('Ctrl Pts',(113.833476788596,17.4540283230382,54.7008539352894));
#137233=CARTESIAN_POINT('Ctrl Pts',(113.821600821234,17.4540986425022,54.7248657155462));
#137234=CARTESIAN_POINT('Ctrl Pts',(113.810214497995,17.454166856576,54.7476545088773));
#137235=CARTESIAN_POINT('Ctrl Pts',(113.801855403344,17.4542169348925,54.764384552145));
#137236=CARTESIAN_POINT('Ctrl Pts',(113.793335740895,17.4542684884077,54.7812963178437));
#137237=CARTESIAN_POINT('Ctrl Pts',(113.785601101182,17.4543156932661,54.7965429892002));
#137238=CARTESIAN_POINT('Ctrl Pts',(113.783009019611,17.4543315128579,54.8016525505132));
#137239=CARTESIAN_POINT('Ctrl Pts',(113.780505517019,17.4543468415418,54.8065753082894));
#137240=CARTESIAN_POINT('Ctrl Pts',(113.778127313472,17.4543614533325,54.8112423088825));
#137241=CARTESIAN_POINT('Ctrl Pts',(113.777935556687,17.4543626314949,54.8116186135216));
#137242=CARTESIAN_POINT('Ctrl Pts',(113.77774461476,17.4543638049951,54.8119932555158));
#137243=CARTESIAN_POINT('Ctrl Pts',(113.777554507073,17.4543649737138,54.8123661987807));
#137244=CARTESIAN_POINT('Ctrl Pts',(113.760997352661,17.4544667615813,54.844847153788));
#137245=CARTESIAN_POINT('Ctrl Pts',(113.742187397006,17.4545848856968,54.8812806335243));
#137246=CARTESIAN_POINT('Ctrl Pts',(113.720936292063,17.4547203115329,54.9215653752202));
#137247=CARTESIAN_POINT('Ctrl Pts',(113.699938910622,17.4548541204781,54.9613691449496));
#137248=CARTESIAN_POINT('Ctrl Pts',(113.676558220886,17.4550048241377,55.0049330567655));
#137249=CARTESIAN_POINT('Ctrl Pts',(113.650573073102,17.455173446629,55.0521281496504));
#137250=CARTESIAN_POINT('Ctrl Pts',(113.625154667817,17.4553383914221,55.0982939058894));
#137251=CARTESIAN_POINT('Ctrl Pts',(113.597244014884,17.4555204858377,55.1479344381161));
#137252=CARTESIAN_POINT('Ctrl Pts',(113.566598142364,17.4557207219892,55.2008949254065));
#137253=CARTESIAN_POINT('Ctrl Pts',(113.5501664346,17.455828084634,55.2292912861119));
#137254=CARTESIAN_POINT('Ctrl Pts',(113.532947775678,17.4559406630743,55.258641488683));
#137255=CARTESIAN_POINT('Ctrl Pts',(113.514900538785,17.4560586081969,55.2889170572746));
#137256=CARTESIAN_POINT('Ctrl Pts',(113.494743755401,17.4561903399573,55.3227315454167));
#137257=CARTESIAN_POINT('Ctrl Pts',(113.473553439861,17.4563287667806,55.3577004992569));
#137258=CARTESIAN_POINT('Ctrl Pts',(113.451267303754,17.4564740880957,55.3937788901019));
#137259=CARTESIAN_POINT('Ctrl Pts',(113.440124235701,17.4565467487532,55.4118180855244));
#137260=CARTESIAN_POINT('Ctrl Pts',(113.428707212121,17.4566211401046,55.4301346399296));
#137261=CARTESIAN_POINT('Ctrl Pts',(113.41700792369,17.4566972750741,55.4487222204307));
#137262=CARTESIAN_POINT('Ctrl Pts',(113.40763168092,17.4567582924566,55.463618995419));
#137263=CARTESIAN_POINT('Ctrl Pts',(113.397662857599,17.4568231073498,55.479335314175));
#137264=CARTESIAN_POINT('Ctrl Pts',(113.388085467126,17.4568853036446,55.4943156320338));
#137265=CARTESIAN_POINT('Ctrl Pts',(113.385712585373,17.4569007133173,55.498027136019));
#137266=CARTESIAN_POINT('Ctrl Pts',(113.383363945006,17.4569159613581,55.5016935984257));
#137267=CARTESIAN_POINT('Ctrl Pts',(113.381054924302,17.456930948487,55.5052916296858));
#137268=CARTESIAN_POINT('Ctrl Pts',(113.334198945699,17.457235075942,55.5783049532101));
#137269=CARTESIAN_POINT('Ctrl Pts',(113.288749634299,17.4575253378865,55.6463050848044));
#137270=CARTESIAN_POINT('Ctrl Pts',(113.24511861625,17.4577997228023,55.7095128221076));
#137271=CARTESIAN_POINT('Ctrl Pts',(113.201487627675,17.4580741075328,55.7727205167098));
#137272=CARTESIAN_POINT('Ctrl Pts',(113.159674881288,17.4583326225352,55.8311365761762));
#137273=CARTESIAN_POINT('Ctrl Pts',(113.12004017196,17.4585737507042,55.8849822108195));
#137274=CARTESIAN_POINT('Ctrl Pts',(113.081271647035,17.4588096092129,55.9376510928206));
#137275=CARTESIAN_POINT('Ctrl Pts',(113.044586785714,17.4590288397472,55.9859477052673));
#137276=CARTESIAN_POINT('Ctrl Pts',(113.010274955306,17.4592303863066,56.0300697377023));
#137277=CARTESIAN_POINT('Ctrl Pts',(112.992863499198,17.4593326606251,56.0524593573176));
#137278=CARTESIAN_POINT('Ctrl Pts',(112.976062363385,17.4594303864457,56.0737738059339));
#137279=CARTESIAN_POINT('Ctrl Pts',(112.959904764964,17.4595234526901,56.0940372932867));
#137280=CARTESIAN_POINT('Ctrl Pts',(112.951825965753,17.4595699858123,56.1041690369631));
#137281=CARTESIAN_POINT('Ctrl Pts',(112.943908050731,17.4596153574017,56.114038040181));
#137282=CARTESIAN_POINT('Ctrl Pts',(112.936154828112,17.4596595514036,56.1236471771745));
#137283=CARTESIAN_POINT('Ctrl Pts',(112.932278216802,17.4596816484046,56.1284517456712));
#137284=CARTESIAN_POINT('Ctrl Pts',(112.928442778582,17.459703451225,56.1331913476027));
#137285=CARTESIAN_POINT('Ctrl Pts',(112.924648979998,17.4597249584811,56.1378663366714));
#137286=CARTESIAN_POINT('Ctrl Pts',(112.922752080705,17.4597357121092,56.1402038312057));
#137287=CARTESIAN_POINT('Ctrl Pts',(112.920865591321,17.4597463918598,56.1425251725237));
#137288=CARTESIAN_POINT('Ctrl Pts',(112.918989568944,17.4597569975594,56.1448304042441));
#137289=CARTESIAN_POINT('Ctrl Pts',(112.917113546568,17.4597676032591,56.1471356359646));
#137290=CARTESIAN_POINT('Ctrl Pts',(112.916020739977,17.459773778669,56.1484778736131));
#137291=CARTESIAN_POINT('Ctrl Pts',(112.913392959572,17.4597885923618,56.1516978140407));
#137292=CARTESIAN_POINT('Ctrl Pts',(112.913390689335,17.4597886051599,56.1517005958662));
#137293=CARTESIAN_POINT('Ctrl Pts',(112.913388419096,17.459788617958,56.15170337769));
#137294=CARTESIAN_POINT('Ctrl Pts',(112.913386148855,17.4597886307561,56.151706159512));
#137295=CARTESIAN_POINT('Ctrl Pts',(112.745210152272,17.460736694941,56.3577793044755));
#137296=CARTESIAN_POINT('Ctrl Pts',(112.565150469579,17.461708681726,56.5542011869675));
#137297=CARTESIAN_POINT('Ctrl Pts',(112.375139748759,17.46268621933,56.7407485428551));
#137298=CARTESIAN_POINT('Ctrl Pts',(112.280133105854,17.4631749947299,56.8340234799187));
#137299=CARTESIAN_POINT('Ctrl Pts',(112.182638636455,17.4636651526536,56.9248297189269));
#137300=CARTESIAN_POINT('Ctrl Pts',(112.082898074606,17.4641543518052,57.0131390517288));
#137301=CARTESIAN_POINT('Ctrl Pts',(112.033027793681,17.464398951381,57.0572937181298));
#137302=CARTESIAN_POINT('Ctrl Pts',(111.982595989662,17.4646433108442,57.1008241579985));
#137303=CARTESIAN_POINT('Ctrl Pts',(111.931632896949,17.4648871353774,57.1437268418812));
#137304=CARTESIAN_POINT('Ctrl Pts',(111.906151350592,17.465009047644,57.1651781838226));
#137305=CARTESIAN_POINT('Ctrl Pts',(111.880536982064,17.4651308261497,57.1864725867688));
#137306=CARTESIAN_POINT('Ctrl Pts',(111.854793571691,17.4652524338651,57.2076096087177));
#137307=CARTESIAN_POINT('Ctrl Pts',(111.830659124467,17.4653664410983,57.2274255667948));
#137308=CARTESIAN_POINT('Ctrl Pts',(111.806411261559,17.465480298222,57.2471032017298));
#137309=CARTESIAN_POINT('Ctrl Pts',(111.782053098436,17.4655939746343,57.2666421490116));
#137310=CARTESIAN_POINT('Ctrl Pts',(111.780429220894,17.4656015530618,57.2679447454971));
#137311=CARTESIAN_POINT('Ctrl Pts',(111.777792341615,17.4656138520919,57.2700576557719));
#137312=CARTESIAN_POINT('Ctrl Pts',(111.777179996071,17.4656167074982,57.270548089188));
#137313=CARTESIAN_POINT('Ctrl Pts',(111.776395605827,17.4656203651599,57.2711763148544));
#137314=CARTESIAN_POINT('Ctrl Pts',(111.775598150403,17.4656240892754,57.2718148987131));
#137315=CARTESIAN_POINT('Ctrl Pts',(111.774787618582,17.4656278798337,57.2724638263153));
#137316=CARTESIAN_POINT('Ctrl Pts',(111.760604535374,17.4656942088818,57.2838190796654));
#137317=CARTESIAN_POINT('Ctrl Pts',(111.742420120335,17.465780887691,57.2983450544814));
#137318=CARTESIAN_POINT('Ctrl Pts',(111.720157327019,17.4658878287095,57.3159423469922));
#137319=CARTESIAN_POINT('Ctrl Pts',(111.697136922665,17.4659984089701,57.3341384818336));
#137320=CARTESIAN_POINT('Ctrl Pts',(111.669755695092,17.4661306561564,57.3556185664265));
#137321=CARTESIAN_POINT('Ctrl Pts',(111.637895660831,17.4662843890616,57.3802271302202));
#137322=CARTESIAN_POINT('Ctrl Pts',(111.604130975223,17.4664473124022,57.4063068391424));
#137323=CARTESIAN_POINT('Ctrl Pts',(111.56533571254,17.4666343715798,57.4359003749058));
#137324=CARTESIAN_POINT('Ctrl Pts',(111.521336071247,17.4668452057531,57.4687707712478));
#137325=CARTESIAN_POINT('Ctrl Pts',(111.477336429953,17.4670560399264,57.5016411675897));
#137326=CARTESIAN_POINT('Ctrl Pts',(111.428131607977,17.4672906533659,57.5377879032397));
#137327=CARTESIAN_POINT('Ctrl Pts',(111.373524006893,17.4675484798121,57.5769274428994));
#137328=CARTESIAN_POINT('Ctrl Pts',(111.337953740903,17.4677164226458,57.6024221324442));
#137329=CARTESIAN_POINT('Ctrl Pts',(111.300090628467,17.4678942104067,57.629185713148));
#137330=CARTESIAN_POINT('Ctrl Pts',(111.259877307962,17.4680816222481,57.6571308871485));
#137331=CARTESIAN_POINT('Ctrl Pts',(111.23977064771,17.4681753281688,57.6711034741488));
#137332=CARTESIAN_POINT('Ctrl Pts',(111.219076435305,17.4682714447304,57.6853714592458));
#137333=CARTESIAN_POINT('Ctrl Pts',(111.197787444961,17.4683699324149,57.6999232647248));
#137334=CARTESIAN_POINT('Ctrl Pts',(111.187142949789,17.4684191762571,57.7071991674643));
#137335=CARTESIAN_POINT('Ctrl Pts',(111.176349760127,17.4684690130712,57.71454602529));
#137336=CARTESIAN_POINT('Ctrl Pts',(111.165406982368,17.4685194385309,57.7219623780656));
#137337=CARTESIAN_POINT('Ctrl Pts',(111.155657403354,17.4685643656064,57.7285700529149));
#137338=CARTESIAN_POINT('Ctrl Pts',(111.144636782127,17.4686150532942,57.7360084489736));
#137339=CARTESIAN_POINT('Ctrl Pts',(111.135424344395,17.4686573498515,57.7422034172612));
#137340=CARTESIAN_POINT('Ctrl Pts',(111.134296883493,17.4686625263005,57.7429615862423));
#137341=CARTESIAN_POINT('Ctrl Pts',(111.133196542218,17.4686675771778,57.7437011845906));
#137342=CARTESIAN_POINT('Ctrl Pts',(111.132128993479,17.468672476629,57.7444184518172));
#137343=CARTESIAN_POINT('Ctrl Pts',(111.071704874938,17.4689497895145,57.7850163546245));
#137344=CARTESIAN_POINT('Ctrl Pts',(111.014241928657,17.469209739296,57.8226602437051));
#137345=CARTESIAN_POINT('Ctrl Pts',(110.959910551484,17.4694526426504,57.8575777780466));
#137346=CARTESIAN_POINT('Ctrl Pts',(110.904095672232,17.4697021784086,57.8934487252678));
#137347=CARTESIAN_POINT('Ctrl Pts',(110.851585419274,17.4699337263767,57.9264422793881));
#137348=CARTESIAN_POINT('Ctrl Pts',(110.802525020451,17.4701476770414,57.9567642234572));
#137349=CARTESIAN_POINT('Ctrl Pts',(110.751292573144,17.4703710999328,57.9884286093784));
#137350=CARTESIAN_POINT('Ctrl Pts',(110.703821995689,17.4705753353621,58.0171795755969));
#137351=CARTESIAN_POINT('Ctrl Pts',(110.660240003903,17.470760841675,58.0432082184106));
#137352=CARTESIAN_POINT('Ctrl Pts',(110.628203113416,17.4708972063795,58.0623417353787));
#137353=CARTESIAN_POINT('Ctrl Pts',(110.598266636585,17.4710234509446,58.0800032780499));
#137354=CARTESIAN_POINT('Ctrl Pts',(110.570469576052,17.4711397500975,58.0962550110909));
#137355=CARTESIAN_POINT('Ctrl Pts',(110.547624402729,17.4712353312222,58.1096115909241));
#137356=CARTESIAN_POINT('Ctrl Pts',(110.526224099794,17.4713241947182,58.1220156960866));
#137357=CARTESIAN_POINT('Ctrl Pts',(110.506286149657,17.4714064277931,58.1334963711835));
#137358=CARTESIAN_POINT('Ctrl Pts',(110.496317174589,17.4714475443306,58.1392367087319));
#137359=CARTESIAN_POINT('Ctrl Pts',(110.486713787606,17.4714870080712,58.1447461885291));
#137360=CARTESIAN_POINT('Ctrl Pts',(110.477477796359,17.4715248232401,58.1500279186985));
#137361=CARTESIAN_POINT('Ctrl Pts',(110.472859800735,17.4715437308245,58.1526687837832));
#137362=CARTESIAN_POINT('Ctrl Pts',(110.468333654039,17.471562226548,58.1552527114472));
#137363=CARTESIAN_POINT('Ctrl Pts',(110.463899573078,17.4715803116796,58.1577800758039));
#137364=CARTESIAN_POINT('Ctrl Pts',(110.459465492116,17.4715983968111,58.1603074401607));
#137365=CARTESIAN_POINT('Ctrl Pts',(110.453789037814,17.4716214930161,58.1635364414641));
#137366=CARTESIAN_POINT('Ctrl Pts',(110.4508737383,17.4716333370874,58.1651928444699));
#137367=CARTESIAN_POINT('Ctrl Pts',(110.450871060701,17.4716333479658,58.1651943658172));
#137368=CARTESIAN_POINT('Ctrl Pts',(110.450868383044,17.4716333588444,58.1651958871963));
#137369=CARTESIAN_POINT('Ctrl Pts',(110.450865705331,17.4716333697233,58.1651974086071));
#137370=CARTESIAN_POINT('Ctrl Pts',(110.424150203037,17.4717419080043,58.1803764985696));
#137371=CARTESIAN_POINT('Ctrl Pts',(110.391741195077,17.4718758027233,58.1987191894422));
#137372=CARTESIAN_POINT('Ctrl Pts',(110.353555787436,17.4720344129501,58.220073765757));
#137373=CARTESIAN_POINT('Ctrl Pts',(110.312314412423,17.4722057167086,58.243137342774));
#137374=CARTESIAN_POINT('Ctrl Pts',(110.264334916551,17.4724058552091,58.2697142697748));
#137375=CARTESIAN_POINT('Ctrl Pts',(110.209484453875,17.4726336795687,58.2995559249602));
#137376=CARTESIAN_POINT('Ctrl Pts',(110.150435248625,17.4728789436324,58.3316819260199));
#137377=CARTESIAN_POINT('Ctrl Pts',(110.083422210429,17.4731563016772,58.3675911586784));
#137378=CARTESIAN_POINT('Ctrl Pts',(110.008254233598,17.4734638408916,58.4069116875536));
#137379=CARTESIAN_POINT('Ctrl Pts',(109.914932187883,17.4738456549278,58.4557286485513));
#137380=CARTESIAN_POINT('Ctrl Pts',(109.80903794466,17.4742740311308,58.5098027933334));
#137381=CARTESIAN_POINT('Ctrl Pts',(109.690191365439,17.4747441717411,58.568335905514));
#137382=CARTESIAN_POINT('Ctrl Pts',(109.644759030211,17.4749238957681,58.5907117786099));
#137383=CARTESIAN_POINT('Ctrl Pts',(109.597434018789,17.475109709447,58.6137386222985));
#137384=CARTESIAN_POINT('Ctrl Pts',(109.548196424467,17.4753012924258,58.6373705006825));
#137385=CARTESIAN_POINT('Ctrl Pts',(109.470298483254,17.4756043925229,58.6747580842652));
#137386=CARTESIAN_POINT('Ctrl Pts',(109.387612572138,17.47592194347,58.7136596031847));
#137387=CARTESIAN_POINT('Ctrl Pts',(109.30006910572,17.4762525214668,58.7538958831759));
#137388=CARTESIAN_POINT('Ctrl Pts',(109.256297372511,17.4764178104652,58.7740140231715));
#137389=CARTESIAN_POINT('Ctrl Pts',(109.211311250656,17.4765863456859,58.7944658539154));
#137390=CARTESIAN_POINT('Ctrl Pts',(109.165103823356,17.4767579389749,58.8152299777297));
#137391=CARTESIAN_POINT('Ctrl Pts',(109.142000109706,17.4768437356193,58.8256120396368));
#137392=CARTESIAN_POINT('Ctrl Pts',(109.118591069714,17.4769302956955,58.8360721748612));
#137393=CARTESIAN_POINT('Ctrl Pts',(109.094875930883,17.4770175935859,58.8466077877838));
#137394=CARTESIAN_POINT('Ctrl Pts',(109.083018361468,17.4770612425311,58.8518755942451));
#137395=CARTESIAN_POINT('Ctrl Pts',(109.071084267344,17.4771050758497,58.8571622701346));
#137396=CARTESIAN_POINT('Ctrl Pts',(109.059073559752,17.4771490902105,58.8624674965145));
#137397=CARTESIAN_POINT('Ctrl Pts',(109.053068205956,17.477171097391,58.8651201097044));
#137398=CARTESIAN_POINT('Ctrl Pts',(109.047043698793,17.4771931498265,58.8677773605172));
#137399=CARTESIAN_POINT('Ctrl Pts',(109.041000027737,17.4772152470961,58.8704392095162));
#137400=CARTESIAN_POINT('Ctrl Pts',(109.035722234518,17.4772345441125,58.87276373851));
#137401=CARTESIAN_POINT('Ctrl Pts',(109.029040845196,17.4772589448399,58.8757021475603));
#137402=CARTESIAN_POINT('Ctrl Pts',(109.024594720515,17.4772751673272,58.8776552791828));
#137403=CARTESIAN_POINT('Ctrl Pts',(109.02394952882,17.4772775214253,58.8779387045006));
#137404=CARTESIAN_POINT('Ctrl Pts',(109.023351416907,17.47727970346,58.8782014046281));
#137405=CARTESIAN_POINT('Ctrl Pts',(109.022811512541,17.4772816729723,58.8784385117749));
#137406=CARTESIAN_POINT('Ctrl Pts',(108.894616013314,17.4777493161777,58.9347374990424));
#137407=CARTESIAN_POINT('Ctrl Pts',(108.768938169259,17.4781914309708,58.9881074799368));
#137408=CARTESIAN_POINT('Ctrl Pts',(108.645940054624,17.4786100115034,59.0388676027788));
#137409=CARTESIAN_POINT('Ctrl Pts',(108.520461269671,17.4790370341191,59.0906514740775));
#137410=CARTESIAN_POINT('Ctrl Pts',(108.3977713007,17.4794395627121,59.1397189720536));
#137411=CARTESIAN_POINT('Ctrl Pts',(108.278015551975,17.4798195257597,59.1863611953479));
#137412=CARTESIAN_POINT('Ctrl Pts',(108.154689973338,17.4802108152235,59.2343937886722));
#137413=CARTESIAN_POINT('Ctrl Pts',(108.034476085892,17.4805781734427,59.2798542298973));
#137414=CARTESIAN_POINT('Ctrl Pts',(107.917505897425,17.4809235174297,59.3230125996528));
#137415=CARTESIAN_POINT('Ctrl Pts',(107.904174509995,17.480962877155,59.3279314679181));
#137416=CARTESIAN_POINT('Ctrl Pts',(107.890885230248,17.4810019507274,59.3328203845218));
#137417=CARTESIAN_POINT('Ctrl Pts',(107.877638233044,17.481040740837,59.3376797126102));
#137418=CARTESIAN_POINT('Ctrl Pts',(107.818808889225,17.4812130060425,59.3592597792801));
#137419=CARTESIAN_POINT('Ctrl Pts',(107.760813566222,17.4813796816511,59.3802565130386));
#137420=CARTESIAN_POINT('Ctrl Pts',(107.703666621925,17.4815409952453,59.4007000127499));
#137421=CARTESIAN_POINT('Ctrl Pts',(107.675093149776,17.4816216520424,59.4109217626055));
#137422=CARTESIAN_POINT('Ctrl Pts',(107.646731772284,17.4817009700903,59.4210052038805));
#137423=CARTESIAN_POINT('Ctrl Pts',(107.618584116815,17.4817789744635,59.4309538003569));
#137424=CARTESIAN_POINT('Ctrl Pts',(107.60451028908,17.4818179766501,59.4359280985951));
#137425=CARTESIAN_POINT('Ctrl Pts',(107.59048989185,17.4818566505234,59.4408686856294));
#137426=CARTESIAN_POINT('Ctrl Pts',(107.576523124441,17.4818949995002,59.4457759870934));
#137427=CARTESIAN_POINT('Ctrl Pts',(107.569539740736,17.4819141739886,59.4482296378254));
#137428=CARTESIAN_POINT('Ctrl Pts',(107.562569764487,17.4819332672591,59.4506749671646));
#137429=CARTESIAN_POINT('Ctrl Pts',(107.555613220062,17.481952279732,59.4531120273421));
#137430=CARTESIAN_POINT('Ctrl Pts',(107.552134947849,17.4819617859685,59.4543305574308));
#137431=CARTESIAN_POINT('Ctrl Pts',(107.548660033593,17.481971272006,59.4555470202291));
#137432=CARTESIAN_POINT('Ctrl Pts',(107.545188480304,17.4819807378965,59.4567614222034));
#137433=CARTESIAN_POINT('Ctrl Pts',(107.542670430008,17.4819876038687,59.457642274374));
#137434=CARTESIAN_POINT('Ctrl Pts',(107.539562333622,17.4819960701084,59.4587288813542));
#137435=CARTESIAN_POINT('Ctrl Pts',(107.53715197661,17.4820026310721,59.4595711238867));
#137436=CARTESIAN_POINT('Ctrl Pts',(107.536239253527,17.4820051154937,59.4598900534879));
#137437=CARTESIAN_POINT('Ctrl Pts',(107.535426584075,17.4820073268524,59.4601739606438));
#137438=CARTESIAN_POINT('Ctrl Pts',(107.534783906329,17.4820090751799,59.4603984520891));
#137439=CARTESIAN_POINT('Ctrl Pts',(107.465097798596,17.4821986478588,59.4847402550293));
#137440=CARTESIAN_POINT('Ctrl Pts',(107.38419840039,17.4824130222309,59.5126143740575));
#137441=CARTESIAN_POINT('Ctrl Pts',(107.291997713868,17.4826501715579,59.5437396635183));
#137442=CARTESIAN_POINT('Ctrl Pts',(107.189531181776,17.4829137256597,59.5783305173583));
#137443=CARTESIAN_POINT('Ctrl Pts',(107.073106034246,17.4832054111588,59.6169360157368));
#137444=CARTESIAN_POINT('Ctrl Pts',(106.942587169386,17.483521877318,59.6591031651156));
#137445=CARTESIAN_POINT('Ctrl Pts',(106.811979200765,17.483838559525,59.7012991015333));
#137446=CARTESIAN_POINT('Ctrl Pts',(106.667257041664,17.4841800456896,59.7470587048764));
#137447=CARTESIAN_POINT('Ctrl Pts',(106.508286258143,17.4845425150198,59.7958945385632));
#137448=CARTESIAN_POINT('Ctrl Pts',(106.431489682309,17.4847176189149,59.8194864510021));
#137449=CARTESIAN_POINT('Ctrl Pts',(106.351368001573,17.4848976137749,59.843796034588));
#137450=CARTESIAN_POINT('Ctrl Pts',(106.267907549805,17.4850820428647,59.8687688203452));
#137451=CARTESIAN_POINT('Ctrl Pts',(106.226177323922,17.4851742574096,59.8812552132238));
#137452=CARTESIAN_POINT('Ctrl Pts',(106.183612405287,17.4852675794758,59.8939074066797));
#137453=CARTESIAN_POINT('Ctrl Pts',(106.140211266131,17.4853619519497,59.9067187973344));
#137454=CARTESIAN_POINT('Ctrl Pts',(106.118510696552,17.4854091381866,59.9131244926617));
#137455=CARTESIAN_POINT('Ctrl Pts',(106.096601071844,17.485456586923,59.9195699872922));
#137456=CARTESIAN_POINT('Ctrl Pts',(106.074482210197,17.4855042909056,59.9260544707709));
#137457=CARTESIAN_POINT('Ctrl Pts',(106.05236334855,17.4855519948882,59.9325389542496));
#137458=CARTESIAN_POINT('Ctrl Pts',(106.028026569481,17.4856042505556,59.9396472395218));
#137459=CARTESIAN_POINT('Ctrl Pts',(106.007497736749,17.4856481610672,59.9456240832683));
#137460=CARTESIAN_POINT('Ctrl Pts',(105.871684204389,17.4859386618359,59.9851653602722));
#137461=CARTESIAN_POINT('Ctrl Pts',(105.741825421019,17.4862113759084,60.0222184875221));
#137462=CARTESIAN_POINT('Ctrl Pts',(105.617995399476,17.4864678570325,60.0570291801906));
#137463=CARTESIAN_POINT('Ctrl Pts',(105.490158559993,17.4867326372197,60.0929662564787));
#137464=CARTESIAN_POINT('Ctrl Pts',(105.368746790353,17.486980116041,60.1265131316419));
#137465=CARTESIAN_POINT('Ctrl Pts',(105.25382206313,17.4872117552075,60.1578862729108));
#137466=CARTESIAN_POINT('Ctrl Pts',(105.132685686557,17.487455914406,60.1909551236868));
#137467=CARTESIAN_POINT('Ctrl Pts',(105.018756426988,17.4876824751316,60.2216087253473));
#137468=CARTESIAN_POINT('Ctrl Pts',(104.912087673554,17.487892886475,60.2500452427954));
#137469=CARTESIAN_POINT('Ctrl Pts',(104.862368767094,17.4879909603867,60.2632996636591));
#137470=CARTESIAN_POINT('Ctrl Pts',(104.814226986751,17.488085522199,60.2760716723553));
#137471=CARTESIAN_POINT('Ctrl Pts',(104.767666547077,17.4881767010475,60.2883777438329));
#137472=CARTESIAN_POINT('Ctrl Pts',(104.712162742519,17.488285393599,60.3030475749378));
#137473=CARTESIAN_POINT('Ctrl Pts',(104.658906133875,17.4883892791678,60.3170553585036));
#137474=CARTESIAN_POINT('Ctrl Pts',(104.607902669725,17.488488556856,60.3304252570649));
#137475=CARTESIAN_POINT('Ctrl Pts',(104.582400937649,17.4885381957001,60.3371102063456));
#137476=CARTESIAN_POINT('Ctrl Pts',(104.557462491691,17.4885866839262,60.3436356843401));
#137477=CARTESIAN_POINT('Ctrl Pts',(104.53308794685,17.4886340426396,60.3500042942641));
#137478=CARTESIAN_POINT('Ctrl Pts',(104.52090067443,17.4886577219963,60.3531885992261));
#137479=CARTESIAN_POINT('Ctrl Pts',(104.508854377289,17.4886811190529,60.3563336871684));
#137480=CARTESIAN_POINT('Ctrl Pts',(104.496949129782,17.4887042366459,60.3594398743735));
#137481=CARTESIAN_POINT('Ctrl Pts',(104.490996506029,17.4887157954424,60.360992967976));
#137482=CARTESIAN_POINT('Ctrl Pts',(104.485079144685,17.4887272843775,60.3625363363941));
#137483=CARTESIAN_POINT('Ctrl Pts',(104.479197054648,17.4887387037962,60.3640700178451));
#137484=CARTESIAN_POINT('Ctrl Pts',(104.47625600963,17.4887444135055,60.3648368585706));
#137485=CARTESIAN_POINT('Ctrl Pts',(104.473323782439,17.4887501058361,60.3656012775543));
#137486=CARTESIAN_POINT('Ctrl Pts',(104.470400374162,17.4887557808304,60.3663632794904));
#137487=CARTESIAN_POINT('Ctrl Pts',(104.467476965886,17.4887614558246,60.3671252814265));
#137488=CARTESIAN_POINT('Ctrl Pts',(104.463225821211,17.488769707859,60.3682331399835));
#137489=CARTESIAN_POINT('Ctrl Pts',(104.461656607159,17.4887727538472,60.3686420388256));
#137490=CARTESIAN_POINT('Ctrl Pts',(104.461654620551,17.4887727577033,60.368642556487));
#137491=CARTESIAN_POINT('Ctrl Pts',(104.461652633928,17.4887727615596,60.3686430741524));
#137492=CARTESIAN_POINT('Ctrl Pts',(104.46165064729,17.4887727654158,60.3686435918218));
#137493=CARTESIAN_POINT('Ctrl Pts',(104.401089705658,17.488890319779,60.3844242917302));
#137494=CARTESIAN_POINT('Ctrl Pts',(104.32621244764,17.4890362204498,60.4039121781988));
#137495=CARTESIAN_POINT('Ctrl Pts',(104.23697820632,17.4892080200877,60.4269529138905));
#137496=CARTESIAN_POINT('Ctrl Pts',(104.139363991414,17.4893959534026,60.4521574014521));
#137497=CARTESIAN_POINT('Ctrl Pts',(104.024569659901,17.4896148896923,60.481613205935));
#137498=CARTESIAN_POINT('Ctrl Pts',(103.892524141172,17.4898603670786,60.5150569402054));
#137499=CARTESIAN_POINT('Ctrl Pts',(103.739662280845,17.4901445427954,60.5537729184988));
#137500=CARTESIAN_POINT('Ctrl Pts',(103.563681221673,17.4904643127914,60.5978322073689));
#137501=CARTESIAN_POINT('Ctrl Pts',(103.364448222258,17.4908107974363,60.6467547950338));
#137502=CARTESIAN_POINT('Ctrl Pts',(103.224908719071,17.4910534695607,60.6810193676571));
#137503=CARTESIAN_POINT('Ctrl Pts',(103.073962711404,17.4913092001858,60.7176677287305));
#137504=CARTESIAN_POINT('Ctrl Pts',(102.911561096065,17.4915744310346,60.7565269092083));
#137505=CARTESIAN_POINT('Ctrl Pts',(102.720876078408,17.4918858537319,60.8021536937697));
#137506=CARTESIAN_POINT('Ctrl Pts',(102.514396679508,17.4922103795442,60.8508255120447));
#137507=CARTESIAN_POINT('Ctrl Pts',(102.292057342075,17.4925416529916,60.9022926937826));
#137508=CARTESIAN_POINT('Ctrl Pts',(102.181980547703,17.4927056613924,60.9277733057449));
#137509=CARTESIAN_POINT('Ctrl Pts',(102.068016539687,17.4928713150982,60.9539396507437));
#137510=CARTESIAN_POINT('Ctrl Pts',(101.95015896678,17.4930378017596,60.9807662437774));
#137511=CARTESIAN_POINT('Ctrl Pts',(101.855388027447,17.4931716760359,61.0023378862116));
#137512=CARTESIAN_POINT('Ctrl Pts',(101.758099528033,17.4933060883184,61.0243364946143));
#137513=CARTESIAN_POINT('Ctrl Pts',(101.658290869385,17.4934406079925,61.0467510037277));
#137514=CARTESIAN_POINT('Ctrl Pts',(101.608386540061,17.4935078678295,61.0579582582844));
#137515=CARTESIAN_POINT('Ctrl Pts',(101.557852170928,17.4935751540335,61.0692694880241));
#137516=CARTESIAN_POINT('Ctrl Pts',(101.506687518559,17.4936424127867,61.0806835666572));
#137517=CARTESIAN_POINT('Ctrl Pts',(101.481105192374,17.4936760421634,61.0863906059737));
#137518=CARTESIAN_POINT('Ctrl Pts',(101.45536529538,17.4937096646441,61.092123357514));
#137519=CARTESIAN_POINT('Ctrl Pts',(101.429467800125,17.4937432734173,61.0978816900964));
#137520=CARTESIAN_POINT('Ctrl Pts',(101.416519052497,17.4937600778038,61.1007608563875));
#137521=CARTESIAN_POINT('Ctrl Pts',(101.403530905305,17.4937768787617,61.1036464179393));
#137522=CARTESIAN_POINT('Ctrl Pts',(101.39050335542,17.4937936754383,61.1065383593248));
#137523=CARTESIAN_POINT('Ctrl Pts',(101.380732693007,17.4938062729458,61.1087073153639));
#137524=CARTESIAN_POINT('Ctrl Pts',(101.37093986658,17.493818868045,61.1108798600595));
#137525=CARTESIAN_POINT('Ctrl Pts',(101.361124874889,17.4938314603758,61.113055987125));
#137526=CARTESIAN_POINT('Ctrl Pts',(101.35902556238,17.4938341537289,61.1135214353812));
#137527=CARTESIAN_POINT('Ctrl Pts',(101.356472721471,17.4938374271047,61.1140873592338));
#137528=CARTESIAN_POINT('Ctrl Pts',(101.35433743764,17.4938401634771,61.1145606492379));
#137529=CARTESIAN_POINT('Ctrl Pts',(101.353144998232,17.4938416915917,61.114824955858));
#137530=CARTESIAN_POINT('Ctrl Pts',(101.352082779859,17.4938430523437,61.1150603780317));
#137531=CARTESIAN_POINT('Ctrl Pts',(101.351302494755,17.4938440517714,61.1152333080974));
#137532=CARTESIAN_POINT('Ctrl Pts',(101.287051625161,17.4939263474572,61.1294728559702));
#137533=CARTESIAN_POINT('Ctrl Pts',(101.223030660778,17.4940069319958,61.1435964727026));
#137534=CARTESIAN_POINT('Ctrl Pts',(101.159246416405,17.4940860895325,61.1576075224112));
#137535=CARTESIAN_POINT('Ctrl Pts',(101.093940945311,17.4941671349424,61.1719527296132));
#137536=CARTESIAN_POINT('Ctrl Pts',(101.028884439126,17.4942467139571,61.1861800242748));
#137537=CARTESIAN_POINT('Ctrl Pts',(100.964031974283,17.4943232536764,61.2002873979025));
#137538=CARTESIAN_POINT('Ctrl Pts',(100.931409334339,17.4943617553387,61.2073838092962));
#137539=CARTESIAN_POINT('Ctrl Pts',(100.898837965544,17.4943994755923,61.2144498474929));
#137540=CARTESIAN_POINT('Ctrl Pts',(100.866342995605,17.4944372461246,61.2214870603931));
#137541=CARTESIAN_POINT('Ctrl Pts',(100.833715473761,17.4944751707287,61.2285529791508));
#137542=CARTESIAN_POINT('Ctrl Pts',(100.801165285133,17.4945131559579,61.2355898468858));
#137543=CARTESIAN_POINT('Ctrl Pts',(100.768675764999,17.4945506989153,61.2425979800308));
#137544=CARTESIAN_POINT('Ctrl Pts',(100.703294203028,17.4946262499601,61.2567010720317));
#137545=CARTESIAN_POINT('Ctrl Pts',(100.638157731775,17.4946999920661,61.2706878073948));
#137546=CARTESIAN_POINT('Ctrl Pts',(100.573274503652,17.4947721938095,61.2845605728875));
#137547=CARTESIAN_POINT('Ctrl Pts',(100.30816172466,17.4950672100317,61.3412446732083));
#137548=CARTESIAN_POINT('Ctrl Pts',(100.047279365178,17.4953366103002,61.3960277355345));
#137549=CARTESIAN_POINT('Ctrl Pts',(99.7906802196189,17.4955847117602,61.4490877200565));
#137550=CARTESIAN_POINT('Ctrl Pts',(99.5091437520911,17.4958569247035,61.5073042841719));
#137551=CARTESIAN_POINT('Ctrl Pts',(99.2327633342877,17.4961035016865,61.5634469666845));
#137552=CARTESIAN_POINT('Ctrl Pts',(98.9616049770858,17.4963293230433,61.6177163292878));
#137553=CARTESIAN_POINT('Ctrl Pts',(98.8355378727401,17.4964343120426,61.6429472735548));
#137554=CARTESIAN_POINT('Ctrl Pts',(98.7105993971195,17.4965348024916,61.6677728386518));
#137555=CARTESIAN_POINT('Ctrl Pts',(98.5867955406294,17.496631224476,61.6922108690025));
#137556=CARTESIAN_POINT('Ctrl Pts',(98.5248936123844,17.4966794354682,61.7044298841779));
#137557=CARTESIAN_POINT('Ctrl Pts',(98.4632753389212,17.4967266287093,61.7165520156652));
#137558=CARTESIAN_POINT('Ctrl Pts',(98.4019414248222,17.4967728546863,61.7285793385115));
#137559=CARTESIAN_POINT('Ctrl Pts',(98.3712744677727,17.4967959676748,61.7345929999346));
#137560=CARTESIAN_POINT('Ctrl Pts',(98.3406786005642,17.4968188388104,61.7405829591975));
#137561=CARTESIAN_POINT('Ctrl Pts',(98.3101539101087,17.4968414741929,61.7465494717433));
#137562=CARTESIAN_POINT('Ctrl Pts',(98.287260392267,17.4968584507298,61.7510243561526));
#137563=CARTESIAN_POINT('Ctrl Pts',(98.2644069113487,17.4968752946523,61.7554860517835));
#137564=CARTESIAN_POINT('Ctrl Pts',(98.2415935035095,17.4968920084843,61.7599346646255));
#137565=CARTESIAN_POINT('Ctrl Pts',(98.2350605450253,17.4968967947385,61.7612085910469));
#137566=CARTESIAN_POINT('Ctrl Pts',(98.2272178784105,17.4969025293887,61.7627373134558));
#137567=CARTESIAN_POINT('Ctrl Pts',(98.2214494621805,17.4969067405201,61.7638613805773));
#137568=CARTESIAN_POINT('Ctrl Pts',(98.2205033486733,17.4969074312137,61.7640457457556));
#137569=CARTESIAN_POINT('Ctrl Pts',(98.2196130357078,17.4969080809985,61.7642192279549));
#137570=CARTESIAN_POINT('Ctrl Pts',(98.2187934546568,17.4969086790445,61.7643789203052));
#137571=CARTESIAN_POINT('Ctrl Pts',(97.9395998248513,17.4971124058273,61.8187787711454));
#137572=CARTESIAN_POINT('Ctrl Pts',(97.6176562614074,17.4973327272939,61.8806636085485));
#137573=CARTESIAN_POINT('Ctrl Pts',(97.2529227856745,17.4975567818557,61.9495667300436));
#137574=CARTESIAN_POINT('Ctrl Pts',(96.9673494327301,17.4977322086172,62.0035154261268));
#137575=CARTESIAN_POINT('Ctrl Pts',(96.6555444295688,17.4979098745043,62.0617643138665));
#137576=CARTESIAN_POINT('Ctrl Pts',(96.3175040235945,17.4980825240508,62.1241144775376));
#137577=CARTESIAN_POINT('Ctrl Pts',(96.2238001826425,17.498130382015,62.1413977659159));
#137578=CARTESIAN_POINT('Ctrl Pts',(96.1280805677447,17.498177848875,62.1589964558432));
#137579=CARTESIAN_POINT('Ctrl Pts',(96.0303453756578,17.4982247570068,62.1769070473104));
#137580=CARTESIAN_POINT('Ctrl Pts',(95.8802390887399,17.4982968007133,62.2044149728001));
#137581=CARTESIAN_POINT('Ctrl Pts',(95.7253783623984,17.4983675280424,62.2326584756737));
#137582=CARTESIAN_POINT('Ctrl Pts',(95.5657645979641,17.498436304944,62.2616269799026));
#137583=CARTESIAN_POINT('Ctrl Pts',(95.4859577157469,17.4984706933949,62.2761112320171));
#137584=CARTESIAN_POINT('Ctrl Pts',(95.4049625740064,17.4985045942078,62.2907767344701));
#137585=CARTESIAN_POINT('Ctrl Pts',(95.3227794507625,17.4985379245222,62.3056224962104));
#137586=CARTESIAN_POINT('Ctrl Pts',(95.2816878891406,17.4985545896794,62.3130453770807));
#137587=CARTESIAN_POINT('Ctrl Pts',(95.2402993321428,17.498571112214,62.3205133227727));
#137588=CARTESIAN_POINT('Ctrl Pts',(95.1986138181634,17.4985874816507,62.3280262223119));
#137589=CARTESIAN_POINT('Ctrl Pts',(95.1777710611737,17.4985956663691,62.3317826720814));
#137590=CARTESIAN_POINT('Ctrl Pts',(95.1568540649386,17.4986038128135,62.3355503603128));
#137591=CARTESIAN_POINT('Ctrl Pts',(95.135862834657,17.498611919662,62.3393292744713));
#137592=CARTESIAN_POINT('Ctrl Pts',(95.1149645103485,17.49861999063,62.3430914633741));
#137593=CARTESIAN_POINT('Ctrl Pts',(95.0951917916129,17.4986275669728,62.3466491388768));
#137594=CARTESIAN_POINT('Ctrl Pts',(95.0729630543763,17.4986360074748,62.3506463463487));
#137595=CARTESIAN_POINT('Ctrl Pts',(95.0728642338951,17.498636044998,62.3506641164075));
#137596=CARTESIAN_POINT('Ctrl Pts',(95.072765364874,17.4986360825382,62.3506818951486));
#137597=CARTESIAN_POINT('Ctrl Pts',(95.0726664469983,17.4986361200954,62.3506996826287));
#137598=CARTESIAN_POINT('Ctrl Pts',(94.7539491580066,17.4987571308559,62.4080116435298));
#137599=CARTESIAN_POINT('Ctrl Pts',(94.4540862260824,17.498854098322,62.4615626426501));
#137600=CARTESIAN_POINT('Ctrl Pts',(94.1730878885652,17.4989323784167,62.5115348283151));
#137601=CARTESIAN_POINT('Ctrl Pts',(93.8708845850804,17.499016565759,62.5652780629681));
#137602=CARTESIAN_POINT('Ctrl Pts',(93.5905003663791,17.4990791528839,62.6148817985568));
#137603=CARTESIAN_POINT('Ctrl Pts',(93.3319416781723,17.499126020286,62.6605119366226));
#137604=CARTESIAN_POINT('Ctrl Pts',(93.0602342843467,17.4991752710761,62.708462543039));
#137605=CARTESIAN_POINT('Ctrl Pts',(92.8126285372438,17.4992071759936,62.7520246011495));
#137606=CARTESIAN_POINT('Ctrl Pts',(92.5891272193619,17.4992275110013,62.7913319494329));
#137607=CARTESIAN_POINT('Ctrl Pts',(92.335540307397,17.4992505833118,62.8359304742344));
#137608=CARTESIAN_POINT('Ctrl Pts',(92.1129838065121,17.4992588015865,62.8750517396529));
#137609=CARTESIAN_POINT('Ctrl Pts',(91.9214587222694,17.4992588252864,62.9088210133816));
#137610=CARTESIAN_POINT('Ctrl Pts',(91.6420934838691,17.49285958709,63.189615652045));
#137611=CARTESIAN_POINT('Ctrl Pts',(91.4789922092691,17.53610702643,62.18563192847));
#137612=CARTESIAN_POINT('Ctrl Pts',(91.2383773640691,17.31069605489,60.70627724341));
#137613=CARTESIAN_POINT('Ctrl Pts',(90.9525691952691,16.49526955095,58.9431717031));
#137614=CARTESIAN_POINT('Ctrl Pts',(90.7669853929691,15.69349549193,57.79357798411));
#137615=CARTESIAN_POINT('Ctrl Pts',(90.6082909803691,14.70024762493,56.80299770092));
#137616=CARTESIAN_POINT('Ctrl Pts',(90.5020501966691,13.74144627107,56.13084913298));
#137617=CARTESIAN_POINT('Ctrl Pts',(90.4359017984691,12.91166468527,55.70386232152));
#137618=CARTESIAN_POINT('Ctrl Pts',(90.3919674335691,12.26996490143,55.4170156774));
#137619=CARTESIAN_POINT('Ctrl Pts',(90.3493777568691,11.625304524,55.14038529705));
#137620=CARTESIAN_POINT('Ctrl Pts',(90.2953449889691,10.75812458152,54.79028890357));
#137621=CARTESIAN_POINT('Ctrl Pts',(90.2336264398691,9.65880570576201,54.39205929398));
#137622=CARTESIAN_POINT('Ctrl Pts',(90.1482830071691,7.87135436875902,53.83794898949));
#137623=CARTESIAN_POINT('Ctrl Pts',(90.0307622873691,4.60885046054901,53.0684560992));
#137624=CARTESIAN_POINT('Ctrl Pts',(89.9936930987691,1.72466757533901,52.81072925206));
#137625=CARTESIAN_POINT('Ctrl Pts',(89.9978563170691,-0.222741235654886,
52.82471933133));
#137626=CARTESIAN_POINT('Ctrl Pts',(92.8081742635691,17.49302494713,62.98048707022));
#137627=CARTESIAN_POINT('Ctrl Pts',(92.5986957331691,17.53515279357,62.00241380564));
#137628=CARTESIAN_POINT('Ctrl Pts',(92.2904281843691,17.31896818594,60.55914785523));
#137629=CARTESIAN_POINT('Ctrl Pts',(91.9177634399691,16.52369843295,58.82356961025));
#137630=CARTESIAN_POINT('Ctrl Pts',(91.6714076249691,15.73549484237,57.68441568033));
#137631=CARTESIAN_POINT('Ctrl Pts',(91.4546567602691,14.75116789232,56.69582182933));
#137632=CARTESIAN_POINT('Ctrl Pts',(91.3031505320691,13.79449439958,56.02158047908));
#137633=CARTESIAN_POINT('Ctrl Pts',(91.2028409584691,12.96185490683,55.59044131214));
#137634=CARTESIAN_POINT('Ctrl Pts',(91.1354530152691,12.32146797839,55.30843405596));
#137635=CARTESIAN_POINT('Ctrl Pts',(91.0705758403691,11.6762140863,55.03376811454));
#137636=CARTESIAN_POINT('Ctrl Pts',(90.9888550570691,10.80763428018,54.68635453666));
#137637=CARTESIAN_POINT('Ctrl Pts',(90.8964011661691,9.70473219682602,54.29014956108));
#137638=CARTESIAN_POINT('Ctrl Pts',(90.7663353867691,7.91003779904601,53.73885583037));
#137639=CARTESIAN_POINT('Ctrl Pts',(90.5830034095691,4.63059635124401,52.97296192257));
#137640=CARTESIAN_POINT('Ctrl Pts',(90.5158616249691,1.73018539026001,52.71855132778));
#137641=CARTESIAN_POINT('Ctrl Pts',(90.5140275106691,-0.223476692403986,
52.73371084717));
#137642=CARTESIAN_POINT('Ctrl Pts',(95.0334241451691,17.49340335946,62.57726075376));
#137643=CARTESIAN_POINT('Ctrl Pts',(94.7354399602691,17.53146746781,61.64878450661));
#137644=CARTESIAN_POINT('Ctrl Pts',(94.2980792778691,17.3287395782,60.27468725031));
#137645=CARTESIAN_POINT('Ctrl Pts',(93.7599791478691,16.56684333187,58.59467001799));
#137646=CARTESIAN_POINT('Ctrl Pts',(93.3979525790691,15.80201717449,57.47859068081));
#137647=CARTESIAN_POINT('Ctrl Pts',(93.0707154216691,14.83409351927,56.49734889427));
#137648=CARTESIAN_POINT('Ctrl Pts',(92.8329885552691,13.88266802702,55.82142820774));
#137649=CARTESIAN_POINT('Ctrl Pts',(92.6675763969691,13.04676841354,55.3837256506));
#137650=CARTESIAN_POINT('Ctrl Pts',(92.5552464285691,12.40954656296,55.10962258496));
#137651=CARTESIAN_POINT('Ctrl Pts',(92.4477320239691,11.76404691488,54.83811150331));
#137652=CARTESIAN_POINT('Ctrl Pts',(92.3130280801691,10.89384905739,54.49495852329));
#137653=CARTESIAN_POINT('Ctrl Pts',(92.1617766247691,9.78542268762302,54.1017826688));
#137654=CARTESIAN_POINT('Ctrl Pts',(91.9461684628691,7.97909093036001,53.55434070925));
#137655=CARTESIAN_POINT('Ctrl Pts',(91.6370372572691,4.67110183200301,52.79259801177));
#137656=CARTESIAN_POINT('Ctrl Pts',(91.5126236727691,1.74147908297301,52.54249043603));
#137657=CARTESIAN_POINT('Ctrl Pts',(91.4993303696691,-0.224968888493586,
52.55999386635));
#137658=CARTESIAN_POINT('Ctrl Pts',(98.3123086382691,17.49367872538,61.95032016408));
#137659=CARTESIAN_POINT('Ctrl Pts',(97.8838690771691,17.52132588781,61.0961871323));
#137660=CARTESIAN_POINT('Ctrl Pts',(97.2563270796691,17.3278166254,59.82631141409));
#137661=CARTESIAN_POINT('Ctrl Pts',(96.4754412409691,16.60157660903,58.23885952741));
#137662=CARTESIAN_POINT('Ctrl Pts',(95.9439265902691,15.8644449042,57.16729227158));
#137663=CARTESIAN_POINT('Ctrl Pts',(95.4548753321691,14.91906406746,56.20859012133));
#137664=CARTESIAN_POINT('Ctrl Pts',(95.0906828307691,13.97865602756,55.53812427992));
#137665=CARTESIAN_POINT('Ctrl Pts',(94.8297011904691,13.1440013253,55.09570191083));
#137666=CARTESIAN_POINT('Ctrl Pts',(94.6507179597691,12.51318114468,54.83035115667));
#137667=CARTESIAN_POINT('Ctrl Pts',(94.4801736252691,11.86966475712,54.56265476203));
#137668=CARTESIAN_POINT('Ctrl Pts',(94.2671175844691,10.99981417036,54.22446202571));
#137669=CARTESIAN_POINT('Ctrl Pts',(94.0289868932691,9.88660333602602,53.83473114943));
#137670=CARTESIAN_POINT('Ctrl Pts',(93.6870297939691,8.06867605678801,53.29066962107));
#137671=CARTESIAN_POINT('Ctrl Pts',(93.1923467916691,4.72816996048401,52.5304743899));
#137672=CARTESIAN_POINT('Ctrl Pts',(92.9840367818691,1.75997518098801,52.28237290523));
#137673=CARTESIAN_POINT('Ctrl Pts',(92.9537596435691,-0.227382347777086,
52.30357915893));
#137674=CARTESIAN_POINT('Ctrl Pts',(101.476063383869,17.49353152741,61.29633982016));
#137675=CARTESIAN_POINT('Ctrl Pts',(100.921772906669,17.50678730304,60.51612407986));
#137676=CARTESIAN_POINT('Ctrl Pts',(100.110868018069,17.31209403281,59.35052803616));
#137677=CARTESIAN_POINT('Ctrl Pts',(99.0967857761691,16.60753119682,57.86441562302));
#137678=CARTESIAN_POINT('Ctrl Pts',(98.4027331908691,15.89075779816,56.84705199828));
#137679=CARTESIAN_POINT('Ctrl Pts',(97.7585857601691,14.96553329684,55.92243481635));
#137680=CARTESIAN_POINT('Ctrl Pts',(97.2730114467691,14.03873742039,55.26579785069));
#137681=CARTESIAN_POINT('Ctrl Pts',(96.9202344708691,13.21083938854,54.82435903563));
#137682=CARTESIAN_POINT('Ctrl Pts',(96.6766080013691,12.58779566903,54.56550800276));
#137683=CARTESIAN_POINT('Ctrl Pts',(96.4451267608691,11.9483583019,54.30142844987));
#137684=CARTESIAN_POINT('Ctrl Pts',(96.1563018818691,11.08137533143,53.96772273336));
#137685=CARTESIAN_POINT('Ctrl Pts',(95.8342360423691,9.96667796475001,53.5814680127));
#137686=CARTESIAN_POINT('Ctrl Pts',(95.3702583734691,8.14278530794401,53.04015645856));
#137687=CARTESIAN_POINT('Ctrl Pts',(94.6966272138691,4.78001049072901,52.27965855516));
#137688=CARTESIAN_POINT('Ctrl Pts',(94.4079250495691,1.77918161124201,52.03051117877));
#137689=CARTESIAN_POINT('Ctrl Pts',(94.3611452467691,-0.229864186975786,
52.05546697121));
#137690=CARTESIAN_POINT('Ctrl Pts',(104.621046699869,17.49157360923,60.55369177597));
#137691=CARTESIAN_POINT('Ctrl Pts',(103.941719998769,17.49095598093,59.85125262095));
#137692=CARTESIAN_POINT('Ctrl Pts',(102.948813513369,17.29010700753,58.79646558991));
#137693=CARTESIAN_POINT('Ctrl Pts',(101.704261160469,16.59820570304,57.42793899511));
#137694=CARTESIAN_POINT('Ctrl Pts',(100.849876330569,15.89691605225,56.47926166912));
#137695=CARTESIAN_POINT('Ctrl Pts',(100.052867821069,14.99073822913,55.60442015319));
#137696=CARTESIAN_POINT('Ctrl Pts',(99.4475331754691,14.08024912469,54.97301510726));
#137697=CARTESIAN_POINT('Ctrl Pts',(99.0041424461691,13.26410825573,54.54036692231));
#137698=CARTESIAN_POINT('Ctrl Pts',(98.6960975395691,12.64985632218,54.28771822127));
#137699=CARTESIAN_POINT('Ctrl Pts',(98.4040997745691,12.01595884731,54.02882577639));
#137700=CARTESIAN_POINT('Ctrl Pts',(98.0400351694691,11.15329344622,53.70144103815));
#137701=CARTESIAN_POINT('Ctrl Pts',(97.6347501637691,10.03867108199,53.32138367282));
#137702=CARTESIAN_POINT('Ctrl Pts',(97.0498718249691,8.21126455271101,52.78612552645));
#137703=CARTESIAN_POINT('Ctrl Pts',(96.1992862091691,4.83024970546001,52.02935270629));
#137704=CARTESIAN_POINT('Ctrl Pts',(95.8317275561691,1.79882218783101,51.77865520573));
#137705=CARTESIAN_POINT('Ctrl Pts',(95.7685464794691,-0.232393034910786,
51.80735253732));
#137706=CARTESIAN_POINT('Ctrl Pts',(107.206331732069,17.48793196066,59.79698581959));
#137707=CARTESIAN_POINT('Ctrl Pts',(106.424335049069,17.47679956275,59.16535434663));
#137708=CARTESIAN_POINT('Ctrl Pts',(105.282246068869,17.26723075518,58.21301206074));
#137709=CARTESIAN_POINT('Ctrl Pts',(103.849819279169,16.57860703868,56.96285248062));
#137710=CARTESIAN_POINT('Ctrl Pts',(102.865084831869,15.8861456528,56.08863860426));
#137711=CARTESIAN_POINT('Ctrl Pts',(101.944004472769,14.9947548764,55.27363787577));
#137712=CARTESIAN_POINT('Ctrl Pts',(101.241437676969,14.09987468339,54.67719491956));
#137713=CARTESIAN_POINT('Ctrl Pts',(100.724490474169,13.29748172548,54.26189382541));
#137714=CARTESIAN_POINT('Ctrl Pts',(100.363674930769,12.69122630203,54.01677538362));
#137715=CARTESIAN_POINT('Ctrl Pts',(100.022315310469,12.06297792511,53.76608434928));
#137716=CARTESIAN_POINT('Ctrl Pts',(99.5969390137691,11.20486683145,53.44885422607));
#137717=CARTESIAN_POINT('Ctrl Pts',(99.1240602916691,10.09129477713,53.08026985688));
#137718=CARTESIAN_POINT('Ctrl Pts',(98.4411431664691,8.26255458396301,52.55881082705));
#137719=CARTESIAN_POINT('Ctrl Pts',(97.4476761906691,4.86917168282301,51.8176534126));
#137720=CARTESIAN_POINT('Ctrl Pts',(97.0175166613691,1.81445350612301,51.56911166491));
#137721=CARTESIAN_POINT('Ctrl Pts',(96.9414792205691,-0.234402174419586,
51.60056036597));
#137722=CARTESIAN_POINT('Ctrl Pts',(109.221604211669,17.48372544845,59.02333129694));
#137723=CARTESIAN_POINT('Ctrl Pts',(108.359784642469,17.46375567822,58.45574398136));
#137724=CARTESIAN_POINT('Ctrl Pts',(107.102015888569,17.24379846808,57.59775863006));
#137725=CARTESIAN_POINT('Ctrl Pts',(105.524816585069,16.55226120142,56.46376307926));
#137726=CARTESIAN_POINT('Ctrl Pts',(104.439982558469,15.8637820089,55.66640186783));
#137727=CARTESIAN_POINT('Ctrl Pts',(103.423883984169,14.98313091293,54.9173947312));
#137728=CARTESIAN_POINT('Ctrl Pts',(102.646954741169,14.10173774314,54.36322879206));
#137729=CARTESIAN_POINT('Ctrl Pts',(102.073834275069,13.31262966272,53.97252742131));
#137730=CARTESIAN_POINT('Ctrl Pts',(101.672467124869,12.71315223001,53.73834234543));
#137731=CARTESIAN_POINT('Ctrl Pts',(101.293368480369,12.09006135913,53.49997643624));
#137732=CARTESIAN_POINT('Ctrl Pts',(100.821239581369,11.23624367659,53.19828953843));
#137733=CARTESIAN_POINT('Ctrl Pts',(100.297134086169,10.12429194288,52.84806009283));
#137734=CARTESIAN_POINT('Ctrl Pts',(99.5401819745691,8.29592164133101,52.35088649986));
#137735=CARTESIAN_POINT('Ctrl Pts',(98.4397626213691,4.89564257240101,51.64188202533));
#137736=CARTESIAN_POINT('Ctrl Pts',(97.9644651398691,1.82535593403501,51.40219205419));
#137737=CARTESIAN_POINT('Ctrl Pts',(97.8800497432691,-0.235801263741986,
51.43506172539));
#137738=CARTESIAN_POINT('Ctrl Pts',(110.673215030269,17.48001284702,58.31066582355));
#137739=CARTESIAN_POINT('Ctrl Pts',(109.754172542369,17.4528430433,57.7969602139));
#137740=CARTESIAN_POINT('Ctrl Pts',(108.413728072469,17.22294323409,57.01954740541));
#137741=CARTESIAN_POINT('Ctrl Pts',(106.733762387369,16.52601355492,55.98868535554));
#137742=CARTESIAN_POINT('Ctrl Pts',(105.578169273769,15.83872897935,55.26157469267));
#137743=CARTESIAN_POINT('Ctrl Pts',(104.495167177069,14.96539903947,54.57518563264));
#137744=CARTESIAN_POINT('Ctrl Pts',(103.666047098169,14.0945150779,54.06328095415));
#137745=CARTESIAN_POINT('Ctrl Pts',(103.053623379069,13.31645894672,53.69908149772));
#137746=CARTESIAN_POINT('Ctrl Pts',(102.623789120869,12.72222884999,53.4775456014));
#137747=CARTESIAN_POINT('Ctrl Pts',(102.218370147569,12.10331314131,53.25326699941));
#137748=CARTESIAN_POINT('Ctrl Pts',(101.713794163769,11.25304338524,52.96950594007));
#137749=CARTESIAN_POINT('Ctrl Pts',(101.154507689069,10.14273559401,52.64069966665));
#137750=CARTESIAN_POINT('Ctrl Pts',(100.347069733169,8.31549541333901,52.17289680127));
#137751=CARTESIAN_POINT('Ctrl Pts',(99.1749900388691,4.91197175937601,51.50467231339));
#137752=CARTESIAN_POINT('Ctrl Pts',(98.6719824568691,1.83221907747001,51.27785989188));
#137753=CARTESIAN_POINT('Ctrl Pts',(98.5843309607691,-0.236680889114086,
51.31085228728));
#137754=CARTESIAN_POINT('Ctrl Pts',(112.026178776769,17.47584264663,57.41496060291));
#137755=CARTESIAN_POINT('Ctrl Pts',(111.054304371469,17.44067220964,56.96322273142));
#137756=CARTESIAN_POINT('Ctrl Pts',(109.637898310969,17.19839289674,56.27995401627));
#137757=CARTESIAN_POINT('Ctrl Pts',(107.864525222969,16.49257767027,55.37376659663));
#137758=CARTESIAN_POINT('Ctrl Pts',(106.645070431869,15.8045298653,54.73368567427));
#137759=CARTESIAN_POINT('Ctrl Pts',(105.502119542669,14.93766113307,54.1273069539));
#137760=CARTESIAN_POINT('Ctrl Pts',(104.626551783569,14.0776072634,53.6717926103));
#137761=CARTESIAN_POINT('Ctrl Pts',(103.979374836369,13.31165186547,53.34497834332));
#137762=CARTESIAN_POINT('Ctrl Pts',(103.524307770069,12.72281268686,53.14263950197));
#137763=CARTESIAN_POINT('Ctrl Pts',(103.095833717869,12.1083681819,52.93935575519));
#137764=CARTESIAN_POINT('Ctrl Pts',(102.563125775069,11.2619717921,52.68248156474));
#137765=CARTESIAN_POINT('Ctrl Pts',(101.973995647869,10.15375628522,52.38598466337));
#137766=CARTESIAN_POINT('Ctrl Pts',(101.124401221169,8.32857766047701,51.96347806666));
#137767=CARTESIAN_POINT('Ctrl Pts',(99.8948724104691,4.92400200723901,51.35987931168));
#137768=CARTESIAN_POINT('Ctrl Pts',(99.3745994012691,1.83743075427201,51.15495858885));
#137769=CARTESIAN_POINT('Ctrl Pts',(99.2892524687691,-0.237347620061986,
51.18649564272));
#137770=CARTESIAN_POINT('Ctrl Pts',(113.188445942169,17.47166983262,56.27542203421));
#137771=CARTESIAN_POINT('Ctrl Pts',(112.172263619869,17.42788547533,55.89634925378));
#137772=CARTESIAN_POINT('Ctrl Pts',(110.692758979669,17.17098864104,55.32530572893));
#137773=CARTESIAN_POINT('Ctrl Pts',(108.843546518669,16.45293860262,54.57208052895));
#137774=CARTESIAN_POINT('Ctrl Pts',(107.573079972769,15.7622252762,54.04093228966));
#137775=CARTESIAN_POINT('Ctrl Pts',(106.383104391469,14.90097081599,53.53723091173));
#137776=CARTESIAN_POINT('Ctrl Pts',(105.471805752069,14.05204799653,53.15666631614));
#137777=CARTESIAN_POINT('Ctrl Pts',(104.798395092669,13.29921052309,52.88163095715));
#137778=CARTESIAN_POINT('Ctrl Pts',(104.324299692669,12.7158750262,52.70763929966));
#137779=CARTESIAN_POINT('Ctrl Pts',(103.878996809469,12.10616052631,52.53481596519));
#137780=CARTESIAN_POINT('Ctrl Pts',(103.326404821569,11.26390566317,52.3171231399));
#137781=CARTESIAN_POINT('Ctrl Pts',(102.717650256469,10.15814664048,52.06780970547));
#137782=CARTESIAN_POINT('Ctrl Pts',(101.841943206069,8.33580711274201,51.71237805453));
#137783=CARTESIAN_POINT('Ctrl Pts',(100.582659540169,4.93206502020601,51.2059184364));
#137784=CARTESIAN_POINT('Ctrl Pts',(100.066369037669,1.84107373378501,51.03478639303));
#137785=CARTESIAN_POINT('Ctrl Pts',(99.9955851491691,-0.237812507849086,
51.06184076114));
#137786=CARTESIAN_POINT('Ctrl Pts',(114.125881804469,17.46819840414,54.80511293345));
#137787=CARTESIAN_POINT('Ctrl Pts',(113.075997776769,17.41492096989,54.51469436962));
#137788=CARTESIAN_POINT('Ctrl Pts',(111.549470398169,17.14056046656,54.08239064277));
#137789=CARTESIAN_POINT('Ctrl Pts',(109.646785590869,16.40654507693,53.5223372395));
#137790=CARTESIAN_POINT('Ctrl Pts',(108.341891044269,15.7114208792,53.13068024962));
#137791=CARTESIAN_POINT('Ctrl Pts',(107.121834027869,14.85569373811,52.76062809667));
#137792=CARTESIAN_POINT('Ctrl Pts',(106.189106230169,14.01930261972,52.47974204073));
#137793=CARTESIAN_POINT('Ctrl Pts',(105.501006553569,13.28178778393,52.27521181241));
#137794=CARTESIAN_POINT('Ctrl Pts',(105.016385994269,12.70458531254,52.14111418883));
#137795=CARTESIAN_POINT('Ctrl Pts',(104.562932235469,12.10030644958,52.0107829688));
#137796=CARTESIAN_POINT('Ctrl Pts',(104.002143959169,11.26286251636,51.84785983031));
#137797=CARTESIAN_POINT('Ctrl Pts',(103.388634838669,10.16016220358,51.66454860331));
#137798=CARTESIAN_POINT('Ctrl Pts',(102.510622200469,8.34157678397201,51.40350477807));
#137799=CARTESIAN_POINT('Ctrl Pts',(101.264203279969,4.93999315991101,51.03437259754));
#137800=CARTESIAN_POINT('Ctrl Pts',(100.787670666569,1.84502567070201,50.91043616355));
#137801=CARTESIAN_POINT('Ctrl Pts',(100.754059651069,-0.238314140392786,
50.9279295742));
#137802=CARTESIAN_POINT('Ctrl Pts',(114.539534408869,17.46722107301,53.67912966544));
#137803=CARTESIAN_POINT('Ctrl Pts',(113.476828137169,17.4073581895,53.45462064778));
#137804=CARTESIAN_POINT('Ctrl Pts',(111.933342665269,17.11996315362,53.12635989279));
#137805=CARTESIAN_POINT('Ctrl Pts',(110.014547047469,16.37339715948,52.71350806941));
#137806=CARTESIAN_POINT('Ctrl Pts',(108.700990537169,15.67453448001,52.42915265115));
#137807=CARTESIAN_POINT('Ctrl Pts',(107.475303053069,14.82273438004,52.1628920189));
#137808=CARTESIAN_POINT('Ctrl Pts',(106.540338441969,13.9958275305,51.96016673408));
#137809=CARTESIAN_POINT('Ctrl Pts',(105.852098050869,13.2701199685,51.81147738317));
#137810=CARTESIAN_POINT('Ctrl Pts',(105.367562667669,12.69751801236,51.70901280385));
#137811=CARTESIAN_POINT('Ctrl Pts',(104.915851437869,12.09743795773,51.61240634049));
#137812=CARTESIAN_POINT('Ctrl Pts',(104.359190902469,11.26379112788,51.49296213066));
#137813=CARTESIAN_POINT('Ctrl Pts',(103.754568792369,10.16369897044,51.36207880897));
#137814=CARTESIAN_POINT('Ctrl Pts',(102.894237682569,8.34833379260701,51.17605601973));
#137815=CARTESIAN_POINT('Ctrl Pts',(101.690546558169,4.94875024428401,50.91587031644));
#137816=CARTESIAN_POINT('Ctrl Pts',(101.268979457369,1.84978306717701,50.82795847283));
#137817=CARTESIAN_POINT('Ctrl Pts',(101.278306997869,-0.238915478837686,
50.83534589793));
#137818=CARTESIAN_POINT('Ctrl Pts',(114.722328637469,17.46712808947,53.051289402));
#137819=CARTESIAN_POINT('Ctrl Pts',(113.654564451069,17.40365408808,52.86334352169));
#137820=CARTESIAN_POINT('Ctrl Pts',(112.104688863969,17.10888025502,52.59292283969));
#137821=CARTESIAN_POINT('Ctrl Pts',(110.180954315469,16.35510969368,52.262432252));
#137822=CARTESIAN_POINT('Ctrl Pts',(108.865472379469,15.65410379572,52.03831580661));
#137823=CARTESIAN_POINT('Ctrl Pts',(107.639522339869,14.80461369374,51.83047343371));
#137824=CARTESIAN_POINT('Ctrl Pts',(106.705667287469,13.98326026859,51.67177167508));
#137825=CARTESIAN_POINT('Ctrl Pts',(106.019208150569,13.26447423575,51.55455277005));
#137826=CARTESIAN_POINT('Ctrl Pts',(105.536071241069,12.69456042945,51.46969752251));
#137827=CARTESIAN_POINT('Ctrl Pts',(105.086676320869,12.0969679499,51.39195280225));
#137828=CARTESIAN_POINT('Ctrl Pts',(104.534087620169,11.26560740794,51.29681409481));
#137829=CARTESIAN_POINT('Ctrl Pts',(103.936593793969,10.16715557418,51.19525657912));
#137830=CARTESIAN_POINT('Ctrl Pts',(103.089545611369,8.35379901046901,51.05114625581));
#137831=CARTESIAN_POINT('Ctrl Pts',(101.915640831969,4.95541579057301,50.85167903847));
#137832=CARTESIAN_POINT('Ctrl Pts',(101.529527658769,1.85347521690601,50.78336841914));
#137833=CARTESIAN_POINT('Ctrl Pts',(101.565834902869,-0.239381754617886,
50.78456512415));
#137834=CARTESIAN_POINT('',(101.414238575321,-1.58575583955758E-11,50.8108648870179));
#137835=CARTESIAN_POINT('Ctrl Pts',(101.414232124329,-1.74238401484672E-11,
50.8108622891728));
#137836=CARTESIAN_POINT('Ctrl Pts',(101.414231512955,2.34246738429908,50.8108623969735));
#137837=CARTESIAN_POINT('Ctrl Pts',(101.783910643607,4.68273078873375,50.8827213256914));
#137838=CARTESIAN_POINT('Ctrl Pts',(103.178130714759,8.98192555702816,51.1537320224966));
#137839=CARTESIAN_POINT('Ctrl Pts',(104.036052367674,10.5874908373517,51.3204960861428));
#137840=CARTESIAN_POINT('Ctrl Pts',(105.408020839001,12.7886822580781,51.5871812855231));
#137841=CARTESIAN_POINT('Ctrl Pts',(106.527871835993,14.0475405981964,51.8048594765732));
#137842=CARTESIAN_POINT('Ctrl Pts',(108.895550762846,15.7646605470862,52.2650921011255));
#137843=CARTESIAN_POINT('Ctrl Pts',(109.922967445704,16.3125473846403,52.4648027231681));
#137844=CARTESIAN_POINT('Ctrl Pts',(112.097867784466,17.1144886571945,52.8875627106287));
#137845=CARTESIAN_POINT('Ctrl Pts',(113.233562723013,17.3623385458543,53.1083205694869));
#137846=CARTESIAN_POINT('Ctrl Pts',(114.384105789773,17.4511159784776,53.3319646111095));
#137847=CARTESIAN_POINT('',(90.732949730332,1.38578833057197E-14,52.6942600470911));
#137848=CARTESIAN_POINT('',(90.7329496419691,1.4210854715202E-14,52.69425954596));
#137849=CARTESIAN_POINT('',(90.1948181095954,4.38657743647023,53.1165555002035));
#137850=CARTESIAN_POINT('Ctrl Pts',(90.7329498186953,1.3510709105438E-14,
52.6942605482239));
#137851=CARTESIAN_POINT('Ctrl Pts',(90.7329485107428,0.219822085862891,
52.6942607788508));
#137852=CARTESIAN_POINT('Ctrl Pts',(90.7292741915679,0.43943636238306,52.6973774297948));
#137853=CARTESIAN_POINT('Ctrl Pts',(90.7218295116067,0.658717449913899,
52.7036013862621));
#137854=CARTESIAN_POINT('Ctrl Pts',(90.716851108255,0.805355009462212,52.7077634678961));
#137855=CARTESIAN_POINT('Ctrl Pts',(90.7101855631875,0.95184333440204,52.7133151173478));
#137856=CARTESIAN_POINT('Ctrl Pts',(90.7017909963613,1.09814271743628,52.7202539366756));
#137857=CARTESIAN_POINT('Ctrl Pts',(90.6890221508373,1.32067644203491,52.7308084672368));
#137858=CARTESIAN_POINT('Ctrl Pts',(90.672255291451,1.54277324072251,52.7445723874834));
#137859=CARTESIAN_POINT('Ctrl Pts',(90.6512991909533,1.76428767234441,52.7615386845998));
#137860=CARTESIAN_POINT('Ctrl Pts',(90.6464708510102,1.81532517229662,52.7654477634888));
#137861=CARTESIAN_POINT('Ctrl Pts',(90.6414199063934,1.86633173329605,52.7695268501241));
#137862=CARTESIAN_POINT('Ctrl Pts',(90.6361436310377,1.91730553703418,52.7737758750406));
#137863=CARTESIAN_POINT('Ctrl Pts',(90.629541216305,1.98109109978426,52.7790928501447));
#137864=CARTESIAN_POINT('Ctrl Pts',(90.6224695805114,2.04579464308325,52.7847639911231));
#137865=CARTESIAN_POINT('Ctrl Pts',(90.6151687013308,2.10936825487059,52.7906050704508));
#137866=CARTESIAN_POINT('Ctrl Pts',(90.6120838169945,2.13623039494425,52.7930731367864));
#137867=CARTESIAN_POINT('Ctrl Pts',(90.6089579305889,2.16289088087897,52.7955709051654));
#137868=CARTESIAN_POINT('Ctrl Pts',(90.6058088683883,2.18919559519112,52.798081728641));
#137869=CARTESIAN_POINT('Ctrl Pts',(90.5822808745777,2.38572939354042,52.8168411673025));
#137870=CARTESIAN_POINT('Ctrl Pts',(90.554990387312,2.58427754605148,52.838383537977));
#137871=CARTESIAN_POINT('Ctrl Pts',(90.5237507685048,2.78470597157349,52.8628583306962));
#137872=CARTESIAN_POINT('Ctrl Pts',(90.492846253712,2.98298442303857,52.8870705849593));
#137873=CARTESIAN_POINT('Ctrl Pts',(90.4580769981051,3.18310296691071,52.9141526371188));
#137874=CARTESIAN_POINT('Ctrl Pts',(90.4192138488107,3.38491904070291,52.9442554065099));
#137875=CARTESIAN_POINT('Ctrl Pts',(90.3809087028403,3.58383740697335,52.973925955515));
#137876=CARTESIAN_POINT('Ctrl Pts',(90.3386264457378,3.7844048324515,53.006531054824));
#137877=CARTESIAN_POINT('Ctrl Pts',(90.2920989964633,3.98647333373282,53.0422219666209));
#137878=CARTESIAN_POINT('Ctrl Pts',(90.2615363499203,4.11920676912283,53.0656663793075));
#137879=CARTESIAN_POINT('Ctrl Pts',(90.2291409815297,4.25258765915242,53.0904424057959));
#137880=CARTESIAN_POINT('Ctrl Pts',(90.194825018716,4.38657155579178,53.1165946859612));
#137881=CARTESIAN_POINT('',(90.6495102260087,12.954682194379,55.6952426313253));
#137882=CARTESIAN_POINT('Origin',(94.1069496688351,2.20409106096583,75.3033561008651));
#137883=CARTESIAN_POINT('Ctrl Pts',(91.9214587222691,17.49925882517,62.90882101338));
#137884=CARTESIAN_POINT('Ctrl Pts',(91.7897413843421,17.5095848512144,62.1618148632487));
#137885=CARTESIAN_POINT('Ctrl Pts',(91.6577816154482,17.411296596711,61.4134338249997));
#137886=CARTESIAN_POINT('Ctrl Pts',(91.4039281348835,17.0053502190289,59.9737591958263));
#137887=CARTESIAN_POINT('Ctrl Pts',(91.2820620248445,16.6977362346282,59.2826221415342));
#137888=CARTESIAN_POINT('Ctrl Pts',(91.0581949381514,15.8978221226527,58.0130088027607));
#137889=CARTESIAN_POINT('Ctrl Pts',(90.9562183026917,15.4056089701893,57.4346705640518));
#137890=CARTESIAN_POINT('Ctrl Pts',(90.7803324463945,14.27602564985,56.4371723049057));
#137891=CARTESIAN_POINT('Ctrl Pts',(90.7064423497252,13.638778302204,56.0181207430154));
#137892=CARTESIAN_POINT('Ctrl Pts',(90.6495104561691,12.95468496362,55.69524393663));
#137893=CARTESIAN_POINT('Origin',(59.0011724705691,9.5,68.602980224451));
#137894=CARTESIAN_POINT('',(83.7957739555191,12.95454545455,56.90402403487));
#137895=CARTESIAN_POINT('',(57.7481818513099,12.9545454545505,61.4969173053291));
#137896=CARTESIAN_POINT('',(62.2792373804991,12.95454545455,60.69796996444));
#137897=CARTESIAN_POINT('Ctrl Pts',(83.7957739555191,12.95454545455,56.90402403487));
#137898=CARTESIAN_POINT('Ctrl Pts',(83.0133127087731,13.2847992676121,57.2025428398695));
#137899=CARTESIAN_POINT('Ctrl Pts',(82.217562215713,13.5674612430145,57.5082348281082));
#137900=CARTESIAN_POINT('Ctrl Pts',(81.0003150353501,13.9277132722418,57.9566193292432));
#137901=CARTESIAN_POINT('Ctrl Pts',(80.5906421136752,14.0372001888329,58.1044625659918));
#137902=CARTESIAN_POINT('Ctrl Pts',(79.9698970938941,14.1865988501334,58.3218159564353));
#137903=CARTESIAN_POINT('Ctrl Pts',(79.7619435503995,14.2339265143701,58.3935360164034));
#137904=CARTESIAN_POINT('Ctrl Pts',(79.4484180778543,14.301340535532,58.4998076676419));
#137905=CARTESIAN_POINT('Ctrl Pts',(79.2912566167019,14.3341531242538,58.5526167490743));
#137906=CARTESIAN_POINT('Ctrl Pts',(79.1071963062216,14.3708970404008,58.6136129848518));
#137907=CARTESIAN_POINT('Ctrl Pts',(79.0149889433721,14.388888047566,58.6439524683737));
#137908=CARTESIAN_POINT('Ctrl Pts',(78.9754334348911,14.3965172099578,58.6569205768522));
#137909=CARTESIAN_POINT('Ctrl Pts',(78.9490546261753,14.4015852985292,58.6655582511411));
#137910=CARTESIAN_POINT('Ctrl Pts',(78.9373941718083,14.4038180465107,58.6693724089674));
#137911=CARTESIAN_POINT('Ctrl Pts',(77.9798750059046,14.5863595677044,58.982145272868));
#137912=CARTESIAN_POINT('Ctrl Pts',(77.0389885802272,14.7155633134542,59.2616322996393));
#137913=CARTESIAN_POINT('Ctrl Pts',(75.1580251893373,14.8862983920454,59.7466792551828));
#137914=CARTESIAN_POINT('Ctrl Pts',(74.2194735186116,14.9279095443054,59.9520359248502));
#137915=CARTESIAN_POINT('Ctrl Pts',(72.3362019298778,14.9285030082817,60.2846641550829));
#137916=CARTESIAN_POINT('Ctrl Pts',(71.3813453465866,14.8873352533677,60.4135762102816));
#137917=CARTESIAN_POINT('Ctrl Pts',(69.929932584552,14.7597504534105,60.5548297946571));
#137918=CARTESIAN_POINT('Ctrl Pts',(69.4429550025655,14.7061728352107,60.5933116755178));
#137919=CARTESIAN_POINT('Ctrl Pts',(68.707957642145,14.6081459867842,60.6394292750915));
#137920=CARTESIAN_POINT('Ctrl Pts',(68.4622043899207,14.5725229325201,60.6528734602013));
#137921=CARTESIAN_POINT('Ctrl Pts',(68.0924816871676,14.5144985780408,60.6703648438653));
#137922=CARTESIAN_POINT('Ctrl Pts',(67.9073472349735,14.4843386444438,60.678442409307));
#137923=CARTESIAN_POINT('Ctrl Pts',(67.6908886492797,14.4471035306693,60.6867510899369));
#137924=CARTESIAN_POINT('Ctrl Pts',(67.5825435380976,14.4279686423172,60.6906339004071));
#137925=CARTESIAN_POINT('Ctrl Pts',(67.5360852400895,14.4196565580321,60.6922405669924));
#137926=CARTESIAN_POINT('Ctrl Pts',(67.5051075729281,14.4140903461212,60.6932990127326));
#137927=CARTESIAN_POINT('Ctrl Pts',(67.4880470149196,14.4110104881042,60.6938742152985));
#137928=CARTESIAN_POINT('Ctrl Pts',(66.5829022554768,14.246975254239,60.7240530637672));
#137929=CARTESIAN_POINT('Ctrl Pts',(65.7032005986795,14.0487671761914,60.7324930540725));
#137930=CARTESIAN_POINT('Ctrl Pts',(63.9702005699335,13.5677992372404,60.7259230034294));
#137931=CARTESIAN_POINT('Ctrl Pts',(63.1168951126647,13.2849117826608,60.7108727796349));
#137932=CARTESIAN_POINT('Ctrl Pts',(62.2792373804991,12.95454545455,60.69796996444));
#137933=CARTESIAN_POINT('',(35.8057492453862,12.954533742859,65.3659544670989));
#137934=CARTESIAN_POINT('',(35.8057492437391,12.9545337474,65.365954457758));
#137935=CARTESIAN_POINT('Ctrl Pts',(27.1339043807864,17.4992593326224,74.332577004777));
#137936=CARTESIAN_POINT('Ctrl Pts',(27.1004755498448,17.5013230293304,74.1844849117931));
#137937=CARTESIAN_POINT('Ctrl Pts',(27.0833154043488,17.4990844600161,74.0324117451327));
#137938=CARTESIAN_POINT('Ctrl Pts',(27.0823021127142,17.4923856215589,73.8767964544402));
#137939=CARTESIAN_POINT('Ctrl Pts',(27.0821988672121,17.4917030688602,73.8609406255081));
#137940=CARTESIAN_POINT('Ctrl Pts',(27.0822632579981,17.4909742525328,73.8450480376792));
#137941=CARTESIAN_POINT('Ctrl Pts',(27.0824951578953,17.4901990342879,73.8291191649141));
#137942=CARTESIAN_POINT('Ctrl Pts',(27.083749085873,17.4860072780265,73.7429886428489));
#137943=CARTESIAN_POINT('Ctrl Pts',(27.0898942862776,17.4804584368264,73.6557991836374));
#137944=CARTESIAN_POINT('Ctrl Pts',(27.1008711748689,17.4735341927033,73.5676395575947));
#137945=CARTESIAN_POINT('Ctrl Pts',(27.1063596191646,17.4700720706418,73.5235597445734));
#137946=CARTESIAN_POINT('Ctrl Pts',(27.1130555616134,17.4662661865554,73.4792375515588));
#137947=CARTESIAN_POINT('Ctrl Pts',(27.1209489341839,17.4621148189795,73.4346850580882));
#137948=CARTESIAN_POINT('Ctrl Pts',(27.1248956204691,17.4600391351915,73.4124088113529));
#137949=CARTESIAN_POINT('Ctrl Pts',(27.1291416643071,17.4578770862192,73.3900749896304));
#137950=CARTESIAN_POINT('Ctrl Pts',(27.1336856062651,17.4556284958465,73.3676851765544));
#137951=CARTESIAN_POINT('Ctrl Pts',(27.1359575772442,17.4545042006602,73.3564902700165));
#137952=CARTESIAN_POINT('Ctrl Pts',(27.1383040227537,17.453358270503,73.3452813656432));
#137953=CARTESIAN_POINT('Ctrl Pts',(27.1407247545212,17.4521906857515,73.3340586634897));
#137954=CARTESIAN_POINT('Ctrl Pts',(27.141935120405,17.4516068933757,73.328447312413));
#137955=CARTESIAN_POINT('Ctrl Pts',(27.1431640578532,17.4510176873753,73.3228325118908));
#137956=CARTESIAN_POINT('Ctrl Pts',(27.1444115426407,17.450423065456,73.3172142871795));
#137957=CARTESIAN_POINT('Ctrl Pts',(27.1450352850345,17.4501257544963,73.3144051748238));
#137958=CARTESIAN_POINT('Ctrl Pts',(27.1456636642631,17.4498270895585,73.3115952064208));
#137959=CARTESIAN_POINT('Ctrl Pts',(27.1462966772528,17.4495270703657,73.3087843851438));
#137960=CARTESIAN_POINT('Ctrl Pts',(27.1469296902425,17.4492270511729,73.3059735638669));
#137961=CARTESIAN_POINT('Ctrl Pts',(27.148048434925,17.4486989193247,73.3010551686142));
#137962=CARTESIAN_POINT('Ctrl Pts',(27.1482096144174,17.4486229497522,73.3003493658695));
#137963=CARTESIAN_POINT('Ctrl Pts',(27.150160414395,17.4477034690033,73.2918068400282));
#137964=CARTESIAN_POINT('Ctrl Pts',(27.1531238189679,17.44622437278,73.2781678243283));
#137965=CARTESIAN_POINT('Ctrl Pts',(27.1574605143924,17.4441195119101,73.2594149631964));
#137966=CARTESIAN_POINT('Ctrl Pts',(27.1618294381679,17.44199900867,73.2405227393166));
#137967=CARTESIAN_POINT('Ctrl Pts',(27.1675921197014,17.4392433624406,73.2164402649787));
#137968=CARTESIAN_POINT('Ctrl Pts',(27.175118673911,17.4357324635244,73.1871573227636));
#137969=CARTESIAN_POINT('Ctrl Pts',(27.1798738414059,17.4335143286463,73.1686567857185));
#137970=CARTESIAN_POINT('Ctrl Pts',(27.1853330904777,17.4309936843549,73.1480806187073));
#137971=CARTESIAN_POINT('Ctrl Pts',(27.1915900942525,17.4281297140575,73.1254281615822));
#137972=CARTESIAN_POINT('Ctrl Pts',(27.2017238681702,17.423491259528,73.0887404932591));
#137973=CARTESIAN_POINT('Ctrl Pts',(27.2140254713927,17.4179557691698,73.0466003184545));
#137974=CARTESIAN_POINT('Ctrl Pts',(27.2291892582858,17.4113126615092,72.9990018979463));
#137975=CARTESIAN_POINT('Ctrl Pts',(27.2334716706586,17.4094365782696,72.9855596050448));
#137976=CARTESIAN_POINT('Ctrl Pts',(27.2379823734776,17.4074718479973,72.9716820713348));
#137977=CARTESIAN_POINT('Ctrl Pts',(27.2427370439477,17.405413012191,72.9573693812311));
#137978=CARTESIAN_POINT('Ctrl Pts',(27.2535323926152,17.4007384820595,72.9248728115929));
#137979=CARTESIAN_POINT('Ctrl Pts',(27.2655909865458,17.395579465856,72.8901326364219));
#137980=CARTESIAN_POINT('Ctrl Pts',(27.2791261782035,17.3898672147487,72.8531515151637));
#137981=CARTESIAN_POINT('Ctrl Pts',(27.2858937740323,17.387011089195,72.8346609545345));
#137982=CARTESIAN_POINT('Ctrl Pts',(27.2930307851191,17.3840165437743,72.815610211533));
#137983=CARTESIAN_POINT('Ctrl Pts',(27.3005652978913,17.3808743509666,72.7960000009259));
#137984=CARTESIAN_POINT('Ctrl Pts',(27.3043325542774,17.3793032545628,72.7861948956223));
#137985=CARTESIAN_POINT('Ctrl Pts',(27.3081991863097,17.3776952390278,72.7762499246924));
#137986=CARTESIAN_POINT('Ctrl Pts',(27.3121687931104,17.3760491150648,72.7661652096357));
#137987=CARTESIAN_POINT('Ctrl Pts',(27.3141535965107,17.3752260530833,72.7611228521074));
#137988=CARTESIAN_POINT('Ctrl Pts',(27.3161641436162,17.3743934635576,72.7560455586216));
#137989=CARTESIAN_POINT('Ctrl Pts',(27.3182008861748,17.373551195464,72.7509333458515));
#137990=CARTESIAN_POINT('Ctrl Pts',(27.3202376287334,17.3727089273704,72.7458211330813));
#137991=CARTESIAN_POINT('Ctrl Pts',(27.3230518402653,17.3715471437269,72.7388108924576));
#137992=CARTESIAN_POINT('Ctrl Pts',(27.3243901532579,17.370995202871,72.7354919671642));
#137993=CARTESIAN_POINT('Ctrl Pts',(27.3586789474081,17.3568539769431,72.6504580873365));
#137994=CARTESIAN_POINT('Ctrl Pts',(27.3948271474531,17.3423208187618,72.5695377921547));
#137995=CARTESIAN_POINT('Ctrl Pts',(27.4317540105819,17.327729922424,72.4927918293785));
#137996=CARTESIAN_POINT('Ctrl Pts',(27.4409480584284,17.3240970820556,72.4736836248356));
#137997=CARTESIAN_POINT('Ctrl Pts',(27.4501903682747,17.3204604130413,72.4548341453743));
#137998=CARTESIAN_POINT('Ctrl Pts',(27.4594642451486,17.3168245836903,72.4362442479077));
#137999=CARTESIAN_POINT('Ctrl Pts',(27.4827249273224,17.307705218389,72.3896171789382));
#138000=CARTESIAN_POINT('Ctrl Pts',(27.5061926001715,17.29859169437,72.3446219551981));
#138001=CARTESIAN_POINT('Ctrl Pts',(27.5296499512157,17.2895528123642,72.3012647331953));
#138002=CARTESIAN_POINT('Ctrl Pts',(27.5413786267377,17.2850333713613,72.2795861221939));
#138003=CARTESIAN_POINT('Ctrl Pts',(27.5531052823504,17.2805324687434,72.2583168748899));
#138004=CARTESIAN_POINT('Ctrl Pts',(27.5648031624215,17.276058236252,72.2374584671607));
#138005=CARTESIAN_POINT('Ctrl Pts',(27.570652102457,17.2738211200063,72.2270292632961));
#138006=CARTESIAN_POINT('Ctrl Pts',(27.5764938488926,17.2715906652919,72.2167027709439));
#138007=CARTESIAN_POINT('Ctrl Pts',(27.5823252955446,17.2693678466743,72.2064791177919));
#138008=CARTESIAN_POINT('Ctrl Pts',(27.5878485743336,17.267262494837,72.19679574247));
#138009=CARTESIAN_POINT('Ctrl Pts',(27.5925029488425,17.2654901196184,72.1886875932158));
#138010=CARTESIAN_POINT('Ctrl Pts',(27.5987284984472,17.2631248903857,72.1779409680902));
#138011=CARTESIAN_POINT('Ctrl Pts',(27.5990758490682,17.2629929239097,72.1773413669067));
#138012=CARTESIAN_POINT('Ctrl Pts',(27.599428091347,17.262859098644,72.1767335553565));
#138013=CARTESIAN_POINT('Ctrl Pts',(27.5997856493164,17.2627232487334,72.1761168028097));
#138014=CARTESIAN_POINT('Ctrl Pts',(27.6731296190087,17.2348570771554,72.0496056242957));
#138015=CARTESIAN_POINT('Ctrl Pts',(27.7532636202495,17.2048468369855,71.9236412018619));
#138016=CARTESIAN_POINT('Ctrl Pts',(27.8389310916625,17.1729569092371,71.7987901761038));
#138017=CARTESIAN_POINT('Ctrl Pts',(27.8797101576983,17.1577768012208,71.7393591208848));
#138018=CARTESIAN_POINT('Ctrl Pts',(27.9217429902264,17.1421714406541,71.6801799654615));
#138019=CARTESIAN_POINT('Ctrl Pts',(27.9648936660156,17.1261728112818,71.6213116197419));
#138020=CARTESIAN_POINT('Ctrl Pts',(28.0317938438829,17.1013687698372,71.5300429958473));
#138021=CARTESIAN_POINT('Ctrl Pts',(28.1013819438649,17.0756201944387,71.4395217235677));
#138022=CARTESIAN_POINT('Ctrl Pts',(28.1733653960537,17.0490115864612,71.3498049863921));
#138023=CARTESIAN_POINT('Ctrl Pts',(28.209357122148,17.0357072824725,71.3049466178042));
#138024=CARTESIAN_POINT('Ctrl Pts',(28.2459476825176,17.0221879445018,71.2602893615747));
#138025=CARTESIAN_POINT('Ctrl Pts',(28.2831003535614,17.008463870423,71.2158399693841));
#138026=CARTESIAN_POINT('Ctrl Pts',(28.3016766890833,17.0016018333835,71.1936152732888));
#138027=CARTESIAN_POINT('Ctrl Pts',(28.3203935521594,16.9946886107542,71.1714425425548));
#138028=CARTESIAN_POINT('Ctrl Pts',(28.3392463464684,16.9877254772434,71.1493226090831));
#138029=CARTESIAN_POINT('Ctrl Pts',(28.3486727436229,16.9842439104881,71.1382626423472));
#138030=CARTESIAN_POINT('Ctrl Pts',(28.3581331235798,16.9807498659209,71.1272158748941));
#138031=CARTESIAN_POINT('Ctrl Pts',(28.3676269112532,16.977243501931,71.1161824095321));
#138032=CARTESIAN_POINT('Ctrl Pts',(28.3759339754674,16.9741754334398,71.1065281273403));
#138033=CARTESIAN_POINT('Ctrl Pts',(28.384266617464,16.9710979328851,71.0968840295599));
#138034=CARTESIAN_POINT('Ctrl Pts',(28.3926244517788,16.9680111060067,71.0872501846531));
#138035=CARTESIAN_POINT('Ctrl Pts',(28.3938184281095,16.9675701307383,71.085873921095));
#138036=CARTESIAN_POINT('Ctrl Pts',(28.396011528671,16.9667601442857,71.0833481357132));
#138037=CARTESIAN_POINT('Ctrl Pts',(28.3962079220283,16.9666876095051,71.0831220218952));
#138038=CARTESIAN_POINT('Ctrl Pts',(28.4028245292768,16.9642438702571,71.0755041149173));
#138039=CARTESIAN_POINT('Ctrl Pts',(28.4139881583462,16.9600125484294,71.0623773395018));
#138040=CARTESIAN_POINT('Ctrl Pts',(28.4298813084446,16.953960153376,71.0438049802813));
#138041=CARTESIAN_POINT('Ctrl Pts',(28.4459334925285,16.9478471953442,71.0250467777077));
#138042=CARTESIAN_POINT('Ctrl Pts',(28.4668103103473,16.9398763984077,71.0007333945629));
#138043=CARTESIAN_POINT('Ctrl Pts',(28.4927033905768,16.9299635737908,70.9709504280054));
#138044=CARTESIAN_POINT('Ctrl Pts',(28.519012725448,16.9198913915686,70.9406886733715));
#138045=CARTESIAN_POINT('Ctrl Pts',(28.5505008736301,16.9078141092849,70.9047799095888));
#138046=CARTESIAN_POINT('Ctrl Pts',(28.5873728555423,16.8935943466494,70.8633366170196));
#138047=CARTESIAN_POINT('Ctrl Pts',(28.6147878724832,16.8830216837946,70.8325227440203));
#138048=CARTESIAN_POINT('Ctrl Pts',(28.6451792624566,16.8712635678662,70.7986497232713));
#138049=CARTESIAN_POINT('Ctrl Pts',(28.6786328453021,16.858247180522,70.7617725771743));
#138050=CARTESIAN_POINT('Ctrl Pts',(28.7254438564832,16.8400335782205,70.7101710340379));
#138051=CARTESIAN_POINT('Ctrl Pts',(28.7783196309919,16.8193690026626,70.6527006291921));
#138052=CARTESIAN_POINT('Ctrl Pts',(28.8376378439644,16.7960271061273,70.5895420513129));
#138053=CARTESIAN_POINT('Ctrl Pts',(28.8838583335065,16.7778392034472,70.5403291663984));
#138054=CARTESIAN_POINT('Ctrl Pts',(28.9339904209272,16.7580247761307,70.4876632911371));
#138055=CARTESIAN_POINT('Ctrl Pts',(28.9882152012452,16.7364598942736,70.4316436451738));
#138056=CARTESIAN_POINT('Ctrl Pts',(29.0501229505528,16.7118395400364,70.367686720346));
#138057=CARTESIAN_POINT('Ctrl Pts',(29.1173684817007,16.6849368572625,70.2993549323575));
#138058=CARTESIAN_POINT('Ctrl Pts',(29.1902208716677,16.6555381225991,70.22679954364));
#138059=CARTESIAN_POINT('Ctrl Pts',(29.2266470666512,16.6408387552674,70.1905218492813));
#138060=CARTESIAN_POINT('Ctrl Pts',(29.2644748191839,16.6255149672994,70.1531884917144));
#138061=CARTESIAN_POINT('Ctrl Pts',(29.3037357471969,16.6095371671074,70.114819153979));
#138062=CARTESIAN_POINT('Ctrl Pts',(29.3233662112033,16.6015482670114,70.0956344851113));
#138063=CARTESIAN_POINT('Ctrl Pts',(29.3433549711418,16.5933958376689,70.0761908328954));
#138064=CARTESIAN_POINT('Ctrl Pts',(29.3637057369433,16.5850759688277,70.0564906734208));
#138065=CARTESIAN_POINT('Ctrl Pts',(29.373881119844,16.5809160344071,70.0466405936834));
#138066=CARTESIAN_POINT('Ctrl Pts',(29.3841470043436,16.5767142384171,70.0367263878862));
#138067=CARTESIAN_POINT('Ctrl Pts',(29.3945038436147,16.5724700796614,70.0267483679313));
#138068=CARTESIAN_POINT('Ctrl Pts',(29.3996822632502,16.5703480002836,70.0217593579538));
#138069=CARTESIAN_POINT('Ctrl Pts',(29.4048834215875,16.568215330108,70.0167543944867));
#138070=CARTESIAN_POINT('Ctrl Pts',(29.410107374287,16.566072005633,70.0117335165982));
#138071=CARTESIAN_POINT('Ctrl Pts',(29.4127193506368,16.5650003433955,70.009223077654));
#138072=CARTESIAN_POINT('Ctrl Pts',(29.4153370255777,16.5639260175764,70.0067086601076));
#138073=CARTESIAN_POINT('Ctrl Pts',(29.4179604059968,16.5628490201828,70.0041902688462));
#138074=CARTESIAN_POINT('Ctrl Pts',(29.4205837864159,16.5617720227891,70.0016718775848));
#138075=CARTESIAN_POINT('Ctrl Pts',(29.424205760984,16.560284485163,69.9981974973265));
#138076=CARTESIAN_POINT('Ctrl Pts',(29.4258476705543,16.5596100052536,69.9966231788122));
#138077=CARTESIAN_POINT('Ctrl Pts',(29.5731714058286,16.4990908990772,69.855364190961));
#138078=CARTESIAN_POINT('Ctrl Pts',(29.7237179933999,16.4362228320212,69.7157522642118));
#138079=CARTESIAN_POINT('Ctrl Pts',(29.8768576760397,16.3710141156729,69.5777144562597));
#138080=CARTESIAN_POINT('Ctrl Pts',(30.0311166199704,16.3053288044226,69.4386677630046));
#138081=CARTESIAN_POINT('Ctrl Pts',(30.188006633286,16.2372682938278,69.3012178920274));
#138082=CARTESIAN_POINT('Ctrl Pts',(30.3468876316625,16.1667922714889,69.1653106062159));
#138083=CARTESIAN_POINT('Ctrl Pts',(30.4802922276503,16.1076170058309,69.0511959119431));
#138084=CARTESIAN_POINT('Ctrl Pts',(30.6151005391363,16.0467378435994,68.9381690077916));
#138085=CARTESIAN_POINT('Ctrl Pts',(30.7509361135523,15.984106325019,68.8262117122634));
#138086=CARTESIAN_POINT('Ctrl Pts',(30.9800432215038,15.8784688574391,68.6373789097902));
#138087=CARTESIAN_POINT('Ctrl Pts',(31.2122750465286,15.7680432382575,68.4518448887416));
#138088=CARTESIAN_POINT('Ctrl Pts',(31.4463514062206,15.6531308717712,68.2701385686671));
#138089=CARTESIAN_POINT('Ctrl Pts',(31.5633895860667,15.5956746885281,68.1792854086299));
#138090=CARTESIAN_POINT('Ctrl Pts',(31.6808886741266,15.537097401388,68.0893890476009));
#138091=CARTESIAN_POINT('Ctrl Pts',(31.798687387191,15.4774338689085,68.0005085340514));
#138092=CARTESIAN_POINT('Ctrl Pts',(31.8575867437232,15.4476021026688,67.9560682772767));
#138093=CARTESIAN_POINT('Ctrl Pts',(31.9165610000085,15.4174982654751,67.9118813578827));
#138094=CARTESIAN_POINT('Ctrl Pts',(31.9755899880513,15.3871250965545,67.8679533533156));
#138095=CARTESIAN_POINT('Ctrl Pts',(32.0051044820726,15.3719385120942,67.845989351032));
#138096=CARTESIAN_POINT('Ctrl Pts',(32.034632659388,15.3566845944791,67.8240900794668));
#138097=CARTESIAN_POINT('Ctrl Pts',(32.06417199853,15.3413636826288,67.8022562455776));
#138098=CARTESIAN_POINT('Ctrl Pts',(32.0900189202792,15.3279578847597,67.7831516409246));
#138099=CARTESIAN_POINT('Ctrl Pts',(32.1158743878235,15.3145007944122,67.7640971371143));
#138100=CARTESIAN_POINT('Ctrl Pts',(32.1417367124484,15.3009926380724,67.7450932124781));
#138101=CARTESIAN_POINT('Ctrl Pts',(32.145431330252,15.2990629014524,67.7423783661015));
#138102=CARTESIAN_POINT('Ctrl Pts',(32.1479130755241,15.2977663283766,67.7405551425058));
#138103=CARTESIAN_POINT('Ctrl Pts',(32.1528209807404,15.2952003023608,67.7369517714385));
#138104=CARTESIAN_POINT('Ctrl Pts',(32.3674042552043,15.1830085951946,67.5794052972008));
#138105=CARTESIAN_POINT('Ctrl Pts',(32.5818793710549,15.0673300016252,67.4254656364288));
#138106=CARTESIAN_POINT('Ctrl Pts',(32.795626850551,14.9481755404271,67.2752501948076));
#138107=CARTESIAN_POINT('Ctrl Pts',(33.0082233998999,14.8296626702406,67.1258435930415));
#138108=CARTESIAN_POINT('Ctrl Pts',(33.2201000592884,14.7077107704291,66.9801208237245));
#138109=CARTESIAN_POINT('Ctrl Pts',(33.4306541547144,14.5822979782621,66.8382362586377));
#138110=CARTESIAN_POINT('Ctrl Pts',(33.6281592547383,14.4646575875059,66.7051449256829));
#138111=CARTESIAN_POINT('Ctrl Pts',(33.8245006551659,14.3439713652497,66.5754308735912));
#138112=CARTESIAN_POINT('Ctrl Pts',(34.0191872456239,14.2202007978378,66.4492573184544));
#138113=CARTESIAN_POINT('Ctrl Pts',(34.1910295959593,14.1109532879997,66.3378887839607));
#138114=CARTESIAN_POINT('Ctrl Pts',(34.3617795191168,13.9992396404704,66.2291951224791));
#138115=CARTESIAN_POINT('Ctrl Pts',(34.5313274049966,13.884910999406,66.1232213719099));
#138116=CARTESIAN_POINT('Ctrl Pts',(34.6992531288876,13.771676206105,66.0182615330689));
#138117=CARTESIAN_POINT('Ctrl Pts',(34.8659996684362,13.6558758152753,65.9159695916096));
#138118=CARTESIAN_POINT('Ctrl Pts',(35.0314688615146,13.5373489443009,65.8164365574236));
#138119=CARTESIAN_POINT('Ctrl Pts',(35.1940003305946,13.420926387893,65.7186706230687));
#138120=CARTESIAN_POINT('Ctrl Pts',(35.355299383326,13.3018728903959,65.6235663722552));
#138121=CARTESIAN_POINT('Ctrl Pts',(35.5152815034465,13.1800262567294,65.5312583148745));
#138122=CARTESIAN_POINT('Ctrl Pts',(35.6125969994222,13.1059081891647,65.4751082627324));
#138123=CARTESIAN_POINT('Ctrl Pts',(35.7094253755256,13.0307564497627,65.41999379509));
#138124=CARTESIAN_POINT('Ctrl Pts',(35.8057492503273,12.9545337292362,65.3659544951215));
#138125=CARTESIAN_POINT('Ctrl Pts',(27.3191400010791,17.49826943671,74.421637315687));
#138126=CARTESIAN_POINT('Ctrl Pts',(26.9498075064491,17.49016994831,74.507602053806));
#138127=CARTESIAN_POINT('Ctrl Pts',(26.4148506048091,17.51742193092,74.633280388995));
#138128=CARTESIAN_POINT('Ctrl Pts',(25.7230268640091,17.62730114969,74.798040434501));
#138129=CARTESIAN_POINT('Ctrl Pts',(25.2463297175291,17.7348343146,74.912517844996));
#138130=CARTESIAN_POINT('Ctrl Pts',(24.7773466811991,17.87289212671,75.026106644434));
#138131=CARTESIAN_POINT('Ctrl Pts',(24.1186923675691,18.11371974695,75.187036750685));
#138132=CARTESIAN_POINT('Ctrl Pts',(23.6367652953191,18.35052078424,75.30659770678));
#138133=CARTESIAN_POINT('Ctrl Pts',(23.3168213892291,18.53758431057,75.386865081271));
#138134=CARTESIAN_POINT('Ctrl Pts',(27.1799956085391,17.51200319618,73.9592992548583));
#138135=CARTESIAN_POINT('Ctrl Pts',(26.8048647613891,17.50670814829,74.002495728156));
#138136=CARTESIAN_POINT('Ctrl Pts',(26.2612602759991,17.53721130111,74.06386792449));
#138137=CARTESIAN_POINT('Ctrl Pts',(25.5574177012091,17.64971366655,74.141020185911));
#138138=CARTESIAN_POINT('Ctrl Pts',(25.0720160815391,17.7583874709,74.193250720675));
#138139=CARTESIAN_POINT('Ctrl Pts',(24.5939754596591,17.89690459352,74.243706306264));
#138140=CARTESIAN_POINT('Ctrl Pts',(23.9217915560591,18.1374439731,74.313235070235));
#138141=CARTESIAN_POINT('Ctrl Pts',(23.4288088080691,18.37287922197,74.362412782871));
#138142=CARTESIAN_POINT('Ctrl Pts',(23.1008469738591,18.55854189444,74.394250202332));
#138143=CARTESIAN_POINT('Ctrl Pts',(27.2466786265891,17.46814185615,73.2575872353228));
#138144=CARTESIAN_POINT('Ctrl Pts',(26.8556174534391,17.45360018152,73.2420308847567));
#138145=CARTESIAN_POINT('Ctrl Pts',(26.2878069083791,17.47344346426,73.2150078795167));
#138146=CARTESIAN_POINT('Ctrl Pts',(25.5515499179291,17.57740259896,73.1712133705486));
#138147=CARTESIAN_POINT('Ctrl Pts',(25.0435347167691,17.68239329966,73.1372119678006));
#138148=CARTESIAN_POINT('Ctrl Pts',(24.5431543670891,17.81947498135,73.0998283922469));
#138149=CARTESIAN_POINT('Ctrl Pts',(23.8397272546891,18.06108459844,73.0415257181794));
#138150=CARTESIAN_POINT('Ctrl Pts',(23.3243855329991,18.30113729463,72.9912760097607));
#138151=CARTESIAN_POINT('Ctrl Pts',(22.9821563396191,18.4915383548,72.9540702371875));
#138152=CARTESIAN_POINT('Ctrl Pts',(27.6908059692291,17.31239362199,72.32988049079));
#138153=CARTESIAN_POINT('Ctrl Pts',(27.2686542733791,17.26783708843,72.2493782757269));
#138154=CARTESIAN_POINT('Ctrl Pts',(26.6529460569991,17.25236955023,72.1211498844787));
#138155=CARTESIAN_POINT('Ctrl Pts',(25.8538764569291,17.32739312776,71.933840809013));
#138156=CARTESIAN_POINT('Ctrl Pts',(25.3030891218091,17.41958132242,71.795811473092));
#138157=CARTESIAN_POINT('Ctrl Pts',(24.7620003303291,17.5512068623,71.651135627332));
#138158=CARTESIAN_POINT('Ctrl Pts',(24.0045728644791,17.79520593481,71.435364902963));
#138159=CARTESIAN_POINT('Ctrl Pts',(23.4552604763591,18.04938472156,71.261698407729));
#138160=CARTESIAN_POINT('Ctrl Pts',(23.0945336287391,18.25428407142,71.13914291643));
#138161=CARTESIAN_POINT('Ctrl Pts',(28.1400244369891,17.16084343501,71.67068573287));
#138162=CARTESIAN_POINT('Ctrl Pts',(27.6924228005891,17.08797999477,71.550588326742));
#138163=CARTESIAN_POINT('Ctrl Pts',(27.0368869496491,17.03881028412,71.358054994454));
#138164=CARTESIAN_POINT('Ctrl Pts',(26.1855308687891,17.08595396583,71.075775732564));
#138165=CARTESIAN_POINT('Ctrl Pts',(25.5993319865391,17.1657036723,70.867651396577));
#138166=CARTESIAN_POINT('Ctrl Pts',(25.0249494825691,17.29190890746,70.649703725504));
#138167=CARTESIAN_POINT('Ctrl Pts',(24.2242629266291,17.53789465026,70.325403445397));
#138168=CARTESIAN_POINT('Ctrl Pts',(23.6493371619591,17.80529216506,70.065939095621));
#138169=CARTESIAN_POINT('Ctrl Pts',(23.2759003039191,18.02368015424,69.884235493212));
#138170=CARTESIAN_POINT('Ctrl Pts',(28.6742783680191,16.97751618649,71.032681520933));
#138171=CARTESIAN_POINT('Ctrl Pts',(28.1995866711491,16.87164529692,70.881260223481));
#138172=CARTESIAN_POINT('Ctrl Pts',(27.5009153879891,16.7825926448,70.634282550969));
#138173=CARTESIAN_POINT('Ctrl Pts',(26.5927471971891,16.79636360817,70.266373192438));
#138174=CARTESIAN_POINT('Ctrl Pts',(25.9682367963491,16.86108071599,69.993353846621));
#138175=CARTESIAN_POINT('Ctrl Pts',(25.3582383912691,16.98057465604,69.7062492802));
#138176=CARTESIAN_POINT('Ctrl Pts',(24.5122060337491,17.22851317371,69.278160128787));
#138177=CARTESIAN_POINT('Ctrl Pts',(23.9121159264291,17.51120598981,68.935601892025));
#138178=CARTESIAN_POINT('Ctrl Pts',(23.5275237426991,17.74508268167,68.696786815993));
#138179=CARTESIAN_POINT('Ctrl Pts',(29.4637252782291,16.69573371735,70.214944809297));
#138180=CARTESIAN_POINT('Ctrl Pts',(28.9514579649091,16.54179580496,70.032096099575));
#138181=CARTESIAN_POINT('Ctrl Pts',(28.1919676268391,16.39358977803,69.724912954889));
#138182=CARTESIAN_POINT('Ctrl Pts',(27.2035620142491,16.3570658,69.254403728281));
#138183=CARTESIAN_POINT('Ctrl Pts',(26.5252463207491,16.39879570663,68.901220520825));
#138184=CARTESIAN_POINT('Ctrl Pts',(25.8658896109391,16.50762402452,68.526884021015));
#138185=CARTESIAN_POINT('Ctrl Pts',(24.9584926272791,16.75742057013,67.966148168991));
#138186=CARTESIAN_POINT('Ctrl Pts',(24.3270071090491,17.06184500929,67.516248000898));
#138187=CARTESIAN_POINT('Ctrl Pts',(23.9306200607191,17.31759555138,67.204119706507));
#138188=CARTESIAN_POINT('Ctrl Pts',(30.5643228338091,16.27458129194,69.243614535439));
#138189=CARTESIAN_POINT('Ctrl Pts',(30.0032041656191,16.05501205067,69.039943888873));
#138190=CARTESIAN_POINT('Ctrl Pts',(29.1623979624891,15.82351514044,68.679348902864));
#138191=CARTESIAN_POINT('Ctrl Pts',(28.0660514701691,15.71423060732,68.099666962869));
#138192=CARTESIAN_POINT('Ctrl Pts',(27.3158303509791,15.72189536398,67.65602497559));
#138193=CARTESIAN_POINT('Ctrl Pts',(26.5917298473491,15.81393917483,67.179483204152));
#138194=CARTESIAN_POINT('Ctrl Pts',(25.6066793437291,16.06376175979,66.459804783254));
#138195=CARTESIAN_POINT('Ctrl Pts',(24.9407056051391,16.39642789448,65.879059404692));
#138196=CARTESIAN_POINT('Ctrl Pts',(24.5357382278291,16.68036788396,65.478569084817));
#138197=CARTESIAN_POINT('Ctrl Pts',(31.9721783881791,15.65771573836,68.134435860703));
#138198=CARTESIAN_POINT('Ctrl Pts',(31.3495795968991,15.35736259841,67.934796110749));
#138199=CARTESIAN_POINT('Ctrl Pts',(30.4027791865191,15.01732558252,67.544277564079));
#138200=CARTESIAN_POINT('Ctrl Pts',(29.1653871408091,14.80802142551,66.859150797452));
#138201=CARTESIAN_POINT('Ctrl Pts',(28.3226115049791,14.76665268063,66.317249241228));
#138202=CARTESIAN_POINT('Ctrl Pts',(27.5181196124491,14.83186560328,65.721961974247));
#138203=CARTESIAN_POINT('Ctrl Pts',(26.4431662662991,15.07435073545,64.810545576925));
#138204=CARTESIAN_POINT('Ctrl Pts',(25.7491319290091,15.43721005654,64.067609764873));
#138205=CARTESIAN_POINT('Ctrl Pts',(25.3476825194191,15.75121540699,63.559397667783));
#138206=CARTESIAN_POINT('Ctrl Pts',(33.9349740065291,14.66621205402,66.73160281835));
#138207=CARTESIAN_POINT('Ctrl Pts',(33.2278434897891,14.26458094051,66.575078838193));
#138208=CARTESIAN_POINT('Ctrl Pts',(32.1291768053591,13.77747533735,66.191659990382));
#138209=CARTESIAN_POINT('Ctrl Pts',(30.6880826567591,13.42159104386,65.400693368417));
#138210=CARTESIAN_POINT('Ctrl Pts',(29.7134712804291,13.30352866128,64.740908745675));
#138211=CARTESIAN_POINT('Ctrl Pts',(28.7987684121191,13.32093273385,63.990845152437));
#138212=CARTESIAN_POINT('Ctrl Pts',(27.6104240691691,13.53598846397,62.81924348911));
#138213=CARTESIAN_POINT('Ctrl Pts',(26.8996906205291,13.92434475631,61.85109790423));
#138214=CARTESIAN_POINT('Ctrl Pts',(26.5224611273491,14.26533563258,61.1967983039));
#138215=CARTESIAN_POINT('Ctrl Pts',(35.3622032127791,13.75469237915,65.830333025965));
#138216=CARTESIAN_POINT('Ctrl Pts',(34.5908441824791,13.30161722205,65.748234026521));
#138217=CARTESIAN_POINT('Ctrl Pts',(33.3708021106091,12.72238358321,65.428350962473));
#138218=CARTESIAN_POINT('Ctrl Pts',(31.7667737502791,12.25520144588,64.605780509743));
#138219=CARTESIAN_POINT('Ctrl Pts',(30.6899215020291,12.0705356095,63.877833376471));
#138220=CARTESIAN_POINT('Ctrl Pts',(29.6962823484591,12.03664559044,63.02007166273));
#138221=CARTESIAN_POINT('Ctrl Pts',(28.4414020511891,12.20135845414,61.65313517891));
#138222=CARTESIAN_POINT('Ctrl Pts',(27.7497515268791,12.5766773768,60.50898741333));
#138223=CARTESIAN_POINT('Ctrl Pts',(27.4156275891691,12.91072398446,59.74451354692));
#138224=CARTESIAN_POINT('Ctrl Pts',(36.2861062865691,13.03336630118,65.305951484901));
#138225=CARTESIAN_POINT('Ctrl Pts',(35.4712170914491,12.56970047636,65.286339892556));
#138226=CARTESIAN_POINT('Ctrl Pts',(34.1668107446491,11.95485361461,65.031531154156));
#138227=CARTESIAN_POINT('Ctrl Pts',(32.4498758951991,11.42267707437,64.209981525113));
#138228=CARTESIAN_POINT('Ctrl Pts',(31.3039856908491,11.18982977636,63.447072574633));
#138229=CARTESIAN_POINT('Ctrl Pts',(30.2605887651091,11.10856325397,62.52302045754));
#138230=CARTESIAN_POINT('Ctrl Pts',(28.9718152012291,11.20940972601,61.02865012207));
#138231=CARTESIAN_POINT('Ctrl Pts',(28.3078068268491,11.54159885331,59.76710225));
#138232=CARTESIAN_POINT('Ctrl Pts',(28.0119699420191,11.84565233006,58.93127622062));
#138233=CARTESIAN_POINT('Ctrl Pts',(35.8057492437391,12.9545337474,65.365954457758));
#138234=CARTESIAN_POINT('Ctrl Pts',(35.0880473119254,12.5659947139585,65.3035861089168));
#138235=CARTESIAN_POINT('Ctrl Pts',(33.9193435259554,12.0333674552047,65.0326040360676));
#138236=CARTESIAN_POINT('Ctrl Pts',(32.3449940438637,11.5497171457426,64.2716514600773));
#138237=CARTESIAN_POINT('Ctrl Pts',(31.20966790579,11.3242173664052,63.5141788914939));
#138238=CARTESIAN_POINT('Ctrl Pts',(30.1739125038161,11.2501013629597,62.6003206815515));
#138239=CARTESIAN_POINT('Ctrl Pts',(28.9865858783025,11.3522173259346,61.2359961916097));
#138240=CARTESIAN_POINT('Ctrl Pts',(28.3556953002107,11.6353649591875,60.1235372995198));
#138241=CARTESIAN_POINT('Ctrl Pts',(28.0568193741291,11.88244542754,59.40530601881));
#138242=CARTESIAN_POINT('Ctrl Pts',(23.3999522633791,18.46444455386,75.10151114459));
#138243=CARTESIAN_POINT('Ctrl Pts',(23.6808182067591,18.30904759158,75.042523107842));
#138244=CARTESIAN_POINT('Ctrl Pts',(24.1204792021491,18.10012856,74.950661190046));
#138245=CARTESIAN_POINT('Ctrl Pts',(24.7331798418691,17.87739478943,74.823594240219));
#138246=CARTESIAN_POINT('Ctrl Pts',(25.2046454214491,17.73925026023,74.726279248655));
#138247=CARTESIAN_POINT('Ctrl Pts',(25.6837459162591,17.63150329689,74.62784130659));
#138248=CARTESIAN_POINT('Ctrl Pts',(26.3276494863891,17.52927130737,74.496133232865));
#138249=CARTESIAN_POINT('Ctrl Pts',(26.8131230416891,17.49914820964,74.397483178755));
#138250=CARTESIAN_POINT('Ctrl Pts',(27.1339043807891,17.4992593337,74.332577004792));
#138251=CARTESIAN_POINT('Ctrl Pts',(45.5703178693691,0.707960234922114,
89.0822394094));
#138252=CARTESIAN_POINT('Ctrl Pts',(44.5186432780591,0.659835674446814,
89.20897170224));
#138253=CARTESIAN_POINT('Ctrl Pts',(42.8940207028191,0.604436397099514,
89.73263017053));
#138254=CARTESIAN_POINT('Ctrl Pts',(41.0311875536291,0.588130384116814,
91.15056935081));
#138255=CARTESIAN_POINT('Ctrl Pts',(39.9406430951691,0.603176446704114,
92.40648659842));
#138256=CARTESIAN_POINT('Ctrl Pts',(39.1329334447691,0.644538603476814,
93.85993788124));
#138257=CARTESIAN_POINT('Ctrl Pts',(38.4383242748091,0.736745229573714,
96.09055788542));
#138258=CARTESIAN_POINT('Ctrl Pts',(38.5013499324291,0.838281509416614,
97.79112213109));
#138259=CARTESIAN_POINT('Ctrl Pts',(38.7409464403291,0.910299463671814,
98.81933316041));
#138260=CARTESIAN_POINT('Ctrl Pts',(45.4721796702991,2.06232273559201,89.00677780565));
#138261=CARTESIAN_POINT('Ctrl Pts',(44.4284729920291,1.94009833564701,89.1407783658));
#138262=CARTESIAN_POINT('Ctrl Pts',(42.8175742166591,1.79034687547301,89.67184802681));
#138263=CARTESIAN_POINT('Ctrl Pts',(40.9686565618091,1.71580235048201,91.08770003869));
#138264=CARTESIAN_POINT('Ctrl Pts',(39.8842055812591,1.72275806456501,92.33729386425));
#138265=CARTESIAN_POINT('Ctrl Pts',(39.0776934503791,1.79009011946901,93.78055230646));
#138266=CARTESIAN_POINT('Ctrl Pts',(38.3772852098791,1.96457065015301,95.99347428737));
#138267=CARTESIAN_POINT('Ctrl Pts',(38.4275709545191,2.17502790110001,97.68027461616));
#138268=CARTESIAN_POINT('Ctrl Pts',(38.6573676897591,2.32868442717401,98.70126826354));
#138269=CARTESIAN_POINT('Ctrl Pts',(44.8750464017491,4.56348845765001,88.64530949828));
#138270=CARTESIAN_POINT('Ctrl Pts',(43.8784111675091,4.31519214834701,88.82035926586));
#138271=CARTESIAN_POINT('Ctrl Pts',(42.3489435586691,4.00766266409601,89.39434894904));
#138272=CARTESIAN_POINT('Ctrl Pts',(40.5839167302391,3.83775650537201,90.80141261252));
#138273=CARTESIAN_POINT('Ctrl Pts',(39.5371780607291,3.83261063261101,92.01797786687));
#138274=CARTESIAN_POINT('Ctrl Pts',(38.7399707710991,3.94455189574301,93.40690693377));
#138275=CARTESIAN_POINT('Ctrl Pts',(38.0091199376791,4.25844260235601,95.52524061768));
#138276=CARTESIAN_POINT('Ctrl Pts',(37.9876278087191,4.65417059800001,97.13918259124));
#138277=CARTESIAN_POINT('Ctrl Pts',(38.1619562805791,4.94855385665801,98.1228027417));
#138278=CARTESIAN_POINT('Ctrl Pts',(43.0040757822791,7.92565778104501,87.57336120223));
#138279=CARTESIAN_POINT('Ctrl Pts',(42.1314449640691,7.58314091906501,87.84274208492));
#138280=CARTESIAN_POINT('Ctrl Pts',(40.8109212819391,7.17442879063501,88.50086965325));
#138281=CARTESIAN_POINT('Ctrl Pts',(39.2628767731891,6.95638763849201,89.85599220205));
#138282=CARTESIAN_POINT('Ctrl Pts',(38.3185027453891,6.95368779388401,90.97257180576));
#138283=CARTESIAN_POINT('Ctrl Pts',(37.5569107613691,7.10414768348401,92.21235388849));
#138284=CARTESIAN_POINT('Ctrl Pts',(36.7719385589291,7.52355677267901,94.07900873911));
#138285=CARTESIAN_POINT('Ctrl Pts',(36.5857472469691,8.06070624920501,95.50005965187));
#138286=CARTESIAN_POINT('Ctrl Pts',(36.6231609183791,8.47348086431201,96.38244933991));
#138287=CARTESIAN_POINT('Ctrl Pts',(40.5611902232291,10.69087199582,86.169912153));
#138288=CARTESIAN_POINT('Ctrl Pts',(39.8202100664191,10.3459022151,86.51638878304));
#138289=CARTESIAN_POINT('Ctrl Pts',(38.7145503345591,9.95494845055102,87.21990143235));
#138290=CARTESIAN_POINT('Ctrl Pts',(37.3925003291091,9.76608299487901,88.47454628703));
#138291=CARTESIAN_POINT('Ctrl Pts',(36.5609603027891,9.78111156877201,89.46176171597));
#138292=CARTESIAN_POINT('Ctrl Pts',(35.8513385718791,9.94505616679701,90.52793264081));
#138293=CARTESIAN_POINT('Ctrl Pts',(35.0423804786691,10.38071351751,92.11239180277));
#138294=CARTESIAN_POINT('Ctrl Pts',(34.7147333582191,10.93606492626,93.31812773795));
#138295=CARTESIAN_POINT('Ctrl Pts',(34.6211328961591,11.37571793371,94.08326873557));
#138296=CARTESIAN_POINT('Ctrl Pts',(37.6648628651591,13.01212937041,84.45051386252));
#138297=CARTESIAN_POINT('Ctrl Pts',(37.0485114028091,12.72504052521,84.83528003923));
#138298=CARTESIAN_POINT('Ctrl Pts',(36.1397513800491,12.42041285003,85.52537905717));
#138299=CARTESIAN_POINT('Ctrl Pts',(35.0291247089391,12.30120930116,86.62813233824));
#138300=CARTESIAN_POINT('Ctrl Pts',(34.3098104197691,12.34107474934,87.46222226458));
#138301=CARTESIAN_POINT('Ctrl Pts',(33.6646869438991,12.5044895076,88.34115329029));
#138302=CARTESIAN_POINT('Ctrl Pts',(32.8688746226891,12.90715384858,89.63210632856));
#138303=CARTESIAN_POINT('Ctrl Pts',(32.4461188939691,13.40839785764,90.61443544277));
#138304=CARTESIAN_POINT('Ctrl Pts',(32.2490596322791,13.81460990432,91.25188364405));
#138305=CARTESIAN_POINT('Ctrl Pts',(34.6138161202091,14.83524066691,82.512754421903));
#138306=CARTESIAN_POINT('Ctrl Pts',(34.1021116145691,14.63448763363,82.887519522589));
#138307=CARTESIAN_POINT('Ctrl Pts',(33.3541271725091,14.44059566195,83.5053711923));
#138308=CARTESIAN_POINT('Ctrl Pts',(32.4209056113491,14.40140301801,84.41848947981));
#138309=CARTESIAN_POINT('Ctrl Pts',(31.8014684235891,14.46612570875,85.08838789903));
#138310=CARTESIAN_POINT('Ctrl Pts',(31.2239907584391,14.6225382638,85.78068774631));
#138311=CARTESIAN_POINT('Ctrl Pts',(30.4702465367691,14.97297661061,86.78797330942));
#138312=CARTESIAN_POINT('Ctrl Pts',(30.0032175967391,15.38999825496,87.55450823221));
#138313=CARTESIAN_POINT('Ctrl Pts',(29.7415966793991,15.73193890552,88.06198850603));
#138314=CARTESIAN_POINT('Ctrl Pts',(32.0109525733291,16.02018950073,80.626324032147));
#138315=CARTESIAN_POINT('Ctrl Pts',(31.5698153999191,15.89672173437,80.952027168743));
#138316=CARTESIAN_POINT('Ctrl Pts',(30.9280379274291,15.7943497689,81.463551765629));
#138317=CARTESIAN_POINT('Ctrl Pts',(30.1155556593891,15.81791239968,82.186276359872));
#138318=CARTESIAN_POINT('Ctrl Pts',(29.5676182319791,15.90095742703,82.706753402063));
#138319=CARTESIAN_POINT('Ctrl Pts',(29.0444936137691,16.05004143134,83.23817878262));
#138320=CARTESIAN_POINT('Ctrl Pts',(28.3388309664491,16.35525555443,84.00675759992));
#138321=CARTESIAN_POINT('Ctrl Pts',(27.8654686878691,16.69852697646,84.59147024585));
#138322=CARTESIAN_POINT('Ctrl Pts',(27.5770904290591,16.97909376117,84.98370283207));
#138323=CARTESIAN_POINT('Ctrl Pts',(30.1132980125691,16.72999540751,78.946185718569));
#138324=CARTESIAN_POINT('Ctrl Pts',(29.7137407941691,16.65934526971,79.210897567761));
#138325=CARTESIAN_POINT('Ctrl Pts',(29.1340526716791,16.61720595081,79.615340806471));
#138326=CARTESIAN_POINT('Ctrl Pts',(28.3933628948891,16.68117614212,80.172130006458));
#138327=CARTESIAN_POINT('Ctrl Pts',(27.8889896965391,16.77573676935,80.56865339757));
#138328=CARTESIAN_POINT('Ctrl Pts',(27.4006391487591,16.91970666313,80.970498491355));
#138329=CARTESIAN_POINT('Ctrl Pts',(26.7293418797291,17.1948500933,81.549382547162));
#138330=CARTESIAN_POINT('Ctrl Pts',(26.2594753174191,17.48867903209,81.989427557792));
#138331=CARTESIAN_POINT('Ctrl Pts',(25.9607500271791,17.72646700966,82.286884785861));
#138332=CARTESIAN_POINT('Ctrl Pts',(28.8360405155491,17.14364644213,77.547996582545));
#138333=CARTESIAN_POINT('Ctrl Pts',(28.4591298614191,17.10612249352,77.7565186051));
#138334=CARTESIAN_POINT('Ctrl Pts',(27.9131147582991,17.10100848932,78.069500245689));
#138335=CARTESIAN_POINT('Ctrl Pts',(27.2114257336291,17.1895306756,78.492997722336));
#138336=CARTESIAN_POINT('Ctrl Pts',(26.7308206771491,17.29099595334,78.792251113258));
#138337=CARTESIAN_POINT('Ctrl Pts',(26.2616100161191,17.43172986728,79.093840232636));
#138338=CARTESIAN_POINT('Ctrl Pts',(25.6095490746191,17.68828983474,79.526837436468));
#138339=CARTESIAN_POINT('Ctrl Pts',(25.1422058870291,17.95143027748,79.855318404731));
#138340=CARTESIAN_POINT('Ctrl Pts',(24.8380947587091,18.16211819104,80.078213338469));
#138341=CARTESIAN_POINT('Ctrl Pts',(27.7757217083991,17.43097964734,75.935707638512));
#138342=CARTESIAN_POINT('Ctrl Pts',(27.4109041085991,17.41739952321,76.076412741866));
#138343=CARTESIAN_POINT('Ctrl Pts',(26.8827892158591,17.43865574786,76.284524941454));
#138344=CARTESIAN_POINT('Ctrl Pts',(26.2010864915091,17.54453132413,76.561822608305));
#138345=CARTESIAN_POINT('Ctrl Pts',(25.7321757229291,17.65084167707,76.756297187885));
#138346=CARTESIAN_POINT('Ctrl Pts',(25.2716674990791,17.78924911077,76.95111769228));
#138347=CARTESIAN_POINT('Ctrl Pts',(24.6267935566291,18.03257374984,77.229569264194));
#138348=CARTESIAN_POINT('Ctrl Pts',(24.1570693932891,18.27376550526,77.439744979685));
#138349=CARTESIAN_POINT('Ctrl Pts',(23.8465745131891,18.46478090637,77.582383835345));
#138350=CARTESIAN_POINT('Ctrl Pts',(27.3559829090791,17.50227562775,74.737748587929));
#138351=CARTESIAN_POINT('Ctrl Pts',(26.9886729618591,17.49501040547,74.829545064085));
#138352=CARTESIAN_POINT('Ctrl Pts',(26.4568742846691,17.5231506785,74.963967484974));
#138353=CARTESIAN_POINT('Ctrl Pts',(25.7693264362491,17.63352646129,75.140665286621));
#138354=CARTESIAN_POINT('Ctrl Pts',(25.2957536935691,17.74108044178,75.26361100159));
#138355=CARTESIAN_POINT('Ctrl Pts',(24.8298434891491,17.87886333591,75.385823935064));
#138356=CARTESIAN_POINT('Ctrl Pts',(24.1759661689291,18.11870473769,75.559169478868));
#138357=CARTESIAN_POINT('Ctrl Pts',(23.6975268624191,18.35411537331,75.688361893926));
#138358=CARTESIAN_POINT('Ctrl Pts',(23.3799146126391,18.53989443776,75.775287078776));
#138359=CARTESIAN_POINT('Ctrl Pts',(27.2374127596391,17.5024417656,74.063277809669));
#138360=CARTESIAN_POINT('Ctrl Pts',(26.8654749426391,17.49516466441,74.128758125854));
#138361=CARTESIAN_POINT('Ctrl Pts',(26.3267139877291,17.52329437382,74.223606886666));
#138362=CARTESIAN_POINT('Ctrl Pts',(25.6296536722291,17.63366412477,74.346321907819));
#138363=CARTESIAN_POINT('Ctrl Pts',(25.1493092353391,17.74121690541,74.430883836857));
#138364=CARTESIAN_POINT('Ctrl Pts',(24.6765124261091,17.87900164837,74.514115976861));
#138365=CARTESIAN_POINT('Ctrl Pts',(24.0126415485491,18.11885073386,74.630983591579));
#138366=CARTESIAN_POINT('Ctrl Pts',(23.5264635813191,18.35427499937,74.7165680779));
#138367=CARTESIAN_POINT('Ctrl Pts',(23.2035020446091,18.54006963518,74.773419590361));
#138368=CARTESIAN_POINT('Ctrl Pts',(38.6333955078091,1.20463046452501,98.36582747163));
#138369=CARTESIAN_POINT('Ctrl Pts',(38.4753072726105,1.12679210517909,97.4433768413534));
#138370=CARTESIAN_POINT('Ctrl Pts',(38.4718338960078,1.01542204172217,95.9047402985046));
#138371=CARTESIAN_POINT('Ctrl Pts',(39.1178057748741,0.912164862004577,
93.839260600352));
#138372=CARTESIAN_POINT('Ctrl Pts',(39.9251685220998,0.864777045730714,
92.3885218066525));
#138373=CARTESIAN_POINT('Ctrl Pts',(41.0140425215617,0.851590513166468,
91.1342818091396));
#138374=CARTESIAN_POINT('Ctrl Pts',(42.7385836460012,0.879209305050257,
89.819425823229));
#138375=CARTESIAN_POINT('Ctrl Pts',(44.1903166991323,0.944541149739843,
89.2952475883841));
#138376=CARTESIAN_POINT('Ctrl Pts',(45.1145255779391,0.998148899213914,
89.12773857891));
#138377=CARTESIAN_POINT('Ctrl Pts',(45.2621172516992,-1.15864950900999,
89.08880321312));
#138378=CARTESIAN_POINT('Ctrl Pts',(40.5154296034891,-0.834138914950386,
89.85429588814));
#138379=CARTESIAN_POINT('Ctrl Pts',(37.7466329253491,-0.935506535982887,
93.79723450388));
#138380=CARTESIAN_POINT('Ctrl Pts',(38.6479058880891,-1.40084793775299,
98.50842201768));
#138381=CARTESIAN_POINT('Ctrl Pts',(45.3589510903891,-0.390141862995886,
89.14750817678));
#138382=CARTESIAN_POINT('Ctrl Pts',(40.5597617275791,-0.273423176279186,
89.8799349496001));
#138383=CARTESIAN_POINT('Ctrl Pts',(37.7778654476491,-0.307631400561986,
93.8550658461399));
#138384=CARTESIAN_POINT('Ctrl Pts',(38.7306673927291,-0.471664968376586,
98.61944068779));
#138385=CARTESIAN_POINT('Ctrl Pts',(45.3590610166491,0.389380164346614,
89.14757463976));
#138386=CARTESIAN_POINT('Ctrl Pts',(40.5598094357291,0.272875683534014,
89.87996448328));
#138387=CARTESIAN_POINT('Ctrl Pts',(37.7779005857991,0.307017177882314,
93.85512864424));
#138388=CARTESIAN_POINT('Ctrl Pts',(38.7307611829491,0.470744074667514,
98.61956668849));
#138389=CARTESIAN_POINT('Ctrl Pts',(45.2620963482791,1.15881536706201,89.0887905755001));
#138390=CARTESIAN_POINT('Ctrl Pts',(40.5154205858591,0.834257573969314,
89.85429029489));
#138391=CARTESIAN_POINT('Ctrl Pts',(37.7466262750891,0.935639663228715,
93.79722263086));
#138392=CARTESIAN_POINT('Ctrl Pts',(38.6478880539091,1.40104845952501,98.50839805774));
#138393=CARTESIAN_POINT('Ctrl Pts',(38.633398543612,-1.20459248515192,98.3658322832796));
#138394=CARTESIAN_POINT('Ctrl Pts',(38.4750595671407,-1.12662990155636,
97.4420569298962));
#138395=CARTESIAN_POINT('Ctrl Pts',(38.4730057154008,-1.05234132108018,
96.4153551870171));
#138396=CARTESIAN_POINT('Ctrl Pts',(38.688099235323,-0.993182043686503,
95.3844390851496));
#138397=CARTESIAN_POINT('Ctrl Pts',(38.7956643429362,-0.963597358655216,
94.8688930962344));
#138398=CARTESIAN_POINT('Ctrl Pts',(38.9575348153517,-0.937796299191181,
94.3522931567739));
#138399=CARTESIAN_POINT('Ctrl Pts',(39.1730608688322,-0.917015017058684,
93.8523939206696));
#138400=CARTESIAN_POINT('Ctrl Pts',(39.388586922313,-0.89623373492617,93.3524946845649));
#138401=CARTESIAN_POINT('Ctrl Pts',(39.6577685563747,-0.880472231343552,
92.8692961516738));
#138402=CARTESIAN_POINT('Ctrl Pts',(39.973796875558,-0.870404943100818,
92.4188366157056));
#138403=CARTESIAN_POINT('Ctrl Pts',(40.2898251947411,-0.860337654858091,
91.9683770797378));
#138404=CARTESIAN_POINT('Ctrl Pts',(40.6527001985936,-0.855964583453665,
91.5506565403542));
#138405=CARTESIAN_POINT('Ctrl Pts',(41.04965023065,-0.857235390346154,91.1775461714496));
#138406=CARTESIAN_POINT('Ctrl Pts',(41.4466002627064,-0.858506197238643,
90.8044358025451));
#138407=CARTESIAN_POINT('Ctrl Pts',(41.8776253226757,-0.86542088368976,
90.4759356036829));
#138408=CARTESIAN_POINT('Ctrl Pts',(42.3262312945887,-0.87728971852162,
90.1987272975449));
#138409=CARTESIAN_POINT('Ctrl Pts',(43.223278104326,-0.901023019208226,
89.6444127270248));
#138410=CARTESIAN_POINT('Ctrl Pts',(44.1906226700922,-0.944565655229909,
89.2951902027352));
#138411=CARTESIAN_POINT('Ctrl Pts',(45.1145147831368,-0.998148588101653,
89.1277405085709));
#138412=CARTESIAN_POINT('Ctrl Pts',(27.2376871946991,-17.50242971854,74.064711156945));
#138413=CARTESIAN_POINT('Ctrl Pts',(26.8658614035591,-17.49515074741,74.130158119919));
#138414=CARTESIAN_POINT('Ctrl Pts',(26.3273110298991,-17.52325375652,74.224981944857));
#138415=CARTESIAN_POINT('Ctrl Pts',(25.6305562435091,-17.63353027567,74.347718111042));
#138416=CARTESIAN_POINT('Ctrl Pts',(25.1504846035391,-17.74097529298,74.432308612216));
#138417=CARTESIAN_POINT('Ctrl Pts',(24.6779517816891,-17.87862088949,74.515594757026));
#138418=CARTESIAN_POINT('Ctrl Pts',(24.0138164969491,-18.11845385552,74.632686329655));
#138419=CARTESIAN_POINT('Ctrl Pts',(23.5273164623691,-18.35399576693,74.718503829381));
#138420=CARTESIAN_POINT('Ctrl Pts',(23.2039932885991,-18.54001387247,74.775558557214));
#138421=CARTESIAN_POINT('Ctrl Pts',(27.4622817506591,-17.50215063165,75.344035218027));
#138422=CARTESIAN_POINT('Ctrl Pts',(27.0993410480891,-17.4949504767,75.459863317511));
#138423=CARTESIAN_POINT('Ctrl Pts',(26.5741073480191,-17.52312828209,75.630219120973));
#138424=CARTESIAN_POINT('Ctrl Pts',(25.8954617502391,-17.63344814792,75.855590909026));
#138425=CARTESIAN_POINT('Ctrl Pts',(25.4282471079291,-17.74090226414,76.012993057361));
#138426=CARTESIAN_POINT('Ctrl Pts',(24.9687583406291,-17.87853649113,76.170072411934));
#138427=CARTESIAN_POINT('Ctrl Pts',(24.3235268820491,-18.11832265721,76.393972063008));
#138428=CARTESIAN_POINT('Ctrl Pts',(23.8516161818191,-18.35378673397,76.562026007774));
#138429=CARTESIAN_POINT('Ctrl Pts',(23.5383556626691,-18.53972438058,76.67570803482));
#138430=CARTESIAN_POINT('Ctrl Pts',(28.3553575821991,-17.3000243591,77.031526632576));
#138431=CARTESIAN_POINT('Ctrl Pts',(27.9871351116891,-17.27423244174,77.21725093699));
#138432=CARTESIAN_POINT('Ctrl Pts',(27.4540754692791,-17.28222627378,77.494120215153));
#138433=CARTESIAN_POINT('Ctrl Pts',(26.7674832235591,-17.37939031724,77.866659505309));
#138434=CARTESIAN_POINT('Ctrl Pts',(26.2961871648991,-17.483225832,78.129325170163));
#138435=CARTESIAN_POINT('Ctrl Pts',(25.8345528030491,-17.62271428892,78.393813226736));
#138436=CARTESIAN_POINT('Ctrl Pts',(25.1896731535291,-17.87276274756,78.774035747848));
#138437=CARTESIAN_POINT('Ctrl Pts',(24.7231787828791,-18.12528329555,79.063320155367));
#138438=CARTESIAN_POINT('Ctrl Pts',(24.4168763580191,-18.32674912521,79.260661805121));
#138439=CARTESIAN_POINT('Ctrl Pts',(30.1193998698591,-16.72712396501,78.954400989807));
#138440=CARTESIAN_POINT('Ctrl Pts',(29.7196308839791,-16.65610278602,79.218655211296));
#138441=CARTESIAN_POINT('Ctrl Pts',(29.1397569070191,-16.61352754412,79.622692280116));
#138442=CARTESIAN_POINT('Ctrl Pts',(28.3990365457491,-16.67711876983,80.179492293071));
#138443=CARTESIAN_POINT('Ctrl Pts',(27.8947871921491,-16.77147652606,80.576206493652));
#138444=CARTESIAN_POINT('Ctrl Pts',(27.4066386321391,-16.91531277421,80.978475817268));
#138445=CARTESIAN_POINT('Ctrl Pts',(26.7351116874891,-17.19062376,81.558839194189));
#138446=CARTESIAN_POINT('Ctrl Pts',(26.2651731610791,-17.48497135719,82.000528837247));
#138447=CARTESIAN_POINT('Ctrl Pts',(25.9663983567091,-17.7233890594,82.299404522218));
#138448=CARTESIAN_POINT('Ctrl Pts',(31.5561577943991,-16.18994150244,80.22094136623));
#138449=CARTESIAN_POINT('Ctrl Pts',(31.1252443032691,-16.07925352154,80.532043662118));
#138450=CARTESIAN_POINT('Ctrl Pts',(30.4987078973991,-15.99141036723,81.017800973616));
#138451=CARTESIAN_POINT('Ctrl Pts',(29.7037869514191,-16.02460055635,81.700406797817));
#138452=CARTESIAN_POINT('Ctrl Pts',(29.1665363909691,-16.11026999969,82.190788103002));
#138453=CARTESIAN_POINT('Ctrl Pts',(28.6519091810491,-16.25790421064,82.690692942473));
#138454=CARTESIAN_POINT('Ctrl Pts',(27.9539338991491,-16.55575169532,83.41372255913));
#138455=CARTESIAN_POINT('Ctrl Pts',(27.4808216495891,-16.88723154289,83.9637329239));
#138456=CARTESIAN_POINT('Ctrl Pts',(27.1894469550491,-17.15778055581,84.3333305677));
#138457=CARTESIAN_POINT('Ctrl Pts',(33.0578858065291,-15.54336585756,81.389299787288));
#138458=CARTESIAN_POINT('Ctrl Pts',(32.5880867582691,-15.38869757245,81.734403671999));
#138459=CARTESIAN_POINT('Ctrl Pts',(31.9034088135191,-15.24938125701,82.2882617717));
#138460=CARTESIAN_POINT('Ctrl Pts',(31.0424761811091,-15.24749815586,83.08721118401));
#138461=CARTESIAN_POINT('Ctrl Pts',(30.4660563986391,-15.32299129414,83.66757894853));
#138462=CARTESIAN_POINT('Ctrl Pts',(29.9214516069391,-15.47480379595,84.26363113591));
#138463=CARTESIAN_POINT('Ctrl Pts',(29.1964456396391,-15.79815807595,85.12912638987));
#138464=CARTESIAN_POINT('Ctrl Pts',(28.7258139100191,-16.17140621328,85.78811940437));
#138465=CARTESIAN_POINT('Ctrl Pts',(28.4483807343891,-16.47717452847,86.22779003313));
#138466=CARTESIAN_POINT('Ctrl Pts',(34.6049178055991,-14.78277420146,82.480029194831));
#138467=CARTESIAN_POINT('Ctrl Pts',(34.0899124633891,-14.58252420113,82.848023844388));
#138468=CARTESIAN_POINT('Ctrl Pts',(33.3369620788591,-14.38812926471,83.45824711867));
#138469=CARTESIAN_POINT('Ctrl Pts',(32.3994019289691,-14.34794908773,84.36615210939));
#138470=CARTESIAN_POINT('Ctrl Pts',(31.7784092493091,-14.41206214076,85.03407623603));
#138471=CARTESIAN_POINT('Ctrl Pts',(31.2011411103491,-14.56803185909,85.72574244534));
#138472=CARTESIAN_POINT('Ctrl Pts',(30.4498066469591,-14.91828463801,86.73422814589));
#138473=CARTESIAN_POINT('Ctrl Pts',(29.9883414176491,-15.33534062518,87.50228846636));
#138474=CARTESIAN_POINT('Ctrl Pts',(29.7317228173191,-15.67683330334,88.01029890114));
#138475=CARTESIAN_POINT('Ctrl Pts',(36.1557734484991,-13.91129254351,83.49443968804));
#138476=CARTESIAN_POINT('Ctrl Pts',(35.5907542250291,-13.66696468785,83.87370698997));
#138477=CARTESIAN_POINT('Ctrl Pts',(34.7611060909791,-13.41714938065,84.52732824685));
#138478=CARTESIAN_POINT('Ctrl Pts',(33.7381310519291,-13.33737915323,85.53560671627));
#138479=CARTESIAN_POINT('Ctrl Pts',(33.0684097051491,-13.38932909829,86.28806646301));
#138480=CARTESIAN_POINT('Ctrl Pts',(32.4570980029091,-13.54895837645,87.07443382171));
#138481=CARTESIAN_POINT('Ctrl Pts',(31.6820799917791,-13.92554710058,88.22604588797));
#138482=CARTESIAN_POINT('Ctrl Pts',(31.2378322667491,-14.38531781278,89.10291972624));
#138483=CARTESIAN_POINT('Ctrl Pts',(31.0092985950491,-14.76017803516,89.67723077357));
#138484=CARTESIAN_POINT('Ctrl Pts',(37.6697908381991,-12.93342159556,84.43736943397));
#138485=CARTESIAN_POINT('Ctrl Pts',(37.0505468967491,-12.64931175638,84.81611293096));
#138486=CARTESIAN_POINT('Ctrl Pts',(36.1365854207591,-12.34691554832,85.49916954727));
#138487=CARTESIAN_POINT('Ctrl Pts',(35.0208060078891,-12.22821099738,86.5981509169));
#138488=CARTESIAN_POINT('Ctrl Pts',(34.2994459610991,-12.26764960418,87.43159373777));
#138489=CARTESIAN_POINT('Ctrl Pts',(33.6542855854991,-12.42996124639,88.31146584508));
#138490=CARTESIAN_POINT('Ctrl Pts',(32.8608868434491,-12.8303717258,89.60620123627));
#138491=CARTESIAN_POINT('Ctrl Pts',(32.4441203154791,-13.32873869874,90.59169511767));
#138492=CARTESIAN_POINT('Ctrl Pts',(32.2519928613791,-13.73206374234,91.23040310054));
#138493=CARTESIAN_POINT('Ctrl Pts',(39.1273312888591,-11.8403276167,85.31977033749));
#138494=CARTESIAN_POINT('Ctrl Pts',(38.4474756767491,-11.52446324037,85.68454099069));
#138495=CARTESIAN_POINT('Ctrl Pts',(37.4387918460291,-11.17680143917,86.38047210049));
#138496=CARTESIAN_POINT('Ctrl Pts',(36.2212968557791,-11.02262212161,87.55888335763));
#138497=CARTESIAN_POINT('Ctrl Pts',(35.4455092049291,-11.04980237437,88.4695866419));
#138498=CARTESIAN_POINT('Ctrl Pts',(34.7681392980591,-11.21304523729,89.44254871937));
#138499=CARTESIAN_POINT('Ctrl Pts',(33.9655380969891,-11.63176263852,90.8826799955));
#138500=CARTESIAN_POINT('Ctrl Pts',(33.5912508076991,-12.16011199612,91.97939523496));
#138501=CARTESIAN_POINT('Ctrl Pts',(33.4470797619991,-12.58335502103,92.68277286242));
#138502=CARTESIAN_POINT('Ctrl Pts',(40.5143347257491,-10.62442344881,86.13753768628));
#138503=CARTESIAN_POINT('Ctrl Pts',(39.7704791065591,-10.28796359687,86.47738091817));
#138504=CARTESIAN_POINT('Ctrl Pts',(38.6600450862691,-9.90660226357599,
87.17143604644));
#138505=CARTESIAN_POINT('Ctrl Pts',(37.3343124845091,-9.72320040582899,
88.41839063577));
#138506=CARTESIAN_POINT('Ctrl Pts',(36.5021983603491,-9.73897061260399,
89.40229438399));
#138507=CARTESIAN_POINT('Ctrl Pts',(35.7943862373391,-9.90058283852199,
90.46707941507));
#138508=CARTESIAN_POINT('Ctrl Pts',(34.9907319257591,-10.32907754693,92.05293918629));
#138509=CARTESIAN_POINT('Ctrl Pts',(34.6711977041091,-10.87458861386,93.26106621997));
#138510=CARTESIAN_POINT('Ctrl Pts',(34.5833472293291,-11.30624036383,94.02751284757));
#138511=CARTESIAN_POINT('Ctrl Pts',(41.7958013258191,-9.28987808742799,
86.87970286268));
#138512=CARTESIAN_POINT('Ctrl Pts',(40.9877508719891,-8.94697080201899,
87.18647982707));
#138513=CARTESIAN_POINT('Ctrl Pts',(39.7729888752691,-8.54808012355799,
87.86595909715));
#138514=CARTESIAN_POINT('Ctrl Pts',(38.3365366245991,-8.34497648694099,
89.17012596732));
#138515=CARTESIAN_POINT('Ctrl Pts',(37.4480998536291,-8.35094758626199,
90.22184936653));
#138516=CARTESIAN_POINT('Ctrl Pts',(36.7124380878191,-8.50750595763099,
91.37510535399));
#138517=CARTESIAN_POINT('Ctrl Pts',(35.9152797461691,-8.93394304236699,
93.10327895919));
#138518=CARTESIAN_POINT('Ctrl Pts',(35.6596789728091,-9.47940936258599,
94.41963511778));
#138519=CARTESIAN_POINT('Ctrl Pts',(35.6331349407091,-9.90524587332399,
95.24555986742));
#138520=CARTESIAN_POINT('Ctrl Pts',(43.3219632460591,-7.36135345490399,
87.75528993168));
#138521=CARTESIAN_POINT('Ctrl Pts',(42.4290781817991,-7.03416672139499,
88.00906536633));
#138522=CARTESIAN_POINT('Ctrl Pts',(41.0743404925991,-6.64178586828799,
88.65318138295));
#138523=CARTESIAN_POINT('Ctrl Pts',(39.4905266686191,-6.43118382119999,
90.01661339155));
#138524=CARTESIAN_POINT('Ctrl Pts',(38.5292058215891,-6.42772090807399,
91.14933865191));
#138525=CARTESIAN_POINT('Ctrl Pts',(37.7614435355091,-6.57146966826899,
92.4133885279));
#138526=CARTESIAN_POINT('Ctrl Pts',(36.9839460387491,-6.97338480763799,
94.32296649059));
#138527=CARTESIAN_POINT('Ctrl Pts',(36.8244342451791,-7.48783164222599,
95.77749406464));
#138528=CARTESIAN_POINT('Ctrl Pts',(36.8845638606391,-7.88177804932599,
96.67778125325));
#138529=CARTESIAN_POINT('Ctrl Pts',(44.8847825465991,-4.53379995664999,
88.65117139258));
#138530=CARTESIAN_POINT('Ctrl Pts',(43.8875433874391,-4.28701338408699,
88.82538752989));
#138531=CARTESIAN_POINT('Ctrl Pts',(42.3572012561891,-3.98133338461999,
89.39823867593));
#138532=CARTESIAN_POINT('Ctrl Pts',(40.5912760574091,-3.81238616029299,
90.80439331935));
#138533=CARTESIAN_POINT('Ctrl Pts',(39.5441584350891,-3.80718625688099,
92.02046230176));
#138534=CARTESIAN_POINT('Ctrl Pts',(38.7467026882691,-3.91832816602299,
93.40922179908));
#138535=CARTESIAN_POINT('Ctrl Pts',(38.0150490895291,-4.23041625890299,
95.52979012452));
#138536=CARTESIAN_POINT('Ctrl Pts',(37.9944515607391,-4.62428373692299,
97.1464303542));
#138537=CARTESIAN_POINT('Ctrl Pts',(38.1700698731891,-4.91739601039799,
98.13189991486));
#138538=CARTESIAN_POINT('Ctrl Pts',(45.4723589720291,-2.05622846366899,
89.00701499552));
#138539=CARTESIAN_POINT('Ctrl Pts',(44.4289451307191,-1.93443369721799,
89.14097418644));
#138540=CARTESIAN_POINT('Ctrl Pts',(42.8186744917191,-1.78523787771199,
89.67173154877));
#138541=CARTESIAN_POINT('Ctrl Pts',(40.9703371621991,-1.71096995167399,
91.08656561906));
#138542=CARTESIAN_POINT('Ctrl Pts',(39.8861319792491,-1.71788080442199,
92.33509446141));
#138543=CARTESIAN_POINT('Ctrl Pts',(39.0794495206591,-1.78492357597099,
93.77723356639));
#138544=CARTESIAN_POINT('Ctrl Pts',(38.3775544718791,-1.95885807874699,
95.99082783574));
#138545=CARTESIAN_POINT('Ctrl Pts',(38.4274398112191,-2.16887299505599,
97.67915781703));
#138546=CARTESIAN_POINT('Ctrl Pts',(38.6575428468991,-2.32228900990999,
98.70137587772));
#138547=CARTESIAN_POINT('Ctrl Pts',(45.5703559106791,-0.706838991786186,
89.08233472503));
#138548=CARTESIAN_POINT('Ctrl Pts',(44.5190093055891,-0.658776199678386,
89.20902470915));
#138549=CARTESIAN_POINT('Ctrl Pts',(42.8950488879291,-0.603452424076586,
89.73237110619));
#138550=CARTESIAN_POINT('Ctrl Pts',(41.0328038634091,-0.587152567652286,
91.14929043576));
#138551=CARTESIAN_POINT('Ctrl Pts',(39.9424972960391,-0.602152125724686,
92.40413647438));
#138552=CARTESIAN_POINT('Ctrl Pts',(39.1345984995491,-0.643420016667986,
93.85645551823));
#138553=CARTESIAN_POINT('Ctrl Pts',(38.4384727545291,-0.735528951145086,
96.08773389849));
#138554=CARTESIAN_POINT('Ctrl Pts',(38.5010964114291,-0.837059021185586,
97.78980341537));
#138555=CARTESIAN_POINT('Ctrl Pts',(38.7410049107391,-0.909108343223786,
98.81920581999));
#138556=CARTESIAN_POINT('Ctrl Pts',(23.3999522626291,-18.46444455277,75.101511144727));
#138557=CARTESIAN_POINT('Ctrl Pts',(23.6819559758774,-18.3084167846969,
75.0422841334927));
#138558=CARTESIAN_POINT('Ctrl Pts',(24.1224882166048,-18.099220390028,74.9502420759054));
#138559=CARTESIAN_POINT('Ctrl Pts',(24.7357218717077,-17.8765903523576,
74.8230687141201));
#138560=CARTESIAN_POINT('Ctrl Pts',(25.2059849516925,-17.7389322063629,
74.7260037905263));
#138561=CARTESIAN_POINT('Ctrl Pts',(25.6838350115992,-17.6315140604179,
74.6278234280083));
#138562=CARTESIAN_POINT('Ctrl Pts',(26.3272794229534,-17.5293070988979,
74.4962086120361));
#138563=CARTESIAN_POINT('Ctrl Pts',(26.8127282037799,-17.4991473899451,
74.3975630489114));
#138564=CARTESIAN_POINT('Ctrl Pts',(27.1339039101791,-17.49925933285,74.332577093855));
#138565=CARTESIAN_POINT('Ctrl Pts',(36.2847637417591,-13.03008673973,65.304882352288));
#138566=CARTESIAN_POINT('Ctrl Pts',(35.4698014376591,-12.56680377023,65.284703747679));
#138567=CARTESIAN_POINT('Ctrl Pts',(33.7713459763991,-11.76550621918,64.954403657768));
#138568=CARTESIAN_POINT('Ctrl Pts',(31.2509181992091,-11.10983496554,63.528029780689));
#138569=CARTESIAN_POINT('Ctrl Pts',(29.1719527512791,-11.10598381288,61.40902742803));
#138570=CARTESIAN_POINT('Ctrl Pts',(28.3093846275791,-11.53960369611,59.76597835192));
#138571=CARTESIAN_POINT('Ctrl Pts',(28.0133963045591,-11.84319082917,58.93048676556));
#138572=CARTESIAN_POINT('Ctrl Pts',(35.3612714178091,-13.75149761196,65.828779517486));
#138573=CARTESIAN_POINT('Ctrl Pts',(34.5898538310391,-13.29877169444,65.746262964501));
#138574=CARTESIAN_POINT('Ctrl Pts',(33.0012696328491,-12.54391137714,65.330700476229));
#138575=CARTESIAN_POINT('Ctrl Pts',(30.6472653659591,-11.99120018154,63.94211678041));
#138576=CARTESIAN_POINT('Ctrl Pts',(28.6504997586391,-12.08505199754,61.9975050885));
#138577=CARTESIAN_POINT('Ctrl Pts',(27.7514021894691,-12.57465019834,60.50747334694));
#138578=CARTESIAN_POINT('Ctrl Pts',(27.4172271538291,-12.90829735611,59.74325498279));
#138579=CARTESIAN_POINT('Ctrl Pts',(33.9310055689291,-14.66551773857,66.731530388817));
#138580=CARTESIAN_POINT('Ctrl Pts',(33.2239791263591,-14.26430514063,66.574557910788));
#138581=CARTESIAN_POINT('Ctrl Pts',(31.7938275819191,-13.62995645862,66.075552147711));
#138582=CARTESIAN_POINT('Ctrl Pts',(29.6808305514691,-13.23557272568,64.786213365519));
#138583=CARTESIAN_POINT('Ctrl Pts',(27.8237882040291,-13.4193547387,63.112257346372));
#138584=CARTESIAN_POINT('Ctrl Pts',(26.8992667269091,-13.92561452162,61.85204205614));
#138585=CARTESIAN_POINT('Ctrl Pts',(26.5219839729091,-14.26629883929,61.19814887933));
#138586=CARTESIAN_POINT('Ctrl Pts',(31.9653864880491,-15.65866033563,68.137112684262));
#138587=CARTESIAN_POINT('Ctrl Pts',(31.3430676569791,-15.35884927897,67.937246194186));
#138588=CARTESIAN_POINT('Ctrl Pts',(30.1109982698091,-14.91655490052,67.428984529203));
#138589=CARTESIAN_POINT('Ctrl Pts',(28.2990532332591,-14.715846867,66.347539498663));
#138590=CARTESIAN_POINT('Ctrl Pts',(26.6499274220891,-14.96778503067,65.039851765409));
#138591=CARTESIAN_POINT('Ctrl Pts',(25.7469355071991,-15.4403980032,64.07345053952));
#138592=CARTESIAN_POINT('Ctrl Pts',(25.3455324472891,-15.75408920875,63.565837580849));
#138593=CARTESIAN_POINT('Ctrl Pts',(30.7929135889891,-16.17250423569,69.060223736395));
#138594=CARTESIAN_POINT('Ctrl Pts',(30.2218145303891,-15.93993030477,68.857014383728));
#138595=CARTESIAN_POINT('Ctrl Pts',(29.1046827678391,-15.6154113433,68.381023828893));
#138596=CARTESIAN_POINT('Ctrl Pts',(27.4656460240191,-15.52077373642,67.452927434318));
#138597=CARTESIAN_POINT('Ctrl Pts',(25.9460657515691,-15.79931084072,66.37136947448));
#138598=CARTESIAN_POINT('Ctrl Pts',(25.0733613416891,-16.2390237074,65.580737057625));
#138599=CARTESIAN_POINT('Ctrl Pts',(24.6690559172891,-16.52770085378,65.16275338086));
#138600=CARTESIAN_POINT('Ctrl Pts',(29.8953539876391,-16.52906213236,69.832873012479));
#138601=CARTESIAN_POINT('Ctrl Pts',(29.3639102670391,-16.34951665805,69.641956269545));
#138602=CARTESIAN_POINT('Ctrl Pts',(28.3335435871991,-16.11400158648,69.215018188098));
#138603=CARTESIAN_POINT('Ctrl Pts',(26.8248918532791,-16.09500778036,68.425440053671));
#138604=CARTESIAN_POINT('Ctrl Pts',(25.4087624306691,-16.38876032548,67.526783025968));
#138605=CARTESIAN_POINT('Ctrl Pts',(24.5693720645591,-16.79958429557,66.874208922604));
#138606=CARTESIAN_POINT('Ctrl Pts',(24.1698056852491,-17.06622361444,66.52747591034));
#138607=CARTESIAN_POINT('Ctrl Pts',(29.2502102588991,-16.77062600901,70.433798567399));
#138608=CARTESIAN_POINT('Ctrl Pts',(28.7480655049691,-16.62976631616,70.259448042778));
#138609=CARTESIAN_POINT('Ctrl Pts',(27.7806025530991,-16.45760049426,69.880735221407));
#138610=CARTESIAN_POINT('Ctrl Pts',(26.3660736362391,-16.49066456513,69.204010259922));
#138611=CARTESIAN_POINT('Ctrl Pts',(25.0269527850791,-16.79338156446,68.445873273539));
#138612=CARTESIAN_POINT('Ctrl Pts',(24.2161158147491,-17.18210581398,67.897653773474));
#138613=CARTESIAN_POINT('Ctrl Pts',(23.8230728735191,-17.43180749021,67.605233264723));
#138614=CARTESIAN_POINT('Ctrl Pts',(28.6545914816891,-16.98327424387,71.053055016883));
#138615=CARTESIAN_POINT('Ctrl Pts',(28.1808726772791,-16.87866687246,70.902653141502));
#138616=CARTESIAN_POINT('Ctrl Pts',(27.2732594603691,-16.7646019857,70.583475740074));
#138617=CARTESIAN_POINT('Ctrl Pts',(25.9477619708291,-16.84407223426,70.02876229231));
#138618=CARTESIAN_POINT('Ctrl Pts',(24.6834075254991,-17.1536727076,69.415215054408));
#138619=CARTESIAN_POINT('Ctrl Pts',(23.9034829216691,-17.52101768117,68.972833511437));
#138620=CARTESIAN_POINT('Ctrl Pts',(23.5194027135091,-17.75422570749,68.735949323231));
#138621=CARTESIAN_POINT('Ctrl Pts',(27.9475189385191,-17.22587397515,71.899449525734));
#138622=CARTESIAN_POINT('Ctrl Pts',(27.5097123036091,-17.16491155286,71.790690508363));
#138623=CARTESIAN_POINT('Ctrl Pts',(26.6764981741391,-17.11951879115,71.565626599136));
#138624=CARTESIAN_POINT('Ctrl Pts',(25.4614629953291,-17.25252680212,71.185898966309));
#138625=CARTESIAN_POINT('Ctrl Pts',(24.2924439417591,-17.56896510761,70.771196353781));
#138626=CARTESIAN_POINT('Ctrl Pts',(23.5559636381791,-17.90994030748,70.472334572156));
#138627=CARTESIAN_POINT('Ctrl Pts',(23.1867259327591,-18.12267084568,70.311239709512));
#138628=CARTESIAN_POINT('Ctrl Pts',(27.2648539692091,-17.45480313428,73.0469627073486));
#138629=CARTESIAN_POINT('Ctrl Pts',(26.8690285353091,-17.43758746319,73.0138154548454));
#138630=CARTESIAN_POINT('Ctrl Pts',(26.1203911687191,-17.4593694823,72.9441921949709));
#138631=CARTESIAN_POINT('Ctrl Pts',(25.0299860121291,-17.64326059802,72.8224812819406));
#138632=CARTESIAN_POINT('Ctrl Pts',(23.9723631160091,-17.96516190501,72.6844389313152));
#138633=CARTESIAN_POINT('Ctrl Pts',(23.2930064261891,-18.27939241191,72.5801519585368));
#138634=CARTESIAN_POINT('Ctrl Pts',(22.9467037503691,-18.47108761386,72.5222039840777));
#138635=CARTESIAN_POINT('Ctrl Pts',(27.1796563116291,-17.51202862775,73.966572328327));
#138636=CARTESIAN_POINT('Ctrl Pts',(26.8047259968491,-17.50681468964,74.010390650564));
#138637=CARTESIAN_POINT('Ctrl Pts',(26.0973706850791,-17.54661535838,74.091520290779));
#138638=CARTESIAN_POINT('Ctrl Pts',(25.0695200383991,-17.74366607108,74.205156866572));
#138639=CARTESIAN_POINT('Ctrl Pts',(24.0728463316691,-18.06641523507,74.311387761375));
#138640=CARTESIAN_POINT('Ctrl Pts',(23.4314520398391,-18.37286820423,74.376831020544));
#138641=CARTESIAN_POINT('Ctrl Pts',(23.1037448949791,-18.55843326238,74.409426084866));
#138642=CARTESIAN_POINT('Ctrl Pts',(27.3183431738691,-17.49816102492,74.423860311524));
#138643=CARTESIAN_POINT('Ctrl Pts',(26.9491251864291,-17.49012345996,74.509981767913));
#138644=CARTESIAN_POINT('Ctrl Pts',(26.2528371755791,-17.52566114193,74.673916363871));
#138645=CARTESIAN_POINT('Ctrl Pts',(25.2425967226391,-17.71957244634,74.916046457473));
#138646=CARTESIAN_POINT('Ctrl Pts',(24.2650229396191,-18.04208213438,75.154402189595));
#138647=CARTESIAN_POINT('Ctrl Pts',(23.6378329271991,-18.35032103048,75.310373646596));
#138648=CARTESIAN_POINT('Ctrl Pts',(23.3180557494591,-18.5372869207,75.390793748559));
#138649=CARTESIAN_POINT('',(35.8057502945591,-12.95453430026,65.365954576197));
#138650=CARTESIAN_POINT('Origin',(34.5527802604367,-16.4090907755983,58.2598936512312));
#138651=CARTESIAN_POINT('Ctrl Pts',(35.8057502945591,-12.95453430026,65.365954576197));
#138652=CARTESIAN_POINT('Ctrl Pts',(34.9431064727227,-13.6345772355473,
65.8486570716842));
#138653=CARTESIAN_POINT('Ctrl Pts',(34.0393676425824,-14.2331179686743,
66.4149091822397));
#138654=CARTESIAN_POINT('Ctrl Pts',(32.1844391548707,-15.3036240490635,
67.6946158550174));
#138655=CARTESIAN_POINT('Ctrl Pts',(31.2351899347247,-15.7743557463479,
68.4071218684895));
#138656=CARTESIAN_POINT('Ctrl Pts',(29.8938281053855,-16.3687270422503,
69.5547353783046));
#138657=CARTESIAN_POINT('Ctrl Pts',(29.4577386201557,-16.5493254346668,
69.9518867018678));
#138658=CARTESIAN_POINT('Ctrl Pts',(28.6465905917344,-16.8721898444551,
70.7770253045269));
#138659=CARTESIAN_POINT('Ctrl Pts',(28.272150570333,-17.0138051923601,71.2027210720561));
#138660=CARTESIAN_POINT('Ctrl Pts',(27.6399192608511,-17.2504252448796,
72.0812690648473));
#138661=CARTESIAN_POINT('Ctrl Pts',(27.1275711711326,-17.4401614887824,
72.9890886567126));
#138662=CARTESIAN_POINT('Ctrl Pts',(27.0341870140578,-17.5053411484124,
73.896354193606));
#138663=CARTESIAN_POINT('Ctrl Pts',(27.1339039101791,-17.49925933285,74.332577093855));
#138664=CARTESIAN_POINT('Origin',(59.0011724705691,-9.5,68.602980224451));
#138665=CARTESIAN_POINT('',(62.2792373804991,-12.95454545455,60.69796996444));
#138666=CARTESIAN_POINT('',(35.8057502945591,-12.95453430026,65.365954576197));
#138667=CARTESIAN_POINT('',(83.7957739555191,-12.95454545455,56.90402403487));
#138668=CARTESIAN_POINT('Ctrl Pts',(62.2792373804991,-12.95454545455,60.69796996444));
#138669=CARTESIAN_POINT('Ctrl Pts',(63.1166098845742,-13.2847992676022,
60.7108683749086));
#138670=CARTESIAN_POINT('Ctrl Pts',(63.9689235685123,-13.5674612430028,
60.7259621828012));
#138671=CARTESIAN_POINT('Ctrl Pts',(65.2661182929138,-13.9277132722346,
60.7309827347046));
#138672=CARTESIAN_POINT('Ctrl Pts',(65.7016502793716,-14.0372001888285,
60.7297935419239));
#138673=CARTESIAN_POINT('Ctrl Pts',(66.3592990316064,-14.1865988501347,
60.7217316183955));
#138674=CARTESIAN_POINT('Ctrl Pts',(66.5792411470865,-14.2339265143736,
60.7180021287601));
#138675=CARTESIAN_POINT('Ctrl Pts',(66.9102057654576,-14.3013405355391,
60.7106327881737));
#138676=CARTESIAN_POINT('Ctrl Pts',(67.0759510003769,-14.3341531242629,
60.7065047068387));
#138677=CARTESIAN_POINT('Ctrl Pts',(67.2697730572207,-14.3708970404124,
60.700870085725));
#138678=CARTESIAN_POINT('Ctrl Pts',(67.3667963501766,-14.3888880475788,
60.6978430990522));
#138679=CARTESIAN_POINT('Ctrl Pts',(67.4084017239288,-14.3965172099711,
60.6965003542154));
#138680=CARTESIAN_POINT('Ctrl Pts',(67.4361439544228,-14.4015852985429,
60.695595029068));
#138681=CARTESIAN_POINT('Ctrl Pts',(67.4484057161541,-14.4038180465247,
60.6951910547581));
#138682=CARTESIAN_POINT('Ctrl Pts',(68.4551540303067,-14.5863595677202,
60.6616105645986));
#138683=CARTESIAN_POINT('Ctrl Pts',(69.4348882544448,-14.7155633134713,
60.6024403511034));
#138684=CARTESIAN_POINT('Ctrl Pts',(71.3683115020908,-14.8862983920642,
60.4149080274217));
#138685=CARTESIAN_POINT('Ctrl Pts',(72.3204976988778,-14.9279095443246,
60.2868765976002));
#138686=CARTESIAN_POINT('Ctrl Pts',(74.2039596689047,-14.9285030083013,
59.9553280722839));
#138687=CARTESIAN_POINT('Ctrl Pts',(75.1453218737733,-14.8873352533871,
59.7498855938032));
#138688=CARTESIAN_POINT('Ctrl Pts',(76.5575153071471,-14.7597504534288,
59.3862081438027));
#138689=CARTESIAN_POINT('Ctrl Pts',(77.028286125825,-14.7061728352285,59.2558131408953));
#138690=CARTESIAN_POINT('Ctrl Pts',(77.7347308696933,-14.6081459868011,
59.0477656063524));
#138691=CARTESIAN_POINT('Ctrl Pts',(77.9702615694473,-14.5725229325366,
58.976346445346));
#138692=CARTESIAN_POINT('Ctrl Pts',(78.3236696704847,-14.5144985780568,
58.8663303577197));
#138693=CARTESIAN_POINT('Ctrl Pts',(78.5004018391417,-14.4843386444595,
58.810601074487));
#138694=CARTESIAN_POINT('Ctrl Pts',(78.7066481109466,-14.4471035306846,
58.744375483863));
#138695=CARTESIAN_POINT('Ctrl Pts',(78.8097872118071,-14.4279686423323,
58.710967921756));
#138696=CARTESIAN_POINT('Ctrl Pts',(78.8539932439514,-14.4196565580471,
58.6965880207475));
#138697=CARTESIAN_POINT('Ctrl Pts',(78.8834647389532,-14.4140903461361,
58.6869876482371));
#138698=CARTESIAN_POINT('Ctrl Pts',(78.8996931502854,-14.4110104881187,
58.6816931073477));
#138699=CARTESIAN_POINT('Ctrl Pts',(79.7605727753105,-14.2469752542833,
58.4004742082687));
#138700=CARTESIAN_POINT('Ctrl Pts',(80.5901085772675,-14.0487671762514,
58.1075295181658));
#138701=CARTESIAN_POINT('Ctrl Pts',(82.2163488264336,-13.5677992372985,
57.508634771837));
#138702=CARTESIAN_POINT('Ctrl Pts',(83.0130461883228,-13.2849117827013,
57.202644532765));
#138703=CARTESIAN_POINT('Ctrl Pts',(83.7957739555191,-12.95454545455,56.90402403487));
#138704=CARTESIAN_POINT('',(90.6495102260261,-12.9546821942561,55.6952426312692));
#138705=CARTESIAN_POINT('',(57.7481818513162,-12.9545454545498,61.4969173053295));
#138706=CARTESIAN_POINT('Ctrl Pts',(90.6495104561691,-12.95468496338,55.69524393652));
#138707=CARTESIAN_POINT('Ctrl Pts',(90.706441946712,-13.6387734581529,56.018118459155));
#138708=CARTESIAN_POINT('Ctrl Pts',(90.780331398439,-14.2760166331061,56.437166363396));
#138709=CARTESIAN_POINT('Ctrl Pts',(90.9562156145685,-15.4055939966706,
57.4346553206896));
#138710=CARTESIAN_POINT('Ctrl Pts',(91.0581912555219,-15.8978053691709,
58.0129879192721));
#138711=CARTESIAN_POINT('Ctrl Pts',(91.2820561979301,-16.6977190109123,
59.2825890972016));
#138712=CARTESIAN_POINT('Ctrl Pts',(91.4039211591117,-17.0053343075513,
59.9737196359998));
#138713=CARTESIAN_POINT('Ctrl Pts',(91.6577724166921,-17.4112866435593,
61.413381658003));
#138714=CARTESIAN_POINT('Ctrl Pts',(91.7897311124809,-17.5095795447499,
62.1617566103703));
#138715=CARTESIAN_POINT('Ctrl Pts',(91.9214475326691,-17.49925970194,62.90875755409));
#138716=CARTESIAN_POINT('Ctrl Pts',(91.6420024106691,-17.49288371527,63.189055042563));
#138717=CARTESIAN_POINT('Ctrl Pts',(91.4789309706691,-17.53604965052,62.18525541893));
#138718=CARTESIAN_POINT('Ctrl Pts',(91.2383497332691,-17.31061722234,60.70610679257));
#138719=CARTESIAN_POINT('Ctrl Pts',(90.9525691954691,-16.49526955095,58.94317170309));
#138720=CARTESIAN_POINT('Ctrl Pts',(90.7669853930691,-15.69349549193,57.79357798409));
#138721=CARTESIAN_POINT('Ctrl Pts',(90.6082909804691,-14.70024762494,56.8029977009));
#138722=CARTESIAN_POINT('Ctrl Pts',(90.5020501967691,-13.74144627108,56.13084913297));
#138723=CARTESIAN_POINT('Ctrl Pts',(90.4359017985691,-12.91166468527,55.70386232151));
#138724=CARTESIAN_POINT('Ctrl Pts',(90.3919674336691,-12.26996490144,55.41701567738));
#138725=CARTESIAN_POINT('Ctrl Pts',(90.3493777569691,-11.625304524,55.14038529704));
#138726=CARTESIAN_POINT('Ctrl Pts',(90.2953449890691,-10.75812458152,54.79028890356));
#138727=CARTESIAN_POINT('Ctrl Pts',(90.2336264398691,-9.65880570576799,
54.39205929397));
#138728=CARTESIAN_POINT('Ctrl Pts',(90.1482830072691,-7.87135436876299,
53.83794898948));
#138729=CARTESIAN_POINT('Ctrl Pts',(90.0307623522691,-4.60885225935899,
53.06845652345));
#138730=CARTESIAN_POINT('Ctrl Pts',(89.9936931463691,-1.72467127219999,
52.8107295824));
#138731=CARTESIAN_POINT('Ctrl Pts',(89.9978563052691,0.222735690736214,
52.82471929149));
#138732=CARTESIAN_POINT('Ctrl Pts',(92.8080572940691,-17.49304845091,62.97994092861));
#138733=CARTESIAN_POINT('Ctrl Pts',(92.5986172762691,-17.53509776596,62.00204648082));
#138734=CARTESIAN_POINT('Ctrl Pts',(92.2903921564691,-17.31889130207,60.55898006565));
#138735=CARTESIAN_POINT('Ctrl Pts',(91.9177634400691,-16.52369843296,58.82356961024));
#138736=CARTESIAN_POINT('Ctrl Pts',(91.6714076250691,-15.73549484237,57.68441568032));
#138737=CARTESIAN_POINT('Ctrl Pts',(91.4546567603691,-14.75116789232,56.69582182932));
#138738=CARTESIAN_POINT('Ctrl Pts',(91.3031505321691,-13.79449439958,56.02158047907));
#138739=CARTESIAN_POINT('Ctrl Pts',(91.2028409584691,-12.96185490683,55.59044131213));
#138740=CARTESIAN_POINT('Ctrl Pts',(91.1354530153691,-12.32146797839,55.30843405595));
#138741=CARTESIAN_POINT('Ctrl Pts',(91.0705758404691,-11.6762140863,55.03376811453));
#138742=CARTESIAN_POINT('Ctrl Pts',(90.9888550571691,-10.80763428019,54.68635453665));
#138743=CARTESIAN_POINT('Ctrl Pts',(90.8964011661691,-9.70473219682899,
54.29014956107));
#138744=CARTESIAN_POINT('Ctrl Pts',(90.7663353867691,-7.91003779904899,
53.73885583036));
#138745=CARTESIAN_POINT('Ctrl Pts',(90.5830035106691,-4.63059815939199,
52.97296234484));
#138746=CARTESIAN_POINT('Ctrl Pts',(90.5158617110691,-1.73018910792199,
52.71855165387));
#138747=CARTESIAN_POINT('Ctrl Pts',(90.5140275158691,0.223471129680114,
52.733710804));
#138748=CARTESIAN_POINT('Ctrl Pts',(95.0332577554691,-17.49342459549,62.57674230611));
#138749=CARTESIAN_POINT('Ctrl Pts',(94.7353286476691,-17.53141586528,61.64843478555));
#138750=CARTESIAN_POINT('Ctrl Pts',(94.2980272562691,-17.32866592076,60.27452483217));
#138751=CARTESIAN_POINT('Ctrl Pts',(93.7599791478691,-16.56684333187,58.59467001798));
#138752=CARTESIAN_POINT('Ctrl Pts',(93.3979525791691,-15.80201717449,57.4785906808));
#138753=CARTESIAN_POINT('Ctrl Pts',(93.0707154216691,-14.83409351927,56.49734889427));
#138754=CARTESIAN_POINT('Ctrl Pts',(92.8329885552691,-13.88266802702,55.82142820773));
#138755=CARTESIAN_POINT('Ctrl Pts',(92.6675763969691,-13.04676841354,55.38372565059));
#138756=CARTESIAN_POINT('Ctrl Pts',(92.5552464286691,-12.40954656296,55.10962258496));
#138757=CARTESIAN_POINT('Ctrl Pts',(92.4477320239691,-11.76404691488,54.83811150331));
#138758=CARTESIAN_POINT('Ctrl Pts',(92.3130280801691,-10.89384905739,54.49495852328));
#138759=CARTESIAN_POINT('Ctrl Pts',(92.1617766247691,-9.78542268762398,
54.10178266879));
#138760=CARTESIAN_POINT('Ctrl Pts',(91.9461684628691,-7.97909093036199,
53.55434070925));
#138761=CARTESIAN_POINT('Ctrl Pts',(91.6370374276691,-4.67110365588999,
52.79259843176));
#138762=CARTESIAN_POINT('Ctrl Pts',(91.5126238322691,-1.74148283807699,
52.5424907566));
#138763=CARTESIAN_POINT('Ctrl Pts',(91.4993304075691,0.224963289364014,
52.55999381651));
#138764=CARTESIAN_POINT('Ctrl Pts',(98.3120694042691,-17.4936941465,61.94984322819));
#138765=CARTESIAN_POINT('Ctrl Pts',(97.8837093615691,-17.5212766318,61.0958639362));
#138766=CARTESIAN_POINT('Ctrl Pts',(97.2562515863691,-17.32774641508,59.82615794485));
#138767=CARTESIAN_POINT('Ctrl Pts',(96.4754412409691,-16.60157660903,58.23885952741));
#138768=CARTESIAN_POINT('Ctrl Pts',(95.9439265902691,-15.8644449042,57.16729227158));
#138769=CARTESIAN_POINT('Ctrl Pts',(95.4548753321691,-14.91906406746,56.20859012133));
#138770=CARTESIAN_POINT('Ctrl Pts',(95.0906828307691,-13.97865602756,55.53812427992));
#138771=CARTESIAN_POINT('Ctrl Pts',(94.8297011904691,-13.1440013253,55.09570191083));
#138772=CARTESIAN_POINT('Ctrl Pts',(94.6507179597691,-12.51318114468,54.83035115667));
#138773=CARTESIAN_POINT('Ctrl Pts',(94.4801736252691,-11.86966475712,54.56265476203));
#138774=CARTESIAN_POINT('Ctrl Pts',(94.2671175844691,-10.99981417036,54.22446202571));
#138775=CARTESIAN_POINT('Ctrl Pts',(94.0289868932691,-9.88660333602599,
53.83473114943));
#138776=CARTESIAN_POINT('Ctrl Pts',(93.6870297939691,-8.06867605678799,
53.29066962107));
#138777=CARTESIAN_POINT('Ctrl Pts',(93.1923470644691,-4.72817180229899,
52.53047480904));
#138778=CARTESIAN_POINT('Ctrl Pts',(92.9840370488691,-1.75997898553199,
52.28237322324));
#138779=CARTESIAN_POINT('Ctrl Pts',(92.9537597297691,0.227376689111014,
52.30357909855));
#138780=CARTESIAN_POINT('Ctrl Pts',(101.475753876769,-17.49353891402,61.29590415825));
#138781=CARTESIAN_POINT('Ctrl Pts',(100.921566523269,-17.50673774598,60.51582742363));
#138782=CARTESIAN_POINT('Ctrl Pts',(100.110769980169,-17.31202591817,59.35038436406));
#138783=CARTESIAN_POINT('Ctrl Pts',(99.0967857761691,-16.60753119682,57.86441562302));
#138784=CARTESIAN_POINT('Ctrl Pts',(98.4027331908691,-15.89075779816,56.84705199828));
#138785=CARTESIAN_POINT('Ctrl Pts',(97.7585857601691,-14.96553329684,55.92243481635));
#138786=CARTESIAN_POINT('Ctrl Pts',(97.2730114467691,-14.03873742039,55.26579785069));
#138787=CARTESIAN_POINT('Ctrl Pts',(96.9202344708691,-13.21083938854,54.82435903563));
#138788=CARTESIAN_POINT('Ctrl Pts',(96.6766080013691,-12.58779566903,54.56550800276));
#138789=CARTESIAN_POINT('Ctrl Pts',(96.4451267608691,-11.9483583019,54.30142844987));
#138790=CARTESIAN_POINT('Ctrl Pts',(96.1563018818691,-11.08137533143,53.96772273336));
#138791=CARTESIAN_POINT('Ctrl Pts',(95.8342360423691,-9.96667796474999,
53.5814680127));
#138792=CARTESIAN_POINT('Ctrl Pts',(95.3702583734691,-8.14278530794399,
53.04015645856));
#138793=CARTESIAN_POINT('Ctrl Pts',(94.6966275852691,-4.78001234482099,
52.27965897447));
#138794=CARTESIAN_POINT('Ctrl Pts',(94.4079254195691,-1.77918545761499,
52.03051149812));
#138795=CARTESIAN_POINT('Ctrl Pts',(94.3611453799691,0.229858466556014,
52.05546690015));
#138796=CARTESIAN_POINT('Ctrl Pts',(104.620667374569,-17.49157325014,60.55329954308));
#138797=CARTESIAN_POINT('Ctrl Pts',(103.941467294069,-17.49090485743,59.85098416646));
#138798=CARTESIAN_POINT('Ctrl Pts',(102.948693194469,-17.29004011696,58.79633328559));
#138799=CARTESIAN_POINT('Ctrl Pts',(101.704261160469,-16.59820570304,57.42793899511));
#138800=CARTESIAN_POINT('Ctrl Pts',(100.849876330569,-15.89691605225,56.47926166912));
#138801=CARTESIAN_POINT('Ctrl Pts',(100.052867821069,-14.99073822913,55.60442015319));
#138802=CARTESIAN_POINT('Ctrl Pts',(99.4475331754691,-14.08024912469,54.97301510726));
#138803=CARTESIAN_POINT('Ctrl Pts',(99.0041424461691,-13.26410825573,54.54036692231));
#138804=CARTESIAN_POINT('Ctrl Pts',(98.6960975395691,-12.64985632218,54.28771822127));
#138805=CARTESIAN_POINT('Ctrl Pts',(98.4040997745691,-12.01595884731,54.02882577639));
#138806=CARTESIAN_POINT('Ctrl Pts',(98.0400351694691,-11.15329344622,53.70144103815));
#138807=CARTESIAN_POINT('Ctrl Pts',(97.6347501637691,-10.03867108199,53.32138367282));
#138808=CARTESIAN_POINT('Ctrl Pts',(97.0498718249691,-8.21126455271099,
52.78612552645));
#138809=CARTESIAN_POINT('Ctrl Pts',(96.1992866781691,-4.83025156960999,
52.02935312355));
#138810=CARTESIAN_POINT('Ctrl Pts',(95.8317280272691,-1.79882607342499,
51.77865552707));
#138811=CARTESIAN_POINT('Ctrl Pts',(95.7685466593691,0.232387251367314,
51.80735245561));
#138812=CARTESIAN_POINT('Ctrl Pts',(107.205895077569,-17.48792573077,59.79663312451));
#138813=CARTESIAN_POINT('Ctrl Pts',(106.424044375869,-17.47674622014,59.16511196524));
#138814=CARTESIAN_POINT('Ctrl Pts',(105.282107586869,-17.26716418147,58.21289119973));
#138815=CARTESIAN_POINT('Ctrl Pts',(103.849819279169,-16.57860703868,56.96285248062));
#138816=CARTESIAN_POINT('Ctrl Pts',(102.865084831869,-15.8861456528,56.08863860426));
#138817=CARTESIAN_POINT('Ctrl Pts',(101.944004472769,-14.9947548764,55.27363787577));
#138818=CARTESIAN_POINT('Ctrl Pts',(101.241437676969,-14.09987468339,54.67719491956));
#138819=CARTESIAN_POINT('Ctrl Pts',(100.724490474169,-13.29748172548,54.26189382541));
#138820=CARTESIAN_POINT('Ctrl Pts',(100.363674930769,-12.69122630203,54.01677538362));
#138821=CARTESIAN_POINT('Ctrl Pts',(100.022315310469,-12.06297792511,53.76608434928));
#138822=CARTESIAN_POINT('Ctrl Pts',(99.5969390137691,-11.20486683145,53.44885422607));
#138823=CARTESIAN_POINT('Ctrl Pts',(99.1240602916691,-10.09129477713,53.08026985688));
#138824=CARTESIAN_POINT('Ctrl Pts',(98.4411431664691,-8.26255458396299,
52.55881082705));
#138825=CARTESIAN_POINT('Ctrl Pts',(97.4476767384691,-4.86917355379199,
51.81765382124));
#138826=CARTESIAN_POINT('Ctrl Pts',(97.0175172127691,-1.81445742157099,
51.56911198349));
#138827=CARTESIAN_POINT('Ctrl Pts',(96.9414794370691,0.234396340647814,
51.60056027643));
#138828=CARTESIAN_POINT('Ctrl Pts',(109.221122985369,-17.48371428409,59.02301436315));
#138829=CARTESIAN_POINT('Ctrl Pts',(108.359464527669,-17.46369969179,58.45552561474));
#138830=CARTESIAN_POINT('Ctrl Pts',(107.101863410569,-17.2437316127,57.59764899938));
#138831=CARTESIAN_POINT('Ctrl Pts',(105.524816585069,-16.55226120142,56.46376307926));
#138832=CARTESIAN_POINT('Ctrl Pts',(104.439982558469,-15.8637820089,55.66640186783));
#138833=CARTESIAN_POINT('Ctrl Pts',(103.423883984169,-14.98313091293,54.9173947312));
#138834=CARTESIAN_POINT('Ctrl Pts',(102.646954741169,-14.10173774314,54.36322879206));
#138835=CARTESIAN_POINT('Ctrl Pts',(102.073834275069,-13.31262966272,53.97252742131));
#138836=CARTESIAN_POINT('Ctrl Pts',(101.672467124869,-12.71315223001,53.73834234543));
#138837=CARTESIAN_POINT('Ctrl Pts',(101.293368480369,-12.09006135913,53.49997643624));
#138838=CARTESIAN_POINT('Ctrl Pts',(100.821239581369,-11.23624367659,53.19828953843));
#138839=CARTESIAN_POINT('Ctrl Pts',(100.297134086169,-10.12429194288,52.84806009283));
#138840=CARTESIAN_POINT('Ctrl Pts',(99.5401819745691,-8.29592164133099,
52.35088649986));
#138841=CARTESIAN_POINT('Ctrl Pts',(98.4397632280691,-4.89564444717199,
51.64188241625));
#138842=CARTESIAN_POINT('Ctrl Pts',(97.9644657491691,-1.82535986943699,
51.40219236142));
#138843=CARTESIAN_POINT('Ctrl Pts',(97.8800499836691,0.235795394943814,
51.4350616318));
#138844=CARTESIAN_POINT('Ctrl Pts',(110.672701851769,-17.47999766231,58.31037897659));
#138845=CARTESIAN_POINT('Ctrl Pts',(109.753831385769,-17.45278452645,57.79676235383));
#138846=CARTESIAN_POINT('Ctrl Pts',(108.413565659369,-17.22287585739,57.01944774531));
#138847=CARTESIAN_POINT('Ctrl Pts',(106.733762387369,-16.52601355492,55.98868535554));
#138848=CARTESIAN_POINT('Ctrl Pts',(105.578169273769,-15.83872897935,55.26157469267));
#138849=CARTESIAN_POINT('Ctrl Pts',(104.495167177069,-14.96539903947,54.57518563264));
#138850=CARTESIAN_POINT('Ctrl Pts',(103.666047098169,-14.0945150779,54.06328095415));
#138851=CARTESIAN_POINT('Ctrl Pts',(103.053623379069,-13.31645894672,53.69908149772));
#138852=CARTESIAN_POINT('Ctrl Pts',(102.623789120869,-12.72222884999,53.4775456014));
#138853=CARTESIAN_POINT('Ctrl Pts',(102.218370147569,-12.10331314131,53.25326699941));
#138854=CARTESIAN_POINT('Ctrl Pts',(101.713794163769,-11.25304338524,52.96950594007));
#138855=CARTESIAN_POINT('Ctrl Pts',(101.154507689069,-10.14273559401,52.64069966665));
#138856=CARTESIAN_POINT('Ctrl Pts',(100.347069733169,-8.31549541333899,
52.17289680127));
#138857=CARTESIAN_POINT('Ctrl Pts',(99.1749906850691,-4.91197363593599,
51.50467268182));
#138858=CARTESIAN_POINT('Ctrl Pts',(98.6719831015691,-1.83222302500599,
51.27786018261));
#138859=CARTESIAN_POINT('Ctrl Pts',(98.5843312103691,0.236674998269714,
51.31085219334));
#138860=CARTESIAN_POINT('Ctrl Pts',(112.025636097869,-17.47582299445,57.414708358));
#138861=CARTESIAN_POINT('Ctrl Pts',(111.053943881869,-17.44061054217,56.96304883204));
#138862=CARTESIAN_POINT('Ctrl Pts',(109.637726867469,-17.19832466102,56.27986640927));
#138863=CARTESIAN_POINT('Ctrl Pts',(107.864525222969,-16.49257767027,55.37376659663));
#138864=CARTESIAN_POINT('Ctrl Pts',(106.645070431869,-15.8045298653,54.73368567427));
#138865=CARTESIAN_POINT('Ctrl Pts',(105.502119542669,-14.93766113307,54.1273069539));
#138866=CARTESIAN_POINT('Ctrl Pts',(104.626551783569,-14.0776072634,53.6717926103));
#138867=CARTESIAN_POINT('Ctrl Pts',(103.979374836369,-13.31165186547,53.34497834332));
#138868=CARTESIAN_POINT('Ctrl Pts',(103.524307770069,-12.72281268686,53.14263950197));
#138869=CARTESIAN_POINT('Ctrl Pts',(103.095833717869,-12.1083681819,52.93935575519));
#138870=CARTESIAN_POINT('Ctrl Pts',(102.563125775069,-11.2619717921,52.68248156474));
#138871=CARTESIAN_POINT('Ctrl Pts',(101.973995647869,-10.15375628522,52.38598466337));
#138872=CARTESIAN_POINT('Ctrl Pts',(101.124401221169,-8.32857766047699,
51.96347806666));
#138873=CARTESIAN_POINT('Ctrl Pts',(99.8948730883691,-4.92400388437899,
51.35987964448));
#138874=CARTESIAN_POINT('Ctrl Pts',(99.3746000680691,-1.83743471054699,
51.15495885151));
#138875=CARTESIAN_POINT('Ctrl Pts',(99.2892527118691,0.237341712479814,
51.18649555293));
#138876=CARTESIAN_POINT('Ctrl Pts',(113.187878522469,-17.47164537042,56.27521036476));
#138877=CARTESIAN_POINT('Ctrl Pts',(112.171887071169,-17.42782008763,55.896203917));
#138878=CARTESIAN_POINT('Ctrl Pts',(110.692580204369,-17.1709192225,55.32523290978));
#138879=CARTESIAN_POINT('Ctrl Pts',(108.843546518669,-16.45293860262,54.57208052895));
#138880=CARTESIAN_POINT('Ctrl Pts',(107.573079972769,-15.7622252762,54.04093228966));
#138881=CARTESIAN_POINT('Ctrl Pts',(106.383104391469,-14.90097081599,53.53723091173));
#138882=CARTESIAN_POINT('Ctrl Pts',(105.471805752069,-14.05204799653,53.15666631614));
#138883=CARTESIAN_POINT('Ctrl Pts',(104.798395092669,-13.29921052309,52.88163095715));
#138884=CARTESIAN_POINT('Ctrl Pts',(104.324299692669,-12.7158750262,52.70763929966));
#138885=CARTESIAN_POINT('Ctrl Pts',(103.878996809469,-12.10616052631,52.53481596519));
#138886=CARTESIAN_POINT('Ctrl Pts',(103.326404821569,-11.26390566317,52.3171231399));
#138887=CARTESIAN_POINT('Ctrl Pts',(102.717650256469,-10.15814664048,52.06780970547));
#138888=CARTESIAN_POINT('Ctrl Pts',(101.841943206069,-8.33580711274199,
51.71237805453));
#138889=CARTESIAN_POINT('Ctrl Pts',(100.582660234469,-4.93206689688699,
51.20591871564));
#138890=CARTESIAN_POINT('Ctrl Pts',(100.066369699469,-1.84107769572599,
51.03478661238));
#138891=CARTESIAN_POINT('Ctrl Pts',(99.9955853506691,0.237806588570414,
51.06184068411));
#138892=CARTESIAN_POINT('Ctrl Pts',(114.125295566369,-17.4681686409,54.80495076776));
#138893=CARTESIAN_POINT('Ctrl Pts',(113.075609260269,-17.41485113758,54.51458434375));
#138894=CARTESIAN_POINT('Ctrl Pts',(111.549286453269,-17.14048950455,54.08233649879));
#138895=CARTESIAN_POINT('Ctrl Pts',(109.646785590869,-16.40654507693,53.5223372395));
#138896=CARTESIAN_POINT('Ctrl Pts',(108.341891044269,-15.7114208792,53.13068024962));
#138897=CARTESIAN_POINT('Ctrl Pts',(107.121834027869,-14.85569373811,52.76062809666));
#138898=CARTESIAN_POINT('Ctrl Pts',(106.189106230169,-14.01930261972,52.47974204073));
#138899=CARTESIAN_POINT('Ctrl Pts',(105.501006553569,-13.28178778393,52.27521181241));
#138900=CARTESIAN_POINT('Ctrl Pts',(105.016385994269,-12.70458531254,52.14111418883));
#138901=CARTESIAN_POINT('Ctrl Pts',(104.562932235469,-12.10030644958,52.0107829688));
#138902=CARTESIAN_POINT('Ctrl Pts',(104.002143959169,-11.26286251636,51.84785983031));
#138903=CARTESIAN_POINT('Ctrl Pts',(103.388634838669,-10.16016220358,51.66454860331));
#138904=CARTESIAN_POINT('Ctrl Pts',(102.510622200469,-8.34157678397199,
51.40350477807));
#138905=CARTESIAN_POINT('Ctrl Pts',(101.264203967269,-4.93999503540199,
51.03437280106));
#138906=CARTESIAN_POINT('Ctrl Pts',(100.787671277369,-1.84502963773899,
50.91043632241));
#138907=CARTESIAN_POINT('Ctrl Pts',(100.754059746769,0.238308208433314,
50.92792952439));
#138908=CARTESIAN_POINT('Ctrl Pts',(114.538941011169,-17.46718763232,53.67900430315));
#138909=CARTESIAN_POINT('Ctrl Pts',(113.476435304769,-17.40728503982,53.4545371021));
#138910=CARTESIAN_POINT('Ctrl Pts',(111.933157162869,-17.11989097826,53.12631997973));
#138911=CARTESIAN_POINT('Ctrl Pts',(110.014547047469,-16.37339715948,52.71350806941));
#138912=CARTESIAN_POINT('Ctrl Pts',(108.700990537169,-15.67453448001,52.42915265115));
#138913=CARTESIAN_POINT('Ctrl Pts',(107.475303053069,-14.82273438004,52.1628920189));
#138914=CARTESIAN_POINT('Ctrl Pts',(106.540338441969,-13.9958275305,51.96016673408));
#138915=CARTESIAN_POINT('Ctrl Pts',(105.852098050869,-13.2701199685,51.81147738317));
#138916=CARTESIAN_POINT('Ctrl Pts',(105.367562667669,-12.69751801236,51.70901280385));
#138917=CARTESIAN_POINT('Ctrl Pts',(104.915851437869,-12.09743795773,51.61240634049));
#138918=CARTESIAN_POINT('Ctrl Pts',(104.359190902469,-11.26379112788,51.49296213066));
#138919=CARTESIAN_POINT('Ctrl Pts',(103.754568792369,-10.16369897044,51.36207880897));
#138920=CARTESIAN_POINT('Ctrl Pts',(102.894237682569,-8.34833379260699,
51.17605601973));
#138921=CARTESIAN_POINT('Ctrl Pts',(101.690547221869,-4.94875211867199,
50.9158704599));
#138922=CARTESIAN_POINT('Ctrl Pts',(101.268979997669,-1.84978703934099,
50.82795858552));
#138923=CARTESIAN_POINT('Ctrl Pts',(101.278306971269,0.238909531620114,
50.8353458769));
#138924=CARTESIAN_POINT('Ctrl Pts',(114.721732415669,-17.46709263224,53.0511844563));
#138925=CARTESIAN_POINT('Ctrl Pts',(113.654169992369,-17.40357906045,52.86327469701));
#138926=CARTESIAN_POINT('Ctrl Pts',(112.104502884069,-17.10880738315,52.59289088903));
#138927=CARTESIAN_POINT('Ctrl Pts',(110.180954315469,-16.35510969368,52.262432252));
#138928=CARTESIAN_POINT('Ctrl Pts',(108.865472379469,-15.65410379572,52.03831580661));
#138929=CARTESIAN_POINT('Ctrl Pts',(107.639522339869,-14.80461369374,51.83047343371));
#138930=CARTESIAN_POINT('Ctrl Pts',(106.705667287469,-13.98326026859,51.67177167508));
#138931=CARTESIAN_POINT('Ctrl Pts',(106.019208150569,-13.26447423575,51.55455277005));
#138932=CARTESIAN_POINT('Ctrl Pts',(105.536071241069,-12.69456042945,51.46969752251));
#138933=CARTESIAN_POINT('Ctrl Pts',(105.086676320869,-12.0969679499,51.39195280225));
#138934=CARTESIAN_POINT('Ctrl Pts',(104.534087620169,-11.26560740794,51.29681409481));
#138935=CARTESIAN_POINT('Ctrl Pts',(103.936593793969,-10.16715557418,51.19525657912));
#138936=CARTESIAN_POINT('Ctrl Pts',(103.089545611369,-8.35379901046899,
51.05114625581));
#138937=CARTESIAN_POINT('Ctrl Pts',(101.915641479169,-4.95541766429799,
50.85167914844));
#138938=CARTESIAN_POINT('Ctrl Pts',(101.529528153669,-1.85347919288199,
50.78336850669));
#138939=CARTESIAN_POINT('Ctrl Pts',(101.565834799469,0.239375795559914,
50.78456512074));
#138940=CARTESIAN_POINT('',(90.1947786764252,-4.3867443600625,53.116590296774));
#138941=CARTESIAN_POINT('Origin',(94.1058924693563,-2.20522353149594,75.3038953413698));
#138942=CARTESIAN_POINT('Ctrl Pts',(90.7329498186947,1.32709932748619E-14,
52.6942605482205));
#138943=CARTESIAN_POINT('Ctrl Pts',(90.7324767382983,-0.227253860817282,
52.6943439650584));
#138944=CARTESIAN_POINT('Ctrl Pts',(90.7281184789287,-0.4477491549907,52.6977472020605));
#138945=CARTESIAN_POINT('Ctrl Pts',(90.720392835498,-0.661516881487571,
52.7039174767894));
#138946=CARTESIAN_POINT('Ctrl Pts',(90.7127053559675,-0.874228616956188,
52.7100572709829));
#138947=CARTESIAN_POINT('Ctrl Pts',(90.7016821327591,-1.08027904536049,
52.7189370153821));
#138948=CARTESIAN_POINT('Ctrl Pts',(90.6878356425394,-1.27973268978521,
52.7300489221175));
#138949=CARTESIAN_POINT('Ctrl Pts',(90.6742009569423,-1.47613536582651,
52.7409908541391));
#138950=CARTESIAN_POINT('Ctrl Pts',(90.6578277551231,-1.66614171826471,
52.7540973949353));
#138951=CARTESIAN_POINT('Ctrl Pts',(90.6392259463126,-1.84984509104067,
52.7689165193269));
#138952=CARTESIAN_POINT('Ctrl Pts',(90.620895075782,-2.03087279521278,52.7835198008339));
#138953=CARTESIAN_POINT('Ctrl Pts',(90.6003995142314,-2.20578003978867,
52.7997863319174));
#138954=CARTESIAN_POINT('Ctrl Pts',(90.5782581940087,-2.37468392683479,
52.8173127062458));
#138955=CARTESIAN_POINT('Ctrl Pts',(90.5706889802761,-2.43242527235826,
52.8233042583265));
#138956=CARTESIAN_POINT('Ctrl Pts',(90.5629277330407,-2.4894652436943,52.829443286268));
#138957=CARTESIAN_POINT('Ctrl Pts',(90.5549961696083,-2.54580919563397,
52.8357144107448));
#138958=CARTESIAN_POINT('Ctrl Pts',(90.5293422811424,-2.72804835580788,
52.8559977671417));
#138959=CARTESIAN_POINT('Ctrl Pts',(90.5019355821923,-2.90298378034419,
52.8776533385827));
#138960=CARTESIAN_POINT('Ctrl Pts',(90.4732449116748,-3.0706739713582,52.9002213305575));
#138961=CARTESIAN_POINT('Ctrl Pts',(90.4457229651428,-3.23153324678687,
52.9218700078892));
#138962=CARTESIAN_POINT('Ctrl Pts',(90.4170197258856,-3.38572597691061,
52.9443585273677));
#138963=CARTESIAN_POINT('Ctrl Pts',(90.3875915344632,-3.53332619020803,
52.9673069738302));
#138964=CARTESIAN_POINT('Ctrl Pts',(90.3562888335583,-3.69032820450255,
52.9917171846222));
#138965=CARTESIAN_POINT('Ctrl Pts',(90.3241654812914,-3.83987120261895,
53.0166475416299));
#138966=CARTESIAN_POINT('Ctrl Pts',(90.2918223241181,-3.982066449326,53.0416713166677));
#138967=CARTESIAN_POINT('Ctrl Pts',(90.2594791669447,-4.12426169603305,
53.0666950917055));
#138968=CARTESIAN_POINT('Ctrl Pts',(90.2269165313409,-4.2591095417022,53.0918123452299));
#138969=CARTESIAN_POINT('Ctrl Pts',(90.1947851173379,-4.38673887645801,
53.1166268251324));
#138970=CARTESIAN_POINT('Ctrl Pts',(114.384013133501,-17.4511087443003,
53.3319432235761));
#138971=CARTESIAN_POINT('Ctrl Pts',(113.233237036033,-17.3623045655773,
53.108253902328));
#138972=CARTESIAN_POINT('Ctrl Pts',(112.09731983445,-17.1143644848258,52.8874528876658));
#138973=CARTESIAN_POINT('Ctrl Pts',(109.922039526642,-16.3121265262524,
52.4646191965448));
#138974=CARTESIAN_POINT('Ctrl Pts',(108.894477527575,-15.7640445013132,
52.2648804337895));
#138975=CARTESIAN_POINT('Ctrl Pts',(106.479013465885,-14.0118510024043,
51.7953596092692));
#138976=CARTESIAN_POINT('Ctrl Pts',(105.376412094549,-12.7334337065386,
51.5810346680078));
#138977=CARTESIAN_POINT('Ctrl Pts',(104.030863071798,-10.5823199299919,
51.3194853359339));
#138978=CARTESIAN_POINT('Ctrl Pts',(103.183629676098,-8.98529837677913,
51.1547991792561));
#138979=CARTESIAN_POINT('Ctrl Pts',(101.788452456429,-4.71138061603123,
50.8836032601707));
#138980=CARTESIAN_POINT('Ctrl Pts',(101.414232739431,-2.35682621946771,
50.8108621807075));
#138981=CARTESIAN_POINT('Ctrl Pts',(101.414232124315,-1.74205094793933E-11,
50.81086228917));
#138982=CARTESIAN_POINT('Origin',(119.365530515369,-0.00786869443873679,
54.30025863205));
#138983=CARTESIAN_POINT('Origin',(115.383008995769,1.4210854715202E-14,
59.12907384506));
#138984=CARTESIAN_POINT('Origin',(114.333554474769,1.4210854715202E-14,
64.528022373109));
#138985=CARTESIAN_POINT('Origin',(127.392589630769,111.0726804259,69.613246531288));
#138986=CARTESIAN_POINT('',(105.588267882983,12.0114366406,65.3748945993009));
#138987=CARTESIAN_POINT('Ctrl Pts',(113.836120912569,9.49997724965368,66.9781228011004));
#138988=CARTESIAN_POINT('Ctrl Pts',(113.620040676569,9.60407357720701,66.93612084843));
#138989=CARTESIAN_POINT('Ctrl Pts',(113.204036263969,9.79597941773501,66.855257378578));
#138990=CARTESIAN_POINT('Ctrl Pts',(112.634681946869,10.03993468234,66.744585558129));
#138991=CARTESIAN_POINT('Ctrl Pts',(112.112598449869,10.24927512774,66.643102300151));
#138992=CARTESIAN_POINT('Ctrl Pts',(111.632740031669,10.43041782041,66.549826807009));
#138993=CARTESIAN_POINT('Ctrl Pts',(111.191763777969,10.58798094238,66.464109278743));
#138994=CARTESIAN_POINT('Ctrl Pts',(110.785976678169,10.72587566292,66.385231863232));
#138995=CARTESIAN_POINT('Ctrl Pts',(110.412223632669,10.84718057429,66.312581268166));
#138996=CARTESIAN_POINT('Ctrl Pts',(110.067718345869,10.95437259849,66.245615889834));
#138997=CARTESIAN_POINT('Ctrl Pts',(109.749884820369,11.04949448021,66.183835002597));
#138998=CARTESIAN_POINT('Ctrl Pts',(109.456458641569,11.13421861423,66.126798446613));
#138999=CARTESIAN_POINT('Ctrl Pts',(109.185588771969,11.20988394979,66.07414641488));
#139000=CARTESIAN_POINT('Ctrl Pts',(108.935411166069,11.27766781735,66.025516571843));
#139001=CARTESIAN_POINT('Ctrl Pts',(108.703758242769,11.33868509469,65.980487580283));
#139002=CARTESIAN_POINT('Ctrl Pts',(108.488694360169,11.39387414376,65.938683187692));
#139003=CARTESIAN_POINT('Ctrl Pts',(108.289535310269,11.44377147107,65.899970396824));
#139004=CARTESIAN_POINT('Ctrl Pts',(108.106685536769,11.48858911862,65.864427823957));
#139005=CARTESIAN_POINT('Ctrl Pts',(107.939918988669,11.52866255842,65.832011529019));
#139006=CARTESIAN_POINT('Ctrl Pts',(107.786401064769,11.56489565973,65.802170518592));
#139007=CARTESIAN_POINT('Ctrl Pts',(107.641419490569,11.59853026744,65.773988814747));
#139008=CARTESIAN_POINT('Ctrl Pts',(107.500358765169,11.63070709409,65.746569250508));
#139009=CARTESIAN_POINT('Ctrl Pts',(107.359302140969,11.66233303899,65.71915048345));
#139010=CARTESIAN_POINT('Ctrl Pts',(107.215797620369,11.69395150831,65.69125589119));
#139011=CARTESIAN_POINT('Ctrl Pts',(107.070978664869,11.72524102839,65.663105797358));
#139012=CARTESIAN_POINT('Ctrl Pts',(106.931199149369,11.75497438103,65.635935276346));
#139013=CARTESIAN_POINT('Ctrl Pts',(106.798191632069,11.78293756265,65.610081104993));
#139014=CARTESIAN_POINT('Ctrl Pts',(106.662552223669,11.81149846886,65.583715343288));
#139015=CARTESIAN_POINT('Ctrl Pts',(106.522208287369,11.84046944262,65.556435109417));
#139016=CARTESIAN_POINT('Ctrl Pts',(106.395784786269,11.86721276223,65.531860747577));
#139017=CARTESIAN_POINT('Ctrl Pts',(106.283189021069,11.88761641784,65.509974238645));
#139018=CARTESIAN_POINT('Ctrl Pts',(106.148953995269,11.91021050843,65.483881462854));
#139019=CARTESIAN_POINT('Ctrl Pts',(106.010964934269,11.93474309679,65.457058971809));
#139020=CARTESIAN_POINT('Ctrl Pts',(105.873653901269,11.95937571227,65.430368280779));
#139021=CARTESIAN_POINT('Ctrl Pts',(105.728095742226,11.9858864817682,65.4020744876716));
#139022=CARTESIAN_POINT('Ctrl Pts',(105.63481165757,12.0031744376127,65.3839418377354));
#139023=CARTESIAN_POINT('Ctrl Pts',(105.588267881069,12.0114366406,65.374894609145));
#139024=CARTESIAN_POINT('',(98.6413355775134,12.9603923092705,64.0245406081078));
#139025=CARTESIAN_POINT('Ctrl Pts',(105.58826788679,12.0114366406,65.3748945797136));
#139026=CARTESIAN_POINT('Ctrl Pts',(105.487707106476,12.02927489928,65.3553474466039));
#139027=CARTESIAN_POINT('Ctrl Pts',(105.382844695789,12.04788335748,65.33496415708));
#139028=CARTESIAN_POINT('Ctrl Pts',(105.273811991669,12.0668309774183,65.313770240584));
#139029=CARTESIAN_POINT('Ctrl Pts',(105.164779287549,12.0857785973567,65.292576324088));
#139030=CARTESIAN_POINT('Ctrl Pts',(105.051576289995,12.1050653790333,65.27057178062));
#139031=CARTESIAN_POINT('Ctrl Pts',(104.933545944418,12.124934015645,65.2476288910684));
#139032=CARTESIAN_POINT('Ctrl Pts',(104.815515598841,12.1448026522567,65.2246860015167));
#139033=CARTESIAN_POINT('Ctrl Pts',(104.692657905241,12.1652531438033,65.2008047658813));
#139034=CARTESIAN_POINT('Ctrl Pts',(104.564552226669,12.18625012801,65.1759034202142));
#139035=CARTESIAN_POINT('Ctrl Pts',(104.436446548096,12.2072471122166,65.151002074547));
#139036=CARTESIAN_POINT('Ctrl Pts',(104.303092884551,12.2287905890833,65.1250806188479));
#139037=CARTESIAN_POINT('Ctrl Pts',(104.164040162969,12.2509033469583,65.0980513729576));
#139038=CARTESIAN_POINT('Ctrl Pts',(104.024987441387,12.2730161048333,65.0710221270673));
#139039=CARTESIAN_POINT('Ctrl Pts',(103.880235661768,12.2956981437167,65.0428850909858));
#139040=CARTESIAN_POINT('Ctrl Pts',(103.72930921272,12.3189383132283,65.0135478147625));
#139041=CARTESIAN_POINT('Ctrl Pts',(103.578382763673,12.34217848274,64.9842105385393));
#139042=CARTESIAN_POINT('Ctrl Pts',(103.421281645198,12.36597678288,64.9536730221743));
#139043=CARTESIAN_POINT('Ctrl Pts',(103.257490308254,12.390312007255,64.9218350525855));
#139044=CARTESIAN_POINT('Ctrl Pts',(103.09369897131,12.41464723163,64.8899970829968));
#139045=CARTESIAN_POINT('Ctrl Pts',(102.923217415897,12.43951938024,64.8568586601843));
#139046=CARTESIAN_POINT('Ctrl Pts',(102.745520526753,12.4648904812933,64.8223177115716));
#139047=CARTESIAN_POINT('Ctrl Pts',(102.567823637608,12.4902615823466,64.7877767629589));
#139048=CARTESIAN_POINT('Ctrl Pts',(102.382911414733,12.5161316358433,64.751833288546));
#139049=CARTESIAN_POINT('Ctrl Pts',(102.190273102186,12.5424417096733,64.7143880069401));
#139050=CARTESIAN_POINT('Ctrl Pts',(101.997634789639,12.5687517835033,64.6769427253342));
#139051=CARTESIAN_POINT('Ctrl Pts',(101.797270387422,12.5955018776666,64.6379956365352));
#139052=CARTESIAN_POINT('Ctrl Pts',(101.588727810885,12.6226092695767,64.5974588637509));
#139053=CARTESIAN_POINT('Ctrl Pts',(101.380185234348,12.6497166614867,64.5569220909665));
#139054=CARTESIAN_POINT('Ctrl Pts',(101.163464483491,12.6771813511433,64.5147956341968));
#139055=CARTESIAN_POINT('Ctrl Pts',(100.937832557286,12.7049367835767,64.4709370117642));
#139056=CARTESIAN_POINT('Ctrl Pts',(100.712200631081,12.73269221601,64.4270783893316));
#139057=CARTESIAN_POINT('Ctrl Pts',(100.477657529529,12.76073839122,64.3814876012362));
#139058=CARTESIAN_POINT('Ctrl Pts',(100.233364830254,12.7889966418833,64.3340016738643));
#139059=CARTESIAN_POINT('Ctrl Pts',(99.9890721309782,12.8172548925466,64.2865157464924));
#139060=CARTESIAN_POINT('Ctrl Pts',(99.7350298339805,12.8457252186633,64.237134679844));
#139061=CARTESIAN_POINT('Ctrl Pts',(99.4698469210946,12.8743478680941,64.1855880860287));
#139062=CARTESIAN_POINT('Ctrl Pts',(99.2046640082087,12.902970517525,64.1340414922134));
#139063=CARTESIAN_POINT('Ctrl Pts',(98.9283404794346,12.93174549027,64.0803293712313));
#139064=CARTESIAN_POINT('Ctrl Pts',(98.6413355057347,12.96039230927,64.0245409773214));
#139065=CARTESIAN_POINT('',(98.6413368503852,-12.9603921337551,64.0245393914519));
#139066=CARTESIAN_POINT('',(98.6413367350691,-12.96039213374,64.024539984441));
#139067=CARTESIAN_POINT('',(105.588202589909,-12.0114482303,65.3748819076663));
#139068=CARTESIAN_POINT('Ctrl Pts',(98.6413365043404,-12.96039213374,64.0245411714316));
#139069=CARTESIAN_POINT('Ctrl Pts',(98.9288825599428,-12.93169130878,64.0804347415339));
#139070=CARTESIAN_POINT('Ctrl Pts',(99.205691626796,-12.902863377555,64.1342412420289));
#139071=CARTESIAN_POINT('Ctrl Pts',(99.4712969064103,-12.8741913427442,
64.1858699360291));
#139072=CARTESIAN_POINT('Ctrl Pts',(99.7369021860247,-12.8455193079333,
64.2374986300293));
#139073=CARTESIAN_POINT('Ctrl Pts',(99.9913036784002,-12.8170031695366,
64.2869495175347));
#139074=CARTESIAN_POINT('Ctrl Pts',(100.235912932002,-12.7887018706566,
64.3344969771415));
#139075=CARTESIAN_POINT('Ctrl Pts',(100.480522185603,-12.7604005717767,
64.3820444367482));
#139076=CARTESIAN_POINT('Ctrl Pts',(100.715339200429,-12.7323141124133,
64.4276884684562));
#139077=CARTESIAN_POINT('Ctrl Pts',(100.941205307535,-12.70452182889,64.4715926112718));
#139078=CARTESIAN_POINT('Ctrl Pts',(101.167071414641,-12.6767295453667,
64.5154967540875));
#139079=CARTESIAN_POINT('Ctrl Pts',(101.383986614025,-12.6492314376833,
64.5576610080107));
#139080=CARTESIAN_POINT('Ctrl Pts',(101.592689687186,-12.62209420599,64.598228978334));
#139081=CARTESIAN_POINT('Ctrl Pts',(101.801392760346,-12.5949569742967,
64.6387969486573));
#139082=CARTESIAN_POINT('Ctrl Pts',(102.001883707283,-12.5681806185933,
64.6777686353807));
#139083=CARTESIAN_POINT('Ctrl Pts',(102.194610984735,-12.5418491480417,
64.7152312100988));
#139084=CARTESIAN_POINT('Ctrl Pts',(102.387338262187,-12.51551767749,64.7526937848169));
#139085=CARTESIAN_POINT('Ctrl Pts',(102.572301870154,-12.48963109209,64.7886472475296));
#139086=CARTESIAN_POINT('Ctrl Pts',(102.75001504787,-12.4642486645433,64.8231913623356));
#139087=CARTESIAN_POINT('Ctrl Pts',(102.927728225585,-12.4388662369967,
64.8577354771415));
#139088=CARTESIAN_POINT('Ctrl Pts',(103.098190973049,-12.4139879673033,
64.8908702440408));
#139089=CARTESIAN_POINT('Ctrl Pts',(103.26192990282,-12.3896522645967,64.9226980266562));
#139090=CARTESIAN_POINT('Ctrl Pts',(103.425668832591,-12.36531656189,64.9545258092716));
#139091=CARTESIAN_POINT('Ctrl Pts',(103.58268394467,-12.34152342617,64.9850466076032));
#139092=CARTESIAN_POINT('Ctrl Pts',(103.733490737885,-12.3182943905,65.0143606249728));
#139093=CARTESIAN_POINT('Ctrl Pts',(103.884297531101,-12.29506535483,65.0436746423425));
#139094=CARTESIAN_POINT('Ctrl Pts',(104.028896005453,-12.27240041921,65.07178187875));
#139095=CARTESIAN_POINT('Ctrl Pts',(104.167764032385,-12.2503109256767,
65.0987752234581));
#139096=CARTESIAN_POINT('Ctrl Pts',(104.306632059317,-12.2282214321433,
65.1257685681661));
#139097=CARTESIAN_POINT('Ctrl Pts',(104.43976963883,-12.2067073806967,65.1516480211745));
#139098=CARTESIAN_POINT('Ctrl Pts',(104.567626845804,-12.18574629921,65.1765010686145));
#139099=CARTESIAN_POINT('Ctrl Pts',(104.695484052777,-12.1647852177233,
65.2013541160545));
#139100=CARTESIAN_POINT('Ctrl Pts',(104.818060887212,-12.1443771061967,
65.2251807579259));
#139101=CARTESIAN_POINT('Ctrl Pts',(104.935782035903,-12.1245571421584,
65.2480635453915));
#139102=CARTESIAN_POINT('Ctrl Pts',(105.053503184595,-12.10473717812,65.270946332857));
#139103=CARTESIAN_POINT('Ctrl Pts',(105.166368647542,-12.08550536157,65.2928852659166));
#139104=CARTESIAN_POINT('Ctrl Pts',(105.275029300469,-12.0666203373025,
65.3140068626255));
#139105=CARTESIAN_POINT('Ctrl Pts',(105.38367608427,-12.0477377234637,65.3351257634363));
#139106=CARTESIAN_POINT('Ctrl Pts',(105.48811913136,-12.0292018133859,65.355427536528));
#139107=CARTESIAN_POINT('Ctrl Pts',(105.588202593739,-12.0114482303,65.3748818879668));
#139108=CARTESIAN_POINT('Ctrl Pts',(105.588202587969,-12.0114482303,65.374881917649));
#139109=CARTESIAN_POINT('Ctrl Pts',(105.632442653569,-12.00359419922,65.383481347831));
#139110=CARTESIAN_POINT('Ctrl Pts',(105.721776657069,-11.98704471645,65.400846175769));
#139111=CARTESIAN_POINT('Ctrl Pts',(105.857335799669,-11.96236204966,65.427196347343));
#139112=CARTESIAN_POINT('Ctrl Pts',(105.999371892069,-11.93673375387,65.454805501442));
#139113=CARTESIAN_POINT('Ctrl Pts',(106.145157650769,-11.91101631839,65.483143524557));
#139114=CARTESIAN_POINT('Ctrl Pts',(106.286567143069,-11.8867305141,65.510630882327));
#139115=CARTESIAN_POINT('Ctrl Pts',(106.385566014869,-11.86929321032,65.529874409723));
#139116=CARTESIAN_POINT('Ctrl Pts',(106.517821024969,-11.84141156517,65.555582307755));
#139117=CARTESIAN_POINT('Ctrl Pts',(106.652849454469,-11.81350628447,65.581829306601));
#139118=CARTESIAN_POINT('Ctrl Pts',(106.786531700769,-11.78539623009,65.607814632638));
#139119=CARTESIAN_POINT('Ctrl Pts',(106.926031207269,-11.7560666564,65.634930725157));
#139120=CARTESIAN_POINT('Ctrl Pts',(107.076045936069,-11.72417565916,65.664090780018));
#139121=CARTESIAN_POINT('Ctrl Pts',(107.238877334269,-11.68894114187,65.69574215549));
#139122=CARTESIAN_POINT('Ctrl Pts',(107.415915338069,-11.64977112412,65.730155029124));
#139123=CARTESIAN_POINT('Ctrl Pts',(107.608289198369,-11.60622911253,65.76754890617));
#139124=CARTESIAN_POINT('Ctrl Pts',(107.816920752269,-11.55785278626,65.808102974495));
#139125=CARTESIAN_POINT('Ctrl Pts',(108.042414036969,-11.50424165311,65.851934647601));
#139126=CARTESIAN_POINT('Ctrl Pts',(108.284998613969,-11.44502211087,65.899088547989));
#139127=CARTESIAN_POINT('Ctrl Pts',(108.546207263869,-11.37939218241,65.949862619481));
#139128=CARTESIAN_POINT('Ctrl Pts',(108.827816386469,-11.30637676569,66.00460216095));
#139129=CARTESIAN_POINT('Ctrl Pts',(109.131558670969,-11.22487329816,66.06364397474));
#139130=CARTESIAN_POINT('Ctrl Pts',(109.459041432369,-11.13368566555,66.127300492802));
#139131=CARTESIAN_POINT('Ctrl Pts',(109.812187865869,-11.03134799395,66.195945548277));
#139132=CARTESIAN_POINT('Ctrl Pts',(110.193003524769,-10.91613450448,66.269968983176));
#139133=CARTESIAN_POINT('Ctrl Pts',(110.603674207869,-10.78597589075,66.349795675867));
#139134=CARTESIAN_POINT('Ctrl Pts',(111.046481677169,-10.63839916197,66.435869158151));
#139135=CARTESIAN_POINT('Ctrl Pts',(111.523670537969,-10.47046824764,66.52862573931));
#139136=CARTESIAN_POINT('Ctrl Pts',(112.038227405869,-10.2783509173,66.628645961495));
#139137=CARTESIAN_POINT('Ctrl Pts',(112.591679391169,-10.05799574284,66.736226666351));
#139138=CARTESIAN_POINT('Ctrl Pts',(113.187817592569,-9.80343559038099,
66.852104772485));
#139139=CARTESIAN_POINT('Ctrl Pts',(113.615465209669,-9.60627779281199,
66.935231463316));
#139140=CARTESIAN_POINT('Ctrl Pts',(113.83612107687,-9.49997725001998,66.9781228330329));
#139141=CARTESIAN_POINT('Origin',(113.570314823169,1.4210854715202E-14,
68.454530393505));
#139142=CARTESIAN_POINT('',(122.781534122803,0.000146553545601451,70.2450189834913));
#139143=CARTESIAN_POINT('Ctrl Pts',(122.781532931853,0.000146553553284748,
70.2450187519928));
#139144=CARTESIAN_POINT('Ctrl Pts',(122.781531239529,-0.0353745236476723,
70.2450184230429));
#139145=CARTESIAN_POINT('Ctrl Pts',(122.78124053361,-0.0707835449077734,
70.2449619152538));
#139146=CARTESIAN_POINT('Ctrl Pts',(122.780675137493,-0.106083713974549,
70.244852012833));
#139147=CARTESIAN_POINT('Ctrl Pts',(122.779055732123,-0.207190321579809,
70.2445372307447));
#139148=CARTESIAN_POINT('Ctrl Pts',(122.775182872892,-0.307404002211838,
70.2437844194156));
#139149=CARTESIAN_POINT('Ctrl Pts',(122.769316063091,-0.406807871668896,
70.242644021423));
#139150=CARTESIAN_POINT('Ctrl Pts',(122.762871839682,-0.515995107010533,
70.2413913850348));
#139151=CARTESIAN_POINT('Ctrl Pts',(122.754021860444,-0.624205283049368,
70.2396711147501));
#139152=CARTESIAN_POINT('Ctrl Pts',(122.743027927957,-0.731526461212833,
70.2375341000902));
#139153=CARTESIAN_POINT('Ctrl Pts',(122.73094004789,-0.849526597371243,
70.2351844425004));
#139154=CARTESIAN_POINT('Ctrl Pts',(122.716260320207,-0.966452014654131,
70.2323309782551));
#139155=CARTESIAN_POINT('Ctrl Pts',(122.699248023636,-1.08240084256692,
70.2290241062858));
#139156=CARTESIAN_POINT('Ctrl Pts',(122.680554797463,-1.20980619642746,
70.2253904930703));
#139157=CARTESIAN_POINT('Ctrl Pts',(122.659045282996,-1.33603243947,70.2212094461342));
#139158=CARTESIAN_POINT('Ctrl Pts',(122.63497587133,-1.4611770396468,70.2165308031054));
#139159=CARTESIAN_POINT('Ctrl Pts',(122.608557608206,-1.59853407279087,
70.2113955873257));
#139160=CARTESIAN_POINT('Ctrl Pts',(122.579055446421,-1.73458805478684,
70.2056609193789));
#139161=CARTESIAN_POINT('Ctrl Pts',(122.546669333643,-1.86950917679617,
70.1993656653502));
#139162=CARTESIAN_POINT('Ctrl Pts',(122.511169293522,-2.01740297551294,
70.1924651221414));
#139163=CARTESIAN_POINT('Ctrl Pts',(122.472204056511,-2.16393559197889,
70.1848910095296));
#139164=CARTESIAN_POINT('Ctrl Pts',(122.429982407261,-2.30908823163419,
70.1766839113411));
#139165=CARTESIAN_POINT('Ctrl Pts',(122.383764360875,-2.46797997442484,
70.1676999883651));
#139166=CARTESIAN_POINT('Ctrl Pts',(122.333644270515,-2.62521813965719,
70.1579575810896));
#139167=CARTESIAN_POINT('Ctrl Pts',(122.279817295125,-2.78082020741005,
70.1474946247605));
#139168=CARTESIAN_POINT('Ctrl Pts',(122.220967597282,-2.95094187232875,
70.1360553452162));
#139169=CARTESIAN_POINT('Ctrl Pts',(122.1576869414,-3.11910785768858,70.1237547703804));
#139170=CARTESIAN_POINT('Ctrl Pts',(122.090160629223,-3.28519814820244,
70.1106289194434));
#139171=CARTESIAN_POINT('Ctrl Pts',(122.016001533456,-3.46760268597425,
70.0962137795481));
#139172=CARTESIAN_POINT('Ctrl Pts',(121.936721757884,-3.64750373124946,
70.0808032753626));
#139173=CARTESIAN_POINT('Ctrl Pts',(121.852816091117,-3.8244629412753,70.0644935845287));
#139174=CARTESIAN_POINT('Ctrl Pts',(121.760024497321,-4.02016280003044,
70.0464566358325));
#139175=CARTESIAN_POINT('Ctrl Pts',(121.661575331438,-4.21226472613055,
70.0273199610365));
#139176=CARTESIAN_POINT('Ctrl Pts',(121.558080406608,-4.40061817325353,
70.0072024851623));
#139177=CARTESIAN_POINT('Ctrl Pts',(121.444803244364,-4.60677460096195,
69.9851835254666));
#139178=CARTESIAN_POINT('Ctrl Pts',(121.325481404919,-4.80844045635922,
69.9619895936845));
#139179=CARTESIAN_POINT('Ctrl Pts',(121.200863122926,-5.00559348100024,
69.9377661326256));
#139180=CARTESIAN_POINT('Ctrl Pts',(121.063713701742,-5.22257146193178,
69.9111068527017));
#139181=CARTESIAN_POINT('Ctrl Pts',(120.920149102657,-5.43408339430728,
69.8832005822919));
#139182=CARTESIAN_POINT('Ctrl Pts',(120.77088450835,-5.64030953171291,69.8541863395183));
#139183=CARTESIAN_POINT('Ctrl Pts',(120.604487294548,-5.87020634573354,
69.8218418362522));
#139184=CARTESIAN_POINT('Ctrl Pts',(120.431006497828,-6.09353431793983,
69.7881204170756));
#139185=CARTESIAN_POINT('Ctrl Pts',(120.251312805852,-6.31035921213186,
69.753191327374));
#139186=CARTESIAN_POINT('Ctrl Pts',(120.049384019086,-6.55401377419899,
69.7139401515053));
#139187=CARTESIAN_POINT('Ctrl Pts',(119.839609656204,-6.78945632053946,
69.673163942518));
#139188=CARTESIAN_POINT('Ctrl Pts',(119.623367581806,-7.01678344073686,
69.6311305314923));
#139189=CARTESIAN_POINT('Ctrl Pts',(119.378320042006,-7.27439265804311,
69.5834978772554));
#139190=CARTESIAN_POINT('Ctrl Pts',(119.124966903649,-7.52158034193558,
69.5342507701456));
#139191=CARTESIAN_POINT('Ctrl Pts',(118.864766581224,-7.75898684155283,
69.4836726986369));
#139192=CARTESIAN_POINT('Ctrl Pts',(118.770447846189,-7.84504315587401,
69.4653389022727));
#139193=CARTESIAN_POINT('Ctrl Pts',(118.67522942243,-7.9298142672405,69.4468302232634));
#139194=CARTESIAN_POINT('Ctrl Pts',(118.579168886261,-8.0133283062913,69.4281578533551));
#139195=CARTESIAN_POINT('Ctrl Pts',(118.579167675758,8.01332909152366,69.4281576180553));
#139196=CARTESIAN_POINT('Ctrl Pts',(118.706407237274,7.90270884529846,69.4528906067866));
#139197=CARTESIAN_POINT('Ctrl Pts',(118.832169568853,7.78988234065932,69.4773364496672));
#139198=CARTESIAN_POINT('Ctrl Pts',(118.956319204754,7.67478356951031,69.501468814699));
#139199=CARTESIAN_POINT('Ctrl Pts',(119.228437971327,7.42250304196803,69.5543636086249));
#139200=CARTESIAN_POINT('Ctrl Pts',(119.492808935974,7.15930596577158,69.6057523749017));
#139201=CARTESIAN_POINT('Ctrl Pts',(119.747642512621,6.88447199855316,69.6552872515001));
#139202=CARTESIAN_POINT('Ctrl Pts',(119.978547509072,6.63544462523624,69.700170860072));
#139203=CARTESIAN_POINT('Ctrl Pts',(120.201622125988,6.37686313990138,69.7435323894544));
#139204=CARTESIAN_POINT('Ctrl Pts',(120.415115575264,6.10870425024106,69.7850315192159));
#139205=CARTESIAN_POINT('Ctrl Pts',(120.608606095043,5.86567008165281,69.822642453955));
#139206=CARTESIAN_POINT('Ctrl Pts',(120.794226723886,5.61476911328383,69.8587236292279));
#139207=CARTESIAN_POINT('Ctrl Pts',(120.970826686337,5.3557943959983,69.8930513558265));
#139208=CARTESIAN_POINT('Ctrl Pts',(121.131776280278,5.11977013523727,69.9243369437748));
#139209=CARTESIAN_POINT('Ctrl Pts',(121.285233194329,4.87703971624811,69.9541660950199));
#139210=CARTESIAN_POINT('Ctrl Pts',(121.429999562862,4.62743401359536,69.9823059669128));
#139211=CARTESIAN_POINT('Ctrl Pts',(121.562804428911,4.39845229469453,70.0081207466524));
#139212=CARTESIAN_POINT('Ctrl Pts',(121.688295552653,4.1636845117424,70.0325138718084));
#139213=CARTESIAN_POINT('Ctrl Pts',(121.805299740365,3.92334839336197,70.0552572954825));
#139214=CARTESIAN_POINT('Ctrl Pts',(121.910633879428,3.70698350411704,70.0757322801725));
#139215=CARTESIAN_POINT('Ctrl Pts',(122.009089634504,3.48610566118503,70.0948702357842));
#139216=CARTESIAN_POINT('Ctrl Pts',(122.099776257765,3.26145942719535,70.1124980176158));
#139217=CARTESIAN_POINT('Ctrl Pts',(122.180315419768,3.06195018556796,70.1281533229478));
#139218=CARTESIAN_POINT('Ctrl Pts',(122.254726843029,2.85946870503029,70.1426175105849));
#139219=CARTESIAN_POINT('Ctrl Pts',(122.322688108602,2.65416502953732,70.1558279083178));
#139220=CARTESIAN_POINT('Ctrl Pts',(122.383730436066,2.4697627220875,70.1676933940108));
#139221=CARTESIAN_POINT('Ctrl Pts',(122.439569095469,2.28308360739369,70.1785473840482));
#139222=CARTESIAN_POINT('Ctrl Pts',(122.489830488269,2.09415146679093,70.1883172578727));
#139223=CARTESIAN_POINT('Ctrl Pts',(122.535556029859,1.92226955163331,70.197205447137));
#139224=CARTESIAN_POINT('Ctrl Pts',(122.576665525928,1.74852291117324,70.2051963635714));
#139225=CARTESIAN_POINT('Ctrl Pts',(122.612786961099,1.57272462037444,70.2122176943462));
#139226=CARTESIAN_POINT('Ctrl Pts',(122.645653698257,1.41276651823369,70.2186063727578));
#139227=CARTESIAN_POINT('Ctrl Pts',(122.674390769341,1.25110983402452,70.2241923213942));
#139228=CARTESIAN_POINT('Ctrl Pts',(122.698498321049,1.08749936217765,70.2288783781316));
#139229=CARTESIAN_POINT('Ctrl Pts',(122.720376484174,0.939019058764628,
70.2331310834647));
#139230=CARTESIAN_POINT('Ctrl Pts',(122.738441782511,0.788929618963829,
70.2366426392626));
#139231=CARTESIAN_POINT('Ctrl Pts',(122.752125116466,0.637035590540334,
70.2393024232196));
#139232=CARTESIAN_POINT('Ctrl Pts',(122.764514347892,0.499506953389438,
70.2417106578718));
#139233=CARTESIAN_POINT('Ctrl Pts',(122.773311270029,0.36049892482727,70.2434206148502));
#139234=CARTESIAN_POINT('Ctrl Pts',(122.777904022792,0.21979855912871,70.2443133600067));
#139235=CARTESIAN_POINT('Ctrl Pts',(122.780278918112,0.147042924934891,
70.2447749951966));
#139236=CARTESIAN_POINT('Ctrl Pts',(122.78152966667,0.0738347930879903,
70.2450181173007));
#139237=CARTESIAN_POINT('Ctrl Pts',(122.781535313754,0.000146553589118155,
70.2450192149898));
#139238=CARTESIAN_POINT('Ctrl Pts',(121.735036999469,-0.251492025179986,
71.3942664706531));
#139239=CARTESIAN_POINT('Ctrl Pts',(121.736666170369,-0.215891144805086,
71.3945831509849));
#139240=CARTESIAN_POINT('Ctrl Pts',(121.741962725169,-0.0671388154477658,
71.395612702069));
#139241=CARTESIAN_POINT('Ctrl Pts',(121.740499271469,0.205652813699514,
71.395328234083));
#139242=CARTESIAN_POINT('Ctrl Pts',(121.717046418369,0.577293639062614,
71.3907694384831));
#139243=CARTESIAN_POINT('Ctrl Pts',(121.668270199469,0.983031965715715,
71.381288254676));
#139244=CARTESIAN_POINT('Ctrl Pts',(121.589935658169,1.42397590041401,71.3660614863309));
#139245=CARTESIAN_POINT('Ctrl Pts',(121.477000594769,1.90145538787401,71.344109024239));
#139246=CARTESIAN_POINT('Ctrl Pts',(121.322206770769,2.41905763331001,71.314020002736));
#139247=CARTESIAN_POINT('Ctrl Pts',(121.115195911069,2.98242360767701,71.273780967021));
#139248=CARTESIAN_POINT('Ctrl Pts',(120.843004798869,3.59315027891601,71.220872110458));
#139249=CARTESIAN_POINT('Ctrl Pts',(120.495342776269,4.24372764292801,71.1532931217909));
#139250=CARTESIAN_POINT('Ctrl Pts',(120.064210631769,4.92582479463801,71.069489104072));
#139251=CARTESIAN_POINT('Ctrl Pts',(119.539917822169,5.63463028088801,70.9675763970829));
#139252=CARTESIAN_POINT('Ctrl Pts',(118.908073927269,6.36718264177401,70.844757772566));
#139253=CARTESIAN_POINT('Ctrl Pts',(118.154101012269,7.11797347893601,70.6981995529159));
#139254=CARTESIAN_POINT('Ctrl Pts',(117.287531488569,7.85964231700502,70.529754660428));
#139255=CARTESIAN_POINT('Ctrl Pts',(116.364458080669,8.54113736259001,70.3503264706501));
#139256=CARTESIAN_POINT('Ctrl Pts',(115.461364070269,9.12444254260202,70.174781901721));
#139257=CARTESIAN_POINT('Ctrl Pts',(114.630345072369,9.60270974752501,70.013247365902));
#139258=CARTESIAN_POINT('Ctrl Pts',(113.875901979669,9.99555594218302,69.866597752494));
#139259=CARTESIAN_POINT('Ctrl Pts',(113.189659887769,10.32266924499,69.733205136871));
#139260=CARTESIAN_POINT('Ctrl Pts',(112.564518764069,10.59800466355,69.6116894056039));
#139261=CARTESIAN_POINT('Ctrl Pts',(111.994010209669,10.83200669423,69.5007932230349));
#139262=CARTESIAN_POINT('Ctrl Pts',(111.472720313369,11.03252162863,69.399464226171));
#139263=CARTESIAN_POINT('Ctrl Pts',(110.995459891769,11.20571011009,69.3066937349319));
#139264=CARTESIAN_POINT('Ctrl Pts',(110.558067988369,11.35623559362,69.221672937274));
#139265=CARTESIAN_POINT('Ctrl Pts',(110.156738142269,11.48782915937,69.14366192843));
#139266=CARTESIAN_POINT('Ctrl Pts',(109.788096674869,11.6034703193,69.072004928438));
#139267=CARTESIAN_POINT('Ctrl Pts',(109.449151069169,11.70555902887,69.006120248052));
#139268=CARTESIAN_POINT('Ctrl Pts',(109.137297799269,11.79604012731,68.945501810536));
#139269=CARTESIAN_POINT('Ctrl Pts',(108.850198007269,11.87652072471,68.889694985726));
#139270=CARTESIAN_POINT('Ctrl Pts',(108.585646974169,11.94836677779,68.838271217513));
#139271=CARTESIAN_POINT('Ctrl Pts',(108.341438482969,12.01277581243,68.790801658613));
#139272=CARTESIAN_POINT('Ctrl Pts',(108.115879319369,12.07068478168,68.7469571798701));
#139273=CARTESIAN_POINT('Ctrl Pts',(107.908033627069,12.12274847362,68.706555868334));
#139274=CARTESIAN_POINT('Ctrl Pts',(107.717523269469,12.16941078817,68.66952422133));
#139275=CARTESIAN_POINT('Ctrl Pts',(107.542993047469,12.21129961914,68.6355988135181));
#139276=CARTESIAN_POINT('Ctrl Pts',(107.381385453769,12.24937353981,68.604185322737));
#139277=CARTESIAN_POINT('Ctrl Pts',(107.228180474569,12.28482690077,68.574405142906));
#139278=CARTESIAN_POINT('Ctrl Pts',(107.078801888769,12.31878946362,68.545368742322));
#139279=CARTESIAN_POINT('Ctrl Pts',(106.929723974469,12.35207976103,68.516390786656));
#139280=CARTESIAN_POINT('Ctrl Pts',(106.779850410769,12.38493913925,68.487258171623));
#139281=CARTESIAN_POINT('Ctrl Pts',(106.631924647569,12.41673973848,68.4585041725629));
#139282=CARTESIAN_POINT('Ctrl Pts',(106.488092805569,12.44721671376,68.430545955138));
#139283=CARTESIAN_POINT('Ctrl Pts',(106.347104704869,12.47683083554,68.403140507774));
#139284=CARTESIAN_POINT('Ctrl Pts',(106.205911688169,12.50644037965,68.375695228581));
#139285=CARTESIAN_POINT('Ctrl Pts',(106.067750102369,12.53503352719,68.3488392027959));
#139286=CARTESIAN_POINT('Ctrl Pts',(105.927289821969,12.56398387632,68.321536353826));
#139287=CARTESIAN_POINT('Ctrl Pts',(105.790462806669,12.58661359322,68.294939743578));
#139288=CARTESIAN_POINT('Ctrl Pts',(105.655382900269,12.6104306869,68.2686827385831));
#139289=CARTESIAN_POINT('Ctrl Pts',(105.514586499069,12.63537735536,68.241314554006));
#139290=CARTESIAN_POINT('Ctrl Pts',(105.372054333269,12.66136914805,68.213608969295));
#139291=CARTESIAN_POINT('Ctrl Pts',(105.224646304969,12.68828209136,68.1849556082059));
#139292=CARTESIAN_POINT('Ctrl Pts',(105.084302374769,12.71309158432,68.1576753755249));
#139293=CARTESIAN_POINT('Ctrl Pts',(104.993587027669,12.72877844949,68.1400420103229));
#139294=CARTESIAN_POINT('Ctrl Pts',(104.951723458469,12.73596373186,68.131904516193));
#139295=CARTESIAN_POINT('Ctrl Pts',(123.952465300269,-0.347324334375986,
70.7269691636091));
#139296=CARTESIAN_POINT('Ctrl Pts',(123.954739795569,-0.297475647665086,
70.727411282907));
#139297=CARTESIAN_POINT('Ctrl Pts',(123.962094199069,-0.0904292661378857,
70.7288408412711));
#139298=CARTESIAN_POINT('Ctrl Pts',(123.959932446069,0.280422996215414,
70.728420636943));
#139299=CARTESIAN_POINT('Ctrl Pts',(123.928784632269,0.770995648308114,
70.722366085071));
#139300=CARTESIAN_POINT('Ctrl Pts',(123.865809617769,1.29342741519301,70.710124921183));
#139301=CARTESIAN_POINT('Ctrl Pts',(123.766849737969,1.84967256667701,70.6908889731791));
#139302=CARTESIAN_POINT('Ctrl Pts',(123.626378368069,2.44310614183101,70.663583968595));
#139303=CARTESIAN_POINT('Ctrl Pts',(123.435749754269,3.08026159298101,70.626529334816));
#139304=CARTESIAN_POINT('Ctrl Pts',(123.182646046169,3.76887936681402,70.57733071228));
#139305=CARTESIAN_POINT('Ctrl Pts',(122.851462108169,4.51172925891301,70.512954754774));
#139306=CARTESIAN_POINT('Ctrl Pts',(122.433221569769,5.29389921289301,70.431656623918));
#139307=CARTESIAN_POINT('Ctrl Pts',(121.921579819569,6.10294846988001,70.3322030460629));
#139308=CARTESIAN_POINT('Ctrl Pts',(121.306988090869,6.93348816094802,70.212737919675));
#139309=CARTESIAN_POINT('Ctrl Pts',(120.573879538169,7.78307150435002,70.07023534144));
#139310=CARTESIAN_POINT('Ctrl Pts',(119.710740143769,8.64212008370501,69.902457201885));
#139311=CARTESIAN_POINT('Ctrl Pts',(118.731411294669,9.47989893856901,69.712094007483));
#139312=CARTESIAN_POINT('Ctrl Pts',(117.700739548969,10.24052756398,69.511750715177));
#139313=CARTESIAN_POINT('Ctrl Pts',(116.702090736569,10.88538371112,69.3176320816061));
#139314=CARTESIAN_POINT('Ctrl Pts',(115.790015237369,11.41020795647,69.1403416793871));
#139315=CARTESIAN_POINT('Ctrl Pts',(114.966933189469,11.83874087279,68.980349938073));
#139316=CARTESIAN_POINT('Ctrl Pts',(114.221954815069,12.19381986534,68.835540088713));
#139317=CARTESIAN_POINT('Ctrl Pts',(113.546053101469,12.49149008357,68.704157449044));
#139318=CARTESIAN_POINT('Ctrl Pts',(112.931611172969,12.74349632572,68.584721441012));
#139319=CARTESIAN_POINT('Ctrl Pts',(112.372113240569,12.95869744806,68.475965517244));
#139320=CARTESIAN_POINT('Ctrl Pts',(111.861422559869,13.1440098487,68.3766968094789));
#139321=CARTESIAN_POINT('Ctrl Pts',(111.394646774969,13.30464238705,68.2859643353231));
#139322=CARTESIAN_POINT('Ctrl Pts',(110.967390651869,13.44473346675,68.2029137436041));
#139323=CARTESIAN_POINT('Ctrl Pts',(110.575721925769,13.56759573733,68.126780675622));
#139324=CARTESIAN_POINT('Ctrl Pts',(110.216251000269,13.67586476001,68.05690625729));
#139325=CARTESIAN_POINT('Ctrl Pts',(109.886051079069,13.77166764477,67.992721574233));
#139326=CARTESIAN_POINT('Ctrl Pts',(109.582506400769,13.85675710051,67.933718171385));
#139327=CARTESIAN_POINT('Ctrl Pts',(109.303181896269,13.93261462941,67.879422716907));
#139328=CARTESIAN_POINT('Ctrl Pts',(109.045629558069,14.00054238633,67.829359363966));
#139329=CARTESIAN_POINT('Ctrl Pts',(108.808137096369,14.06151437864,67.7831952754649));
#139330=CARTESIAN_POINT('Ctrl Pts',(108.589621961869,14.1162502982,67.740720024114));
#139331=CARTESIAN_POINT('Ctrl Pts',(108.389578174769,14.16524723555,67.701835256892));
#139332=CARTESIAN_POINT('Ctrl Pts',(108.206580960669,14.2091681233,67.666264024338));
#139333=CARTESIAN_POINT('Ctrl Pts',(108.037100660769,14.24909690253,67.6333202268571));
#139334=CARTESIAN_POINT('Ctrl Pts',(107.876321113269,14.2863032376,67.6020676927461));
#139335=CARTESIAN_POINT('Ctrl Pts',(107.719480082869,14.32196243997,67.571580732629));
#139336=CARTESIAN_POINT('Ctrl Pts',(107.562912614569,14.35692548367,67.5411469478801));
#139337=CARTESIAN_POINT('Ctrl Pts',(107.405377034369,14.39146426087,67.510524980273));
#139338=CARTESIAN_POINT('Ctrl Pts',(107.250163184169,14.42483253046,67.480354313537));
#139339=CARTESIAN_POINT('Ctrl Pts',(107.101721753269,14.45627778599,67.451500078315));
#139340=CARTESIAN_POINT('Ctrl Pts',(106.959668596669,14.48613647781,67.42388760403));
#139341=CARTESIAN_POINT('Ctrl Pts',(106.812895930169,14.51683767398,67.395357745367));
#139342=CARTESIAN_POINT('Ctrl Pts',(106.685780281469,14.54339449682,67.370648842976));
#139343=CARTESIAN_POINT('Ctrl Pts',(106.475408024369,14.58594290389,67.329756414555));
#139344=CARTESIAN_POINT('Ctrl Pts',(106.330012623469,14.60975916719,67.3014942705451));
#139345=CARTESIAN_POINT('Ctrl Pts',(106.205346414169,14.63184978471,67.277261493309));
#139346=CARTESIAN_POINT('Ctrl Pts',(106.069531214769,14.65588498744,67.250861561116));
#139347=CARTESIAN_POINT('Ctrl Pts',(105.936535264969,14.68014815303,67.2250096382841));
#139348=CARTESIAN_POINT('Ctrl Pts',(105.780150023969,14.70869883296,67.1946112750921));
#139349=CARTESIAN_POINT('Ctrl Pts',(105.630239251269,14.73519937094,67.1654714273339));
#139350=CARTESIAN_POINT('Ctrl Pts',(105.535552987169,14.75157065244,67.1470661902031));
#139351=CARTESIAN_POINT('Ctrl Pts',(105.492059043269,14.75903578704,67.138611781753));
#139352=CARTESIAN_POINT('Ctrl Pts',(123.605514838569,-0.310954453434086,
68.4357418369039));
#139353=CARTESIAN_POINT('Ctrl Pts',(123.607544422969,-0.266513035153486,
68.436136350125));
#139354=CARTESIAN_POINT('Ctrl Pts',(123.614117840269,-0.0815901707869558,
68.4374140993829));
#139355=CARTESIAN_POINT('Ctrl Pts',(123.612221102869,0.252046526328314,
68.43704540915));
#139356=CARTESIAN_POINT('Ctrl Pts',(123.583993648769,0.697482664288614,
68.431558520501));
#139357=CARTESIAN_POINT('Ctrl Pts',(123.526407302269,1.17562742021101,68.420364812818));
#139358=CARTESIAN_POINT('Ctrl Pts',(123.435275065569,1.68811393160701,68.402650412068));
#139359=CARTESIAN_POINT('Ctrl Pts',(123.305254160569,2.23754109181001,68.377376782234));
#139360=CARTESIAN_POINT('Ctrl Pts',(123.128225417769,2.82932420565001,68.342965708767));
#139361=CARTESIAN_POINT('Ctrl Pts',(122.892614676469,3.47040693548102,68.297167391501));
#139362=CARTESIAN_POINT('Ctrl Pts',(122.583819451269,4.16311397020101,68.237143380635));
#139363=CARTESIAN_POINT('Ctrl Pts',(122.192364578769,4.89534244964002,68.161051881783));
#139364=CARTESIAN_POINT('Ctrl Pts',(121.711277500669,5.65621136960901,68.067537560153));
#139365=CARTESIAN_POINT('Ctrl Pts',(121.130955643569,6.44055099962301,67.954733855254));
#139366=CARTESIAN_POINT('Ctrl Pts',(120.436278634169,7.24571922941301,67.8197016495811));
#139367=CARTESIAN_POINT('Ctrl Pts',(119.614569649869,8.06368227897601,67.659976806111));
#139368=CARTESIAN_POINT('Ctrl Pts',(118.678034752669,8.86498585846002,67.477931954842));
#139369=CARTESIAN_POINT('Ctrl Pts',(117.688198282369,9.59558203551501,67.2855262755941));
#139370=CARTESIAN_POINT('Ctrl Pts',(116.725814032569,10.21707861463,67.098456794081));
#139371=CARTESIAN_POINT('Ctrl Pts',(115.844500760869,10.72423372488,66.9271459930001));
#139372=CARTESIAN_POINT('Ctrl Pts',(115.047468284869,11.13922296445,66.7722178007911));
#139373=CARTESIAN_POINT('Ctrl Pts',(114.324781261069,11.4836885343,66.631740972675));
#139374=CARTESIAN_POINT('Ctrl Pts',(113.668143996269,11.77288234189,66.5041029812041));
#139375=CARTESIAN_POINT('Ctrl Pts',(113.070375479869,12.0180557003,66.3879079723501));
#139376=CARTESIAN_POINT('Ctrl Pts',(112.525378103069,12.22768318143,66.28197068511));
#139377=CARTESIAN_POINT('Ctrl Pts',(112.027374735769,12.4083943625,66.1851681535581));
#139378=CARTESIAN_POINT('Ctrl Pts',(111.571750599769,12.56519111328,66.096603351202));
#139379=CARTESIAN_POINT('Ctrl Pts',(111.154333909969,12.70205725169,66.015465361097));
#139380=CARTESIAN_POINT('Ctrl Pts',(110.771404393669,12.82217899627,65.941031031893));
#139381=CARTESIAN_POINT('Ctrl Pts',(110.419723152469,12.92810249213,65.872670782376));
#139382=CARTESIAN_POINT('Ctrl Pts',(110.096486076369,13.02188567459,65.8098395460521));
#139383=CARTESIAN_POINT('Ctrl Pts',(109.799182493169,13.10522599551,65.752049295257));
#139384=CARTESIAN_POINT('Ctrl Pts',(109.525464755369,13.17956110573,65.698843691253));
#139385=CARTESIAN_POINT('Ctrl Pts',(109.272976618669,13.24615345175,65.64976472428));
#139386=CARTESIAN_POINT('Ctrl Pts',(109.040013032869,13.30596297823,65.604480964464));
#139387=CARTESIAN_POINT('Ctrl Pts',(108.825547120869,13.35968474504,65.562792806159));
#139388=CARTESIAN_POINT('Ctrl Pts',(108.629121421369,13.40779565601,65.524611327444));
#139389=CARTESIAN_POINT('Ctrl Pts',(108.449337565069,13.450945346,65.4896647114781));
#139390=CARTESIAN_POINT('Ctrl Pts',(108.282845082069,13.49017017699,65.457301689655));
#139391=CARTESIAN_POINT('Ctrl Pts',(108.124940203269,13.52671123059,65.4266079373401));
#139392=CARTESIAN_POINT('Ctrl Pts',(107.970931288969,13.56172653136,65.396671487568));
#139393=CARTESIAN_POINT('Ctrl Pts',(107.817206225169,13.59605474132,65.36679021304));
#139394=CARTESIAN_POINT('Ctrl Pts',(107.662578501669,13.62995615997,65.336733478351));
#139395=CARTESIAN_POINT('Ctrl Pts',(107.510130596069,13.6627294738,65.307100459463));
#139396=CARTESIAN_POINT('Ctrl Pts',(107.363438577269,13.69380725163,65.2785862772031));
#139397=CARTESIAN_POINT('Ctrl Pts',(107.221789626269,13.72357312524,65.251052372917));
#139398=CARTESIAN_POINT('Ctrl Pts',(107.077134525369,13.75386002214,65.222934129361));
#139399=CARTESIAN_POINT('Ctrl Pts',(106.945826768369,13.7811896625,65.197410359595));
#139400=CARTESIAN_POINT('Ctrl Pts',(106.761987215069,13.81857739095,65.161675392064));
#139401=CARTESIAN_POINT('Ctrl Pts',(106.619843652369,13.84194334108,65.134045344527));
#139402=CARTESIAN_POINT('Ctrl Pts',(106.491225279869,13.86468918368,65.109044340758));
#139403=CARTESIAN_POINT('Ctrl Pts',(106.353519635369,13.88907030211,65.082276941433));
#139404=CARTESIAN_POINT('Ctrl Pts',(106.216904540369,13.91398950909,65.055721524524));
#139405=CARTESIAN_POINT('Ctrl Pts',(106.063926293969,13.941918642,65.0259854173001));
#139406=CARTESIAN_POINT('Ctrl Pts',(105.917646289669,13.96777740158,64.9975513229521));
#139407=CARTESIAN_POINT('Ctrl Pts',(105.824467051569,13.98388893623,64.979439023457));
#139408=CARTESIAN_POINT('Ctrl Pts',(105.781591860669,13.99124786247,64.971104889017));
#139409=CARTESIAN_POINT('Ctrl Pts',(121.290407464969,-0.204882710558486,
68.4579759859419));
#139410=CARTESIAN_POINT('Ctrl Pts',(121.291722773869,-0.176211439766586,
68.458231657368));
#139411=CARTESIAN_POINT('Ctrl Pts',(121.296018466569,-0.0558111958484758,
68.4590666596059));
#139412=CARTESIAN_POINT('Ctrl Pts',(121.294894640169,0.169287343740214,
68.458848208792));
#139413=CARTESIAN_POINT('Ctrl Pts',(121.275184333069,0.483084097755514,
68.455016894092));
#139414=CARTESIAN_POINT('Ctrl Pts',(121.233313886869,0.832067022022413,
68.446878063204));
#139415=CARTESIAN_POINT('Ctrl Pts',(121.165010752469,1.21693268067301,68.43360121256));
#139416=CARTESIAN_POINT('Ctrl Pts',(121.065468336969,1.63801635965901,68.414252030502));
#139417=CARTESIAN_POINT('Ctrl Pts',(120.928103238269,2.09747231783601,68.3875508269161));
#139418=CARTESIAN_POINT('Ctrl Pts',(120.743510246669,2.59992041829301,68.351669405084));
#139419=CARTESIAN_POINT('Ctrl Pts',(120.500011077769,3.14638720868801,68.304337725156));
#139420=CARTESIAN_POINT('Ctrl Pts',(120.186675852369,3.73296277122801,68.243431223252));
#139421=CARTESIAN_POINT('Ctrl Pts',(119.794700622469,4.35331508274601,68.167238576668));
#139422=CARTESIAN_POINT('Ctrl Pts',(119.314325889769,5.00291352389501,68.073862721656));
#139423=CARTESIAN_POINT('Ctrl Pts',(118.731733404269,5.67854631422901,67.960617649101));
#139424=CARTESIAN_POINT('Ctrl Pts',(118.030855054569,6.37668456263001,67.824380018941));
#139425=CARTESIAN_POINT('Ctrl Pts',(117.219127524269,7.07160901930201,67.666595383297));
#139426=CARTESIAN_POINT('Ctrl Pts',(116.348385995069,7.71461639877401,67.4973395310339));
#139427=CARTESIAN_POINT('Ctrl Pts',(115.491766329969,8.26798544955901,67.330828704796));
#139428=CARTESIAN_POINT('Ctrl Pts',(114.700170236569,8.72360902037701,67.176957243574));
#139429=CARTESIAN_POINT('Ctrl Pts',(113.979110609969,9.09909850463502,67.036796751032));
#139430=CARTESIAN_POINT('Ctrl Pts',(113.321435688169,9.41261032332302,66.908957058466));
#139431=CARTESIAN_POINT('Ctrl Pts',(112.720982650669,9.67708291583402,66.792240228967));
#139432=CARTESIAN_POINT('Ctrl Pts',(112.171841675469,9.902328359459,66.6854975037769));
#139433=CARTESIAN_POINT('Ctrl Pts',(111.669134764169,10.09570047157,66.587780691319));
#139434=CARTESIAN_POINT('Ctrl Pts',(111.208133592469,10.26299232414,66.498170693874));
#139435=CARTESIAN_POINT('Ctrl Pts',(110.785032929769,10.4086021075,66.415927845836));
#139436=CARTESIAN_POINT('Ctrl Pts',(110.396312672269,10.53606279464,66.340367904965));
#139437=CARTESIAN_POINT('Ctrl Pts',(110.038870817469,10.64819187163,66.270887900006));
#139438=CARTESIAN_POINT('Ctrl Pts',(109.709907973469,10.74727470395,66.2069436815879));
#139439=CARTESIAN_POINT('Ctrl Pts',(109.406977840669,10.83516748103,66.14805973489));
#139440=CARTESIAN_POINT('Ctrl Pts',(109.127876237269,10.91340649905,66.093807608205));
#139441=CARTESIAN_POINT('Ctrl Pts',(108.870510477969,10.98330151766,66.043780522695));
#139442=CARTESIAN_POINT('Ctrl Pts',(108.632791943669,11.04599917505,65.997572489929));
#139443=CARTESIAN_POINT('Ctrl Pts',(108.413036697869,11.1024184024,65.954856184158));
#139444=CARTESIAN_POINT('Ctrl Pts',(108.210380230269,11.15318242101,65.915463560757));
#139445=CARTESIAN_POINT('Ctrl Pts',(108.024506582569,11.19870926078,65.8793332033499));
#139446=CARTESIAN_POINT('Ctrl Pts',(107.854094394369,11.23960977399,65.8462082642299));
#139447=CARTESIAN_POINT('Ctrl Pts',(107.696315795769,11.2767815596,65.8155390584099));
#139448=CARTESIAN_POINT('Ctrl Pts',(107.546794808369,11.31138233835,65.7864749776119));
#139449=CARTESIAN_POINT('Ctrl Pts',(107.401045681469,11.34451971807,65.7581440758939));
#139450=CARTESIAN_POINT('Ctrl Pts',(107.255610411169,11.37699645313,65.729874182013));
#139451=CARTESIAN_POINT('Ctrl Pts',(107.109463370769,11.40903903339,65.7014659333571));
#139452=CARTESIAN_POINT('Ctrl Pts',(106.965082265369,11.44007717534,65.6734009494109));
#139453=CARTESIAN_POINT('Ctrl Pts',(106.823492358169,11.47008321468,65.645878522126));
#139454=CARTESIAN_POINT('Ctrl Pts',(106.683022261469,11.49957838658,65.618573765051));
#139455=CARTESIAN_POINT('Ctrl Pts',(106.544542981469,11.52865699124,65.591655985468));
#139456=CARTESIAN_POINT('Ctrl Pts',(106.401009057569,11.5582405323,65.563755677742));
#139457=CARTESIAN_POINT('Ctrl Pts',(106.294551394269,11.58057728559,65.5430623009789));
#139458=CARTESIAN_POINT('Ctrl Pts',(106.161891727069,11.60262990991,65.517275745167));
#139459=CARTESIAN_POINT('Ctrl Pts',(106.021746980969,11.62728669818,65.4900342301539));
#139460=CARTESIAN_POINT('Ctrl Pts',(105.878527906069,11.65267667008,65.462195123188));
#139461=CARTESIAN_POINT('Ctrl Pts',(105.731357675069,11.67950920349,65.4335879854359));
#139462=CARTESIAN_POINT('Ctrl Pts',(105.588315833369,11.70562561188,65.405783329264));
#139463=CARTESIAN_POINT('Ctrl Pts',(105.452624863869,11.72961264266,65.379407545042));
#139464=CARTESIAN_POINT('Ctrl Pts',(105.363840824969,11.74496663286,65.3621495899899));
#139465=CARTESIAN_POINT('Ctrl Pts',(105.322770210069,11.75201580539,65.354166231342));
#139466=CARTESIAN_POINT('',(122.019294419317,7.00634560479863E-5,71.2800197814689));
#139467=CARTESIAN_POINT('Origin',(121.309092222769,1.20142455100609E-5,
69.958803843484));
#139468=CARTESIAN_POINT('',(105.406714409596,13.3449720448593,67.5261054277314));
#139469=CARTESIAN_POINT('Ctrl Pts',(122.019295120988,7.90940703660764E-5,
71.2800210882645));
#139470=CARTESIAN_POINT('Ctrl Pts',(122.019289267816,0.0647943413365559,
71.2800206364224));
#139471=CARTESIAN_POINT('Ctrl Pts',(122.018318643201,0.131954861220223,
71.2797688245955));
#139472=CARTESIAN_POINT('Ctrl Pts',(122.016222139614,0.201503059088793,
71.2792342641219));
#139473=CARTESIAN_POINT('Ctrl Pts',(122.013660899416,0.286468160628148,
71.2785812064394));
#139474=CARTESIAN_POINT('Ctrl Pts',(122.009418906529,0.374996384007158,
71.2775060829595));
#139475=CARTESIAN_POINT('Ctrl Pts',(122.003193436169,0.466992869080882,
71.2759496210239));
#139476=CARTESIAN_POINT('Ctrl Pts',(122.000532207089,0.506319009454073,
71.2752842734237));
#139477=CARTESIAN_POINT('Ctrl Pts',(121.997509100327,0.546278850207114,
71.2745310758335));
#139478=CARTESIAN_POINT('Ctrl Pts',(121.994103439403,0.586864690865039,
71.2736859574118));
#139479=CARTESIAN_POINT('Ctrl Pts',(121.993986998336,0.588252338875545,
71.2736570624357));
#139480=CARTESIAN_POINT('Ctrl Pts',(121.99387011027,0.589640718656464,71.2736280600436));
#139481=CARTESIAN_POINT('Ctrl Pts',(121.993752774232,0.591029829879343,
71.2735989500439));
#139482=CARTESIAN_POINT('Ctrl Pts',(121.985566143102,0.687949253089373,
71.2715679216144));
#139483=CARTESIAN_POINT('Ctrl Pts',(121.975194990935,0.78842994343254,71.2690123528165));
#139484=CARTESIAN_POINT('Ctrl Pts',(121.962330547539,0.892356419153909,
71.2658712651658));
#139485=CARTESIAN_POINT('Ctrl Pts',(121.957679506311,0.929930242469154,
71.2647356289231));
#139486=CARTESIAN_POINT('Ctrl Pts',(121.95270301165,0.967954403017347,71.2635235422822));
#139487=CARTESIAN_POINT('Ctrl Pts',(121.947388177942,1.00642321275053,71.2622324436963));
#139488=CARTESIAN_POINT('Ctrl Pts',(121.942961170466,1.03846592897076,71.261157019063));
#139489=CARTESIAN_POINT('Ctrl Pts',(121.938299456839,1.07081714263468,71.2600267821974));
#139490=CARTESIAN_POINT('Ctrl Pts',(121.933394121336,1.10347377448982,71.2588399639624));
#139491=CARTESIAN_POINT('Ctrl Pts',(121.928880251392,1.1335242754022,71.2577478586096));
#139492=CARTESIAN_POINT('Ctrl Pts',(121.924160093542,1.16383339195402,71.2566078426418));
#139493=CARTESIAN_POINT('Ctrl Pts',(121.919226920107,1.19439871366745,71.2554185770162));
#139494=CARTESIAN_POINT('Ctrl Pts',(121.91676033339,1.20968137452416,71.2548239442034));
#139495=CARTESIAN_POINT('Ctrl Pts',(121.914240493777,1.22502808690805,71.2542170008458));
#139496=CARTESIAN_POINT('Ctrl Pts',(121.911666584572,1.240438548423,71.2535975820344));
#139497=CARTESIAN_POINT('Ctrl Pts',(121.91037962997,1.24814377918047,71.2532878726287));
#139498=CARTESIAN_POINT('Ctrl Pts',(121.909079158038,1.25586494723633,71.2529750444866));
#139499=CARTESIAN_POINT('Ctrl Pts',(121.907765067742,1.2636020148263,71.2526590774403));
#139500=CARTESIAN_POINT('Ctrl Pts',(121.906450977447,1.27133908241627,71.252343110394));
#139501=CARTESIAN_POINT('Ctrl Pts',(121.905345477426,1.27780513545291,71.2520773879648));
#139502=CARTESIAN_POINT('Ctrl Pts',(121.903781841349,1.28686087846409,71.2517017397815));
#139503=CARTESIAN_POINT('Ctrl Pts',(121.893675018398,1.34539418595264,71.2492736750057));
#139504=CARTESIAN_POINT('Ctrl Pts',(121.882990116065,1.4036627614239,71.2467149294755));
#139505=CARTESIAN_POINT('Ctrl Pts',(121.871758031279,1.46167228038696,71.2440313578717));
#139506=CARTESIAN_POINT('Ctrl Pts',(121.839585104505,1.62783341977771,71.2363445967452));
#139507=CARTESIAN_POINT('Ctrl Pts',(121.802924103343,1.7918689670011,71.2276340039114));
#139508=CARTESIAN_POINT('Ctrl Pts',(121.762233017693,1.95384294374939,71.2179845293854));
#139509=CARTESIAN_POINT('Ctrl Pts',(121.7171041166,2.13348198408125,71.207282672344));
#139510=CARTESIAN_POINT('Ctrl Pts',(121.667018015079,2.31058496009605,71.1954259703313));
#139511=CARTESIAN_POINT('Ctrl Pts',(121.612456284331,2.48510922069926,71.1825013370691));
#139512=CARTESIAN_POINT('Ctrl Pts',(121.605844188692,2.50625904653242,71.1809350577363));
#139513=CARTESIAN_POINT('Ctrl Pts',(121.599166336251,2.52737100916192,71.1793530879279));
#139514=CARTESIAN_POINT('Ctrl Pts',(121.592423339081,2.54844495564597,71.1777555334907));
#139515=CARTESIAN_POINT('Ctrl Pts',(121.570387141685,2.61731487104202,71.1725347060102));
#139516=CARTESIAN_POINT('Ctrl Pts',(121.547771847224,2.68542579166921,71.1671755693551));
#139517=CARTESIAN_POINT('Ctrl Pts',(121.524426417993,2.75331290177076,71.1616399870936));
#139518=CARTESIAN_POINT('Ctrl Pts',(121.501839088884,2.8189955021176,71.156284162743));
#139519=CARTESIAN_POINT('Ctrl Pts',(121.478567927336,2.8844685952812,71.1507630994509));
#139520=CARTESIAN_POINT('Ctrl Pts',(121.454433664412,2.95020029573306,71.1450338015792));
#139521=CARTESIAN_POINT('Ctrl Pts',(121.44085225073,2.98719042129487,71.1418096730964));
#139522=CARTESIAN_POINT('Ctrl Pts',(121.426677824928,3.02513969909136,71.1384410813606));
#139523=CARTESIAN_POINT('Ctrl Pts',(121.411873730377,3.06403062878303,71.1349206106562));
#139524=CARTESIAN_POINT('Ctrl Pts',(121.379422169101,3.14928213697947,71.1272035043927));
#139525=CARTESIAN_POINT('Ctrl Pts',(121.343945536334,3.23906194266524,71.1187567522501));
#139526=CARTESIAN_POINT('Ctrl Pts',(121.305061550388,3.33313900792745,71.1095025213745));
#139527=CARTESIAN_POINT('Ctrl Pts',(121.267663668914,3.42362054809094,71.1006019773332));
#139528=CARTESIAN_POINT('Ctrl Pts',(121.227113224768,3.51807739288653,71.090954361199));
#139529=CARTESIAN_POINT('Ctrl Pts',(121.18306369568,3.61625626876824,71.0804886127768));
#139530=CARTESIAN_POINT('Ctrl Pts',(121.170900807039,3.64336526990759,71.0775988263196));
#139531=CARTESIAN_POINT('Ctrl Pts',(121.158471137288,3.67075774226389,71.0746466598495));
#139532=CARTESIAN_POINT('Ctrl Pts',(121.145767408056,3.69842763712042,71.071630613055));
#139533=CARTESIAN_POINT('Ctrl Pts',(121.096880958574,3.80490683644929,71.0600242715965));
#139534=CARTESIAN_POINT('Ctrl Pts',(121.04393485288,3.91549749133993,71.047471771854));
#139535=CARTESIAN_POINT('Ctrl Pts',(120.986524703389,4.02987745307783,71.0338891741002));
#139536=CARTESIAN_POINT('Ctrl Pts',(120.930069118973,4.14235560620328,71.0205324157416));
#139537=CARTESIAN_POINT('Ctrl Pts',(120.869295767781,4.25849825442164,71.0061793466359));
#139538=CARTESIAN_POINT('Ctrl Pts',(120.803842983608,4.37795570528577,70.990753891926));
#139539=CARTESIAN_POINT('Ctrl Pts',(120.734846789541,4.50388021051043,70.974493351138));
#139540=CARTESIAN_POINT('Ctrl Pts',(120.660650628725,4.63348670967809,70.9570411482275));
#139541=CARTESIAN_POINT('Ctrl Pts',(120.580836495019,4.76636918385725,70.9383084113126));
#139542=CARTESIAN_POINT('Ctrl Pts',(120.54978599603,4.81806512965831,70.9310207192506));
#139543=CARTESIAN_POINT('Ctrl Pts',(120.517885643202,4.87025653226186,70.9235392920141));
#139544=CARTESIAN_POINT('Ctrl Pts',(120.485112661211,4.92291812442057,70.915859214682));
#139545=CARTESIAN_POINT('Ctrl Pts',(120.468726170215,4.94924892049992,70.912019176016));
#139546=CARTESIAN_POINT('Ctrl Pts',(120.452121524324,4.97569726616381,70.9081294795746));
#139547=CARTESIAN_POINT('Ctrl Pts',(120.435296012009,5.00225991615915,70.9041895297866));
#139548=CARTESIAN_POINT('Ctrl Pts',(120.426883255851,5.01554124115682,70.9022195548926));
#139549=CARTESIAN_POINT('Ctrl Pts',(120.418415283273,5.02885114240544,70.9002370170293));
#139550=CARTESIAN_POINT('Ctrl Pts',(120.409891760874,5.04218921203787,70.8982418433462));
#139551=CARTESIAN_POINT('Ctrl Pts',(120.402622319957,5.05356482702362,70.8965402232263));
#139552=CARTESIAN_POINT('Ctrl Pts',(120.394502748834,5.06621986006523,70.8946399061895));
#139553=CARTESIAN_POINT('Ctrl Pts',(120.387604345069,5.07693276007905,70.8930256645897));
#139554=CARTESIAN_POINT('Ctrl Pts',(120.386414272748,5.07878088701002,70.8927471850585));
#139555=CARTESIAN_POINT('Ctrl Pts',(120.385260645217,5.08057129006946,70.8924772403038));
#139556=CARTESIAN_POINT('Ctrl Pts',(120.384154213863,5.08228751718077,70.892218343275));
#139557=CARTESIAN_POINT('Ctrl Pts',(120.38328842148,5.08363048017059,70.8920157540457));
#139558=CARTESIAN_POINT('Ctrl Pts',(120.382422028954,5.08497378351582,70.8918130272488));
#139559=CARTESIAN_POINT('Ctrl Pts',(120.381555035884,5.08631742674835,70.8916101627974));
#139560=CARTESIAN_POINT('Ctrl Pts',(120.297380541915,5.21676886076607,70.8719144891612));
#139561=CARTESIAN_POINT('Ctrl Pts',(120.207542559621,5.35042682384027,70.8509208255));
#139562=CARTESIAN_POINT('Ctrl Pts',(120.111639563024,5.48684674179412,70.8285420924557));
#139563=CARTESIAN_POINT('Ctrl Pts',(120.033812301504,5.59755432140991,70.810381288613));
#139564=CARTESIAN_POINT('Ctrl Pts',(119.951991106251,5.71008018537599,70.7913083616764));
#139565=CARTESIAN_POINT('Ctrl Pts',(119.865981203322,5.824171158714,70.7712801501997));
#139566=CARTESIAN_POINT('Ctrl Pts',(119.831507080685,5.869900616284,70.7632525278548));
#139567=CARTESIAN_POINT('Ctrl Pts',(119.796360255117,5.91588136703911,70.7550714751542));
#139568=CARTESIAN_POINT('Ctrl Pts',(119.760529634078,5.96209610073101,70.7467344750781));
#139569=CARTESIAN_POINT('Ctrl Pts',(119.72111031052,6.01293958286343,70.7375624625932));
#139570=CARTESIAN_POINT('Ctrl Pts',(119.680863335153,6.06406627492084,70.7282016956236));
#139571=CARTESIAN_POINT('Ctrl Pts',(119.639775001278,6.11545251694759,70.7186490114928));
#139572=CARTESIAN_POINT('Ctrl Pts',(119.61923083434,6.14114563796097,70.7138726694273));
#139573=CARTESIAN_POINT('Ctrl Pts',(119.598476329699,6.16690364875147,70.7090483520244));
#139574=CARTESIAN_POINT('Ctrl Pts',(119.577509905512,6.19272351736988,70.7041756832797));
#139575=CARTESIAN_POINT('Ctrl Pts',(119.567026693418,6.20563345167909,70.7017393489074));
#139576=CARTESIAN_POINT('Ctrl Pts',(119.556490501579,6.21855885061051,70.6992909269887));
#139577=CARTESIAN_POINT('Ctrl Pts',(119.545901136964,6.23149933351409,70.6968303719765));
#139578=CARTESIAN_POINT('Ctrl Pts',(119.540606454656,6.23796957496588,70.6956000944704));
#139579=CARTESIAN_POINT('Ctrl Pts',(119.535298479164,6.24444358742153,70.6943667837094));
#139580=CARTESIAN_POINT('Ctrl Pts',(119.529977186838,6.25092132305579,70.6931304340879));
#139581=CARTESIAN_POINT('Ctrl Pts',(119.525986217594,6.25577962478147,70.6922031718717));
#139582=CARTESIAN_POINT('Ctrl Pts',(119.521987757632,6.26064002079604,70.6912742002981));
#139583=CARTESIAN_POINT('Ctrl Pts',(119.517981797084,6.26550249087177,70.6903435170244));
#139584=CARTESIAN_POINT('Ctrl Pts',(119.516646476901,6.26712331423035,70.6900332892666));
#139585=CARTESIAN_POINT('Ctrl Pts',(119.516325625924,6.26751317211349,70.6899587459064));
#139586=CARTESIAN_POINT('Ctrl Pts',(119.513973335985,6.27036565154658,70.689412263098));
#139587=CARTESIAN_POINT('Ctrl Pts',(119.445940346586,6.3528651341979,70.6736068734286));
#139588=CARTESIAN_POINT('Ctrl Pts',(119.379990061922,6.43080116154606,70.658306683783));
#139589=CARTESIAN_POINT('Ctrl Pts',(119.316404933559,6.50440018602863,70.6435704089504));
#139590=CARTESIAN_POINT('Ctrl Pts',(119.291094816403,6.53369634348217,70.6377046215869));
#139591=CARTESIAN_POINT('Ctrl Pts',(119.266158907851,6.56230510491915,70.6319280753122));
#139592=CARTESIAN_POINT('Ctrl Pts',(119.241612972835,6.59023986855823,70.626244060308));
#139593=CARTESIAN_POINT('Ctrl Pts',(119.177469096201,6.66323949279387,70.6113904905832));
#139594=CARTESIAN_POINT('Ctrl Pts',(119.11599130841,6.73163862511283,70.5971694189702));
#139595=CARTESIAN_POINT('Ctrl Pts',(119.057421138099,6.79566735526086,70.5836315498303));
#139596=CARTESIAN_POINT('Ctrl Pts',(118.996896118557,6.86183312057973,70.5696418381751));
#139597=CARTESIAN_POINT('Ctrl Pts',(118.93947591326,6.92333197083014,70.5563816727075));
#139598=CARTESIAN_POINT('Ctrl Pts',(118.885381777702,6.98038540499861,70.5438977543021));
#139599=CARTESIAN_POINT('Ctrl Pts',(118.830325629018,7.03845348062509,70.531191821195));
#139600=CARTESIAN_POINT('Ctrl Pts',(118.778714658739,7.09191663079638,70.5192899446257));
#139601=CARTESIAN_POINT('Ctrl Pts',(118.730739096332,7.14097469522637,70.5082324977803));
#139602=CARTESIAN_POINT('Ctrl Pts',(118.681463061506,7.19136257543249,70.4968753169885));
#139603=CARTESIAN_POINT('Ctrl Pts',(118.636022019864,7.23710338697868,70.4864089350787));
#139604=CARTESIAN_POINT('Ctrl Pts',(118.594580255186,7.27837773112763,70.4768684059795));
#139605=CARTESIAN_POINT('Ctrl Pts',(118.558239789795,7.3145713847215,70.468502274126));
#139606=CARTESIAN_POINT('Ctrl Pts',(118.524973858968,7.34732992666515,70.4608479323379));
#139607=CARTESIAN_POINT('Ctrl Pts',(118.494869538803,7.37675286197228,70.4539240473464));
#139608=CARTESIAN_POINT('Ctrl Pts',(118.463440223853,7.40747080197225,70.4466954183359));
#139609=CARTESIAN_POINT('Ctrl Pts',(118.435456902054,7.43455317802427,70.4402629544865));
#139610=CARTESIAN_POINT('Ctrl Pts',(118.41099536373,7.45808970851861,70.4346429705706));
#139611=CARTESIAN_POINT('Ctrl Pts',(118.39784091329,7.47074672623445,70.4316207648975));
#139612=CARTESIAN_POINT('Ctrl Pts',(118.385704538703,7.48237792553573,70.4288334372906));
#139613=CARTESIAN_POINT('Ctrl Pts',(118.374595490617,7.49299443529233,70.4262829948165));
#139614=CARTESIAN_POINT('Ctrl Pts',(118.369040966574,7.49830269017064,70.4250077735794));
#139615=CARTESIAN_POINT('Ctrl Pts',(118.363743263503,7.50335725592985,70.4237917504513));
#139616=CARTESIAN_POINT('Ctrl Pts',(118.358703359586,7.50815932475693,70.4226351631851));
#139617=CARTESIAN_POINT('Ctrl Pts',(118.356183407627,7.51056035917047,70.422056869552));
#139618=CARTESIAN_POINT('Ctrl Pts',(118.353727904802,7.51289826832515,70.42149343346));
#139619=CARTESIAN_POINT('Ctrl Pts',(118.351336966545,7.51517319233377,70.4209448794642));
#139620=CARTESIAN_POINT('Ctrl Pts',(118.350141497417,7.51631065433808,70.4206706024662));
#139621=CARTESIAN_POINT('Ctrl Pts',(118.348962169391,7.51743236999189,70.4204000459041));
#139622=CARTESIAN_POINT('Ctrl Pts',(118.347798996254,7.51853835607367,70.4201332127564));
#139623=CARTESIAN_POINT('Ctrl Pts',(118.347217409686,7.51909134911456,70.4199997961826));
#139624=CARTESIAN_POINT('Ctrl Pts',(118.346996942952,7.51930102883103,70.4199491531009));
#139625=CARTESIAN_POINT('Ctrl Pts',(118.346601988741,7.51967648864734,70.4198585474782));
#139626=CARTESIAN_POINT('Ctrl Pts',(118.34620703453,7.52005194846366,70.4197679418556));
#139627=CARTESIAN_POINT('Ctrl Pts',(118.345637604999,7.52059320757401,70.4196374001701));
#139628=CARTESIAN_POINT('Ctrl Pts',(118.344357955025,7.52180914202048,70.4193438863148));
#139629=CARTESIAN_POINT('Ctrl Pts',(118.200158384446,7.65882881815134,70.3862687698805));
#139630=CARTESIAN_POINT('Ctrl Pts',(118.050682131663,7.79545090863632,70.3520656867254));
#139631=CARTESIAN_POINT('Ctrl Pts',(117.895912984387,7.93140957380592,70.3167280067712));
#139632=CARTESIAN_POINT('Ctrl Pts',(117.802236164841,8.01370100957925,70.2953392382312));
#139633=CARTESIAN_POINT('Ctrl Pts',(117.706621202113,8.09574957147887,70.2735349854436));
#139634=CARTESIAN_POINT('Ctrl Pts',(117.609073502286,8.17749823024438,70.251315515606));
#139635=CARTESIAN_POINT('Ctrl Pts',(117.444287644727,8.31559500610868,70.2137805004471));
#139636=CARTESIAN_POINT('Ctrl Pts',(117.273984287767,8.45283498799986,70.1750601865364));
#139637=CARTESIAN_POINT('Ctrl Pts',(117.098159722788,8.58895961478438,70.1351500200475));
#139638=CARTESIAN_POINT('Ctrl Pts',(116.951603325369,8.70242461840276,70.1018833930451));
#139639=CARTESIAN_POINT('Ctrl Pts',(116.80121154568,8.81511488236514,70.0677902031773));
#139640=CARTESIAN_POINT('Ctrl Pts',(116.647007803204,8.92689034648425,70.0328727497835));
#139641=CARTESIAN_POINT('Ctrl Pts',(116.458342625104,9.06364537918784,69.9901519476967));
#139642=CARTESIAN_POINT('Ctrl Pts',(116.263970617385,9.19903062515022,69.9461971697683));
#139643=CARTESIAN_POINT('Ctrl Pts',(116.063915585821,9.33278943972281,69.9010088645471));
#139644=CARTESIAN_POINT('Ctrl Pts',(115.956162455114,9.40483427117338,69.8766696548764));
#139645=CARTESIAN_POINT('Ctrl Pts',(115.846761399342,9.47640759478814,69.8519727368525));
#139646=CARTESIAN_POINT('Ctrl Pts',(115.73572181815,9.54747187918183,69.8269192787979));
#139647=CARTESIAN_POINT('Ctrl Pts',(115.528407371014,9.68015116950339,69.7801436718507));
#139648=CARTESIAN_POINT('Ctrl Pts',(115.315378836785,9.81105470690549,69.732124750275));
#139649=CARTESIAN_POINT('Ctrl Pts',(115.09668957018,9.93994417389922,69.6828685683572));
#139650=CARTESIAN_POINT('Ctrl Pts',(115.033851659791,9.9769791180592,69.6687153563888));
#139651=CARTESIAN_POINT('Ctrl Pts',(114.970546664127,10.013847921227,69.6544600469835));
#139652=CARTESIAN_POINT('Ctrl Pts',(114.906776553754,10.0505453006162,69.6401029203365));
#139653=CARTESIAN_POINT('Ctrl Pts',(114.683663611381,10.1789386849936,69.5898715384005));
#139654=CARTESIAN_POINT('Ctrl Pts',(114.45485392192,10.3052317113346,69.538393175952));
#139655=CARTESIAN_POINT('Ctrl Pts',(114.220422929518,10.4292047081467,69.4856780824899));
#139656=CARTESIAN_POINT('Ctrl Pts',(114.197912463071,10.4411088081827,69.4806162886951));
#139657=CARTESIAN_POINT('Ctrl Pts',(114.175350201025,10.4529915373186,69.4755430985869));
#139658=CARTESIAN_POINT('Ctrl Pts',(114.152736231951,10.4648527141662,69.4704585254692));
#139659=CARTESIAN_POINT('Ctrl Pts',(114.071950519389,10.5072253565056,69.4522944932711));
#139660=CARTESIAN_POINT('Ctrl Pts',(113.990504886149,10.5493229216099,69.4339851843099));
#139661=CARTESIAN_POINT('Ctrl Pts',(113.908402120511,10.5911370811685,69.4155309622082));
#139662=CARTESIAN_POINT('Ctrl Pts',(113.779449253332,10.656811552934,69.3865462522161));
#139663=CARTESIAN_POINT('Ctrl Pts',(113.648875154649,10.721786775683,69.3572040269525));
#139664=CARTESIAN_POINT('Ctrl Pts',(113.516693352567,10.7860324519638,69.3275062031431));
#139665=CARTESIAN_POINT('Ctrl Pts',(113.499773738249,10.7942560655561,69.3237048044859));
#139666=CARTESIAN_POINT('Ctrl Pts',(113.482827787115,10.8024677267741,69.319897582974));
#139667=CARTESIAN_POINT('Ctrl Pts',(113.465855531575,10.8106673757003,69.3160845426478));
#139668=CARTESIAN_POINT('Ctrl Pts',(113.416531260478,10.8344969548387,69.3050031967232));
#139669=CARTESIAN_POINT('Ctrl Pts',(113.366984821204,10.8582250772314,69.2938727050108));
#139670=CARTESIAN_POINT('Ctrl Pts',(113.31721717765,10.8818501694279,69.282693199195));
#139671=CARTESIAN_POINT('Ctrl Pts',(113.283770946889,10.8977273584796,69.2751800379398));
#139672=CARTESIAN_POINT('Ctrl Pts',(113.250224804113,10.9135580175483,69.2676447391799));
#139673=CARTESIAN_POINT('Ctrl Pts',(113.216579071131,10.9293416679507,69.2600873575252));
#139674=CARTESIAN_POINT('Ctrl Pts',(113.19975620464,10.937233493152,69.2563086666978));
#139675=CARTESIAN_POINT('Ctrl Pts',(113.182908440637,10.9451135663309,69.2525244552646));
#139676=CARTESIAN_POINT('Ctrl Pts',(113.16603581926,10.95298182955,69.2487347296099));
#139677=CARTESIAN_POINT('Ctrl Pts',(113.151272275554,10.9598665598666,69.2454187196621));
#139678=CARTESIAN_POINT('Ctrl Pts',(113.136489700425,10.9667422481908,69.2420984878953));
#139679=CARTESIAN_POINT('Ctrl Pts',(113.121688121565,10.9736088558954,69.2387740388456));
#139680=CARTESIAN_POINT('Ctrl Pts',(113.119573610299,10.9745897998531,69.2382991175528));
#139681=CARTESIAN_POINT('Ctrl Pts',(113.116366937548,10.976076666686,69.2375788978328));
#139682=CARTESIAN_POINT('Ctrl Pts',(113.115343424368,10.9765511317019,69.2373490167771));
#139683=CARTESIAN_POINT('Ctrl Pts',(113.022976761086,11.0193690955673,69.2166034646097));
#139684=CARTESIAN_POINT('Ctrl Pts',(112.930834667136,11.0613846056466,69.1959129276571));
#139685=CARTESIAN_POINT('Ctrl Pts',(112.838937704407,11.1026247607013,69.1752819476934));
#139686=CARTESIAN_POINT('Ctrl Pts',(112.647247007684,11.18864886662,69.1322471530072));
#139687=CARTESIAN_POINT('Ctrl Pts',(112.456623792903,11.2713003057167,69.0894716794575));
#139688=CARTESIAN_POINT('Ctrl Pts',(112.267226049986,11.3508294215004,69.0469910784709));
#139689=CARTESIAN_POINT('Ctrl Pts',(112.091732133461,11.4245202469117,69.0076290093744));
#139690=CARTESIAN_POINT('Ctrl Pts',(111.917290107844,11.4955301585317,68.9685200568115));
#139691=CARTESIAN_POINT('Ctrl Pts',(111.744005625658,11.5640455179087,68.9296884945963));
#139692=CARTESIAN_POINT('Ctrl Pts',(111.583303488104,11.627585914419,68.8936765276053));
#139693=CARTESIAN_POINT('Ctrl Pts',(111.423596748605,11.6889807462734,68.857903100716));
#139694=CARTESIAN_POINT('Ctrl Pts',(111.264959024318,11.7483700241455,68.8223854153186));
#139695=CARTESIAN_POINT('Ctrl Pts',(111.117639763161,11.8035220037654,68.7894018409872));
#139696=CARTESIAN_POINT('Ctrl Pts',(110.971242327098,11.8569443146203,68.7566387989538));
#139697=CARTESIAN_POINT('Ctrl Pts',(110.825819706005,11.9087425450732,68.7241088364224));
#139698=CARTESIAN_POINT('Ctrl Pts',(110.822811595885,11.9098140068585,68.7234359444833));
#139699=CARTESIAN_POINT('Ctrl Pts',(110.819803902725,11.9108847735399,68.7227631522441));
#139700=CARTESIAN_POINT('Ctrl Pts',(110.81679662689,11.9119548460335,68.722090459795));
#139701=CARTESIAN_POINT('Ctrl Pts',(110.692917690131,11.9560344217133,68.694380189795));
#139702=CARTESIAN_POINT('Ctrl Pts',(110.569747036027,11.9989362809017,68.6668392805372));
#139703=CARTESIAN_POINT('Ctrl Pts',(110.447309202222,12.040723069193,68.6394738570784));
#139704=CARTESIAN_POINT('Ctrl Pts',(110.439135614158,12.0435126317275,68.6376470222547));
#139705=CARTESIAN_POINT('Ctrl Pts',(110.430965292181,12.0462972237657,68.6358209693533));
#139706=CARTESIAN_POINT('Ctrl Pts',(110.422798243196,12.0490768635367,68.6339957001427));
#139707=CARTESIAN_POINT('Ctrl Pts',(110.36979535197,12.0671162979387,68.6221499838254));
#139708=CARTESIAN_POINT('Ctrl Pts',(110.316930317783,12.0849471593495,68.6103372761136));
#139709=CARTESIAN_POINT('Ctrl Pts',(110.264205167338,12.1025741348408,68.5985580867996));
#139710=CARTESIAN_POINT('Ctrl Pts',(110.233780465725,12.1127456652231,68.5917609830058));
#139711=CARTESIAN_POINT('Ctrl Pts',(110.203402341482,12.1228493053584,68.5849750381828));
#139712=CARTESIAN_POINT('Ctrl Pts',(110.173071187232,12.1328859391197,68.5782003503594));
#139713=CARTESIAN_POINT('Ctrl Pts',(110.157905610107,12.1379042560003,68.5748130064478));
#139714=CARTESIAN_POINT('Ctrl Pts',(110.142751775457,12.1429058211661,68.5714284767039));
#139715=CARTESIAN_POINT('Ctrl Pts',(110.127609731102,12.1478907445677,68.5680467728983));
#139716=CARTESIAN_POINT('Ctrl Pts',(110.116253197836,12.1516294371188,68.5655104950441));
#139717=CARTESIAN_POINT('Ctrl Pts',(110.104903296609,12.1553587686674,68.5629758067734));
#139718=CARTESIAN_POINT('Ctrl Pts',(110.093560047501,12.1590787853552,68.5604427130416));
#139719=CARTESIAN_POINT('Ctrl Pts',(110.089778964465,12.1603187909178,68.5595983484643));
#139720=CARTESIAN_POINT('Ctrl Pts',(110.084399591553,12.1620814929756,68.558397087533));
#139721=CARTESIAN_POINT('Ctrl Pts',(110.0822190165,12.1627956987876,68.5579101510084));
#139722=CARTESIAN_POINT('Ctrl Pts',(110.072323754785,12.1660367032268,68.5557004750138));
#139723=CARTESIAN_POINT('Ctrl Pts',(110.062433616717,12.1692706333837,68.5534919885118));
#139724=CARTESIAN_POINT('Ctrl Pts',(110.052548615494,12.1724975198481,68.5512846947003));
#139725=CARTESIAN_POINT('Ctrl Pts',(109.938374789075,12.2097687317332,68.5257899906722));
#139726=CARTESIAN_POINT('Ctrl Pts',(109.8248863585,12.2461004228557,68.5004544222776));
#139727=CARTESIAN_POINT('Ctrl Pts',(109.712102670886,12.281538637848,68.4752827117343));
#139728=CARTESIAN_POINT('Ctrl Pts',(109.607043021169,12.3145498519027,68.4518348962885));
#139729=CARTESIAN_POINT('Ctrl Pts',(109.502594871715,12.3467857576586,68.4285292596018));
#139730=CARTESIAN_POINT('Ctrl Pts',(109.398772151862,12.3782819466524,68.4053692677365));
#139731=CARTESIAN_POINT('Ctrl Pts',(109.30209569012,12.4076102103943,68.3838034094094));
#139732=CARTESIAN_POINT('Ctrl Pts',(109.205961515276,12.4362970684511,68.3623638344511));
#139733=CARTESIAN_POINT('Ctrl Pts',(109.110380718673,12.4643700095465,68.3410532969063));
#139734=CARTESIAN_POINT('Ctrl Pts',(109.02135376668,12.490518027433,68.3212039938));
#139735=CARTESIAN_POINT('Ctrl Pts',(108.932806884898,12.5161334224034,68.3014666347423));
#139736=CARTESIAN_POINT('Ctrl Pts',(108.844745739944,12.5412378420218,68.2818427936572));
#139737=CARTESIAN_POINT('Ctrl Pts',(108.76259187315,12.5646582182426,68.2635353502629));
#139738=CARTESIAN_POINT('Ctrl Pts',(108.680860819629,12.5876338582503,68.2453267170413));
#139739=CARTESIAN_POINT('Ctrl Pts',(108.599570303343,12.6101796727279,68.2272207144974));
#139740=CARTESIAN_POINT('Ctrl Pts',(108.523569128167,12.6312584956201,68.2102928176904));
#139741=CARTESIAN_POINT('Ctrl Pts',(108.447952977039,12.6519616243288,68.1934546206468));
#139742=CARTESIAN_POINT('Ctrl Pts',(108.372726394293,12.6723051469411,68.176707307025));
#139743=CARTESIAN_POINT('Ctrl Pts',(108.30264726269,12.6912566444887,68.1611059444154));
#139744=CARTESIAN_POINT('Ctrl Pts',(108.232906198054,12.7098960577254,68.1455834507468));
#139745=CARTESIAN_POINT('Ctrl Pts',(108.163504487578,12.7282358457574,68.1301403141801));
#139746=CARTESIAN_POINT('Ctrl Pts',(108.099358819916,12.7451866952396,68.1158667422599));
#139747=CARTESIAN_POINT('Ctrl Pts',(108.035503077865,12.7618815736574,68.1016609676239));
#139748=CARTESIAN_POINT('Ctrl Pts',(107.971945043125,12.7783284770643,68.0875246872087));
#139749=CARTESIAN_POINT('Ctrl Pts',(107.913572073927,12.7934336418153,68.074541644787));
#139750=CARTESIAN_POINT('Ctrl Pts',(107.855450122654,12.8083296560643,68.0616172015617));
#139751=CARTESIAN_POINT('Ctrl Pts',(107.797560039676,12.8230276174717,68.048747775443));
#139752=CARTESIAN_POINT('Ctrl Pts',(107.760781209992,12.8323655522525,68.0405715489289));
#139753=CARTESIAN_POINT('Ctrl Pts',(107.72409599404,12.8416235330491,68.0324175337652));
#139754=CARTESIAN_POINT('Ctrl Pts',(107.687502594336,12.8508023216245,68.024285416003));
#139755=CARTESIAN_POINT('Ctrl Pts',(107.670503421704,12.8550662548149,68.0205077054097));
#139756=CARTESIAN_POINT('Ctrl Pts',(107.65352406376,12.8593130984262,68.0167347204085));
#139757=CARTESIAN_POINT('Ctrl Pts',(107.636564348739,12.8635429281521,68.0129664310072));
#139758=CARTESIAN_POINT('Ctrl Pts',(107.622044777864,12.8671641748781,68.0097403187187));
#139759=CARTESIAN_POINT('Ctrl Pts',(107.607539604355,12.8707729513676,68.0065176480808));
#139760=CARTESIAN_POINT('Ctrl Pts',(107.593048900532,12.8743692770539,68.003298435271));
#139761=CARTESIAN_POINT('Ctrl Pts',(107.577340550319,12.8782678001381,67.9998087136645));
#139762=CARTESIAN_POINT('Ctrl Pts',(107.561649142762,12.8821517050661,67.9963230454734));
#139763=CARTESIAN_POINT('Ctrl Pts',(107.545974860605,12.8860209974835,67.9928414660428));
#139764=CARTESIAN_POINT('Ctrl Pts',(107.530300578449,12.889890289901,67.9893598866122));
#139765=CARTESIAN_POINT('Ctrl Pts',(107.522944596978,12.8916999342926,67.9877262919716));
#139766=CARTESIAN_POINT('Ctrl Pts',(107.513208003348,12.8940940479048,67.985564593278));
#139767=CARTESIAN_POINT('Ctrl Pts',(107.503465179159,12.8964896935383,67.9834015112883));
#139768=CARTESIAN_POINT('Ctrl Pts',(107.493720506002,12.8988815104539,67.9812385969309));
#139769=CARTESIAN_POINT('Ctrl Pts',(107.483974020144,12.9012694810469,67.9790758600759));
#139770=CARTESIAN_POINT('Ctrl Pts',(107.454759494175,12.9084272843738,67.9725931818126));
#139771=CARTESIAN_POINT('Ctrl Pts',(107.425528681299,12.9155505295199,67.9661120982754));
#139772=CARTESIAN_POINT('Ctrl Pts',(107.396282628794,12.9226386763674,67.9596328889247));
#139773=CARTESIAN_POINT('Ctrl Pts',(107.375802408792,12.9276023140007,67.9550956737599));
#139774=CARTESIAN_POINT('Ctrl Pts',(107.355314482445,12.9325488044428,67.9505593124497));
#139775=CARTESIAN_POINT('Ctrl Pts',(107.334819026733,12.9374780121642,67.9460238496044));
#139776=CARTESIAN_POINT('Ctrl Pts',(107.284986691471,12.9494628118774,67.9349963951164));
#139777=CARTESIAN_POINT('Ctrl Pts',(107.235109852007,12.9613454408864,67.9239742535486));
#139778=CARTESIAN_POINT('Ctrl Pts',(107.185183076581,12.9731273009532,67.9129565133477));
#139779=CARTESIAN_POINT('Ctrl Pts',(107.177432063034,12.974956406803,67.9112460352959));
#139780=CARTESIAN_POINT('Ctrl Pts',(107.169679845774,12.9767830839771,67.9095356632865));
#139781=CARTESIAN_POINT('Ctrl Pts',(107.161926525056,12.978607292919,67.9078254173392));
#139782=CARTESIAN_POINT('Ctrl Pts',(107.122808841323,12.9878109401107,67.8991967455085));
#139783=CARTESIAN_POINT('Ctrl Pts',(107.083663058977,12.9969517614264,67.8905712807437));
#139784=CARTESIAN_POINT('Ctrl Pts',(107.044502082751,13.0060246694447,67.8819515950965));
#139785=CARTESIAN_POINT('Ctrl Pts',(107.040777543951,13.0068875794435,67.881131790364));
#139786=CARTESIAN_POINT('Ctrl Pts',(107.037041572928,13.0077523596621,67.8803097895492));
#139787=CARTESIAN_POINT('Ctrl Pts',(107.033299158713,13.0086179012633,67.8794865887452));
#139788=CARTESIAN_POINT('Ctrl Pts',(107.001299623324,13.0160187199605,67.8724478052909));
#139789=CARTESIAN_POINT('Ctrl Pts',(106.968831198066,13.0234723671859,67.8653217039039));
#139790=CARTESIAN_POINT('Ctrl Pts',(106.939044759508,13.030304302297,67.8587372704961));
#139791=CARTESIAN_POINT('Ctrl Pts',(106.935687244491,13.031074395193,67.8579950758895));
#139792=CARTESIAN_POINT('Ctrl Pts',(106.93236376191,13.031836624841,67.8572597550974));
#139793=CARTESIAN_POINT('Ctrl Pts',(106.929078782905,13.0325900521754,67.8565322009618));
#139794=CARTESIAN_POINT('Ctrl Pts',(106.91249838228,13.0363928548811,67.8528599890459));
#139795=CARTESIAN_POINT('Ctrl Pts',(106.896778178434,13.0399979246535,67.8493611719163));
#139796=CARTESIAN_POINT('Ctrl Pts',(106.881919084311,13.043408582267,67.8460359447363));
#139797=CARTESIAN_POINT('Ctrl Pts',(106.864662306634,13.047369588213,67.8421741543944));
#139798=CARTESIAN_POINT('Ctrl Pts',(106.848566718302,13.0510684622532,67.8385464484074));
#139799=CARTESIAN_POINT('Ctrl Pts',(106.833626578492,13.0545108729687,67.8351517377061));
#139800=CARTESIAN_POINT('Ctrl Pts',(106.819724341824,13.0577141367323,67.8319928601997));
#139801=CARTESIAN_POINT('Ctrl Pts',(106.806822543637,13.06069531364,67.8290357206569));
#139802=CARTESIAN_POINT('Ctrl Pts',(106.794915963268,13.0634580977053,67.8262793282536));
#139803=CARTESIAN_POINT('Ctrl Pts',(106.788962673084,13.0648394897379,67.8249011320519));
#139804=CARTESIAN_POINT('Ctrl Pts',(106.783258186263,13.0661662732176,67.8235731169913));
#139805=CARTESIAN_POINT('Ctrl Pts',(106.777801832488,13.0674388372552,67.8222951621539));
#139806=CARTESIAN_POINT('Ctrl Pts',(106.7750736556,13.068075119274,67.8216561847352));
#139807=CARTESIAN_POINT('Ctrl Pts',(106.772407511919,13.0686978459035,67.8210297220832));
#139808=CARTESIAN_POINT('Ctrl Pts',(106.769803319567,13.0693070619732,67.8204157585113));
#139809=CARTESIAN_POINT('Ctrl Pts',(106.767199127215,13.069916278043,67.8198017949394));
#139810=CARTESIAN_POINT('Ctrl Pts',(106.765788256114,13.0702464080975,67.8194689818855));
#139811=CARTESIAN_POINT('Ctrl Pts',(106.762176514847,13.0710942211172,67.8186113489208));
#139812=CARTESIAN_POINT('Ctrl Pts',(106.755061254481,13.0727644432987,67.816921781094));
#139813=CARTESIAN_POINT('Ctrl Pts',(106.747578771434,13.0745366460299,67.8151138078794));
#139814=CARTESIAN_POINT('Ctrl Pts',(106.739731130454,13.0764100827743,67.8131877287666));
#139815=CARTESIAN_POINT('Ctrl Pts',(106.721835157183,13.0806823187216,67.8087954457347));
#139816=CARTESIAN_POINT('Ctrl Pts',(106.702043963982,13.0854801299258,67.8037897445064));
#139817=CARTESIAN_POINT('Ctrl Pts',(106.680330865469,13.0908060953199,67.7981637067688));
#139818=CARTESIAN_POINT('Ctrl Pts',(106.672900165201,13.0926287579148,67.7962383528126));
#139819=CARTESIAN_POINT('Ctrl Pts',(106.665243984317,13.0945133706204,67.7942402645645));
#139820=CARTESIAN_POINT('Ctrl Pts',(106.657359828321,13.0964603835544,67.7921688682916));
#139821=CARTESIAN_POINT('Ctrl Pts',(106.64710361838,13.0989931814114,67.7894742647021));
#139822=CARTESIAN_POINT('Ctrl Pts',(106.637434211784,13.1013940754706,67.7869072339959));
#139823=CARTESIAN_POINT('Ctrl Pts',(106.623515944922,13.1048499015932,67.7832060106365));
#139824=CARTESIAN_POINT('Ctrl Pts',(106.616286187049,13.1066450091568,67.7812834329918));
#139825=CARTESIAN_POINT('Ctrl Pts',(106.609356367751,13.108364189616,67.779441852242));
#139826=CARTESIAN_POINT('Ctrl Pts',(106.602726151841,13.1100077596478,67.7776812720829));
#139827=CARTESIAN_POINT('Ctrl Pts',(106.59659230068,13.1115282853869,67.7760524960676));
#139828=CARTESIAN_POINT('Ctrl Pts',(106.590715050085,13.1129840540664,67.7744930809063));
#139829=CARTESIAN_POINT('Ctrl Pts',(106.585097803888,13.1143743934587,67.7730037378273));
#139830=CARTESIAN_POINT('Ctrl Pts',(106.569098466814,13.1183344314928,67.7687617122677));
#139831=CARTESIAN_POINT('Ctrl Pts',(106.555212866438,13.1217626845447,67.7650890351599));
#139832=CARTESIAN_POINT('Ctrl Pts',(106.543469016872,13.1246550059365,67.7619920879952));
#139833=CARTESIAN_POINT('Ctrl Pts',(106.538052846431,13.1259889216633,67.7605638004819));
#139834=CARTESIAN_POINT('Ctrl Pts',(106.533091358535,13.1272090379781,67.7592577974129));
#139835=CARTESIAN_POINT('Ctrl Pts',(106.528584066935,13.128315652714,67.7580740539427));
#139836=CARTESIAN_POINT('Ctrl Pts',(106.521443854595,13.1300686930967,67.756198830309));
#139837=CARTESIAN_POINT('Ctrl Pts',(106.515443483395,13.1315369037267,67.7546304291683));
#139838=CARTESIAN_POINT('Ctrl Pts',(106.510576637615,13.132722318494,67.7533678281773));
#139839=CARTESIAN_POINT('Ctrl Pts',(106.508143214724,13.1333150258776,67.7527365276818));
#139840=CARTESIAN_POINT('Ctrl Pts',(106.505993172956,13.133837032103,67.7521816760642));
#139841=CARTESIAN_POINT('Ctrl Pts',(106.504125557165,13.1342886081154,67.7517031047385));
#139842=CARTESIAN_POINT('Ctrl Pts',(106.502257941373,13.1347401841277,67.7512245334127));
#139843=CARTESIAN_POINT('Ctrl Pts',(106.49588082428,13.1362765541258,67.7496003744427));
#139844=CARTESIAN_POINT('Ctrl Pts',(106.490817428601,13.1374893006029,67.7483228513659));
#139845=CARTESIAN_POINT('Ctrl Pts',(106.48119359659,13.1397943285143,67.7458947046714));
#139846=CARTESIAN_POINT('Ctrl Pts',(106.471701611211,13.1420471000255,67.7435349913479));
#139847=CARTESIAN_POINT('Ctrl Pts',(106.462350082912,13.1442457702362,67.7412455172647));
#139848=CARTESIAN_POINT('Ctrl Pts',(106.452021098116,13.14667425363,67.7387167388404));
#139849=CARTESIAN_POINT('Ctrl Pts',(106.441862393324,13.1490369570712,67.7362734421338));
#139850=CARTESIAN_POINT('Ctrl Pts',(106.431801048307,13.1513488950868,67.7339015993084));
#139851=CARTESIAN_POINT('Ctrl Pts',(106.416822847289,13.1547906488759,67.730370665963));
#139852=CARTESIAN_POINT('Ctrl Pts',(106.402058175558,13.15812035499,67.7269976603332));
#139853=CARTESIAN_POINT('Ctrl Pts',(106.387310281136,13.1613785817389,67.7237446851911));
#139854=CARTESIAN_POINT('Ctrl Pts',(106.383182383448,13.1622905510192,67.722834185822));
#139855=CARTESIAN_POINT('Ctrl Pts',(106.379056104298,13.1631968581735,67.7219331480982));
#139856=CARTESIAN_POINT('Ctrl Pts',(106.374927825296,13.1640982503239,67.7210408740254));
#139857=CARTESIAN_POINT('Ctrl Pts',(106.372078037868,13.1647204892804,67.7204249293584));
#139858=CARTESIAN_POINT('Ctrl Pts',(106.369600961509,13.1652606190883,67.7198905614545));
#139859=CARTESIAN_POINT('Ctrl Pts',(106.366447297663,13.1659433443158,67.7192190674479));
#139860=CARTESIAN_POINT('Ctrl Pts',(106.364378343724,13.1663912446366,67.7187785353438));
#139861=CARTESIAN_POINT('Ctrl Pts',(106.362017963058,13.1669005568351,67.718278940623));
#139862=CARTESIAN_POINT('Ctrl Pts',(106.359057790106,13.1675369937063,67.7176561793993));
#139863=CARTESIAN_POINT('Ctrl Pts',(106.351585486534,13.1691435381826,67.716084156078));
#139864=CARTESIAN_POINT('Ctrl Pts',(106.344551231825,13.1706374186641,67.714636281189));
#139865=CARTESIAN_POINT('Ctrl Pts',(106.337977136572,13.172014705402,67.7133168711505));
#139866=CARTESIAN_POINT('Ctrl Pts',(106.331084534732,13.1734587199378,67.7119335373667));
#139867=CARTESIAN_POINT('Ctrl Pts',(106.324698195333,13.1747744827679,67.7106915025314));
#139868=CARTESIAN_POINT('Ctrl Pts',(106.318853271182,13.1759554068276,67.7095975998564));
#139869=CARTESIAN_POINT('Ctrl Pts',(106.313548534001,13.1770271900716,67.7086047954943));
#139870=CARTESIAN_POINT('Ctrl Pts',(106.308691606398,13.1779874404298,67.7077343662016));
#139871=CARTESIAN_POINT('Ctrl Pts',(106.304319984305,13.1788283115832,67.7069935851384));
#139872=CARTESIAN_POINT('Ctrl Pts',(106.300005982892,13.1796580995351,67.7062625680274));
#139873=CARTESIAN_POINT('Ctrl Pts',(106.296642203784,13.1802964496147,67.7057071864585));
#139874=CARTESIAN_POINT('Ctrl Pts',(106.293337987742,13.180883497628,67.7052366830344));
#139875=CARTESIAN_POINT('Ctrl Pts',(106.289604539133,13.1815468058258,67.7047050590935));
#139876=CARTESIAN_POINT('Ctrl Pts',(106.285946224121,13.1821450426698,67.7042816525951));
#139877=CARTESIAN_POINT('Ctrl Pts',(106.281022253892,13.1828882466645,67.7038243463946));
#139878=CARTESIAN_POINT('Ctrl Pts',(106.271740419626,13.1842892088927,67.70296231024));
#139879=CARTESIAN_POINT('Ctrl Pts',(106.261586075307,13.1856188361054,67.7023892838068));
#139880=CARTESIAN_POINT('Ctrl Pts',(106.250595879928,13.1868548838305,67.7021085788158));
#139881=CARTESIAN_POINT('Ctrl Pts',(106.24031401124,13.1880112673127,67.7018459654812));
#139882=CARTESIAN_POINT('Ctrl Pts',(106.229300211162,13.1890858286411,67.701839117714));
#139883=CARTESIAN_POINT('Ctrl Pts',(106.217628154117,13.1900446528357,67.7020972302163));
#139884=CARTESIAN_POINT('Ctrl Pts',(106.216824056165,13.1901107070511,67.7021150118065));
#139885=CARTESIAN_POINT('Ctrl Pts',(106.216016853597,13.1901762051296,67.7021340538944));
#139886=CARTESIAN_POINT('Ctrl Pts',(106.215206579378,13.1902411328607,67.7021543608706));
#139887=CARTESIAN_POINT('Ctrl Pts',(106.205123047467,13.1910491319709,67.7024070729002));
#139888=CARTESIAN_POINT('Ctrl Pts',(106.196684534129,13.1916384135438,67.7027328843449));
#139889=CARTESIAN_POINT('Ctrl Pts',(106.188340648465,13.1921930927188,67.7030670039973));
#139890=CARTESIAN_POINT('Ctrl Pts',(106.186281512678,13.1923299785518,67.7031494593138));
#139891=CARTESIAN_POINT('Ctrl Pts',(106.184228288793,13.1924645903933,67.703232430564));
#139892=CARTESIAN_POINT('Ctrl Pts',(106.182158194736,13.1925993098119,67.703315008817));
#139893=CARTESIAN_POINT('Ctrl Pts',(106.175310982203,13.1930449187873,67.7035881514053));
#139894=CARTESIAN_POINT('Ctrl Pts',(106.168503036321,13.1934317655783,67.7039321299558));
#139895=CARTESIAN_POINT('Ctrl Pts',(106.161795839839,13.1937842631555,67.7042881765257));
#139896=CARTESIAN_POINT('Ctrl Pts',(106.148013987272,13.1945085701969,67.7050197759869));
#139897=CARTESIAN_POINT('Ctrl Pts',(106.13465843368,13.1950869560501,67.7058015508074));
#139898=CARTESIAN_POINT('Ctrl Pts',(106.122049394182,13.1958248934581,67.706094333502));
#139899=CARTESIAN_POINT('Ctrl Pts',(106.112676661907,13.1963734276872,67.7063119689382));
#139900=CARTESIAN_POINT('Ctrl Pts',(106.103735822729,13.1970865540103,67.7061195139772));
#139901=CARTESIAN_POINT('Ctrl Pts',(106.095200154032,13.1979828221813,67.7055165398966));
#139902=CARTESIAN_POINT('Ctrl Pts',(106.090932319683,13.1984309562668,67.7052150528563));
#139903=CARTESIAN_POINT('Ctrl Pts',(106.086765773032,13.1989248004721,67.7048108946205));
#139904=CARTESIAN_POINT('Ctrl Pts',(106.082697785093,13.1994661513858,67.7043038387365));
#139905=CARTESIAN_POINT('Ctrl Pts',(106.079433660559,13.1999005275013,67.7038969807084));
#139906=CARTESIAN_POINT('Ctrl Pts',(106.075433665888,13.2004973756032,67.7032766697359));
#139907=CARTESIAN_POINT('Ctrl Pts',(106.072621105963,13.2009398356224,67.7027971657393));
#139908=CARTESIAN_POINT('Ctrl Pts',(106.071928450406,13.201048801262,67.7026790771948));
#139909=CARTESIAN_POINT('Ctrl Pts',(106.071307549541,13.2011484789228,67.702569477134));
#139910=CARTESIAN_POINT('Ctrl Pts',(106.070786735959,13.2012342432933,67.7024735795054));
#139911=CARTESIAN_POINT('Ctrl Pts',(106.062743425631,13.2025587660585,67.7009925613209));
#139912=CARTESIAN_POINT('Ctrl Pts',(106.052634650792,13.2044505865399,67.698700221847));
#139913=CARTESIAN_POINT('Ctrl Pts',(106.040575469081,13.2068972755518,67.6956180730002));
#139914=CARTESIAN_POINT('Ctrl Pts',(106.034052331577,13.2082207558042,67.6939508553383));
#139915=CARTESIAN_POINT('Ctrl Pts',(106.026958761435,13.2097069844791,67.6920525515875));
#139916=CARTESIAN_POINT('Ctrl Pts',(106.019310196946,13.2113605995131,67.6899257675537));
#139917=CARTESIAN_POINT('Ctrl Pts',(106.007982879047,13.2138095588178,67.6867760577111));
#139918=CARTESIAN_POINT('Ctrl Pts',(105.995440848126,13.2166267903083,67.6831257606122));
#139919=CARTESIAN_POINT('Ctrl Pts',(105.981708195429,13.2198130341267,67.6789775432847));
#139920=CARTESIAN_POINT('Ctrl Pts',(105.976918915918,13.2209242405757,67.6775308473918));
#139921=CARTESIAN_POINT('Ctrl Pts',(105.971984418664,13.2220803488126,67.6760235041644));
#139922=CARTESIAN_POINT('Ctrl Pts',(105.966904141517,13.2232814677876,67.6744552939442));
#139923=CARTESIAN_POINT('Ctrl Pts',(105.960175911557,13.2248722086941,67.6723783838305));
#139924=CARTESIAN_POINT('Ctrl Pts',(105.952029538102,13.2268285903403,67.6698157172125));
#139925=CARTESIAN_POINT('Ctrl Pts',(105.945397850862,13.228429470037,67.6677187219855));
#139926=CARTESIAN_POINT('Ctrl Pts',(105.940283703307,13.229664017851,67.666101585558));
#139927=CARTESIAN_POINT('Ctrl Pts',(105.936067560064,13.2306871257169,67.664760947505));
#139928=CARTESIAN_POINT('Ctrl Pts',(105.934085177048,13.231167367077,67.6641321742009));
#139929=CARTESIAN_POINT('Ctrl Pts',(105.929532171261,13.2322703535704,67.6626880493931));
#139930=CARTESIAN_POINT('Ctrl Pts',(105.924436613309,13.2334938104782,67.661093619133));
#139931=CARTESIAN_POINT('Ctrl Pts',(105.918796795571,13.2348382984781,67.6593483847178));
#139932=CARTESIAN_POINT('Ctrl Pts',(105.909551022734,13.23704241769,67.6564872920905));
#139933=CARTESIAN_POINT('Ctrl Pts',(105.898845834699,13.2395716061723,67.6532215584016));
#139934=CARTESIAN_POINT('Ctrl Pts',(105.886639951472,13.2424306572284,67.649542283528));
#139935=CARTESIAN_POINT('Ctrl Pts',(105.872690840467,13.2456980341,67.6453375395795));
#139936=CARTESIAN_POINT('Ctrl Pts',(105.856771681814,13.2493967029723,67.6405907412848));
#139937=CARTESIAN_POINT('Ctrl Pts',(105.838891079168,13.2535316119723,67.6353019750921));
#139938=CARTESIAN_POINT('Ctrl Pts',(105.823539175591,13.2570817565354,67.630761153385));
#139939=CARTESIAN_POINT('Ctrl Pts',(105.806740930001,13.2609535270673,67.6258207238569));
#139940=CARTESIAN_POINT('Ctrl Pts',(105.788540076225,13.2651488956576,67.6204880111972));
#139941=CARTESIAN_POINT('Ctrl Pts',(105.778599083373,13.267440333723,67.6175753753901));
#139942=CARTESIAN_POINT('Ctrl Pts',(105.768240401289,13.269828281464,67.6145458546616));
#139943=CARTESIAN_POINT('Ctrl Pts',(105.757477831466,13.2723128046513,67.6114019202545));
#139944=CARTESIAN_POINT('Ctrl Pts',(105.756521354661,13.2725336058947,67.6111225166934));
#139945=CARTESIAN_POINT('Ctrl Pts',(105.755569399813,13.2727533590239,67.6108445215215));
#139946=CARTESIAN_POINT('Ctrl Pts',(105.754621927495,13.2729720724131,67.610567924591));
#139947=CARTESIAN_POINT('Ctrl Pts',(105.738323688053,13.2767343387243,67.6058099565607));
#139948=CARTESIAN_POINT('Ctrl Pts',(105.723346557623,13.2801893902145,67.6014647422791));
#139949=CARTESIAN_POINT('Ctrl Pts',(105.709403813386,13.2833878795956,67.5974636595106));
#139950=CARTESIAN_POINT('Ctrl Pts',(105.6926733995,13.2872258651633,67.5926626124879));
#139951=CARTESIAN_POINT('Ctrl Pts',(105.677434081816,13.2906942185066,67.5883574104592));
#139952=CARTESIAN_POINT('Ctrl Pts',(105.663267608136,13.293874588328,67.584443733116));
#139953=CARTESIAN_POINT('Ctrl Pts',(105.654765750246,13.295783253312,67.582094981454));
#139954=CARTESIAN_POINT('Ctrl Pts',(105.646651510083,13.2975881134783,67.5798874653339));
#139955=CARTESIAN_POINT('Ctrl Pts',(105.638840450611,13.2993065510575,67.5777996826804));
#139956=CARTESIAN_POINT('Ctrl Pts',(105.630171984851,13.3012136185134,67.5754827277899));
#139957=CARTESIAN_POINT('Ctrl Pts',(105.621973986663,13.302993911731,67.5733372110151));
#139958=CARTESIAN_POINT('Ctrl Pts',(105.614251444181,13.3046459269888,67.5713643636819));
#139959=CARTESIAN_POINT('Ctrl Pts',(105.60758463171,13.3060720992562,67.5696612195124));
#139960=CARTESIAN_POINT('Ctrl Pts',(105.601272756613,13.3074025696676,67.5680868753423));
#139961=CARTESIAN_POINT('Ctrl Pts',(105.595327344932,13.308635035678,67.5666436941515));
#139962=CARTESIAN_POINT('Ctrl Pts',(105.588366685201,13.3100779595644,67.5649540730222));
#139963=CARTESIAN_POINT('Ctrl Pts',(105.579139427266,13.3119575615898,67.5627781036788));
#139964=CARTESIAN_POINT('Ctrl Pts',(105.568996708876,13.3139954644155,67.5604370755091));
#139965=CARTESIAN_POINT('Ctrl Pts',(105.560440831955,13.3157145346964,67.558462304238));
#139966=CARTESIAN_POINT('Ctrl Pts',(105.551234493553,13.3175459511269,67.5563702709175));
#139967=CARTESIAN_POINT('Ctrl Pts',(105.542217628589,13.3193176560284,67.5543595389247));
#139968=CARTESIAN_POINT('Ctrl Pts',(105.52456366563,13.3227864462153,67.5504227617565));
#139969=CARTESIAN_POINT('Ctrl Pts',(105.505715838934,13.3264175887521,67.5463440398532));
#139970=CARTESIAN_POINT('Ctrl Pts',(105.485721490407,13.3301897222825,67.54213280598));
#139971=CARTESIAN_POINT('Ctrl Pts',(105.479197662337,13.3314205076005,67.5407587494202));
#139972=CARTESIAN_POINT('Ctrl Pts',(105.47255214769,13.3326661856339,67.5393706573031));
#139973=CARTESIAN_POINT('Ctrl Pts',(105.465787761714,13.3339256480176,67.5379690826581));
#139974=CARTESIAN_POINT('Ctrl Pts',(105.447000822801,13.3374235919477,67.5340764459385));
#139975=CARTESIAN_POINT('Ctrl Pts',(105.427296437372,13.3410278363802,67.5300797135526));
#139976=CARTESIAN_POINT('Ctrl Pts',(105.406695522736,13.3447315623451,67.5259830318283));
#139977=CARTESIAN_POINT('Ctrl Pts',(105.406714415269,13.34497198119,67.526105385012));
#139978=CARTESIAN_POINT('Ctrl Pts',(105.724920227002,13.896301628367,66.3930340896861));
#139979=CARTESIAN_POINT('Ctrl Pts',(105.782792744022,13.149274277058,65.4129414870055));
#139980=CARTESIAN_POINT('Ctrl Pts',(105.588267881069,12.0114366406,65.374894609145));
#139981=CARTESIAN_POINT('Ctrl Pts',(105.479711788869,13.16446974828,67.8027942772491));
#139982=CARTESIAN_POINT('Ctrl Pts',(105.404457854469,13.17797674511,67.7881663212369));
#139983=CARTESIAN_POINT('Ctrl Pts',(105.217622405069,13.21120999594,67.751849007578));
#139984=CARTESIAN_POINT('Ctrl Pts',(104.909728623269,13.26478499412,67.692000220443));
#139985=CARTESIAN_POINT('Ctrl Pts',(104.545556898969,13.32647740523,67.62121205483));
#139986=CARTESIAN_POINT('Ctrl Pts',(104.149966793169,13.3916066705,67.544316744054));
#139987=CARTESIAN_POINT('Ctrl Pts',(103.719952703269,13.46028345385,67.460730055209));
#139988=CARTESIAN_POINT('Ctrl Pts',(103.252302141369,13.53257321139,67.369827540788));
#139989=CARTESIAN_POINT('Ctrl Pts',(102.743743443769,13.60837809399,67.270973250634));
#139990=CARTESIAN_POINT('Ctrl Pts',(102.190923130269,13.68750427689,67.163515330951));
#139991=CARTESIAN_POINT('Ctrl Pts',(101.590499923169,13.76962735539,67.046804299923));
#139992=CARTESIAN_POINT('Ctrl Pts',(100.939068251569,13.85431465257,66.920178178317));
#139993=CARTESIAN_POINT('Ctrl Pts',(100.232496010669,13.94110230146,66.782833762325));
#139994=CARTESIAN_POINT('Ctrl Pts',(99.4656780020691,14.02948909557,66.633778696936));
#139995=CARTESIAN_POINT('Ctrl Pts',(98.7641160173691,14.10476175395,66.49740818094));
#139996=CARTESIAN_POINT('Ctrl Pts',(98.3174346082691,14.14979091774,66.410581677263));
#139997=CARTESIAN_POINT('Ctrl Pts',(98.147852524169,14.16647603684,66.37761809484));
#139998=CARTESIAN_POINT('Ctrl Pts',(105.898861939469,14.14039115007,66.547598800864));
#139999=CARTESIAN_POINT('Ctrl Pts',(105.822628287069,14.15407399291,66.532780405995));
#140000=CARTESIAN_POINT('Ctrl Pts',(105.633399482669,14.18773289908,66.4959978689441));
#140001=CARTESIAN_POINT('Ctrl Pts',(105.321708482069,14.24196843757,66.4354109735431));
#140002=CARTESIAN_POINT('Ctrl Pts',(104.953242302369,14.30438814198,66.363788046205));
#140003=CARTESIAN_POINT('Ctrl Pts',(104.553186949569,14.37025226255,66.286024775006));
#140004=CARTESIAN_POINT('Ctrl Pts',(104.118570678569,14.43966385608,66.201543508307));
#140005=CARTESIAN_POINT('Ctrl Pts',(103.646007691069,14.51271290559,66.109686110311));
#140006=CARTESIAN_POINT('Ctrl Pts',(103.132149783669,14.5893076241,66.009801752982));
#140007=CARTESIAN_POINT('Ctrl Pts',(102.573627663069,14.66924981062,65.901235508739));
#140008=CARTESIAN_POINT('Ctrl Pts',(101.967092525769,14.7522086941,65.7833364328971));
#140009=CARTESIAN_POINT('Ctrl Pts',(101.309152996869,14.83774177889,65.655445305682));
#140010=CARTESIAN_POINT('Ctrl Pts',(100.595686651869,14.92537590466,65.516760804898));
#140011=CARTESIAN_POINT('Ctrl Pts',(99.8215835246691,15.01460202113,65.366289648841));
#140012=CARTESIAN_POINT('Ctrl Pts',(99.1135435814691,15.09056933134,65.228659939006));
#140013=CARTESIAN_POINT('Ctrl Pts',(98.6628310930692,15.13600478504,65.1410498689811));
#140014=CARTESIAN_POINT('Ctrl Pts',(98.4917311527691,15.15283924478,65.107791243718));
#140015=CARTESIAN_POINT('Ctrl Pts',(106.014802693469,13.27644852387,65.1534015425141));
#140016=CARTESIAN_POINT('Ctrl Pts',(105.939436344769,13.28997569756,65.1387517352451));
#140017=CARTESIAN_POINT('Ctrl Pts',(105.752326277969,13.32325778875,65.102381041112));
#140018=CARTESIAN_POINT('Ctrl Pts',(105.443996797269,13.37690857839,65.04244756226));
#140019=CARTESIAN_POINT('Ctrl Pts',(105.079332320269,13.43868444028,64.971563614758));
#140020=CARTESIAN_POINT('Ctrl Pts',(104.683229864969,13.50389802402,64.89456871282));
#140021=CARTESIAN_POINT('Ctrl Pts',(104.252687713469,13.57265912066,64.810879378689));
#140022=CARTESIAN_POINT('Ctrl Pts',(103.784473491969,13.64503600057,64.719867299405));
#140023=CARTESIAN_POINT('Ctrl Pts',(103.275306754669,13.7209315102,64.6208948177041));
#140024=CARTESIAN_POINT('Ctrl Pts',(102.721832206769,13.80015132265,64.513309727095));
#140025=CARTESIAN_POINT('Ctrl Pts',(102.120707706969,13.88237030275,64.3964623779141));
#140026=CARTESIAN_POINT('Ctrl Pts',(101.468529313469,13.96715464695,64.26969110755));
#140027=CARTESIAN_POINT('Ctrl Pts',(100.761166032169,14.05403942194,64.132192928096));
#140028=CARTESIAN_POINT('Ctrl Pts',(99.9935121174691,14.14252252124,63.9829753782081));
#140029=CARTESIAN_POINT('Ctrl Pts',(99.2912068414691,14.21787488508,63.8464603803061));
#140030=CARTESIAN_POINT('Ctrl Pts',(98.8440628998692,14.26295066722,63.759543968979));
#140031=CARTESIAN_POINT('Ctrl Pts',(98.6743066545691,14.2796529219,63.726546532871));
#140032=CARTESIAN_POINT('Ctrl Pts',(105.677598220969,11.68990176436,65.423193389316));
#140033=CARTESIAN_POINT('Ctrl Pts',(105.603824591269,11.70314306676,65.408853176808));
#140034=CARTESIAN_POINT('Ctrl Pts',(105.420605380269,11.73573317384,65.373238792213));
#140035=CARTESIAN_POINT('Ctrl Pts',(105.118449004669,11.78831012897,65.314505249415));
#140036=CARTESIAN_POINT('Ctrl Pts',(104.760765985569,11.84890363658,65.244978366641));
#140037=CARTESIAN_POINT('Ctrl Pts',(104.371922642669,11.91292257259,65.169394500257));
#140038=CARTESIAN_POINT('Ctrl Pts',(103.948862216169,11.98048909485,65.087159473402));
#140039=CARTESIAN_POINT('Ctrl Pts',(103.488634081469,12.05163160054,64.997699739869));
#140040=CARTESIAN_POINT('Ctrl Pts',(102.988082222469,12.12624308094,64.90040182923));
#140041=CARTESIAN_POINT('Ctrl Pts',(102.443877051669,12.20413632354,64.79461853202));
#140042=CARTESIAN_POINT('Ctrl Pts',(101.852688662669,12.28499654291,64.679702576745));
#140043=CARTESIAN_POINT('Ctrl Pts',(101.211090034869,12.36840589771,64.554987814772));
#140044=CARTESIAN_POINT('Ctrl Pts',(100.514934437469,12.45391456276,64.419668199267));
#140045=CARTESIAN_POINT('Ctrl Pts',(99.7591238753691,12.54103318314,64.272752775408));
#140046=CARTESIAN_POINT('Ctrl Pts',(99.0673497588691,12.61525625766,64.138284837753));
#140047=CARTESIAN_POINT('Ctrl Pts',(98.6267591070691,12.6596715379,64.052642263281));
#140048=CARTESIAN_POINT('Ctrl Pts',(98.4594704271691,12.67613101083,64.0201244757));
#140049=CARTESIAN_POINT('',(98.4192401217934,14.401804164717,65.9071352125797));
#140050=CARTESIAN_POINT('Ctrl Pts',(105.406733283589,13.3452126550092,67.5262279087238));
#140051=CARTESIAN_POINT('Ctrl Pts',(105.381157881525,13.3502102353128,67.5203514165497));
#140052=CARTESIAN_POINT('Ctrl Pts',(105.355581691314,13.3551935844434,67.5144734853879));
#140053=CARTESIAN_POINT('Ctrl Pts',(105.330004713402,13.3601628548922,67.5085941118163));
#140054=CARTESIAN_POINT('Ctrl Pts',(105.219236633267,13.3816836361654,67.4831318806979));
#140055=CARTESIAN_POINT('Ctrl Pts',(105.108453784641,13.4029403629768,67.4576425972809));
#140056=CARTESIAN_POINT('Ctrl Pts',(104.997656804334,13.4239440458079,67.4321261008341));
#140057=CARTESIAN_POINT('Ctrl Pts',(104.8775148326,13.4467192501681,67.4044574569204));
#140058=CARTESIAN_POINT('Ctrl Pts',(104.75735624808,13.4691969250606,67.3767568164943));
#140059=CARTESIAN_POINT('Ctrl Pts',(104.637180377502,13.4913896737591,67.3490236875475));
#140060=CARTESIAN_POINT('Ctrl Pts',(104.506635316763,13.5154972896464,67.3188976482232));
#140061=CARTESIAN_POINT('Ctrl Pts',(104.376069842465,13.5392686921611,67.2887332689063));
#140062=CARTESIAN_POINT('Ctrl Pts',(104.245490553519,13.5627177176572,67.2585313722496));
#140063=CARTESIAN_POINT('Ctrl Pts',(104.199920013792,13.570901134465,67.2479912878111));
#140064=CARTESIAN_POINT('Ctrl Pts',(104.15434779278,13.5790452879071,67.23744663432));
#140065=CARTESIAN_POINT('Ctrl Pts',(104.108773106829,13.587150789758,67.2268972399986));
#140066=CARTESIAN_POINT('Ctrl Pts',(104.012396744216,13.604291418799,67.2045885343815));
#140067=CARTESIAN_POINT('Ctrl Pts',(103.916009401996,13.6212591286287,67.1822587779171));
#140068=CARTESIAN_POINT('Ctrl Pts',(103.819603561869,13.6380596778537,67.1599064253125));
#140069=CARTESIAN_POINT('Ctrl Pts',(103.69951747087,13.6589869606865,67.1320636447776));
#140070=CARTESIAN_POINT('Ctrl Pts',(103.579402664645,13.6796548805289,67.1041858011181));
#140071=CARTESIAN_POINT('Ctrl Pts',(103.459256116394,13.7000647957269,67.0762721529889));
#140072=CARTESIAN_POINT('Ctrl Pts',(103.424986105314,13.7058864196534,67.0683102011509));
#140073=CARTESIAN_POINT('Ctrl Pts',(103.3907135111,13.7116870525938,67.0603453362345));
#140074=CARTESIAN_POINT('Ctrl Pts',(103.356438263105,13.7174667259815,67.0523775410846));
#140075=CARTESIAN_POINT('Ctrl Pts',(103.282396499432,13.7299520393233,67.035165423303));
#140076=CARTESIAN_POINT('Ctrl Pts',(103.208342351437,13.7423395448488,67.0179396313692));
#140077=CARTESIAN_POINT('Ctrl Pts',(103.134276238954,13.7546294882771,67.0007002135295));
#140078=CARTESIAN_POINT('Ctrl Pts',(103.080099922966,13.7636190765831,66.9880902881936));
#140079=CARTESIAN_POINT('Ctrl Pts',(103.025917145159,13.7725564742551,66.9754730625563));
#140080=CARTESIAN_POINT('Ctrl Pts',(102.971728141044,13.7814417670877,66.9628485678601));
#140081=CARTESIAN_POINT('Ctrl Pts',(102.944633638987,13.785884413504,66.956536320512));
#140082=CARTESIAN_POINT('Ctrl Pts',(102.917537580353,13.790314033716,66.9502222559043));
#140083=CARTESIAN_POINT('Ctrl Pts',(102.890439979525,13.7947306404591,66.9439063755002));
#140084=CARTESIAN_POINT('Ctrl Pts',(102.877853347631,13.7967821210921,66.9409726965283));
#140085=CARTESIAN_POINT('Ctrl Pts',(102.865266383003,13.798830794026,66.9380386257926));
#140086=CARTESIAN_POINT('Ctrl Pts',(102.852679087662,13.8008766604567,66.9351041635364));
#140087=CARTESIAN_POINT('Ctrl Pts',(102.851716868426,13.801033054025,66.934879842429));
#140088=CARTESIAN_POINT('Ctrl Pts',(102.850754647258,13.8011894311932,66.9346555190337));
#140089=CARTESIAN_POINT('Ctrl Pts',(102.849792424158,13.8013457919615,66.9344311933506));
#140090=CARTESIAN_POINT('Ctrl Pts',(102.836242855166,13.8035475900876,66.9312723455542));
#140091=CARTESIAN_POINT('Ctrl Pts',(102.821186091383,13.8059902555839,66.9277616759329));
#140092=CARTESIAN_POINT('Ctrl Pts',(102.809142570649,13.8079414318969,66.9249532893378));
#140093=CARTESIAN_POINT('Ctrl Pts',(102.707658542477,13.8243829058051,66.9012885827612));
#140094=CARTESIAN_POINT('Ctrl Pts',(102.590169504002,13.8431985272868,66.8739607615462));
#140095=CARTESIAN_POINT('Ctrl Pts',(102.456651461361,13.8641900914516,66.84295154119));
#140096=CARTESIAN_POINT('Ctrl Pts',(102.40815704942,13.8718143311405,66.8316888393396));
#140097=CARTESIAN_POINT('Ctrl Pts',(102.357548086328,13.8797251196032,66.8199404576736));
#140098=CARTESIAN_POINT('Ctrl Pts',(102.304823305587,13.8879112722829,66.807705396231));
#140099=CARTESIAN_POINT('Ctrl Pts',(102.156756066627,13.9109004816824,66.7733456181368));
#140100=CARTESIAN_POINT('Ctrl Pts',(101.992002262485,13.9360651677371,66.7351478329039));
#140101=CARTESIAN_POINT('Ctrl Pts',(101.810533783638,13.9631224600473,66.693087689397));
#140102=CARTESIAN_POINT('Ctrl Pts',(101.777387409099,13.9680646469805,66.6854051360481));
#140103=CARTESIAN_POINT('Ctrl Pts',(101.743683378144,13.973069837667,66.6775937132222));
#140104=CARTESIAN_POINT('Ctrl Pts',(101.709421523332,13.978136122441,66.6696532620346));
#140105=CARTESIAN_POINT('Ctrl Pts',(101.658173465491,13.9857141492748,66.6577761262525));
#140106=CARTESIAN_POINT('Ctrl Pts',(101.605677362654,13.993428876382,66.645610310142));
#140107=CARTESIAN_POINT('Ctrl Pts',(101.551932634488,14.0012737256221,66.633155264118));
#140108=CARTESIAN_POINT('Ctrl Pts',(101.460383484212,14.0146366973312,66.6119392505836));
#140109=CARTESIAN_POINT('Ctrl Pts',(101.365211319469,14.0283773475413,66.5898840144221));
#140110=CARTESIAN_POINT('Ctrl Pts',(101.266413361469,14.0424614193033,66.5669867527179));
#140111=CARTESIAN_POINT('Ctrl Pts',(101.217014382469,14.0495034551843,66.5555381218657));
#140112=CARTESIAN_POINT('Ctrl Pts',(101.166708953445,14.0566313162386,66.5438789734973));
#140113=CARTESIAN_POINT('Ctrl Pts',(101.115496747552,14.0638405167275,66.5320089592876));
#140114=CARTESIAN_POINT('Ctrl Pts',(101.098208266896,14.0662742358189,66.5280018186564));
#140115=CARTESIAN_POINT('Ctrl Pts',(101.080816446376,14.068717223697,66.5239706465975));
#140116=CARTESIAN_POINT('Ctrl Pts',(101.063321273766,14.0711693046102,66.5199154291647));
#140117=CARTESIAN_POINT('Ctrl Pts',(101.054904210371,14.0723490197782,66.5179644325686));
#140118=CARTESIAN_POINT('Ctrl Pts',(101.046463224621,14.0735308396377,66.5160078703168));
#140119=CARTESIAN_POINT('Ctrl Pts',(101.037998315012,14.0747147445836,66.5140457408203));
#140120=CARTESIAN_POINT('Ctrl Pts',(101.011938782694,14.0783594390487,66.5080052537521));
#140121=CARTESIAN_POINT('Ctrl Pts',(100.987109945946,14.0818214043664,66.5022498544524));
#140122=CARTESIAN_POINT('Ctrl Pts',(100.959139465562,14.0857075368092,66.4957659427328));
#140123=CARTESIAN_POINT('Ctrl Pts',(100.757973610972,14.1136569013962,66.4491331490066));
#140124=CARTESIAN_POINT('Ctrl Pts',(100.559239103292,14.1405560928714,66.4030589659381));
#140125=CARTESIAN_POINT('Ctrl Pts',(100.362947071848,14.1664684645508,66.3575511814201));
#140126=CARTESIAN_POINT('Ctrl Pts',(100.105330190568,14.200476286109,66.2978260186857));
#140127=CARTESIAN_POINT('Ctrl Pts',(99.851920383257,14.2327846518942,66.239076482115));
#140128=CARTESIAN_POINT('Ctrl Pts',(99.6027376068943,14.2635287439544,66.1813184830871));
#140129=CARTESIAN_POINT('Ctrl Pts',(99.321969064362,14.298169877845,66.1162392290418));
#140130=CARTESIAN_POINT('Ctrl Pts',(99.0465670949617,14.3308252092359,66.0524188394242));
#140131=CARTESIAN_POINT('Ctrl Pts',(98.7765544539798,14.3616741416806,65.989877742702));
#140132=CARTESIAN_POINT('Ctrl Pts',(98.6563816132559,14.3754038834872,65.9620429671605));
#140133=CARTESIAN_POINT('Ctrl Pts',(98.5372762547796,14.3887756405978,65.9344615703069));
#140134=CARTESIAN_POINT('Ctrl Pts',(98.4192401229391,14.4018041902007,65.9071352198517));
#140135=CARTESIAN_POINT('Origin',(98.3551330948655,12.9603930090967,65.4969839076243));
#140136=CARTESIAN_POINT('Ctrl Pts',(98.6918699825692,14.27197610448,66.217974461185));
#140137=CARTESIAN_POINT('Ctrl Pts',(98.4405864664691,14.28636537759,66.202563237184));
#140138=CARTESIAN_POINT('Ctrl Pts',(97.8913074767691,14.33180917892,66.112649421504));
#140139=CARTESIAN_POINT('Ctrl Pts',(97.0444533364691,14.44268121769,65.764243077902));
#140140=CARTESIAN_POINT('Ctrl Pts',(96.2125088153692,14.58833219957,65.116820696336));
#140141=CARTESIAN_POINT('Ctrl Pts',(95.5548624757691,14.72994024583,64.167499731003));
#140142=CARTESIAN_POINT('Ctrl Pts',(95.218166978169,14.82374422835,63.013795844258));
#140143=CARTESIAN_POINT('Ctrl Pts',(95.2531311970691,14.84218773752,62.15671974562));
#140144=CARTESIAN_POINT('Ctrl Pts',(95.348322967069,14.83944476018,61.72939797364));
#140145=CARTESIAN_POINT('Ctrl Pts',(95.3600036087691,14.8389630281,61.68154891083));
#140146=CARTESIAN_POINT('Ctrl Pts',(98.8538498000691,14.9154835018,64.9403367841401));
#140147=CARTESIAN_POINT('Ctrl Pts',(98.7129574471692,14.92892963799,64.938434414967));
#140148=CARTESIAN_POINT('Ctrl Pts',(98.3961279961691,14.97159179509,64.9087219556159));
#140149=CARTESIAN_POINT('Ctrl Pts',(97.8612535104691,15.07891262045,64.741238167691));
#140150=CARTESIAN_POINT('Ctrl Pts',(97.2821719387691,15.22467284488,64.362639344877));
#140151=CARTESIAN_POINT('Ctrl Pts',(96.7867641037691,15.37029300066,63.735122492223));
#140152=CARTESIAN_POINT('Ctrl Pts',(96.5173669447691,15.46821211358,62.92168774703));
#140153=CARTESIAN_POINT('Ctrl Pts',(96.536945970469,15.48743521164,62.30909927009));
#140154=CARTESIAN_POINT('Ctrl Pts',(96.6048510481691,15.48457264358,62.0084034354399));
#140155=CARTESIAN_POINT('Ctrl Pts',(96.6132000082691,15.48406241972,61.97480249097));
#140156=CARTESIAN_POINT('Ctrl Pts',(98.8945644152691,14.04213367577,63.796526009201));
#140157=CARTESIAN_POINT('Ctrl Pts',(98.8227012415692,14.0568598104,63.796087997308));
#140158=CARTESIAN_POINT('Ctrl Pts',(98.6604006711691,14.10329713546,63.782568224124));
#140159=CARTESIAN_POINT('Ctrl Pts',(98.3828403562691,14.21543756603,63.699343015961));
#140160=CARTESIAN_POINT('Ctrl Pts',(98.0785794391691,14.36104952961,63.505004006583));
#140161=CARTESIAN_POINT('Ctrl Pts',(97.8158867698691,14.50122456514,63.177410967091));
#140162=CARTESIAN_POINT('Ctrl Pts',(97.6721106794691,14.59355874085,62.7493551232801));
#140163=CARTESIAN_POINT('Ctrl Pts',(97.6820951225691,14.61172380317,62.42647002956));
#140164=CARTESIAN_POINT('Ctrl Pts',(97.7178785373692,14.60902354021,62.26827135895));
#140165=CARTESIAN_POINT('Ctrl Pts',(97.7222791533691,14.60855198458,62.25059797219));
#140166=CARTESIAN_POINT('Ctrl Pts',(98.768177115269,12.63514813157,64.0742499004729));
#140167=CARTESIAN_POINT('Ctrl Pts',(98.6462677492691,12.65193637148,64.061583167723));
#140168=CARTESIAN_POINT('Ctrl Pts',(98.3866060319691,12.70445557414,64.002017605271));
#140169=CARTESIAN_POINT('Ctrl Pts',(98.0220088521691,12.82436049343,63.8115282798));
#140170=CARTESIAN_POINT('Ctrl Pts',(97.705131857869,12.96973360554,63.509444739474));
#140171=CARTESIAN_POINT('Ctrl Pts',(97.4836391437691,13.10113643407,63.122239518025));
#140172=CARTESIAN_POINT('Ctrl Pts',(97.3823820385691,13.18447315457,62.6908108836));
#140173=CARTESIAN_POINT('Ctrl Pts',(97.3993641377692,13.20093369833,62.37669544903));
#140174=CARTESIAN_POINT('Ctrl Pts',(97.4343536442692,13.19849491242,62.21644116502));
#140175=CARTESIAN_POINT('Ctrl Pts',(97.4386343186691,13.19808565216,62.19844345297));
#140176=CARTESIAN_POINT('',(97.4407949555856,13.49843642512,62.3530207360974));
#140177=CARTESIAN_POINT('Ctrl Pts',(98.6413355057991,12.96039230927,64.024540977121));
#140178=CARTESIAN_POINT('Ctrl Pts',(98.605473984333,12.9675617061125,64.0175707852277));
#140179=CARTESIAN_POINT('Ctrl Pts',(98.5683962081428,12.9757376510516,64.0090060419383));
#140180=CARTESIAN_POINT('Ctrl Pts',(98.5302868961479,12.9849201440874,63.9985400265442));
#140181=CARTESIAN_POINT('Ctrl Pts',(98.4921775841531,12.9941026371232,63.98807401115));
#140182=CARTESIAN_POINT('Ctrl Pts',(98.45303623735,13.0042916782556,63.9757060755926));
#140183=CARTESIAN_POINT('Ctrl Pts',(98.4131060346052,13.0154872674846,63.9611280617728));
#140184=CARTESIAN_POINT('Ctrl Pts',(98.376063601498,13.025873186829,63.9476043362559));
#140185=CARTESIAN_POINT('Ctrl Pts',(98.3383426214638,13.0371253307708,63.9321781167114));
#140186=CARTESIAN_POINT('Ctrl Pts',(98.3001875346592,13.0492436993101,63.914610488346));
#140187=CARTESIAN_POINT('Ctrl Pts',(98.297213024295,13.0501884282004,63.9132409437577));
#140188=CARTESIAN_POINT('Ctrl Pts',(98.2942359013327,13.0511384215843,63.9118583908725));
#140189=CARTESIAN_POINT('Ctrl Pts',(98.2912562947423,13.0520936794616,63.9104627199178));
#140190=CARTESIAN_POINT('Ctrl Pts',(98.2730008826755,13.05794634009,63.9019117425944));
#140191=CARTESIAN_POINT('Ctrl Pts',(98.254435686774,13.0640722403333,63.8927621878895));
#140192=CARTESIAN_POINT('Ctrl Pts',(98.2358838421152,13.070370855523,63.8831220800602));
#140193=CARTESIAN_POINT('Ctrl Pts',(98.2175389480234,13.0765992080511,63.8735895100968));
#140194=CARTESIAN_POINT('Ctrl Pts',(98.1992074642894,13.0829964436594,63.8635773538434));
#140195=CARTESIAN_POINT('Ctrl Pts',(98.181180023402,13.0894653644266,63.8532366540782));
#140196=CARTESIAN_POINT('Ctrl Pts',(98.1762937331504,13.0912187483196,63.8504338347112));
#140197=CARTESIAN_POINT('Ctrl Pts',(98.1714296390673,13.0929773986825,63.8476071390264));
#140198=CARTESIAN_POINT('Ctrl Pts',(98.166593201586,13.0947393800183,63.8447601481387));
#140199=CARTESIAN_POINT('Ctrl Pts',(98.1148083545813,13.1136053188947,63.8142767627726));
#140200=CARTESIAN_POINT('Ctrl Pts',(98.0648576610132,13.1327059816041,63.7806779492109));
#140201=CARTESIAN_POINT('Ctrl Pts',(98.0171010756302,13.1520413681468,63.7442058273393));
#140202=CARTESIAN_POINT('Ctrl Pts',(97.9693425234032,13.1713775510129,63.7077322033716));
#140203=CARTESIAN_POINT('Ctrl Pts',(97.9237785922256,13.1909484770466,63.6683852876198));
#140204=CARTESIAN_POINT('Ctrl Pts',(97.8807376519285,13.210754146248,63.6264486452522));
#140205=CARTESIAN_POINT('Ctrl Pts',(97.8652768701684,13.2178685616632,63.6113845395212));
#140206=CARTESIAN_POINT('Ctrl Pts',(97.8501413162752,13.2250132665962,63.5959866436732));
#140207=CARTESIAN_POINT('Ctrl Pts',(97.8353450915221,13.232188261047,63.5802693034007));
#140208=CARTESIAN_POINT('Ctrl Pts',(97.8191490387139,13.2400420609832,63.5630649909962));
#140209=CARTESIAN_POINT('Ctrl Pts',(97.8033595729907,13.2479321527512,63.5454779222972));
#140210=CARTESIAN_POINT('Ctrl Pts',(97.7879943189786,13.2558585363509,63.5275277284681));
#140211=CARTESIAN_POINT('Ctrl Pts',(97.7807787322864,13.2595807987993,63.5190982433705));
#140212=CARTESIAN_POINT('Ctrl Pts',(97.7739289245749,13.2631676096328,63.5109134644787));
#140213=CARTESIAN_POINT('Ctrl Pts',(97.7670570401342,13.266821070005,63.5025229127333));
#140214=CARTESIAN_POINT('Ctrl Pts',(97.7603420894826,13.2703910960028,63.4943239767068));
#140215=CARTESIAN_POINT('Ctrl Pts',(97.7536059018193,13.2740247621372,63.485928455883));
#140216=CARTESIAN_POINT('Ctrl Pts',(97.74652470328,13.2779106371597,63.476885421999));
#140217=CARTESIAN_POINT('Ctrl Pts',(97.7454211026964,13.2785162484723,63.475476070543));
#140218=CARTESIAN_POINT('Ctrl Pts',(97.7443092042379,13.279127985696,63.4740509297644));
#140219=CARTESIAN_POINT('Ctrl Pts',(97.7431878773281,13.279746562645,63.4726082223633));
#140220=CARTESIAN_POINT('Ctrl Pts',(97.7067057287732,13.2998718409635,63.4256700232804));
#140221=CARTESIAN_POINT('Ctrl Pts',(97.6731726327694,13.3186120473381,63.3767606726784));
#140222=CARTESIAN_POINT('Ctrl Pts',(97.6427496914699,13.3359671817688,63.3262726338115));
#140223=CARTESIAN_POINT('Ctrl Pts',(97.6121486921119,13.3534238915703,63.275489100762));
#140224=CARTESIAN_POINT('Ctrl Pts',(97.5846943551583,13.3694792690058,63.2231087895806));
#140225=CARTESIAN_POINT('Ctrl Pts',(97.5604980861838,13.3841333140753,63.1695378143773));
#140226=CARTESIAN_POINT('Ctrl Pts',(97.5360840546123,13.3989192432347,63.1154847088631));
#140227=CARTESIAN_POINT('Ctrl Pts',(97.5149869650521,13.4122785029845,63.0602198511968));
#140228=CARTESIAN_POINT('Ctrl Pts',(97.497268174044,13.4242110933247,63.0041605469673));
#140229=CARTESIAN_POINT('Ctrl Pts',(97.4899793158144,13.4291197216427,62.9810998132641));
#140230=CARTESIAN_POINT('Ctrl Pts',(97.4832615175028,13.4337869294389,62.9579046074509));
#140231=CARTESIAN_POINT('Ctrl Pts',(97.4771165116137,13.4382127167133,62.9346037225659));
#140232=CARTESIAN_POINT('Ctrl Pts',(97.4619819936829,13.4491129758948,62.8772160379222));
#140233=CARTESIAN_POINT('Ctrl Pts',(97.4503255590828,13.4585488113325,62.8191883236414));
#140234=CARTESIAN_POINT('Ctrl Pts',(97.4421362402369,13.4665202230264,62.7609433102217));
#140235=CARTESIAN_POINT('Ctrl Pts',(97.4338962979358,13.4745409111509,62.7023382468543));
#140236=CARTESIAN_POINT('Ctrl Pts',(97.4291662775862,13.4810790144791,62.6435135913618));
#140237=CARTESIAN_POINT('Ctrl Pts',(97.4278843900862,13.4861345330108,62.5848843420891));
#140238=CARTESIAN_POINT('Ctrl Pts',(97.4265906202032,13.4912369133828,62.5257116323384));
#140239=CARTESIAN_POINT('Ctrl Pts',(97.4288089871018,13.4948290961008,62.4667383536048));
#140240=CARTESIAN_POINT('Ctrl Pts',(97.4344276219277,13.4969110811646,62.408369305678));
#140241=CARTESIAN_POINT('Ctrl Pts',(97.4362098135436,13.4975714722454,62.3898550524705));
#140242=CARTESIAN_POINT('Ctrl Pts',(97.4383337629024,13.4980799202305,62.3714014050411));
#140243=CARTESIAN_POINT('Ctrl Pts',(97.4407949555856,13.49843642512,62.3530207360974));
#140244=CARTESIAN_POINT('',(95.9574505237762,14.9983370670242,62.1685354760649));
#140245=CARTESIAN_POINT('Ctrl Pts',(98.4192401195208,14.4018041137337,65.9071351980887));
#140246=CARTESIAN_POINT('Ctrl Pts',(98.3548599127743,14.4089099341238,65.8922317214608));
#140247=CARTESIAN_POINT('Ctrl Pts',(98.2858505689251,14.417160748693,65.873809883599));
#140248=CARTESIAN_POINT('Ctrl Pts',(98.212727410607,14.4267274727341,65.8508614541008));
#140249=CARTESIAN_POINT('Ctrl Pts',(98.1455872512908,14.435511439278,65.8297906846208));
#140250=CARTESIAN_POINT('Ctrl Pts',(98.0749795403419,14.4454051014527,65.8049036302979));
#140251=CARTESIAN_POINT('Ctrl Pts',(98.001322024238,14.4564991321363,65.7754036828193));
#140252=CARTESIAN_POINT('Ctrl Pts',(97.9947582500405,14.4574877442454,65.7727748812477));
#140253=CARTESIAN_POINT('Ctrl Pts',(97.9881702673191,14.458485857057,65.7701094381682));
#140254=CARTESIAN_POINT('Ctrl Pts',(97.9815583771808,14.4594935156246,65.767406783545));
#140255=CARTESIAN_POINT('Ctrl Pts',(97.9116352015369,14.4701498764441,65.7388252145884));
#140256=CARTESIAN_POINT('Ctrl Pts',(97.8390711057577,14.4818801472515,65.7060692153778));
#140257=CARTESIAN_POINT('Ctrl Pts',(97.7644638927116,14.4947164022248,65.6684025466324));
#140258=CARTESIAN_POINT('Ctrl Pts',(97.7528484664463,14.4967148493866,65.6625383091732));
#140259=CARTESIAN_POINT('Ctrl Pts',(97.7411835148542,14.4987400037317,65.6565550210306));
#140260=CARTESIAN_POINT('Ctrl Pts',(97.72947128728,14.5007918709519,65.6504498792864));
#140261=CARTESIAN_POINT('Ctrl Pts',(97.6860006840233,14.5084074936246,65.6277902961367));
#140262=CARTESIAN_POINT('Ctrl Pts',(97.6418829950394,14.5163917403531,65.6034511475642));
#140263=CARTESIAN_POINT('Ctrl Pts',(97.5972596749744,14.5247411162083,65.5772822763999));
#140264=CARTESIAN_POINT('Ctrl Pts',(97.5749480149419,14.5289158041359,65.5641978408177));
#140265=CARTESIAN_POINT('Ctrl Pts',(97.5525102327289,14.5331816709044,65.5506558940559));
#140266=CARTESIAN_POINT('Ctrl Pts',(97.529965780174,14.5375376166696,65.5366371873412));
#140267=CARTESIAN_POINT('Ctrl Pts',(97.5186935538966,14.5397155895522,65.5296278339839));
#140268=CARTESIAN_POINT('Ctrl Pts',(97.5073946597482,14.5419160749039,65.5224992888258));
#140269=CARTESIAN_POINT('Ctrl Pts',(97.4960716716008,14.5441388904471,65.5152491116246));
#140270=CARTESIAN_POINT('Ctrl Pts',(97.4847486834535,14.5463617059903,65.5079989344235));
#140271=CARTESIAN_POINT('Ctrl Pts',(97.4718880028697,14.5489087097035,65.4996291420303));
#140272=CARTESIAN_POINT('Ctrl Pts',(97.462033008452,14.5508741142754,65.4931312351855));
#140273=CARTESIAN_POINT('Ctrl Pts',(97.3831930531109,14.5665973508509,65.4411479804269));
#140274=CARTESIAN_POINT('Ctrl Pts',(97.3062831928474,14.5826460682807,65.3857544981588));
#140275=CARTESIAN_POINT('Ctrl Pts',(97.2315642963389,14.5988726037447,65.3270122750896));
#140276=CARTESIAN_POINT('Ctrl Pts',(97.1942048480847,14.6069858714767,65.297641163555));
#140277=CARTESIAN_POINT('Ctrl Pts',(97.1573958789567,14.6151423536242,65.267437499745));
#140278=CARTESIAN_POINT('Ctrl Pts',(97.1211760870691,14.623321403787,65.2364175858901));
#140279=CARTESIAN_POINT('Ctrl Pts',(97.1030661911253,14.6274109288684,65.2209076289627));
#140280=CARTESIAN_POINT('Ctrl Pts',(97.0851035896286,14.6315060984733,65.2051936103958));
#140281=CARTESIAN_POINT('Ctrl Pts',(97.0672931597619,14.6356043747053,65.1892774460997));
#140282=CARTESIAN_POINT('Ctrl Pts',(97.0583879448286,14.6376535128213,65.1813193639516));
#140283=CARTESIAN_POINT('Ctrl Pts',(97.0495207728092,14.6397034277684,65.173310745412));
#140284=CARTESIAN_POINT('Ctrl Pts',(97.0406922544568,14.6417538041061,65.1652518268546));
#140285=CARTESIAN_POINT('Ctrl Pts',(97.0329673008984,14.6435478834017,65.1582002731169));
#140286=CARTESIAN_POINT('Ctrl Pts',(97.0252719415541,14.6453423159601,65.151110208431));
#140287=CARTESIAN_POINT('Ctrl Pts',(97.0176065863376,14.6471368914392,65.1439817888684));
#140288=CARTESIAN_POINT('Ctrl Pts',(97.0165115355924,14.6473932593647,65.1429634432166));
#140289=CARTESIAN_POINT('Ctrl Pts',(97.0144528815075,14.6478756252705,65.1410452550338));
#140290=CARTESIAN_POINT('Ctrl Pts',(97.0143232723051,14.6479060033694,65.1409244040454));
#140291=CARTESIAN_POINT('Ctrl Pts',(97.0119524859554,14.6484616736518,65.1387138212454));
#140292=CARTESIAN_POINT('Ctrl Pts',(97.0043001237704,14.6502753896007,65.1314987778178));
#140293=CARTESIAN_POINT('Ctrl Pts',(96.991581820615,14.6533604270402,65.1190391432065));
#140294=CARTESIAN_POINT('Ctrl Pts',(96.982050505149,14.6556724072393,65.1097016784032));
#140295=CARTESIAN_POINT('Ctrl Pts',(96.9696745896939,14.6586976140359,65.0974183794051));
#140296=CARTESIAN_POINT('Ctrl Pts',(96.9545534271432,14.6624254448703,65.0820823431156));
#140297=CARTESIAN_POINT('Ctrl Pts',(96.9369042316537,14.6667765134425,65.0641823502017));
#140298=CARTESIAN_POINT('Ctrl Pts',(96.9155414545847,14.6720913792892,65.0420933193525));
#140299=CARTESIAN_POINT('Ctrl Pts',(96.8908164867911,14.6783548011537,65.015465716334));
#140300=CARTESIAN_POINT('Ctrl Pts',(96.8784540028943,14.6814865120859,65.0021519148247));
#140301=CARTESIAN_POINT('Ctrl Pts',(96.865253244134,14.6848551342965,64.9877016437808));
#140302=CARTESIAN_POINT('Ctrl Pts',(96.851272898472,14.6884568977787,64.9720607676581));
#140303=CARTESIAN_POINT('Ctrl Pts',(96.844282725641,14.6902577795197,64.9642403295968));
#140304=CARTESIAN_POINT('Ctrl Pts',(96.8370976548813,14.6921169087872,64.9561222326553));
#140305=CARTESIAN_POINT('Ctrl Pts',(96.8297262224199,14.6940336711822,64.9476989950849));
#140306=CARTESIAN_POINT('Ctrl Pts',(96.8260405061892,14.6949920523797,64.9434873762997));
#140307=CARTESIAN_POINT('Ctrl Pts',(96.8223081994494,14.6959648392636,64.9391994718284));
#140308=CARTESIAN_POINT('Ctrl Pts',(96.818530410879,14.6969519411706,64.9348343262526));
#140309=CARTESIAN_POINT('Ctrl Pts',(96.8147526223086,14.6979390430776,64.9304691806768));
#140310=CARTESIAN_POINT('Ctrl Pts',(96.8098803509342,14.6992159243711,64.9248006981191));
#140311=CARTESIAN_POINT('Ctrl Pts',(96.8070617302252,14.699956091772,64.9215061981443));
#140312=CARTESIAN_POINT('Ctrl Pts',(96.8032885852447,14.7009469164348,64.9170960176601));
#140313=CARTESIAN_POINT('Ctrl Pts',(96.7995557144585,14.7019290499594,64.9127106355594));
#140314=CARTESIAN_POINT('Ctrl Pts',(96.7958627355554,14.702902482579,64.9083506489919));
#140315=CARTESIAN_POINT('Ctrl Pts',(96.7502411896542,14.7149278696991,64.8544891641206));
#140316=CARTESIAN_POINT('Ctrl Pts',(96.7107031946376,14.7256243960024,64.8045047207743));
#140317=CARTESIAN_POINT('Ctrl Pts',(96.676558228223,14.7349808674531,64.7595146643301));
#140318=CARTESIAN_POINT('Ctrl Pts',(96.6473952891325,14.7429721538906,64.7210890217384));
#140319=CARTESIAN_POINT('Ctrl Pts',(96.6221675546253,14.7499867814444,64.6863063983579));
#140320=CARTESIAN_POINT('Ctrl Pts',(96.6004730779209,14.7560178220167,64.6558527121837));
#140321=CARTESIAN_POINT('Ctrl Pts',(96.5629238633939,14.7664564621993,64.6031428906529));
#140322=CARTESIAN_POINT('Ctrl Pts',(96.5242227079699,14.7772898571612,64.5464888620646));
#140323=CARTESIAN_POINT('Ctrl Pts',(96.4851640788121,14.7884057688328,64.4855046878037));
#140324=CARTESIAN_POINT('Ctrl Pts',(96.4484138417273,14.7988647224149,64.4281247205381));
#140325=CARTESIAN_POINT('Ctrl Pts',(96.4113473941561,14.8095737125234,64.366911150988));
#140326=CARTESIAN_POINT('Ctrl Pts',(96.3745927052218,14.8204105290804,64.3015517348863));
#140327=CARTESIAN_POINT('Ctrl Pts',(96.3481442829553,14.8282086280069,64.2545195469866));
#140328=CARTESIAN_POINT('Ctrl Pts',(96.3218566407735,14.8360723462582,64.2053407521427));
#140329=CARTESIAN_POINT('Ctrl Pts',(96.2959506744976,14.8439462867232,64.1539029936064));
#140330=CARTESIAN_POINT('Ctrl Pts',(96.2638834095475,14.8536929115896,64.0902316287224));
#140331=CARTESIAN_POINT('Ctrl Pts',(96.2324644575906,14.8634547627218,64.0230936187831));
#140332=CARTESIAN_POINT('Ctrl Pts',(96.2023566467437,14.8730978451295,63.9523310853555));
#140333=CARTESIAN_POINT('Ctrl Pts',(96.1854403500314,14.8785158824641,63.9125726313894));
#140334=CARTESIAN_POINT('Ctrl Pts',(96.1689371821935,14.8838961256817,63.8716702383139));
#140335=CARTESIAN_POINT('Ctrl Pts',(96.1529581626964,14.8892124571374,63.8295981632268));
#140336=CARTESIAN_POINT('Ctrl Pts',(96.1307488356699,14.8966016554485,63.771121954817));
#140337=CARTESIAN_POINT('Ctrl Pts',(96.1095562915821,14.9038653249061,63.7104017724764));
#140338=CARTESIAN_POINT('Ctrl Pts',(96.0897091813706,14.9109207031831,63.6474492675876));
#140339=CARTESIAN_POINT('Ctrl Pts',(96.0797856262649,14.9144483923216,63.6159730151432));
#140340=CARTESIAN_POINT('Ctrl Pts',(96.0701989423633,14.9179239040919,63.5839392466392));
#140341=CARTESIAN_POINT('Ctrl Pts',(96.0609934095968,14.921336373574,63.5513530352228));
#140342=CARTESIAN_POINT('Ctrl Pts',(96.053607930715,14.9240741533347,63.5252095427864));
#140343=CARTESIAN_POINT('Ctrl Pts',(96.0462305073155,14.9268664675079,63.4977564710501));
#140344=CARTESIAN_POINT('Ctrl Pts',(96.0394561086189,14.9294780313795,63.4712938920148));
#140345=CARTESIAN_POINT('Ctrl Pts',(96.0377866473881,14.9301216168592,63.46477253835));
#140346=CARTESIAN_POINT('Ctrl Pts',(96.0361538646799,14.9307544694931,63.4583113444831));
#140347=CARTESIAN_POINT('Ctrl Pts',(96.0345667776102,14.931373538865,63.4519447433593));
#140348=CARTESIAN_POINT('Ctrl Pts',(96.0131082811534,14.9397437777626,63.3658639666528));
#140349=CARTESIAN_POINT('Ctrl Pts',(95.9957427903507,14.9471044693013,63.2816295298594));
#140350=CARTESIAN_POINT('Ctrl Pts',(95.9818299032794,14.9535676953711,63.1995854857261));
#140351=CARTESIAN_POINT('Ctrl Pts',(95.9675042100614,14.9602226903695,63.1151071311908));
#140352=CARTESIAN_POINT('Ctrl Pts',(95.9568390643428,14.965926347952,63.0329510722339));
#140353=CARTESIAN_POINT('Ctrl Pts',(95.9491875207717,14.9708082268386,62.9534723392464));
#140354=CARTESIAN_POINT('Ctrl Pts',(95.942031555446,14.9753739142338,62.8791413167404));
#140355=CARTESIAN_POINT('Ctrl Pts',(95.9375121760969,14.9792210400244,62.8071517437967));
#140356=CARTESIAN_POINT('Ctrl Pts',(95.9351384484719,14.9824588177391,62.7377790576165));
#140357=CARTESIAN_POINT('Ctrl Pts',(95.9323603880237,14.9862481076789,62.6565896601325));
#140358=CARTESIAN_POINT('Ctrl Pts',(95.9323866516514,14.9892056743569,62.5789843422128));
#140359=CARTESIAN_POINT('Ctrl Pts',(95.9344117700746,14.9915124506985,62.5050586921308));
#140360=CARTESIAN_POINT('Ctrl Pts',(95.9365700339944,14.9939708907046,62.4262726510363));
#140361=CARTESIAN_POINT('Ctrl Pts',(95.9409989357065,14.9956903942518,62.3516658234036));
#140362=CARTESIAN_POINT('Ctrl Pts',(95.9467749196894,14.99686525085,62.281333677442));
#140363=CARTESIAN_POINT('Ctrl Pts',(95.9499705646574,14.9975152569073,62.2424214212794));
#140364=CARTESIAN_POINT('Ctrl Pts',(95.9535794175851,14.9979980947992,62.2048173203955));
#140365=CARTESIAN_POINT('Ctrl Pts',(95.9574505343397,14.99834334873,62.1685355389868));
#140366=CARTESIAN_POINT('Ctrl Pts',(95.9574504676803,14.9983112794787,62.1685352218286));
#140367=CARTESIAN_POINT('Ctrl Pts',(96.0005011109051,14.9981619617962,62.1743324282915));
#140368=CARTESIAN_POINT('Ctrl Pts',(96.0441829211307,14.9961208430062,62.180187222598));
#140369=CARTESIAN_POINT('Ctrl Pts',(96.0882590761874,14.992038585098,62.1860688983633));
#140370=CARTESIAN_POINT('Ctrl Pts',(96.1314805172245,14.9880354893368,62.1918365181106));
#140371=CARTESIAN_POINT('Ctrl Pts',(96.1750806514507,14.9820691038472,62.1976299162011));
#140372=CARTESIAN_POINT('Ctrl Pts',(96.2188022886828,14.9740352308408,62.2034157554569));
#140373=CARTESIAN_POINT('Ctrl Pts',(96.2620787520592,14.966083158756,62.2091426832782));
#140374=CARTESIAN_POINT('Ctrl Pts',(96.3054736560346,14.956105021506,62.2148621223634));
#140375=CARTESIAN_POINT('Ctrl Pts',(96.3487121925896,14.9440435852066,62.2205385368215));
#140376=CARTESIAN_POINT('Ctrl Pts',(96.3914593744506,14.9321192128278,62.2261504455607));
#140377=CARTESIAN_POINT('Ctrl Pts',(96.4340530118707,14.9181583406398,62.2317202050112));
#140378=CARTESIAN_POINT('Ctrl Pts',(96.4762123767249,14.9021542371481,62.2372116669386));
#140379=CARTESIAN_POINT('Ctrl Pts',(96.4929937416756,14.8957838683741,62.2393975211857));
#140380=CARTESIAN_POINT('Ctrl Pts',(96.5097061892548,14.889090334833,62.2415709577068));
#140381=CARTESIAN_POINT('Ctrl Pts',(96.526331738287,14.8820755052874,62.2437296705194));
#140382=CARTESIAN_POINT('Ctrl Pts',(96.5677011654777,14.8646204739027,62.2491012051589));
#140383=CARTESIAN_POINT('Ctrl Pts',(96.6085321883246,14.8451724086258,62.2543818537009));
#140384=CARTESIAN_POINT('Ctrl Pts',(96.6485498202056,14.8237961698842,62.2595354128814));
#140385=CARTESIAN_POINT('Ctrl Pts',(96.6887339095709,14.8023310144636,62.2647104088251));
#140386=CARTESIAN_POINT('Ctrl Pts',(96.7280970216981,14.7789217013327,62.2697571489435));
#140387=CARTESIAN_POINT('Ctrl Pts',(96.7663731273024,14.7536856636138,62.2746411252101));
#140388=CARTESIAN_POINT('Ctrl Pts',(96.8042656201698,14.7287025477986,62.2794761530409));
#140389=CARTESIAN_POINT('Ctrl Pts',(96.8410921005653,14.7019295529653,62.2841515753469));
#140390=CARTESIAN_POINT('Ctrl Pts',(96.8766177138151,14.6735272668377,62.2886374649293));
#140391=CARTESIAN_POINT('Ctrl Pts',(96.9121727657077,14.6451014448811,62.2931270717874));
#140392=CARTESIAN_POINT('Ctrl Pts',(96.9464241864178,14.6150441406749,62.2974267552004));
#140393=CARTESIAN_POINT('Ctrl Pts',(96.9791697210766,14.5835564888875,62.3015113349985));
#140394=CARTESIAN_POINT('Ctrl Pts',(97.0120092150943,14.5519784870843,62.3056076350053));
#140395=CARTESIAN_POINT('Ctrl Pts',(97.043333705804,14.5189625652565,62.3094875393312));
#140396=CARTESIAN_POINT('Ctrl Pts',(97.0729806653625,14.484743219441,62.3131315012315));
#140397=CARTESIAN_POINT('Ctrl Pts',(97.1030081825707,14.4500846233949,62.316822238167));
#140398=CARTESIAN_POINT('Ctrl Pts',(97.1313144664109,14.4141922439907,62.3202708953771));
#140399=CARTESIAN_POINT('Ctrl Pts',(97.1577795236448,14.3773316661675,62.3234639139798));
#140400=CARTESIAN_POINT('Ctrl Pts',(97.1843342351965,14.3403462176542,62.3266677494081));
#140401=CARTESIAN_POINT('Ctrl Pts',(97.2090351572593,14.3023868126045,62.3296142099809));
#140402=CARTESIAN_POINT('Ctrl Pts',(97.2318130930835,14.2637318774777,62.3322966586155));
#140403=CARTESIAN_POINT('Ctrl Pts',(97.2549393663752,14.2244858017705,62.3350201292886));
#140404=CARTESIAN_POINT('Ctrl Pts',(97.276083437397,14.1845235730453,62.3374714655972));
#140405=CARTESIAN_POINT('Ctrl Pts',(97.2952267179217,14.1441346156089,62.3396509096967));
#140406=CARTESIAN_POINT('Ctrl Pts',(97.3136023357209,14.1053652916048,62.3417429561323));
#140407=CARTESIAN_POINT('Ctrl Pts',(97.3301350398945,14.0662033083041,62.3435845683744));
#140408=CARTESIAN_POINT('Ctrl Pts',(97.3448517592675,14.0268930901495,62.3451816578265));
#140409=CARTESIAN_POINT('Ctrl Pts',(97.3605291573088,13.9850167778082,62.3468830021556));
#140410=CARTESIAN_POINT('Ctrl Pts',(97.3741457445416,13.9429731857398,62.3483068521509));
#140411=CARTESIAN_POINT('Ctrl Pts',(97.3857801232169,13.9010337028441,62.3494664591817));
#140412=CARTESIAN_POINT('Ctrl Pts',(97.3977004858437,13.8580633080815,62.350654570442));
#140413=CARTESIAN_POINT('Ctrl Pts',(97.4075405333139,13.8152027833417,62.3515653653733));
#140414=CARTESIAN_POINT('Ctrl Pts',(97.415426538954,13.7727089150853,62.3522183319137));
#140415=CARTESIAN_POINT('Ctrl Pts',(97.423434730561,13.7295566457809,62.352881415534));
#140416=CARTESIAN_POINT('Ctrl Pts',(97.4294285686737,13.6867828301511,62.3532787166675));
#140417=CARTESIAN_POINT('Ctrl Pts',(97.4335730705108,13.6446135218585,62.3534346198244));
#140418=CARTESIAN_POINT('Ctrl Pts',(97.4378188709953,13.6014135242178,62.3535943335186));
#140419=CARTESIAN_POINT('Ctrl Pts',(97.4401245654739,13.5588481660462,62.3535008046023));
#140420=CARTESIAN_POINT('Ctrl Pts',(97.4406905904248,13.5171113558476,62.3531828726247));
#140421=CARTESIAN_POINT('Ctrl Pts',(97.4407752648613,13.510867742592,62.3531353116276));
#140422=CARTESIAN_POINT('Ctrl Pts',(97.4408210370043,13.5046425807729,62.3530827318652));
#140423=CARTESIAN_POINT('Ctrl Pts',(97.440828605087,13.4984364247508,62.3530252326599));
#140424=CARTESIAN_POINT('Ctrl Pts',(95.6383694486691,14.96466568086,62.13083612273));
#140425=CARTESIAN_POINT('Ctrl Pts',(95.6497349713691,14.96550769017,62.04287213666));
#140426=CARTESIAN_POINT('Ctrl Pts',(95.6643822846691,14.96457285862,61.95567204144));
#140427=CARTESIAN_POINT('Ctrl Pts',(95.6821735052692,14.96198967028,61.8696850735));
#140428=CARTESIAN_POINT('Ctrl Pts',(96.8005714632691,15.21737516854,62.287692685));
#140429=CARTESIAN_POINT('Ctrl Pts',(96.8092255620691,15.21825422082,62.21975234547));
#140430=CARTESIAN_POINT('Ctrl Pts',(96.8206378887691,15.21727770737,62.15269641207));
#140431=CARTESIAN_POINT('Ctrl Pts',(96.8346416864691,15.21458604043,62.08693395755));
#140432=CARTESIAN_POINT('Ctrl Pts',(97.6471925791692,14.37376668098,62.39128093599));
#140433=CARTESIAN_POINT('Ctrl Pts',(97.6521322186691,14.37452207443,62.35267039112));
#140434=CARTESIAN_POINT('Ctrl Pts',(97.6586006697691,14.37368470574,62.31451148597));
#140435=CARTESIAN_POINT('Ctrl Pts',(97.6665135970691,14.37135516796,62.2770259460699));
#140436=CARTESIAN_POINT('Ctrl Pts',(97.4109254415691,13.19841717584,62.34771705287));
#140437=CARTESIAN_POINT('Ctrl Pts',(97.414514065169,13.1990002828,62.32116035078));
#140438=CARTESIAN_POINT('Ctrl Pts',(97.4188104715692,13.19835677621,62.294461464));
#140439=CARTESIAN_POINT('Ctrl Pts',(97.4238493419691,13.19653177145,62.26767738332));
#140440=CARTESIAN_POINT('',(95.9754884183226,14.9956963974856,61.9308509078933));
#140441=CARTESIAN_POINT('',(97.4550857102592,13.496508878909,62.2658809045985));
#140442=CARTESIAN_POINT('Ctrl Pts',(95.9754884244307,14.9956951278022,61.9308509489964));
#140443=CARTESIAN_POINT('Ctrl Pts',(96.0191083210387,14.9961786137454,61.9393038707493));
#140444=CARTESIAN_POINT('Ctrl Pts',(96.0635504718247,14.9946955776386,61.9479826282064));
#140445=CARTESIAN_POINT('Ctrl Pts',(96.1085757343769,14.9910370652072,61.9568462597379));
#140446=CARTESIAN_POINT('Ctrl Pts',(96.1505747912088,14.9876244460949,61.9651141552109));
#140447=CARTESIAN_POINT('Ctrl Pts',(96.193080514892,14.9823184951072,61.9735427871285));
#140448=CARTESIAN_POINT('Ctrl Pts',(96.2358578027182,14.9749781871825,61.9820900878307));
#140449=CARTESIAN_POINT('Ctrl Pts',(96.278072462214,14.9677344226667,61.99052497015));
#140450=CARTESIAN_POINT('Ctrl Pts',(96.3205511352868,14.9585088652372,61.9990753497081));
#140451=CARTESIAN_POINT('Ctrl Pts',(96.3630342769716,14.9472028291044,62.0076931693938));
#140452=CARTESIAN_POINT('Ctrl Pts',(96.4048605947515,14.9360715934809,62.0161777505818));
#140453=CARTESIAN_POINT('Ctrl Pts',(96.4466906368304,14.9229232703164,62.0247275977974));
#140454=CARTESIAN_POINT('Ctrl Pts',(96.4882518102421,14.9077073157761,62.0332907098102));
#140455=CARTESIAN_POINT('Ctrl Pts',(96.4992763656077,14.9036711175772,62.0355621688364));
#140456=CARTESIAN_POINT('Ctrl Pts',(96.510281893819,14.8994896941963,62.0378345323532));
#140457=CARTESIAN_POINT('Ctrl Pts',(96.521263097106,14.8951626834577,62.0401067716795));
#140458=CARTESIAN_POINT('Ctrl Pts',(96.5620779388225,14.8790800872441,62.0485522112201));
#140459=CARTESIAN_POINT('Ctrl Pts',(96.6025573539562,14.8609822885599,62.0569960680615));
#140460=CARTESIAN_POINT('Ctrl Pts',(96.6424231041339,14.8408826368191,62.0653838282803));
#140461=CARTESIAN_POINT('Ctrl Pts',(96.6820560401633,14.8209003661205,62.073722604365));
#140462=CARTESIAN_POINT('Ctrl Pts',(96.7210816886419,14.7989394613249,62.0820057905489));
#140463=CARTESIAN_POINT('Ctrl Pts',(96.759225816053,14.7750648426393,62.0901780232053));
#140464=CARTESIAN_POINT('Ctrl Pts',(96.7969762923547,14.7514366123435,62.0982659176249));
#140465=CARTESIAN_POINT('Ctrl Pts',(96.8338625952804,14.7259341211053,62.106244985407));
#140466=CARTESIAN_POINT('Ctrl Pts',(96.8696294257684,14.6986706484175,62.1140620170905));
#140467=CARTESIAN_POINT('Ctrl Pts',(96.9052869047156,14.671490529572,62.1218551494111));
#140468=CARTESIAN_POINT('Ctrl Pts',(96.939831034534,14.642560483646,62.1294870870391));
#140469=CARTESIAN_POINT('Ctrl Pts',(96.9730303594275,14.6120396990625,62.1369078063701));
#140470=CARTESIAN_POINT('Ctrl Pts',(97.0061957622891,14.5815500996622,62.1443209434421));
#140471=CARTESIAN_POINT('Ctrl Pts',(97.0380184890529,14.5494734876474,62.1515231584376));
#140472=CARTESIAN_POINT('Ctrl Pts',(97.068299307024,14.5160096404253,62.1584694107072));
#140473=CARTESIAN_POINT('Ctrl Pts',(97.09931311718,14.4817357510665,62.1655838073326));
#140474=CARTESIAN_POINT('Ctrl Pts',(97.1287087824755,14.4460071930328,62.1724295492829));
#140475=CARTESIAN_POINT('Ctrl Pts',(97.1563155440183,14.4090742021617,62.1789655383446));
#140476=CARTESIAN_POINT('Ctrl Pts',(97.1834562895665,14.3727646587185,62.1853911966296));
#140477=CARTESIAN_POINT('Ctrl Pts',(97.2088678516148,14.335291837961,62.1915174128252));
#140478=CARTESIAN_POINT('Ctrl Pts',(97.2324352222714,14.2969167745708,62.1973135863302));
#140479=CARTESIAN_POINT('Ctrl Pts',(97.2566095827945,14.2575533415002,62.2032590432931));
#140480=CARTESIAN_POINT('Ctrl Pts',(97.2788432203137,14.2172413970997,62.2088571516982));
#140481=CARTESIAN_POINT('Ctrl Pts',(97.299066299966,14.1762750641382,62.2140850483323));
#140482=CARTESIAN_POINT('Ctrl Pts',(97.3192893796184,14.1353087311766,62.2193129449663));
#140483=CARTESIAN_POINT('Ctrl Pts',(97.3375020484776,14.0936888593738,62.2241706315931));
#140484=CARTESIAN_POINT('Ctrl Pts',(97.3536889863142,14.0517091014271,62.2286458580523));
#140485=CARTESIAN_POINT('Ctrl Pts',(97.3698918780564,14.0096879680761,62.2331254953113));
#140486=CARTESIAN_POINT('Ctrl Pts',(97.3840653445013,13.967306988715,62.2372221744852));
#140487=CARTESIAN_POINT('Ctrl Pts',(97.396245092228,13.9248481617357,62.2409331441791));
#140488=CARTESIAN_POINT('Ctrl Pts',(97.4086654939252,13.8815504105422,62.2447174371971));
#140489=CARTESIAN_POINT('Ctrl Pts',(97.4190129936999,13.8381724103773,62.2481006829844));
#140490=CARTESIAN_POINT('Ctrl Pts',(97.4273730516207,13.7949890382272,62.2510901819957));
#140491=CARTESIAN_POINT('Ctrl Pts',(97.4358374764906,13.7512665649319,62.2541170019076));
#140492=CARTESIAN_POINT('Ctrl Pts',(97.442265119551,13.7077441406454,62.2567402848846));
#140493=CARTESIAN_POINT('Ctrl Pts',(97.4467854389199,13.6646730669697,62.2589767561171));
#140494=CARTESIAN_POINT('Ctrl Pts',(97.4514017019649,13.6206878107326,62.2612606964008));
#140495=CARTESIAN_POINT('Ctrl Pts',(97.4540294770364,13.577173683171,62.2631413499673));
#140496=CARTESIAN_POINT('Ctrl Pts',(97.4548393150145,13.534355713319,62.2646443224215));
#140497=CARTESIAN_POINT('Ctrl Pts',(97.4550791011521,13.5216776766181,62.2650893397822));
#140498=CARTESIAN_POINT('Ctrl Pts',(97.4551596851296,13.5090603723168,62.2655012899924));
#140499=CARTESIAN_POINT('Ctrl Pts',(97.4550858933237,13.4965088789097,62.2658809401734));
#140500=CARTESIAN_POINT('Origin',(98.1267616152515,12.5716410462426,62.320869231712));
#140501=CARTESIAN_POINT('Origin',(98.8206098656912,12.3624040386408,62.2958872923182));
#140502=CARTESIAN_POINT('Ctrl Pts',(100.169335608469,14.99405726692,61.51611510888));
#140503=CARTESIAN_POINT('Ctrl Pts',(99.7148652716691,15.00734885163,60.98676941964));
#140504=CARTESIAN_POINT('Ctrl Pts',(98.8332753637691,14.83573834731,59.9502829098));
#140505=CARTESIAN_POINT('Ctrl Pts',(97.5676198956691,13.94788897315,58.43673095921));
#140506=CARTESIAN_POINT('Ctrl Pts',(96.8532769472691,12.93890086152,57.61785572376));
#140507=CARTESIAN_POINT('Ctrl Pts',(96.5377967531691,12.32169782044,57.28766800809));
#140508=CARTESIAN_POINT('Ctrl Pts',(99.1305766688691,14.99446242178,61.72461748813));
#140509=CARTESIAN_POINT('Ctrl Pts',(98.7164568384691,15.01076845648,61.17415228594));
#140510=CARTESIAN_POINT('Ctrl Pts',(97.9131284468691,14.83848819158,60.09687442266));
#140511=CARTESIAN_POINT('Ctrl Pts',(96.7645667377691,13.93938484243,58.54312551318));
#140512=CARTESIAN_POINT('Ctrl Pts',(96.1205077616691,12.92500300104,57.71449926823));
#140513=CARTESIAN_POINT('Ctrl Pts',(95.8379926099691,12.30969319204,57.38425138438));
#140514=CARTESIAN_POINT('Ctrl Pts',(96.3176189348691,14.99514161892,62.26071968093));
#140515=CARTESIAN_POINT('Ctrl Pts',(96.0154143699691,15.01926889724,61.65498469172));
#140516=CARTESIAN_POINT('Ctrl Pts',(95.4288082679691,14.84230328349,60.47059453057));
#140517=CARTESIAN_POINT('Ctrl Pts',(94.6024390106691,13.90781835228,58.81819612913));
#140518=CARTESIAN_POINT('Ctrl Pts',(94.1494817780691,12.87788125739,57.96906759383));
#140519=CARTESIAN_POINT('Ctrl Pts',(93.9560138780691,12.26890002092,57.6409827674));
#140520=CARTESIAN_POINT('Ctrl Pts',(93.4953850345691,14.99506638051,62.7559974319));
#140521=CARTESIAN_POINT('Ctrl Pts',(93.3103671812691,15.0242959982,62.09949931116));
#140522=CARTESIAN_POINT('Ctrl Pts',(92.9497536882691,14.83329013866,60.81498722494));
#140523=CARTESIAN_POINT('Ctrl Pts',(92.4556410153691,13.85106768651,59.08485218125));
#140524=CARTESIAN_POINT('Ctrl Pts',(92.1957994607691,12.80282306576,58.22524694262));
#140525=CARTESIAN_POINT('Ctrl Pts',(92.0912558337691,12.20332775014,57.90308798197));
#140526=CARTESIAN_POINT('Ctrl Pts',(91.7184465780691,14.9948609804,63.073805056447));
#140527=CARTESIAN_POINT('Ctrl Pts',(91.6074520331691,15.02536787074,62.38713311363));
#140528=CARTESIAN_POINT('Ctrl Pts',(91.3893306495691,14.82127594063,61.04190429299));
#140529=CARTESIAN_POINT('Ctrl Pts',(91.1046486454691,13.80536352591,59.26795531069));
#140530=CARTESIAN_POINT('Ctrl Pts',(90.9665687706691,12.7445626307,58.40207411475));
#140531=CARTESIAN_POINT('Ctrl Pts',(90.9180991174691,12.15223092569,58.08340275416));
#140532=CARTESIAN_POINT('Ctrl Pts',(95.9574506170498,14.9983799452468,62.1685358987961));
#140533=CARTESIAN_POINT('Ctrl Pts',(94.6103064012642,14.9990728434965,62.4078600669976));
#140534=CARTESIAN_POINT('Ctrl Pts',(93.2623353470216,14.9994593482969,62.640153612899));
#140535=CARTESIAN_POINT('Ctrl Pts',(91.9155436377164,14.9994907910626,62.8752831531645));
#140536=CARTESIAN_POINT('',(91.0790838175691,12.28284151812,58.13147659972));
#140537=CARTESIAN_POINT('Ctrl Pts',(91.9155428607298,14.9991665213478,62.8752787466432));
#140538=CARTESIAN_POINT('Ctrl Pts',(91.8320338374965,15.0060364948596,62.4015881812362));
#140539=CARTESIAN_POINT('Ctrl Pts',(91.7477460466049,14.9479895031152,61.9239636529671));
#140540=CARTESIAN_POINT('Ctrl Pts',(91.5847899897675,14.709291500823,61.0000296041516));
#140541=CARTESIAN_POINT('Ctrl Pts',(91.5063590297402,14.5281607691405,60.5547834032252));
#140542=CARTESIAN_POINT('Ctrl Pts',(91.360391355721,14.0537134211762,59.726275526801));
#140543=CARTESIAN_POINT('Ctrl Pts',(91.2926247379441,13.7595734546084,59.342158909907));
#140544=CARTESIAN_POINT('Ctrl Pts',(91.1722735521674,13.077960345171,58.6612811253686));
#140545=CARTESIAN_POINT('Ctrl Pts',(91.1199115659794,12.6926154932127,58.3651666009541));
#140546=CARTESIAN_POINT('Ctrl Pts',(91.0790838175691,12.28284151812,58.13147659972));
#140547=CARTESIAN_POINT('',(96.4484017897691,12.44788635501,57.38025496851));
#140548=CARTESIAN_POINT('Ctrl Pts',(96.4484001507624,12.4478935028557,57.3802439116704));
#140549=CARTESIAN_POINT('Ctrl Pts',(95.7943735804126,12.4360471853169,57.4695350918061));
#140550=CARTESIAN_POINT('Ctrl Pts',(95.1433169455258,12.4214640739689,57.5574467728654));
#140551=CARTESIAN_POINT('Ctrl Pts',(94.4942820323385,12.403912404117,57.645899157917));
#140552=CARTESIAN_POINT('Ctrl Pts',(93.3510410917193,12.3729960587199,57.8017033925302));
#140553=CARTESIAN_POINT('Ctrl Pts',(92.2140755027029,12.3328695466178,57.9591853627902));
#140554=CARTESIAN_POINT('Ctrl Pts',(91.0788501393933,12.2836266462612,58.1301510978283));
#140555=CARTESIAN_POINT('Ctrl Pts',(95.9754884061691,14.99569893684,61.9308508253));
#140556=CARTESIAN_POINT('Ctrl Pts',(96.0318216593838,14.9774616413474,61.3605505558174));
#140557=CARTESIAN_POINT('Ctrl Pts',(96.0870995927844,14.8752077739731,60.8239709384119));
#140558=CARTESIAN_POINT('Ctrl Pts',(96.1885970738804,14.5572749510219,59.8513640078858));
#140559=CARTESIAN_POINT('Ctrl Pts',(96.2348131316939,14.3415143833096,59.4152840448726));
#140560=CARTESIAN_POINT('Ctrl Pts',(96.3152663723759,13.8490496175605,58.6542136864889));
#140561=CARTESIAN_POINT('Ctrl Pts',(96.3494921073714,13.5735114454258,58.3292420428182));
#140562=CARTESIAN_POINT('Ctrl Pts',(96.4064692538042,13.0105709490317,57.7832918174657));
#140563=CARTESIAN_POINT('Ctrl Pts',(96.4293880105424,12.7235448882221,57.561431885349));
#140564=CARTESIAN_POINT('Ctrl Pts',(96.4484017897691,12.44788635501,57.38025496851));
#140565=CARTESIAN_POINT('Ctrl Pts',(95.2659401102691,14.82531735257,61.99879853622));
#140566=CARTESIAN_POINT('Ctrl Pts',(95.3458225527691,14.82663418575,61.58784104641));
#140567=CARTESIAN_POINT('Ctrl Pts',(95.5189963877691,14.73079097291,60.6969433442));
#140568=CARTESIAN_POINT('Ctrl Pts',(95.7720667392691,14.25687316564,59.39501574815));
#140569=CARTESIAN_POINT('Ctrl Pts',(96.0056186731692,13.40283085562,58.19350120435));
#140570=CARTESIAN_POINT('Ctrl Pts',(96.1266411507691,12.63732789559,57.57089763824));
#140571=CARTESIAN_POINT('Ctrl Pts',(96.176798873169,12.21892969183,57.31285981381));
#140572=CARTESIAN_POINT('Ctrl Pts',(96.5343893935691,15.50721522815,62.24751894428));
#140573=CARTESIAN_POINT('Ctrl Pts',(96.6237567750691,15.50871098773,61.78776591757));
#140574=CARTESIAN_POINT('Ctrl Pts',(96.8172823823691,15.40154840317,60.7921679457));
#140575=CARTESIAN_POINT('Ctrl Pts',(97.1010190211691,14.87088436705,59.33247676506));
#140576=CARTESIAN_POINT('Ctrl Pts',(97.3638686534691,13.90970119862,57.9802393816401));
#140577=CARTESIAN_POINT('Ctrl Pts',(97.4995976301692,13.05070844107,57.2819778141701));
#140578=CARTESIAN_POINT('Ctrl Pts',(97.5558445876691,12.5815240184,56.99261374721));
#140579=CARTESIAN_POINT('Ctrl Pts',(97.6826966252692,14.63050777912,62.4679543560901));
#140580=CARTESIAN_POINT('Ctrl Pts',(97.7598693410691,14.63177349529,62.07093713223));
#140581=CARTESIAN_POINT('Ctrl Pts',(97.9272289328691,14.53916408337,61.20995096898));
#140582=CARTESIAN_POINT('Ctrl Pts',(98.1715383149691,14.08145795388,59.9530944278801));
#140583=CARTESIAN_POINT('Ctrl Pts',(98.3967202681692,13.25802442806,58.7946394875));
#140584=CARTESIAN_POINT('Ctrl Pts',(98.5135412854691,12.51923031731,58.1936504526901));
#140585=CARTESIAN_POINT('Ctrl Pts',(98.5619593906691,12.11534109209,57.9445621383801));
#140586=CARTESIAN_POINT('Ctrl Pts',(97.3966210806691,13.19858904608,62.40781584814));
#140587=CARTESIAN_POINT('Ctrl Pts',(97.453876354069,13.19947903431,62.11326447128));
#140588=CARTESIAN_POINT('Ctrl Pts',(97.5784992177692,13.13063919407,61.47213861681));
#140589=CARTESIAN_POINT('Ctrl Pts',(97.7584124008692,12.7920945857,60.5465701472));
#140590=CARTESIAN_POINT('Ctrl Pts',(97.922072057769,12.19364636594,59.70461840367));
#140591=CARTESIAN_POINT('Ctrl Pts',(98.0080108677692,11.65117167077,59.26250375952));
#140592=CARTESIAN_POINT('Ctrl Pts',(98.043642175869,11.35392852974,59.07919748546));
#140593=CARTESIAN_POINT('',(98.1061411588691,11.63978271644,58.91650643966));
#140594=CARTESIAN_POINT('Origin',(96.6336399486667,11.6397563224413,58.6303566427588));
#140595=CARTESIAN_POINT('Ctrl Pts',(97.4550854747306,13.4965088789073,62.265880858822));
#140596=CARTESIAN_POINT('Ctrl Pts',(97.4710316674903,13.4939105765947,62.1838452181956));
#140597=CARTESIAN_POINT('Ctrl Pts',(97.4868368133731,13.4890042223143,62.1025351947875));
#140598=CARTESIAN_POINT('Ctrl Pts',(97.5025133966026,13.4818673165301,62.0218865595026));
#140599=CARTESIAN_POINT('Ctrl Pts',(97.5183414772651,13.4746614401742,61.9404585412976));
#140600=CARTESIAN_POINT('Ctrl Pts',(97.5340386156073,13.4651816199485,61.859704152008));
#140601=CARTESIAN_POINT('Ctrl Pts',(97.5496185369051,13.4534544942426,61.7795527920009));
#140602=CARTESIAN_POINT('Ctrl Pts',(97.5652427832381,13.4416940047444,61.6991734005564));
#140603=CARTESIAN_POINT('Ctrl Pts',(97.5807492628728,13.4276733183867,61.6193998689467));
#140604=CARTESIAN_POINT('Ctrl Pts',(97.5961509203515,13.4113674093164,61.540165617543));
#140605=CARTESIAN_POINT('Ctrl Pts',(97.6005894255313,13.4066683136528,61.5173316053105));
#140606=CARTESIAN_POINT('Ctrl Pts',(97.6050192133311,13.4017791063397,61.4945424413528));
#140607=CARTESIAN_POINT('Ctrl Pts',(97.6094405582086,13.3966984044635,61.4717967133184));
#140608=CARTESIAN_POINT('Ctrl Pts',(97.6217225074074,13.3825848430778,61.4086118942317));
#140609=CARTESIAN_POINT('Ctrl Pts',(97.6339394170431,13.3669950677195,61.3457616858146));
#140610=CARTESIAN_POINT('Ctrl Pts',(97.6460994865771,13.3499001745025,61.2832038634467));
#140611=CARTESIAN_POINT('Ctrl Pts',(97.6654943689363,13.322634422283,61.183426341445));
#140612=CARTESIAN_POINT('Ctrl Pts',(97.6847450916549,13.2916668606854,61.0843903797846));
#140613=CARTESIAN_POINT('Ctrl Pts',(97.7037650545336,13.2570607508129,60.986541612079));
#140614=CARTESIAN_POINT('Ctrl Pts',(97.7226733142535,13.2226578806529,60.8892675046138));
#140615=CARTESIAN_POINT('Ctrl Pts',(97.7413534008831,13.1846592194458,60.793167275849));
#140616=CARTESIAN_POINT('Ctrl Pts',(97.7597222786598,13.1431769134627,60.698668092815));
#140617=CARTESIAN_POINT('Ctrl Pts',(97.7770207196428,13.1041119672744,60.6096758004973));
#140618=CARTESIAN_POINT('Ctrl Pts',(97.7940431028222,13.0619580618998,60.5221037113969));
#140619=CARTESIAN_POINT('Ctrl Pts',(97.810723134052,13.0168479924667,60.4362928354362));
#140620=CARTESIAN_POINT('Ctrl Pts',(97.8153555595118,13.0043198963704,60.4124611962112));
#140621=CARTESIAN_POINT('Ctrl Pts',(97.8199616014906,12.9915640125088,60.3887652855272));
#140622=CARTESIAN_POINT('Ctrl Pts',(97.824540077791,12.9785846860467,60.3652111844326));
#140623=CARTESIAN_POINT('Ctrl Pts',(97.84505639357,12.920423860736,60.2596644164161));
#140624=CARTESIAN_POINT('Ctrl Pts',(97.8650117626206,12.8576748931493,60.1570034319238));
#140625=CARTESIAN_POINT('Ctrl Pts',(97.8843730926296,12.7905931363591,60.0573985277848));
#140626=CARTESIAN_POINT('Ctrl Pts',(97.9037787186106,12.7233579060411,59.9575657417781));
#140627=CARTESIAN_POINT('Ctrl Pts',(97.9225876941704,12.6517700260684,59.860802443492));
#140628=CARTESIAN_POINT('Ctrl Pts',(97.9407669328909,12.5760343521528,59.7672788340814));
#140629=CARTESIAN_POINT('Ctrl Pts',(97.9541162592562,12.5204203496004,59.6986028458245));
#140630=CARTESIAN_POINT('Ctrl Pts',(97.9671260345575,12.4625686736672,59.6316736884987));
#140631=CARTESIAN_POINT('Ctrl Pts',(97.9797826669382,12.4025427161283,59.5665612844729));
#140632=CARTESIAN_POINT('Ctrl Pts',(97.9812479553316,12.3955933684475,59.5590230668007));
#140633=CARTESIAN_POINT('Ctrl Pts',(97.9827083599984,12.3886146548968,59.5515099735276));
#140634=CARTESIAN_POINT('Ctrl Pts',(97.9841638984601,12.3816064428523,59.5440219145336));
#140635=CARTESIAN_POINT('Ctrl Pts',(97.9960965004404,12.3241526502376,59.4826343044275));
#140636=CARTESIAN_POINT('Ctrl Pts',(98.007702617975,12.2647194408385,59.4229263001133));
#140637=CARTESIAN_POINT('Ctrl Pts',(98.0189889056623,12.2032956677188,59.3648636713558));
#140638=CARTESIAN_POINT('Ctrl Pts',(98.0302418362812,12.1420534349835,59.3069726489878));
#140639=CARTESIAN_POINT('Ctrl Pts',(98.0411768994689,12.0788318970064,59.2507169060417));
#140640=CARTESIAN_POINT('Ctrl Pts',(98.0517931981222,12.0135865599172,59.1961010571825));
#140641=CARTESIAN_POINT('Ctrl Pts',(98.062222148816,11.9494926204258,59.1424490252025));
#140642=CARTESIAN_POINT('Ctrl Pts',(98.0723435436394,11.8834451697451,59.0903792238159));
#140643=CARTESIAN_POINT('Ctrl Pts',(98.082148346113,11.8153772009759,59.0399381404546));
#140644=CARTESIAN_POINT('Ctrl Pts',(98.0903722575035,11.7582842666511,58.9976299959384));
#140645=CARTESIAN_POINT('Ctrl Pts',(98.0983733254029,11.6997692909013,58.9564682759002));
#140646=CARTESIAN_POINT('Ctrl Pts',(98.106141158279,11.63978271644,58.9165064395453));
#140647=CARTESIAN_POINT('Origin',(97.1688706058691,111.0726804259,63.738321366581));
#140648=CARTESIAN_POINT('',(98.1858652500691,10.88568327564,58.50636359317));
#140649=CARTESIAN_POINT('Ctrl Pts',(98.1061411591776,11.63978271644,58.91650643972));
#140650=CARTESIAN_POINT('Ctrl Pts',(98.108957693088,11.6180159291794,58.9020167011815));
#140651=CARTESIAN_POINT('Ctrl Pts',(98.111757780675,11.5959177554122,58.887611571194));
#140652=CARTESIAN_POINT('Ctrl Pts',(98.1145737776585,11.5732403953004,58.8731245948671));
#140653=CARTESIAN_POINT('Ctrl Pts',(98.1157390292683,11.5638565676433,58.8671299249208));
#140654=CARTESIAN_POINT('Ctrl Pts',(98.1169069832582,11.5543731003895,58.8611213525139));
#140655=CARTESIAN_POINT('Ctrl Pts',(98.1180781549355,11.5447817294967,58.8550962266101));
#140656=CARTESIAN_POINT('Ctrl Pts',(98.121010950369,11.5207634499409,58.8400083773408));
#140657=CARTESIAN_POINT('Ctrl Pts',(98.1239728709995,11.4960136689371,58.8247706926541));
#140658=CARTESIAN_POINT('Ctrl Pts',(98.1268620657231,11.4713264099956,58.8099071485045));
#140659=CARTESIAN_POINT('Ctrl Pts',(98.1270884423703,11.469392092844,58.8087425474262));
#140660=CARTESIAN_POINT('Ctrl Pts',(98.1273143750141,11.4674581802752,58.8075802305365));
#140661=CARTESIAN_POINT('Ctrl Pts',(98.1275398164358,11.4655250607335,58.8064204407522));
#140662=CARTESIAN_POINT('Ctrl Pts',(98.1283628179086,11.4584679715023,58.8021864863481));
#140663=CARTESIAN_POINT('Ctrl Pts',(98.1291792664275,11.4514214597892,58.7979862438015));
#140664=CARTESIAN_POINT('Ctrl Pts',(98.1299883415914,11.4443905815583,58.7938239336896));
#140665=CARTESIAN_POINT('Ctrl Pts',(98.1333240402532,11.4154032981102,58.7766633373815));
#140666=CARTESIAN_POINT('Ctrl Pts',(98.1365184813657,11.3868197450042,58.7602294445414));
#140667=CARTESIAN_POINT('Ctrl Pts',(98.1396491641854,11.3578775779917,58.7441235580485));
#140668=CARTESIAN_POINT('Ctrl Pts',(98.1401405593415,11.3533347860531,58.7415955617414));
#140669=CARTESIAN_POINT('Ctrl Pts',(98.1406303646256,11.3487831606216,58.7390757445758));
#140670=CARTESIAN_POINT('Ctrl Pts',(98.141119084895,11.3442187888434,58.7365615092952));
#140671=CARTESIAN_POINT('Ctrl Pts',(98.1434235917695,11.3226959939062,58.7247059083503));
#140672=CARTESIAN_POINT('Ctrl Pts',(98.1457009550164,11.3009021167795,58.7129899485201));
#140673=CARTESIAN_POINT('Ctrl Pts',(98.148004722259,11.2783989497205,58.7011381526501));
#140674=CARTESIAN_POINT('Ctrl Pts',(98.1490995696116,11.267704495687,58.6955056794158));
#140675=CARTESIAN_POINT('Ctrl Pts',(98.1502004020906,11.2568493114865,58.6898424155362));
#140676=CARTESIAN_POINT('Ctrl Pts',(98.1513132659929,11.2457821220828,58.6841172556582));
#140677=CARTESIAN_POINT('Ctrl Pts',(98.1515191903653,11.2437342489988,58.6830578718898));
#140678=CARTESIAN_POINT('Ctrl Pts',(98.1517255276039,11.2416791064181,58.6819963641191));
#140679=CARTESIAN_POINT('Ctrl Pts',(98.1519322820927,11.2396167148383,58.680932709793));
#140680=CARTESIAN_POINT('Ctrl Pts',(98.1541341104614,11.2176533112195,58.6696053413607));
#140681=CARTESIAN_POINT('Ctrl Pts',(98.156385810195,11.1948478916945,58.6580214082935));
#140682=CARTESIAN_POINT('Ctrl Pts',(98.1586590821498,11.171568427522,58.6463264963344));
#140683=CARTESIAN_POINT('Ctrl Pts',(98.1601802832843,11.1559905521009,58.6385006340118));
#140684=CARTESIAN_POINT('Ctrl Pts',(98.161711085333,11.1402017840564,58.6306253795112));
#140685=CARTESIAN_POINT('Ctrl Pts',(98.1632426453179,11.1243220713734,58.6227462257746));
#140686=CARTESIAN_POINT('Ctrl Pts',(98.1633263038242,11.1234546727363,58.6223158422186));
#140687=CARTESIAN_POINT('Ctrl Pts',(98.1634099653807,11.122586987239,58.6218854429707));
#140688=CARTESIAN_POINT('Ctrl Pts',(98.1634936289301,11.1217190315489,58.6214550334704));
#140689=CARTESIAN_POINT('Ctrl Pts',(98.1672305078062,11.0829513088304,58.6022305542108));
#140690=CARTESIAN_POINT('Ctrl Pts',(98.1709714100823,11.0436418556078,58.5829853763942));
#140691=CARTESIAN_POINT('Ctrl Pts',(98.174663363706,11.00463610201,58.5639920163024));
#140692=CARTESIAN_POINT('Ctrl Pts',(98.175041887474,11.0006369713794,58.5620446900463));
#140693=CARTESIAN_POINT('Ctrl Pts',(98.1754199002714,10.996640893791,58.5600999924886));
#140694=CARTESIAN_POINT('Ctrl Pts',(98.1757974296572,10.9926477485928,58.5581577818497));
#140695=CARTESIAN_POINT('Ctrl Pts',(98.1791845957236,10.9568215416152,58.5407324098953));
#140696=CARTESIAN_POINT('Ctrl Pts',(98.1825328300625,10.9212333134944,58.52350732206));
#140697=CARTESIAN_POINT('Ctrl Pts',(98.1858652500111,10.88568327564,58.5063635931587));
#140698=CARTESIAN_POINT('',(98.2872556700151,9.75862481052195,57.9847577051873));
#140699=CARTESIAN_POINT('Ctrl Pts',(98.1858652500691,10.88568327564,58.50636359317));
#140700=CARTESIAN_POINT('Ctrl Pts',(98.1966659246691,10.77045641959,58.45079921683));
#140701=CARTESIAN_POINT('Ctrl Pts',(98.2187284794691,10.53376517775,58.33729777984));
#140702=CARTESIAN_POINT('Ctrl Pts',(98.2525318077691,10.1617048254,58.1633955988));
#140703=CARTESIAN_POINT('Ctrl Pts',(98.2756771376691,9.89580942135701,58.044323793));
#140704=CARTESIAN_POINT('Ctrl Pts',(98.2872556111691,9.75862550816901,57.98475800809));
#140705=CARTESIAN_POINT('',(98.6928295681274,5.40399176655855E-8,55.8982712910719));
#140706=CARTESIAN_POINT('Ctrl Pts',(98.2872556700071,9.75862481052194,57.9847577051857));
#140707=CARTESIAN_POINT('Ctrl Pts',(98.2938324661056,9.68069541295108,57.9509231912672));
#140708=CARTESIAN_POINT('Ctrl Pts',(98.3005315104572,9.60020361132716,57.9164597677727));
#140709=CARTESIAN_POINT('Ctrl Pts',(98.3073332358664,9.51720250231419,57.8814680986399));
#140710=CARTESIAN_POINT('Ctrl Pts',(98.3114852418091,9.46653578510105,57.8601079863974));
#140711=CARTESIAN_POINT('Ctrl Pts',(98.315675509981,9.41493407546324,57.8385510330277));
#140712=CARTESIAN_POINT('Ctrl Pts',(98.3198995954507,9.36240953697897,57.8168201056097));
#140713=CARTESIAN_POINT('Ctrl Pts',(98.3272912721984,9.27049747398018,57.7787934150857));
#140714=CARTESIAN_POINT('Ctrl Pts',(98.3347860684279,9.17575904375019,57.740236223455));
#140715=CARTESIAN_POINT('Ctrl Pts',(98.3423907023324,9.07784748703031,57.7011139687803));
#140716=CARTESIAN_POINT('Ctrl Pts',(98.3462510395746,9.02814468297722,57.6812543544166));
#140717=CARTESIAN_POINT('Ctrl Pts',(98.3501396227374,8.97762411472197,57.6612494281096));
#140718=CARTESIAN_POINT('Ctrl Pts',(98.3540569257759,8.92624000370595,57.6410967515864));
#140719=CARTESIAN_POINT('Ctrl Pts',(98.3622776065608,8.81840755624538,57.5988052262606));
#140720=CARTESIAN_POINT('Ctrl Pts',(98.3706251328623,8.70677272130092,57.555861140571));
#140721=CARTESIAN_POINT('Ctrl Pts',(98.3790873026441,8.59108494554968,57.5123272682698));
#140722=CARTESIAN_POINT('Ctrl Pts',(98.3826010515574,8.54304788096543,57.4942506873886));
#140723=CARTESIAN_POINT('Ctrl Pts',(98.3861345253723,8.49431200908934,57.4760726311964));
#140724=CARTESIAN_POINT('Ctrl Pts',(98.3896865688376,8.44485924296572,57.4577990429139));
#140725=CARTESIAN_POINT('Ctrl Pts',(98.3987630183157,8.31849380356387,57.4111049913216));
#140726=CARTESIAN_POINT('Ctrl Pts',(98.4079611173156,8.18744778524474,57.3637851103391));
#140727=CARTESIAN_POINT('Ctrl Pts',(98.4172610042855,8.05137118275037,57.3159415782706));
#140728=CARTESIAN_POINT('Ctrl Pts',(98.4203655829907,8.00594476802641,57.2999699851403));
#140729=CARTESIAN_POINT('Ctrl Pts',(98.4234814533572,7.95995772525002,57.2839403017396));
#140730=CARTESIAN_POINT('Ctrl Pts',(98.4266076415366,7.91339695145371,57.2678575380585));
#140731=CARTESIAN_POINT('Ctrl Pts',(98.4365115964214,7.76588957933778,57.216906361488));
#140732=CARTESIAN_POINT('Ctrl Pts',(98.4465198842675,7.61262391526305,57.1654184410462));
#140733=CARTESIAN_POINT('Ctrl Pts',(98.4565927279828,7.45322050326538,57.1135984110812));
#140734=CARTESIAN_POINT('Ctrl Pts',(98.4592236929996,7.4115853094341,57.100063336989));
#140735=CARTESIAN_POINT('Ctrl Pts',(98.4618590112775,7.36953140210051,57.0865058674196));
#140736=CARTESIAN_POINT('Ctrl Pts',(98.4644977943282,7.32705180073446,57.0729305732268));
#140737=CARTESIAN_POINT('Ctrl Pts',(98.4737471702992,7.17815369256111,57.0253468963982));
#140738=CARTESIAN_POINT('Ctrl Pts',(98.4830399243306,7.02402682490015,56.9775400598888));
#140739=CARTESIAN_POINT('Ctrl Pts',(98.4923349328763,6.86431827542829,56.9297216249575));
#140740=CARTESIAN_POINT('Ctrl Pts',(98.4937450242413,6.84008982578176,56.9224673699615));
#140741=CARTESIAN_POINT('Ctrl Pts',(98.495155148829,6.81573291735723,56.9152129440496));
#140742=CARTESIAN_POINT('Ctrl Pts',(98.4965651426352,6.79124631741037,56.907959190947));
#140743=CARTESIAN_POINT('Ctrl Pts',(98.4986643177188,6.75479107890955,56.8971599252279));
#140744=CARTESIAN_POINT('Ctrl Pts',(98.5007632042589,6.71804838275074,56.8863621439284));
#140745=CARTESIAN_POINT('Ctrl Pts',(98.5028612343922,6.68101408690589,56.8755687684378));
#140746=CARTESIAN_POINT('Ctrl Pts',(98.5117937371179,6.52333811108084,56.8296152549685));
#140747=CARTESIAN_POINT('Ctrl Pts',(98.5207113052586,6.36037729196436,56.783738572884));
#140748=CARTESIAN_POINT('Ctrl Pts',(98.5295639120642,6.19183044120843,56.7381960862364));
#140749=CARTESIAN_POINT('Ctrl Pts',(98.5318613063152,6.14808981492023,56.7263770763899));
#140750=CARTESIAN_POINT('Ctrl Pts',(98.5341542738737,6.10397297544074,56.7145808397893));
#140751=CARTESIAN_POINT('Ctrl Pts',(98.536441828956,6.05947465891517,56.7028124478262));
#140752=CARTESIAN_POINT('Ctrl Pts',(98.5379673597325,6.02979950403509,56.6949643115041));
#140753=CARTESIAN_POINT('Ctrl Pts',(98.5394904824751,5.99995469400219,56.687128563381));
#140754=CARTESIAN_POINT('Ctrl Pts',(98.541010884844,5.96993866215367,56.6793068102967));
#140755=CARTESIAN_POINT('Ctrl Pts',(98.5490671310346,5.81089093427212,56.6378612234056));
#140756=CARTESIAN_POINT('Ctrl Pts',(98.557047457191,5.64703601870898,56.5968062092273));
#140757=CARTESIAN_POINT('Ctrl Pts',(98.5649017095693,5.47807690593747,56.5563997852451));
#140758=CARTESIAN_POINT('Ctrl Pts',(98.5683654825653,5.40356491115158,56.5385803068891));
#140759=CARTESIAN_POINT('Ctrl Pts',(98.5718046102653,5.32806022579709,56.5208876169778));
#140760=CARTESIAN_POINT('Ctrl Pts',(98.5752141681515,5.25153744002567,56.5033470498056));
#140761=CARTESIAN_POINT('Ctrl Pts',(98.5761510227838,5.23051104049898,56.4985273745994));
#140762=CARTESIAN_POINT('Ctrl Pts',(98.5770856425293,5.2094077745652,56.4937191968305));
#140763=CARTESIAN_POINT('Ctrl Pts',(98.5780179284323,5.18822710561756,56.4889230255777));
#140764=CARTESIAN_POINT('Ctrl Pts',(98.5896228921777,4.92457311873915,56.4292209606589));
#140765=CARTESIAN_POINT('Ctrl Pts',(98.6008697818594,4.64892682249802,56.3713610178423));
#140766=CARTESIAN_POINT('Ctrl Pts',(98.6114959693711,4.3619790174758,56.3166942950998));
#140767=CARTESIAN_POINT('Ctrl Pts',(98.6118749303484,4.35174561810061,56.3147447196141));
#140768=CARTESIAN_POINT('Ctrl Pts',(98.6122531015984,4.34149785024426,56.3127992069021));
#140769=CARTESIAN_POINT('Ctrl Pts',(98.6126304712299,4.33123575067178,56.3108578181371));
#140770=CARTESIAN_POINT('Ctrl Pts',(98.6185074083927,4.17141972598951,56.2806237483352));
#140771=CARTESIAN_POINT('Ctrl Pts',(98.624187943365,4.00812585773189,56.2514000749912));
#140772=CARTESIAN_POINT('Ctrl Pts',(98.6296439055601,3.84092052918692,56.2233317228906));
#140773=CARTESIAN_POINT('Ctrl Pts',(98.6343618715543,3.69633209072024,56.1990600131557));
#140774=CARTESIAN_POINT('Ctrl Pts',(98.6389117954758,3.54881871977499,56.1756528006555));
#140775=CARTESIAN_POINT('Ctrl Pts',(98.6432694545152,3.39810126942076,56.1532347002108));
#140776=CARTESIAN_POINT('Ctrl Pts',(98.6433517135133,3.39525619449609,56.1528115164634));
#140777=CARTESIAN_POINT('Ctrl Pts',(98.6434339037304,3.39240997828525,56.1523886865624));
#140778=CARTESIAN_POINT('Ctrl Pts',(98.6435160249773,3.38956261908564,56.1519662114799));
#140779=CARTESIAN_POINT('Ctrl Pts',(98.6483479194062,3.22202815546134,56.1271083936297));
#140780=CARTESIAN_POINT('Ctrl Pts',(98.6529418144172,3.05053624630029,56.1034749704414));
#140781=CARTESIAN_POINT('Ctrl Pts',(98.6572541559725,2.87474284373071,56.0812900070522));
#140782=CARTESIAN_POINT('Ctrl Pts',(98.6612410191838,2.71221762616855,56.0607794762317));
#140783=CARTESIAN_POINT('Ctrl Pts',(98.6649871771304,2.54601565953765,56.04150726062));
#140784=CARTESIAN_POINT('Ctrl Pts',(98.6684507060235,2.37587034056348,56.0236890380562));
#140785=CARTESIAN_POINT('Ctrl Pts',(98.6688289428818,2.35728951364044,56.0217431878175));
#140786=CARTESIAN_POINT('Ctrl Pts',(98.669203783092,2.33866168424419,56.0198148117289));
#140787=CARTESIAN_POINT('Ctrl Pts',(98.6695751687599,2.31998634897416,56.0179042076281));
#140788=CARTESIAN_POINT('Ctrl Pts',(98.6729603432827,2.14976096168309,56.000489081296));
#140789=CARTESIAN_POINT('Ctrl Pts',(98.6760593868739,1.97558797111138,55.9845459635106));
#140790=CARTESIAN_POINT('Ctrl Pts',(98.6788217101339,1.79709173088618,55.9703351132181));
#140791=CARTESIAN_POINT('Ctrl Pts',(98.6814391775938,1.62795580560928,55.9568694776945));
#140792=CARTESIAN_POINT('Ctrl Pts',(98.6837542976694,1.45493804794544,55.9449592770681));
#140793=CARTESIAN_POINT('Ctrl Pts',(98.6857145488864,1.27772726544477,55.9348747091783));
#140794=CARTESIAN_POINT('Ctrl Pts',(98.6858230330464,1.26792007200714,55.9343166093458));
#140795=CARTESIAN_POINT('Ctrl Pts',(98.6859304278319,1.25810003896687,55.9337641138303));
#140796=CARTESIAN_POINT('Ctrl Pts',(98.6860367234487,1.24826711449324,55.9332172730186));
#140797=CARTESIAN_POINT('Ctrl Pts',(98.6864430693246,1.21067790404311,55.9311268151483));
#140798=CARTESIAN_POINT('Ctrl Pts',(98.6868334406238,1.17290063339673,55.9291185389282));
#140799=CARTESIAN_POINT('Ctrl Pts',(98.6872072395185,1.13493594641422,55.9271955199121));
#140800=CARTESIAN_POINT('Ctrl Pts',(98.6892422221279,0.928254014288536,
55.9167264941582));
#140801=CARTESIAN_POINT('Ctrl Pts',(98.6907866121855,0.716014733679109,
55.9087813358087));
#140802=CARTESIAN_POINT('Ctrl Pts',(98.6917376176423,0.498367644923183,
55.9038888613311));
#140803=CARTESIAN_POINT('Ctrl Pts',(98.692450329743,0.335256368631961,55.900222293766));
#140804=CARTESIAN_POINT('Ctrl Pts',(98.6928296276282,0.1691084573483,55.898270985022));
#140805=CARTESIAN_POINT('Ctrl Pts',(98.6928295681199,5.40399167993425E-8,
55.8982712910703));
#140806=CARTESIAN_POINT('',(98.2872554315585,-9.75846368330451,57.9847589320145));
#140807=CARTESIAN_POINT('Ctrl Pts',(98.6928295681281,6.6572433925823E-14,
55.898271291072));
#140808=CARTESIAN_POINT('Ctrl Pts',(98.6928296474929,-0.233002523781841,
55.8982708828174));
#140809=CARTESIAN_POINT('Ctrl Pts',(98.6921101359835,-0.460828478822231,
55.901972430164));
#140810=CARTESIAN_POINT('Ctrl Pts',(98.6907814689873,-0.683286144820053,
55.9088077951516));
#140811=CARTESIAN_POINT('Ctrl Pts',(98.6895584056879,-0.888062667241723,
55.9150998789302));
#140812=CARTESIAN_POINT('Ctrl Pts',(98.6878190826087,-1.08829092549095,
55.924047875812));
#140813=CARTESIAN_POINT('Ctrl Pts',(98.6856443363506,-1.2838487345319,55.9352359196192));
#140814=CARTESIAN_POINT('Ctrl Pts',(98.6852103789473,-1.3228711072297,55.9374684257888));
#140815=CARTESIAN_POINT('Ctrl Pts',(98.6847590680062,-1.3617075926073,55.9397902077243));
#140816=CARTESIAN_POINT('Ctrl Pts',(98.6842910076255,-1.40035752210753,
55.9421981576195));
#140817=CARTESIAN_POINT('Ctrl Pts',(98.6821032008459,-1.58101493574617,
55.9534533916101));
#140818=CARTESIAN_POINT('Ctrl Pts',(98.6795477347256,-1.75758682047222,
55.966600059531));
#140819=CARTESIAN_POINT('Ctrl Pts',(98.67667745122,-1.93039577447675,55.9813663143511));
#140820=CARTESIAN_POINT('Ctrl Pts',(98.6737209928796,-2.10839299056471,
55.9965758980511));
#140821=CARTESIAN_POINT('Ctrl Pts',(98.670430508282,-2.28239809007581,56.0135038891433));
#140822=CARTESIAN_POINT('Ctrl Pts',(98.6668533640194,-2.4527727677904,56.0319066092901));
#140823=CARTESIAN_POINT('Ctrl Pts',(98.6658545410567,-2.50034539217089,
56.0370450823593));
#140824=CARTESIAN_POINT('Ctrl Pts',(98.6648333089686,-2.54763501352004,
56.042298839829));
#140825=CARTESIAN_POINT('Ctrl Pts',(98.6637905639107,-2.59464960347772,
56.0476632713666));
#140826=CARTESIAN_POINT('Ctrl Pts',(98.6633077144648,-2.61641999551992,
56.0501473040416));
#140827=CARTESIAN_POINT('Ctrl Pts',(98.662820251386,-2.6381314155892,56.0526550716774));
#140828=CARTESIAN_POINT('Ctrl Pts',(98.6623282582051,-2.65978465620982,
56.0551861445406));
#140829=CARTESIAN_POINT('Ctrl Pts',(98.6585713879635,-2.82512925543108,
56.0745134699746));
#140830=CARTESIAN_POINT('Ctrl Pts',(98.6545512559065,-2.9870775460763,56.0951951515127));
#140831=CARTESIAN_POINT('Ctrl Pts',(98.6502908550547,-3.14611017159622,
56.1171129019404));
#140832=CARTESIAN_POINT('Ctrl Pts',(98.6459153901131,-3.30943791979361,
56.1396226027721));
#140833=CARTESIAN_POINT('Ctrl Pts',(98.6412864794858,-3.46969054367775,
56.1634361641968));
#140834=CARTESIAN_POINT('Ctrl Pts',(98.6364185581575,-3.6273878627602,56.1884793274269));
#140835=CARTESIAN_POINT('Ctrl Pts',(98.6348423095874,-3.67845076147005,
56.1965883841619));
#140836=CARTESIAN_POINT('Ctrl Pts',(98.6332409224524,-3.72924572385145,
56.2048267671867));
#140837=CARTESIAN_POINT('Ctrl Pts',(98.6316146662119,-3.77979033808198,
56.2131930889267));
#140838=CARTESIAN_POINT('Ctrl Pts',(98.631368185853,-3.7874510340703,56.2144611141826));
#140839=CARTESIAN_POINT('Ctrl Pts',(98.6311211340222,-3.79510597914968,
56.2157320793639));
#140840=CARTESIAN_POINT('Ctrl Pts',(98.6308735113466,-3.80275523505594,
56.2170059812372));
#140841=CARTESIAN_POINT('Ctrl Pts',(98.6255167623133,-3.96822935443883,
56.2445639284743));
#140842=CARTESIAN_POINT('Ctrl Pts',(98.6199010201482,-4.13104773944181,
56.2734542528777));
#140843=CARTESIAN_POINT('Ctrl Pts',(98.614091333514,-4.29051457498224,56.3033423413468));
#140844=CARTESIAN_POINT('Ctrl Pts',(98.6080973471629,-4.45504015026177,
56.3341785646449));
#140845=CARTESIAN_POINT('Ctrl Pts',(98.60189696042,-4.61599801174581,56.3660766493794));
#140846=CARTESIAN_POINT('Ctrl Pts',(98.5955713922438,-4.77264457106099,
56.3986187291727));
#140847=CARTESIAN_POINT('Ctrl Pts',(98.5944765483748,-4.79975731734657,
56.4042511870888));
#140848=CARTESIAN_POINT('Ctrl Pts',(98.5933779763023,-4.82674095913177,
56.4099028241245));
#140849=CARTESIAN_POINT('Ctrl Pts',(98.5922761238409,-4.85359170514252,
56.4155713353442));
#140850=CARTESIAN_POINT('Ctrl Pts',(98.5921063773628,-4.85772821137103,
56.4164446009122));
#140851=CARTESIAN_POINT('Ctrl Pts',(98.5919365365544,-4.86186154246186,
56.4173183517196));
#140852=CARTESIAN_POINT('Ctrl Pts',(98.5917665996274,-4.8659917644681,56.4181925969701));
#140853=CARTESIAN_POINT('Ctrl Pts',(98.5875838950192,-4.9676500615998,56.439710637237));
#140854=CARTESIAN_POINT('Ctrl Pts',(98.5833437983902,-5.06742568600838,
56.4615239092009));
#140855=CARTESIAN_POINT('Ctrl Pts',(98.5790151557521,-5.16630175587408,
56.4837927191261));
#140856=CARTESIAN_POINT('Ctrl Pts',(98.5746405785477,-5.26622707599619,
56.5062978405731));
#140857=CARTESIAN_POINT('Ctrl Pts',(98.5701755389641,-5.36523370042368,
56.5292683593524));
#140858=CARTESIAN_POINT('Ctrl Pts',(98.5655779015931,-5.4643255132017,56.5529210461131));
#140859=CARTESIAN_POINT('Ctrl Pts',(98.5609687180466,-5.56366617802217,
56.5766331325279));
#140860=CARTESIAN_POINT('Ctrl Pts',(98.5562262616802,-5.66309253484219,
56.6010308600264));
#140861=CARTESIAN_POINT('Ctrl Pts',(98.5512983893228,-5.76360426017417,
56.6263824488875));
#140862=CARTESIAN_POINT('Ctrl Pts',(98.5503261219759,-5.78343518545595,
56.6313843077533));
#140863=CARTESIAN_POINT('Ctrl Pts',(98.5493466068255,-5.80330832208338,
56.6364234523898));
#140864=CARTESIAN_POINT('Ctrl Pts',(98.5483593988895,-5.82323128918212,
56.6415021715976));
#140865=CARTESIAN_POINT('Ctrl Pts',(98.5476218816008,-5.83811521802843,
56.6452963501927));
#140866=CARTESIAN_POINT('Ctrl Pts',(98.5468803236845,-5.85302723303626,
56.6491113152531));
#140867=CARTESIAN_POINT('Ctrl Pts',(98.5461347475265,-5.86796609953466,
56.6529469518745));
#140868=CARTESIAN_POINT('Ctrl Pts',(98.539662373568,-5.99765094721716,56.6862442539868));
#140869=CARTESIAN_POINT('Ctrl Pts',(98.5328863818807,-6.12935871916372,
56.7211035119263));
#140870=CARTESIAN_POINT('Ctrl Pts',(98.5258273229773,-6.26228133553224,
56.7574190434097));
#140871=CARTESIAN_POINT('Ctrl Pts',(98.5187946772217,-6.39470659031704,
56.7935986916948));
#140872=CARTESIAN_POINT('Ctrl Pts',(98.5114810749149,-6.52833747013118,
56.8312237430612));
#140873=CARTESIAN_POINT('Ctrl Pts',(98.5039165891754,-6.66238366461827,
56.8701394614732));
#140874=CARTESIAN_POINT('Ctrl Pts',(98.500829836016,-6.71708236174012,56.8860193534973));
#140875=CARTESIAN_POINT('Ctrl Pts',(98.4977014210483,-6.77185032717012,
56.9021135744207));
#140876=CARTESIAN_POINT('Ctrl Pts',(98.4945338538751,-6.82663436643004,
56.9184092135179));
#140877=CARTESIAN_POINT('Ctrl Pts',(98.493003329194,-6.85310525706257,56.9262830411173));
#140878=CARTESIAN_POINT('Ctrl Pts',(98.4914635315537,-6.87957978561574,
56.93420457341));
#140879=CARTESIAN_POINT('Ctrl Pts',(98.4899146152936,-6.90605554898886,
56.9421730165938));
#140880=CARTESIAN_POINT('Ctrl Pts',(98.4799287769744,-7.0767443713754,56.9935454421638));
#140881=CARTESIAN_POINT('Ctrl Pts',(98.4695631611305,-7.24748321033599,
57.046871644524));
#140882=CARTESIAN_POINT('Ctrl Pts',(98.4588614968984,-7.41761929184993,
57.1019266614792));
#140883=CARTESIAN_POINT('Ctrl Pts',(98.4499447236189,-7.55937900628529,
57.1477992560068));
#140884=CARTESIAN_POINT('Ctrl Pts',(98.4407948299866,-7.70072045197103,
57.1948711448736));
#140885=CARTESIAN_POINT('Ctrl Pts',(98.4314420591005,-7.84127558167099,
57.242986739758));
#140886=CARTESIAN_POINT('Ctrl Pts',(98.4289556404352,-7.87864193034442,
57.2557781910477));
#140887=CARTESIAN_POINT('Ctrl Pts',(98.4264548838178,-7.91595286969873,
57.2686434042667));
#140888=CARTESIAN_POINT('Ctrl Pts',(98.4239404978578,-7.95319956841815,
57.2815787339915));
#140889=CARTESIAN_POINT('Ctrl Pts',(98.4133514625485,-8.11005957883956,
57.3360543257941));
#140890=CARTESIAN_POINT('Ctrl Pts',(98.4025199853583,-8.26577859095142,
57.3917771663333));
#140891=CARTESIAN_POINT('Ctrl Pts',(98.3914982332011,-8.41970398105144,
57.4484788828979));
#140892=CARTESIAN_POINT('Ctrl Pts',(98.381644947558,-8.55731103433506,57.4991693903411));
#140893=CARTESIAN_POINT('Ctrl Pts',(98.3716397225239,-8.6934847827116,57.5506415552392));
#140894=CARTESIAN_POINT('Ctrl Pts',(98.3615259095763,-8.82777412625757,
57.6026723526391));
#140895=CARTESIAN_POINT('Ctrl Pts',(98.3580260822914,-8.87424418765305,
57.6206773133141));
#140896=CARTESIAN_POINT('Ctrl Pts',(98.3545128408008,-8.92048773989161,
57.6387512835947));
#140897=CARTESIAN_POINT('Ctrl Pts',(98.3509861898095,-8.96651232671047,
57.656894239467));
#140898=CARTESIAN_POINT('Ctrl Pts',(98.3363782376875,-9.15715352210037,
57.7320452627451));
#140899=CARTESIAN_POINT('Ctrl Pts',(98.3215409859264,-9.34403834396314,
57.8083759256478));
#140900=CARTESIAN_POINT('Ctrl Pts',(98.3064659623698,-9.52768824794068,
57.8859298118043));
#140901=CARTESIAN_POINT('Ctrl Pts',(98.3001053609739,-9.60517561180472,
57.9186521060475));
#140902=CARTESIAN_POINT('Ctrl Pts',(98.293702309927,-9.68208699449254,57.9515927836448));
#140903=CARTESIAN_POINT('Ctrl Pts',(98.2872556496088,-9.75846110048999,
57.9847578103677));
#140904=CARTESIAN_POINT('',(98.1858622879398,-10.8854244761627,58.5063788330415));
#140905=CARTESIAN_POINT('Ctrl Pts',(98.287255431523,-9.75846368326178,57.9847589321044));
#140906=CARTESIAN_POINT('Ctrl Pts',(98.2752326904077,-9.90087388729895,
58.0466102646848));
#140907=CARTESIAN_POINT('Ctrl Pts',(98.2514522368865,-10.1736221482937,
58.1689494817128));
#140908=CARTESIAN_POINT('Ctrl Pts',(98.2176663389691,-10.54488259149,58.34276199094));
#140909=CARTESIAN_POINT('Ctrl Pts',(98.1962080794691,-10.77506402066,58.45315461531));
#140910=CARTESIAN_POINT('Ctrl Pts',(98.1858622898691,-10.88542445529,58.50637882297));
#140911=CARTESIAN_POINT('',(98.1061703786691,-11.63926799201,58.91635611737));
#140912=CARTESIAN_POINT('Ctrl Pts',(98.1858622879714,-10.8854244761627,
58.5063788330476));
#140913=CARTESIAN_POINT('Ctrl Pts',(98.1822193745813,-10.9242853208731,
58.5251199041985));
#140914=CARTESIAN_POINT('Ctrl Pts',(98.1785918743415,-10.9628736870434,
58.5437816819218));
#140915=CARTESIAN_POINT('Ctrl Pts',(98.1749505020994,-11.0013736886429,
58.5625148246342));
#140916=CARTESIAN_POINT('Ctrl Pts',(98.1749372589513,-11.0015137076219,
58.5625829543851));
#140917=CARTESIAN_POINT('Ctrl Pts',(98.1749240156201,-11.0016537254113,
58.5626510850778));
#140918=CARTESIAN_POINT('Ctrl Pts',(98.1749107721045,-11.0017937420141,
58.5627192167188));
#140919=CARTESIAN_POINT('Ctrl Pts',(98.1712560546698,-11.0404331137333,
58.5815210141535));
#140920=CARTESIAN_POINT('Ctrl Pts',(98.1675872573881,-11.0789841252467,
58.6003952458404));
#140921=CARTESIAN_POINT('Ctrl Pts',(98.1639481760854,-11.116772737625,58.6191166027382));
#140922=CARTESIAN_POINT('Ctrl Pts',(98.1639103076985,-11.1171659670351,
58.6193114177278));
#140923=CARTESIAN_POINT('Ctrl Pts',(98.1638724425624,-11.1175591133193,
58.6195062159939));
#140924=CARTESIAN_POINT('Ctrl Pts',(98.1638345806645,-11.1179521764361,
58.6197009976006));
#140925=CARTESIAN_POINT('Ctrl Pts',(98.1602339848412,-11.1553317452324,
58.6382243648567));
#140926=CARTESIAN_POINT('Ctrl Pts',(98.1566627809925,-11.1919582746467,
58.6565965241752));
#140927=CARTESIAN_POINT('Ctrl Pts',(98.1531490508319,-11.2272122368966,
58.6746730085577));
#140928=CARTESIAN_POINT('Ctrl Pts',(98.153061326564,-11.2280923921411,58.6751243085397));
#140929=CARTESIAN_POINT('Ctrl Pts',(98.1529736355007,-11.2289717013682,
58.6755754376997));
#140930=CARTESIAN_POINT('Ctrl Pts',(98.1528859765534,-11.2298501688127,
58.6760264016383));
#140931=CARTESIAN_POINT('Ctrl Pts',(98.1503402480423,-11.2553619926082,
58.6891229740981));
#140932=CARTESIAN_POINT('Ctrl Pts',(98.1478217144922,-11.2801692510307,
58.702079641213));
#140933=CARTESIAN_POINT('Ctrl Pts',(98.1452503468445,-11.3048609610118,
58.7153081150659));
#140934=CARTESIAN_POINT('Ctrl Pts',(98.1443264877432,-11.3137323726955,
58.7200609344367));
#140935=CARTESIAN_POINT('Ctrl Pts',(98.1433957829007,-11.3225883365942,
58.7248489719439));
#140936=CARTESIAN_POINT('Ctrl Pts',(98.1424543184985,-11.3314550087017,
58.7296923622527));
#140937=CARTESIAN_POINT('Ctrl Pts',(98.1423123309019,-11.3327922419092,
58.7304228214688));
#140938=CARTESIAN_POINT('Ctrl Pts',(98.1421701018987,-11.3341298086781,
58.731154522607));
#140939=CARTESIAN_POINT('Ctrl Pts',(98.1420276323736,-11.3354676606157,
58.7318874611152));
#140940=CARTESIAN_POINT('Ctrl Pts',(98.1397828557107,-11.3565471076515,
58.7434357782575));
#140941=CARTESIAN_POINT('Ctrl Pts',(98.1374784063472,-11.3776920623505,
58.7552910832167));
#140942=CARTESIAN_POINT('Ctrl Pts',(98.135115269475,-11.3988808424873,58.7674483078894));
#140943=CARTESIAN_POINT('Ctrl Pts',(98.1337707147605,-11.4109366292514,
58.7743654077578));
#140944=CARTESIAN_POINT('Ctrl Pts',(98.1324071370899,-11.4230079261992,
58.7813803717716));
#140945=CARTESIAN_POINT('Ctrl Pts',(98.1310252011188,-11.435094523445,58.7884897805351));
#140946=CARTESIAN_POINT('Ctrl Pts',(98.1308171645218,-11.4369140394091,
58.7895600307038));
#140947=CARTESIAN_POINT('Ctrl Pts',(98.1306087354596,-11.438733601095,58.7906322999199));
#140948=CARTESIAN_POINT('Ctrl Pts',(98.1303998967675,-11.4405534015101,
58.7917066764878));
#140949=CARTESIAN_POINT('Ctrl Pts',(98.1271948586614,-11.4684817974332,
58.8081950858267));
#140950=CARTESIAN_POINT('Ctrl Pts',(98.1238938833199,-11.496462789953,58.8251770470384));
#140951=CARTESIAN_POINT('Ctrl Pts',(98.1205589506922,-11.5240776285944,
58.8423337024545));
#140952=CARTESIAN_POINT('Ctrl Pts',(98.1199696640494,-11.5289572040972,
58.8453653042888));
#140953=CARTESIAN_POINT('Ctrl Pts',(98.1193793015924,-11.5338254501362,
58.8484024406795));
#140954=CARTESIAN_POINT('Ctrl Pts',(98.1187881861463,-11.538680182265,58.8514434508447));
#140955=CARTESIAN_POINT('Ctrl Pts',(98.1185110438627,-11.5409563054102,
58.852869217177));
#140956=CARTESIAN_POINT('Ctrl Pts',(98.1182337152748,-11.5432295396573,
58.8542959419573));
#140957=CARTESIAN_POINT('Ctrl Pts',(98.1179562112343,-11.5454998274262,
58.8557235693581));
#140958=CARTESIAN_POINT('Ctrl Pts',(98.1145024686386,-11.5737552342998,
58.8734914460235));
#140959=CARTESIAN_POINT('Ctrl Pts',(98.1110218674615,-11.6015576167855,
58.8913974974267));
#140960=CARTESIAN_POINT('Ctrl Pts',(98.1074882690966,-11.6290487900927,
58.9095761943874));
#140961=CARTESIAN_POINT('Ctrl Pts',(98.1070498095344,-11.6324599779435,
58.9118318620347));
#140962=CARTESIAN_POINT('Ctrl Pts',(98.106610530279,-11.6358663095293,58.9140917466174));
#140963=CARTESIAN_POINT('Ctrl Pts',(98.1061703789843,-11.63926799201,58.9163561174312));
#140964=CARTESIAN_POINT('',(97.4550855056363,-13.496463426129,62.2658808648332));
#140965=CARTESIAN_POINT('Ctrl Pts',(98.1061703781116,-11.63926799201,58.9163561172616));
#140966=CARTESIAN_POINT('Ctrl Pts',(98.0966576593874,-11.7127292568203,
58.9652945684228));
#140967=CARTESIAN_POINT('Ctrl Pts',(98.0867888698576,-11.7839934899085,
59.016064839334));
#140968=CARTESIAN_POINT('Ctrl Pts',(98.0765879384257,-11.8531333041328,
59.068543821195));
#140969=CARTESIAN_POINT('Ctrl Pts',(98.0662437675195,-11.9232439660403,
59.1217597026055));
#140970=CARTESIAN_POINT('Ctrl Pts',(98.0555579974791,-11.9911706438039,
59.176732947));
#140971=CARTESIAN_POINT('Ctrl Pts',(98.0445455451492,-12.0569745023016,
59.2333868161265));
#140972=CARTESIAN_POINT('Ctrl Pts',(98.0334164928612,-12.1234750927278,
59.2906405370001));
#140973=CARTESIAN_POINT('Ctrl Pts',(98.021953738878,-12.1878082086981,59.3496109954792));
#140974=CARTESIAN_POINT('Ctrl Pts',(98.0101634916104,-12.2500142572324,
59.4102662590643));
#140975=CARTESIAN_POINT('Ctrl Pts',(98.0003308970524,-12.301891613187,59.4608503224098));
#140976=CARTESIAN_POINT('Ctrl Pts',(97.9902703516646,-12.3522893588823,
59.5126070912772));
#140977=CARTESIAN_POINT('Ctrl Pts',(97.9799811312989,-12.4012149719552,
59.5655402787358));
#140978=CARTESIAN_POINT('Ctrl Pts',(97.9791397502712,-12.405215769017,59.5698687874157));
#140979=CARTESIAN_POINT('Ctrl Pts',(97.9782968381121,-12.4092067130191,
59.5742051729851));
#140980=CARTESIAN_POINT('Ctrl Pts',(97.9774523937125,-12.4131878324592,
59.5785494411326));
#140981=CARTESIAN_POINT('Ctrl Pts',(97.9642635778662,-12.4753662910788,
59.6463996780582));
#140982=CARTESIAN_POINT('Ctrl Pts',(97.9507110349178,-12.5351261696814,
59.7161210881153));
#140983=CARTESIAN_POINT('Ctrl Pts',(97.9367891102262,-12.5924643940136,
59.7877427208916));
#140984=CARTESIAN_POINT('Ctrl Pts',(97.9228467908142,-12.6498866151409,
59.8594692747337));
#140985=CARTESIAN_POINT('Ctrl Pts',(97.9085339122914,-12.7048802027885,
59.9331021117221));
#140986=CARTESIAN_POINT('Ctrl Pts',(97.8938417282283,-12.7573923544939,
60.0086863934301));
#140987=CARTESIAN_POINT('Ctrl Pts',(97.87921585619,-12.8096674967059,60.0839295313886));
#140988=CARTESIAN_POINT('Ctrl Pts',(97.8642140129851,-12.8594836321143,
60.1611070065553));
#140989=CARTESIAN_POINT('Ctrl Pts',(97.8488258520106,-12.9067380051098,
60.2402720326482));
#140990=CARTESIAN_POINT('Ctrl Pts',(97.8390598470948,-12.9367277121149,
60.2905136460074));
#140991=CARTESIAN_POINT('Ctrl Pts',(97.8291382141621,-12.965684591652,60.3415559413888));
#140992=CARTESIAN_POINT('Ctrl Pts',(97.8190581603176,-12.993571479285,60.3934130640865));
#140993=CARTESIAN_POINT('Ctrl Pts',(97.813338575709,-13.009394947666,60.4228376292132));
#140994=CARTESIAN_POINT('Ctrl Pts',(97.8075699015489,-13.0249019223777,
60.4525146740103));
#140995=CARTESIAN_POINT('Ctrl Pts',(97.8017575137646,-13.0400726694135,
60.4824165743383));
#140996=CARTESIAN_POINT('Ctrl Pts',(97.7893783643013,-13.0723831332008,
60.5461012607575));
#140997=CARTESIAN_POINT('Ctrl Pts',(97.7768006366382,-13.1031654309393,
60.6108074090894));
#140998=CARTESIAN_POINT('Ctrl Pts',(97.7640835268832,-13.1322806911523,
60.6762307023581));
#140999=CARTESIAN_POINT('Ctrl Pts',(97.7512575615967,-13.1616451712891,
60.7422140039539));
#141000=CARTESIAN_POINT('Ctrl Pts',(97.7382898944951,-13.1893137939528,
60.8089263874268));
#141001=CARTESIAN_POINT('Ctrl Pts',(97.7252453091653,-13.2151926323364,
60.8760346476848));
#141002=CARTESIAN_POINT('Ctrl Pts',(97.7121335901379,-13.2412046556442,
60.9434882792618));
#141003=CARTESIAN_POINT('Ctrl Pts',(97.6989442439426,-13.2654083480943,
61.011341438086));
#141004=CARTESIAN_POINT('Ctrl Pts',(97.6857459106975,-13.287758912407,61.0792409073627));
#141005=CARTESIAN_POINT('Ctrl Pts',(97.6724397736567,-13.3102920358071,
61.1476949785263));
#141006=CARTESIAN_POINT('Ctrl Pts',(97.6591245885233,-13.3309415965499,
61.2161956772425));
#141007=CARTESIAN_POINT('Ctrl Pts',(97.6458722845238,-13.3497138986142,
61.2843726625986));
#141008=CARTESIAN_POINT('Ctrl Pts',(97.6428236518917,-13.3540323818497,
61.3000564699068));
#141009=CARTESIAN_POINT('Ctrl Pts',(97.6397783505005,-13.3582517361044,
61.3157231270329));
#141010=CARTESIAN_POINT('Ctrl Pts',(97.6367372604432,-13.3623724257183,
61.3313681010267));
#141011=CARTESIAN_POINT('Ctrl Pts',(97.62311532789,-13.3808302007058,61.4014465191353));
#141012=CARTESIAN_POINT('Ctrl Pts',(97.6095678838933,-13.3971449365558,
61.4711414460592));
#141013=CARTESIAN_POINT('Ctrl Pts',(97.5960759980443,-13.4115039866449,
61.540550717809));
#141014=CARTESIAN_POINT('Ctrl Pts',(97.5826014167824,-13.4258446199289,
61.6098709657708));
#141015=CARTESIAN_POINT('Ctrl Pts',(97.5691821716715,-13.43823474134,61.6789066596063));
#141016=CARTESIAN_POINT('Ctrl Pts',(97.5557971529493,-13.4488343816429,
61.7477663459257));
#141017=CARTESIAN_POINT('Ctrl Pts',(97.5422439188024,-13.4595672322934,
61.8174914222474));
#141018=CARTESIAN_POINT('Ctrl Pts',(97.5287256767822,-13.4684643880439,
61.8870365323244));
#141019=CARTESIAN_POINT('Ctrl Pts',(97.515216014868,-13.4756434557848,61.9565374549115));
#141020=CARTESIAN_POINT('Ctrl Pts',(97.5015833205085,-13.4828879032713,
62.0266713221648));
#141021=CARTESIAN_POINT('Ctrl Pts',(97.4879592676874,-13.4883829249004,
62.0967606847404));
#141022=CARTESIAN_POINT('Ctrl Pts',(97.4743136522677,-13.4921990177858,
62.1669609501112));
#141023=CARTESIAN_POINT('Ctrl Pts',(97.4679101303506,-13.4939898079903,
62.1999040548421));
#141024=CARTESIAN_POINT('Ctrl Pts',(97.4615018253202,-13.4954101432466,
62.2328717624063));
#141025=CARTESIAN_POINT('Ctrl Pts',(97.4550854749278,-13.4964634261277,
62.2658808588604));
#141026=CARTESIAN_POINT('',(97.4550855974691,-13.49646342613,62.26588088268));
#141027=CARTESIAN_POINT('Origin',(98.9275259828691,-15.39012394141,62.55209572828));
#141028=CARTESIAN_POINT('',(97.4408144041081,-13.4984402470751,62.3529940555964));
#141029=CARTESIAN_POINT('Origin',(98.6415803004823,-11.8684041259695,62.3485284784612));
#141030=CARTESIAN_POINT('Ctrl Pts',(97.4408111863691,-13.49844024719,62.35299362778));
#141031=CARTESIAN_POINT('Ctrl Pts',(97.4173636613705,-13.4950477422291,
62.527984492391));
#141032=CARTESIAN_POINT('Ctrl Pts',(97.4236570627935,-13.4751288891508,
62.7187077839406));
#141033=CARTESIAN_POINT('Ctrl Pts',(97.4949557198421,-13.420461087357,63.0077137348997));
#141034=CARTESIAN_POINT('Ctrl Pts',(97.5289803287109,-13.3981068997297,
63.1043922603008));
#141035=CARTESIAN_POINT('Ctrl Pts',(97.5966941058591,-13.3583782377447,
63.2460891480223));
#141036=CARTESIAN_POINT('Ctrl Pts',(97.6220365677761,-13.3441024536591,
63.2927595285971));
#141037=CARTESIAN_POINT('Ctrl Pts',(97.664279676,-13.3211394323945,63.3613732688597));
#141038=CARTESIAN_POINT('Ctrl Pts',(97.6864575470268,-13.3092705854783,
63.3953315107788));
#141039=CARTESIAN_POINT('Ctrl Pts',(97.7102234673853,-13.296820734136,63.4286582671533));
#141040=CARTESIAN_POINT('Ctrl Pts',(97.7264199637094,-13.2883917211465,
63.4507233650114));
#141041=CARTESIAN_POINT('Ctrl Pts',(97.7358935390684,-13.2834963577579,
63.4632223753341));
#141042=CARTESIAN_POINT('Ctrl Pts',(97.8011573536291,-13.249950498071,63.547199335367));
#141043=CARTESIAN_POINT('Ctrl Pts',(97.8662462666935,-13.2196202737384,
63.616343275454));
#141044=CARTESIAN_POINT('Ctrl Pts',(97.9727587025035,-13.1733574136564,
63.7099617869203));
#141045=CARTESIAN_POINT('Ctrl Pts',(98.009738986224,-13.1578085396986,63.7394884174016));
#141046=CARTESIAN_POINT('Ctrl Pts',(98.0671760684826,-13.1342933478661,
63.7810613979237));
#141047=CARTESIAN_POINT('Ctrl Pts',(98.0963859781652,-13.1224877817258,
63.8011690100459));
#141048=CARTESIAN_POINT('Ctrl Pts',(98.1262839966426,-13.1106102602497,
63.8202246363938));
#141049=CARTESIAN_POINT('Ctrl Pts',(98.1463633209196,-13.1026759225243,
63.8326911146773));
#141050=CARTESIAN_POINT('Ctrl Pts',(98.1579299503343,-13.0981323525652,
63.8396610984129));
#141051=CARTESIAN_POINT('Ctrl Pts',(98.3063545768017,-13.0400815536355,
63.927021476433));
#141052=CARTESIAN_POINT('Ctrl Pts',(98.466686355582,-12.9953063983198,63.9905955773411));
#141053=CARTESIAN_POINT('Ctrl Pts',(98.6413367350691,-12.96039213374,64.024539984441));
#141054=CARTESIAN_POINT('Ctrl Pts',(95.3600739029692,-14.83896505265,61.68126243292));
#141055=CARTESIAN_POINT('Ctrl Pts',(95.3488967629692,-14.83942460114,61.7270366935901));
#141056=CARTESIAN_POINT('Ctrl Pts',(95.2537938103691,-14.84221155252,62.15207107076));
#141057=CARTESIAN_POINT('Ctrl Pts',(95.2173222593691,-14.82409468882,63.006826791351));
#141058=CARTESIAN_POINT('Ctrl Pts',(95.5518922378691,-14.73065279882,64.161325047946));
#141059=CARTESIAN_POINT('Ctrl Pts',(96.2081398692692,-14.58918963245,65.112261313913));
#141060=CARTESIAN_POINT('Ctrl Pts',(97.039871915969,-14.44338212505,65.761701368215));
#141061=CARTESIAN_POINT('Ctrl Pts',(97.8878639618691,-14.33215462512,66.111820330221));
#141062=CARTESIAN_POINT('Ctrl Pts',(98.4384132164691,-14.28651698832,66.202335719855));
#141063=CARTESIAN_POINT('Ctrl Pts',(98.6904498008691,-14.27205827794,66.217885926039));
#141064=CARTESIAN_POINT('Ctrl Pts',(96.6132510546691,-15.48406398727,61.9746008524));
#141065=CARTESIAN_POINT('Ctrl Pts',(96.605261792769,-15.48455020164,62.00674475245));
#141066=CARTESIAN_POINT('Ctrl Pts',(96.5374119126691,-15.48745755549,62.30580352411));
#141067=CARTESIAN_POINT('Ctrl Pts',(96.5166513377691,-15.46857722262,62.91670103595));
#141068=CARTESIAN_POINT('Ctrl Pts',(96.7844491779691,-15.3710316785,63.73087440493));
#141069=CARTESIAN_POINT('Ctrl Pts',(97.2789917563691,-15.22554231463,64.359787283689));
#141070=CARTESIAN_POINT('Ctrl Pts',(97.8582212558691,-15.079599962,64.7398975319179));
#141071=CARTESIAN_POINT('Ctrl Pts',(98.3940856313691,-14.97191574057,64.908401892465));
#141072=CARTESIAN_POINT('Ctrl Pts',(98.7117257326691,-14.92907221933,64.938374720735));
#141073=CARTESIAN_POINT('Ctrl Pts',(98.8530540086691,-14.91555874585,64.9403245206161));
#141074=CARTESIAN_POINT('Ctrl Pts',(97.7223056686691,-14.60855129545,62.25049179));
#141075=CARTESIAN_POINT('Ctrl Pts',(97.7180946320691,-14.60900131952,62.26739880163));
#141076=CARTESIAN_POINT('Ctrl Pts',(97.6823397918691,-14.61174526606,62.4247344993));
#141077=CARTESIAN_POINT('Ctrl Pts',(97.6717261099691,-14.5939010951,62.74672635053));
#141078=CARTESIAN_POINT('Ctrl Pts',(97.8146542530691,-14.50192493123,63.1751821767));
#141079=CARTESIAN_POINT('Ctrl Pts',(98.076899205869,-14.36189982535,63.503526109119));
#141080=CARTESIAN_POINT('Ctrl Pts',(98.3812567346691,-14.21614048141,63.698666180833));
#141081=CARTESIAN_POINT('Ctrl Pts',(98.6593498648691,-14.10364740799,63.782416805214));
#141082=CARTESIAN_POINT('Ctrl Pts',(98.8220717947691,-14.05701178061,63.7960633438949));
#141083=CARTESIAN_POINT('Ctrl Pts',(98.8941584479691,-14.04221545444,63.7965231491));
#141084=CARTESIAN_POINT('Ctrl Pts',(97.438659219569,-13.19808298716,62.19833602395));
#141085=CARTESIAN_POINT('Ctrl Pts',(97.4345632129691,-13.19847470795,62.21555337483));
#141086=CARTESIAN_POINT('Ctrl Pts',(97.3996126441691,-13.20095540206,62.37497098533));
#141087=CARTESIAN_POINT('Ctrl Pts',(97.3821583556691,-13.1847805085,62.68826097786));
#141088=CARTESIAN_POINT('Ctrl Pts',(97.4826980927691,-13.10177672665,63.119849099336));
#141089=CARTESIAN_POINT('Ctrl Pts',(97.7035745284691,-12.97055464874,63.507460358022));
#141090=CARTESIAN_POINT('Ctrl Pts',(98.0201427273691,-12.82509013543,63.810230114874));
#141091=CARTESIAN_POINT('Ctrl Pts',(98.3850210303692,-12.7048499061,64.001503994499));
#141092=CARTESIAN_POINT('Ctrl Pts',(98.6452233244691,-12.65210512052,64.06142072345));
#141093=CARTESIAN_POINT('Ctrl Pts',(98.7674875616692,-12.63524209323,64.074178388114));
#141094=CARTESIAN_POINT('',(98.4192415713824,-14.4018367539862,65.9071444853374));
#141095=CARTESIAN_POINT('Origin',(98.3551473045331,-12.9603609055107,65.4970333128763));
#141096=CARTESIAN_POINT('',(95.9574099869533,-14.9983144997034,62.1685143007228));
#141097=CARTESIAN_POINT('Ctrl Pts',(95.9574099809601,-14.998310267243,62.1685142604261));
#141098=CARTESIAN_POINT('Ctrl Pts',(96.0012696150027,-14.9981600557221,
62.1743656086402));
#141099=CARTESIAN_POINT('Ctrl Pts',(96.045922325758,-14.9960467811955,62.1803077696328));
#141100=CARTESIAN_POINT('Ctrl Pts',(96.0911271820895,-14.9917723025715,
62.1863059731721));
#141101=CARTESIAN_POINT('Ctrl Pts',(96.1336142904867,-14.9877548086256,
62.1919435604722));
#141102=CARTESIAN_POINT('Ctrl Pts',(96.1765884876485,-14.9818276967302,
62.1976305608909));
#141103=CARTESIAN_POINT('Ctrl Pts',(96.2198092128224,-14.9738563958951,
62.203332991161));
#141104=CARTESIAN_POINT('Ctrl Pts',(96.262472893195,-14.9659878321537,62.2089619263863));
#141105=CARTESIAN_POINT('Ctrl Pts',(96.3053763103589,-14.9561268512073,
62.2146058264365));
#141106=CARTESIAN_POINT('Ctrl Pts',(96.3482551438108,-14.944182080057,62.2202279883614));
#141107=CARTESIAN_POINT('Ctrl Pts',(96.3904901203016,-14.9324166683583,
62.2257657294241));
#141108=CARTESIAN_POINT('Ctrl Pts',(96.432700618763,-14.9186291541119,62.2312822920534));
#141109=CARTESIAN_POINT('Ctrl Pts',(96.4746100837264,-14.9027767896463,
62.2367398532758));
#141110=CARTESIAN_POINT('Ctrl Pts',(96.4846316619751,-14.8989861015271,
62.2380448896651));
#141111=CARTESIAN_POINT('Ctrl Pts',(96.4946359428567,-14.895077562312,62.2393465433086));
#141112=CARTESIAN_POINT('Ctrl Pts',(96.5046190037531,-14.8910510095824,
62.2406442824845));
#141113=CARTESIAN_POINT('Ctrl Pts',(96.5457967195746,-14.8744424517706,
62.2459971432502));
#141114=CARTESIAN_POINT('Ctrl Pts',(96.5866136873752,-14.8558221045463,
62.2512833241223));
#141115=CARTESIAN_POINT('Ctrl Pts',(96.6267891696673,-14.8352101723846,
62.256465459109));
#141116=CARTESIAN_POINT('Ctrl Pts',(96.6665575653341,-14.8148070950125,
62.26159508501));
#141117=CARTESIAN_POINT('Ctrl Pts',(96.7056966429397,-14.7924525602942,
62.2666226596332));
#141118=CARTESIAN_POINT('Ctrl Pts',(96.7439344194183,-14.768217200915,62.2715124359294));
#141119=CARTESIAN_POINT('Ctrl Pts',(96.7819897340631,-14.7440974870707,
62.2763788793431));
#141120=CARTESIAN_POINT('Ctrl Pts',(96.8191515649532,-14.7181149926537,
62.2811087349992));
#141121=CARTESIAN_POINT('Ctrl Pts',(96.8551635552591,-14.6903894065228,
62.2856687884924));
#141122=CARTESIAN_POINT('Ctrl Pts',(96.8910568242675,-14.6627552237698,
62.2902138087853));
#141123=CARTESIAN_POINT('Ctrl Pts',(96.9258071117811,-14.633389754186,62.2945900522334));
#141124=CARTESIAN_POINT('Ctrl Pts',(96.9591833549712,-14.6024578646699,
62.2987681021177));
#141125=CARTESIAN_POINT('Ctrl Pts',(96.9755304033134,-14.5873080142103,
62.3008144313898));
#141126=CARTESIAN_POINT('Ctrl Pts',(96.9915482527109,-14.5717830782717,
62.3028132785694));
#141127=CARTESIAN_POINT('Ctrl Pts',(97.00721250667,-14.555906054082,62.3047615892805));
#141128=CARTESIAN_POINT('Ctrl Pts',(97.0391864667746,-14.5234977862291,
62.3087384916667));
#141129=CARTESIAN_POINT('Ctrl Pts',(97.0696845088655,-14.4896205716953,
62.3125045103739));
#141130=CARTESIAN_POINT('Ctrl Pts',(97.0985277703137,-14.4544960363077,
62.3160376868357));
#141131=CARTESIAN_POINT('Ctrl Pts',(97.127520425927,-14.4191895727894,62.3195891634454));
#141132=CARTESIAN_POINT('Ctrl Pts',(97.1548406995405,-14.3826235179928,
62.3229053300049));
#141133=CARTESIAN_POINT('Ctrl Pts',(97.1803516998964,-14.3450501607815,
62.3259701517649));
#141134=CARTESIAN_POINT('Ctrl Pts',(97.2059642027226,-14.3073273077244,
62.3290471677539));
#141135=CARTESIAN_POINT('Ctrl Pts',(97.2297527999203,-14.2685898948594,
62.3318708142175));
#141136=CARTESIAN_POINT('Ctrl Pts',(97.251628667622,-14.2291095152601,62.3344316956302));
#141137=CARTESIAN_POINT('Ctrl Pts',(97.2737184624237,-14.1892430516328,
62.3370176202522));
#141138=CARTESIAN_POINT('Ctrl Pts',(97.2938578932226,-14.1486198206857,
62.3393356171633));
#141139=CARTESIAN_POINT('Ctrl Pts',(97.3120080591549,-14.1075240544886,
62.3413831196368));
#141140=CARTESIAN_POINT('Ctrl Pts',(97.3206890515527,-14.0878684747397,
62.3423624139018));
#141141=CARTESIAN_POINT('Ctrl Pts',(97.3289157554256,-14.0681047891605,
62.3432799340599));
#141142=CARTESIAN_POINT('Ctrl Pts',(97.3366880569937,-14.0482636570666,
62.344135952151));
#141143=CARTESIAN_POINT('Ctrl Pts',(97.3531769291343,-14.0061708628855,
62.3459519873024));
#141144=CARTESIAN_POINT('Ctrl Pts',(97.3676175655061,-13.963730686189,62.3474907783583));
#141145=CARTESIAN_POINT('Ctrl Pts',(97.3800460797385,-13.9212249218851,
62.3487600116083));
#141146=CARTESIAN_POINT('Ctrl Pts',(97.3927201547522,-13.8778793348564,
62.3500543221848));
#141147=CARTESIAN_POINT('Ctrl Pts',(97.4033021998725,-13.8344662432008,
62.3510683756366));
#141148=CARTESIAN_POINT('Ctrl Pts',(97.4118785175442,-13.7912598252116,
62.3518165265851));
#141149=CARTESIAN_POINT('Ctrl Pts',(97.420562430531,-13.7475113554538,62.3525740635592));
#141150=CARTESIAN_POINT('Ctrl Pts',(97.4271905740984,-13.7039753017101,
62.3530590688327));
#141151=CARTESIAN_POINT('Ctrl Pts',(97.4318936058219,-13.6609018927404,
62.3532916397747));
#141152=CARTESIAN_POINT('Ctrl Pts',(97.4366956008386,-13.6169221138694,
62.3535291045783));
#141153=CARTESIAN_POINT('Ctrl Pts',(97.4394912825679,-13.5734250601916,
62.3535034923263));
#141154=CARTESIAN_POINT('Ctrl Pts',(97.4404525837326,-13.5306342066661,
62.3532402240524));
#141155=CARTESIAN_POINT('Ctrl Pts',(97.4406946885919,-13.5198572785274,
62.3531739196196));
#141156=CARTESIAN_POINT('Ctrl Pts',(97.4408205713521,-13.5091249202389,
62.3530925565016));
#141157=CARTESIAN_POINT('Ctrl Pts',(97.4408332182749,-13.4984402468452,
62.3529965689936));
#141158=CARTESIAN_POINT('Ctrl Pts',(95.9574099789773,-14.9983102672498,
62.1685142601616));
#141159=CARTESIAN_POINT('Ctrl Pts',(95.9514096344211,-14.9977629302669,
62.2247096010251));
#141160=CARTESIAN_POINT('Ctrl Pts',(95.9470290608532,-14.9969313978935,
62.2791925737174));
#141161=CARTESIAN_POINT('Ctrl Pts',(95.9439607817034,-14.9958717399714,
62.3318365274954));
#141162=CARTESIAN_POINT('Ctrl Pts',(95.94075500107,-14.9947645946698,62.3868396609303));
#141163=CARTESIAN_POINT('Ctrl Pts',(95.9389816069068,-14.9934084729966,
62.439835565818));
#141164=CARTESIAN_POINT('Ctrl Pts',(95.9383155634341,-14.9918643947086,
62.4907304568309));
#141165=CARTESIAN_POINT('Ctrl Pts',(95.9381103916246,-14.9913887480739,
62.5064084077641));
#141166=CARTESIAN_POINT('Ctrl Pts',(95.9380104850422,-14.990895242425,62.521887319159));
#141167=CARTESIAN_POINT('Ctrl Pts',(95.9380068387977,-14.9903855965846,
62.5371652841353));
#141168=CARTESIAN_POINT('Ctrl Pts',(95.9379943682758,-14.9886425566529,
62.5894174579373));
#141169=CARTESIAN_POINT('Ctrl Pts',(95.9391054646362,-14.9867110841805,
62.6393159758539));
#141170=CARTESIAN_POINT('Ctrl Pts',(95.9410004067022,-14.9846569562105,
62.6868137064653));
#141171=CARTESIAN_POINT('Ctrl Pts',(95.9411425522047,-14.9845028696779,
62.6903766590784));
#141172=CARTESIAN_POINT('Ctrl Pts',(95.9412891231093,-14.9843480907103,
62.6939261214091));
#141173=CARTESIAN_POINT('Ctrl Pts',(95.9414399831782,-14.984192645958,62.6974620824213));
#141174=CARTESIAN_POINT('Ctrl Pts',(95.9425209711992,-14.983078806382,62.722799015682));
#141175=CARTESIAN_POINT('Ctrl Pts',(95.943821969844,-14.9819308181225,62.7474425085392));
#141176=CARTESIAN_POINT('Ctrl Pts',(95.9452943492417,-14.9807582395695,
62.771390098375));
#141177=CARTESIAN_POINT('Ctrl Pts',(95.9462186984745,-14.9800221031582,
62.7864242236333));
#141178=CARTESIAN_POINT('Ctrl Pts',(95.9472415248629,-14.9792519192772,
62.8016628127833));
#141179=CARTESIAN_POINT('Ctrl Pts',(95.9482960543119,-14.9784952260472,
62.8162039813757));
#141180=CARTESIAN_POINT('Ctrl Pts',(95.9489212660038,-14.9780465961345,
62.824825180743));
#141181=CARTESIAN_POINT('Ctrl Pts',(95.9495565466789,-14.9776029280011,
62.8332013115559));
#141182=CARTESIAN_POINT('Ctrl Pts',(95.9501796139764,-14.9771758460696,
62.8411452441104));
#141183=CARTESIAN_POINT('Ctrl Pts',(95.9524166031059,-14.9756425002467,
62.8696662254577));
#141184=CARTESIAN_POINT('Ctrl Pts',(95.9550153969764,-14.9739649344671,
62.8993025836247));
#141185=CARTESIAN_POINT('Ctrl Pts',(95.9580817994832,-14.972120655243,62.9300357303402));
#141186=CARTESIAN_POINT('Ctrl Pts',(95.9627412086753,-14.9693182665968,
62.976734852844));
#141187=CARTESIAN_POINT('Ctrl Pts',(95.968479815432,-14.9661307753707,63.0259682427745));
#141188=CARTESIAN_POINT('Ctrl Pts',(95.9756655139945,-14.9624862295701,
63.077650834127));
#141189=CARTESIAN_POINT('Ctrl Pts',(95.977905960307,-14.9613498878312,63.0937650741281));
#141190=CARTESIAN_POINT('Ctrl Pts',(95.9802872866223,-14.9601690919896,
63.1101170981702));
#141191=CARTESIAN_POINT('Ctrl Pts',(95.9828211744858,-14.9589416115939,
63.1267034101123));
#141192=CARTESIAN_POINT('Ctrl Pts',(95.990825716738,-14.95506400563,63.1790995072962));
#141193=CARTESIAN_POINT('Ctrl Pts',(96.0003510877725,-14.9507205586402,
63.2338378254576));
#141194=CARTESIAN_POINT('Ctrl Pts',(96.0117803923567,-14.945840314384,63.2907734730001));
#141195=CARTESIAN_POINT('Ctrl Pts',(96.0174950446489,-14.9434001922559,
63.3192412967713));
#141196=CARTESIAN_POINT('Ctrl Pts',(96.0236860222231,-14.9408258612085,
63.3482575912512));
#141197=CARTESIAN_POINT('Ctrl Pts',(96.0304031093579,-14.9381084849442,
63.3777984390504));
#141198=CARTESIAN_POINT('Ctrl Pts',(96.0337616529253,-14.936749796812,63.39256886295));
#141199=CARTESIAN_POINT('Ctrl Pts',(96.0372517238174,-14.935355342873,63.4074704247759));
#141200=CARTESIAN_POINT('Ctrl Pts',(96.0408796711626,-14.9339240340903,
63.4224996477211));
#141201=CARTESIAN_POINT('Ctrl Pts',(96.0426936448352,-14.9332083796989,
63.4300142591937));
#141202=CARTESIAN_POINT('Ctrl Pts',(96.0445420876175,-14.9324835113438,
63.4375607859244));
#141203=CARTESIAN_POINT('Ctrl Pts',(96.0464257961909,-14.9317492929014,
63.4451387756133));
#141204=CARTESIAN_POINT('Ctrl Pts',(96.0478696280205,-14.9311865264672,
63.450947180837));
#141205=CARTESIAN_POINT('Ctrl Pts',(96.0495783943475,-14.9305236394949,
63.4577406841441));
#141206=CARTESIAN_POINT('Ctrl Pts',(96.0509917948209,-14.9299779874319,
63.4632961350523));
#141207=CARTESIAN_POINT('Ctrl Pts',(96.0514224003701,-14.9298117494756,
63.4649886546417));
#141208=CARTESIAN_POINT('Ctrl Pts',(96.0518252088932,-14.9296564667047,
63.4665663717365));
#141209=CARTESIAN_POINT('Ctrl Pts',(96.0521835178952,-14.929518450927,63.4679666720874));
#141210=CARTESIAN_POINT('Ctrl Pts',(96.0691237899622,-14.922993287423,63.5341706155741));
#141211=CARTESIAN_POINT('Ctrl Pts',(96.0881777231867,-14.9159073862417,
63.601199258289));
#141212=CARTESIAN_POINT('Ctrl Pts',(96.109570791596,-14.9082293103102,63.668841239143));
#141213=CARTESIAN_POINT('Ctrl Pts',(96.1302222508339,-14.9008174015045,
63.7341383523783));
#141214=CARTESIAN_POINT('Ctrl Pts',(96.1530535583824,-14.8928536236557,
63.8000071753183));
#141215=CARTESIAN_POINT('Ctrl Pts',(96.1782714395541,-14.8843122721267,
63.8662087137561));
#141216=CARTESIAN_POINT('Ctrl Pts',(96.1830084378664,-14.8827078404338,
63.8786441984709));
#141217=CARTESIAN_POINT('Ctrl Pts',(96.1878296557326,-14.8810830375917,
63.8910912759394));
#141218=CARTESIAN_POINT('Ctrl Pts',(96.1927364758324,-14.8794377055759,
63.9035481533974));
#141219=CARTESIAN_POINT('Ctrl Pts',(96.2200589510483,-14.8702760607002,
63.9729113496606));
#141220=CARTESIAN_POINT('Ctrl Pts',(96.2500368149232,-14.8604768525931,
64.0425820309446));
#141221=CARTESIAN_POINT('Ctrl Pts',(96.2828300686085,-14.8500536955576,
64.1123257811251));
#141222=CARTESIAN_POINT('Ctrl Pts',(96.3142549584493,-14.8400654655157,
64.1791593343775));
#141223=CARTESIAN_POINT('Ctrl Pts',(96.3482652772853,-14.8295042523752,
64.2460600637489));
#141224=CARTESIAN_POINT('Ctrl Pts',(96.3849873652349,-14.8183938641851,
64.3127789400618));
#141225=CARTESIAN_POINT('Ctrl Pts',(96.4209821229657,-14.807503532139,64.378176359518));
#141226=CARTESIAN_POINT('Ctrl Pts',(96.4595824246679,-14.7960855115134,
64.4433992698679));
#141227=CARTESIAN_POINT('Ctrl Pts',(96.5008913544073,-14.7841744147628,
64.5081688476521));
#141228=CARTESIAN_POINT('Ctrl Pts',(96.5166722132981,-14.7796241313678,
64.5329121555488));
#141229=CARTESIAN_POINT('Ctrl Pts',(96.5328481906253,-14.7750020211855,
64.5575888206246));
#141230=CARTESIAN_POINT('Ctrl Pts',(96.5494243368809,-14.7703105239057,
64.5821814293567));
#141231=CARTESIAN_POINT('Ctrl Pts',(96.5577124100088,-14.7679647752658,
64.5944777337228));
#141232=CARTESIAN_POINT('Ctrl Pts',(96.566100525408,-14.7656016812886,64.6067530242521));
#141233=CARTESIAN_POINT('Ctrl Pts',(96.5745892679672,-14.7632215783835,
64.6190050019048));
#141234=CARTESIAN_POINT('Ctrl Pts',(96.5788336392468,-14.7620315269309,
64.6251309907311));
#141235=CARTESIAN_POINT('Ctrl Pts',(96.583103167319,-14.7608372233412,64.6312511513545));
#141236=CARTESIAN_POINT('Ctrl Pts',(96.5873979238826,-14.7596387109044,
64.6373651927919));
#141237=CARTESIAN_POINT('Ctrl Pts',(96.5895453021644,-14.759039454686,64.6404222135105));
#141238=CARTESIAN_POINT('Ctrl Pts',(96.5916989875691,-14.7584391462613,
64.6434777044337));
#141239=CARTESIAN_POINT('Ctrl Pts',(96.5938589888889,-14.7578377911593,
64.6465316287433));
#141240=CARTESIAN_POINT('Ctrl Pts',(96.5958381016573,-14.757286796329,64.6493298032349));
#141241=CARTESIAN_POINT('Ctrl Pts',(96.5987682376394,-14.7564721479833,
64.6534559247871));
#141242=CARTESIAN_POINT('Ctrl Pts',(96.6000499109288,-14.756116149547,64.6552560745118));
#141243=CARTESIAN_POINT('Ctrl Pts',(96.6001670543419,-14.7560836117137,
64.655420606054));
#141244=CARTESIAN_POINT('Ctrl Pts',(96.6002703991504,-14.7560549081226,
64.6555657297191));
#141245=CARTESIAN_POINT('Ctrl Pts',(96.6003579493328,-14.7560305913982,
64.6556886648793));
#141246=CARTESIAN_POINT('Ctrl Pts',(96.6173725778219,-14.751304844188,64.6795800608916));
#141247=CARTESIAN_POINT('Ctrl Pts',(96.6362979304481,-14.7460791896076,
64.7055873977613));
#141248=CARTESIAN_POINT('Ctrl Pts',(96.657330736075,-14.7403386778775,64.7335281250405));
#141249=CARTESIAN_POINT('Ctrl Pts',(96.663756580762,-14.7385848635051,64.742064445735));
#141250=CARTESIAN_POINT('Ctrl Pts',(96.6703793071634,-14.7367830111207,
64.7507809081317));
#141251=CARTESIAN_POINT('Ctrl Pts',(96.6772049534311,-14.7349327574401,
64.7596714255857));
#141252=CARTESIAN_POINT('Ctrl Pts',(96.7003374256768,-14.7286621509313,
64.7898018542933));
#141253=CARTESIAN_POINT('Ctrl Pts',(96.7257991469457,-14.7218349641208,
64.8219349205996));
#141254=CARTESIAN_POINT('Ctrl Pts',(96.7538385481015,-14.714442632941,64.8558164648191));
#141255=CARTESIAN_POINT('Ctrl Pts',(96.781397335869,-14.7071770110771,64.889117257557));
#141256=CARTESIAN_POINT('Ctrl Pts',(96.8114468393952,-14.6993651700304,
64.9241073165543));
#141257=CARTESIAN_POINT('Ctrl Pts',(96.8442357055063,-14.6910095669947,
64.9604980558787));
#141258=CARTESIAN_POINT('Ctrl Pts',(96.875624641371,-14.6830107088789,64.9953350819245));
#141259=CARTESIAN_POINT('Ctrl Pts',(96.9095246271991,-14.6745133307496,
65.03145575547));
#141260=CARTESIAN_POINT('Ctrl Pts',(96.9461565118213,-14.6655327595853,
65.0685618480512));
#141261=CARTESIAN_POINT('Ctrl Pts',(96.9817089216784,-14.6568168294584,
65.1045744918245));
#141262=CARTESIAN_POINT('Ctrl Pts',(97.0198351312783,-14.6476455649945,
65.1415154605205));
#141263=CARTESIAN_POINT('Ctrl Pts',(97.0607314266875,-14.6380485623792,
65.1790675346859));
#141264=CARTESIAN_POINT('Ctrl Pts',(97.0996415206312,-14.6289176552982,
65.2147958254501));
#141265=CARTESIAN_POINT('Ctrl Pts',(97.1410595728877,-14.6194012540219,
65.2510772824833));
#141266=CARTESIAN_POINT('Ctrl Pts',(97.1851428296347,-14.6095412396628,
65.287597215422));
#141267=CARTESIAN_POINT('Ctrl Pts',(97.2196328613478,-14.6018269228671,
65.3161698241211));
#141268=CARTESIAN_POINT('Ctrl Pts',(97.2557541868158,-14.5939025487894,
65.3448876692596));
#141269=CARTESIAN_POINT('Ctrl Pts',(97.2935742074652,-14.5857964285298,
65.3735807790044));
#141270=CARTESIAN_POINT('Ctrl Pts',(97.3062872473112,-14.5830715905185,
65.3832258463848));
#141271=CARTESIAN_POINT('Ctrl Pts',(97.319192159892,-14.5803262824039,65.3928679693906));
#141272=CARTESIAN_POINT('Ctrl Pts',(97.33229128162,-14.5775617856489,65.4025002359996));
#141273=CARTESIAN_POINT('Ctrl Pts',(97.3464079637588,-14.5745825384311,
65.4128807522524));
#141274=CARTESIAN_POINT('Ctrl Pts',(97.360750198253,-14.5715810050985,65.4232498158811));
#141275=CARTESIAN_POINT('Ctrl Pts',(97.3753212746219,-14.568558755652,65.4335994685519));
#141276=CARTESIAN_POINT('Ctrl Pts',(97.3893671939351,-14.5656454312828,
65.443576108757));
#141277=CARTESIAN_POINT('Ctrl Pts',(97.4036256790824,-14.5627128946341,
65.4535345687424));
#141278=CARTESIAN_POINT('Ctrl Pts',(97.4180996460052,-14.5597626309598,
65.4634676907597));
#141279=CARTESIAN_POINT('Ctrl Pts',(97.4253366294665,-14.5582874991226,
65.4684342517683));
#141280=CARTESIAN_POINT('Ctrl Pts',(97.4326274834083,-14.5568079365226,
65.473394478516));
#141281=CARTESIAN_POINT('Ctrl Pts',(97.4399725384888,-14.5553241507323,
65.4783474185003));
#141282=CARTESIAN_POINT('Ctrl Pts',(97.443645066029,-14.5545822578372,65.4808238884924));
#141283=CARTESIAN_POINT('Ctrl Pts',(97.4473311438567,-14.5538393092137,
65.4832985368107));
#141284=CARTESIAN_POINT('Ctrl Pts',(97.4510308137269,-14.5530953309797,
65.4857712454299));
#141285=CARTESIAN_POINT('Ctrl Pts',(97.454730483597,-14.5523513527457,65.4882439540491));
#141286=CARTESIAN_POINT('Ctrl Pts',(97.4594831837347,-14.551398281015,65.491403251175));
#141287=CARTESIAN_POINT('Ctrl Pts',(97.4621706409605,-14.5508603339509,
65.4931834338171));
#141288=CARTESIAN_POINT('Ctrl Pts',(97.5231372774435,-14.5386566706569,
65.5335679828131));
#141289=CARTESIAN_POINT('Ctrl Pts',(97.5838904468826,-14.5270214011671,
65.5705895517535));
#141290=CARTESIAN_POINT('Ctrl Pts',(97.6440811651151,-14.5159906565726,
65.6045419319516));
#141291=CARTESIAN_POINT('Ctrl Pts',(97.7050374390766,-14.5048196137732,
65.6389261468234));
#141292=CARTESIAN_POINT('Ctrl Pts',(97.7654169391016,-14.4942684085919,
65.6701626512717));
#141293=CARTESIAN_POINT('Ctrl Pts',(97.824906488088,-14.484354276746,65.6985487188738));
#141294=CARTESIAN_POINT('Ctrl Pts',(97.8856406114176,-14.4742327324329,
65.7275286482894));
#141295=CARTESIAN_POINT('Ctrl Pts',(97.9454472157503,-14.4647750504268,
65.7535377111398));
#141296=CARTESIAN_POINT('Ctrl Pts',(98.004043176135,-14.4559808830376,65.7768830527672));
#141297=CARTESIAN_POINT('Ctrl Pts',(98.0200331420063,-14.4535810855858,
65.7832536491944));
#141298=CARTESIAN_POINT('Ctrl Pts',(98.0359332350288,-14.4512305993524,
65.789425832096));
#141299=CARTESIAN_POINT('Ctrl Pts',(98.0517383197579,-14.4489292049126,
65.7954057135219));
#141300=CARTESIAN_POINT('Ctrl Pts',(98.1165405888195,-14.4394932806982,
65.8199237652603));
#141301=CARTESIAN_POINT('Ctrl Pts',(98.17974232874,-14.4308834625626,65.8412111725943));
#141302=CARTESIAN_POINT('Ctrl Pts',(98.2410749986541,-14.423052262834,65.8596960227291));
#141303=CARTESIAN_POINT('Ctrl Pts',(98.3024076685682,-14.4152210631054,
65.878180872864));
#141304=CARTESIAN_POINT('Ctrl Pts',(98.3618713705022,-14.4081682887106,
65.8938632586274));
#141305=CARTESIAN_POINT('Ctrl Pts',(98.4192415713824,-14.4018367539862,
65.9071444853374));
#141306=CARTESIAN_POINT('Ctrl Pts',(91.7279224053691,-15.00086655583,62.66821414647));
#141307=CARTESIAN_POINT('Ctrl Pts',(92.8206547514691,-15.00091548588,62.47811409076));
#141308=CARTESIAN_POINT('Ctrl Pts',(94.9571365614691,-15.00012240043,62.10622675894));
#141309=CARTESIAN_POINT('Ctrl Pts',(97.3520603458691,-14.99728767361,61.67409908363));
#141310=CARTESIAN_POINT('Ctrl Pts',(98.9140829208691,-14.9946683359,61.38022674646));
#141311=CARTESIAN_POINT('Ctrl Pts',(99.7424919119691,-14.99311894757,61.22079195603));
#141312=CARTESIAN_POINT('Ctrl Pts',(100.309755217069,-14.99193659845,61.10860712166));
#141313=CARTESIAN_POINT('Ctrl Pts',(100.617471098369,-14.99125877485,61.04648221514));
#141314=CARTESIAN_POINT('Ctrl Pts',(91.9040967972691,-15.00296392531,63.719058961888));
#141315=CARTESIAN_POINT('Ctrl Pts',(93.0606464640691,-15.0026956181,63.506039291405));
#141316=CARTESIAN_POINT('Ctrl Pts',(95.3224996923691,-15.0032813732,63.093090511071));
#141317=CARTESIAN_POINT('Ctrl Pts',(97.8588287799691,-15.00640433575,62.62496746378));
#141318=CARTESIAN_POINT('Ctrl Pts',(99.5138086795691,-15.00944466321,62.31213308663));
#141319=CARTESIAN_POINT('Ctrl Pts',(100.390785755669,-15.01129179849,62.14422141575));
#141320=CARTESIAN_POINT('Ctrl Pts',(100.993297194369,-15.01272721411,62.02642432059));
#141321=CARTESIAN_POINT('Ctrl Pts',(101.318242921569,-15.01358278139,61.96242696786));
#141322=CARTESIAN_POINT('Ctrl Pts',(92.2448361102691,-14.79056277436,65.751541377466));
#141323=CARTESIAN_POINT('Ctrl Pts',(93.5247227957691,-14.79469787263,65.492534702806));
#141324=CARTESIAN_POINT('Ctrl Pts',(96.0287721259691,-14.80601079336,64.996333659406));
#141325=CARTESIAN_POINT('Ctrl Pts',(98.8382499265691,-14.82557675296,64.452349667076));
#141326=CARTESIAN_POINT('Ctrl Pts',(100.673211451469,-14.84109633199,64.097462534948));
#141327=CARTESIAN_POINT('Ctrl Pts',(101.644481448969,-14.84982392585,63.909951340424));
#141328=CARTESIAN_POINT('Ctrl Pts',(102.315435468069,-14.8565128255,63.778640063626));
#141329=CARTESIAN_POINT('Ctrl Pts',(102.672968839569,-14.85993777441,63.710281289207));
#141330=CARTESIAN_POINT('Ctrl Pts',(92.8846953387691,-13.59339522536,69.569112430703));
#141331=CARTESIAN_POINT('Ctrl Pts',(94.3995479103691,-13.62144836123,69.235119209287));
#141332=CARTESIAN_POINT('Ctrl Pts',(97.3641245099691,-13.67740135474,68.599574225623));
#141333=CARTESIAN_POINT('Ctrl Pts',(100.691605655469,-13.74147687523,67.919598525714));
#141334=CARTESIAN_POINT('Ctrl Pts',(102.867637731469,-13.78402627843,67.484518318603));
#141335=CARTESIAN_POINT('Ctrl Pts',(104.018563150869,-13.80621016489,67.257624542188));
#141336=CARTESIAN_POINT('Ctrl Pts',(104.818068817069,-13.82296220245,67.099320059727));
#141337=CARTESIAN_POINT('Ctrl Pts',(105.237162052669,-13.82954337409,67.020632065286));
#141338=CARTESIAN_POINT('Ctrl Pts',(93.4372496265691,-11.36012668785,72.8749686356714));
#141339=CARTESIAN_POINT('Ctrl Pts',(95.1718643785691,-11.41712605373,72.5027022658309));
#141340=CARTESIAN_POINT('Ctrl Pts',(98.5659480545691,-11.5258471646,71.79092364103));
#141341=CARTESIAN_POINT('Ctrl Pts',(102.374754293569,-11.63978355673,71.024735995695));
#141342=CARTESIAN_POINT('Ctrl Pts',(104.865797163869,-11.71128588736,70.534131296002));
#141343=CARTESIAN_POINT('Ctrl Pts',(106.185002256269,-11.74808512595,70.277403513677));
#141344=CARTESIAN_POINT('Ctrl Pts',(107.098214269869,-11.77444776282,70.101421471233));
#141345=CARTESIAN_POINT('Ctrl Pts',(107.578337843769,-11.78460067693,70.010906079548));
#141346=CARTESIAN_POINT('Ctrl Pts',(93.8521515924691,-8.31376415398099,
75.380290328567));
#141347=CARTESIAN_POINT('Ctrl Pts',(95.7842091872691,-8.37610151927799,
74.996687936449));
#141348=CARTESIAN_POINT('Ctrl Pts',(99.5633456799691,-8.49649192700699,
74.256622113144));
#141349=CARTESIAN_POINT('Ctrl Pts',(103.803511293669,-8.62652182891199,
73.4457843508907));
#141350=CARTESIAN_POINT('Ctrl Pts',(106.574368779969,-8.70918767776199,
72.9222235420443));
#141351=CARTESIAN_POINT('Ctrl Pts',(108.046575455569,-8.75337472261899,
72.645850034118));
#141352=CARTESIAN_POINT('Ctrl Pts',(109.052811928669,-8.78167412688299,
72.4603562024988));
#141353=CARTESIAN_POINT('Ctrl Pts',(109.595630317769,-8.79651115761099,
72.3582991883668));
#141354=CARTESIAN_POINT('Ctrl Pts',(94.0472766649691,-6.14488949293299,
76.567167410547));
#141355=CARTESIAN_POINT('Ctrl Pts',(96.0854968862691,-6.19932125750799,
76.182430497497));
#141356=CARTESIAN_POINT('Ctrl Pts',(100.071511458569,-6.30590151645599,
75.436192057807));
#141357=CARTESIAN_POINT('Ctrl Pts',(104.544032724869,-6.42467485066199,
74.609669612437));
#141358=CARTESIAN_POINT('Ctrl Pts',(107.464659287669,-6.50123978999499,
74.073144793283));
#141359=CARTESIAN_POINT('Ctrl Pts',(109.020613207169,-6.54339816253699,
73.7885097201805));
#141360=CARTESIAN_POINT('Ctrl Pts',(110.072680416569,-6.56809626639499,
73.5995632553892));
#141361=CARTESIAN_POINT('Ctrl Pts',(110.653470670069,-6.58429622250299,
73.4915052896967));
#141362=CARTESIAN_POINT('Ctrl Pts',(94.1596433973691,-4.29694974983499,
77.257573104574));
#141363=CARTESIAN_POINT('Ctrl Pts',(96.2671293792691,-4.33699728402899,
76.872950615596));
#141364=CARTESIAN_POINT('Ctrl Pts',(100.388073242369,-4.41679216450099,
76.124486128563));
#141365=CARTESIAN_POINT('Ctrl Pts',(105.012816858869,-4.50905954903699,
75.289931616852));
#141366=CARTESIAN_POINT('Ctrl Pts',(108.030893246069,-4.56946366778099,
74.746434477664));
#141367=CARTESIAN_POINT('Ctrl Pts',(109.642849121469,-4.60376584696699,
74.45726477928));
#141368=CARTESIAN_POINT('Ctrl Pts',(110.721584350869,-4.62195018599999,
74.266525935187));
#141369=CARTESIAN_POINT('Ctrl Pts',(111.330637583069,-4.63685072441499,
74.154803592336));
#141370=CARTESIAN_POINT('Ctrl Pts',(94.2215314633691,-2.87401142301499,
77.640260609653));
#141371=CARTESIAN_POINT('Ctrl Pts',(96.3708143948691,-2.90124327492399,
77.25556064955));
#141372=CARTESIAN_POINT('Ctrl Pts',(100.573127343269,-2.95640194059799,
76.505561208076));
#141373=CARTESIAN_POINT('Ctrl Pts',(105.290085863569,-3.02238747552899,
75.666090425013));
#141374=CARTESIAN_POINT('Ctrl Pts',(108.366745098769,-3.06612832963899,
75.11841156241));
#141375=CARTESIAN_POINT('Ctrl Pts',(110.013387788769,-3.09171881003499,
74.826511058606));
#141376=CARTESIAN_POINT('Ctrl Pts',(111.106033315769,-3.10383313136499,
74.634769909069));
#141377=CARTESIAN_POINT('Ctrl Pts',(111.734449639069,-3.11622061397699,
74.520727967092));
#141378=CARTESIAN_POINT('Ctrl Pts',(94.2650345463691,-1.31031824892799,
77.910754859622));
#141379=CARTESIAN_POINT('Ctrl Pts',(96.4453247786691,-1.32158371898399,
77.525392447647));
#141380=CARTESIAN_POINT('Ctrl Pts',(100.707884176569,-1.34593412180199,
76.773013051733));
#141381=CARTESIAN_POINT('Ctrl Pts',(105.493651081669,-1.37849110683099,
75.928270717931));
#141382=CARTESIAN_POINT('Ctrl Pts',(108.613311575269,-1.40102659958799,
75.376389135756));
#141383=CARTESIAN_POINT('Ctrl Pts',(110.286981216069,-1.41501268170799,
75.081756321705));
#141384=CARTESIAN_POINT('Ctrl Pts',(111.386572784969,-1.42033729508099,
74.88908018054));
#141385=CARTESIAN_POINT('Ctrl Pts',(112.032792121069,-1.42836747710599,
74.772757830664));
#141386=CARTESIAN_POINT('Ctrl Pts',(94.2748040922691,-0.278275671875586,
77.974281587457));
#141387=CARTESIAN_POINT('Ctrl Pts',(96.4657713563691,-0.279825571159086,
77.588107109206));
#141388=CARTESIAN_POINT('Ctrl Pts',(100.748949641169,-0.283983060529886,
76.833828722269));
#141389=CARTESIAN_POINT('Ctrl Pts',(105.558826386669,-0.291328739675386,
75.986054822495));
#141390=CARTESIAN_POINT('Ctrl Pts',(108.692803760269,-0.296740586015386,
75.432041328266));
#141391=CARTESIAN_POINT('Ctrl Pts',(110.377140334169,-0.300757700117286,
75.135908202226));
#141392=CARTESIAN_POINT('Ctrl Pts',(111.475574778769,-0.300917836469986,
74.943110155442));
#141393=CARTESIAN_POINT('Ctrl Pts',(112.131539947869,-0.304306622775186,
74.825323634026));
#141394=CARTESIAN_POINT('Ctrl Pts',(94.2720112807691,0.226163356373814,
77.96047019643));
#141395=CARTESIAN_POINT('Ctrl Pts',(96.4654988279691,0.227634972375714,
77.573615266263));
#141396=CARTESIAN_POINT('Ctrl Pts',(100.753485332469,0.231339974406114,
76.818101757373));
#141397=CARTESIAN_POINT('Ctrl Pts',(105.569346130169,0.237025460465514,
75.969015910907));
#141398=CARTESIAN_POINT('Ctrl Pts',(108.706464376969,0.241496016631014,
75.414309396842));
#141399=CARTESIAN_POINT('Ctrl Pts',(110.394133361669,0.243542056646714,
75.117607997261));
#141400=CARTESIAN_POINT('Ctrl Pts',(111.490264022669,0.246460875082214,
74.925066840918));
#141401=CARTESIAN_POINT('Ctrl Pts',(112.150634911769,0.246228592821014,
74.806547696003));
#141402=CARTESIAN_POINT('',(91.9155434736732,-14.9991665202076,62.8752787211534));
#141403=CARTESIAN_POINT('Ctrl Pts',(95.9574100500792,-14.998343644201,62.1685145911545));
#141404=CARTESIAN_POINT('Ctrl Pts',(95.9452997971755,-14.9983495824529,
62.1707000739723));
#141405=CARTESIAN_POINT('Ctrl Pts',(95.8963891825556,-14.9983766962934,
62.1792257798343));
#141406=CARTESIAN_POINT('Ctrl Pts',(95.8106852915384,-14.9984234747686,
62.194055653576));
#141407=CARTESIAN_POINT('Ctrl Pts',(95.7734726089319,-14.9984437860115,
62.2004947939475));
#141408=CARTESIAN_POINT('Ctrl Pts',(95.7293234569771,-14.9984677764014,
62.2081217736258));
#141409=CARTESIAN_POINT('Ctrl Pts',(95.6782392676023,-14.9984951851695,
62.2169307774249));
#141410=CARTESIAN_POINT('Ctrl Pts',(95.5938716127534,-14.9985404518853,
62.2314792121007));
#141411=CARTESIAN_POINT('Ctrl Pts',(95.4905877629147,-14.9985950833701,
62.2492520642195));
#141412=CARTESIAN_POINT('Ctrl Pts',(95.368397778593,-14.9986573431981,62.2702154651726));
#141413=CARTESIAN_POINT('Ctrl Pts',(95.3073027864321,-14.9986884731122,
62.2806971656492));
#141414=CARTESIAN_POINT('Ctrl Pts',(95.241481260621,-14.9987214974988,62.2919765031988));
#141415=CARTESIAN_POINT('Ctrl Pts',(95.1709350275728,-14.9987561261751,
62.3040485648304));
#141416=CARTESIAN_POINT('Ctrl Pts',(95.1442556676702,-14.9987692221389,
62.3086140088394));
#141417=CARTESIAN_POINT('Ctrl Pts',(95.1169005706544,-14.9987825469947,
62.3132928296912));
#141418=CARTESIAN_POINT('Ctrl Pts',(95.0888698437195,-14.9987960828689,
62.3180847692762));
#141419=CARTESIAN_POINT('Ctrl Pts',(95.0798407948187,-14.9988004429438,
62.3196283131502));
#141420=CARTESIAN_POINT('Ctrl Pts',(95.0707416449853,-14.9988048249041,
62.321183593822));
#141421=CARTESIAN_POINT('Ctrl Pts',(95.0615723979527,-14.9988092281285,
62.3227506025527));
#141422=CARTESIAN_POINT('Ctrl Pts',(95.0427547880724,-14.9988182646565,
62.3259665000923));
#141423=CARTESIAN_POINT('Ctrl Pts',(95.0236419465857,-14.9988273907554,
62.3292317934443));
#141424=CARTESIAN_POINT('Ctrl Pts',(95.0042339067701,-14.9988366008968,
62.3325464059602));
#141425=CARTESIAN_POINT('Ctrl Pts',(94.9872518719314,-14.9988446597705,
62.3354466919116));
#141426=CARTESIAN_POINT('Ctrl Pts',(94.9700438258722,-14.9988527829859,
62.3383847378479));
#141427=CARTESIAN_POINT('Ctrl Pts',(94.9526097917505,-14.9988609666919,
62.3413604926689));
#141428=CARTESIAN_POINT('Ctrl Pts',(94.9501192154474,-14.9988621357928,
62.3417856005005));
#141429=CARTESIAN_POINT('Ctrl Pts',(94.946312537638,-14.9988639207714,62.3424353129184));
#141430=CARTESIAN_POINT('Ctrl Pts',(94.9451242269272,-14.9988644776858,
62.3426381247191));
#141431=CARTESIAN_POINT('Ctrl Pts',(94.7930204559396,-14.9989357627347,
62.3685980352097));
#141432=CARTESIAN_POINT('Ctrl Pts',(94.6327281907657,-14.99900408532,62.3961886287692));
#141433=CARTESIAN_POINT('Ctrl Pts',(94.4642319885938,-14.9990675132126,
62.4254070205069));
#141434=CARTESIAN_POINT('Ctrl Pts',(94.3799838875078,-14.9990992271589,
62.4400162163758));
#141435=CARTESIAN_POINT('Ctrl Pts',(94.2936848021655,-14.9991297146013,
62.4550323617557));
#141436=CARTESIAN_POINT('Ctrl Pts',(94.2053324757767,-14.9991587135592,
62.4704557980971));
#141437=CARTESIAN_POINT('Ctrl Pts',(94.1611563125823,-14.9991732130382,
62.4781675162678));
#141438=CARTESIAN_POINT('Ctrl Pts',(94.1164668391261,-14.9991873402925,
62.4859810571776));
#141439=CARTESIAN_POINT('Ctrl Pts',(94.0712637660084,-14.9992010617574,
62.493896493564));
#141440=CARTESIAN_POINT('Ctrl Pts',(94.0486622294495,-14.9992079224898,
62.4978542117572));
#141441=CARTESIAN_POINT('Ctrl Pts',(94.0259322929752,-14.9992146817712,
62.5018374038195));
#141442=CARTESIAN_POINT('Ctrl Pts',(94.0030739193293,-14.9992213353548,
62.5058460818041));
#141443=CARTESIAN_POINT('Ctrl Pts',(93.9802155456834,-14.9992279889383,
62.5098547597888));
#141444=CARTESIAN_POINT('Ctrl Pts',(93.9551481387037,-14.9992351163016,
62.5142543317982));
#141445=CARTESIAN_POINT('Ctrl Pts',(93.9341134493102,-14.9992409747461,
62.5179485865606));
#141446=CARTESIAN_POINT('Ctrl Pts',(93.2610033887235,-14.9994284449695,
62.6361647389558));
#141447=CARTESIAN_POINT('Ctrl Pts',(92.5882566618296,-14.9995133827134,
62.7549799849729));
#141448=CARTESIAN_POINT('Ctrl Pts',(91.9155442365578,-14.9994907910654,
62.8752830475864));
#141449=CARTESIAN_POINT('Ctrl Pts',(91.9155434736732,-14.9991665202076,
62.8752787211533));
#141450=CARTESIAN_POINT('Ctrl Pts',(92.086693919164,-14.9860768545361,63.846009912322));
#141451=CARTESIAN_POINT('Ctrl Pts',(92.4297074936291,-14.7677508465704,
65.7913694335692));
#141452=CARTESIAN_POINT('Ctrl Pts',(93.087950234184,-13.5971624559109,69.5243543489225));
#141453=CARTESIAN_POINT('Ctrl Pts',(93.6699893115637,-11.3677658456745,
72.8250712227319));
#141454=CARTESIAN_POINT('Ctrl Pts',(94.1113790316493,-8.32212329542681,
75.3288531905138));
#141455=CARTESIAN_POINT('Ctrl Pts',(94.3207457772408,-6.1521930131437,76.5155659174532));
#141456=CARTESIAN_POINT('Ctrl Pts',(94.4424043515144,-4.3023274699128,77.2059794423346));
#141457=CARTESIAN_POINT('Ctrl Pts',(94.5098992359463,-2.87767097403913,
77.5886523041447));
#141458=CARTESIAN_POINT('Ctrl Pts',(94.5463398268069,-1.68049722662779,
77.795390819026));
#141459=CARTESIAN_POINT('Ctrl Pts',(94.5585266384417,-0.993628204659395,
77.8644736013413));
#141460=CARTESIAN_POINT('Ctrl Pts',(94.5611174495922,-0.79195163185674,
77.8790704031872));
#141461=CARTESIAN_POINT('',(111.837855320939,-3.16944077116514E-5,74.8658931845202));
#141462=CARTESIAN_POINT('Ctrl Pts',(94.5668566070111,2.94209101525666E-14,
77.9116179430022));
#141463=CARTESIAN_POINT('Ctrl Pts',(96.6609425362034,-9.94245023112965E-6,
77.5423740937652));
#141464=CARTESIAN_POINT('Ctrl Pts',(98.7546944933837,-8.73790753213637E-7,
77.1735054108323));
#141465=CARTESIAN_POINT('Ctrl Pts',(100.849271657605,-2.47060687980083E-5,
76.8043622416323));
#141466=CARTESIAN_POINT('Ctrl Pts',(102.94384882182,-4.85383468428085E-5,
76.4352190724334));
#141467=CARTESIAN_POINT('Ctrl Pts',(105.039251179636,-0.000105274089662958,
76.0658014187793));
#141468=CARTESIAN_POINT('Ctrl Pts',(107.130561787693,-4.76672842314452E-5,
75.6962533003417));
#141469=CARTESIAN_POINT('Ctrl Pts',(107.653389439708,-3.32655828735113E-5,
75.6038662707323));
#141470=CARTESIAN_POINT('Ctrl Pts',(108.175961359368,-1.17169284003341E-5,
75.5114710868269));
#141471=CARTESIAN_POINT('Ctrl Pts',(108.702045166413,-9.48554258586864E-5,
75.4187174262545));
#141472=CARTESIAN_POINT('Ctrl Pts',(109.228128973458,-0.000177993923317082,
75.3259637656821));
#141473=CARTESIAN_POINT('Ctrl Pts',(109.757724660669,-0.000365821513508409,
75.2328516293625));
#141474=CARTESIAN_POINT('Ctrl Pts',(110.274862201896,-0.000138237845730693,
75.1419811030903));
#141475=CARTESIAN_POINT('Ctrl Pts',(110.792000729337,8.93462560637043E-5,
75.0511104035223));
#141476=CARTESIAN_POINT('Ctrl Pts',(111.296681089265,0.000732349520133465,
74.9624813188668));
#141477=CARTESIAN_POINT('Ctrl Pts',(111.837855320796,-3.1694407687799E-5,
74.8658931837171));
#141478=CARTESIAN_POINT('',(105.406754466169,-13.34496396307,67.526113924257));
#141479=CARTESIAN_POINT('Ctrl Pts',(105.406754466169,-13.34496396307,67.526113924257));
#141480=CARTESIAN_POINT('Ctrl Pts',(105.667201640758,-13.1524845173195,
67.8633312808299));
#141481=CARTESIAN_POINT('Ctrl Pts',(106.505311711911,-12.4720154542567,
68.9441574710452));
#141482=CARTESIAN_POINT('Ctrl Pts',(107.85098938429,-11.0326717788794,70.6411848672459));
#141483=CARTESIAN_POINT('Ctrl Pts',(109.342844894738,-8.78940909978976,
72.4057715996434));
#141484=CARTESIAN_POINT('Ctrl Pts',(110.383862574518,-6.57696435517895,
73.5414086564304));
#141485=CARTESIAN_POINT('Ctrl Pts',(111.048812787947,-4.63025152828649,
74.2062402037403));
#141486=CARTESIAN_POINT('Ctrl Pts',(111.444414280311,-3.11083529273396,
74.5731246015333));
#141487=CARTESIAN_POINT('Ctrl Pts',(111.719571250065,-1.51676729084888,
74.8123187261577));
#141488=CARTESIAN_POINT('Ctrl Pts',(111.814574930745,-0.48158953538163,
74.8700323543884));
#141489=CARTESIAN_POINT('Ctrl Pts',(111.837855321069,-3.16944077378891E-5,
74.865893185247));
#141490=CARTESIAN_POINT('Ctrl Pts',(98.4192401226558,-14.4018041922808,
65.9071352203558));
#141491=CARTESIAN_POINT('Ctrl Pts',(98.5394222325127,-14.3885387757991,
65.9349583803957));
#141492=CARTESIAN_POINT('Ctrl Pts',(98.6603383966166,-14.374958657731,65.9629600008797));
#141493=CARTESIAN_POINT('Ctrl Pts',(98.7819870929894,-14.3610525428478,
65.991138645606));
#141494=CARTESIAN_POINT('Ctrl Pts',(99.055167133486,-14.3298243164859,66.0544179370163));
#141495=CARTESIAN_POINT('Ctrl Pts',(99.3320414430944,-14.29695261602,66.1185900405074));
#141496=CARTESIAN_POINT('Ctrl Pts',(99.6125904245059,-14.2623012850507,
66.1836375765257));
#141497=CARTESIAN_POINT('Ctrl Pts',(99.864228609599,-14.231220801378,66.2419819120712));
#141498=CARTESIAN_POINT('Ctrl Pts',(100.1188231284,-14.1987084989489,66.3010305345064));
#141499=CARTESIAN_POINT('Ctrl Pts',(100.376356493531,-14.1646597066291,
66.3607696469528));
#141500=CARTESIAN_POINT('Ctrl Pts',(100.608382744196,-14.1339832402317,
66.4145919634202));
#141501=CARTESIAN_POINT('Ctrl Pts',(100.842794518842,-14.1020595156083,
66.4689747570966));
#141502=CARTESIAN_POINT('Ctrl Pts',(101.079575550411,-14.06880806769,66.5239068806237));
#141503=CARTESIAN_POINT('Ctrl Pts',(101.29374443798,-14.0387320706242,66.5735930894793));
#141504=CARTESIAN_POINT('Ctrl Pts',(101.509851670884,-14.0075697765779,
66.6237287128978));
#141505=CARTESIAN_POINT('Ctrl Pts',(101.727881568406,-13.9752609413613,
66.6743045521247));
#141506=CARTESIAN_POINT('Ctrl Pts',(101.73469078124,-13.9742519158197,66.6758840678586));
#141507=CARTESIAN_POINT('Ctrl Pts',(101.74150186925,-13.9732417718155,66.6774640129205));
#141508=CARTESIAN_POINT('Ctrl Pts',(101.748314831864,-13.9722305075756,
66.6790443870086));
#141509=CARTESIAN_POINT('Ctrl Pts',(101.939045528263,-13.9439198968092,
66.7232873790084));
#141510=CARTESIAN_POINT('Ctrl Pts',(102.131245435303,-13.914731514922,66.7678663795309));
#141511=CARTESIAN_POINT('Ctrl Pts',(102.324901610156,-13.8846258365114,
66.8127747496898));
#141512=CARTESIAN_POINT('Ctrl Pts',(102.506628542656,-13.8563746713085,
66.854916759149));
#141513=CARTESIAN_POINT('Ctrl Pts',(102.68963784033,-13.8273157158036,66.8973488050202));
#141514=CARTESIAN_POINT('Ctrl Pts',(102.873920096121,-13.7974174109149,
66.9400655525872));
#141515=CARTESIAN_POINT('Ctrl Pts',(103.041030899371,-13.7703050352588,
66.9788019462107));
#141516=CARTESIAN_POINT('Ctrl Pts',(103.209188482724,-13.7425024380409,
67.0177724546423));
#141517=CARTESIAN_POINT('Ctrl Pts',(103.378384309845,-13.7139852922797,
67.0569727401741));
#141518=CARTESIAN_POINT('Ctrl Pts',(103.531978313377,-13.6880977591102,
67.0925583033458));
#141519=CARTESIAN_POINT('Ctrl Pts',(103.686427861312,-13.6616213783368,
67.1283332103164));
#141520=CARTESIAN_POINT('Ctrl Pts',(103.841739997656,-13.6345361019978,
67.1642967862645));
#141521=CARTESIAN_POINT('Ctrl Pts',(103.982895043955,-13.609919716404,67.1969821922314));
#141522=CARTESIAN_POINT('Ctrl Pts',(104.124762558038,-13.5848004539271,
67.2298234324098));
#141523=CARTESIAN_POINT('Ctrl Pts',(104.267363231029,-13.5591467521705,
67.2628229687538));
#141524=CARTESIAN_POINT('Ctrl Pts',(104.397096995614,-13.5358077928613,
67.2928449454364));
#141525=CARTESIAN_POINT('Ctrl Pts',(104.527437651834,-13.5120264782336,
67.3229979540809));
#141526=CARTESIAN_POINT('Ctrl Pts',(104.658378047142,-13.4877790297983,
67.3532794135337));
#141527=CARTESIAN_POINT('Ctrl Pts',(104.777697437958,-13.4656835506351,
67.3808733831903));
#141528=CARTESIAN_POINT('Ctrl Pts',(104.8975148222,-13.4432010017889,67.4085740120716));
#141529=CARTESIAN_POINT('Ctrl Pts',(105.017830159682,-13.4203108238425,
67.4363803810496));
#141530=CARTESIAN_POINT('Ctrl Pts',(105.127759789782,-13.3993965426938,
67.4617864840467));
#141531=CARTESIAN_POINT('Ctrl Pts',(105.238105118067,-13.3781419657311,
67.4872808601476));
#141532=CARTESIAN_POINT('Ctrl Pts',(105.348864990805,-13.3565297908362,
67.5128625834291));
#141533=CARTESIAN_POINT('Ctrl Pts',(105.368155212552,-13.3527657593702,
67.5173179615599));
#141534=CARTESIAN_POINT('Ctrl Pts',(105.387458008218,-13.3489908797117,
67.5217759890865));
#141535=CARTESIAN_POINT('Ctrl Pts',(105.406773374803,-13.3452050513228,
67.5262366617009));
#141536=CARTESIAN_POINT('Ctrl Pts',(98.147874059069,-14.16647195032,66.377624860735));
#141537=CARTESIAN_POINT('Ctrl Pts',(98.3192707537691,-14.14960825726,66.410941169501));
#141538=CARTESIAN_POINT('Ctrl Pts',(98.7692528742691,-14.10423461334,66.49840926967));
#141539=CARTESIAN_POINT('Ctrl Pts',(99.475313200169,-14.0284261438,66.63565417898));
#141540=CARTESIAN_POINT('Ctrl Pts',(100.245778761469,-13.93952753982,66.785418260323));
#141541=CARTESIAN_POINT('Ctrl Pts',(100.955266880469,-13.85227099363,66.923329468429));
#141542=CARTESIAN_POINT('Ctrl Pts',(101.608963576769,-13.76716640219,67.050395868438));
#141543=CARTESIAN_POINT('Ctrl Pts',(102.211049942569,-13.68468735089,67.167430186381));
#141544=CARTESIAN_POINT('Ctrl Pts',(102.764974645969,-13.60527459453,67.275102778783));
#141545=CARTESIAN_POINT('Ctrl Pts',(103.274134623369,-13.52925563303,67.374073946483));
#141546=CARTESIAN_POINT('Ctrl Pts',(103.741928092369,-13.45682638993,67.465004239355));
#141547=CARTESIAN_POINT('Ctrl Pts',(104.171681279769,-13.38808134065,67.548540213642));
#141548=CARTESIAN_POINT('Ctrl Pts',(104.566639668869,-13.32295149178,67.625312730527));
#141549=CARTESIAN_POINT('Ctrl Pts',(104.929858598669,-13.26132355552,67.695915690707));
#141550=CARTESIAN_POINT('Ctrl Pts',(105.230722483069,-13.20889210549,67.7543979974229));
#141551=CARTESIAN_POINT('Ctrl Pts',(105.410854685069,-13.1768266842,67.7894123252601));
#141552=CARTESIAN_POINT('Ctrl Pts',(105.479818269769,-13.16444861054,67.8028175550729));
#141553=CARTESIAN_POINT('Ctrl Pts',(98.4917532848691,-15.15283943808,65.107798179803));
#141554=CARTESIAN_POINT('Ctrl Pts',(98.6646840855691,-15.13582480531,65.141412690049));
#141555=CARTESIAN_POINT('Ctrl Pts',(99.118727448469,-15.09004172714,65.229670219725));
#141556=CARTESIAN_POINT('Ctrl Pts',(99.8313090557691,-15.01353347332,65.368182744046));
#141557=CARTESIAN_POINT('Ctrl Pts',(100.609097474869,-14.92379033494,65.519370251844));
#141558=CARTESIAN_POINT('Ctrl Pts',(101.325512002269,-14.83568226642,65.658627824088));
#141559=CARTESIAN_POINT('Ctrl Pts',(101.985742908669,-14.74972723616,65.7869643522));
#141560=CARTESIAN_POINT('Ctrl Pts',(102.593961489469,-14.66640829463,65.905190657944));
#141561=CARTESIAN_POINT('Ctrl Pts',(103.153601372269,-14.58617629943,66.013974174222));
#141562=CARTESIAN_POINT('Ctrl Pts',(103.668070041369,-14.50936478303,66.113977252218));
#141563=CARTESIAN_POINT('Ctrl Pts',(104.140776933769,-14.43617487359,66.205862622613));
#141564=CARTESIAN_POINT('Ctrl Pts',(104.575141584369,-14.36669236077,66.29029497901));
#141565=CARTESIAN_POINT('Ctrl Pts',(104.974569077469,-14.30082583635,66.36793620605));
#141566=CARTESIAN_POINT('Ctrl Pts',(105.342082261369,-14.23846949589,66.439373888846));
#141567=CARTESIAN_POINT('Ctrl Pts',(105.646666250369,-14.18538993416,66.498579314229));
#141568=CARTESIAN_POINT('Ctrl Pts',(105.829109116169,-14.15291324103,66.53404279186));
#141569=CARTESIAN_POINT('Ctrl Pts',(105.898970538669,-14.14037401648,66.547622544524));
#141570=CARTESIAN_POINT('Ctrl Pts',(98.6743292104692,-14.27965323873,63.726550398401));
#141571=CARTESIAN_POINT('Ctrl Pts',(98.8459019370691,-14.26277222601,63.7599009244629));
#141572=CARTESIAN_POINT('Ctrl Pts',(99.2963500670691,-14.21735160134,63.847459608161));
#141573=CARTESIAN_POINT('Ctrl Pts',(100.003158681069,-14.14146283465,63.984849970664));
#141574=CARTESIAN_POINT('Ctrl Pts',(100.774464507769,-14.0524673241,64.134777383871));
#141575=CARTESIAN_POINT('Ctrl Pts',(101.484747401269,-13.96511306951,64.272843081282));
#141576=CARTESIAN_POINT('Ctrl Pts',(102.139193869169,-13.87991089399,64.400055222849));
#141577=CARTESIAN_POINT('Ctrl Pts',(102.741983879469,-13.79733546902,64.517226316099));
#141578=CARTESIAN_POINT('Ctrl Pts',(103.296564374369,-13.71782870864,64.625026382081));
#141579=CARTESIAN_POINT('Ctrl Pts',(103.806333500569,-13.64171880499,64.724115956905));
#141580=CARTESIAN_POINT('Ctrl Pts',(104.274690762969,-13.5692022788,64.815155840681));
#141581=CARTESIAN_POINT('Ctrl Pts',(104.704973095269,-13.50037260886,64.898794670833));
#141582=CARTESIAN_POINT('Ctrl Pts',(105.100444294269,-13.43515822974,64.97566686835));
#141583=CARTESIAN_POINT('Ctrl Pts',(105.464155970669,-13.37344671233,65.0463656092431));
#141584=CARTESIAN_POINT('Ctrl Pts',(105.765446720569,-13.32094089436,65.104930890615));
#141585=CARTESIAN_POINT('Ctrl Pts',(105.945844060969,-13.28882828145,65.1399967563969));
#141586=CARTESIAN_POINT('Ctrl Pts',(106.014910668569,-13.27643171644,65.153422011931));
#141587=CARTESIAN_POINT('Ctrl Pts',(98.4594923245691,-12.67612886135,64.020128731373));
#141588=CARTESIAN_POINT('Ctrl Pts',(98.6285710756692,-12.65949322928,64.052994475293));
#141589=CARTESIAN_POINT('Ctrl Pts',(99.0724168983691,-12.61473821638,64.139269794044));
#141590=CARTESIAN_POINT('Ctrl Pts',(99.7686239528691,-12.53998707959,64.274599411849));
#141591=CARTESIAN_POINT('Ctrl Pts',(100.528025108069,-12.45236451727,64.422212779784));
#141592=CARTESIAN_POINT('Ctrl Pts',(101.227047832369,-12.3663945711,64.558089711098));
#141593=CARTESIAN_POINT('Ctrl Pts',(101.870871722769,-12.28257494254,64.683237022467));
#141594=CARTESIAN_POINT('Ctrl Pts',(102.463692673469,-12.20136491585,64.798470317158));
#141595=CARTESIAN_POINT('Ctrl Pts',(103.008982077969,-12.12318998103,64.904464369116));
#141596=CARTESIAN_POINT('Ctrl Pts',(103.510120935269,-12.04836852325,65.00187638123));
#141597=CARTESIAN_POINT('Ctrl Pts',(103.970490511369,-11.97708860212,65.091363608305));
#141598=CARTESIAN_POINT('Ctrl Pts',(104.393276049869,-11.90945781675,65.173545202099));
#141599=CARTESIAN_POINT('Ctrl Pts',(104.781481886469,-11.84544104117,65.249005149184));
#141600=CARTESIAN_POINT('Ctrl Pts',(105.138212451569,-11.78491368068,65.318346892732));
#141601=CARTESIAN_POINT('Ctrl Pts',(105.433455477569,-11.7334614892,65.375736609798));
#141602=CARTESIAN_POINT('Ctrl Pts',(105.610096402769,-11.7020174754,65.410072298793));
#141603=CARTESIAN_POINT('Ctrl Pts',(105.677703407669,-11.68988289124,65.423213834872));
#141604=CARTESIAN_POINT('Ctrl Pts',(105.406773374803,-13.3452050513228,
67.5262366617009));
#141605=CARTESIAN_POINT('Ctrl Pts',(105.416734125676,-13.3624674052046,
67.4907943810988));
#141606=CARTESIAN_POINT('Ctrl Pts',(105.426800824707,-13.3786476915153,
67.4538067765956));
#141607=CARTESIAN_POINT('Ctrl Pts',(105.436918323535,-13.3934812987196,
67.4153185213962));
#141608=CARTESIAN_POINT('Ctrl Pts',(105.44680434208,-13.4079755248515,67.3777108467017));
#141609=CARTESIAN_POINT('Ctrl Pts',(105.45673880432,-13.4211833350787,67.3386701059155));
#141610=CARTESIAN_POINT('Ctrl Pts',(105.466659412237,-13.4328491135877,
67.2982858097589));
#141611=CARTESIAN_POINT('Ctrl Pts',(105.476285818735,-13.444168936625,67.2590991334795));
#141612=CARTESIAN_POINT('Ctrl Pts',(105.485899070319,-13.4540361373327,
67.2186473412336));
#141613=CARTESIAN_POINT('Ctrl Pts',(105.495433165373,-13.4622186730866,
67.1770603204156));
#141614=CARTESIAN_POINT('Ctrl Pts',(105.504813767443,-13.4702694751185,
67.1361428246943));
#141615=CARTESIAN_POINT('Ctrl Pts',(105.514117612121,-13.4766886950509,
67.0941263620656));
#141616=CARTESIAN_POINT('Ctrl Pts',(105.52327463302,-13.4812672146046,67.0511825584069));
#141617=CARTESIAN_POINT('Ctrl Pts',(105.532244290811,-13.4857520524174,
67.0091174340333));
#141618=CARTESIAN_POINT('Ctrl Pts',(105.541072907105,-13.4884700626533,
66.96616275373));
#141619=CARTESIAN_POINT('Ctrl Pts',(105.549689835139,-13.4892465523338,
66.9225244285964));
#141620=CARTESIAN_POINT('Ctrl Pts',(105.553743287625,-13.4896118175436,
66.9019967095727));
#141621=CARTESIAN_POINT('Ctrl Pts',(105.557749842784,-13.4895478405243,
66.8813183408023));
#141622=CARTESIAN_POINT('Ctrl Pts',(105.561701940056,-13.4890388168851,
66.8605139917143));
#141623=CARTESIAN_POINT('Ctrl Pts',(105.569908612252,-13.4879818109819,
66.8173130122237));
#141624=CARTESIAN_POINT('Ctrl Pts',(105.577880147696,-13.4850031947318,
66.7735680660603));
#141625=CARTESIAN_POINT('Ctrl Pts',(105.585548195281,-13.4799888463478,
66.7295266454243));
#141626=CARTESIAN_POINT('Ctrl Pts',(105.593127183416,-13.4750327364015,
66.685996737618));
#141627=CARTESIAN_POINT('Ctrl Pts',(105.600409498371,-13.4680874471808,
66.6421777804316));
#141628=CARTESIAN_POINT('Ctrl Pts',(105.60733124381,-13.4590851280279,66.5983365748304));
#141629=CARTESIAN_POINT('Ctrl Pts',(105.614188221935,-13.4501670442791,
66.5549055948175));
#141630=CARTESIAN_POINT('Ctrl Pts',(105.620691159308,-13.4392299403628,
66.511453466019));
#141631=CARTESIAN_POINT('Ctrl Pts',(105.626782851463,-13.4262553715034,
66.4682576499431));
#141632=CARTESIAN_POINT('Ctrl Pts',(105.632831399466,-13.4133726944771,
66.4253677664004));
#141633=CARTESIAN_POINT('Ctrl Pts',(105.638474338109,-13.3984811831692,
66.3827313295392));
#141634=CARTESIAN_POINT('Ctrl Pts',(105.643663200714,-13.3816131129061,
66.3406271353247));
#141635=CARTESIAN_POINT('Ctrl Pts',(105.648825111233,-13.3648326590884,
66.2987416395013));
#141636=CARTESIAN_POINT('Ctrl Pts',(105.653537512519,-13.3460961921019,
66.2573836419157));
#141637=CARTESIAN_POINT('Ctrl Pts',(105.657762469329,-13.3254859593339,
66.2168233627578));
#141638=CARTESIAN_POINT('Ctrl Pts',(105.661980909241,-13.3049075173765,
66.1763256468989));
#141639=CARTESIAN_POINT('Ctrl Pts',(105.665713305536,-13.2824613297786,
66.1366239365531));
#141640=CARTESIAN_POINT('Ctrl Pts',(105.668933485206,-13.2582774310437,
66.0979715501854));
#141641=CARTESIAN_POINT('Ctrl Pts',(105.67215525787,-13.2340815687411,66.059300042813));
#141642=CARTESIAN_POINT('Ctrl Pts',(105.674864251458,-13.2081466988365,
66.0216795698616));
#141643=CARTESIAN_POINT('Ctrl Pts',(105.677047053913,-13.1806462961128,
65.9853374431438));
#141644=CARTESIAN_POINT('Ctrl Pts',(105.679235389074,-13.1530761886772,
65.948903200776));
#141645=CARTESIAN_POINT('Ctrl Pts',(105.680894856989,-13.1239331775076,
65.9137543455201));
#141646=CARTESIAN_POINT('Ctrl Pts',(105.682025272019,-13.0934279909319,
65.8800841419623));
#141647=CARTESIAN_POINT('Ctrl Pts',(105.683166173587,-13.0626398164298,
65.8461015895171));
#141648=CARTESIAN_POINT('Ctrl Pts',(105.683768196746,-13.0304647557896,
65.8136256862783));
#141649=CARTESIAN_POINT('Ctrl Pts',(105.683844504273,-12.9971465327891,
65.7828111360314));
#141650=CARTESIAN_POINT('Ctrl Pts',(105.683921267299,-12.9636294248799,
65.7518126459323));
#141651=CARTESIAN_POINT('Ctrl Pts',(105.683466115453,-12.9289562400225,
65.7224956156532));
#141652=CARTESIAN_POINT('Ctrl Pts',(105.68250488943,-12.8933912866128,65.6949683115688));
#141653=CARTESIAN_POINT('Ctrl Pts',(105.681529725943,-12.8573106529629,
65.6670418705413));
#141654=CARTESIAN_POINT('Ctrl Pts',(105.680033833554,-12.8203130016877,
65.6409575062467));
#141655=CARTESIAN_POINT('Ctrl Pts',(105.678055280779,-12.7826789266197,
65.6167754398037));
#141656=CARTESIAN_POINT('Ctrl Pts',(105.676291466558,-12.7491293960437,
65.5952179290623));
#141657=CARTESIAN_POINT('Ctrl Pts',(105.674144315099,-12.7150744959912,
65.5751713377354));
#141658=CARTESIAN_POINT('Ctrl Pts',(105.671646638611,-12.6807085185017,
65.5566441699934));
#141659=CARTESIAN_POINT('Ctrl Pts',(105.668775916753,-12.6412097430363,
65.5353498407728));
#141660=CARTESIAN_POINT('Ctrl Pts',(105.665442179767,-12.6013009501918,
65.5160633596856));
#141661=CARTESIAN_POINT('Ctrl Pts',(105.661701496265,-12.561260204733,65.4987500365353));
#141662=CARTESIAN_POINT('Ctrl Pts',(105.657902192529,-12.5205919809412,
65.4811653963796));
#141663=CARTESIAN_POINT('Ctrl Pts',(105.653683288102,-12.4797882328283,
65.4656157553205));
#141664=CARTESIAN_POINT('Ctrl Pts',(105.64910744664,-12.4391121897216,65.4520189555552));
#141665=CARTESIAN_POINT('Ctrl Pts',(105.644402469273,-12.3972882183761,
65.4380384372859));
#141666=CARTESIAN_POINT('Ctrl Pts',(105.639320327356,-12.3555997906835,
65.4261219763008));
#141667=CARTESIAN_POINT('Ctrl Pts',(105.633930130516,-12.3142947246995,
65.4161401886094));
#141668=CARTESIAN_POINT('Ctrl Pts',(105.628448069826,-12.2722857062425,
65.4059882836706));
#141669=CARTESIAN_POINT('Ctrl Pts',(105.622647554534,-12.2306734997387,
65.3978368288397));
#141670=CARTESIAN_POINT('Ctrl Pts',(105.616599251241,-12.189673606019,65.3915189375991));
#141671=CARTESIAN_POINT('Ctrl Pts',(105.610377006754,-12.1474946096516,
65.3850193521732));
#141672=CARTESIAN_POINT('Ctrl Pts',(105.603892691435,-12.1059638194751,
65.3804595659265));
#141673=CARTESIAN_POINT('Ctrl Pts',(105.597218269814,-12.0652648663608,
65.3776369306512));
#141674=CARTESIAN_POINT('Ctrl Pts',(105.594248782885,-12.047157678023,65.3763811246751));
#141675=CARTESIAN_POINT('Ctrl Pts',(105.591241585468,-12.029214467156,65.3754689690382));
#141676=CARTESIAN_POINT('Ctrl Pts',(105.588202588019,-12.0114482303019,
65.3748819173935));
#141677=CARTESIAN_POINT('Ctrl Pts',(104.952232036869,-12.73587741823,68.1320028366331));
#141678=CARTESIAN_POINT('Ctrl Pts',(104.959822185469,-12.73457436689,68.133478219418));
#141679=CARTESIAN_POINT('Ctrl Pts',(105.015863075569,-12.7249411692,68.144371519325));
#141680=CARTESIAN_POINT('Ctrl Pts',(105.118775843869,-12.70706879104,68.1643758348569));
#141681=CARTESIAN_POINT('Ctrl Pts',(105.261221405869,-12.68166925282,68.192064585411));
#141682=CARTESIAN_POINT('Ctrl Pts',(105.402364938369,-12.65578816422,68.219500245804));
#141683=CARTESIAN_POINT('Ctrl Pts',(105.543618402569,-12.6301955777,68.246957274863));
#141684=CARTESIAN_POINT('Ctrl Pts',(105.687431557269,-12.60472429698,68.274911859823));
#141685=CARTESIAN_POINT('Ctrl Pts',(105.823449722569,-12.58115097953,68.30135124478));
#141686=CARTESIAN_POINT('Ctrl Pts',(105.963723330769,-12.55697430171,68.3286178081799));
#141687=CARTESIAN_POINT('Ctrl Pts',(106.097164283069,-12.52886481947,68.35455623118));
#141688=CARTESIAN_POINT('Ctrl Pts',(106.234154640669,-12.5005565727,68.381184592121));
#141689=CARTESIAN_POINT('Ctrl Pts',(106.374425007569,-12.47109589523,68.408450525463));
#141690=CARTESIAN_POINT('Ctrl Pts',(106.520440250569,-12.44039854804,68.436833155168));
#141691=CARTESIAN_POINT('Ctrl Pts',(106.676875480469,-12.40715650872,68.467241235266));
#141692=CARTESIAN_POINT('Ctrl Pts',(106.847058876369,-12.37032464115,68.500321701448));
#141693=CARTESIAN_POINT('Ctrl Pts',(107.032307995569,-12.32930601219,68.536330662197));
#141694=CARTESIAN_POINT('Ctrl Pts',(107.233857295369,-12.28362359072,68.575508072906));
#141695=CARTESIAN_POINT('Ctrl Pts',(107.452609118669,-12.23279531428,68.6180293321429));
#141696=CARTESIAN_POINT('Ctrl Pts',(107.689333475969,-12.17635893667,68.664044115523));
#141697=CARTESIAN_POINT('Ctrl Pts',(107.945108470469,-12.1136901956,68.713761986126));
#141698=CARTESIAN_POINT('Ctrl Pts',(108.221352645369,-12.04394693307,68.767458682204));
#141699=CARTESIAN_POINT('Ctrl Pts',(108.519904230369,-11.96606158696,68.825491521187));
#141700=CARTESIAN_POINT('Ctrl Pts',(108.842656572169,-11.87879604663,68.888228534223));
#141701=CARTESIAN_POINT('Ctrl Pts',(109.191603713569,-11.78073386166,68.956057325939));
#141702=CARTESIAN_POINT('Ctrl Pts',(109.568887864469,-11.67018852649,69.029394301794));
#141703=CARTESIAN_POINT('Ctrl Pts',(109.976855656869,-11.54513335067,69.1086956031249));
#141704=CARTESIAN_POINT('Ctrl Pts',(110.418012265769,-11.40313753581,69.1944481890609));
#141705=CARTESIAN_POINT('Ctrl Pts',(110.895045258669,-11.2412511075,69.28717447242));
#141706=CARTESIAN_POINT('Ctrl Pts',(111.410817072669,-11.05585348146,69.387430857371));
#141707=CARTESIAN_POINT('Ctrl Pts',(111.968193872269,-10.84255144708,69.495774472649));
#141708=CARTESIAN_POINT('Ctrl Pts',(112.570412941369,-10.59580176849,69.612834585628));
#141709=CARTESIAN_POINT('Ctrl Pts',(113.220235519769,-10.3088878416,69.7391479296449));
#141710=CARTESIAN_POINT('Ctrl Pts',(113.920526429469,-9.97338727422198,
69.8752713724391));
#141711=CARTESIAN_POINT('Ctrl Pts',(114.673362321169,-9.57892440546198,
70.021608576066));
#141712=CARTESIAN_POINT('Ctrl Pts',(115.480641495669,-9.11187730365798,
70.178528534627));
#141713=CARTESIAN_POINT('Ctrl Pts',(116.342765158169,-8.55458391315699,
70.346109234944));
#141714=CARTESIAN_POINT('Ctrl Pts',(117.226756584969,-7.90619100724499,
70.517940619224));
#141715=CARTESIAN_POINT('Ctrl Pts',(118.060477130769,-7.20202699572299,
70.680000285382));
#141716=CARTESIAN_POINT('Ctrl Pts',(118.784806129869,-6.495187570145,70.8207962827541));
#141717=CARTESIAN_POINT('Ctrl Pts',(119.382258340369,-5.82452362446499,
70.9369298076469));
#141718=CARTESIAN_POINT('Ctrl Pts',(119.873935776169,-5.19148602277899,
71.032502696561));
#141719=CARTESIAN_POINT('Ctrl Pts',(120.279478642169,-4.59391006016099,
71.11133263759));
#141720=CARTESIAN_POINT('Ctrl Pts',(120.613855905469,-4.02868582297099,
71.176329317749));
#141721=CARTESIAN_POINT('Ctrl Pts',(120.887058111969,-3.49549879784399,
71.229434712121));
#141722=CARTESIAN_POINT('Ctrl Pts',(121.107492496269,-2.99524221621799,
71.272283029704));
#141723=CARTESIAN_POINT('Ctrl Pts',(121.282922740269,-2.52901011200199,
71.30638338495));
#141724=CARTESIAN_POINT('Ctrl Pts',(121.421275086969,-2.09491375878399,
71.333276491063));
#141725=CARTESIAN_POINT('Ctrl Pts',(121.528476941569,-1.69170413216199,
71.3541145246909));
#141726=CARTESIAN_POINT('Ctrl Pts',(121.609328944569,-1.31874211906699,
71.369830640449));
#141727=CARTESIAN_POINT('Ctrl Pts',(121.667923195969,-0.974734023751388,
71.381220265999));
#141728=CARTESIAN_POINT('Ctrl Pts',(121.707625940769,-0.658282511519486,
71.388937736322));
#141729=CARTESIAN_POINT('Ctrl Pts',(121.731363094969,-0.367700522520886,
71.393551794715));
#141730=CARTESIAN_POINT('Ctrl Pts',(121.741634599469,-0.101175225261786,
71.395548382888));
#141731=CARTESIAN_POINT('Ctrl Pts',(121.740745608969,0.102180689578914,
71.395375579788));
#141732=CARTESIAN_POINT('Ctrl Pts',(121.736614525769,0.216805681933914,
71.3945725745509));
#141733=CARTESIAN_POINT('Ctrl Pts',(121.735103526269,0.249988879730614,
71.394278864527));
#141734=CARTESIAN_POINT('Ctrl Pts',(105.492580541969,-14.75894581259,67.138711581365));
#141735=CARTESIAN_POINT('Ctrl Pts',(105.500469740069,-14.75759123539,67.140245093777));
#141736=CARTESIAN_POINT('Ctrl Pts',(105.558768713869,-14.7475691159,67.15157732288));
#141737=CARTESIAN_POINT('Ctrl Pts',(105.666629227569,-14.72884244559,67.172543387499));
#141738=CARTESIAN_POINT('Ctrl Pts',(105.819635636069,-14.70155594623,67.202284968906));
#141739=CARTESIAN_POINT('Ctrl Pts',(105.965965642769,-14.67472441123,67.2307287827801));
#141740=CARTESIAN_POINT('Ctrl Pts',(106.095643432669,-14.65123731042,67.2559357174571));
#141741=CARTESIAN_POINT('Ctrl Pts',(106.240626942769,-14.62551395671,67.284117797616));
#141742=CARTESIAN_POINT('Ctrl Pts',(106.346379463669,-14.6074213232,67.304674107888));
#141743=CARTESIAN_POINT('Ctrl Pts',(106.565377381869,-14.5688173883,67.347243203358));
#141744=CARTESIAN_POINT('Ctrl Pts',(106.702418711469,-14.53959176337,67.37388147231));
#141745=CARTESIAN_POINT('Ctrl Pts',(106.845617522769,-14.51009959534,67.401716640428));
#141746=CARTESIAN_POINT('Ctrl Pts',(106.986141518569,-14.48055441258,67.429031874481));
#141747=CARTESIAN_POINT('Ctrl Pts',(107.135114434969,-14.44924442858,67.4579894205271));
#141748=CARTESIAN_POINT('Ctrl Pts',(107.296863943769,-14.41487311883,67.4894304969489));
#141749=CARTESIAN_POINT('Ctrl Pts',(107.476158454069,-14.37607194618,67.524281993211));
#141750=CARTESIAN_POINT('Ctrl Pts',(107.670628850969,-14.33300989809,67.562083397709));
#141751=CARTESIAN_POINT('Ctrl Pts',(107.882299752669,-14.2850339185,67.603228258333));
#141752=CARTESIAN_POINT('Ctrl Pts',(108.111834366569,-14.23169947047,67.647845490204));
#141753=CARTESIAN_POINT('Ctrl Pts',(108.359969891769,-14.17254283898,67.696078390983));
#141754=CARTESIAN_POINT('Ctrl Pts',(108.628544882169,-14.1067388206,67.748284341169));
#141755=CARTESIAN_POINT('Ctrl Pts',(108.919099624169,-14.03338368093,67.804762743585));
#141756=CARTESIAN_POINT('Ctrl Pts',(109.233784324169,-13.95129086149,67.8659315580971));
#141757=CARTESIAN_POINT('Ctrl Pts',(109.574509226469,-13.85916720993,67.932162100438));
#141758=CARTESIAN_POINT('Ctrl Pts',(109.943480085769,-13.75547965436,68.003883128056));
#141759=CARTESIAN_POINT('Ctrl Pts',(110.343130829169,-13.63838326156,68.0815677507689));
#141760=CARTESIAN_POINT('Ctrl Pts',(110.776141189469,-13.50565488543,68.165736858487));
#141761=CARTESIAN_POINT('Ctrl Pts',(111.245388189769,-13.354622112,68.256949690632));
#141762=CARTESIAN_POINT('Ctrl Pts',(111.754109128869,-13.18198856946,68.3558355175029));
#141763=CARTESIAN_POINT('Ctrl Pts',(112.305743248969,-12.9837090819,68.463062863392));
#141764=CARTESIAN_POINT('Ctrl Pts',(112.903812062269,-12.75484751004,68.579316244352));
#141765=CARTESIAN_POINT('Ctrl Pts',(113.552372588269,-12.48912859477,68.705384268995));
#141766=CARTESIAN_POINT('Ctrl Pts',(114.255050788269,-12.17890247091,68.841971756345));
#141767=CARTESIAN_POINT('Ctrl Pts',(115.015487040869,-11.81462198028,68.989786327825));
#141768=CARTESIAN_POINT('Ctrl Pts',(115.837112874269,-11.38417047417,69.149495008306));
#141769=CARTESIAN_POINT('Ctrl Pts',(116.723420541269,-10.87148884659,69.32177662635));
#141770=CARTESIAN_POINT('Ctrl Pts',(117.676819254069,-10.25533692963,69.507099487684));
#141771=CARTESIAN_POINT('Ctrl Pts',(118.663346228469,-9.53199294674199,
69.69886186288));
#141772=CARTESIAN_POINT('Ctrl Pts',(119.604511054069,-8.73743036268499,
69.881806685573));
#141773=CARTESIAN_POINT('Ctrl Pts',(120.432208031169,-7.93008953233,70.042695482718));
#141774=CARTESIAN_POINT('Ctrl Pts',(121.123557856069,-7.15431205073399,
70.1770809460259));
#141775=CARTESIAN_POINT('Ctrl Pts',(121.698017157269,-6.41492080923599,
70.2887450798039));
#141776=CARTESIAN_POINT('Ctrl Pts',(122.176477179669,-5.71015914524499,
70.381748750991));
#141777=CARTESIAN_POINT('Ctrl Pts',(122.575512542569,-5.03589455575199,
70.459313755258));
#141778=CARTESIAN_POINT('Ctrl Pts',(122.905036512669,-4.39304561090499,
70.523367046078));
#141779=CARTESIAN_POINT('Ctrl Pts',(123.173320684769,-3.78433296845899,
70.575516466625));
#141780=CARTESIAN_POINT('Ctrl Pts',(123.387691659769,-3.21470112064199,
70.617186170945));
#141781=CARTESIAN_POINT('Ctrl Pts',(123.557630545669,-2.68164729664499,
70.650219108973));
#141782=CARTESIAN_POINT('Ctrl Pts',(123.690314882669,-2.18277829981599,
70.6760104601161));
#141783=CARTESIAN_POINT('Ctrl Pts',(123.791288846669,-1.71727622468999,
70.695637908411));
#141784=CARTESIAN_POINT('Ctrl Pts',(123.865481191169,-1.28212654844499,
70.710059511236));
#141785=CARTESIAN_POINT('Ctrl Pts',(123.916585892469,-0.875408245070486,
70.719993308449));
#141786=CARTESIAN_POINT('Ctrl Pts',(123.947740644269,-0.495009380945386,
70.726049208952));
#141787=CARTESIAN_POINT('Ctrl Pts',(123.961550139369,-0.138830407839186,
70.728733516261));
#141788=CARTESIAN_POINT('Ctrl Pts',(123.960405633669,0.139179398717814,
70.7285110457929));
#141789=CARTESIAN_POINT('Ctrl Pts',(123.954664204369,0.298769253595514,
70.727395019413));
#141790=CARTESIAN_POINT('Ctrl Pts',(123.952552482969,0.345228639253714,
70.7269845403021));
#141791=CARTESIAN_POINT('Ctrl Pts',(105.782108038469,-13.99115798116,64.971205130231));
#141792=CARTESIAN_POINT('Ctrl Pts',(105.789883742369,-13.98982295888,64.972716581491));
#141793=CARTESIAN_POINT('Ctrl Pts',(105.847325736169,-13.97994844163,64.983882229722));
#141794=CARTESIAN_POINT('Ctrl Pts',(105.953308498869,-13.96154598928,65.004483294697));
#141795=CARTESIAN_POINT('Ctrl Pts',(106.102306891869,-13.93497562281,65.033445792928));
#141796=CARTESIAN_POINT('Ctrl Pts',(106.246668546069,-13.9085047979,65.061506995923));
#141797=CARTESIAN_POINT('Ctrl Pts',(106.380739495269,-13.88421863053,65.0875678785401));
#141798=CARTESIAN_POINT('Ctrl Pts',(106.525278836269,-13.85859094267,65.115663620517));
#141799=CARTESIAN_POINT('Ctrl Pts',(106.642517668469,-13.83841829919,65.138452654689));
#141800=CARTESIAN_POINT('Ctrl Pts',(106.831638412269,-13.80528974637,65.175214186783));
#141801=CARTESIAN_POINT('Ctrl Pts',(106.967313339269,-13.776487716,65.2015868526511));
#141802=CARTESIAN_POINT('Ctrl Pts',(107.108155939969,-13.74744486562,65.228964017536));
#141803=CARTESIAN_POINT('Ctrl Pts',(107.248583679469,-13.71793175401,65.256260541156));
#141804=CARTESIAN_POINT('Ctrl Pts',(107.396434109969,-13.68685427579,65.284999896966));
#141805=CARTESIAN_POINT('Ctrl Pts',(107.556166762269,-13.6529115428,65.316048934241));
#141806=CARTESIAN_POINT('Ctrl Pts',(107.732003454369,-13.61485775391,65.3502282953701));
#141807=CARTESIAN_POINT('Ctrl Pts',(107.922974224169,-13.57257121709,65.387349437894));
#141808=CARTESIAN_POINT('Ctrl Pts',(108.130803810969,-13.52546568065,65.427747618817));
#141809=CARTESIAN_POINT('Ctrl Pts',(108.356246177969,-13.47308236608,65.471569394495));
#141810=CARTESIAN_POINT('Ctrl Pts',(108.600050976669,-13.41495811582,65.518960483128));
#141811=CARTESIAN_POINT('Ctrl Pts',(108.863768157469,-13.3503439869,65.570222166064));
#141812=CARTESIAN_POINT('Ctrl Pts',(109.148891803169,-13.2783596142,65.625644865033));
#141813=CARTESIAN_POINT('Ctrl Pts',(109.457453719869,-13.19786360029,65.685623525096));
#141814=CARTESIAN_POINT('Ctrl Pts',(109.791357738969,-13.1075836821,65.750528215431));
#141815=CARTESIAN_POINT('Ctrl Pts',(110.152729267069,-13.00603104747,65.820772075312));
#141816=CARTESIAN_POINT('Ctrl Pts',(110.543891519569,-12.89142088912,65.896806694317));
#141817=CARTESIAN_POINT('Ctrl Pts',(110.967397812269,-12.7616046191,65.9791283892041));
#141818=CARTESIAN_POINT('Ctrl Pts',(111.425984045469,-12.61400152053,66.0682689678321));
#141819=CARTESIAN_POINT('Ctrl Pts',(111.922678886269,-12.44544668515,66.164817146322));
#141820=CARTESIAN_POINT('Ctrl Pts',(112.460702669569,-12.25205607655,66.269398897531));
#141821=CARTESIAN_POINT('Ctrl Pts',(113.043328192369,-12.02909960586,66.382650391923));
#141822=CARTESIAN_POINT('Ctrl Pts',(113.674301370969,-11.77057982886,66.50529976548));
#141823=CARTESIAN_POINT('Ctrl Pts',(114.356919990569,-11.46920106834,66.637988045937));
#141824=CARTESIAN_POINT('Ctrl Pts',(115.094530093269,-11.11584303338,66.7813656412041));
#141825=CARTESIAN_POINT('Ctrl Pts',(115.890049008869,-10.69904980887,66.9359996256221));
#141826=CARTESIAN_POINT('Ctrl Pts',(116.746364059269,-10.20368723669,67.102451240462));
#141827=CARTESIAN_POINT('Ctrl Pts',(117.665122384669,-9.60987310153999,
67.281040658987));
#141828=CARTESIAN_POINT('Ctrl Pts',(118.612735427169,-8.91497428887999,
67.4652388943169));
#141829=CARTESIAN_POINT('Ctrl Pts',(119.513123375969,-8.15471945445799,
67.64025745555));
#141830=CARTESIAN_POINT('Ctrl Pts',(120.301590500069,-7.38552056524799,
67.7935207036991));
#141831=CARTESIAN_POINT('Ctrl Pts',(120.957304631269,-6.64963540465299,
67.920979255265));
#141832=CARTESIAN_POINT('Ctrl Pts',(121.500346848769,-5.95060712404298,
68.02653649615));
#141833=CARTESIAN_POINT('Ctrl Pts',(121.951133607369,-5.28652420202899,
68.114161002909));
#141834=CARTESIAN_POINT('Ctrl Pts',(122.325630154769,-4.65364222513899,
68.186956120831));
#141835=CARTESIAN_POINT('Ctrl Pts',(122.633779086469,-4.05241178798398,
68.246854504334));
#141836=CARTESIAN_POINT('Ctrl Pts',(122.883903474669,-3.48486000988298,
68.29547400286));
#141837=CARTESIAN_POINT('Ctrl Pts',(123.083495799869,-2.95447007060999,
68.3342710143309));
#141838=CARTESIAN_POINT('Ctrl Pts',(123.241447072969,-2.45897223933399,
68.364973784855));
#141839=CARTESIAN_POINT('Ctrl Pts',(123.364460387569,-1.99640755164799,
68.388885270283));
#141840=CARTESIAN_POINT('Ctrl Pts',(123.457797735369,-1.56602595675199,
68.407028303353));
#141841=CARTESIAN_POINT('Ctrl Pts',(123.526070346269,-1.16546601408599,
68.420299220781));
#141842=CARTESIAN_POINT('Ctrl Pts',(123.572847816969,-0.793005447135286,
68.429391885375));
#141843=CARTESIAN_POINT('Ctrl Pts',(123.601187468069,-0.446693568883186,
68.434900583011));
#141844=CARTESIAN_POINT('Ctrl Pts',(123.613654237269,-0.124539644830986,
68.437323889562));
#141845=CARTESIAN_POINT('Ctrl Pts',(123.612606703869,0.125137778209914,
68.43712026868));
#141846=CARTESIAN_POINT('Ctrl Pts',(123.607476427469,0.267662725948114,
68.436123038987));
#141847=CARTESIAN_POINT('Ctrl Pts',(123.605592689969,0.309083579287614,
68.4357568756719));
#141848=CARTESIAN_POINT('Ctrl Pts',(105.323272139269,-11.75192916108,65.354263847219));
#141849=CARTESIAN_POINT('Ctrl Pts',(105.330716840869,-11.75065117009,65.355710957828));
#141850=CARTESIAN_POINT('Ctrl Pts',(105.385659479669,-11.74120713008,65.36639077824));
#141851=CARTESIAN_POINT('Ctrl Pts',(105.486165841169,-11.72375024912,65.385927333345));
#141852=CARTESIAN_POINT('Ctrl Pts',(105.623474984369,-11.69926846146,65.412617660244));
#141853=CARTESIAN_POINT('Ctrl Pts',(105.762096000969,-11.67384963606,65.439562990768));
#141854=CARTESIAN_POINT('Ctrl Pts',(105.908979459969,-11.64723301644,65.468114385421));
#141855=CARTESIAN_POINT('Ctrl Pts',(106.052223395469,-11.62188433502,65.4959583248361));
#141856=CARTESIAN_POINT('Ctrl Pts',(106.202961689969,-11.59564540853,65.5252590273339));
#141857=CARTESIAN_POINT('Ctrl Pts',(106.304946603769,-11.5784856336,65.545082985332));
#141858=CARTESIAN_POINT('Ctrl Pts',(106.436636461069,-11.55091900332,65.570681028241));
#141859=CARTESIAN_POINT('Ctrl Pts',(106.570607248369,-11.5231865736,65.596722441247));
#141860=CARTESIAN_POINT('Ctrl Pts',(106.710754259169,-11.49376699648,65.623964396482));
#141861=CARTESIAN_POINT('Ctrl Pts',(106.855330995369,-11.46336761397,65.6520674073999));
#141862=CARTESIAN_POINT('Ctrl Pts',(107.009181549769,-11.43067481148,65.681973074956));
#141863=CARTESIAN_POINT('Ctrl Pts',(107.174933624769,-11.3948007436,65.714192175322));
#141864=CARTESIAN_POINT('Ctrl Pts',(107.355697843669,-11.35477596077,65.7493293554091));
#141865=CARTESIAN_POINT('Ctrl Pts',(107.552324357569,-11.31020904411,65.787549868703));
#141866=CARTESIAN_POINT('Ctrl Pts',(107.765831816469,-11.26059968008,65.829051721663));
#141867=CARTESIAN_POINT('Ctrl Pts',(107.997006189069,-11.20548633686,65.873987691913));
#141868=CARTESIAN_POINT('Ctrl Pts',(108.246555722369,-11.14434248276,65.922495449414));
#141869=CARTESIAN_POINT('Ctrl Pts',(108.515839748269,-11.07635590836,65.9748392228171));
#141870=CARTESIAN_POINT('Ctrl Pts',(108.806544761969,-11.0005169271,66.031346835236));
#141871=CARTESIAN_POINT('Ctrl Pts',(109.120555891769,-10.91561419867,66.092384720314));
#141872=CARTESIAN_POINT('Ctrl Pts',(109.459764211569,-10.82028799318,66.158320467413));
#141873=CARTESIAN_POINT('Ctrl Pts',(109.826170050169,-10.71292885861,66.229542903018));
#141874=CARTESIAN_POINT('Ctrl Pts',(110.221958031369,-10.59160565353,66.306476677071));
#141875=CARTESIAN_POINT('Ctrl Pts',(110.649452476469,-10.45400509277,66.389573594144));
#141876=CARTESIAN_POINT('Ctrl Pts',(111.111073583469,-10.29734567721,66.479304095394));
#141877=CARTESIAN_POINT('Ctrl Pts',(111.609403251769,-10.11821332882,66.57617005376));
#141878=CARTESIAN_POINT('Ctrl Pts',(112.146988908369,-9.91247889809999,
66.6806666413349));
#141879=CARTESIAN_POINT('Ctrl Pts',(112.726669146869,-9.674955179165,66.7933456276021));
#141880=CARTESIAN_POINT('Ctrl Pts',(113.350784637569,-9.399379472793,66.91466199502));
#141881=CARTESIAN_POINT('Ctrl Pts',(114.021822999269,-9.07787643283398,
67.045099290116));
#141882=CARTESIAN_POINT('Ctrl Pts',(114.741201918669,-8.70091715272899,
67.1849330846709));
#141883=CARTESIAN_POINT('Ctrl Pts',(115.510044455069,-8.25606505541699,
67.334381680369));
#141884=CARTESIAN_POINT('Ctrl Pts',(116.327775191169,-7.727398351337,67.493333226842));
#141885=CARTESIAN_POINT('Ctrl Pts',(117.161896987269,-7.11545897401699,
67.655470888542));
#141886=CARTESIAN_POINT('Ctrl Pts',(117.943360470569,-6.45526160155699,
67.807372760021));
#141887=CARTESIAN_POINT('Ctrl Pts',(118.617414974669,-5.79730247204099,
67.938396336759));
#141888=CARTESIAN_POINT('Ctrl Pts',(119.169198736969,-5.17776199838799,
68.0456527702781));
#141889=CARTESIAN_POINT('Ctrl Pts',(119.620614028269,-4.59645101100099,
68.133399452039));
#141890=CARTESIAN_POINT('Ctrl Pts',(119.990692591969,-4.05100634772499,
68.205335796626));
#141891=CARTESIAN_POINT('Ctrl Pts',(120.293622463469,-3.53881544589199,
68.2642196925429));
#141892=CARTESIAN_POINT('Ctrl Pts',(120.539431774469,-3.05896406432699,
68.3120004208479));
#141893=CARTESIAN_POINT('Ctrl Pts',(120.736593729869,-2.61145663953499,
68.350325013936));
#141894=CARTESIAN_POINT('Ctrl Pts',(120.893084592369,-2.19551447993599,
68.3807439079669));
#141895=CARTESIAN_POINT('Ctrl Pts',(121.016074373769,-1.80954750839099,
68.404650818987));
#141896=CARTESIAN_POINT('Ctrl Pts',(121.110882458469,-1.45286318504499,
68.423079735776));
#141897=CARTESIAN_POINT('Ctrl Pts',(121.181947857769,-1.12490935506699,
68.4368935189959));
#141898=CARTESIAN_POINT('Ctrl Pts',(121.232955753569,-0.825229271576386,
68.44680849902));
#141899=CARTESIAN_POINT('Ctrl Pts',(121.267112993769,-0.552680304641586,
68.453448027053));
#141900=CARTESIAN_POINT('Ctrl Pts',(121.287242493169,-0.305782037849186,
68.457360824907));
#141901=CARTESIAN_POINT('Ctrl Pts',(121.295793245269,-0.0828610884916358,
68.459022931039));
#141902=CARTESIAN_POINT('Ctrl Pts',(121.295028528269,0.0841858380577142,
68.458874284375));
#141903=CARTESIAN_POINT('Ctrl Pts',(121.291680659969,0.176941526223414,
68.458223521449));
#141904=CARTESIAN_POINT('Ctrl Pts',(121.290461830169,0.203667660114414,
68.457986603741));
#141905=CARTESIAN_POINT('Ctrl Pts',(105.406735574489,-13.3447234534956,
67.5259914523896));
#141906=CARTESIAN_POINT('Ctrl Pts',(105.419348855129,-13.3424555725803,
67.5284994651872));
#141907=CARTESIAN_POINT('Ctrl Pts',(105.432007480475,-13.340144416473,67.5310693565358));
#141908=CARTESIAN_POINT('Ctrl Pts',(105.44466272379,-13.3377895139349,67.5337091593829));
#141909=CARTESIAN_POINT('Ctrl Pts',(105.4595503261,-13.3350192114135,67.5368146180442));
#141910=CARTESIAN_POINT('Ctrl Pts',(105.474434021802,-13.3321885390212,
67.5400163316475));
#141911=CARTESIAN_POINT('Ctrl Pts',(105.489300427801,-13.3293085895235,
67.5432963615387));
#141912=CARTESIAN_POINT('Ctrl Pts',(105.505021656339,-13.3262630421172,
67.5467649940739));
#141913=CARTESIAN_POINT('Ctrl Pts',(105.52072783756,-13.3231632268862,67.5503189569254));
#141914=CARTESIAN_POINT('Ctrl Pts',(105.536428766284,-13.3200260560355,
67.5539280211083));
#141915=CARTESIAN_POINT('Ctrl Pts',(105.550053300076,-13.3173037654616,
67.557059798711));
#141916=CARTESIAN_POINT('Ctrl Pts',(105.563676092547,-13.3145537563832,
67.5602320101648));
#141917=CARTESIAN_POINT('Ctrl Pts',(105.577277511334,-13.3117813163253,
67.5634408239287));
#141918=CARTESIAN_POINT('Ctrl Pts',(105.579350383511,-13.3113587932084,
67.5639298509103));
#141919=CARTESIAN_POINT('Ctrl Pts',(105.581422673761,-13.310935731282,67.5644197761276));
#141920=CARTESIAN_POINT('Ctrl Pts',(105.583494211195,-13.3105121282584,
67.564910642499));
#141921=CARTESIAN_POINT('Ctrl Pts',(105.595509025827,-13.3080552516775,
67.5677576431688));
#141922=CARTESIAN_POINT('Ctrl Pts',(105.607502181302,-13.3055808108532,
67.5706348249016));
#141923=CARTESIAN_POINT('Ctrl Pts',(105.619424338444,-13.3030823900979,
67.5735715360503));
#141924=CARTESIAN_POINT('Ctrl Pts',(105.624099925604,-13.3021025687565,
67.574723244485));
#141925=CARTESIAN_POINT('Ctrl Pts',(105.628764089798,-13.3011189716412,
67.5758843118018));
#141926=CARTESIAN_POINT('Ctrl Pts',(105.633411799757,-13.3001308573854,
67.5770573205464));
#141927=CARTESIAN_POINT('Ctrl Pts',(105.650114324641,-13.2965798606385,
67.5812727745909));
#141928=CARTESIAN_POINT('Ctrl Pts',(105.666708531094,-13.2929881960317,
67.585592200278));
#141929=CARTESIAN_POINT('Ctrl Pts',(105.683281251363,-13.2893570357737,
67.5900082142077));
#141930=CARTESIAN_POINT('Ctrl Pts',(105.710542028484,-13.2833840724412,
67.5972721980045));
#141931=CARTESIAN_POINT('Ctrl Pts',(105.737741142737,-13.2773032862321,
67.6048004028214));
#141932=CARTESIAN_POINT('Ctrl Pts',(105.765107084503,-13.2711032057106,
67.6125810102969));
#141933=CARTESIAN_POINT('Ctrl Pts',(105.780782298461,-13.2675517990181,
67.6170377429738));
#141934=CARTESIAN_POINT('Ctrl Pts',(105.796510488709,-13.2639611441589,
67.6215771922203));
#141935=CARTESIAN_POINT('Ctrl Pts',(105.81234015007,-13.2603311242177,67.6261905806811));
#141936=CARTESIAN_POINT('Ctrl Pts',(105.825404534772,-13.2573352308815,
67.6299980583176));
#141937=CARTESIAN_POINT('Ctrl Pts',(105.838534840569,-13.2543118163068,
67.633857648385));
#141938=CARTESIAN_POINT('Ctrl Pts',(105.851663194163,-13.2512384347092,
67.6378180818378));
#141939=CARTESIAN_POINT('Ctrl Pts',(105.853208076029,-13.2508767738607,
67.6382841267064));
#141940=CARTESIAN_POINT('Ctrl Pts',(105.854752981239,-13.2505144320582,
67.6387515407154));
#141941=CARTESIAN_POINT('Ctrl Pts',(105.856297837123,-13.2501513809293,
67.6392203828757));
#141942=CARTESIAN_POINT('Ctrl Pts',(105.871928249551,-13.2464781328706,
67.6439639944989));
#141943=CARTESIAN_POINT('Ctrl Pts',(105.887507214198,-13.2427762158654,
67.6487775733898));
#141944=CARTESIAN_POINT('Ctrl Pts',(105.902910700177,-13.2390652774627,
67.6536389990103));
#141945=CARTESIAN_POINT('Ctrl Pts',(105.906042369124,-13.2383108098976,
67.6546273711018));
#141946=CARTESIAN_POINT('Ctrl Pts',(105.909166936774,-13.2375560028952,
67.6556176432816));
#141947=CARTESIAN_POINT('Ctrl Pts',(105.912283569683,-13.2368010670366,
67.6566095252591));
#141948=CARTESIAN_POINT('Ctrl Pts',(105.914589339976,-13.2362425448344,
67.6573433466827));
#141949=CARTESIAN_POINT('Ctrl Pts',(105.916890635439,-13.2356839325614,
67.6580781031648));
#141950=CARTESIAN_POINT('Ctrl Pts',(105.919187076455,-13.2351252969899,
67.6588137177562));
#141951=CARTESIAN_POINT('Ctrl Pts',(105.921483517471,-13.2345666614184,
67.6595493323476));
#141952=CARTESIAN_POINT('Ctrl Pts',(105.926365493087,-13.233377729542,67.6611160596461));
#141953=CARTESIAN_POINT('Ctrl Pts',(105.930102670479,-13.2324674516722,
67.6623162717565));
#141954=CARTESIAN_POINT('Ctrl Pts',(105.937577025265,-13.2306468959328,
67.6647166959771));
#141955=CARTESIAN_POINT('Ctrl Pts',(105.944480659722,-13.2289649159458,
67.6669365825435));
#141956=CARTESIAN_POINT('Ctrl Pts',(105.950857804366,-13.2274131285108,
67.6689851561453));
#141957=CARTESIAN_POINT('Ctrl Pts',(105.958938076775,-13.2254469091608,
67.6715808370775));
#141958=CARTESIAN_POINT('Ctrl Pts',(105.966180881029,-13.2236889322356,
67.6739019442468));
#141959=CARTESIAN_POINT('Ctrl Pts',(105.972589215247,-13.222136306475,67.675952322906));
#141960=CARTESIAN_POINT('Ctrl Pts',(105.976296102932,-13.2212381933123,
67.6771383602045));
#141961=CARTESIAN_POINT('Ctrl Pts',(105.979724062723,-13.220408854815,67.6782336403411));
#141962=CARTESIAN_POINT('Ctrl Pts',(105.982875322055,-13.2196480918367,
67.6792378960421));
#141963=CARTESIAN_POINT('Ctrl Pts',(105.991474365275,-13.2175721491608,
67.6819782729092));
#141964=CARTESIAN_POINT('Ctrl Pts',(105.997989368553,-13.216008835081,67.6840398857284));
#141965=CARTESIAN_POINT('Ctrl Pts',(106.002298346939,-13.2149771010983,
67.6853994996504));
#141966=CARTESIAN_POINT('Ctrl Pts',(106.004452836132,-13.214461234107,67.6860793066115));
#141967=CARTESIAN_POINT('Ctrl Pts',(106.006055362552,-13.214078368262,67.6865835393359));
#141968=CARTESIAN_POINT('Ctrl Pts',(106.00704938813,-13.213845890555,67.6868871294661));
#141969=CARTESIAN_POINT('Ctrl Pts',(106.0079275809,-13.213640503243,67.6871553425417));
#141970=CARTESIAN_POINT('Ctrl Pts',(106.008771662554,-13.2134477302784,
67.6874045785535));
#141971=CARTESIAN_POINT('Ctrl Pts',(106.011353112438,-13.2128765343337,
67.6881335578442));
#141972=CARTESIAN_POINT('Ctrl Pts',(106.01169360327,-13.2128011941214,67.6882297095327));
#141973=CARTESIAN_POINT('Ctrl Pts',(106.012064263459,-13.2127192510605,
67.6883342516613));
#141974=CARTESIAN_POINT('Ctrl Pts',(106.01246908579,-13.2126297834597,67.6884483843945));
#141975=CARTESIAN_POINT('Ctrl Pts',(106.018706785095,-13.2112512231658,
67.6902069970421));
#141976=CARTESIAN_POINT('Ctrl Pts',(106.025629390392,-13.2098534637644,
67.6919178460703));
#141977=CARTESIAN_POINT('Ctrl Pts',(106.033070473643,-13.2084838648189,
67.693516276775));
#141978=CARTESIAN_POINT('Ctrl Pts',(106.039796379662,-13.2072459007375,
67.6949610791423));
#141979=CARTESIAN_POINT('Ctrl Pts',(106.046946255791,-13.2060309835752,
67.6963139902179));
#141980=CARTESIAN_POINT('Ctrl Pts',(106.054358327978,-13.2048662938512,
67.6975448752181));
#141981=CARTESIAN_POINT('Ctrl Pts',(106.057014045171,-13.2044489899657,
67.6979858966186));
#141982=CARTESIAN_POINT('Ctrl Pts',(106.059703006123,-13.2040380529815,
67.698411432947));
#141983=CARTESIAN_POINT('Ctrl Pts',(106.062416233874,-13.2036344373729,
67.6988207497283));
#141984=CARTESIAN_POINT('Ctrl Pts',(106.067640753954,-13.2028572457602,
67.6996089193695));
#141985=CARTESIAN_POINT('Ctrl Pts',(106.072917428486,-13.20210323266,67.7003487886868));
#141986=CARTESIAN_POINT('Ctrl Pts',(106.078291363442,-13.2013858193255,
67.7010093557201));
#141987=CARTESIAN_POINT('Ctrl Pts',(106.082994471742,-13.2007579604781,
67.7015874643728));
#141988=CARTESIAN_POINT('Ctrl Pts',(106.08777242606,-13.200158185367,67.7021047405022));
#141989=CARTESIAN_POINT('Ctrl Pts',(106.092620378955,-13.1995878076451,
67.7025577171331));
#141990=CARTESIAN_POINT('Ctrl Pts',(106.094961596148,-13.1993123556846,
67.7027764726986));
#141991=CARTESIAN_POINT('Ctrl Pts',(106.097318554236,-13.1990436338865,
67.7029805142864));
#141992=CARTESIAN_POINT('Ctrl Pts',(106.099686672438,-13.1987809372948,
67.7031713487706));
#141993=CARTESIAN_POINT('Ctrl Pts',(106.106306020717,-13.1980466495254,
67.7037047680541));
#141994=CARTESIAN_POINT('Ctrl Pts',(106.113015286185,-13.1973595556006,
67.7041346722277));
#141995=CARTESIAN_POINT('Ctrl Pts',(106.119760232682,-13.1967182146413,
67.7044643428826));
#141996=CARTESIAN_POINT('Ctrl Pts',(106.120291884984,-13.1966676626618,
67.7044903282871));
#141997=CARTESIAN_POINT('Ctrl Pts',(106.120823733892,-13.196617393249,67.7045156950284));
#141998=CARTESIAN_POINT('Ctrl Pts',(106.121355741848,-13.1965674055061,
67.7045404452821));
#141999=CARTESIAN_POINT('Ctrl Pts',(106.126806388336,-13.1960552599398,
67.704794022098));
#142000=CARTESIAN_POINT('Ctrl Pts',(106.132300873379,-13.1955789258494,
67.7049683496596));
#142001=CARTESIAN_POINT('Ctrl Pts',(106.137816755595,-13.1951304042744,
67.7050744113511));
#142002=CARTESIAN_POINT('Ctrl Pts',(106.142627707291,-13.1947392038194,
67.7051669183437));
#142003=CARTESIAN_POINT('Ctrl Pts',(106.147452442908,-13.1943684627235,
67.7052090760339));
#142004=CARTESIAN_POINT('Ctrl Pts',(106.15229430885,-13.1940239170325,67.705183407132));
#142005=CARTESIAN_POINT('Ctrl Pts',(106.154293195483,-13.1938816768746,
67.7051728101379));
#142006=CARTESIAN_POINT('Ctrl Pts',(106.156057216663,-13.1937568448576,
67.7051595416078));
#142007=CARTESIAN_POINT('Ctrl Pts',(106.157935224526,-13.1936307172706,
67.7051301165763));
#142008=CARTESIAN_POINT('Ctrl Pts',(106.159344479978,-13.1935360712399,
67.7051080360584));
#142009=CARTESIAN_POINT('Ctrl Pts',(106.160816586509,-13.1934404193615,
67.7050774867419));
#142010=CARTESIAN_POINT('Ctrl Pts',(106.162480765056,-13.1933340722082,
67.7050369249592));
#142011=CARTESIAN_POINT('Ctrl Pts',(106.164364380857,-13.1932137022041,
67.7049910147323));
#142012=CARTESIAN_POINT('Ctrl Pts',(106.166494087513,-13.1930794657017,
67.7049328065703));
#142013=CARTESIAN_POINT('Ctrl Pts',(106.169036390997,-13.192916817047,67.7048600150695));
#142014=CARTESIAN_POINT('Ctrl Pts',(106.173988369297,-13.1926000049064,
67.7047182295057));
#142015=CARTESIAN_POINT('Ctrl Pts',(106.1787882912,-13.1922750737932,67.7045866164252));
#142016=CARTESIAN_POINT('Ctrl Pts',(106.183439168815,-13.1919492595683,
67.7044538112829));
#142017=CARTESIAN_POINT('Ctrl Pts',(106.18609681466,-13.1917630799065,67.7043779225876));
#142018=CARTESIAN_POINT('Ctrl Pts',(106.188706333932,-13.191576536862,67.7043018744545));
#142019=CARTESIAN_POINT('Ctrl Pts',(106.191262452227,-13.1913884722509,
67.7042303695505));
#142020=CARTESIAN_POINT('Ctrl Pts',(106.19531464786,-13.191090334799,67.7041170133492));
#142021=CARTESIAN_POINT('Ctrl Pts',(106.199200076115,-13.1907929689485,
67.7040122321995));
#142022=CARTESIAN_POINT('Ctrl Pts',(106.202979797795,-13.1905041748381,
67.7038985058269));
#142023=CARTESIAN_POINT('Ctrl Pts',(106.204080645818,-13.1904200632415,
67.703865382898));
#142024=CARTESIAN_POINT('Ctrl Pts',(106.205172202955,-13.1903366268841,
67.703831634868));
#142025=CARTESIAN_POINT('Ctrl Pts',(106.206255281634,-13.1902539498646,
67.7037971082059));
#142026=CARTESIAN_POINT('Ctrl Pts',(106.210961647814,-13.189894688496,67.7036470774486));
#142027=CARTESIAN_POINT('Ctrl Pts',(106.21550436911,-13.1895485333888,67.7034855994441));
#142028=CARTESIAN_POINT('Ctrl Pts',(106.219845269805,-13.1892023369266,
67.7033519059895));
#142029=CARTESIAN_POINT('Ctrl Pts',(106.224742564287,-13.1888117668255,
67.7032010764121));
#142030=CARTESIAN_POINT('Ctrl Pts',(106.229383204607,-13.1884212700987,
67.7030852992312));
#142031=CARTESIAN_POINT('Ctrl Pts',(106.233759144139,-13.1880288718173,
67.7030159462491));
#142032=CARTESIAN_POINT('Ctrl Pts',(106.2387553242,-13.1875808554644,67.7029367632569));
#142033=CARTESIAN_POINT('Ctrl Pts',(106.243406787408,-13.1871305335341,
67.7029176584391));
#142034=CARTESIAN_POINT('Ctrl Pts',(106.247754302878,-13.1866931537782,
67.7029267676943));
#142035=CARTESIAN_POINT('Ctrl Pts',(106.251285121241,-13.186337937452,67.7029341657417));
#142036=CARTESIAN_POINT('Ctrl Pts',(106.254616705439,-13.1859916872872,
67.7029590202608));
#142037=CARTESIAN_POINT('Ctrl Pts',(106.257788816691,-13.1856684565596,
67.7029683476007));
#142038=CARTESIAN_POINT('Ctrl Pts',(106.263348662761,-13.1851019212311,
67.7029846958843));
#142039=CARTESIAN_POINT('Ctrl Pts',(106.268332466383,-13.1845596796241,
67.7030583307742));
#142040=CARTESIAN_POINT('Ctrl Pts',(106.272752463344,-13.1840366895586,
67.7032011751615));
#142041=CARTESIAN_POINT('Ctrl Pts',(106.274940771102,-13.1837777610508,
67.7032718963597));
#142042=CARTESIAN_POINT('Ctrl Pts',(106.276991551938,-13.1835237709647,
67.7033589856214));
#142043=CARTESIAN_POINT('Ctrl Pts',(106.278909589549,-13.1832751579372,
67.7034610233969));
#142044=CARTESIAN_POINT('Ctrl Pts',(106.281805657742,-13.1828997741193,
67.7036150914685));
#142045=CARTESIAN_POINT('Ctrl Pts',(106.28439497079,-13.1825356113142,67.7038060310672));
#142046=CARTESIAN_POINT('Ctrl Pts',(106.28668290027,-13.182182080024,67.7040347302797));
#142047=CARTESIAN_POINT('Ctrl Pts',(106.28838368379,-13.1819192746371,67.7042047389513));
#142048=CARTESIAN_POINT('Ctrl Pts',(106.289172451088,-13.1818103688079,
67.7042586550601));
#142049=CARTESIAN_POINT('Ctrl Pts',(106.290712328531,-13.1815248738751,
67.7045027578366));
#142050=CARTESIAN_POINT('Ctrl Pts',(106.291243926355,-13.181426315067,67.7045870272085));
#142051=CARTESIAN_POINT('Ctrl Pts',(106.291865315224,-13.1813067816776,
67.7046937549635));
#142052=CARTESIAN_POINT('Ctrl Pts',(106.29264608939,-13.1811529706491,67.7048346699659));
#142053=CARTESIAN_POINT('Ctrl Pts',(106.308230747469,-13.1780828225921,
67.7076474066395));
#142054=CARTESIAN_POINT('Ctrl Pts',(106.325794339231,-13.174397015322,67.7112173579816));
#142055=CARTESIAN_POINT('Ctrl Pts',(106.34552537209,-13.1700711157576,67.7155433191232));
#142056=CARTESIAN_POINT('Ctrl Pts',(106.356609505867,-13.1676409921134,
67.7179734773591));
#142057=CARTESIAN_POINT('Ctrl Pts',(106.368378129295,-13.1650086066466,
67.7206425875831));
#142058=CARTESIAN_POINT('Ctrl Pts',(106.380848846052,-13.1621681033657,
67.7235563945947));
#142059=CARTESIAN_POINT('Ctrl Pts',(106.390746763908,-13.1599136164191,
67.7258690621831));
#142060=CARTESIAN_POINT('Ctrl Pts',(106.401669238631,-13.1573934798774,
67.728475184187));
#142061=CARTESIAN_POINT('Ctrl Pts',(106.412902229041,-13.1547957200748,
67.7311586306529));
#142062=CARTESIAN_POINT('Ctrl Pts',(106.421342471128,-13.1528438158342,
67.7331749181213));
#142063=CARTESIAN_POINT('Ctrl Pts',(106.429956610801,-13.1508478008114,
67.7352358032063));
#142064=CARTESIAN_POINT('Ctrl Pts',(106.43842557944,-13.1488848065073,67.7372594300533));
#142065=CARTESIAN_POINT('Ctrl Pts',(106.458165770223,-13.1443092928029,
67.7419762712338));
#142066=CARTESIAN_POINT('Ctrl Pts',(106.47783830857,-13.1397336851529,67.7466869839844));
#142067=CARTESIAN_POINT('Ctrl Pts',(106.497415498927,-13.1351634667802,
67.7513934960968));
#142068=CARTESIAN_POINT('Ctrl Pts',(106.517010927316,-13.1305889908104,
67.7561043927769));
#142069=CARTESIAN_POINT('Ctrl Pts',(106.536598800992,-13.1260326377809,
67.7607696183555));
#142070=CARTESIAN_POINT('Ctrl Pts',(106.556115761675,-13.1214660922766,
67.7654617021941));
#142071=CARTESIAN_POINT('Ctrl Pts',(106.614593983727,-13.1077834566277,
67.7795204854777));
#142072=CARTESIAN_POINT('Ctrl Pts',(106.672439179494,-13.0940112378979,
67.7938147099477));
#142073=CARTESIAN_POINT('Ctrl Pts',(106.730750213752,-13.0801193452713,
67.8080999015867));
#142074=CARTESIAN_POINT('Ctrl Pts',(106.769636311969,-13.0708552067089,
67.8176263209374));
#142075=CARTESIAN_POINT('Ctrl Pts',(106.808539671188,-13.0615329788697,
67.8271947355138));
#142076=CARTESIAN_POINT('Ctrl Pts',(106.847463012598,-13.0521360046979,
67.8368067246768));
#142077=CARTESIAN_POINT('Ctrl Pts',(106.866924683304,-13.0474375176119,
67.8416127192583));
#142078=CARTESIAN_POINT('Ctrl Pts',(106.886392130002,-13.0427202088031,
67.8464296643369));
#142079=CARTESIAN_POINT('Ctrl Pts',(106.905867009676,-13.0379817218561,
67.8512578091657));
#142080=CARTESIAN_POINT('Ctrl Pts',(106.910735729595,-13.0367971001194,
67.8524648453729));
#142081=CARTESIAN_POINT('Ctrl Pts',(106.915604914056,-13.0356111545458,
67.8536725814496));
#142082=CARTESIAN_POINT('Ctrl Pts',(106.920474588092,-13.0344238482103,
67.8548810207559));
#142083=CARTESIAN_POINT('Ctrl Pts',(106.925344262128,-13.0332365418749,
67.8560894600622));
#142084=CARTESIAN_POINT('Ctrl Pts',(106.930697157267,-13.031927921499,67.8574217098111));
#142085=CARTESIAN_POINT('Ctrl Pts',(106.931726432134,-13.0316795015703,
67.8576719813984));
#142086=CARTESIAN_POINT('Ctrl Pts',(106.933784981867,-13.0311826617128,
67.8581725245729));
#142087=CARTESIAN_POINT('Ctrl Pts',(106.936923967831,-13.0304423944958,
67.8589040957394));
#142088=CARTESIAN_POINT('Ctrl Pts',(106.94114463868,-13.0294576651308,67.8598669197149));
#142089=CARTESIAN_POINT('Ctrl Pts',(106.950441317851,-13.0272886466725,
67.8619876881709));
#142090=CARTESIAN_POINT('Ctrl Pts',(106.9649906445,-13.0239350581153,67.8652288807271));
#142091=CARTESIAN_POINT('Ctrl Pts',(106.984801432774,-13.0193731607089,
67.8695970565263));
#142092=CARTESIAN_POINT('Ctrl Pts',(107.000966852782,-13.0156506946166,
67.8731614475788));
#142093=CARTESIAN_POINT('Ctrl Pts',(107.020635638888,-13.0111238244378,
67.8774751049033));
#142094=CARTESIAN_POINT('Ctrl Pts',(107.043812218085,-13.0057758568377,
67.8825361178667));
#142095=CARTESIAN_POINT('Ctrl Pts',(107.069602003937,-12.9998248949646,
67.8881677703815));
#142096=CARTESIAN_POINT('Ctrl Pts',(107.099727177575,-12.9928579994466,
67.8947252155551));
#142097=CARTESIAN_POINT('Ctrl Pts',(107.134152385793,-12.98485017791,67.9022020853204));
#142098=CARTESIAN_POINT('Ctrl Pts',(107.151364989902,-12.9808462671417,
67.9059405202031));
#142099=CARTESIAN_POINT('Ctrl Pts',(107.169653865867,-12.9765817338447,
67.9099090152389));
#142100=CARTESIAN_POINT('Ctrl Pts',(107.1890184561,-12.9720518542785,67.9141073841192));
#142101=CARTESIAN_POINT('Ctrl Pts',(107.198700751216,-12.9697869144955,
67.9162065685594));
#142102=CARTESIAN_POINT('Ctrl Pts',(107.208651974163,-12.9674556316093,
67.9183632178064));
#142103=CARTESIAN_POINT('Ctrl Pts',(107.218872157659,-12.9650573413603,
67.9205773271656));
#142104=CARTESIAN_POINT('Ctrl Pts',(107.223982249406,-12.9638581962358,
67.9216843818451));
#142105=CARTESIAN_POINT('Ctrl Pts',(107.229159581246,-12.9626422988637,
67.9228058013249));
#142106=CARTESIAN_POINT('Ctrl Pts',(107.234404161833,-12.9614095624508,
67.9239415850425));
#142107=CARTESIAN_POINT('Ctrl Pts',(107.237026452127,-12.9607931942444,
67.9245094769013));
#142108=CARTESIAN_POINT('Ctrl Pts',(107.239665554605,-12.9601726162525,
67.9250809598053));
#142109=CARTESIAN_POINT('Ctrl Pts',(107.242321470771,-12.9595478173416,
67.9256560337469));
#142110=CARTESIAN_POINT('Ctrl Pts',(107.243649428854,-12.9592354178861,
67.9259435707177));
#142111=CARTESIAN_POINT('Ctrl Pts',(107.24498159036,-12.9589219631993,67.9262320054471));
#142112=CARTESIAN_POINT('Ctrl Pts',(107.246317955505,-12.9586074518708,
67.9265213379387));
#142113=CARTESIAN_POINT('Ctrl Pts',(107.247654320651,-12.9582929405424,
67.9268106704303));
#142114=CARTESIAN_POINT('Ctrl Pts',(107.250177381402,-12.9576989554457,
67.9273568967762));
#142115=CARTESIAN_POINT('Ctrl Pts',(107.25033966209,-12.9576607465408,67.9273920287038));
#142116=CARTESIAN_POINT('Ctrl Pts',(107.263428087531,-12.9545790834838,
67.9302255242923));
#142117=CARTESIAN_POINT('Ctrl Pts',(107.286145037413,-12.9491868368947,
67.9352153777412));
#142118=CARTESIAN_POINT('Ctrl Pts',(107.318469490553,-12.9414271973423,
67.942368949705));
#142119=CARTESIAN_POINT('Ctrl Pts',(107.337445418838,-12.9368719350143,
67.9465684227163));
#142120=CARTESIAN_POINT('Ctrl Pts',(107.359732422305,-12.931500312654,67.9515128573504));
#142121=CARTESIAN_POINT('Ctrl Pts',(107.385329787984,-12.9252967084814,
67.957197178429));
#142122=CARTESIAN_POINT('Ctrl Pts',(107.393979922269,-12.9232003205242,
67.9591180847155));
#142123=CARTESIAN_POINT('Ctrl Pts',(107.403007784403,-12.9210087677287,
67.9611237406437));
#142124=CARTESIAN_POINT('Ctrl Pts',(107.412413111063,-12.9187212637526,
67.9632140784353));
#142125=CARTESIAN_POINT('Ctrl Pts',(107.413588776895,-12.9184353257555,
67.9634753706593));
#142126=CARTESIAN_POINT('Ctrl Pts',(107.414770340603,-12.9181478884549,
67.9637379859997));
#142127=CARTESIAN_POINT('Ctrl Pts',(107.415957801536,-12.9178589502324,
67.9640019243639));
#142128=CARTESIAN_POINT('Ctrl Pts',(107.417145262469,-12.9175700120099,
67.9642658627281));
#142129=CARTESIAN_POINT('Ctrl Pts',(107.421399590165,-12.9165345440671,
67.9652114953958));
#142130=CARTESIAN_POINT('Ctrl Pts',(107.424537922514,-12.9157701484059,
67.9659090759425));
#142131=CARTESIAN_POINT('Ctrl Pts',(107.430814587213,-12.9142413570834,
67.9673042370359));
#142132=CARTESIAN_POINT('Ctrl Pts',(107.43708970593,-12.9127112789761,67.9686990791321));
#142133=CARTESIAN_POINT('Ctrl Pts',(107.443363264349,-12.9111799206928,
67.970093600068));
#142134=CARTESIAN_POINT('Ctrl Pts',(107.455910381186,-12.9081172041261,
67.9728826419399));
#142135=CARTESIAN_POINT('Ctrl Pts',(107.468451256819,-12.9050493668033,
67.9756703991361));
#142136=CARTESIAN_POINT('Ctrl Pts',(107.480985748233,-12.901976467266,67.9784568517438));
#142137=CARTESIAN_POINT('Ctrl Pts',(107.531123713887,-12.8896848691169,
67.9896026621746));
#142138=CARTESIAN_POINT('Ctrl Pts',(107.581159531596,-12.877312267325,68.0007275954188));
#142139=CARTESIAN_POINT('Ctrl Pts',(107.631093001679,-12.8648609057211,
68.0118313415621));
#142140=CARTESIAN_POINT('Ctrl Pts',(107.695290512925,-12.8488526766662,
68.02610699408));
#142141=CARTESIAN_POINT('Ctrl Pts',(107.75930625601,-12.832715850264,68.0403476199207));
#142142=CARTESIAN_POINT('Ctrl Pts',(107.823178038429,-12.816449128691,68.0545552102772));
#142143=CARTESIAN_POINT('Ctrl Pts',(107.858666485858,-12.8074110108942,
68.0624492333398));
#142144=CARTESIAN_POINT('Ctrl Pts',(107.894110420149,-12.7983327871238,
68.0703330675227));
#142145=CARTESIAN_POINT('Ctrl Pts',(107.929507029907,-12.7892133079803,
68.0782085743562));
#142146=CARTESIAN_POINT('Ctrl Pts',(107.983521817539,-12.7752970958739,
68.0902265001408));
#142147=CARTESIAN_POINT('Ctrl Pts',(108.037442841,-12.7612838820349,68.1022230318144));
#142148=CARTESIAN_POINT('Ctrl Pts',(108.091265807375,-12.7471725434948,
68.1141982544549));
#142149=CARTESIAN_POINT('Ctrl Pts',(108.294350377707,-12.6939277055151,
68.1593831097012));
#142150=CARTESIAN_POINT('Ctrl Pts',(108.496034079401,-12.6392855691849,
68.2042656174757));
#142151=CARTESIAN_POINT('Ctrl Pts',(108.696127954478,-12.5831843055722,
68.248843918316));
#142152=CARTESIAN_POINT('Ctrl Pts',(108.832191396481,-12.5450355565164,
68.2791570753214));
#142153=CARTESIAN_POINT('Ctrl Pts',(108.967522039852,-12.5062122247552,
68.3093291886953));
#142154=CARTESIAN_POINT('Ctrl Pts',(109.102170552872,-12.4667056364051,
68.3393417122603));
#142155=CARTESIAN_POINT('Ctrl Pts',(109.453424423852,-12.363645886424,68.4176345566715));
#142156=CARTESIAN_POINT('Ctrl Pts',(109.799724391402,-12.2559464931104,
68.4948956137196));
#142157=CARTESIAN_POINT('Ctrl Pts',(110.140821024858,-12.1434889766497,
68.5710707710017));
#142158=CARTESIAN_POINT('Ctrl Pts',(110.173727741523,-12.1326398293169,
68.5784196395386));
#142159=CARTESIAN_POINT('Ctrl Pts',(110.206586003916,-12.1217464208938,
68.5857584201245));
#142160=CARTESIAN_POINT('Ctrl Pts',(110.239395571674,-12.1108086599221,
68.5930870754831));
#142161=CARTESIAN_POINT('Ctrl Pts',(110.345808727803,-12.0753335913508,
68.6168565244638));
#142162=CARTESIAN_POINT('Ctrl Pts',(110.451708902476,-12.0393922845856,
68.6405191617746));
#142163=CARTESIAN_POINT('Ctrl Pts',(110.557091482789,-12.0029811494992,
68.6640737449812));
#142164=CARTESIAN_POINT('Ctrl Pts',(110.636352799546,-11.9755952712735,
68.681789835013));
#142165=CARTESIAN_POINT('Ctrl Pts',(110.715321294688,-11.9479436164212,
68.6994447990933));
#142166=CARTESIAN_POINT('Ctrl Pts',(110.793993320436,-11.9200246667457,
68.7170379770568));
#142167=CARTESIAN_POINT('Ctrl Pts',(110.885628874946,-11.887505249449,68.7375301482316));
#142168=CARTESIAN_POINT('Ctrl Pts',(110.976862459063,-11.8546231658946,
68.7579384497065));
#142169=CARTESIAN_POINT('Ctrl Pts',(111.067688403721,-11.821376277975,68.7782617217179));
#142170=CARTESIAN_POINT('Ctrl Pts',(111.11310137605,-11.8047528340152,68.7884233577236));
#142171=CARTESIAN_POINT('Ctrl Pts',(111.158412439001,-11.7880381911324,
68.7985637379712));
#142172=CARTESIAN_POINT('Ctrl Pts',(111.203620891663,-11.7712321070967,
68.8086827088724));
#142173=CARTESIAN_POINT('Ctrl Pts',(111.226225117994,-11.7628290650789,
68.813742194323));
#142174=CARTESIAN_POINT('Ctrl Pts',(111.248803691776,-11.754403162908,68.8187963275252));
#142175=CARTESIAN_POINT('Ctrl Pts',(111.271356510201,-11.7459543749221,
68.8238450891866));
#142176=CARTESIAN_POINT('Ctrl Pts',(111.282632919414,-11.7417299809291,
68.8263694700173));
#142177=CARTESIAN_POINT('Ctrl Pts',(111.293902889791,-11.737499865492,68.8288925079705));
#142178=CARTESIAN_POINT('Ctrl Pts',(111.305166409589,-11.7332640252594,
68.8314142006312));
#142179=CARTESIAN_POINT('Ctrl Pts',(111.315021989413,-11.7295576650559,
68.8336206817094));
#142180=CARTESIAN_POINT('Ctrl Pts',(111.324872630526,-11.7258469218158,
68.8358261327756));
#142181=CARTESIAN_POINT('Ctrl Pts',(111.334718215831,-11.7221317721431,
68.8380306137598));
#142182=CARTESIAN_POINT('Ctrl Pts',(111.336124728018,-11.7216010364755,
68.8383455396147));
#142183=CARTESIAN_POINT('Ctrl Pts',(111.337531120636,-11.7210703090457,
68.8386605681555));
#142184=CARTESIAN_POINT('Ctrl Pts',(111.340784955608,-11.7198418175818,
68.8393889026379));
#142185=CARTESIAN_POINT('Ctrl Pts',(111.676598330681,-11.5930548513553,
68.9145569621135));
#142186=CARTESIAN_POINT('Ctrl Pts',(112.010698132989,-11.4596490571931,
68.9894187938631));
#142187=CARTESIAN_POINT('Ctrl Pts',(112.342633408572,-11.3190643094168,
69.0638575505441));
#142188=CARTESIAN_POINT('Ctrl Pts',(112.566856914298,-11.2240987925921,
69.114141205861));
#142189=CARTESIAN_POINT('Ctrl Pts',(112.790091959944,-11.1258569855089,
69.1642315263753));
#142190=CARTESIAN_POINT('Ctrl Pts',(113.012189026206,-11.0241600292873,
69.2140865598598));
#142191=CARTESIAN_POINT('Ctrl Pts',(113.289691953154,-10.8970930513742,
69.2763787726652));
#142192=CARTESIAN_POINT('Ctrl Pts',(113.565421268222,-10.7646317480393,
69.3383038963364));
#142193=CARTESIAN_POINT('Ctrl Pts',(113.838972335797,-10.6264708943272,
69.3997865989108));
#142194=CARTESIAN_POINT('Ctrl Pts',(114.104544539504,-10.4923398791873,
69.4594759905747));
#142195=CARTESIAN_POINT('Ctrl Pts',(114.368063772043,-10.3528368900573,
69.5187486148448));
#142196=CARTESIAN_POINT('Ctrl Pts',(114.629112607753,-10.2076787365451,
69.5775221736678));
#142197=CARTESIAN_POINT('Ctrl Pts',(114.721749901965,-10.1561670776727,
69.5983788974519));
#142198=CARTESIAN_POINT('Ctrl Pts',(114.81407565261,-10.1039432332318,69.6191726327996));
#142199=CARTESIAN_POINT('Ctrl Pts',(114.906069691261,-10.0509944466622,
69.6398991964471));
#142200=CARTESIAN_POINT('Ctrl Pts',(115.158260743509,-9.90584145201093,
69.6967186814093));
#142201=CARTESIAN_POINT('Ctrl Pts',(115.407962187416,-9.75524064263987,
69.7530347717736));
#142202=CARTESIAN_POINT('Ctrl Pts',(115.654720644459,-9.59893015320212,
69.8087507530049));
#142203=CARTESIAN_POINT('Ctrl Pts',(115.820069278053,-9.49418916010859,
69.8460850817907));
#142204=CARTESIAN_POINT('Ctrl Pts',(115.984095575379,-9.38688437968712,
69.8831495949633));
#142205=CARTESIAN_POINT('Ctrl Pts',(116.146651119149,-9.27693621160278,
69.9199097730351));
#142206=CARTESIAN_POINT('Ctrl Pts',(116.370838736652,-9.1253017777346,69.9706073779878));
#142207=CARTESIAN_POINT('Ctrl Pts',(116.59227521728,-8.96861412888962,70.0207329109146));
#142208=CARTESIAN_POINT('Ctrl Pts',(116.810505003658,-8.80664115597571,
70.0702052203824));
#142209=CARTESIAN_POINT('Ctrl Pts',(117.023958781536,-8.64821299840652,
70.1185948171075));
#142210=CARTESIAN_POINT('Ctrl Pts',(117.234345143066,-8.48472837853567,
70.1663595531027));
#142211=CARTESIAN_POINT('Ctrl Pts',(117.441174068438,-8.31595777817756,
70.2134049767224));
#142212=CARTESIAN_POINT('Ctrl Pts',(117.642407602492,-8.15175296836516,
70.2591776694877));
#142213=CARTESIAN_POINT('Ctrl Pts',(117.840273614692,-7.98254426435186,
70.3042696055394));
#142214=CARTESIAN_POINT('Ctrl Pts',(118.0342763988,-7.80811648244908,70.3485728169649));
#142215=CARTESIAN_POINT('Ctrl Pts',(118.123449679351,-7.72794084165549,
70.3689367654512));
#142216=CARTESIAN_POINT('Ctrl Pts',(118.211806116165,-7.64666247736764,
70.3891337632917));
#142217=CARTESIAN_POINT('Ctrl Pts',(118.299294254877,-7.56426025759235,
70.4091516254367));
#142218=CARTESIAN_POINT('Ctrl Pts',(118.489293739946,-7.38530594954026,
70.4526247585464));
#142219=CARTESIAN_POINT('Ctrl Pts',(118.67518421981,-7.20105610757558,70.4952581234905));
#142220=CARTESIAN_POINT('Ctrl Pts',(118.856312446238,-7.01133104918698,
70.5369285437103));
#142221=CARTESIAN_POINT('Ctrl Pts',(118.99619198796,-6.86481244883354,70.569109277761));
#142222=CARTESIAN_POINT('Ctrl Pts',(119.133230427345,-6.71502846719137,
70.6007154059949));
#142223=CARTESIAN_POINT('Ctrl Pts',(119.267107529061,-6.56189725353795,
70.6316812677236));
#142224=CARTESIAN_POINT('Ctrl Pts',(119.383489889386,-6.42877686285118,
70.6586005842556));
#142225=CARTESIAN_POINT('Ctrl Pts',(119.497465439713,-6.29314640495762,
70.6850316807826));
#142226=CARTESIAN_POINT('Ctrl Pts',(119.6087870881,-6.15498623441501,70.7109234456726));
#142227=CARTESIAN_POINT('Ctrl Pts',(119.6444020833,-6.11078482451875,70.7192069655057));
#142228=CARTESIAN_POINT('Ctrl Pts',(119.67974539263,-6.06632450162849,70.7274352643774));
#142229=CARTESIAN_POINT('Ctrl Pts',(119.714807140622,-6.02160798752607,
70.7356067925721));
#142230=CARTESIAN_POINT('Ctrl Pts',(119.787134197516,-5.92936461562263,
70.7524634132056));
#142231=CARTESIAN_POINT('Ctrl Pts',(119.858268463629,-5.83602393539941,
70.7690801116031));
#142232=CARTESIAN_POINT('Ctrl Pts',(119.928141526215,-5.74158973693852,
70.7854436423368));
#142233=CARTESIAN_POINT('Ctrl Pts',(119.963078057509,-5.69437263770807,
70.7936254077037));
#142234=CARTESIAN_POINT('Ctrl Pts',(119.99769927408,-5.64688214208205,70.8017438526601));
#142235=CARTESIAN_POINT('Ctrl Pts',(120.03199650483,-5.59911866729075,70.8097971234142));
#142236=CARTESIAN_POINT('Ctrl Pts',(120.049145120205,-5.5752369298951,70.8138237587912));
#142237=CARTESIAN_POINT('Ctrl Pts',(120.066212738068,-5.55128694670323,
70.8178340985175));
#142238=CARTESIAN_POINT('Ctrl Pts',(120.083198268887,-5.52726876482581,
70.8218278966712));
#142239=CARTESIAN_POINT('Ctrl Pts',(120.098060608353,-5.50625285568306,
70.8253224700557));
#142240=CARTESIAN_POINT('Ctrl Pts',(120.112860099865,-5.48518473185981,
70.8288043786772));
#142241=CARTESIAN_POINT('Ctrl Pts',(120.127596010453,-5.46406442325504,
70.8322734515337));
#142242=CARTESIAN_POINT('Ctrl Pts',(120.129701140537,-5.4610472363115,70.8327690333704));
#142243=CARTESIAN_POINT('Ctrl Pts',(120.132551182633,-5.4569573991032,70.8334400539826));
#142244=CARTESIAN_POINT('Ctrl Pts',(120.133907505838,-5.45500966753072,
70.8337594106343));
#142245=CARTESIAN_POINT('Ctrl Pts',(120.250042395984,-5.28823555987381,
70.8611042570002));
#142246=CARTESIAN_POINT('Ctrl Pts',(120.360277472768,-5.12122346206651,
70.8870716294798));
#142247=CARTESIAN_POINT('Ctrl Pts',(120.464639371518,-4.95442575006959,
70.9116486720203));
#142248=CARTESIAN_POINT('Ctrl Pts',(120.520202986649,-4.86562050615205,
70.9247338050923));
#142249=CARTESIAN_POINT('Ctrl Pts',(120.574102616812,-4.77687589085944,
70.9374249284167));
#142250=CARTESIAN_POINT('Ctrl Pts',(120.626348178696,-4.68825898388539,
70.9497208309657));
#142251=CARTESIAN_POINT('Ctrl Pts',(120.723100044827,-4.5241522002407,70.9724912151761));
#142252=CARTESIAN_POINT('Ctrl Pts',(120.814176502228,-4.36048177456388,
70.9939065657032));
#142253=CARTESIAN_POINT('Ctrl Pts',(120.899680756234,-4.19745355593584,
71.0140330377286));
#142254=CARTESIAN_POINT('Ctrl Pts',(120.94056301105,-4.11950467194616,71.0236561327133));
#142255=CARTESIAN_POINT('Ctrl Pts',(120.980172134073,-4.04170283677841,
71.0329845449487));
#142256=CARTESIAN_POINT('Ctrl Pts',(121.018523425566,-3.96407181115534,
71.0420253267797));
#142257=CARTESIAN_POINT('Ctrl Pts',(121.099100190346,-3.80096760664018,
71.0610201747404));
#142258=CARTESIAN_POINT('Ctrl Pts',(121.1740756497,-3.63888509553889,71.0786695045519));
#142259=CARTESIAN_POINT('Ctrl Pts',(121.243628132454,-3.47805224050065,
71.0950745582767));
#142260=CARTESIAN_POINT('Ctrl Pts',(121.290992880891,-3.36852620465547,
71.1062462837421));
#142261=CARTESIAN_POINT('Ctrl Pts',(121.335843774898,-3.25958000608234,
71.1168408835626));
#142262=CARTESIAN_POINT('Ctrl Pts',(121.378250394056,-3.15128934077509,
71.1268891787873));
#142263=CARTESIAN_POINT('Ctrl Pts',(121.43227088005,-3.01334119766261,71.1396893925801));
#142264=CARTESIAN_POINT('Ctrl Pts',(121.482324676729,-2.87646114422512,
71.1516021824958));
#142265=CARTESIAN_POINT('Ctrl Pts',(121.528620957139,-2.7410992539322,71.162625975379));
#142266=CARTESIAN_POINT('Ctrl Pts',(121.553709517772,-2.6677448729351,71.1685999131058));
#142267=CARTESIAN_POINT('Ctrl Pts',(121.577694962148,-2.59483551362207,
71.1743129425307));
#142268=CARTESIAN_POINT('Ctrl Pts',(121.600612981877,-2.52243699463433,
71.1797659749776));
#142269=CARTESIAN_POINT('Ctrl Pts',(121.64447704994,-2.3838694568596,71.1902028359817));
#142270=CARTESIAN_POINT('Ctrl Pts',(121.684455689974,-2.24700129479839,
71.1997183239856));
#142271=CARTESIAN_POINT('Ctrl Pts',(121.72077379674,-2.11198800006035,71.2083759721307));
#142272=CARTESIAN_POINT('Ctrl Pts',(121.758884318929,-1.97031136482238,
71.2174609030676));
#142273=CARTESIAN_POINT('Ctrl Pts',(121.792964243599,-1.83067690477613,
71.2256013439609));
#142274=CARTESIAN_POINT('Ctrl Pts',(121.823259728927,-1.69320953569154,
71.2328601754872));
#142275=CARTESIAN_POINT('Ctrl Pts',(121.833105683649,-1.64853299471043,
71.2352192770422));
#142276=CARTESIAN_POINT('Ctrl Pts',(121.842551798816,-1.60408495489313,
71.2374851732322));
#142277=CARTESIAN_POINT('Ctrl Pts',(121.851606188792,-1.55986862758669,
71.2396597694634));
#142278=CARTESIAN_POINT('Ctrl Pts',(121.877212802925,-1.4348209507498,71.2458097195688));
#142279=CARTESIAN_POINT('Ctrl Pts',(121.899687221721,-1.31162984135314,
71.251229551335));
#142280=CARTESIAN_POINT('Ctrl Pts',(121.919209628913,-1.19044907925386,
71.2559200140058));
#142281=CARTESIAN_POINT('Ctrl Pts',(121.941356854127,-1.05297537514837,
71.2612411166804));
#142282=CARTESIAN_POINT('Ctrl Pts',(121.959684929351,-0.917991321981767,
71.2656471422445));
#142283=CARTESIAN_POINT('Ctrl Pts',(121.974343097486,-0.785644001935815,
71.2691750218849));
#142284=CARTESIAN_POINT('Ctrl Pts',(121.990228746996,-0.642213859750984,
71.2729983277007));
#142285=CARTESIAN_POINT('Ctrl Pts',(122.001804504546,-0.501879910786403,
71.2757906643818));
#142286=CARTESIAN_POINT('Ctrl Pts',(122.00923088834,-0.364773384560142,
71.2775855021344));
#142287=CARTESIAN_POINT('Ctrl Pts',(122.015963003551,-0.24048450366651,
71.2792125463153));
#142288=CARTESIAN_POINT('Ctrl Pts',(122.019284931663,-0.118846386916853,
71.2800198326534));
#142289=CARTESIAN_POINT('Ctrl Pts',(122.019294419317,7.00634560479863E-5,
71.2800197814689));
#142290=CARTESIAN_POINT('Ctrl Pts',(105.189140139769,-13.40679170556,67.435700227319));
#142291=CARTESIAN_POINT('Ctrl Pts',(105.299653563669,-13.41337593904,67.406356677722));
#142292=CARTESIAN_POINT('Ctrl Pts',(105.401917646169,-13.41098220979,67.394906186081));
#142293=CARTESIAN_POINT('Ctrl Pts',(105.556077554169,-13.41563420522,67.36049564276));
#142294=CARTESIAN_POINT('Ctrl Pts',(105.693195182669,-13.42587977367,67.321725313285));
#142295=CARTESIAN_POINT('Ctrl Pts',(105.787908303369,-13.42998293955,67.302642707235));
#142296=CARTESIAN_POINT('Ctrl Pts',(105.843699474669,-13.42556821351,67.304299111144));
#142297=CARTESIAN_POINT('Ctrl Pts',(105.901721494369,-13.41833028344,67.309756553462));
#142298=CARTESIAN_POINT('Ctrl Pts',(105.999937763269,-13.41754327638,67.292509415534));
#142299=CARTESIAN_POINT('Ctrl Pts',(106.191477591769,-13.42342170879,67.242225690654));
#142300=CARTESIAN_POINT('Ctrl Pts',(106.517706045669,-13.42874124418,67.170350527559));
#142301=CARTESIAN_POINT('Ctrl Pts',(106.972945214669,-13.43533245482,67.064406479912));
#142302=CARTESIAN_POINT('Ctrl Pts',(107.704900537069,-13.44597315009,66.883611271943));
#142303=CARTESIAN_POINT('Ctrl Pts',(108.977104518069,-13.46320029547,66.539642935235));
#142304=CARTESIAN_POINT('Ctrl Pts',(110.926077218569,-13.48513863723,65.918375229425));
#142305=CARTESIAN_POINT('Ctrl Pts',(112.473091744269,-13.49504460676,65.294246012061));
#142306=CARTESIAN_POINT('Ctrl Pts',(113.297333561069,-13.49824966426,64.913239003008));
#142307=CARTESIAN_POINT('Ctrl Pts',(105.478427326569,-13.19592113931,67.814696830677));
#142308=CARTESIAN_POINT('Ctrl Pts',(105.591643512169,-13.20306212524,67.784735120544));
#142309=CARTESIAN_POINT('Ctrl Pts',(105.695005130969,-13.2003702312,67.773227229612));
#142310=CARTESIAN_POINT('Ctrl Pts',(105.852272395169,-13.20541340111,67.738120811063));
#142311=CARTESIAN_POINT('Ctrl Pts',(105.993070604769,-13.21654104784,67.698517329733));
#142312=CARTESIAN_POINT('Ctrl Pts',(106.089820788269,-13.22091338784,67.679141475208));
#142313=CARTESIAN_POINT('Ctrl Pts',(106.145526268469,-13.21592737404,67.681167947591));
#142314=CARTESIAN_POINT('Ctrl Pts',(106.202588490469,-13.20778342815,67.687361817172));
#142315=CARTESIAN_POINT('Ctrl Pts',(106.301625528069,-13.20677245091,67.670083535681));
#142316=CARTESIAN_POINT('Ctrl Pts',(106.497013492869,-13.21312249052,67.618572997914));
#142317=CARTESIAN_POINT('Ctrl Pts',(106.828733086469,-13.21866923959,67.545296939605));
#142318=CARTESIAN_POINT('Ctrl Pts',(107.291294977669,-13.22548051179,67.437274779936));
#142319=CARTESIAN_POINT('Ctrl Pts',(108.035171310469,-13.23648940418,67.252647434483));
#142320=CARTESIAN_POINT('Ctrl Pts',(109.327875563169,-13.2542371189,66.900862712001));
#142321=CARTESIAN_POINT('Ctrl Pts',(111.307648267369,-13.27658471517,66.264026081233));
#142322=CARTESIAN_POINT('Ctrl Pts',(112.877927795969,-13.28622829001,65.622947147765));
#142323=CARTESIAN_POINT('Ctrl Pts',(113.714069025669,-13.2891351954,65.231473861432));
#142324=CARTESIAN_POINT('Ctrl Pts',(106.340768199269,-12.49617988855,68.938679513356));
#142325=CARTESIAN_POINT('Ctrl Pts',(106.461348540569,-12.50489810892,68.907399560009));
#142326=CARTESIAN_POINT('Ctrl Pts',(106.568694932869,-12.50140712085,68.895202904603));
#142327=CARTESIAN_POINT('Ctrl Pts',(106.735211577569,-12.50762735198,68.8582212536));
#142328=CARTESIAN_POINT('Ctrl Pts',(106.886027864869,-12.52127083058,68.816883431501));
#142329=CARTESIAN_POINT('Ctrl Pts',(106.988265476969,-12.52637208736,68.7968524246));
#142330=CARTESIAN_POINT('Ctrl Pts',(107.043686493669,-12.51965320266,68.799585472983));
#142331=CARTESIAN_POINT('Ctrl Pts',(107.098110445069,-12.50876138298,68.807353899232));
#142332=CARTESIAN_POINT('Ctrl Pts',(107.199726651269,-12.50704598615,68.789813299972));
#142333=CARTESIAN_POINT('Ctrl Pts',(107.406494709669,-12.51480155187,68.734910758024));
#142334=CARTESIAN_POINT('Ctrl Pts',(107.754339071769,-12.52098631199,68.657515777145));
#142335=CARTESIAN_POINT('Ctrl Pts',(108.238521910769,-12.5283887722,68.543365540915));
#142336=CARTESIAN_POINT('Ctrl Pts',(109.017525905269,-12.54039893825,68.347482153695));
#142337=CARTESIAN_POINT('Ctrl Pts',(110.370669954069,-12.55953474246,67.972787846649));
#142338=CARTESIAN_POINT('Ctrl Pts',(112.441188500469,-12.58287697068,67.290442003463));
#142339=CARTESIAN_POINT('Ctrl Pts',(114.080031548069,-12.59161918337,66.599933992995));
#142340=CARTESIAN_POINT('Ctrl Pts',(114.951331881769,-12.59359707781,66.177945211323));
#142341=CARTESIAN_POINT('Ctrl Pts',(107.705305680269,-11.02502719391,70.672420612353));
#142342=CARTESIAN_POINT('Ctrl Pts',(107.833381308469,-11.03528783259,70.641686343356));
#142343=CARTESIAN_POINT('Ctrl Pts',(107.951392073669,-11.03147444739,70.625804113145));
#142344=CARTESIAN_POINT('Ctrl Pts',(108.132218771569,-11.03935848219,70.586956173343));
#142345=CARTESIAN_POINT('Ctrl Pts',(108.293216363269,-11.05563644096,70.546564593204));
#142346=CARTESIAN_POINT('Ctrl Pts',(108.400946594669,-11.06130905076,70.526510377485));
#142347=CARTESIAN_POINT('Ctrl Pts',(108.456184132269,-11.05215576087,70.528338166625));
#142348=CARTESIAN_POINT('Ctrl Pts',(108.508445485069,-11.03741701809,70.535283131199));
#142349=CARTESIAN_POINT('Ctrl Pts',(108.615264948969,-11.0346333001,70.516278570094));
#142350=CARTESIAN_POINT('Ctrl Pts',(108.839308569169,-11.04433520867,70.457395905042));
#142351=CARTESIAN_POINT('Ctrl Pts',(109.211536657569,-11.05132191043,70.373703522875));
#142352=CARTESIAN_POINT('Ctrl Pts',(109.729138867969,-11.05938103001,70.250016451));
#142353=CARTESIAN_POINT('Ctrl Pts',(110.561966036269,-11.072549911,70.03691849479));
#142354=CARTESIAN_POINT('Ctrl Pts',(112.007824449569,-11.09321823243,69.627472483783));
#142355=CARTESIAN_POINT('Ctrl Pts',(114.216996636269,-11.11743227536,68.876876679782));
#142356=CARTESIAN_POINT('Ctrl Pts',(115.960380806369,-11.12475694542,68.113039813493));
#142357=CARTESIAN_POINT('Ctrl Pts',(116.885619574069,-11.12546079243,67.64590027152));
#142358=CARTESIAN_POINT('Ctrl Pts',(109.191315175669,-8.78258410338099,
72.435524489286));
#142359=CARTESIAN_POINT('Ctrl Pts',(109.318496917169,-8.79074914635699,
72.409211353215));
#142360=CARTESIAN_POINT('Ctrl Pts',(109.457842018369,-8.79007298746399,
72.3857653537551));
#142361=CARTESIAN_POINT('Ctrl Pts',(109.652915194969,-8.79836367012399,
72.3469077691189));
#142362=CARTESIAN_POINT('Ctrl Pts',(109.812649879569,-8.81202888418299,
72.3129069755914));
#142363=CARTESIAN_POINT('Ctrl Pts',(109.920220140069,-8.81641528675999,
72.2941525170867));
#142364=CARTESIAN_POINT('Ctrl Pts',(109.977236747169,-8.80705067009099,
72.2917242776799));
#142365=CARTESIAN_POINT('Ctrl Pts',(110.033657601769,-8.79212768276199,
72.2920076171935));
#142366=CARTESIAN_POINT('Ctrl Pts',(110.149585959269,-8.78926868864499,
72.269245222296));
#142367=CARTESIAN_POINT('Ctrl Pts',(110.390312409269,-8.79939079703399,
72.208516320971));
#142368=CARTESIAN_POINT('Ctrl Pts',(110.787643550469,-8.80677737047199,
72.1183221609802));
#142369=CARTESIAN_POINT('Ctrl Pts',(111.341319341869,-8.81519511236299,
71.984258610211));
#142370=CARTESIAN_POINT('Ctrl Pts',(112.231076887069,-8.82897614512199,
71.753069698651));
#142371=CARTESIAN_POINT('Ctrl Pts',(113.775050360169,-8.85050085119999,
71.307507313673));
#142372=CARTESIAN_POINT('Ctrl Pts',(116.129334143269,-8.87550178253899,
70.487298823422));
#142373=CARTESIAN_POINT('Ctrl Pts',(117.980858361269,-8.88284629712299,
69.650145847141));
#142374=CARTESIAN_POINT('Ctrl Pts',(118.962042593769,-8.88349197063399,
69.138257608636));
#142375=CARTESIAN_POINT('Ctrl Pts',(110.232926505569,-6.57248630373099,
73.5692045140896));
#142376=CARTESIAN_POINT('Ctrl Pts',(110.350595026869,-6.57646225464799,
73.5475367647887));
#142377=CARTESIAN_POINT('Ctrl Pts',(110.514246826669,-6.57982144133399,
73.5174352873947));
#142378=CARTESIAN_POINT('Ctrl Pts',(110.718524840469,-6.58683805357799,
73.4794333787347));
#142379=CARTESIAN_POINT('Ctrl Pts',(110.863485607269,-6.59434132275299,
73.4525971677378));
#142380=CARTESIAN_POINT('Ctrl Pts',(110.963557032969,-6.59638291515199,
73.4355706395166));
#142381=CARTESIAN_POINT('Ctrl Pts',(111.025104038669,-6.58935878847399,
73.4281786648391));
#142382=CARTESIAN_POINT('Ctrl Pts',(111.092548007969,-6.57825182407899,
73.420294394042));
#142383=CARTESIAN_POINT('Ctrl Pts',(111.218265532969,-6.57629110243299,
73.393596872829));
#142384=CARTESIAN_POINT('Ctrl Pts',(111.468139343069,-6.58471600587499,
73.3330060922452));
#142385=CARTESIAN_POINT('Ctrl Pts',(111.881580646269,-6.59151971225099,
73.2383699264408));
#142386=CARTESIAN_POINT('Ctrl Pts',(112.460108658969,-6.59931301435299,
73.0968990798939));
#142387=CARTESIAN_POINT('Ctrl Pts',(113.387924113269,-6.61202441850599,
72.8532330466304));
#142388=CARTESIAN_POINT('Ctrl Pts',(114.997470218769,-6.63187069013699,
72.3831353278457));
#142389=CARTESIAN_POINT('Ctrl Pts',(117.446904114169,-6.65506062627299,
71.516844779856));
#142390=CARTESIAN_POINT('Ctrl Pts',(119.367596957269,-6.66229891622699,
70.632566385416));
#142391=CARTESIAN_POINT('Ctrl Pts',(120.384430332969,-6.66327650304099,
70.092315923963));
#142392=CARTESIAN_POINT('Ctrl Pts',(110.901961917469,-4.62825007550899,
74.232635396243));
#142393=CARTESIAN_POINT('Ctrl Pts',(111.006547711069,-4.62839570152099,
74.214148267874));
#142394=CARTESIAN_POINT('Ctrl Pts',(111.193027963169,-4.63438875271899,
74.179690962165));
#142395=CARTESIAN_POINT('Ctrl Pts',(111.402994344069,-4.63938360278399,
74.142365011593));
#142396=CARTESIAN_POINT('Ctrl Pts',(111.526432862869,-4.64076307547399,
74.121036795092));
#142397=CARTESIAN_POINT('Ctrl Pts',(111.614963911669,-4.64062253314799,
74.105572716154));
#142398=CARTESIAN_POINT('Ctrl Pts',(111.682764776369,-4.63679325639199,
74.094106144587));
#142399=CARTESIAN_POINT('Ctrl Pts',(111.764602035069,-4.63067007736599,
74.079412733284));
#142400=CARTESIAN_POINT('Ctrl Pts',(111.899222872569,-4.62973342336699,
74.049659910301));
#142401=CARTESIAN_POINT('Ctrl Pts',(112.152730704169,-4.63547879755899,
73.989765470765));
#142402=CARTESIAN_POINT('Ctrl Pts',(112.575258310169,-4.64094937026599,
73.8923029904515));
#142403=CARTESIAN_POINT('Ctrl Pts',(113.169259174669,-4.64722823235099,
73.7460063308676));
#142404=CARTESIAN_POINT('Ctrl Pts',(114.119837515269,-4.65744614110199,
73.4944221208521));
#142405=CARTESIAN_POINT('Ctrl Pts',(115.768577097969,-4.67339593125899,
73.0090005205452));
#142406=CARTESIAN_POINT('Ctrl Pts',(118.273335469269,-4.69224475007099,
72.1147099921028));
#142407=CARTESIAN_POINT('Ctrl Pts',(120.232682197569,-4.69862092546799,
71.202748992289));
#142408=CARTESIAN_POINT('Ctrl Pts',(121.269225159869,-4.69980354156199,
70.646094772409));
#142409=CARTESIAN_POINT('Ctrl Pts',(111.302429095369,-3.11051865222899,
74.598597220957));
#142410=CARTESIAN_POINT('Ctrl Pts',(111.394664964469,-3.10840859475799,
74.582176303359));
#142411=CARTESIAN_POINT('Ctrl Pts',(111.599388335569,-3.11523302300199,
74.54494440117));
#142412=CARTESIAN_POINT('Ctrl Pts',(111.812891893969,-3.11842203978399,
74.507953556329));
#142413=CARTESIAN_POINT('Ctrl Pts',(111.914920967869,-3.11592395483799,
74.490718133494));
#142414=CARTESIAN_POINT('Ctrl Pts',(111.991551157469,-3.11454821759999,
74.476683595707));
#142415=CARTESIAN_POINT('Ctrl Pts',(112.065694454869,-3.11329885156799,
74.462165162077));
#142416=CARTESIAN_POINT('Ctrl Pts',(112.161368620869,-3.11103482700299,
74.44237079032));
#142417=CARTESIAN_POINT('Ctrl Pts',(112.302906402769,-3.11077709479499,
74.410512416406));
#142418=CARTESIAN_POINT('Ctrl Pts',(112.557032270969,-3.11418756663799,
74.35133796726));
#142419=CARTESIAN_POINT('Ctrl Pts',(112.984043669169,-3.11832910238899,
74.252142747192));
#142420=CARTESIAN_POINT('Ctrl Pts',(113.586802782869,-3.12303242315999,
74.102855342059));
#142421=CARTESIAN_POINT('Ctrl Pts',(114.549613779969,-3.13070244834699,
73.8464836526737));
#142422=CARTESIAN_POINT('Ctrl Pts',(116.219395574769,-3.14265309403299,
73.351981889596));
#142423=CARTESIAN_POINT('Ctrl Pts',(118.752714943269,-3.15700449747199,
72.4416801021735));
#142424=CARTESIAN_POINT('Ctrl Pts',(120.730863957769,-3.16240049109099,
71.514613718839));
#142425=CARTESIAN_POINT('Ctrl Pts',(121.776847155169,-3.16372012641999,
70.949175311126));
#142426=CARTESIAN_POINT('Ctrl Pts',(111.595468274169,-1.45466988121399,
74.846425761956));
#142427=CARTESIAN_POINT('Ctrl Pts',(111.672253123969,-1.45163639103699,
74.831834122798));
#142428=CARTESIAN_POINT('Ctrl Pts',(111.896696929169,-1.45746867042799,
74.792127065424));
#142429=CARTESIAN_POINT('Ctrl Pts',(112.113181296169,-1.45871739800999,
74.755147828598));
#142430=CARTESIAN_POINT('Ctrl Pts',(112.186881942369,-1.45424709587499,
74.742277395159));
#142431=CARTESIAN_POINT('Ctrl Pts',(112.247193366669,-1.45261550698799,
74.730167292197));
#142432=CARTESIAN_POINT('Ctrl Pts',(112.329914138269,-1.45373145173099,
74.712493047907));
#142433=CARTESIAN_POINT('Ctrl Pts',(112.443345128069,-1.45470158497499,
74.687471532958));
#142434=CARTESIAN_POINT('Ctrl Pts',(112.592014534569,-1.45484197653799,
74.653711867639));
#142435=CARTESIAN_POINT('Ctrl Pts',(112.844283022569,-1.45592779359099,
74.595400592069));
#142436=CARTESIAN_POINT('Ctrl Pts',(113.273006027669,-1.45860301392999,
74.494769001152));
#142437=CARTESIAN_POINT('Ctrl Pts',(113.881141937569,-1.46150941159199,
74.343021342311));
#142438=CARTESIAN_POINT('Ctrl Pts',(114.850437750669,-1.46639764963599,
74.082853248785));
#142439=CARTESIAN_POINT('Ctrl Pts',(116.531353108869,-1.47415976484399,
73.5814438142693));
#142440=CARTESIAN_POINT('Ctrl Pts',(119.077925826669,-1.48453718184899,
72.659858147644));
#142441=CARTESIAN_POINT('Ctrl Pts',(121.062922877469,-1.49054042270799,
71.723311212546));
#142442=CARTESIAN_POINT('Ctrl Pts',(122.112156142069,-1.49316944729799,
71.152601994141));
#142443=CARTESIAN_POINT('Ctrl Pts',(111.696491028569,-0.360124565212986,
74.900584192463));
#142444=CARTESIAN_POINT('Ctrl Pts',(111.761426133369,-0.357775193352486,
74.887267715531));
#142445=CARTESIAN_POINT('Ctrl Pts',(111.999128447469,-0.361200807995286,
74.845983993127));
#142446=CARTESIAN_POINT('Ctrl Pts',(112.217455760169,-0.361051136160086,
74.808705222488));
#142447=CARTESIAN_POINT('Ctrl Pts',(112.267551186169,-0.357445487552886,
74.799599156875));
#142448=CARTESIAN_POINT('Ctrl Pts',(112.313688292569,-0.356642658628786,
74.789619793948));
#142449=CARTESIAN_POINT('Ctrl Pts',(112.404015928469,-0.358478224453286,
74.769559885122));
#142450=CARTESIAN_POINT('Ctrl Pts',(112.532089053369,-0.360155784921286,
74.740675828192));
#142451=CARTESIAN_POINT('Ctrl Pts',(112.685292843269,-0.360040770149286,
74.705871242989));
#142452=CARTESIAN_POINT('Ctrl Pts',(112.934525079669,-0.359694178076486,
74.648368228787));
#142453=CARTESIAN_POINT('Ctrl Pts',(113.362220200769,-0.360955145893786,
74.54721473497));
#142454=CARTESIAN_POINT('Ctrl Pts',(113.971187372169,-0.361918458962486,
74.394502753305));
#142455=CARTESIAN_POINT('Ctrl Pts',(114.940214773769,-0.363780597524286,
74.13302532246));
#142456=CARTESIAN_POINT('Ctrl Pts',(116.620643502969,-0.366578249264186,
73.6295086638907));
#142457=CARTESIAN_POINT('Ctrl Pts',(119.163972296969,-0.370652417349286,
72.7054355250659));
#142458=CARTESIAN_POINT('Ctrl Pts',(121.144272815269,-0.373784456041386,
71.768179001727));
#142459=CARTESIAN_POINT('Ctrl Pts',(122.190927037569,-0.375416645258886,
71.197391893318));
#142460=CARTESIAN_POINT('Ctrl Pts',(111.719449830669,0.168542024809114,
74.886725365525));
#142461=CARTESIAN_POINT('Ctrl Pts',(111.777956490669,0.170096013221014,
74.874161149833));
#142462=CARTESIAN_POINT('Ctrl Pts',(112.022380833669,0.168541949368414,
74.832039678843));
#142463=CARTESIAN_POINT('Ctrl Pts',(112.241742962669,0.169476862651314,
74.794498014263));
#142464=CARTESIAN_POINT('Ctrl Pts',(112.278226804169,0.171833202524114,
74.787818476474));
#142465=CARTESIAN_POINT('Ctrl Pts',(112.315978018769,0.171867884708614,
74.779355268586));
#142466=CARTESIAN_POINT('Ctrl Pts',(112.410919825469,0.170092732407714,
74.75789040944));
#142467=CARTESIAN_POINT('Ctrl Pts',(112.547469632369,0.168715079612914,
74.726766261338));
#142468=CARTESIAN_POINT('Ctrl Pts',(112.702898853469,0.169203428043914,
74.69149379952));
#142469=CARTESIAN_POINT('Ctrl Pts',(112.950064158069,0.170274286069014,
74.634528449429));
#142470=CARTESIAN_POINT('Ctrl Pts',(113.376613512969,0.170027200701914,
74.533302102221));
#142471=CARTESIAN_POINT('Ctrl Pts',(113.985227807269,0.170539620258414,
74.380372401485));
#142472=CARTESIAN_POINT('Ctrl Pts',(114.952812262469,0.171032612972814,
74.118724642226));
#142473=CARTESIAN_POINT('Ctrl Pts',(116.630740742369,0.172350907441314,
73.6151214271312));
#142474=CARTESIAN_POINT('Ctrl Pts',(119.168949242269,0.174425178655114,
72.6917147397916));
#142475=CARTESIAN_POINT('Ctrl Pts',(121.144176338569,0.175723369492814,
71.756197744828));
#142476=CARTESIAN_POINT('Ctrl Pts',(122.188142213169,0.176373882112714,
71.186651895743));
#142477=CARTESIAN_POINT('Ctrl Pts',(111.837855321069,-3.16944077378891E-5,
74.865893185247));
#142478=CARTESIAN_POINT('Ctrl Pts',(111.905501829069,-0.000126979998721889,
74.853819715785));
#142479=CARTESIAN_POINT('Ctrl Pts',(112.067033374169,-0.00145620723710179,
74.825979590322));
#142480=CARTESIAN_POINT('Ctrl Pts',(112.232987931369,-0.000804753782924589,
74.797596316915));
#142481=CARTESIAN_POINT('Ctrl Pts',(112.273760035969,0.00190512480894021,
74.790159935677));
#142482=CARTESIAN_POINT('Ctrl Pts',(112.314147583869,0.00217643220178221,
74.781227585595));
#142483=CARTESIAN_POINT('Ctrl Pts',(112.407642187069,0.000395759237193011,
74.760204664648));
#142484=CARTESIAN_POINT('Ctrl Pts',(112.541521774169,-0.00105456873310479,
74.729786169022));
#142485=CARTESIAN_POINT('Ctrl Pts',(112.696237777969,-0.000677150123564289,
74.694665286851));
#142486=CARTESIAN_POINT('Ctrl Pts',(112.944044643669,0.000162384145561411,
74.637532653636));
#142487=CARTESIAN_POINT('Ctrl Pts',(113.370937985569,-0.000398344211388589,
74.536336212313));
#142488=CARTESIAN_POINT('Ctrl Pts',(113.979637815569,-0.000339910781080989,
74.38348544604));
#142489=CARTESIAN_POINT('Ctrl Pts',(114.947637210069,-0.000572835564488789,
74.121909214046));
#142490=CARTESIAN_POINT('Ctrl Pts',(116.626285365669,-0.000492304917713389,
73.618367621019));
#142491=CARTESIAN_POINT('Ctrl Pts',(119.105257840569,-0.000471121657127989,
72.7169063002584));
#142492=CARTESIAN_POINT('Ctrl Pts',(121.026723756869,8.56223467947709E-5,
71.813563678684));
#142493=CARTESIAN_POINT('Ctrl Pts',(122.019294640269,7.00634385962609E-5,
71.280020192514));
#142494=CARTESIAN_POINT('Ctrl Pts',(111.719593813469,-0.171868557479286,
74.886637782194));
#142495=CARTESIAN_POINT('Ctrl Pts',(111.778059621769,-0.173417549884886,
74.874078349544));
#142496=CARTESIAN_POINT('Ctrl Pts',(112.022526849069,-0.171875263124186,
74.831951508582));
#142497=CARTESIAN_POINT('Ctrl Pts',(112.241895554969,-0.172815126157786,
74.794408177235));
#142498=CARTESIAN_POINT('Ctrl Pts',(112.278293639269,-0.175163590064086,
74.78774392618));
#142499=CARTESIAN_POINT('Ctrl Pts',(112.315992195369,-0.175193426080186,
74.779290235468));
#142500=CARTESIAN_POINT('Ctrl Pts',(112.410963116769,-0.173418660436886,
74.757816516147));
#142501=CARTESIAN_POINT('Ctrl Pts',(112.547566271969,-0.172042908902086,
74.726678270653));
#142502=CARTESIAN_POINT('Ctrl Pts',(112.703009488169,-0.172533610923386,
74.691402866405));
#142503=CARTESIAN_POINT('Ctrl Pts',(112.950161776769,-0.173609024219986,
74.634440900189));
#142504=CARTESIAN_POINT('Ctrl Pts',(113.376703920169,-0.173368321007886,
74.533214092014));
#142505=CARTESIAN_POINT('Ctrl Pts',(113.985315989269,-0.173890031129486,
74.380283018442));
#142506=CARTESIAN_POINT('Ctrl Pts',(114.952891357869,-0.174397850254086,
74.118634182427));
#142507=CARTESIAN_POINT('Ctrl Pts',(116.630804091769,-0.175742056888286,
73.615030414165));
#142508=CARTESIAN_POINT('Ctrl Pts',(119.169069409069,-0.177855112533286,
72.6915955064676));
#142509=CARTESIAN_POINT('Ctrl Pts',(121.144345474869,-0.179181240266986,
71.756041340767));
#142510=CARTESIAN_POINT('Ctrl Pts',(122.188370590769,-0.179846170816786,
71.186449512022));
#142511=CARTESIAN_POINT('Ctrl Pts',(111.696720868469,0.357553932207514,
74.900699702834));
#142512=CARTESIAN_POINT('Ctrl Pts',(111.761627617569,0.355206270543514,
74.88738629695));
#142513=CARTESIAN_POINT('Ctrl Pts',(111.999361718969,0.358626044628914,
74.846098758947));
#142514=CARTESIAN_POINT('Ctrl Pts',(112.217693493969,0.358473043628614,
74.808819236382));
#142515=CARTESIAN_POINT('Ctrl Pts',(112.267732763269,0.354869659983714,
74.799722194961));
#142516=CARTESIAN_POINT('Ctrl Pts',(112.313836230769,0.354068889305514,
74.789747953326));
#142517=CARTESIAN_POINT('Ctrl Pts',(112.404182058769,0.355906032159314,
74.769682354654));
#142518=CARTESIAN_POINT('Ctrl Pts',(112.532289985869,0.357585071714214,
74.740789115781));
#142519=CARTESIAN_POINT('Ctrl Pts',(112.685504442769,0.357469385220414,
74.705982084654));
#142520=CARTESIAN_POINT('Ctrl Pts',(112.934729378669,0.357119416652214,
74.648481010021));
#142521=CARTESIAN_POINT('Ctrl Pts',(113.362421902569,0.358376964644214,
74.547326339107));
#142522=CARTESIAN_POINT('Ctrl Pts',(113.971390825869,0.359335555158114,
74.394612156851));
#142523=CARTESIAN_POINT('Ctrl Pts',(114.940417238669,0.361190320974714,
74.133131773532));
#142524=CARTESIAN_POINT('Ctrl Pts',(116.620844208169,0.363975801124614,
73.6296104139194));
#142525=CARTESIAN_POINT('Ctrl Pts',(119.164253646169,0.368034378933414,
72.705499511873));
#142526=CARTESIAN_POINT('Ctrl Pts',(121.144623526169,0.371158886658614,
71.768193655697));
#142527=CARTESIAN_POINT('Ctrl Pts',(122.191347654569,0.372788308176714,
71.197352785866));
#142528=CARTESIAN_POINT('Ctrl Pts',(111.595710961569,1.45325035480701,74.846630855493));
#142529=CARTESIAN_POINT('Ctrl Pts',(111.672482312469,1.45021612247701,74.832040780653));
#142530=CARTESIAN_POINT('Ctrl Pts',(111.896943450769,1.45604747320501,74.792331548089));
#142531=CARTESIAN_POINT('Ctrl Pts',(112.113430453969,1.45729453350601,74.755352280744));
#142532=CARTESIAN_POINT('Ctrl Pts',(112.187106546769,1.45282267665201,74.742485580224));
#142533=CARTESIAN_POINT('Ctrl Pts',(112.247403885269,1.45119094433001,74.730377126641));
#142534=CARTESIAN_POINT('Ctrl Pts',(112.330132104869,1.45230888561001,74.712700186003));
#142535=CARTESIAN_POINT('Ctrl Pts',(112.443578434869,1.45328172180801,74.687674215795));
#142536=CARTESIAN_POINT('Ctrl Pts',(112.592253937869,1.45342243526401,74.653912939217));
#142537=CARTESIAN_POINT('Ctrl Pts',(112.844520708369,1.45450628572401,74.595602400977));
#142538=CARTESIAN_POINT('Ctrl Pts',(113.273244987869,1.45718026009701,74.49496960171));
#142539=CARTESIAN_POINT('Ctrl Pts',(113.881385280069,1.46008513257001,74.343219868355));
#142540=CARTESIAN_POINT('Ctrl Pts',(114.850686264869,1.46497102099801,74.083048585761));
#142541=CARTESIAN_POINT('Ctrl Pts',(116.531610508469,1.47272962768101,73.5816333668206));
#142542=CARTESIAN_POINT('Ctrl Pts',(119.078282948369,1.48310419649501,72.6600059770705));
#142543=CARTESIAN_POINT('Ctrl Pts',(121.063366585069,1.48910835453501,71.72340298214));
#142544=CARTESIAN_POINT('Ctrl Pts',(122.112678824069,1.49173876143601,71.152635474748));
#142545=CARTESIAN_POINT('Ctrl Pts',(111.302470472569,3.11036131899101,74.598635134671));
#142546=CARTESIAN_POINT('Ctrl Pts',(111.394705080869,3.10825098976601,74.582214427328));
#142547=CARTESIAN_POINT('Ctrl Pts',(111.599430723269,3.11507552701201,74.544982169353));
#142548=CARTESIAN_POINT('Ctrl Pts',(111.812934849969,3.11826434695701,74.50799132848));
#142549=CARTESIAN_POINT('Ctrl Pts',(111.914961677469,3.11576585252101,74.49075633246));
#142550=CARTESIAN_POINT('Ctrl Pts',(111.991590635469,3.11438998720401,74.476721939464));
#142551=CARTESIAN_POINT('Ctrl Pts',(112.065734580169,3.11314088897001,74.462203188155));
#142552=CARTESIAN_POINT('Ctrl Pts',(112.161410197369,3.11087726918001,74.442408279252));
#142553=CARTESIAN_POINT('Ctrl Pts',(112.302948742769,3.11061961324801,74.410549673625));
#142554=CARTESIAN_POINT('Ctrl Pts',(112.557074701769,3.11402984287401,74.351375293478));
#142555=CARTESIAN_POINT('Ctrl Pts',(112.984086541969,3.11817123287701,74.252179898395));
#142556=CARTESIAN_POINT('Ctrl Pts',(113.586846597569,3.12287438806101,74.102892171601));
#142557=CARTESIAN_POINT('Ctrl Pts',(114.549658879369,3.13054413896501,73.8465199768088));
#142558=CARTESIAN_POINT('Ctrl Pts',(116.219442899969,3.14249435186701,73.3520172503437));
#142559=CARTESIAN_POINT('Ctrl Pts',(118.752854170869,3.15684575437601,72.4416818256266));
#142560=CARTESIAN_POINT('Ctrl Pts',(120.731086507869,3.16224156635401,71.514566000912));
#142561=CARTESIAN_POINT('Ctrl Pts',(121.777147093869,3.16356103770801,70.949073117786));
#142562=CARTESIAN_POINT('Ctrl Pts',(110.901961451069,4.62824984549301,74.232635559883));
#142563=CARTESIAN_POINT('Ctrl Pts',(111.006547427469,4.62839545723401,74.214148401757));
#142564=CARTESIAN_POINT('Ctrl Pts',(111.193027966069,4.63438852139201,74.179691041673));
#142565=CARTESIAN_POINT('Ctrl Pts',(111.402994594569,4.63938337439001,74.142365049295));
#142566=CARTESIAN_POINT('Ctrl Pts',(111.526433112769,4.64076284552401,74.121036832436));
#142567=CARTESIAN_POINT('Ctrl Pts',(111.614964129869,4.64062229704501,74.105572759132));
#142568=CARTESIAN_POINT('Ctrl Pts',(111.682764955069,4.63679301361201,74.09410619405));
#142569=CARTESIAN_POINT('Ctrl Pts',(111.764602222569,4.63066983700401,74.079412776184));
#142570=CARTESIAN_POINT('Ctrl Pts',(111.899223119269,4.62973319388701,74.049659934194));
#142571=CARTESIAN_POINT('Ctrl Pts',(112.152730985569,4.63547857422301,73.98976548501));
#142572=CARTESIAN_POINT('Ctrl Pts',(112.575258551469,4.64094913902301,73.8923030139087));
#142573=CARTESIAN_POINT('Ctrl Pts',(113.169259448369,4.64722800682301,73.7460063403004));
#142574=CARTESIAN_POINT('Ctrl Pts',(114.119837790469,4.65744591559201,73.4944221223189));
#142575=CARTESIAN_POINT('Ctrl Pts',(115.768577398569,4.67339571091001,73.0090004995231));
#142576=CARTESIAN_POINT('Ctrl Pts',(118.273423680269,4.69224519885701,72.114678555699));
#142577=CARTESIAN_POINT('Ctrl Pts',(120.232851148669,4.69862127106701,71.202670417722));
#142578=CARTESIAN_POINT('Ctrl Pts',(121.269469905269,4.69980362325801,70.645963403317));
#142579=CARTESIAN_POINT('Ctrl Pts',(110.232925928169,6.57248641407201,73.5692045744232));
#142580=CARTESIAN_POINT('Ctrl Pts',(110.350594809869,6.57646238792501,73.547536757197));
#142581=CARTESIAN_POINT('Ctrl Pts',(110.514246798369,6.57982157032801,73.517435246692));
#142582=CARTESIAN_POINT('Ctrl Pts',(110.718525112169,6.58683820167901,73.4794332803124));
#142583=CARTESIAN_POINT('Ctrl Pts',(110.863485898169,6.59434146833501,73.4525970688935));
#142584=CARTESIAN_POINT('Ctrl Pts',(110.963557254469,6.59638304026101,73.4355705602877));
#142585=CARTESIAN_POINT('Ctrl Pts',(111.025104194869,6.58935890101301,73.4281785994106));
#142586=CARTESIAN_POINT('Ctrl Pts',(111.092548167869,6.57825194271401,73.4202943209154));
#142587=CARTESIAN_POINT('Ctrl Pts',(111.218265769069,6.57629123923301,73.3935967718485));
#142588=CARTESIAN_POINT('Ctrl Pts',(111.468139625369,6.58471615098001,73.3330059774607));
#142589=CARTESIAN_POINT('Ctrl Pts',(111.881580876669,6.59151984344101,73.2383698280508));
#142590=CARTESIAN_POINT('Ctrl Pts',(112.460108929569,6.59931315242701,73.0968989644948));
#142591=CARTESIAN_POINT('Ctrl Pts',(113.387924384169,6.61202455237501,72.8532329259722));
#142592=CARTESIAN_POINT('Ctrl Pts',(114.997470519269,6.63187082303001,72.3831351861819));
#142593=CARTESIAN_POINT('Ctrl Pts',(117.446990386569,6.65506156567701,71.516814210058));
#142594=CARTESIAN_POINT('Ctrl Pts',(119.367762586869,6.66229965768501,70.632490081439));
#142595=CARTESIAN_POINT('Ctrl Pts',(120.384670436869,6.66327684772201,70.092188313576));
#142596=CARTESIAN_POINT('Ctrl Pts',(109.191314516269,8.78258400348901,72.4355246472895));
#142597=CARTESIAN_POINT('Ctrl Pts',(109.318496766669,8.79074911336402,72.4092113893872));
#142598=CARTESIAN_POINT('Ctrl Pts',(109.457841968569,8.79007292918101,72.3857653855102));
#142599=CARTESIAN_POINT('Ctrl Pts',(109.652915483569,8.79836364817301,72.346907721148));
#142600=CARTESIAN_POINT('Ctrl Pts',(109.812650199469,8.81202886086001,72.3129069288903));
#142601=CARTESIAN_POINT('Ctrl Pts',(109.920220362869,8.81641523097701,72.294152507876));
#142602=CARTESIAN_POINT('Ctrl Pts',(109.977236887169,8.80705059642201,72.2917242903443));
#142603=CARTESIAN_POINT('Ctrl Pts',(110.033657738369,8.79212761653301,72.2920076209844));
#142604=CARTESIAN_POINT('Ctrl Pts',(110.149586182069,8.78926864593201,72.2692451879473));
#142605=CARTESIAN_POINT('Ctrl Pts',(110.390312685769,8.79939076523601,72.2085162678206));
#142606=CARTESIAN_POINT('Ctrl Pts',(110.787643766769,8.80677732173501,72.1183221319088));
#142607=CARTESIAN_POINT('Ctrl Pts',(111.341319601969,8.81519507323601,71.98425856008));
#142608=CARTESIAN_POINT('Ctrl Pts',(112.231077144669,8.82897610251101,71.753069645188));
#142609=CARTESIAN_POINT('Ctrl Pts',(113.775050646669,8.85050081128701,71.307507238708));
#142610=CARTESIAN_POINT('Ctrl Pts',(116.129417060569,8.87550261923901,70.48726993864));
#142611=CARTESIAN_POINT('Ctrl Pts',(117.981018021169,8.88284688927401,69.650073667281));
#142612=CARTESIAN_POINT('Ctrl Pts',(118.962274274669,8.88349208348702,69.138136754579));
#142613=CARTESIAN_POINT('Ctrl Pts',(107.705304995269,11.02502713784,70.67242078014));
#142614=CARTESIAN_POINT('Ctrl Pts',(107.833381203869,11.0352878678,70.641686335191));
#142615=CARTESIAN_POINT('Ctrl Pts',(107.951392012169,11.03147444484,70.625804130375));
#142616=CARTESIAN_POINT('Ctrl Pts',(108.132219055569,11.03935852329,70.586956090092));
#142617=CARTESIAN_POINT('Ctrl Pts',(108.293216685169,11.0556364815,70.546564513235));
#142618=CARTESIAN_POINT('Ctrl Pts',(108.400946813269,11.06130905511,70.526510351234));
#142619=CARTESIAN_POINT('Ctrl Pts',(108.456184265469,11.05215574674,70.528338167977));
#142620=CARTESIAN_POINT('Ctrl Pts',(108.508445607669,11.03741701131,70.535283122245));
#142621=CARTESIAN_POINT('Ctrl Pts',(108.615265154269,11.03463331631,70.516278516022));
#142622=CARTESIAN_POINT('Ctrl Pts',(108.839308828169,11.04433523527,70.457395828984));
#142623=CARTESIAN_POINT('Ctrl Pts',(109.211536858369,11.05132192073,70.373703475901));
#142624=CARTESIAN_POINT('Ctrl Pts',(109.729139110969,11.05938104937,70.250016380467));
#142625=CARTESIAN_POINT('Ctrl Pts',(110.561966276769,11.0725499267,70.036918422342));
#142626=CARTESIAN_POINT('Ctrl Pts',(112.007824717869,11.09321824995,69.627472389874));
#142627=CARTESIAN_POINT('Ctrl Pts',(114.217074442569,11.11743314014,68.876850220292));
#142628=CARTESIAN_POINT('Ctrl Pts',(115.960531140069,11.12475758935,68.112973926865));
#142629=CARTESIAN_POINT('Ctrl Pts',(116.885838043069,11.12546097109,67.645789953276));
#142630=CARTESIAN_POINT('Ctrl Pts',(106.340746064769,12.49620299268,68.938652400208));
#142631=CARTESIAN_POINT('Ctrl Pts',(106.461326845869,12.50492126694,68.907372247313));
#142632=CARTESIAN_POINT('Ctrl Pts',(106.568673101969,12.50143025146,68.895175686918));
#142633=CARTESIAN_POINT('Ctrl Pts',(106.735189843669,12.50765049241,68.858193961533));
#142634=CARTESIAN_POINT('Ctrl Pts',(106.886006010469,12.52129392982,68.816856127653));
#142635=CARTESIAN_POINT('Ctrl Pts',(106.988243444669,12.52639514863,68.796825178415));
#142636=CARTESIAN_POINT('Ctrl Pts',(107.043664387869,12.5196762878,68.799558268862));
#142637=CARTESIAN_POINT('Ctrl Pts',(107.098088360869,12.50878453451,68.807326697118));
#142638=CARTESIAN_POINT('Ctrl Pts',(107.199704553969,12.50706917166,68.789786078134));
#142639=CARTESIAN_POINT('Ctrl Pts',(107.406472387069,12.51482471433,68.734883578961));
#142640=CARTESIAN_POINT('Ctrl Pts',(107.754316317369,12.52100944962,68.657488725541));
#142641=CARTESIAN_POINT('Ctrl Pts',(108.238498666269,12.528411906,68.543338618884));
#142642=CARTESIAN_POINT('Ctrl Pts',(109.017501812769,12.54042205079,68.347455503471));
#142643=CARTESIAN_POINT('Ctrl Pts',(110.370644427969,12.5595578317,67.972761728283));
#142644=CARTESIAN_POINT('Ctrl Pts',(112.441233465469,12.58290086265,67.290392999253));
#142645=CARTESIAN_POINT('Ctrl Pts',(114.080143265369,12.59164302917,66.599850642037));
#142646=CARTESIAN_POINT('Ctrl Pts',(114.951507165569,12.59362065671,66.177822481062));
#142647=CARTESIAN_POINT('Ctrl Pts',(105.478381382169,13.19595788191,67.814637903535));
#142648=CARTESIAN_POINT('Ctrl Pts',(105.591597695769,13.20309884871,67.784676078824));
#142649=CARTESIAN_POINT('Ctrl Pts',(105.694959142869,13.20040697058,67.773168259565));
#142650=CARTESIAN_POINT('Ctrl Pts',(105.852226219569,13.20545010774,67.738061839862));
#142651=CARTESIAN_POINT('Ctrl Pts',(105.993023940669,13.21657762319,67.698458452134));
#142652=CARTESIAN_POINT('Ctrl Pts',(106.089773756169,13.22094990211,67.679082686242));
#142653=CARTESIAN_POINT('Ctrl Pts',(106.145479184669,13.21596396795,67.681109146461));
#142654=CARTESIAN_POINT('Ctrl Pts',(106.202541533469,13.20782017102,67.68730292165));
#142655=CARTESIAN_POINT('Ctrl Pts',(106.301578493169,13.20680924394,67.67002461521));
#142656=CARTESIAN_POINT('Ctrl Pts',(106.496965899669,13.21315921563,67.618514237609));
#142657=CARTESIAN_POINT('Ctrl Pts',(106.828684605869,13.21870592217,67.545238419545));
#142658=CARTESIAN_POINT('Ctrl Pts',(107.291245390969,13.22551716859,67.437216561838));
#142659=CARTESIAN_POINT('Ctrl Pts',(108.035119877169,13.23652600666,67.252589805463));
#142660=CARTESIAN_POINT('Ctrl Pts',(109.327820975069,13.2542736501,66.90080626753));
#142661=CARTESIAN_POINT('Ctrl Pts',(111.307658395069,13.27662197795,66.26394965669));
#142662=CARTESIAN_POINT('Ctrl Pts',(112.877999996569,13.28626564592,65.62284046902));
#142663=CARTESIAN_POINT('Ctrl Pts',(113.714201400569,13.28917245567,65.231331633562));
#142664=CARTESIAN_POINT('Ctrl Pts',(105.189070557869,13.40684195318,67.435610002882));
#142665=CARTESIAN_POINT('Ctrl Pts',(105.299583835569,13.4134261125,67.40626642105));
#142666=CARTESIAN_POINT('Ctrl Pts',(105.401847697369,13.41103243054,67.3948159773));
#142667=CARTESIAN_POINT('Ctrl Pts',(105.556007154469,13.41568435939,67.360405502425));
#142668=CARTESIAN_POINT('Ctrl Pts',(105.693123942669,13.42592971861,67.321635373775));
#142669=CARTESIAN_POINT('Ctrl Pts',(105.787836502669,13.43003279964,67.302552890253));
#142670=CARTESIAN_POINT('Ctrl Pts',(105.843627630969,13.42561819941,67.304209229825));
#142671=CARTESIAN_POINT('Ctrl Pts',(105.901649868169,13.41838048947,67.309666484894));
#142672=CARTESIAN_POINT('Ctrl Pts',(105.999865994969,13.4175935476,67.29241931739));
#142673=CARTESIAN_POINT('Ctrl Pts',(106.191404943369,13.42347187295,67.242135867778));
#142674=CARTESIAN_POINT('Ctrl Pts',(106.517632051069,13.42879134615,67.170261061005));
#142675=CARTESIAN_POINT('Ctrl Pts',(106.972869502569,13.43538250913,67.064317489389));
#142676=CARTESIAN_POINT('Ctrl Pts',(107.704821982669,13.44602311522,66.883523192121));
#142677=CARTESIAN_POINT('Ctrl Pts',(108.977021096569,13.4632501382,66.539556699398));
#142678=CARTESIAN_POINT('Ctrl Pts',(110.926054857169,13.48518915223,65.918270879432));
#142679=CARTESIAN_POINT('Ctrl Pts',(112.473128590069,13.49509526728,65.294113763225));
#142680=CARTESIAN_POINT('Ctrl Pts',(113.297428787769,13.49830029927,64.91307310569));
#142681=CARTESIAN_POINT('Ctrl Pts',(111.837855321069,-3.16944077378891E-5,
74.865893185247));
#142682=CARTESIAN_POINT('Ctrl Pts',(111.814564406692,0.481394395961152,
74.8700371574733));
#142683=CARTESIAN_POINT('Ctrl Pts',(111.719575962393,1.51657032727011,74.8123455490061));
#142684=CARTESIAN_POINT('Ctrl Pts',(111.444434225665,3.11067739388218,74.5731663746096));
#142685=CARTESIAN_POINT('Ctrl Pts',(111.048792048017,4.63025083099635,74.2062440518196));
#142686=CARTESIAN_POINT('Ctrl Pts',(110.383842672146,6.57696395825753,73.5414122769946));
#142687=CARTESIAN_POINT('Ctrl Pts',(109.342826174747,8.7894085376038,72.4057751166405));
#142688=CARTESIAN_POINT('Ctrl Pts',(107.850972194421,11.0326713699803,70.6411881108118));
#142689=CARTESIAN_POINT('Ctrl Pts',(106.505291772843,12.472019416551,68.9441554245893));
#142690=CARTESIAN_POINT('Ctrl Pts',(105.66717799772,13.1524911207421,67.8633232117159));
#142691=CARTESIAN_POINT('Ctrl Pts',(105.406714415269,13.34497198119,67.526105385012));
#142692=CARTESIAN_POINT('Ctrl Pts',(94.2719755564691,-0.232535619158986,
77.960293090095));
#142693=CARTESIAN_POINT('Ctrl Pts',(96.4654948137691,-0.234045302815186,
77.573429542034));
#142694=CARTESIAN_POINT('Ctrl Pts',(100.753541807869,-0.237849509244786,
76.817900401937));
#142695=CARTESIAN_POINT('Ctrl Pts',(105.569477935369,-0.243699651693586,
75.968797979103));
#142696=CARTESIAN_POINT('Ctrl Pts',(108.706635670869,-0.248295135150586,
75.414082723585));
#142697=CARTESIAN_POINT('Ctrl Pts',(110.394346681069,-0.250417836874586,
75.117374150089));
#142698=CARTESIAN_POINT('Ctrl Pts',(111.490448059869,-0.253375583460886,
74.924836266052));
#142699=CARTESIAN_POINT('Ctrl Pts',(112.150874686469,-0.253183225873986,
74.806307851534));
#142700=CARTESIAN_POINT('Ctrl Pts',(94.2748484062691,0.273581135887814,
77.974569798547));
#142701=CARTESIAN_POINT('Ctrl Pts',(96.4658642089691,0.275086851522514,
77.588391617785));
#142702=CARTESIAN_POINT('Ctrl Pts',(100.749136226669,0.279152495519414,
76.834104579055));
#142703=CARTESIAN_POINT('Ctrl Pts',(105.559122588369,0.286383475540014,
75.986316878894));
#142704=CARTESIAN_POINT('Ctrl Pts',(108.693165039069,0.291717408504714,
75.43229368399));
#142705=CARTESIAN_POINT('Ctrl Pts',(110.377550127869,0.295689160759514,
75.136153730842));
#142706=CARTESIAN_POINT('Ctrl Pts',(111.475979202669,0.295825796724414,
74.943355140899));
#142707=CARTESIAN_POINT('Ctrl Pts',(112.131988786069,0.299193462052214,
74.825561946835));
#142708=CARTESIAN_POINT('Ctrl Pts',(94.2651023215691,1.30788160650201,77.911176272393));
#142709=CARTESIAN_POINT('Ctrl Pts',(96.4454408924691,1.31912219392701,77.525812822656));
#142710=CARTESIAN_POINT('Ctrl Pts',(100.708094210469,1.34342458471501,76.773429707576));
#142711=CARTESIAN_POINT('Ctrl Pts',(105.493968389769,1.37592947659601,75.928679146587));
#142712=CARTESIAN_POINT('Ctrl Pts',(108.613695916869,1.39843192417101,75.376791007982));
#142713=CARTESIAN_POINT('Ctrl Pts',(110.287407697569,1.41239992444901,75.082153932159));
#142714=CARTESIAN_POINT('Ctrl Pts',(111.387010027669,1.41771395267601,74.889476340583));
#142715=CARTESIAN_POINT('Ctrl Pts',(112.033257179669,1.42573735113301,74.77315042647));
#142716=CARTESIAN_POINT('Ctrl Pts',(94.2215315361691,2.87400974300901,77.640261060409));
#142717=CARTESIAN_POINT('Ctrl Pts',(96.3708145483691,2.90124158064901,77.255561094568));
#142718=CARTESIAN_POINT('Ctrl Pts',(100.573127653869,2.95640021853601,76.505561640338));
#142719=CARTESIAN_POINT('Ctrl Pts',(105.290086356369,3.02238572421201,75.666090838628));
#142720=CARTESIAN_POINT('Ctrl Pts',(108.366745704269,3.06612655879001,75.118411963246));
#142721=CARTESIAN_POINT('Ctrl Pts',(110.013388461769,3.09171703117801,74.826511452526));
#142722=CARTESIAN_POINT('Ctrl Pts',(111.106033966669,3.10383133871601,74.634770306963));
#142723=CARTESIAN_POINT('Ctrl Pts',(111.734450365969,3.11621882693801,74.520728353414));
#142724=CARTESIAN_POINT('Ctrl Pts',(94.1596433975691,4.29694974764301,77.25757310543));
#142725=CARTESIAN_POINT('Ctrl Pts',(96.2671294098691,4.33699728228101,76.872950610942));
#142726=CARTESIAN_POINT('Ctrl Pts',(100.388073332769,4.41679216356601,76.124486113148));
#142727=CARTESIAN_POINT('Ctrl Pts',(105.012817018869,4.50905954978901,75.289931588994));
#142728=CARTESIAN_POINT('Ctrl Pts',(108.030893450169,4.56946366906201,74.746434441845));
#142729=CARTESIAN_POINT('Ctrl Pts',(109.642849346369,4.60376585045201,74.457264740274));
#142730=CARTESIAN_POINT('Ctrl Pts',(110.721584552469,4.62195018338701,74.266525899993));
#142731=CARTESIAN_POINT('Ctrl Pts',(111.330637817569,4.63685072964401,74.154803550323));
#142732=CARTESIAN_POINT('Ctrl Pts',(94.0472766649691,6.14488949419901,76.567167410036));
#142733=CARTESIAN_POINT('Ctrl Pts',(96.0854969155691,6.19932125964201,76.182430491435));
#142734=CARTESIAN_POINT('Ctrl Pts',(100.071511546369,6.30590152019101,75.436192040905));
#142735=CARTESIAN_POINT('Ctrl Pts',(104.544032878269,6.42467485629401,74.609669583592));
#142736=CARTESIAN_POINT('Ctrl Pts',(107.464659485969,6.50123979669401,74.073144756336));
#142737=CARTESIAN_POINT('Ctrl Pts',(109.020613419869,6.54339817072601,73.7885096808893));
#142738=CARTESIAN_POINT('Ctrl Pts',(110.072680623769,6.56809627052501,73.5995632178325));
#142739=CARTESIAN_POINT('Ctrl Pts',(110.653470886869,6.58429623151501,73.4915052484874));
#142740=CARTESIAN_POINT('Ctrl Pts',(93.8521515925691,8.31376415356201,75.380290328722));
#142741=CARTESIAN_POINT('Ctrl Pts',(95.7842092150691,8.37610151972701,74.996687931097));
#142742=CARTESIAN_POINT('Ctrl Pts',(99.5633457638691,8.49649192920001,74.256622096991));
#142743=CARTESIAN_POINT('Ctrl Pts',(103.803511437969,8.62652183262401,73.4457843236508));
#142744=CARTESIAN_POINT('Ctrl Pts',(106.574368969069,8.70918768300001,72.9222235065084));
#142745=CARTESIAN_POINT('Ctrl Pts',(108.046575652369,8.75337472812401,72.6458499975918));
#142746=CARTESIAN_POINT('Ctrl Pts',(109.052812137369,8.78167413182101,72.4603561642308));
#142747=CARTESIAN_POINT('Ctrl Pts',(109.595630513669,8.79651116265801,72.3582991515531));
#142748=CARTESIAN_POINT('Ctrl Pts',(93.4372496266691,11.3601266881,72.8749686355627));
#142749=CARTESIAN_POINT('Ctrl Pts',(95.1718644035691,11.41712605481,72.5027022603797));
#142750=CARTESIAN_POINT('Ctrl Pts',(98.5659481303691,11.52584716743,71.790923625058));
#142751=CARTESIAN_POINT('Ctrl Pts',(102.374754422069,11.63978356045,71.024735970194));
#142752=CARTESIAN_POINT('Ctrl Pts',(104.865797334769,11.71128589282,70.534131262146));
#142753=CARTESIAN_POINT('Ctrl Pts',(106.185002428269,11.74808513017,70.277403481005));
#142754=CARTESIAN_POINT('Ctrl Pts',(107.098214469969,11.77444777076,70.10142143118));
#142755=CARTESIAN_POINT('Ctrl Pts',(107.578338009969,11.78460067935,70.010906049077));
#142756=CARTESIAN_POINT('Ctrl Pts',(92.8846953388691,13.59339522532,69.569112430708));
#142757=CARTESIAN_POINT('Ctrl Pts',(94.3995479321691,13.62144836159,69.235119204506));
#142758=CARTESIAN_POINT('Ctrl Pts',(97.3641245763691,13.67740135604,68.599574211411));
#142759=CARTESIAN_POINT('Ctrl Pts',(100.691605767869,13.74147687714,67.919598503328));
#142760=CARTESIAN_POINT('Ctrl Pts',(102.867637880669,13.78402628147,67.4845182886));
#142761=CARTESIAN_POINT('Ctrl Pts',(104.018563300369,13.80621016716,67.257624514061));
#142762=CARTESIAN_POINT('Ctrl Pts',(104.818068993669,13.82296220744,67.099320022254));
#142763=CARTESIAN_POINT('Ctrl Pts',(105.237162196869,13.82954337535,67.020632040054));
#142764=CARTESIAN_POINT('Ctrl Pts',(92.2448326917691,14.79056917055,65.751520981076));
#142765=CARTESIAN_POINT('Ctrl Pts',(93.5247181401691,14.79470414109,65.492514703334));
#142766=CARTESIAN_POINT('Ctrl Pts',(96.0287650471691,14.80601682355,64.996314397124));
#142767=CARTESIAN_POINT('Ctrl Pts',(98.8382401202691,14.82558254573,64.452331124048));
#142768=CARTESIAN_POINT('Ctrl Pts',(100.673199852269,14.84110198079,64.097444414381));
#142769=CARTESIAN_POINT('Ctrl Pts',(101.644468893269,14.84982950274,63.909933430294));
#142770=CARTESIAN_POINT('Ctrl Pts',(102.315422239769,14.85651834918,63.778622292892));
#142771=CARTESIAN_POINT('Ctrl Pts',(102.672955266469,14.85994328065,63.710263579365));
#142772=CARTESIAN_POINT('Ctrl Pts',(91.9040896551691,15.00296837733,63.719016359691));
#142773=CARTESIAN_POINT('Ctrl Pts',(93.0606367533691,15.00269997783,63.505997650065));
#142774=CARTESIAN_POINT('Ctrl Pts',(95.3224849385691,15.0032855081,63.09305060872));
#142775=CARTESIAN_POINT('Ctrl Pts',(97.8588083377691,15.00640812609,62.62492914454));
#142776=CARTESIAN_POINT('Ctrl Pts',(99.5137844899691,15.00944819208,62.31209564356));
#142777=CARTESIAN_POINT('Ctrl Pts',(100.390759595169,15.01129518319,62.1441843822));
#142778=CARTESIAN_POINT('Ctrl Pts',(100.993269605169,15.01273048873,62.02638756854));
#142779=CARTESIAN_POINT('Ctrl Pts',(101.318214643569,15.01358600216,61.96239030853));
#142780=CARTESIAN_POINT('Ctrl Pts',(91.7279117369691,15.00086642868,62.66815051123));
#142781=CARTESIAN_POINT('Ctrl Pts',(92.8206402341691,15.00091537795,62.47805184071));
#142782=CARTESIAN_POINT('Ctrl Pts',(94.9571144835691,15.00012220898,62.10616698998));
#142783=CARTESIAN_POINT('Ctrl Pts',(97.3520297403691,14.99728712131,61.67404148758));
#142784=CARTESIAN_POINT('Ctrl Pts',(98.9140467094691,14.99466744079,61.3801702936));
#142785=CARTESIAN_POINT('Ctrl Pts',(99.7424527660691,14.99311784675,61.22073601459));
#142786=CARTESIAN_POINT('Ctrl Pts',(100.309713938069,14.99193533907,61.10855151957));
#142787=CARTESIAN_POINT('Ctrl Pts',(100.617428775669,14.99125742262,61.04642672594));
#142788=CARTESIAN_POINT('Origin',(57.8121127436691,0.499074165591614,68.674471503788));
#142789=CARTESIAN_POINT('',(88.0907987596691,-14.9986801145128,63.5496776718788));
#142790=CARTESIAN_POINT('Ctrl Pts',(88.0907987596691,-14.99868011451,63.549677671879));
#142791=CARTESIAN_POINT('Ctrl Pts',(89.3657116351038,-14.997869438043,63.3248649301893));
#142792=CARTESIAN_POINT('Ctrl Pts',(90.6406264262481,-14.9978694380615,
63.1000630530281));
#142793=CARTESIAN_POINT('Ctrl Pts',(91.9155434702571,-14.9991665204688,
62.8752787017783));
#142794=CARTESIAN_POINT('',(88.2224712981462,-14.9706103812352,64.2964297435509));
#142795=CARTESIAN_POINT('Origin',(88.0541760202691,0.499074165591714,63.341979795825));
#142796=CARTESIAN_POINT('',(86.2245100263342,-14.5670381546171,67.3623544040121));
#142797=CARTESIAN_POINT('Ctrl Pts',(86.2245100263343,-14.5670381546171,
67.3623544040121));
#142798=CARTESIAN_POINT('Ctrl Pts',(86.2554419271589,-14.5670466650294,
67.3569163665417));
#142799=CARTESIAN_POINT('Ctrl Pts',(86.2870207042859,-14.5672200014156,
67.3506752471842));
#142800=CARTESIAN_POINT('Ctrl Pts',(86.3191954228747,-14.5675775833023,
67.343555076842));
#142801=CARTESIAN_POINT('Ctrl Pts',(86.3720903212892,-14.5681654441572,
67.3318495918071));
#142802=CARTESIAN_POINT('Ctrl Pts',(86.4265983686621,-14.5692515099211,
67.3177684420538));
#142803=CARTESIAN_POINT('Ctrl Pts',(86.4824665885848,-14.570911942245,67.3009764873743));
#142804=CARTESIAN_POINT('Ctrl Pts',(86.5377339405401,-14.5725545164628,
67.284365131749));
#142805=CARTESIAN_POINT('Ctrl Pts',(86.5943325024795,-14.5747592405898,
67.2651006452783));
#142806=CARTESIAN_POINT('Ctrl Pts',(86.6519673512887,-14.5775977677942,
67.2428541575597));
#142807=CARTESIAN_POINT('Ctrl Pts',(86.708850881912,-14.5803992924359,67.2208976713098));
#142808=CARTESIAN_POINT('Ctrl Pts',(86.7667439050915,-14.5838182728098,
67.1960361291941));
#142809=CARTESIAN_POINT('Ctrl Pts',(86.8253125521276,-14.5879205216877,
67.1679535725664));
#142810=CARTESIAN_POINT('Ctrl Pts',(86.8831432720715,-14.5919710848816,
67.1402248379989));
#142811=CARTESIAN_POINT('Ctrl Pts',(86.9416326729376,-14.5966878749362,
67.1093554830591));
#142812=CARTESIAN_POINT('Ctrl Pts',(87.0004097878607,-14.602130222003,67.0750456413716));
#142813=CARTESIAN_POINT('Ctrl Pts',(87.004855976204,-14.6025419077436,67.0724502772002));
#142814=CARTESIAN_POINT('Ctrl Pts',(87.0093037872775,-14.6029577430099,
67.0698352291958));
#142815=CARTESIAN_POINT('Ctrl Pts',(87.0137530489033,-14.6033777523591,
67.0672003692174));
#142816=CARTESIAN_POINT('Ctrl Pts',(87.0673706317975,-14.6084392407573,
67.0354479493357));
#142817=CARTESIAN_POINT('Ctrl Pts',(87.1212027637474,-14.6141080608135,
67.000817354719));
#142818=CARTESIAN_POINT('Ctrl Pts',(87.1748912039063,-14.6203899220705,
66.9631099249675));
#142819=CARTESIAN_POINT('Ctrl Pts',(87.228031685852,-14.6266076690142,66.9257873470718));
#142820=CARTESIAN_POINT('Ctrl Pts',(87.2810314455855,-14.6334261169198,
66.8854503046114));
#142821=CARTESIAN_POINT('Ctrl Pts',(87.3334965537328,-14.6408362228309,
66.8419190364476));
#142822=CARTESIAN_POINT('Ctrl Pts',(87.3853068214865,-14.648153839908,66.7989311014396));
#142823=CARTESIAN_POINT('Ctrl Pts',(87.4365956948904,-14.656048538499,66.75282810209));
#142824=CARTESIAN_POINT('Ctrl Pts',(87.4869378782774,-14.6644957728132,
66.7034509629592));
#142825=CARTESIAN_POINT('Ctrl Pts',(87.529302299325,-14.6716043677747,66.6618986549041));
#142826=CARTESIAN_POINT('Ctrl Pts',(87.5709955263894,-14.6791040253077,
66.6180279110203));
#142827=CARTESIAN_POINT('Ctrl Pts',(87.6117384985287,-14.6869704165268,
66.5717523386305));
#142828=CARTESIAN_POINT('Ctrl Pts',(87.6121077818064,-14.6870417153688,
66.5713329093609));
#142829=CARTESIAN_POINT('Ctrl Pts',(87.6124769868582,-14.6871130442736,
66.5709132825869));
#142830=CARTESIAN_POINT('Ctrl Pts',(87.6128461134674,-14.6871844032196,
66.5704934582473));
#142831=CARTESIAN_POINT('Ctrl Pts',(87.6444349017475,-14.6932910955579,
66.5345661047386));
#142832=CARTESIAN_POINT('Ctrl Pts',(87.6754500449891,-14.6996181921391,
66.4971912644075));
#142833=CARTESIAN_POINT('Ctrl Pts',(87.7057467458941,-14.7061432798311,
66.4583601287152));
#142834=CARTESIAN_POINT('Ctrl Pts',(87.721072110393,-14.7094439477019,66.4387176828179));
#142835=CARTESIAN_POINT('Ctrl Pts',(87.7362136452609,-14.7127952215432,
66.4187025888031));
#142836=CARTESIAN_POINT('Ctrl Pts',(87.7511514388679,-14.7161936925683,
66.3983146178697));
#142837=CARTESIAN_POINT('Ctrl Pts',(87.7586203356714,-14.7178929280808,
66.3881206324029));
#142838=CARTESIAN_POINT('Ctrl Pts',(87.766038297027,-14.7196039590666,66.3778334269534));
#142839=CARTESIAN_POINT('Ctrl Pts',(87.7734027995865,-14.7213263313501,
66.367452998191));
#142840=CARTESIAN_POINT('Ctrl Pts',(87.7770850508662,-14.7221875174919,
66.3622627838098));
#142841=CARTESIAN_POINT('Ctrl Pts',(87.7807539374385,-14.723051538708,66.357049263553));
#142842=CARTESIAN_POINT('Ctrl Pts',(87.7844091396446,-14.7239183361676,
66.3518124403372));
#142843=CARTESIAN_POINT('Ctrl Pts',(87.7870489286653,-14.7245443377642,
66.3480304037633));
#142844=CARTESIAN_POINT('Ctrl Pts',(87.7890837516772,-14.7250289729097,
66.345100062789));
#142845=CARTESIAN_POINT('Ctrl Pts',(87.7918098054448,-14.7256815781967,
66.3411505749329));
#142846=CARTESIAN_POINT('Ctrl Pts',(87.7928584009643,-14.725932607354,66.339631376992));
#142847=CARTESIAN_POINT('Ctrl Pts',(87.7940089138699,-14.7262085113202,
66.3379611222576));
#142848=CARTESIAN_POINT('Ctrl Pts',(87.7953333722025,-14.7265269972584,
66.3360320656442));
#142849=CARTESIAN_POINT('Ctrl Pts',(87.8270421704474,-14.7341518549904,
66.289848606751));
#142850=CARTESIAN_POINT('Ctrl Pts',(87.8561396361996,-14.7415770020337,
66.244320185919));
#142851=CARTESIAN_POINT('Ctrl Pts',(87.8828760026715,-14.748749880654,66.1997346079998));
#142852=CARTESIAN_POINT('Ctrl Pts',(87.910460227642,-14.7561502242182,66.1537351408298));
#142853=CARTESIAN_POINT('Ctrl Pts',(87.9355316640307,-14.763282194667,66.1087389913815));
#142854=CARTESIAN_POINT('Ctrl Pts',(87.9583700286187,-14.7701074924571,
66.0650087511747));
#142855=CARTESIAN_POINT('Ctrl Pts',(87.9822638228765,-14.7772482078318,
66.0192576047507));
#142856=CARTESIAN_POINT('Ctrl Pts',(88.0037139084123,-14.7840533931963,
65.9748918859642));
#142857=CARTESIAN_POINT('Ctrl Pts',(88.0230383633048,-14.7904978943206,
65.9321581299024));
#142858=CARTESIAN_POINT('Ctrl Pts',(88.0318926560556,-14.7934507072152,
65.9125779042962));
#142859=CARTESIAN_POINT('Ctrl Pts',(88.0403006154473,-14.7963280359603,
65.8933395819523));
#142860=CARTESIAN_POINT('Ctrl Pts',(88.0482922250197,-14.7991285520152,
65.8744635085759));
#142861=CARTESIAN_POINT('Ctrl Pts',(88.065125839151,-14.805027589776,65.8347027404038));
#142862=CARTESIAN_POINT('Ctrl Pts',(88.0801135053758,-14.8105852644645,
65.7965526375944));
#142863=CARTESIAN_POINT('Ctrl Pts',(88.0935327480613,-14.815798128202,65.76019469969));
#142864=CARTESIAN_POINT('Ctrl Pts',(88.1075745036794,-14.8212528144604,
65.722150132586));
#142865=CARTESIAN_POINT('Ctrl Pts',(88.1198994082141,-14.8263301020729,
65.6860675199005));
#142866=CARTESIAN_POINT('Ctrl Pts',(88.1308005801532,-14.831034908916,65.6521039125264));
#142867=CARTESIAN_POINT('Ctrl Pts',(88.1419307746528,-14.8358385589768,
65.6174267642257));
#142868=CARTESIAN_POINT('Ctrl Pts',(88.1515771757746,-14.8402541052123,
65.5849580331557));
#142869=CARTESIAN_POINT('Ctrl Pts',(88.1600199398178,-14.8442931348452,
65.5548203474047));
#142870=CARTESIAN_POINT('Ctrl Pts',(88.168631899223,-14.848413107766,65.5240786939688));
#142871=CARTESIAN_POINT('Ctrl Pts',(88.1759918859795,-14.8521415135935,
65.495761910864));
#142872=CARTESIAN_POINT('Ctrl Pts',(88.1823584667009,-14.8554942316909,
65.4699627854301));
#142873=CARTESIAN_POINT('Ctrl Pts',(88.1847937175939,-14.8567766641453,
65.4600944831181));
#142874=CARTESIAN_POINT('Ctrl Pts',(88.1870831946187,-14.8580041512027,
65.4505941995436));
#142875=CARTESIAN_POINT('Ctrl Pts',(88.1892397344708,-14.8591776291228,
65.4414659667121));
#142876=CARTESIAN_POINT('Ctrl Pts',(88.192226482607,-14.8608028636333,65.4288236163428));
#142877=CARTESIAN_POINT('Ctrl Pts',(88.1949583819352,-14.8623245059375,
65.4168949795531));
#142878=CARTESIAN_POINT('Ctrl Pts',(88.1974665021121,-14.8637450227631,
65.405689057559));
#142879=CARTESIAN_POINT('Ctrl Pts',(88.1987205622005,-14.8644552811758,
65.400086096562));
#142880=CARTESIAN_POINT('Ctrl Pts',(88.1999186773672,-14.8651402523145,
65.3946638134873));
#142881=CARTESIAN_POINT('Ctrl Pts',(88.2010643297083,-14.8658002411051,
65.3894231368125));
#142882=CARTESIAN_POINT('Ctrl Pts',(88.2016371558788,-14.8661302355004,
65.3868027984751));
#142883=CARTESIAN_POINT('Ctrl Pts',(88.2021968663335,-14.8664539838941,
65.3842278616828));
#142884=CARTESIAN_POINT('Ctrl Pts',(88.2027438845188,-14.8667715226077,
65.3816984385093));
#142885=CARTESIAN_POINT('Ctrl Pts',(88.2030173936114,-14.8669302919645,
65.3804337269225));
#142886=CARTESIAN_POINT('Ctrl Pts',(88.203287729636,-14.8670875088745,65.379180393737));
#142887=CARTESIAN_POINT('Ctrl Pts',(88.2035549440709,-14.8672431778277,
65.3779384523255));
#142888=CARTESIAN_POINT('Ctrl Pts',(88.2036885512884,-14.8673210123043,
65.3773174816197));
#142889=CARTESIAN_POINT('Ctrl Pts',(88.2037365216033,-14.8673487925349,
65.3770956790665));
#142890=CARTESIAN_POINT('Ctrl Pts',(88.2038261467464,-14.8674010463921,
65.3766785694427));
#142891=CARTESIAN_POINT('Ctrl Pts',(88.2039157718895,-14.8674533002492,
65.3762614598189));
#142892=CARTESIAN_POINT('Ctrl Pts',(88.2040470524583,-14.8675300544217,
65.3756490465892));
#142893=CARTESIAN_POINT('Ctrl Pts',(88.2043472736409,-14.8677055452291,
65.3742468165999));
#142894=CARTESIAN_POINT('Ctrl Pts',(88.227475833264,-14.8812250762862,65.2662212614667));
#142895=CARTESIAN_POINT('Ctrl Pts',(88.2436194410596,-14.8941054177045,
65.1564485646021));
#142896=CARTESIAN_POINT('Ctrl Pts',(88.2523597375445,-14.9060423907878,
65.045853643057));
#142897=CARTESIAN_POINT('Ctrl Pts',(88.2545110024111,-14.9089804594049,
65.0186327164501));
#142898=CARTESIAN_POINT('Ctrl Pts',(88.2562138322223,-14.9118613774451,
64.9913618680356));
#142899=CARTESIAN_POINT('Ctrl Pts',(88.2574686769471,-14.9146825923509,
64.9640590854486));
#142900=CARTESIAN_POINT('Ctrl Pts',(88.2585275283017,-14.9170631635605,
64.9410207064748));
#142901=CARTESIAN_POINT('Ctrl Pts',(88.259267407385,-14.9194012251429,64.9179595883371));
#142902=CARTESIAN_POINT('Ctrl Pts',(88.2596886006513,-14.9216952433542,
64.8948864854724));
#142903=CARTESIAN_POINT('Ctrl Pts',(88.2598991972844,-14.9228422524599,
64.88334993404));
#142904=CARTESIAN_POINT('Ctrl Pts',(88.2600301224623,-14.9239782506498,
64.8718103864186));
#142905=CARTESIAN_POINT('Ctrl Pts',(88.2600814136634,-14.9251030462851,
64.8602691814297));
#142906=CARTESIAN_POINT('Ctrl Pts',(88.2601262934643,-14.9260872424659,
64.8501706270644));
#142907=CARTESIAN_POINT('Ctrl Pts',(88.2601102035016,-14.927062861686,64.8400708037766));
#142908=CARTESIAN_POINT('Ctrl Pts',(88.2600331691618,-14.9280297754665,
64.829970607531));
#142909=CARTESIAN_POINT('Ctrl Pts',(88.2600221642561,-14.9281679060066,
64.8285277223531));
#142910=CARTESIAN_POINT('Ctrl Pts',(88.2599973832409,-14.92843383089,64.825744595575));
#142911=CARTESIAN_POINT('Ctrl Pts',(88.2599964232447,-14.9284436337292,
64.8256419317284));
#142912=CARTESIAN_POINT('Ctrl Pts',(88.2599806488439,-14.9286047113654,
64.8239549868249));
#142913=CARTESIAN_POINT('Ctrl Pts',(88.2600688441228,-14.9290215173409,
64.8195787139235));
#142914=CARTESIAN_POINT('Ctrl Pts',(88.2602191362165,-14.9296883818484,
64.812510127624));
#142915=CARTESIAN_POINT('Ctrl Pts',(88.2603693339231,-14.9303548275483,
64.8054459805742));
#142916=CARTESIAN_POINT('Ctrl Pts',(88.260581556943,-14.931271041923,64.7956927273991));
#142917=CARTESIAN_POINT('Ctrl Pts',(88.2607625743269,-14.9324242352605,
64.7832444165503));
#142918=CARTESIAN_POINT('Ctrl Pts',(88.2609427967042,-14.9335723639107,
64.7708507771936));
#142919=CARTESIAN_POINT('Ctrl Pts',(88.2610920711133,-14.9349554320682,
64.7557854023437));
#142920=CARTESIAN_POINT('Ctrl Pts',(88.2610675057493,-14.9365532924553,
64.7380430085675));
#142921=CARTESIAN_POINT('Ctrl Pts',(88.2610452719137,-14.9379994979787,
64.7219845668633));
#142922=CARTESIAN_POINT('Ctrl Pts',(88.2608800214993,-14.9396215991874,
64.7037329239017));
#142923=CARTESIAN_POINT('Ctrl Pts',(88.2604296824915,-14.9413988229924,
64.6832882670058));
#142924=CARTESIAN_POINT('Ctrl Pts',(88.2599427492754,-14.9433204626641,
64.661182292702));
#142925=CARTESIAN_POINT('Ctrl Pts',(88.2591231165921,-14.9454236237161,
64.6365118554533));
#142926=CARTESIAN_POINT('Ctrl Pts',(88.2577455814398,-14.9476738742103,
64.6092883924997));
#142927=CARTESIAN_POINT('Ctrl Pts',(88.2563947050679,-14.9498805766806,
64.5825917722334));
#142928=CARTESIAN_POINT('Ctrl Pts',(88.2545072049435,-14.9522287813219,
64.5534394929417));
#142929=CARTESIAN_POINT('Ctrl Pts',(88.2518258964013,-14.9546770210727,
64.5218605477094));
#142930=CARTESIAN_POINT('Ctrl Pts',(88.2490652167,-14.9571977327618,64.4893468135673));
#142931=CARTESIAN_POINT('Ctrl Pts',(88.2454633288124,-14.9598246464015,
64.4542597760387));
#142932=CARTESIAN_POINT('Ctrl Pts',(88.2406896430595,-14.9625011974931,
64.4166609082583));
#142933=CARTESIAN_POINT('Ctrl Pts',(88.2362931783414,-14.9649662450579,
64.3820331375601));
#142934=CARTESIAN_POINT('Ctrl Pts',(88.2309022872888,-14.9674733471412,
64.345274641701));
#142935=CARTESIAN_POINT('Ctrl Pts',(88.2242201005126,-14.9699684545082,
64.3064647140518));
#142936=CARTESIAN_POINT('Ctrl Pts',(88.2236467622574,-14.9701825371959,
64.3031347837538));
#142937=CARTESIAN_POINT('Ctrl Pts',(88.2230638949306,-14.9703965253424,
64.2997897727192));
#142938=CARTESIAN_POINT('Ctrl Pts',(88.2224712981462,-14.9706103812352,
64.2964297435509));
#142939=CARTESIAN_POINT('',(69.482779745793,-14.5670748341037,70.3143821603081));
#142940=CARTESIAN_POINT('',(68.9413550361439,-14.5670748341037,70.4098499446415));
#142941=CARTESIAN_POINT('',(69.0831878262454,-14.4277621758119,70.9275690132791));
#142942=CARTESIAN_POINT('Ctrl Pts',(69.0831878262454,-14.4277621758119,
70.9275690132791));
#142943=CARTESIAN_POINT('Ctrl Pts',(69.0731820518308,-14.4438343998325,
70.8709989238709));
#142944=CARTESIAN_POINT('Ctrl Pts',(69.071801460729,-14.458723937518,70.8159229870168));
#142945=CARTESIAN_POINT('Ctrl Pts',(69.0785459095066,-14.4728469146059,
70.7612092128021));
#142946=CARTESIAN_POINT('Ctrl Pts',(69.0838687136473,-14.4839929464615,
70.7180284112939));
#142947=CARTESIAN_POINT('Ctrl Pts',(69.094251884068,-14.4946539059933,70.6750710969902));
#142948=CARTESIAN_POINT('Ctrl Pts',(69.1093808572375,-14.5044009701503,
70.634246903647));
#142949=CARTESIAN_POINT('Ctrl Pts',(69.1134215889724,-14.5070042711821,
70.6233433471565));
#142950=CARTESIAN_POINT('Ctrl Pts',(69.1178008736704,-14.5095426677788,
70.6125920261805));
#142951=CARTESIAN_POINT('Ctrl Pts',(69.1225127424941,-14.5120085718611,
70.6020294622628));
#142952=CARTESIAN_POINT('Ctrl Pts',(69.1448664004014,-14.5237071098194,
70.5519194211572));
#142953=CARTESIAN_POINT('Ctrl Pts',(69.1747054265118,-14.5337740168253,
70.5060577501982));
#142954=CARTESIAN_POINT('Ctrl Pts',(69.2107935956292,-14.5419633333216,
70.4662869693077));
#142955=CARTESIAN_POINT('Ctrl Pts',(69.2468817647466,-14.550152649818,70.4265161884173));
#142956=CARTESIAN_POINT('Ctrl Pts',(69.2892192207947,-14.5564675938574,
70.3928371138276));
#142957=CARTESIAN_POINT('Ctrl Pts',(69.3348500498842,-14.560698920749,70.3671498835826));
#142958=CARTESIAN_POINT('Ctrl Pts',(69.3747126952468,-14.5643953664779,
70.3447097708335));
#142959=CARTESIAN_POINT('Ctrl Pts',(69.4170887498322,-14.5665026120276,
70.3283689348563));
#142960=CARTESIAN_POINT('Ctrl Pts',(69.4627495397367,-14.5669736346079,
70.3183391465774));
#142961=CARTESIAN_POINT('Ctrl Pts',(69.4693567235523,-14.5670417922717,
70.3168878213829));
#142962=CARTESIAN_POINT('Ctrl Pts',(69.4760326811777,-14.5670756030821,
70.3155686193061));
#142963=CARTESIAN_POINT('Ctrl Pts',(69.4827797457826,-14.5670748341036,
70.3143821603099));
#142964=CARTESIAN_POINT('',(69.9613703778984,-11.9506558356043,75.9079897530419));
#142965=CARTESIAN_POINT('Origin',(68.3580209600691,0.499074165591714,66.814943349163));
#142966=CARTESIAN_POINT('',(70.5465863733413,-11.5358762249694,76.3475293475958));
#142967=CARTESIAN_POINT('Ctrl Pts',(70.5465865011915,-11.5358771324844,
76.3475300730731));
#142968=CARTESIAN_POINT('Ctrl Pts',(70.5313040392169,-11.5358611953978,
76.3502432234202));
#142969=CARTESIAN_POINT('Ctrl Pts',(70.5161018493598,-11.5364564485583,
76.352177065221));
#142970=CARTESIAN_POINT('Ctrl Pts',(70.5009632632138,-11.5376480599897,
76.3533544936938));
#142971=CARTESIAN_POINT('Ctrl Pts',(70.4995823522497,-11.537756756355,76.3534618963186));
#142972=CARTESIAN_POINT('Ctrl Pts',(70.4982019647776,-11.5378704373222,
76.3535629778345));
#142973=CARTESIAN_POINT('Ctrl Pts',(70.4968220853222,-11.5379891051123,
76.3536577391986));
#142974=CARTESIAN_POINT('Ctrl Pts',(70.4816890378852,-11.5392905269794,
76.3546969808609));
#142975=CARTESIAN_POINT('Ctrl Pts',(70.466616928596,-11.5411889943885,76.3549795204622));
#142976=CARTESIAN_POINT('Ctrl Pts',(70.4515726992923,-11.5436640619456,
76.354532064538));
#142977=CARTESIAN_POINT('Ctrl Pts',(70.4361732910351,-11.5461975633306,
76.3540740446344));
#142978=CARTESIAN_POINT('Ctrl Pts',(70.4208024273472,-11.5493354437837,
76.3528510340008));
#142979=CARTESIAN_POINT('Ctrl Pts',(70.4054325685759,-11.5530882736582,
76.3508492610654));
#142980=CARTESIAN_POINT('Ctrl Pts',(70.4013883728073,-11.554075737429,76.3503225443431));
#142981=CARTESIAN_POINT('Ctrl Pts',(70.3973443191322,-11.5551059379066,
76.3497416918571));
#142982=CARTESIAN_POINT('Ctrl Pts',(70.3933000862645,-11.5561794006954,
76.3491059929155));
#142983=CARTESIAN_POINT('Ctrl Pts',(70.372629786894,-11.5616659287797,76.3458569002287));
#142984=CARTESIAN_POINT('Ctrl Pts',(70.3519362330081,-11.5682204805058,
76.3412564835926));
#142985=CARTESIAN_POINT('Ctrl Pts',(70.3314707729455,-11.5758188287446,
76.3352764690793));
#142986=CARTESIAN_POINT('Ctrl Pts',(70.3270314425513,-11.5774670486321,
76.3339792952017));
#142987=CARTESIAN_POINT('Ctrl Pts',(70.3226029447382,-11.5791642675993,
76.3326173286124));
#142988=CARTESIAN_POINT('Ctrl Pts',(70.3181880005322,-11.5809100473327,
76.3311904857735));
#142989=CARTESIAN_POINT('Ctrl Pts',(70.297673760895,-11.5890218924964,76.3245605954383));
#142990=CARTESIAN_POINT('Ctrl Pts',(70.2774513760942,-11.5981849144579,
76.3165268005299));
#142991=CARTESIAN_POINT('Ctrl Pts',(70.2577328684847,-11.6082908082475,
76.3071659887023));
#142992=CARTESIAN_POINT('Ctrl Pts',(70.2531703837878,-11.6106291183609,
76.3050000762733));
#142993=CARTESIAN_POINT('Ctrl Pts',(70.2486349115508,-11.6130177658129,
76.302763286082));
#142994=CARTESIAN_POINT('Ctrl Pts',(70.2441291287376,-11.6154551612671,
76.3004568668291));
#142995=CARTESIAN_POINT('Ctrl Pts',(70.2195057584611,-11.6287751310191,
76.2878526607157));
#142996=CARTESIAN_POINT('Ctrl Pts',(70.1957811556634,-11.64359859179,76.2731068200489));
#142997=CARTESIAN_POINT('Ctrl Pts',(70.1732440005013,-11.6597303060056,
76.2563626943157));
#142998=CARTESIAN_POINT('Ctrl Pts',(70.1671237010594,-11.6641111127578,
76.2518155781139));
#142999=CARTESIAN_POINT('Ctrl Pts',(70.1610912386706,-11.6685884171355,
76.2471209830158));
#143000=CARTESIAN_POINT('Ctrl Pts',(70.1551530632265,-11.6731583054232,
76.2422815649606));
#143001=CARTESIAN_POINT('Ctrl Pts',(70.1407842417427,-11.6842162321592,
76.2305714471351));
#143002=CARTESIAN_POINT('Ctrl Pts',(70.1269668641474,-11.6958163819125,
76.2180134052578));
#143003=CARTESIAN_POINT('Ctrl Pts',(70.1137575779468,-11.7079088255401,
76.2046488610965));
#143004=CARTESIAN_POINT('Ctrl Pts',(70.0987377197503,-11.7216587576543,
76.1894524640228));
#143005=CARTESIAN_POINT('Ctrl Pts',(70.0845018742824,-11.7360358510045,
76.1732255334069));
#143006=CARTESIAN_POINT('Ctrl Pts',(70.0712089922545,-11.750870538935,76.1561403878423));
#143007=CARTESIAN_POINT('Ctrl Pts',(70.0574121206845,-11.7662676728092,
76.1384074719393));
#143008=CARTESIAN_POINT('Ctrl Pts',(70.0446317261883,-11.7821570931785,
76.1197506601893));
#143009=CARTESIAN_POINT('Ctrl Pts',(70.0330087939373,-11.7983289080146,
76.1003981507878));
#143010=CARTESIAN_POINT('Ctrl Pts',(70.0320519553556,-11.7996602257954,
76.0988049876128));
#143011=CARTESIAN_POINT('Ctrl Pts',(70.03110293782,-11.8009934499662,76.0972071254132));
#143012=CARTESIAN_POINT('Ctrl Pts',(70.0301618072275,-11.8023284599218,
76.0956046994724));
#143013=CARTESIAN_POINT('Ctrl Pts',(70.025118225905,-11.8094828668982,76.0870171924787));
#143014=CARTESIAN_POINT('Ctrl Pts',(70.0203012914773,-11.8166885762045,
76.0782985593257));
#143015=CARTESIAN_POINT('Ctrl Pts',(70.0157173732272,-11.8239292805152,
76.0694689672843));
#143016=CARTESIAN_POINT('Ctrl Pts',(70.0071740977884,-11.8374241396995,
76.0530128193545));
#143017=CARTESIAN_POINT('Ctrl Pts',(69.9994952539932,-11.8510449978951,
76.0361560556408));
#143018=CARTESIAN_POINT('Ctrl Pts',(69.9926445641082,-11.8648198974923,
76.0188632102975));
#143019=CARTESIAN_POINT('Ctrl Pts',(69.9858613355384,-11.8784591504816,
76.0017406540947));
#143020=CARTESIAN_POINT('Ctrl Pts',(69.9798896952674,-11.8922500478019,
75.9841898344588));
#143021=CARTESIAN_POINT('Ctrl Pts',(69.9747409884352,-11.9062242291212,
75.9661574739964));
#143022=CARTESIAN_POINT('Ctrl Pts',(69.969592281603,-11.9201984104406,75.948125113534));
#143023=CARTESIAN_POINT('Ctrl Pts',(69.9652659732438,-11.9343565179746,
75.9296105175509));
#143024=CARTESIAN_POINT('Ctrl Pts',(69.9618267835144,-11.9487252623603,
75.9105519754272));
#143025=CARTESIAN_POINT('Ctrl Pts',(69.9616728578679,-11.9493683551943,
75.9096989842725));
#143026=CARTESIAN_POINT('Ctrl Pts',(69.961520718983,-11.9500118681541,75.9088449031724));
#143027=CARTESIAN_POINT('Ctrl Pts',(69.961370373637,-11.9506558025134,75.9079897288741));
#143028=CARTESIAN_POINT('',(80.8778403488691,-11.53587675694,74.525850965447));
#143029=CARTESIAN_POINT('Ctrl Pts',(63.5269668554091,-14.97035104563,67.431942152481));
#143030=CARTESIAN_POINT('Ctrl Pts',(63.4204723176291,-14.97157761715,67.728904162768));
#143031=CARTESIAN_POINT('Ctrl Pts',(63.2791491661791,-14.96118285201,68.415759542565));
#143032=CARTESIAN_POINT('Ctrl Pts',(63.3636705257291,-14.90657053402,69.163225313652));
#143033=CARTESIAN_POINT('Ctrl Pts',(63.4869154152091,-14.86162731758,69.560641054351));
#143034=CARTESIAN_POINT('Ctrl Pts',(63.5016556949791,-14.85641574646,69.604876045245));
#143035=CARTESIAN_POINT('Ctrl Pts',(64.6260804730591,-15.20847950524,67.822908934237));
#143036=CARTESIAN_POINT('Ctrl Pts',(64.5533052413691,-15.20970453555,68.02494034063));
#143037=CARTESIAN_POINT('Ctrl Pts',(64.4577204629591,-15.19922013264,68.498512102653));
#143038=CARTESIAN_POINT('Ctrl Pts',(64.5278151508691,-15.14370900441,69.017398832301));
#143039=CARTESIAN_POINT('Ctrl Pts',(64.6218784967391,-15.09809367435,69.289035305194));
#143040=CARTESIAN_POINT('Ctrl Pts',(64.6330779166991,-15.09280488929,69.319208806332));
#143041=CARTESIAN_POINT('Ctrl Pts',(65.4174681368491,-14.3663713944,68.109543058174));
#143042=CARTESIAN_POINT('Ctrl Pts',(65.374277542859,-14.367601875,68.229634464589));
#143043=CARTESIAN_POINT('Ctrl Pts',(65.3173415915791,-14.35743446355,68.509807748111));
#143044=CARTESIAN_POINT('Ctrl Pts',(65.3563485675191,-14.30510185249,68.8160557029299));
#143045=CARTESIAN_POINT('Ctrl Pts',(65.4101046346091,-14.2618633586,68.977254924068));
#143046=CARTESIAN_POINT('Ctrl Pts',(65.4165145100791,-14.25684762985,68.995173914932));
#143047=CARTESIAN_POINT('Ctrl Pts',(65.1907448967991,-13.19994060407,68.034548919224));
#143048=CARTESIAN_POINT('Ctrl Pts',(65.1464477785891,-13.20117863405,68.159243937098));
#143049=CARTESIAN_POINT('Ctrl Pts',(65.0863781932991,-13.19145029757,68.439507002547));
#143050=CARTESIAN_POINT('Ctrl Pts',(65.1055421371491,-13.14352035198,68.739930520519));
#143051=CARTESIAN_POINT('Ctrl Pts',(65.1440468058491,-13.10357408963,68.905167920781));
#143052=CARTESIAN_POINT('Ctrl Pts',(65.148717761429,-13.0989365799,68.923639577176));
#143053=CARTESIAN_POINT('',(65.1554522360012,-13.4300820896322,68.8079743462767));
#143054=CARTESIAN_POINT('Origin',(63.6782406040291,-13.4300822103766,69.0684425118754));
#143055=CARTESIAN_POINT('',(65.176702388046,-13.4988189934219,68.1867892363913));
#143056=CARTESIAN_POINT('Ctrl Pts',(65.1766881521841,-13.49881898955,68.1867857093006));
#143057=CARTESIAN_POINT('Ctrl Pts',(65.1631764280226,-13.4974095391694,
68.2413218051627));
#143058=CARTESIAN_POINT('Ctrl Pts',(65.1528655627841,-13.4948284037889,
68.2960765161634));
#143059=CARTESIAN_POINT('Ctrl Pts',(65.1456380345049,-13.4910755834085,
68.3506775411135));
#143060=CARTESIAN_POINT('Ctrl Pts',(65.1383292863499,-13.4872805904355,
68.4058921490608));
#143061=CARTESIAN_POINT('Ctrl Pts',(65.1341731466497,-13.4822874307076,
68.4609493248272));
#143062=CARTESIAN_POINT('Ctrl Pts',(65.1330085931394,-13.4760961042247,
68.5155010552506));
#143063=CARTESIAN_POINT('Ctrl Pts',(65.1318220968064,-13.469788119144,68.5710806636891));
#143064=CARTESIAN_POINT('Ctrl Pts',(65.1337405720278,-13.4622363895776,
68.6261353347979));
#143065=CARTESIAN_POINT('Ctrl Pts',(65.1385592353595,-13.4534409155254,
68.680339376681));
#143066=CARTESIAN_POINT('Ctrl Pts',(65.1423934985484,-13.4464422604907,
68.7234701264704));
#143067=CARTESIAN_POINT('Ctrl Pts',(65.1480632663611,-13.4386561212723,
68.7660631216691));
#143068=CARTESIAN_POINT('Ctrl Pts',(65.1554529407002,-13.43008249787,68.8079742555258));
#143069=CARTESIAN_POINT('Origin',(63.7199392236019,-13.4984347767573,67.8257809705908));
#143070=CARTESIAN_POINT('Ctrl Pts',(66.3247580495291,-14.30756367035,64.653048442206));
#143071=CARTESIAN_POINT('Ctrl Pts',(66.2370201501591,-14.30418007722,64.660179387221));
#143072=CARTESIAN_POINT('Ctrl Pts',(65.8957020926591,-14.29548166727,64.699341304182));
#143073=CARTESIAN_POINT('Ctrl Pts',(65.2897313547191,-14.31367841804,64.848477924246));
#143074=CARTESIAN_POINT('Ctrl Pts',(64.4888593299491,-14.40595071535,65.229365043181));
#143075=CARTESIAN_POINT('Ctrl Pts',(63.6868754779191,-14.55587601027,65.891174774896));
#143076=CARTESIAN_POINT('Ctrl Pts',(63.0361776061691,-14.69164668395,66.864705767423));
#143077=CARTESIAN_POINT('Ctrl Pts',(62.8000900869391,-14.70223108065,67.6910995312599));
#143078=CARTESIAN_POINT('Ctrl Pts',(62.7500345788591,-14.67447645787,68.1072094165649));
#143079=CARTESIAN_POINT('Ctrl Pts',(62.7478962467391,-14.67314451722,68.126114759757));
#143080=CARTESIAN_POINT('Ctrl Pts',(66.3548790151891,-15.30077409373,65.9656697779481));
#143081=CARTESIAN_POINT('Ctrl Pts',(66.3133354429391,-15.29804521015,65.97128019847));
#143082=CARTESIAN_POINT('Ctrl Pts',(66.1545084345491,-15.29119071457,65.99560282881));
#143083=CARTESIAN_POINT('Ctrl Pts',(65.8756710738591,-15.30514064789,66.049701459109));
#143084=CARTESIAN_POINT('Ctrl Pts',(65.4157972527891,-15.38496723526,66.200633846256));
#143085=CARTESIAN_POINT('Ctrl Pts',(64.8331603453191,-15.53410391348,66.579998802577));
#143086=CARTESIAN_POINT('Ctrl Pts',(64.2808612154091,-15.68485087802,67.30171533471));
#143087=CARTESIAN_POINT('Ctrl Pts',(64.0735921049591,-15.69860285338,68.005645199803));
#143088=CARTESIAN_POINT('Ctrl Pts',(64.0381426791891,-15.66572474596,68.369480153518));
#143089=CARTESIAN_POINT('Ctrl Pts',(64.0366658453191,-15.66414383633,68.3860269579031));
#143090=CARTESIAN_POINT('Ctrl Pts',(66.4883687499992,-14.4250384257,67.353342695188));
#143091=CARTESIAN_POINT('Ctrl Pts',(66.4727224083191,-14.42173227018,67.35612722381));
#143092=CARTESIAN_POINT('Ctrl Pts',(66.4137416085591,-14.41325195438,67.367025031932));
#143093=CARTESIAN_POINT('Ctrl Pts',(66.3111555793591,-14.43094640088,67.38243504645));
#143094=CARTESIAN_POINT('Ctrl Pts',(66.1137087919391,-14.52174664686,67.430437654035));
#143095=CARTESIAN_POINT('Ctrl Pts',(65.8332830717091,-14.67157866592,67.593155113558));
#143096=CARTESIAN_POINT('Ctrl Pts',(65.5518702100291,-14.8091207025,67.943351706207));
#143097=CARTESIAN_POINT('Ctrl Pts',(65.4451062657591,-14.82007975348,68.3024447707801));
#143098=CARTESIAN_POINT('Ctrl Pts',(65.4282236829991,-14.79171913615,68.489615271462));
#143099=CARTESIAN_POINT('Ctrl Pts',(65.4275278935291,-14.790357748,68.4981302604861));
#143100=CARTESIAN_POINT('Ctrl Pts',(66.5523790655891,-12.81429647004,67.019249257931));
#143101=CARTESIAN_POINT('Ctrl Pts',(66.5088000219191,-12.80992853736,67.021561612314));
#143102=CARTESIAN_POINT('Ctrl Pts',(66.3377354711091,-12.79845784797,67.0378320936299));
#143103=CARTESIAN_POINT('Ctrl Pts',(66.0323010044891,-12.82303958328,67.120998532188));
#143104=CARTESIAN_POINT('Ctrl Pts',(65.6789083917491,-12.93402369634,67.326374170474));
#143105=CARTESIAN_POINT('Ctrl Pts',(65.3922421976991,-13.0851346569,67.618765808573));
#143106=CARTESIAN_POINT('Ctrl Pts',(65.2034480648691,-13.19838884926,67.958796807735));
#143107=CARTESIAN_POINT('Ctrl Pts',(65.1387376786991,-13.20421087014,68.1971895314531));
#143108=CARTESIAN_POINT('Ctrl Pts',(65.1203415613491,-13.18415927923,68.3120587081699));
#143109=CARTESIAN_POINT('Ctrl Pts',(65.1195350329091,-13.18320165728,68.3172685415469));
#143110=CARTESIAN_POINT('',(66.3723478475728,-13.1050046819904,67.0702812784609));
#143111=CARTESIAN_POINT('Ctrl Pts',(66.3723470578469,-13.10500468188,67.0702768035153));
#143112=CARTESIAN_POINT('Ctrl Pts',(66.3391116532978,-13.1050449423269,
67.0761335665632));
#143113=CARTESIAN_POINT('Ctrl Pts',(66.3045689466359,-13.1065804249721,
67.083375400249));
#143114=CARTESIAN_POINT('Ctrl Pts',(66.2688718737599,-13.1096111298157,
67.0922994496814));
#143115=CARTESIAN_POINT('Ctrl Pts',(66.2340002184672,-13.1125717561663,
67.101017149777));
#143116=CARTESIAN_POINT('Ctrl Pts',(66.1980266690957,-13.116959256602,67.1113407048153));
#143117=CARTESIAN_POINT('Ctrl Pts',(66.1611425862324,-13.1227736311227,
67.1235543419997));
#143118=CARTESIAN_POINT('Ctrl Pts',(66.1254109251342,-13.1284063388857,
67.1353863711779));
#143119=CARTESIAN_POINT('Ctrl Pts',(66.0888246147659,-13.1353781499622,
67.1489927704856));
#143120=CARTESIAN_POINT('Ctrl Pts',(66.0516068828885,-13.1436890643524,
67.1646309082111));
#143121=CARTESIAN_POINT('Ctrl Pts',(66.0440858281265,-13.1453685552589,
67.1677911032115));
#143122=CARTESIAN_POINT('Ctrl Pts',(66.0365391564341,-13.1471027316143,
67.171034249684));
#143123=CARTESIAN_POINT('Ctrl Pts',(66.0289689707891,-13.1488915934185,
67.1743624337803));
#143124=CARTESIAN_POINT('Ctrl Pts',(65.9928233038006,-13.1574329431415,
67.190253646977));
#143125=CARTESIAN_POINT('Ctrl Pts',(65.9561376823215,-13.1672210194115,
67.2080846714309));
#143126=CARTESIAN_POINT('Ctrl Pts',(65.9191702216006,-13.1782558222285,
67.2280750892431));
#143127=CARTESIAN_POINT('Ctrl Pts',(65.8833564575203,-13.1889462461054,
67.2474416373758));
#143128=CARTESIAN_POINT('Ctrl Pts',(65.84727825624,-13.2008067940272,67.2688354021097));
#143129=CARTESIAN_POINT('Ctrl Pts',(65.8112155646009,-13.2138374659941,
67.2924385375834));
#143130=CARTESIAN_POINT('Ctrl Pts',(65.7892798381047,-13.2217635869611,
67.3067955337108));
#143131=CARTESIAN_POINT('Ctrl Pts',(65.7673507305799,-13.2301226399125,
67.321969602589));
#143132=CARTESIAN_POINT('Ctrl Pts',(65.7454995863913,-13.2389146248483,
67.3379971598794));
#143133=CARTESIAN_POINT('Ctrl Pts',(65.7296903107005,-13.2452756150335,
67.3495930776797));
#143134=CARTESIAN_POINT('Ctrl Pts',(65.7139219774182,-13.2518632236623,
67.3616356827555));
#143135=CARTESIAN_POINT('Ctrl Pts',(65.6982237003632,-13.2586774507346,
67.3741373222992));
#143136=CARTESIAN_POINT('Ctrl Pts',(65.6903745618356,-13.2620845642708,
67.3803881420711));
#143137=CARTESIAN_POINT('Ctrl Pts',(65.6825429382797,-13.2655483324178,
67.3867537216006));
#143138=CARTESIAN_POINT('Ctrl Pts',(65.6747326640873,-13.2690687551758,
67.3932354506086));
#143139=CARTESIAN_POINT('Ctrl Pts',(65.6708275269912,-13.2708289665547,
67.3964763151126));
#143140=CARTESIAN_POINT('Ctrl Pts',(65.6669277271924,-13.2726033415864,
67.3997462169384));
#143141=CARTESIAN_POINT('Ctrl Pts',(65.6630337500704,-13.2743918802709,
67.4030453243454));
#143142=CARTESIAN_POINT('Ctrl Pts',(65.660251867848,-13.2756696237743,67.4054022278293));
#143143=CARTESIAN_POINT('Ctrl Pts',(65.6580604087891,-13.2766808889237,
67.4072712987835));
#143144=CARTESIAN_POINT('Ctrl Pts',(65.6551995973018,-13.2780122901473,
67.4097290096595));
#143145=CARTESIAN_POINT('Ctrl Pts',(65.6540559493652,-13.2785445357248,
67.4107115126957));
#143146=CARTESIAN_POINT('Ctrl Pts',(65.6528056389096,-13.2791279425155,
67.4117884475048));
#143147=CARTESIAN_POINT('Ctrl Pts',(65.6513697753868,-13.2797999872823,
67.4130304286083));
#143148=CARTESIAN_POINT('Ctrl Pts',(65.618531420134,-13.2951697243408,67.4414346718029));
#143149=CARTESIAN_POINT('Ctrl Pts',(65.5878590939958,-13.3097312798685,
67.4704571260051));
#143150=CARTESIAN_POINT('Ctrl Pts',(65.5592488544451,-13.3234846538655,
67.499768352367));
#143151=CARTESIAN_POINT('Ctrl Pts',(65.5295341230282,-13.3377689737737,
67.5302111320333));
#143152=CARTESIAN_POINT('Ctrl Pts',(65.5020432606503,-13.3511815083625,
67.5609651215252));
#143153=CARTESIAN_POINT('Ctrl Pts',(65.4766259981956,-13.3637222576317,
67.5917070571682));
#143154=CARTESIAN_POINT('Ctrl Pts',(65.4506520266231,-13.3765376843756,
67.6231223271604));
#143155=CARTESIAN_POINT('Ctrl Pts',(65.4268428557283,-13.3884427185039,
67.6545249450618));
#143156=CARTESIAN_POINT('Ctrl Pts',(65.4050124114097,-13.3994373600167,
67.6856194723999));
#143157=CARTESIAN_POINT('Ctrl Pts',(65.3824046098077,-13.4108235082041,
67.7178212404772));
#143158=CARTESIAN_POINT('Ctrl Pts',(65.3619183401328,-13.4212332733158,
67.749692514182));
#143159=CARTESIAN_POINT('Ctrl Pts',(65.3433293485563,-13.4306666553519,
67.7809589504468));
#143160=CARTESIAN_POINT('Ctrl Pts',(65.331487643871,-13.4366759820976,67.8008765400204));
#143161=CARTESIAN_POINT('Ctrl Pts',(65.3204155466602,-13.4422890882589,
67.8205497791698));
#143162=CARTESIAN_POINT('Ctrl Pts',(65.3100532853308,-13.447505973836,67.8399185337666));
#143163=CARTESIAN_POINT('Ctrl Pts',(65.2930999158816,-13.4560411560468,
67.8716071432325));
#143164=CARTESIAN_POINT('Ctrl Pts',(65.278046340807,-13.4635157666288,67.9024779678514));
#143165=CARTESIAN_POINT('Ctrl Pts',(65.264630059606,-13.4699298055819,67.9323119524872));
#143166=CARTESIAN_POINT('Ctrl Pts',(65.2506946713848,-13.4765920185706,
67.9633002831475));
#143167=CARTESIAN_POINT('Ctrl Pts',(65.2385250554639,-13.4821100002037,
67.9931701882726));
#143168=CARTESIAN_POINT('Ctrl Pts',(65.227835380454,-13.4864837504812,68.0217317365142));
#143169=CARTESIAN_POINT('Ctrl Pts',(65.2169231989982,-13.4909485407229,
68.0508877956813));
#143170=CARTESIAN_POINT('Ctrl Pts',(65.2075526093426,-13.494220969315,68.0786809186596));
#143171=CARTESIAN_POINT('Ctrl Pts',(65.1994379493454,-13.4963010362577,
68.104960526297));
#143172=CARTESIAN_POINT('Ctrl Pts',(65.1911190497657,-13.4984334568423,
68.1319015709006));
#143173=CARTESIAN_POINT('Ctrl Pts',(65.1841195422163,-13.4993127388276,
68.1572524438131));
#143174=CARTESIAN_POINT('Ctrl Pts',(65.1781597320144,-13.4989388822135,
68.1808971743649));
#143175=CARTESIAN_POINT('Ctrl Pts',(65.1776619856803,-13.4989076587763,
68.18287191476));
#143176=CARTESIAN_POINT('Ctrl Pts',(65.1771715099249,-13.4988676945552,
68.1848347781111));
#143177=CARTESIAN_POINT('Ctrl Pts',(65.1766881521841,-13.49881898955,68.1867857093006));
#143178=CARTESIAN_POINT('Ctrl Pts',(65.9990563614061,-14.4574811117313,
64.9541310528021));
#143179=CARTESIAN_POINT('Ctrl Pts',(66.0069547419919,-14.4793092068606,
64.9989444984957));
#143180=CARTESIAN_POINT('Ctrl Pts',(66.0150536595875,-14.4988596768414,
65.044891079552));
#143181=CARTESIAN_POINT('Ctrl Pts',(66.0233037502849,-14.516005350927,65.0916919095426));
#143182=CARTESIAN_POINT('Ctrl Pts',(66.0320127944002,-14.5341048406751,
65.1410962746547));
#143183=CARTESIAN_POINT('Ctrl Pts',(66.0408901082891,-14.5495248096361,
65.1914514973418));
#143184=CARTESIAN_POINT('Ctrl Pts',(66.049879846746,-14.5621739529066,65.2424419490977));
#143185=CARTESIAN_POINT('Ctrl Pts',(66.0592376012889,-14.5753409186053,
65.2955198149165));
#143186=CARTESIAN_POINT('Ctrl Pts',(66.0687170259418,-14.5855064940319,
65.3492851484083));
#143187=CARTESIAN_POINT('Ctrl Pts',(66.0782602192334,-14.5926194563088,
65.4034105789931));
#143188=CARTESIAN_POINT('Ctrl Pts',(66.0887744064903,-14.6004561431542,
65.4630431249489));
#143189=CARTESIAN_POINT('Ctrl Pts',(66.0993658663221,-14.6045887182656,
65.523112024764));
#143190=CARTESIAN_POINT('Ctrl Pts',(66.1099657432096,-14.6049928480227,
65.5832278089851));
#143191=CARTESIAN_POINT('Ctrl Pts',(66.1155120833583,-14.6052043071859,
65.6146831354134));
#143192=CARTESIAN_POINT('Ctrl Pts',(66.1210608803727,-14.6043955326921,
65.6461521569814));
#143193=CARTESIAN_POINT('Ctrl Pts',(66.1266031485341,-14.6025651695425,
65.6775840264054));
#143194=CARTESIAN_POINT('Ctrl Pts',(66.1363407838677,-14.5993492643643,
65.7328090847001));
#143195=CARTESIAN_POINT('Ctrl Pts',(66.1460503077678,-14.5929783595983,
65.7878746692027));
#143196=CARTESIAN_POINT('Ctrl Pts',(66.155666603048,-14.5834926139621,65.8424115397955));
#143197=CARTESIAN_POINT('Ctrl Pts',(66.1657629405947,-14.5735333430542,
65.8996708728552));
#143198=CARTESIAN_POINT('Ctrl Pts',(66.1757564492557,-14.5601408008186,
65.956347045915));
#143199=CARTESIAN_POINT('Ctrl Pts',(66.1855765340643,-14.5434124527068,
66.0120397024279));
#143200=CARTESIAN_POINT('Ctrl Pts',(66.1956851946349,-14.5261925206731,
66.0693689589401));
#143201=CARTESIAN_POINT('Ctrl Pts',(66.2056100906302,-14.5054382282124,
66.1256560523008));
#143202=CARTESIAN_POINT('Ctrl Pts',(66.2152795913734,-14.481302712779,66.1804947231858));
#143203=CARTESIAN_POINT('Ctrl Pts',(66.2252319917202,-14.456461067016,66.2369378035087));
#143204=CARTESIAN_POINT('Ctrl Pts',(66.2349138675465,-14.4280375351101,
66.291846655123));
#143205=CARTESIAN_POINT('Ctrl Pts',(66.2442524298549,-14.3962441949578,
66.3448084647408));
#143206=CARTESIAN_POINT('Ctrl Pts',(66.2463349419034,-14.3891542370238,
66.356619020049));
#143207=CARTESIAN_POINT('Ctrl Pts',(66.2484004002693,-14.3818968727244,
66.3683328586023));
#143208=CARTESIAN_POINT('Ctrl Pts',(66.2504480296382,-14.3744747519765,
66.37994558372));
#143209=CARTESIAN_POINT('Ctrl Pts',(66.2597159703859,-14.3408808915069,
66.4325068772548));
#143210=CARTESIAN_POINT('Ctrl Pts',(66.2686129326532,-14.3039273404708,
66.4829645574844));
#143211=CARTESIAN_POINT('Ctrl Pts',(66.2770714108995,-14.263898617603,66.5309354107161));
#143212=CARTESIAN_POINT('Ctrl Pts',(66.2851736588896,-14.2255557112358,
66.5768859632702));
#143213=CARTESIAN_POINT('Ctrl Pts',(66.2928736045143,-14.1843911377398,
66.6205548920699));
#143214=CARTESIAN_POINT('Ctrl Pts',(66.3001161560663,-14.1406963638839,
66.6616296477246));
#143215=CARTESIAN_POINT('Ctrl Pts',(66.307148361561,-14.0982706211612,66.7015114656637));
#143216=CARTESIAN_POINT('Ctrl Pts',(66.3137493144063,-14.0534593449539,
66.7389473766632));
#143217=CARTESIAN_POINT('Ctrl Pts',(66.3198728148747,-14.0065712294518,
66.7736754547477));
#143218=CARTESIAN_POINT('Ctrl Pts',(66.3257509833222,-13.9615616401617,
66.8070121865545));
#143219=CARTESIAN_POINT('Ctrl Pts',(66.3311891229665,-13.9146383488563,
66.8378533321756));
#143220=CARTESIAN_POINT('Ctrl Pts',(66.3361511159024,-13.8661143232919,
66.8659942805906));
#143221=CARTESIAN_POINT('Ctrl Pts',(66.3373696432826,-13.8541981729645,
66.8729049144006));
#143222=CARTESIAN_POINT('Ctrl Pts',(66.3385594824833,-13.8421856810548,
66.8796528600556));
#143223=CARTESIAN_POINT('Ctrl Pts',(66.3397201532679,-13.8300818586723,
66.886235398542));
#143224=CARTESIAN_POINT('Ctrl Pts',(66.3450140367401,-13.7748756571299,
66.9162587196766));
#143225=CARTESIAN_POINT('Ctrl Pts',(66.3496974087145,-13.7178145654519,
66.942815204432));
#143226=CARTESIAN_POINT('Ctrl Pts',(66.3537436587053,-13.6592730960824,
66.9657431428049));
#143227=CARTESIAN_POINT('Ctrl Pts',(66.3573093551042,-13.6076843146192,
66.9859480405442));
#143228=CARTESIAN_POINT('Ctrl Pts',(66.3603800645005,-13.5549457672634,
67.0033339489328));
#143229=CARTESIAN_POINT('Ctrl Pts',(66.3629385113433,-13.5013556708403,
67.0177941584979));
#143230=CARTESIAN_POINT('Ctrl Pts',(66.3653860939825,-13.4500877736746,
67.0316277693041));
#143231=CARTESIAN_POINT('Ctrl Pts',(66.3673646518407,-13.3980405699007,
67.0427826803886));
#143232=CARTESIAN_POINT('Ctrl Pts',(66.3688628389521,-13.3455170266702,
67.0511848303657));
#143233=CARTESIAN_POINT('Ctrl Pts',(66.3702937991307,-13.2953503297189,
67.0592099574937));
#143234=CARTESIAN_POINT('Ctrl Pts',(66.371286385483,-13.2447495890845,67.0647230188068));
#143235=CARTESIAN_POINT('Ctrl Pts',(66.3718366772028,-13.1940136326873,
67.0676908984141));
#143236=CARTESIAN_POINT('Ctrl Pts',(66.3721582180026,-13.1643681202944,
67.0694250593116));
#143237=CARTESIAN_POINT('Ctrl Pts',(66.3723288762056,-13.1346770820982,
67.0702909089734));
#143238=CARTESIAN_POINT('Ctrl Pts',(66.3723491609777,-13.1050046822981,
67.0702887165938));
#143239=CARTESIAN_POINT('Origin',(58.0356083261291,-9.5,68.77323523472));
#143240=CARTESIAN_POINT('',(91.0790815025691,-12.28281717502,58.13146250234));
#143241=CARTESIAN_POINT('Ctrl Pts',(91.0790815025691,-12.28281717502,58.13146250234));
#143242=CARTESIAN_POINT('Ctrl Pts',(91.1199088515142,-12.6925940776003,
58.3651513297703));
#143243=CARTESIAN_POINT('Ctrl Pts',(91.1722707753266,-13.0779420821198,
58.6612655335377));
#143244=CARTESIAN_POINT('Ctrl Pts',(91.2926220959915,-13.7595612344036,
59.3421440579158));
#143245=CARTESIAN_POINT('Ctrl Pts',(91.3603889077048,-14.0537040594648,
59.7262617256362));
#143246=CARTESIAN_POINT('Ctrl Pts',(91.506357098809,-14.5281559853725,60.5547725075601));
#143247=CARTESIAN_POINT('Ctrl Pts',(91.5847883885152,-14.709288519388,61.000020579335));
#143248=CARTESIAN_POINT('Ctrl Pts',(91.7477452037583,-14.9479889262476,
61.9239589072862));
#143249=CARTESIAN_POINT('Ctrl Pts',(91.8320334198305,-15.0060365273816,
62.4015858279761));
#143250=CARTESIAN_POINT('Ctrl Pts',(91.9155434595542,-14.9991665213493,
62.8752786410684));
#143251=CARTESIAN_POINT('',(91.0413458950691,-11.874941516,57.91633991463));
#143252=CARTESIAN_POINT('Ctrl Pts',(91.0413458950691,-11.874941516,57.91633991463));
#143253=CARTESIAN_POINT('Ctrl Pts',(91.0543131272762,-12.024294137281,57.9879089911249));
#143254=CARTESIAN_POINT('Ctrl Pts',(91.0660084826674,-12.16018136282,58.0593039544405));
#143255=CARTESIAN_POINT('Ctrl Pts',(91.07908074693,-12.2828100865246,58.1314583314809));
#143256=CARTESIAN_POINT('',(87.2166270801612,-11.8742918211854,58.592003722724));
#143257=CARTESIAN_POINT('Ctrl Pts',(87.2164851556291,-11.87468271151,58.59119882454));
#143258=CARTESIAN_POINT('Ctrl Pts',(88.491322681793,-11.8750882864112,58.365587681618));
#143259=CARTESIAN_POINT('Ctrl Pts',(89.7663021731098,-11.8751032627281,
58.1407816630862));
#143260=CARTESIAN_POINT('Ctrl Pts',(91.0413458950691,-11.874941516,57.91633991463));
#143261=CARTESIAN_POINT('Origin',(88.0778048294691,-9.5,63.475985431442));
#143262=CARTESIAN_POINT('Origin',(88.0778048294691,-9.5,63.475985431442));
#143263=CARTESIAN_POINT('',(86.3881929029811,-11.4435878621033,59.6524812960673));
#143264=CARTESIAN_POINT('Ctrl Pts',(87.2166270533076,-11.8742914943215,
58.5920035689655));
#143265=CARTESIAN_POINT('Ctrl Pts',(87.1733550876063,-11.8742658138293,
58.5996210997768));
#143266=CARTESIAN_POINT('Ctrl Pts',(87.1305249711706,-11.8729960713397,
58.6098208361203));
#143267=CARTESIAN_POINT('Ctrl Pts',(87.0885121797564,-11.8704898997059,
58.6225169055592));
#143268=CARTESIAN_POINT('Ctrl Pts',(87.0465172644131,-11.8679847944259,
58.6352075729329));
#143269=CARTESIAN_POINT('Ctrl Pts',(87.0053394416954,-11.8642443312419,
58.6503923191013));
#143270=CARTESIAN_POINT('Ctrl Pts',(86.9653398723854,-11.859298361522,58.6679403817511));
#143271=CARTESIAN_POINT('Ctrl Pts',(86.9253413449803,-11.8543525206343,
58.6854879873107));
#143272=CARTESIAN_POINT('Ctrl Pts',(86.8865214517456,-11.8482012828593,
58.7053986005361));
#143273=CARTESIAN_POINT('Ctrl Pts',(86.8492206895109,-11.8408962348827,
58.7274988317037));
#143274=CARTESIAN_POINT('Ctrl Pts',(86.8119302495413,-11.833593208437,58.7495929470594));
#143275=CARTESIAN_POINT('Ctrl Pts',(86.77615850976,-11.8251370862027,58.7738752269925));
#143276=CARTESIAN_POINT('Ctrl Pts',(86.7422186640335,-11.8156002149462,
58.8001330226941));
#143277=CARTESIAN_POINT('Ctrl Pts',(86.7082697178207,-11.8060607865134,
58.8263978590496));
#143278=CARTESIAN_POINT('Ctrl Pts',(86.6761540216081,-11.7954401303729,
58.8546389828117));
#143279=CARTESIAN_POINT('Ctrl Pts',(86.6461520958714,-11.7838301429435,
58.8846081166276));
#143280=CARTESIAN_POINT('Ctrl Pts',(86.6176861844754,-11.7728145542652,
58.9130429149572));
#143281=CARTESIAN_POINT('Ctrl Pts',(86.5911231320854,-11.7609085815675,
58.943032806359));
#143282=CARTESIAN_POINT('Ctrl Pts',(86.5666708390468,-11.7482055380309,
58.9743400397999));
#143283=CARTESIAN_POINT('Ctrl Pts',(86.5406752356164,-11.7347007398667,
59.007623234294));
#143284=CARTESIAN_POINT('Ctrl Pts',(86.5170617786849,-11.7202932043829,
59.0424004060605));
#143285=CARTESIAN_POINT('Ctrl Pts',(86.4960387773943,-11.7051095247828,
59.0783644560062));
#143286=CARTESIAN_POINT('Ctrl Pts',(86.4750173510482,-11.6899269826728,
59.1143258116941));
#143287=CARTESIAN_POINT('Ctrl Pts',(86.4565862107747,-11.6739685704833,
59.1514734922184));
#143288=CARTESIAN_POINT('Ctrl Pts',(86.4409079191863,-11.6573746042409,
59.1894795581048));
#143289=CARTESIAN_POINT('Ctrl Pts',(86.425225638195,-11.6407764155988,59.2274952947838));
#143290=CARTESIAN_POINT('Ctrl Pts',(86.4122977726285,-11.6235425217402,
59.2663694576407));
#143291=CARTESIAN_POINT('Ctrl Pts',(86.4022383956474,-11.6058246270749,
59.3057587287828));
#143292=CARTESIAN_POINT('Ctrl Pts',(86.3921809072349,-11.5881100588044,
59.3451406049005));
#143293=CARTESIAN_POINT('Ctrl Pts',(86.3849909337562,-11.5699118565233,
59.3850369848708));
#143294=CARTESIAN_POINT('Ctrl Pts',(86.3807318812011,-11.5513902301268,
59.4250956854601));
#143295=CARTESIAN_POINT('Ctrl Pts',(86.37647211738,-11.5328655106001,59.4651610758927));
#143296=CARTESIAN_POINT('Ctrl Pts',(86.3751442993911,-11.5140174524455,
59.5053884234905));
#143297=CARTESIAN_POINT('Ctrl Pts',(86.3767601154266,-11.4950120983375,
59.5454225279031));
#143298=CARTESIAN_POINT('Ctrl Pts',(86.3782101629784,-11.4779565260503,
59.5813494860583));
#143299=CARTESIAN_POINT('Ctrl Pts',(86.3820301552334,-11.4607744513163,
59.6171205724333));
#143300=CARTESIAN_POINT('Ctrl Pts',(86.3881929029811,-11.4435878621033,
59.6524812960673));
#143301=CARTESIAN_POINT('',(87.1036278102967,-13.9987735363373,63.7099253475457));
#143302=CARTESIAN_POINT('Origin',(87.0929970764191,-9.5,63.649633609109));
#143303=CARTESIAN_POINT('Ctrl Pts',(88.0907987596691,-14.99868011451,63.549677671879));
#143304=CARTESIAN_POINT('Ctrl Pts',(87.8327127247742,-14.9994907916134,
63.5951963601042));
#143305=CARTESIAN_POINT('Ctrl Pts',(87.5759653099965,-14.8914956855539,
63.6389755291981));
#143306=CARTESIAN_POINT('Ctrl Pts',(87.2105814416028,-14.5207989635053,
63.6982800998973));
#143307=CARTESIAN_POINT('Ctrl Pts',(87.1040483163665,-14.2605452795666,
63.7134684546579));
#143308=CARTESIAN_POINT('Ctrl Pts',(87.1036271773116,-13.9987735308997,
63.7099254590822));
#143309=CARTESIAN_POINT('Origin',(88.0541760202691,0.499074165591714,63.341979795825));
#143310=CARTESIAN_POINT('',(87.2268050854822,-13.9725532728231,64.4084965381912));
#143311=CARTESIAN_POINT('Origin',(87.0693682672991,0.499074165591714,63.515627973491));
#143312=CARTESIAN_POINT('Origin',(88.2115792922668,-13.9725914352474,64.234869837276));
#143313=CARTESIAN_POINT('Ctrl Pts',(85.9869779804892,-14.45602459315,67.672990289305));
#143314=CARTESIAN_POINT('Ctrl Pts',(86.1188182448091,-14.45335775601,67.662512009987));
#143315=CARTESIAN_POINT('Ctrl Pts',(86.5288714744991,-14.45079478986,67.60303640583));
#143316=CARTESIAN_POINT('Ctrl Pts',(87.1981096901091,-14.47737661549,67.359429353844));
#143317=CARTESIAN_POINT('Ctrl Pts',(87.9232293938691,-14.55613194807,66.826118621937));
#143318=CARTESIAN_POINT('Ctrl Pts',(88.4877746877692,-14.66433129533,66.054781967478));
#143319=CARTESIAN_POINT('Ctrl Pts',(88.7930035000691,-14.7713702607,65.092548915634));
#143320=CARTESIAN_POINT('Ctrl Pts',(88.7694653550692,-14.8243760301,64.337245624157));
#143321=CARTESIAN_POINT('Ctrl Pts',(88.6750970702691,-14.84113316934,63.942676946827));
#143322=CARTESIAN_POINT('Ctrl Pts',(88.6595111695691,-14.84334740449,63.885082644327));
#143323=CARTESIAN_POINT('Ctrl Pts',(85.9335802203091,-15.01572702015,66.7387418852801));
#143324=CARTESIAN_POINT('Ctrl Pts',(86.0152075191491,-15.01321673433,66.731223622732));
#143325=CARTESIAN_POINT('Ctrl Pts',(86.2682166275592,-15.0109676354,66.693423484771));
#143326=CARTESIAN_POINT('Ctrl Pts',(86.6862036438991,-15.03579852014,66.553203088848));
#143327=CARTESIAN_POINT('Ctrl Pts',(87.1727929355791,-15.11147478167,66.234254228036));
#143328=CARTESIAN_POINT('Ctrl Pts',(87.5896609990691,-15.21882727978,65.731333854876));
#143329=CARTESIAN_POINT('Ctrl Pts',(87.8421542441691,-15.32805298848,65.053945148687));
#143330=CARTESIAN_POINT('Ctrl Pts',(87.8414001753692,-15.38310788666,64.498042625236));
#143331=CARTESIAN_POINT('Ctrl Pts',(87.7768598826691,-15.40041417173,64.2066844999171));
#143332=CARTESIAN_POINT('Ctrl Pts',(87.766043127269,-15.40269862144,64.164158809273));
#143333=CARTESIAN_POINT('Ctrl Pts',(85.8554993785191,-14.34158763438,65.885303472011));
#143334=CARTESIAN_POINT('Ctrl Pts',(85.9044684357291,-14.33888878869,65.880917669075));
#143335=CARTESIAN_POINT('Ctrl Pts',(86.0563563157591,-14.33626164914,65.858358908938));
#143336=CARTESIAN_POINT('Ctrl Pts',(86.3066718932891,-14.36320147278,65.772958420671));
#143337=CARTESIAN_POINT('Ctrl Pts',(86.5940361948891,-14.44258635333,65.580259831417));
#143338=CARTESIAN_POINT('Ctrl Pts',(86.8359877173291,-14.55095884767,65.281614918033));
#143339=CARTESIAN_POINT('Ctrl Pts',(86.9797906777992,-14.65755071071,64.885100969035));
#143340=CARTESIAN_POINT('Ctrl Pts',(86.9776694167192,-14.71013751451,64.562268729993));
#143341=CARTESIAN_POINT('Ctrl Pts',(86.9396893054491,-14.7267823752,64.393163885495));
#143342=CARTESIAN_POINT('Ctrl Pts',(86.9333411474091,-14.72898225425,64.368481564751));
#143343=CARTESIAN_POINT('Ctrl Pts',(85.8531929635192,-13.30094292267,66.210694673787));
#143344=CARTESIAN_POINT('Ctrl Pts',(85.9290760517791,-13.2979530039,66.205583603029));
#143345=CARTESIAN_POINT('Ctrl Pts',(86.1658664817091,-13.29474229664,66.172222829911));
#143346=CARTESIAN_POINT('Ctrl Pts',(86.5478136567391,-13.32493761335,66.022545122284));
#143347=CARTESIAN_POINT('Ctrl Pts',(86.9315779387592,-13.41004735564,65.705553711945));
#143348=CARTESIAN_POINT('Ctrl Pts',(87.1964183130791,-13.51999438146,65.284226038267));
#143349=CARTESIAN_POINT('Ctrl Pts',(87.3154153783191,-13.62252047174,64.803248481328));
#143350=CARTESIAN_POINT('Ctrl Pts',(87.2895346633291,-13.67129736704,64.447291703555));
#143351=CARTESIAN_POINT('Ctrl Pts',(87.2406750363991,-13.68692121071,64.26219383718));
#143352=CARTESIAN_POINT('Ctrl Pts',(87.2327457050291,-13.68899054109,64.235172662353));
#143353=CARTESIAN_POINT('',(86.0102737124181,-13.5950714519424,66.1461371018416));
#143354=CARTESIAN_POINT('Ctrl Pts',(86.0102754056894,-13.5950714520587,
66.1461466969166));
#143355=CARTESIAN_POINT('Ctrl Pts',(86.0492876851558,-13.5950562057199,
66.1392620846122));
#143356=CARTESIAN_POINT('Ctrl Pts',(86.0892387535854,-13.5958711067968,
66.1306186693381));
#143357=CARTESIAN_POINT('Ctrl Pts',(86.1299313365959,-13.5975161552896,
66.1199521500868));
#143358=CARTESIAN_POINT('Ctrl Pts',(86.1697969025363,-13.5991277705844,
66.1095024121958));
#143359=CARTESIAN_POINT('Ctrl Pts',(86.2103742594308,-13.6015361331266,
66.0971104528392));
#143360=CARTESIAN_POINT('Ctrl Pts',(86.2514298118022,-13.6047412429161,
66.0825351254452));
#143361=CARTESIAN_POINT('Ctrl Pts',(86.2911847028321,-13.6078448131536,
66.0684215520355));
#143362=CARTESIAN_POINT('Ctrl Pts',(86.3313879017758,-13.6116954475604,
66.0522602815009));
#143363=CARTESIAN_POINT('Ctrl Pts',(86.3717816078402,-13.6162931461365,
66.0338465287676));
#143364=CARTESIAN_POINT('Ctrl Pts',(86.4121185431954,-13.6208843829483,
66.0154586553582));
#143365=CARTESIAN_POINT('Ctrl Pts',(86.4526455344907,-13.6262205855055,
65.9948240255609));
#143366=CARTESIAN_POINT('Ctrl Pts',(86.493059073377,-13.632301753808,65.9717611584834));
#143367=CARTESIAN_POINT('Ctrl Pts',(86.5317954639478,-13.6381305556647,
65.949655392658));
#143368=CARTESIAN_POINT('Ctrl Pts',(86.5704272936403,-13.6446437746059,
65.9253183810991));
#143369=CARTESIAN_POINT('Ctrl Pts',(86.6086463440478,-13.6518414106316,
65.8986178782715));
#143370=CARTESIAN_POINT('Ctrl Pts',(86.6462018383928,-13.6589140818826,
65.8723809474148));
#143371=CARTESIAN_POINT('Ctrl Pts',(86.6833585620957,-13.6666476109382,
65.8438614184352));
#143372=CARTESIAN_POINT('Ctrl Pts',(86.7197870729016,-13.6750419977982,
65.8129673352123));
#143373=CARTESIAN_POINT('Ctrl Pts',(86.7553577534027,-13.683238710933,65.782800755811));
#143374=CARTESIAN_POINT('Ctrl Pts',(86.7902338105182,-13.6920655241485,
65.7503697580506));
#143375=CARTESIAN_POINT('Ctrl Pts',(86.8240766932061,-13.7015224374449,
65.7156270904934));
#143376=CARTESIAN_POINT('Ctrl Pts',(86.8332160850262,-13.7040763107902,
65.7062447085431));
#143377=CARTESIAN_POINT('Ctrl Pts',(86.8422799602235,-13.7066761366659,
65.6966939774646));
#143378=CARTESIAN_POINT('Ctrl Pts',(86.8512612876911,-13.7093219150721,
65.6869745180572));
#143379=CARTESIAN_POINT('Ctrl Pts',(86.8697546103514,-13.7147697994666,
65.6669613184994));
#143380=CARTESIAN_POINT('Ctrl Pts',(86.8878980994665,-13.7204125149521,
65.6462324301027));
#143381=CARTESIAN_POINT('Ctrl Pts',(86.9056284488882,-13.7262500615288,
65.6247880383187));
#143382=CARTESIAN_POINT('Ctrl Pts',(86.914493623599,-13.7291688348171,65.6140658424267));
#143383=CARTESIAN_POINT('Ctrl Pts',(86.923255526305,-13.7321363158782,65.6031647811458));
#143384=CARTESIAN_POINT('Ctrl Pts',(86.931905959028,-13.7351525047121,65.5920854172301));
#143385=CARTESIAN_POINT('Ctrl Pts',(86.9362311753895,-13.7366605991291,
65.5865457352722));
#143386=CARTESIAN_POINT('Ctrl Pts',(86.9405285254553,-13.7381808704892,
65.5809614786555));
#143387=CARTESIAN_POINT('Ctrl Pts',(86.94479697978,-13.7397133187925,65.5753327385516));
#143388=CARTESIAN_POINT('Ctrl Pts',(86.9473884578402,-13.740643703858,65.5719153993049));
#143389=CARTESIAN_POINT('Ctrl Pts',(86.9495048194128,-13.7414089232411,
65.5691004992296));
#143390=CARTESIAN_POINT('Ctrl Pts',(86.9519942293893,-13.7423179797889,
65.5657627451645));
#143391=CARTESIAN_POINT('Ctrl Pts',(86.9536051561832,-13.7429062410893,
65.5636028448244));
#143392=CARTESIAN_POINT('Ctrl Pts',(86.9553717945738,-13.7435547347487,
65.5612236041841));
#143393=CARTESIAN_POINT('Ctrl Pts',(86.957514624389,-13.744347194532,65.5583131708614));
#143394=CARTESIAN_POINT('Ctrl Pts',(86.9847172363177,-13.7544072449398,
65.5213660518397));
#143395=CARTESIAN_POINT('Ctrl Pts',(87.0095589313433,-13.764145285636,65.4840751543646));
#143396=CARTESIAN_POINT('Ctrl Pts',(87.0321894775652,-13.7735613166208,
65.4467565493519));
#143397=CARTESIAN_POINT('Ctrl Pts',(87.0553307906926,-13.7831898655431,
65.4085956708822));
#143398=CARTESIAN_POINT('Ctrl Pts',(87.0761605696567,-13.7924817053338,
65.3704059473313));
#143399=CARTESIAN_POINT('Ctrl Pts',(87.0948671719668,-13.8014368359929,
65.3324778916709));
#143400=CARTESIAN_POINT('Ctrl Pts',(87.114960647704,-13.8110558837302,65.2917379190378));
#143401=CARTESIAN_POINT('Ctrl Pts',(87.1326049450955,-13.8202864456207,
65.251300355813));
#143402=CARTESIAN_POINT('Ctrl Pts',(87.1480577281618,-13.8291285216646,
65.211465491273));
#143403=CARTESIAN_POINT('Ctrl Pts',(87.1633255765337,-13.8378647781534,
65.1721073595302));
#143404=CARTESIAN_POINT('Ctrl Pts',(87.1764547697631,-13.8462217917393,
65.1333371825646));
#143405=CARTESIAN_POINT('Ctrl Pts',(87.1877068794637,-13.8541995624225,
65.0953888662222));
#143406=CARTESIAN_POINT('Ctrl Pts',(87.1993786382646,-13.8624748652468,
65.0560252617927));
#143407=CARTESIAN_POINT('Ctrl Pts',(87.2090313008149,-13.870342109828,65.0175459071096));
#143408=CARTESIAN_POINT('Ctrl Pts',(87.2169608558396,-13.8778012961662,
64.9801544525308));
#143409=CARTESIAN_POINT('Ctrl Pts',(87.2245979934478,-13.8849854108275,
64.9441418789246));
#143410=CARTESIAN_POINT('Ctrl Pts',(87.2306372077812,-13.8917910081719,
64.9091377462617));
#143411=CARTESIAN_POINT('Ctrl Pts',(87.2353388130221,-13.8982180881996,
64.8752784912196));
#143412=CARTESIAN_POINT('Ctrl Pts',(87.2404731788812,-13.9052367506725,
64.8383026512263));
#143413=CARTESIAN_POINT('Ctrl Pts',(87.2440130153083,-13.9118040074304,
64.8026923280386));
#143414=CARTESIAN_POINT('Ctrl Pts',(87.2462835806719,-13.9179198584735,
64.7685728342865));
#143415=CARTESIAN_POINT('Ctrl Pts',(87.2486150854234,-13.9241998519917,
64.7335376121884));
#143416=CARTESIAN_POINT('Ctrl Pts',(87.2496087866808,-13.9300038842062,
64.700073851738));
#143417=CARTESIAN_POINT('Ctrl Pts',(87.2495938463983,-13.9353319551167,
64.6682673708162));
#143418=CARTESIAN_POINT('Ctrl Pts',(87.2495783399401,-13.940861938145,64.6352555542241));
#143419=CARTESIAN_POINT('Ctrl Pts',(87.2484768178698,-13.9458792023638,
64.6040285120549));
#143420=CARTESIAN_POINT('Ctrl Pts',(87.2466246838941,-13.9503837477732,
64.5746365608777));
#143421=CARTESIAN_POINT('Ctrl Pts',(87.2447359087654,-13.9549774075446,
64.5446631425953));
#143422=CARTESIAN_POINT('Ctrl Pts',(87.2420668685604,-13.9590378613946,
64.5165974609744));
#143423=CARTESIAN_POINT('Ctrl Pts',(87.2389334330773,-13.9625651093231,
64.4904556039545));
#143424=CARTESIAN_POINT('Ctrl Pts',(87.2357270569359,-13.9661744651449,
64.4637052122221));
#143425=CARTESIAN_POINT('Ctrl Pts',(87.2320346909611,-13.969225501994,64.4389685682266));
#143426=CARTESIAN_POINT('Ctrl Pts',(87.2281486846861,-13.9717182198705,
64.4162347826597));
#143427=CARTESIAN_POINT('Ctrl Pts',(87.2277032801709,-13.9720039290842,
64.4136290918749));
#143428=CARTESIAN_POINT('Ctrl Pts',(87.2272552806075,-13.9722823035597,
64.4110496898349));
#143429=CARTESIAN_POINT('Ctrl Pts',(87.2268050864046,-13.9725533432969,
64.4084965434475));
#143430=CARTESIAN_POINT('Ctrl Pts',(86.2245100214957,-14.5670381546648,
67.3623544046571));
#143431=CARTESIAN_POINT('Ctrl Pts',(86.21790608955,-14.5762309095507,67.3249068234169));
#143432=CARTESIAN_POINT('Ctrl Pts',(86.2112032324775,-14.5831956362181,
67.2868968861811));
#143433=CARTESIAN_POINT('Ctrl Pts',(86.2044540605054,-14.5878733629712,
67.248623365796));
#143434=CARTESIAN_POINT('Ctrl Pts',(86.197437632731,-14.5927363197972,67.2088342786954));
#143435=CARTESIAN_POINT('Ctrl Pts',(86.1903713000755,-14.595128429718,67.168761175206));
#143436=CARTESIAN_POINT('Ctrl Pts',(86.1833095869423,-14.5950365325702,
67.1287136717026));
#143437=CARTESIAN_POINT('Ctrl Pts',(86.1755325592852,-14.5949353267232,
67.0846095660177));
#143438=CARTESIAN_POINT('Ctrl Pts',(86.1677612647959,-14.5918224815627,
67.0405372500604));
#143439=CARTESIAN_POINT('Ctrl Pts',(86.1600605535813,-14.5857283801364,
66.996864939702));
#143440=CARTESIAN_POINT('Ctrl Pts',(86.1555769842231,-14.5821802239129,
66.9714376996629));
#143441=CARTESIAN_POINT('Ctrl Pts',(86.1511171770846,-14.5776222205114,
66.9461451210373));
#143442=CARTESIAN_POINT('Ctrl Pts',(86.146692761572,-14.5720643646981,66.9210532283303));
#143443=CARTESIAN_POINT('Ctrl Pts',(86.1394556395654,-14.5629732473513,
66.8800098208153));
#143444=CARTESIAN_POINT('Ctrl Pts',(86.1323177597175,-14.5512087224418,
66.8395292495397));
#143445=CARTESIAN_POINT('Ctrl Pts',(86.1253401741445,-14.5368699810008,
66.7999577493598));
#143446=CARTESIAN_POINT('Ctrl Pts',(86.1181504314958,-14.5220952627563,
66.7591830573775));
#143447=CARTESIAN_POINT('Ctrl Pts',(86.1111308966058,-14.5045878930689,
66.7193736581523));
#143448=CARTESIAN_POINT('Ctrl Pts',(86.1043425244012,-14.4845020933198,
66.6808752405993));
#143449=CARTESIAN_POINT('Ctrl Pts',(86.0973159958783,-14.4637116238834,
66.6410261838784));
#143450=CARTESIAN_POINT('Ctrl Pts',(86.0905371172554,-14.4401588108996,
66.6025816115021));
#143451=CARTESIAN_POINT('Ctrl Pts',(86.0840673353281,-14.4140575196726,
66.5658900139963));
#143452=CARTESIAN_POINT('Ctrl Pts',(86.0814287747804,-14.4034126728985,
66.5509261399891));
#143453=CARTESIAN_POINT('Ctrl Pts',(86.0788415569041,-14.392344423101,66.5362534449891));
#143454=CARTESIAN_POINT('Ctrl Pts',(86.076309583227,-14.3808692039259,66.521894057092));
#143455=CARTESIAN_POINT('Ctrl Pts',(86.0701221752456,-14.3528271024801,
66.486803885308));
#143456=CARTESIAN_POINT('Ctrl Pts',(86.0642677470609,-14.3223642102344,
66.4536021666565));
#143457=CARTESIAN_POINT('Ctrl Pts',(86.0587985898109,-14.2897543905021,
66.4225854143852));
#143458=CARTESIAN_POINT('Ctrl Pts',(86.0534543531146,-14.2578894088772,
66.3922771131036));
#143459=CARTESIAN_POINT('Ctrl Pts',(86.0484779941468,-14.2239742656419,
66.3640551372869));
#143460=CARTESIAN_POINT('Ctrl Pts',(86.0439131969578,-14.1883035423802,
66.3381672267215));
#143461=CARTESIAN_POINT('Ctrl Pts',(86.0395484851462,-14.1541963475362,
66.3134140417839));
#143462=CARTESIAN_POINT('Ctrl Pts',(86.0355600908499,-14.1184841072631,
66.2907950438382));
#143463=CARTESIAN_POINT('Ctrl Pts',(86.0319811186901,-14.0814617480119,
66.2704980036799));
#143464=CARTESIAN_POINT('Ctrl Pts',(86.030405635642,-14.0651643037178,66.2615631359944));
#143465=CARTESIAN_POINT('Ctrl Pts',(86.0289094185842,-14.0486134846307,
66.2530778102736));
#143466=CARTESIAN_POINT('Ctrl Pts',(86.0274949090129,-14.0318368536377,
66.2450558766909));
#143467=CARTESIAN_POINT('Ctrl Pts',(86.0241177110331,-13.991781978473,66.2259031905307));
#143468=CARTESIAN_POINT('Ctrl Pts',(86.0212088028127,-13.9504617089997,
66.2094036096931));
#143469=CARTESIAN_POINT('Ctrl Pts',(86.0187949238061,-13.9081978233312,
66.1956794901586));
#143470=CARTESIAN_POINT('Ctrl Pts',(86.0165451824516,-13.8688077747309,
66.1828885759558));
#143471=CARTESIAN_POINT('Ctrl Pts',(86.0147255938159,-13.8285977890043,
66.1725095723019));
#143472=CARTESIAN_POINT('Ctrl Pts',(86.0133551556414,-13.7878683714231,
66.1646254052992));
#143473=CARTESIAN_POINT('Ctrl Pts',(86.0120724941042,-13.7497476751854,
66.1572462196087));
#143474=CARTESIAN_POINT('Ctrl Pts',(86.0111834231525,-13.7111723372268,
66.152053375483));
#143475=CARTESIAN_POINT('Ctrl Pts',(86.0106990615863,-13.6724238593391,
66.1490866930459));
#143476=CARTESIAN_POINT('Ctrl Pts',(86.0103773263657,-13.6466853388875,
66.1471160861796));
#143477=CARTESIAN_POINT('Ctrl Pts',(86.0102340649736,-13.6208711820731,
66.1461271215101));
#143478=CARTESIAN_POINT('Ctrl Pts',(86.0102709048271,-13.5950714516843,
66.1461211485216));
#143479=CARTESIAN_POINT('Origin',(68.9005579452291,-13.59506522122,70.178478144643));
#143480=CARTESIAN_POINT('',(69.2684768035491,-13.5950670495485,69.0981773024547));
#143481=CARTESIAN_POINT('',(69.2686191785991,-13.59506704669,69.098152274888));
#143482=CARTESIAN_POINT('Origin',(69.4419826548991,-13.59506522122,70.083010360306));
#143483=CARTESIAN_POINT('Ctrl Pts',(69.3960064164891,-14.36360211489,70.934760808954));
#143484=CARTESIAN_POINT('Ctrl Pts',(69.3948941469191,-14.36432617912,70.932322575951));
#143485=CARTESIAN_POINT('Ctrl Pts',(69.381319711449,-14.37348187874,70.9013962234701));
#143486=CARTESIAN_POINT('Ctrl Pts',(69.365369560429,-14.39219596977,70.83622702643));
#143487=CARTESIAN_POINT('Ctrl Pts',(69.3732349764891,-14.41738726414,70.7437279326));
#143488=CARTESIAN_POINT('Ctrl Pts',(69.4081799305892,-14.43748604032,70.665615251245));
#143489=CARTESIAN_POINT('Ctrl Pts',(69.4631712916492,-14.45027727949,70.610789156178));
#143490=CARTESIAN_POINT('Ctrl Pts',(69.5265616814791,-14.45439606951,70.5852234897169));
#143491=CARTESIAN_POINT('Ctrl Pts',(69.5705096728792,-14.45215669278,70.585314755206));
#143492=CARTESIAN_POINT('Ctrl Pts',(69.5901759596291,-14.45019796276,70.5887204004031));
#143493=CARTESIAN_POINT('Ctrl Pts',(68.4737857702591,-14.59510829149,71.468546571735));
#143494=CARTESIAN_POINT('Ctrl Pts',(68.4681080885491,-14.59879574582,71.456943752246));
#143495=CARTESIAN_POINT('Ctrl Pts',(68.398951202899,-14.64525476894,71.309844593959));
#143496=CARTESIAN_POINT('Ctrl Pts',(68.3208252767391,-14.73575279283,71.000643124038));
#143497=CARTESIAN_POINT('Ctrl Pts',(68.3692877416891,-14.85190586561,70.541515055448));
#143498=CARTESIAN_POINT('Ctrl Pts',(68.5773966848091,-14.94278494479,70.12318452394));
#143499=CARTESIAN_POINT('Ctrl Pts',(68.9244124274791,-15.00011120262,69.805528015821));
#143500=CARTESIAN_POINT('Ctrl Pts',(69.3392401939591,-15.01849094173,69.647259299348));
#143501=CARTESIAN_POINT('Ctrl Pts',(69.6249372840391,-15.00849600097,69.643102053229));
#143502=CARTESIAN_POINT('Ctrl Pts',(69.7505968801491,-14.99973699477,69.6606970664251));
#143503=CARTESIAN_POINT('Ctrl Pts',(67.8246108602491,-13.72054945886,71.520893278361));
#143504=CARTESIAN_POINT('Ctrl Pts',(67.8160399692091,-13.72604884949,71.503718416127));
#143505=CARTESIAN_POINT('Ctrl Pts',(67.7116892300791,-13.79531380705,71.2859739195089));
#143506=CARTESIAN_POINT('Ctrl Pts',(67.5949376413891,-13.92962281055,70.828058226473));
#143507=CARTESIAN_POINT('Ctrl Pts',(67.6719744253092,-14.10119003487,70.144322017472));
#143508=CARTESIAN_POINT('Ctrl Pts',(67.9941451974891,-14.23515457677,69.5162707493999));
#143509=CARTESIAN_POINT('Ctrl Pts',(68.5315781770691,-14.31958028328,69.035370936371));
#143510=CARTESIAN_POINT('Ctrl Pts',(69.1744797319091,-14.34663621025,68.793437652579));
#143511=CARTESIAN_POINT('Ctrl Pts',(69.6165656972991,-14.33192284069,68.785276381127));
#143512=CARTESIAN_POINT('Ctrl Pts',(69.8106988187391,-14.31902626561,68.810980738384));
#143513=CARTESIAN_POINT('Ctrl Pts',(68.283664590389,-12.8650716666,71.0244553278579));
#143514=CARTESIAN_POINT('Ctrl Pts',(68.2775948930291,-12.8689004296,71.0124695659739));
#143515=CARTESIAN_POINT('Ctrl Pts',(68.203716840389,-12.91713341696,70.8604945354981));
#143516=CARTESIAN_POINT('Ctrl Pts',(68.121582769839,-13.01091631349,70.5405079572659));
#143517=CARTESIAN_POINT('Ctrl Pts',(68.178409428339,-13.13105810204,70.063149520895));
#143518=CARTESIAN_POINT('Ctrl Pts',(68.4087959210191,-13.22498253222,69.6256866190019));
#143519=CARTESIAN_POINT('Ctrl Pts',(68.7900615322991,-13.28420786759,69.291147994876));
#143520=CARTESIAN_POINT('Ctrl Pts',(69.2442495489591,-13.30319304647,69.122225590261));
#143521=CARTESIAN_POINT('Ctrl Pts',(69.5561652089491,-13.29286878287,69.115456077889));
#143522=CARTESIAN_POINT('Ctrl Pts',(69.6931588369591,-13.28382045211,69.132756842017));
#143523=CARTESIAN_POINT('',(68.0516610740254,-13.4647404820174,70.8358748491249));
#143524=CARTESIAN_POINT('Ctrl Pts',(68.0516610740254,-13.4647404820174,
70.835874849125));
#143525=CARTESIAN_POINT('Ctrl Pts',(68.0421205335876,-13.46988128998,70.7818800903522));
#143526=CARTESIAN_POINT('Ctrl Pts',(68.0356143114983,-13.4748971670155,
70.7278391604887));
#143527=CARTESIAN_POINT('Ctrl Pts',(68.0320569230294,-13.4797508904263,
70.6741055266695));
#143528=CARTESIAN_POINT('Ctrl Pts',(68.028342778009,-13.484818493471,70.6180041168247));
#143529=CARTESIAN_POINT('Ctrl Pts',(68.02784208004,-13.4897095996712,70.5622381436379));
#143530=CARTESIAN_POINT('Ctrl Pts',(68.0303533192616,-13.4944247707082,
70.5071605870412));
#143531=CARTESIAN_POINT('Ctrl Pts',(68.0329792081805,-13.4993552111341,
70.4495684849789));
#143532=CARTESIAN_POINT('Ctrl Pts',(68.0388979933081,-13.5040932318593,
70.3927295676384));
#143533=CARTESIAN_POINT('Ctrl Pts',(68.0478686063493,-13.5086485211404,
70.3369881668536));
#143534=CARTESIAN_POINT('Ctrl Pts',(68.0568392193905,-13.5132038104215,
70.2812467660689));
#143535=CARTESIAN_POINT('Ctrl Pts',(68.0688612106036,-13.5175763912568,
70.2266027815759));
#143536=CARTESIAN_POINT('Ctrl Pts',(68.0836892332499,-13.5217849262162,
70.1733404031047));
#143537=CARTESIAN_POINT('Ctrl Pts',(68.0876485063194,-13.5229086592671,
70.1591186618967));
#143538=CARTESIAN_POINT('Ctrl Pts',(68.0918074778127,-13.5240202220121,
70.1449963682538));
#143539=CARTESIAN_POINT('Ctrl Pts',(68.0961615044139,-13.5251191716146,
70.130977824729));
#143540=CARTESIAN_POINT('Ctrl Pts',(68.1118919831629,-13.5290895202027,
70.0803308211147));
#143541=CARTESIAN_POINT('Ctrl Pts',(68.1301665305715,-13.532894769871,70.0310417949526));
#143542=CARTESIAN_POINT('Ctrl Pts',(68.1506864552881,-13.5365283692355,
69.9833257802005));
#143543=CARTESIAN_POINT('Ctrl Pts',(68.1715708548488,-13.5402265085816,
69.9347622337311));
#143544=CARTESIAN_POINT('Ctrl Pts',(68.1947809799418,-13.5437468823172,
69.8878278111564));
#143545=CARTESIAN_POINT('Ctrl Pts',(68.220028013724,-13.5470886456198,69.8427012760628));
#143546=CARTESIAN_POINT('Ctrl Pts',(68.2460472991032,-13.5505326261599,
69.796194418865));
#143547=CARTESIAN_POINT('Ctrl Pts',(68.2742298660689,-13.5537869291663,
69.7516075202316));
#143548=CARTESIAN_POINT('Ctrl Pts',(68.304289181768,-13.5568565394829,69.7090893843644));
#143549=CARTESIAN_POINT('Ctrl Pts',(68.3191133708432,-13.5583703624912,
69.688120946775));
#143550=CARTESIAN_POINT('Ctrl Pts',(68.3343944672205,-13.5598393527349,
69.6676549694699));
#143551=CARTESIAN_POINT('Ctrl Pts',(68.3501007657274,-13.5612645825095,
69.6477055627966));
#143552=CARTESIAN_POINT('Ctrl Pts',(68.35475770232,-13.5616871648695,69.6417905394767));
#143553=CARTESIAN_POINT('Ctrl Pts',(68.3594520305785,-13.5621059021736,
69.6359209138541));
#143554=CARTESIAN_POINT('Ctrl Pts',(68.364182573376,-13.5625208751211,69.6300969152317));
#143555=CARTESIAN_POINT('Ctrl Pts',(68.3968043587475,-13.5653825252549,
69.5899346672198));
#143556=CARTESIAN_POINT('Ctrl Pts',(68.4311388118727,-13.5680575385359,
69.5519512465469));
#143557=CARTESIAN_POINT('Ctrl Pts',(68.4668297458609,-13.5705432646287,
69.5161993167051));
#143558=CARTESIAN_POINT('Ctrl Pts',(68.5034294369521,-13.5730922818991,
69.4795370766932));
#143559=CARTESIAN_POINT('Ctrl Pts',(68.5414557353341,-13.5754422829169,
69.4452211726811));
#143560=CARTESIAN_POINT('Ctrl Pts',(68.5805740405099,-13.5775926222074,
69.4132822919613));
#143561=CARTESIAN_POINT('Ctrl Pts',(68.6212598754391,-13.5798291288511,
69.3800635719029));
#143562=CARTESIAN_POINT('Ctrl Pts',(68.66312708886,-13.5818496788251,69.3494160245309));
#143563=CARTESIAN_POINT('Ctrl Pts',(68.7058501301954,-13.5836554461766,
69.3213494005411));
#143564=CARTESIAN_POINT('Ctrl Pts',(68.723546776751,-13.5844034272561,69.3097237037455));
#143565=CARTESIAN_POINT('Ctrl Pts',(68.7413908401205,-13.5851145762207,
69.2985405620008));
#143566=CARTESIAN_POINT('Ctrl Pts',(68.7593615209816,-13.5857890505673,
69.2877995937322));
#143567=CARTESIAN_POINT('Ctrl Pts',(68.7699968921183,-13.5861882165785,
69.281442896132));
#143568=CARTESIAN_POINT('Ctrl Pts',(68.7806766317356,-13.5865745387272,
69.2752410529925));
#143569=CARTESIAN_POINT('Ctrl Pts',(68.7913955230437,-13.5869482277688,
69.2691925544764));
#143570=CARTESIAN_POINT('Ctrl Pts',(68.8361426982761,-13.5885082332348,
69.2439424408949));
#143571=CARTESIAN_POINT('Ctrl Pts',(68.8815567060986,-13.5898425649172,
69.2213712387007));
#143572=CARTESIAN_POINT('Ctrl Pts',(68.9272883543862,-13.5909523521958,
69.2013656174685));
#143573=CARTESIAN_POINT('Ctrl Pts',(68.9742558909504,-13.5920921312446,
69.1808193484865));
#143574=CARTESIAN_POINT('Ctrl Pts',(69.0215587529483,-13.5929950826377,
69.1629791935471));
#143575=CARTESIAN_POINT('Ctrl Pts',(69.0688746875484,-13.593661482091,69.1477194858201));
#143576=CARTESIAN_POINT('Ctrl Pts',(69.1180508388671,-13.5943540809085,
69.1318598456671));
#143577=CARTESIAN_POINT('Ctrl Pts',(69.1672412886183,-13.5947911796269,
69.1187875750068));
#143578=CARTESIAN_POINT('Ctrl Pts',(69.216140495377,-13.594971802996,69.1083583062007));
#143579=CARTESIAN_POINT('Ctrl Pts',(69.2336267898101,-13.5950363936842,
69.1046288128786));
#143580=CARTESIAN_POINT('Ctrl Pts',(69.2510763346266,-13.595068174289,69.1012372658518));
#143581=CARTESIAN_POINT('Ctrl Pts',(69.2684767416407,-13.5950670565703,
69.0981769504524));
#143582=CARTESIAN_POINT('Origin',(69.0364672392459,-13.4647383323567,70.6622289425537));
#143583=CARTESIAN_POINT('Origin',(68.3580209600691,0.499074165591714,66.814943349163));
#143584=CARTESIAN_POINT('',(68.8731212986265,-11.1474493393501,75.4949909016172));
#143585=CARTESIAN_POINT('Origin',(67.3732132070591,0.499074165591714,66.988591526828));
#143586=CARTESIAN_POINT('Origin',(69.8579284813091,-11.14744746673,75.321341605509));
#143587=CARTESIAN_POINT('Ctrl Pts',(70.5727142903791,-11.62540260925,76.212415349127));
#143588=CARTESIAN_POINT('Ctrl Pts',(70.5474025662891,-11.62160041199,76.221790216259));
#143589=CARTESIAN_POINT('Ctrl Pts',(70.4849770218291,-11.61987597393,76.2350078033179));
#143590=CARTESIAN_POINT('Ctrl Pts',(70.3779197843791,-11.64555877,76.220765968497));
#143591=CARTESIAN_POINT('Ctrl Pts',(70.2560676070191,-11.71486549074,76.152463833801));
#143592=CARTESIAN_POINT('Ctrl Pts',(70.1558432364391,-11.81914313621,76.032792395521));
#143593=CARTESIAN_POINT('Ctrl Pts',(70.1050930198391,-11.92846628364,75.894132175066));
#143594=CARTESIAN_POINT('Ctrl Pts',(70.0998645202791,-11.99631186027,75.801284231172));
#143595=CARTESIAN_POINT('Ctrl Pts',(70.1022592401991,-12.02298947846,75.763694284642));
#143596=CARTESIAN_POINT('Ctrl Pts',(70.8569680292191,-11.22017028,76.869673584669));
#143597=CARTESIAN_POINT('Ctrl Pts',(70.7478285345391,-11.20473814975,76.9076141171011));
#143598=CARTESIAN_POINT('Ctrl Pts',(70.4658852850292,-11.19636485193,76.967431120053));
#143599=CARTESIAN_POINT('Ctrl Pts',(70.0286683689591,-11.30538170868,76.912662413182));
#143600=CARTESIAN_POINT('Ctrl Pts',(69.6654256755191,-11.51820751993,76.714360538357));
#143601=CARTESIAN_POINT('Ctrl Pts',(69.4246643242891,-11.77129992332,76.433832422159));
#143602=CARTESIAN_POINT('Ctrl Pts',(69.3125109709092,-12.01186619021,76.132469357613));
#143603=CARTESIAN_POINT('Ctrl Pts',(69.3008812463991,-12.16248052272,75.924831943563));
#143604=CARTESIAN_POINT('Ctrl Pts',(69.3072602647691,-12.22316470436,75.8378355297749));
#143605=CARTESIAN_POINT('Ctrl Pts',(70.9671564453892,-10.40460940052,76.8651302226241));
#143606=CARTESIAN_POINT('Ctrl Pts',(70.8026967635191,-10.38178139262,76.921572843059));
#143607=CARTESIAN_POINT('Ctrl Pts',(70.3760114274691,-10.36915940562,77.0119477511941));
#143608=CARTESIAN_POINT('Ctrl Pts',(69.7215419928391,-10.53124236333,76.9327305518971));
#143609=CARTESIAN_POINT('Ctrl Pts',(69.2001137835892,-10.83431808305,76.65410085986));
#143610=CARTESIAN_POINT('Ctrl Pts',(68.8680419533291,-11.17951523624,76.2751089113451));
#143611=CARTESIAN_POINT('Ctrl Pts',(68.7168083006591,-11.50052073533,75.874419214426));
#143612=CARTESIAN_POINT('Ctrl Pts',(68.7018554092492,-11.70191427611,75.5961943394401));
#143613=CARTESIAN_POINT('Ctrl Pts',(68.7112204234791,-11.78351622729,75.478665827774));
#143614=CARTESIAN_POINT('Ctrl Pts',(70.7997299180591,-9.94514372726199,
76.203054889814));
#143615=CARTESIAN_POINT('Ctrl Pts',(70.6604448068091,-9.92610417687498,
76.250548674226));
#143616=CARTESIAN_POINT('Ctrl Pts',(70.2998144530591,-9.91562637911499,
76.326723169705));
#143617=CARTESIAN_POINT('Ctrl Pts',(69.7451628261291,-10.05063858235,76.26211134095));
#143618=CARTESIAN_POINT('Ctrl Pts',(69.2974090212691,-10.30588263055,76.028313862207));
#143619=CARTESIAN_POINT('Ctrl Pts',(69.0090622832791,-10.59991903937,75.705782364097));
#143620=CARTESIAN_POINT('Ctrl Pts',(68.8777969001991,-10.87496707353,75.362484500442));
#143621=CARTESIAN_POINT('Ctrl Pts',(68.8657218477491,-11.04743048786,75.124208776502));
#143622=CARTESIAN_POINT('Ctrl Pts',(68.8742684640891,-11.11720392997,75.023715091041));
#143623=CARTESIAN_POINT('Ctrl Pts',(70.6107884237591,-10.75942680297,76.71163854688));
#143624=CARTESIAN_POINT('Ctrl Pts',(70.4329281245592,-10.7588937036665,
76.7430935490508));
#143625=CARTESIAN_POINT('Ctrl Pts',(70.2423398126716,-10.768156222049,76.7431479729786));
#143626=CARTESIAN_POINT('Ctrl Pts',(69.9571737741532,-10.7967434261519,
76.6853219130463));
#143627=CARTESIAN_POINT('Ctrl Pts',(69.8623280976091,-10.8087213986076,
76.6564591267567));
#143628=CARTESIAN_POINT('Ctrl Pts',(69.7235605112814,-10.8303617139236,
76.5982160113568));
#143629=CARTESIAN_POINT('Ctrl Pts',(69.677892530448,-10.8381873784676,76.5763169357272));
#143630=CARTESIAN_POINT('Ctrl Pts',(69.6107045260779,-10.8508442144416,
76.5397381599502));
#143631=CARTESIAN_POINT('Ctrl Pts',(69.5774393211989,-10.8574022172182,
76.5205169934371));
#143632=CARTESIAN_POINT('Ctrl Pts',(69.5393026779042,-10.8654549938392,
76.4964694047508));
#143633=CARTESIAN_POINT('Ctrl Pts',(69.5204148930439,-10.8695818254951,
76.4840415082369));
#143634=CARTESIAN_POINT('Ctrl Pts',(69.5123601399464,-10.8713719912073,
76.4786288640684));
#143635=CARTESIAN_POINT('Ctrl Pts',(69.5069993437469,-10.872570218032,76.4750012569881));
#143636=CARTESIAN_POINT('Ctrl Pts',(69.5033202961855,-10.8733985090141,
76.4724895148948));
#143637=CARTESIAN_POINT('Ctrl Pts',(69.3948927597608,-10.8979106828788,
76.398089236559));
#143638=CARTESIAN_POINT('Ctrl Pts',(69.2671450458483,-10.9327842016567,
76.2910185912873));
#143639=CARTESIAN_POINT('Ctrl Pts',(69.0294099549965,-11.0240081109645,
75.972523756007));
#143640=CARTESIAN_POINT('Ctrl Pts',(68.9196520979315,-11.080358483221,75.7588815978788));
#143641=CARTESIAN_POINT('Ctrl Pts',(68.8731215714991,-11.1474472924843,
75.4949903331303));
#143642=CARTESIAN_POINT('Ctrl Pts',(70.5465863094391,-11.53587577121,76.347528984853));
#143643=CARTESIAN_POINT('Ctrl Pts',(70.5665960457121,-11.4425022179353,
76.4608199972518));
#143644=CARTESIAN_POINT('Ctrl Pts',(70.5828633060719,-11.3232077539368,
76.5532835146138));
#143645=CARTESIAN_POINT('Ctrl Pts',(70.604920056824,-11.0556680213945,76.6787881629939));
#143646=CARTESIAN_POINT('Ctrl Pts',(70.6106952853454,-10.9075952019447,
76.7117484109232));
#143647=CARTESIAN_POINT('Ctrl Pts',(70.6107884237367,-10.759426838634,76.7116385469064));
#143648=CARTESIAN_POINT('Origin',(93.9117403164691,-10.75942675157,71.587718899901));
#143649=CARTESIAN_POINT('Ctrl Pts',(79.7232095658691,-10.75961935955,75.104974613695));
#143650=CARTESIAN_POINT('Ctrl Pts',(79.8754552241483,-10.8828544446583,
75.0780971616129));
#143651=CARTESIAN_POINT('Ctrl Pts',(80.0491425096114,-11.019491411425,75.0240272782727));
#143652=CARTESIAN_POINT('Ctrl Pts',(80.4350484926432,-11.2915328846245,
74.8368221251738));
#143653=CARTESIAN_POINT('Ctrl Pts',(80.6471382934547,-11.4268302101939,
74.7029558455787));
#143654=CARTESIAN_POINT('Ctrl Pts',(80.8778403488691,-11.53587675694,74.525850965447));
#143655=CARTESIAN_POINT('Ctrl Pts',(79.3965414347691,-10.75937454605,75.186662823148));
#143656=CARTESIAN_POINT('Ctrl Pts',(79.3992528435091,-10.7645545324,75.1866956812119));
#143657=CARTESIAN_POINT('Ctrl Pts',(79.4725942355591,-10.90537889734,75.186841976488));
#143658=CARTESIAN_POINT('Ctrl Pts',(79.6130654149191,-11.21423607471,75.144851871569));
#143659=CARTESIAN_POINT('Ctrl Pts',(79.8139675630191,-11.69507199961,74.9338518091059));
#143660=CARTESIAN_POINT('Ctrl Pts',(79.9721744722591,-12.03339183741,74.641026175075));
#143661=CARTESIAN_POINT('Ctrl Pts',(80.0647903183391,-12.1995563218,74.42412393955));
#143662=CARTESIAN_POINT('Ctrl Pts',(80.0853956808191,-12.23499347946,74.373394440298));
#143663=CARTESIAN_POINT('Ctrl Pts',(79.7916100122891,-10.5653046013,75.021875684663));
#143664=CARTESIAN_POINT('Ctrl Pts',(79.7941034949391,-10.57001050956,75.021940607005));
#143665=CARTESIAN_POINT('Ctrl Pts',(79.8614679630191,-10.6979216525,75.022938558934));
#143666=CARTESIAN_POINT('Ctrl Pts',(79.9858550612891,-10.97673091235,74.981925321278));
#143667=CARTESIAN_POINT('Ctrl Pts',(80.1528636967791,-11.40236933979,74.784369362516));
#143668=CARTESIAN_POINT('Ctrl Pts',(80.278150309989,-11.69585236607,74.521057735256));
#143669=CARTESIAN_POINT('Ctrl Pts',(80.3509919691591,-11.83827309688,74.3307566055));
#143670=CARTESIAN_POINT('Ctrl Pts',(80.3672219688891,-11.86855566293,74.286462610011));
#143671=CARTESIAN_POINT('Ctrl Pts',(80.2102524607391,-10.35643022745,75.066664900866));
#143672=CARTESIAN_POINT('Ctrl Pts',(80.2128494848392,-10.36134940962,75.066774703059));
#143673=CARTESIAN_POINT('Ctrl Pts',(80.2829816961191,-10.49495458286,75.0688538343589));
#143674=CARTESIAN_POINT('Ctrl Pts',(80.4106556196692,-10.77987219022,75.0227015441689));
#143675=CARTESIAN_POINT('Ctrl Pts',(80.5737969977991,-11.19462437857,74.8135437512119));
#143676=CARTESIAN_POINT('Ctrl Pts',(80.6877425938991,-11.46754862033,74.5509908140901));
#143677=CARTESIAN_POINT('Ctrl Pts',(80.7524414512091,-11.59633911287,74.368633104737));
#143678=CARTESIAN_POINT('Ctrl Pts',(80.7668633987791,-11.6235324656,74.326529759673));
#143679=CARTESIAN_POINT('Ctrl Pts',(80.5677595186891,-10.17501563828,75.311967698886));
#143680=CARTESIAN_POINT('Ctrl Pts',(80.570760600919,-10.18079229193,75.312126115391));
#143681=CARTESIAN_POINT('Ctrl Pts',(80.6518451898191,-10.33754660207,75.31529717998));
#143682=CARTESIAN_POINT('Ctrl Pts',(80.8015117797791,-10.66349284216,75.258929767445));
#143683=CARTESIAN_POINT('Ctrl Pts',(80.9915946672691,-11.11387280127,75.015471749357));
#143684=CARTESIAN_POINT('Ctrl Pts',(81.1180732976791,-11.39467620639,74.724768670296));
#143685=CARTESIAN_POINT('Ctrl Pts',(81.1879083750491,-11.52270795576,74.530089402506));
#143686=CARTESIAN_POINT('Ctrl Pts',(81.2034554272791,-11.54950255337,74.48548859231));
#143687=CARTESIAN_POINT('Origin',(70.3503323584791,15.19124921296,75.234517520424));
#143688=CARTESIAN_POINT('',(68.8731215366466,11.1474497637427,75.4949903427175));
#143689=CARTESIAN_POINT('',(68.8731214546391,11.14744746373,75.494989659206));
#143690=CARTESIAN_POINT('Ctrl Pts',(68.873121472862,11.1474474374557,75.494989762555));
#143691=CARTESIAN_POINT('Ctrl Pts',(68.9196357623451,11.0803819298226,75.7587895431469));
#143692=CARTESIAN_POINT('Ctrl Pts',(69.0293411064219,11.0240431945441,75.9724005246367));
#143693=CARTESIAN_POINT('Ctrl Pts',(69.2076201138475,10.9556252471803,76.2112882368804));
#143694=CARTESIAN_POINT('Ctrl Pts',(69.2696540133536,10.9355009565293,76.2780069134329));
#143695=CARTESIAN_POINT('Ctrl Pts',(69.3598779034547,10.9093370612364,76.3617636879751));
#143696=CARTESIAN_POINT('Ctrl Pts',(69.3895069124018,10.9012861862527,76.386976797235));
#143697=CARTESIAN_POINT('Ctrl Pts',(69.432655939315,10.890215508948,76.4211964872657));
#143698=CARTESIAN_POINT('Ctrl Pts',(69.4539089655518,10.8849315790885,76.4374067439443));
#143699=CARTESIAN_POINT('Ctrl Pts',(69.4780260298471,10.8792069596395,76.4548468328527));
#143700=CARTESIAN_POINT('Ctrl Pts',(69.4899020813184,10.8764546412619,76.46321167396));
#143701=CARTESIAN_POINT('Ctrl Pts',(69.4949513584603,10.8752986458172,76.4667218509199));
#143702=CARTESIAN_POINT('Ctrl Pts',(69.4983084054692,10.8745332198706,76.4690455074634));
#143703=CARTESIAN_POINT('Ctrl Pts',(69.498981060932,10.8743795455877,76.4695120379923));
#143704=CARTESIAN_POINT('Ctrl Pts',(69.6725708456909,10.8351263615574,76.58862513492));
#143705=CARTESIAN_POINT('Ctrl Pts',(69.8620431857368,10.8062726507668,76.6660209055238));
#143706=CARTESIAN_POINT('Ctrl Pts',(70.2422605680285,10.768156393542,76.7431422960647));
#143707=CARTESIAN_POINT('Ctrl Pts',(70.4328762301428,10.7588938387249,76.7431026435897));
#143708=CARTESIAN_POINT('Ctrl Pts',(70.6107879836103,10.7594268536258,76.7116386626372));
#143709=CARTESIAN_POINT('Ctrl Pts',(70.102712361999,12.02753207592,75.757282539526));
#143710=CARTESIAN_POINT('Ctrl Pts',(70.0996331790591,11.99950461932,75.796911436068));
#143711=CARTESIAN_POINT('Ctrl Pts',(70.1043339346791,11.93010065,75.892059102544));
#143712=CARTESIAN_POINT('Ctrl Pts',(70.1558442152191,11.81914181107,76.032794052158));
#143713=CARTESIAN_POINT('Ctrl Pts',(70.256068577559,11.71486478129,76.152464588268));
#143714=CARTESIAN_POINT('Ctrl Pts',(70.3779204807191,11.64555844469,76.220766236192));
#143715=CARTESIAN_POINT('Ctrl Pts',(70.4854323625891,11.61976697429,76.235068208024));
#143716=CARTESIAN_POINT('Ctrl Pts',(70.5482524904191,11.62162458361,76.221609172899));
#143717=CARTESIAN_POINT('Ctrl Pts',(70.5739515098291,11.62559101398,76.211953819954));
#143718=CARTESIAN_POINT('Ctrl Pts',(69.3084586152291,12.23351299725,75.822967076824));
#143719=CARTESIAN_POINT('Ctrl Pts',(69.3003664827991,12.16956777349,75.915049294702));
#143720=CARTESIAN_POINT('Ctrl Pts',(69.3108335232591,12.01546339144,76.127964138853));
#143721=CARTESIAN_POINT('Ctrl Pts',(69.4246666664091,11.77129665272,76.433835944702));
#143722=CARTESIAN_POINT('Ctrl Pts',(69.6654281435891,11.51820560131,76.714362465994));
#143723=CARTESIAN_POINT('Ctrl Pts',(70.0286715861291,11.30538064205,76.912663256773));
#143724=CARTESIAN_POINT('Ctrl Pts',(70.4677430073291,11.19590164666,76.96766322359));
#143725=CARTESIAN_POINT('Ctrl Pts',(70.7516719479191,11.20485608161,76.906794945282));
#143726=CARTESIAN_POINT('Ctrl Pts',(70.8623006925891,11.22093455699,76.867807281098));
#143727=CARTESIAN_POINT('Ctrl Pts',(68.7129713268991,11.79743625123,75.458569937586));
#143728=CARTESIAN_POINT('Ctrl Pts',(68.7011960208591,11.71139085457,75.583084770824));
#143729=CARTESIAN_POINT('Ctrl Pts',(68.7145463530291,11.50532104132,75.868429277325));
#143730=CARTESIAN_POINT('Ctrl Pts',(68.8680451809691,11.17951080797,76.275113604241));
#143731=CARTESIAN_POINT('Ctrl Pts',(69.2001172342691,10.83431545673,76.654103547953));
#143732=CARTESIAN_POINT('Ctrl Pts',(69.7215468729191,10.53124087494,76.93273179034));
#143733=CARTESIAN_POINT('Ctrl Pts',(70.3787919557391,10.36847068451,77.012283454108));
#143734=CARTESIAN_POINT('Ctrl Pts',(70.8085139955891,10.38195929028,76.920335313241));
#143735=CARTESIAN_POINT('Ctrl Pts',(70.9751918492591,10.40573993406,76.8623542019151));
#143736=CARTESIAN_POINT('Ctrl Pts',(68.8758599429291,11.12910515526,75.006533496628));
#143737=CARTESIAN_POINT('Ctrl Pts',(68.8651925032291,11.05554582734,75.112981674439));
#143738=CARTESIAN_POINT('Ctrl Pts',(68.8758335592991,10.87908010167,75.35735252033));
#143739=CARTESIAN_POINT('Ctrl Pts',(69.0090650491591,10.59991528949,75.705786421317));
#143740=CARTESIAN_POINT('Ctrl Pts',(69.2974119850591,10.30588041722,76.028316179364));
#143741=CARTESIAN_POINT('Ctrl Pts',(69.7451669278891,10.05063733625,76.262112423484));
#143742=CARTESIAN_POINT('Ctrl Pts',(70.3021709983891,9.91505270512101,76.326997017962));
#143743=CARTESIAN_POINT('Ctrl Pts',(70.6653612936691,9.92625183784202,76.24950570992));
#143744=CARTESIAN_POINT('Ctrl Pts',(70.8065354647891,9.94608665721,76.20071911601));
#143745=CARTESIAN_POINT('Origin',(70.4377543611373,10.7600784829335,75.7271941746767));
#143746=CARTESIAN_POINT('Origin',(69.8579298464391,11.14744710765,75.321341757772));
#143747=CARTESIAN_POINT('Origin',(68.3580209600691,-0.499074165591386,66.814943349163));
#143748=CARTESIAN_POINT('',(68.0516611136485,13.4647404820328,70.8358748421131));
#143749=CARTESIAN_POINT('Origin',(67.3732132070591,-0.499074165591386,66.988591526828));
#143750=CARTESIAN_POINT('Origin',(69.0364886624041,13.4646700573952,70.6621973310861));
#143751=CARTESIAN_POINT('Ctrl Pts',(69.5909480384691,14.4501205633,70.5888558711801));
#143752=CARTESIAN_POINT('Ctrl Pts',(69.5710297789591,14.45212989413,70.5853163357091));
#143753=CARTESIAN_POINT('Ctrl Pts',(69.526803187669,14.45441189054,70.5851259273609));
#143754=CARTESIAN_POINT('Ctrl Pts',(69.463170177939,14.45027710795,70.610789854498));
#143755=CARTESIAN_POINT('Ctrl Pts',(69.408179216219,14.43748579055,70.665616301966));
#143756=CARTESIAN_POINT('Ctrl Pts',(69.3732345852692,14.41738679729,70.7437295812081));
#143757=CARTESIAN_POINT('Ctrl Pts',(69.3653696994291,14.39219576725,70.836228061593));
#143758=CARTESIAN_POINT('Ctrl Pts',(69.3811532223691,14.37367712896,70.900715547079));
#143759=CARTESIAN_POINT('Ctrl Pts',(69.3943519653192,14.36469356993,70.931081264837));
#143760=CARTESIAN_POINT('Ctrl Pts',(69.3951714436091,14.36415051983,70.9329126925041));
#143761=CARTESIAN_POINT('Ctrl Pts',(69.7555290321091,14.99939089597,69.6613979532501));
#143762=CARTESIAN_POINT('Ctrl Pts',(69.6283184250891,15.0083774287,69.643055967434));
#143763=CARTESIAN_POINT('Ctrl Pts',(69.3408205475991,15.0185610031,69.646655229886));
#143764=CARTESIAN_POINT('Ctrl Pts',(68.9244052019191,15.00011063687,69.805532218907));
#143765=CARTESIAN_POINT('Ctrl Pts',(68.5773922830591,14.94278376454,70.12319038474));
#143766=CARTESIAN_POINT('Ctrl Pts',(68.3692854484991,14.85190392646,70.541523557376));
#143767=CARTESIAN_POINT('Ctrl Pts',(68.3208257724191,14.73575126236,71.000647874436));
#143768=CARTESIAN_POINT('Ctrl Pts',(68.3981360480691,14.64620032309,71.306615498519));
#143769=CARTESIAN_POINT('Ctrl Pts',(68.4653464484391,14.60065890237,71.45103966638));
#143770=CARTESIAN_POINT('Ctrl Pts',(68.4695255391492,14.59789853672,71.459752952336));
#143771=CARTESIAN_POINT('Ctrl Pts',(69.8183183999891,14.31851666367,68.8120051244791));
#143772=CARTESIAN_POINT('Ctrl Pts',(69.6217976430991,14.33174843893,68.785184513493));
#143773=CARTESIAN_POINT('Ctrl Pts',(69.1769289671191,14.34673924446,68.7925142553861));
#143774=CARTESIAN_POINT('Ctrl Pts',(68.5315669763691,14.319579466,69.035377325048));
#143775=CARTESIAN_POINT('Ctrl Pts',(67.9941383798391,14.23515281344,69.516279580646));
#143776=CARTESIAN_POINT('Ctrl Pts',(67.6719708568691,14.10118718706,70.144334725471));
#143777=CARTESIAN_POINT('Ctrl Pts',(67.5949383401392,13.92962044387,70.828065237159));
#143778=CARTESIAN_POINT('Ctrl Pts',(67.7104711173591,13.79671729307,71.2811918084051));
#143779=CARTESIAN_POINT('Ctrl Pts',(67.8118731588091,13.7288264298,71.494978799744));
#143780=CARTESIAN_POINT('Ctrl Pts',(67.8181804147791,13.7247103957,71.507876616965));
#143781=CARTESIAN_POINT('Ctrl Pts',(69.6985357447892,13.28346290429,69.1334466308519));
#143782=CARTESIAN_POINT('Ctrl Pts',(69.559856613789,13.29274633139,69.1153792244139));
#143783=CARTESIAN_POINT('Ctrl Pts',(69.245979860049,13.30326537476,69.121580881155));
#143784=CARTESIAN_POINT('Ctrl Pts',(68.7900536127391,13.28420727445,69.291152448768));
#143785=CARTESIAN_POINT('Ctrl Pts',(68.4087910751191,13.2249812931,69.6256927678659));
#143786=CARTESIAN_POINT('Ctrl Pts',(68.178406861629,13.13105608861,70.0631583819599));
#143787=CARTESIAN_POINT('Ctrl Pts',(68.1215832668291,13.01091468929,70.5405128677461));
#143788=CARTESIAN_POINT('Ctrl Pts',(68.2028599044891,12.91811333149,70.8571528134859));
#143789=CARTESIAN_POINT('Ctrl Pts',(68.2746450030891,12.87083467023,71.0063696573741));
#143790=CARTESIAN_POINT('Ctrl Pts',(68.2791110289791,12.86796872275,71.015371154369));
#143791=CARTESIAN_POINT('',(69.2684762522038,13.5950670419766,69.0981773334213));
#143792=CARTESIAN_POINT('Ctrl Pts',(69.2684762020613,13.5950670489771,69.0981770483176));
#143793=CARTESIAN_POINT('Ctrl Pts',(69.220057547122,13.5950701709265,69.1066927282233));
#143794=CARTESIAN_POINT('Ctrl Pts',(69.1712548530349,13.5948186616202,69.117773390592));
#143795=CARTESIAN_POINT('Ctrl Pts',(69.122350723928,13.5943139780203,69.1315625395245));
#143796=CARTESIAN_POINT('Ctrl Pts',(69.0747459064741,13.5938227031304,69.1449853308053));
#143797=CARTESIAN_POINT('Ctrl Pts',(69.0270447253686,13.5930915155534,69.1609745635876));
#143798=CARTESIAN_POINT('Ctrl Pts',(68.9795563737709,13.5921205463393,69.1796595201576));
#143799=CARTESIAN_POINT('Ctrl Pts',(68.9339098572451,13.5911872361529,69.1976197809407));
#143800=CARTESIAN_POINT('Ctrl Pts',(68.8884598373705,13.590032367056,69.2180707031689));
#143801=CARTESIAN_POINT('Ctrl Pts',(68.843528998897,13.5886551324547,69.2411245525615));
#143802=CARTESIAN_POINT('Ctrl Pts',(68.8260648327327,13.5881198151817,69.2500853525421));
#143803=CARTESIAN_POINT('Ctrl Pts',(68.8086796450837,13.587550894111,69.2594393750054));
#143804=CARTESIAN_POINT('Ctrl Pts',(68.7913945439412,13.5869482908414,69.2691931008479));
#143805=CARTESIAN_POINT('Ctrl Pts',(68.7806744900466,13.586574562075,69.2752422680377));
#143806=CARTESIAN_POINT('Ctrl Pts',(68.7699935966165,13.5861881975767,69.2814448130544));
#143807=CARTESIAN_POINT('Ctrl Pts',(68.7593570820778,13.5857889863606,69.2878022461852));
#143808=CARTESIAN_POINT('Ctrl Pts',(68.7161705873195,13.5841681045361,69.3136147669676));
#143809=CARTESIAN_POINT('Ctrl Pts',(68.6737122633642,13.5823353232669,69.3419823375415));
#143810=CARTESIAN_POINT('Ctrl Pts',(68.6322838040265,13.5802888544023,69.372904327941));
#143811=CARTESIAN_POINT('Ctrl Pts',(68.5919679036079,13.5782973433426,69.4029959100473));
#143812=CARTESIAN_POINT('Ctrl Pts',(68.5526271061992,13.5761034412783,69.4355067406709));
#143813=CARTESIAN_POINT('Ctrl Pts',(68.5145832966752,13.5737070098349,69.4704155296987));
#143814=CARTESIAN_POINT('Ctrl Pts',(68.4779560546146,13.5713998099078,69.5040244842636));
#143815=CARTESIAN_POINT('Ctrl Pts',(68.4425309391481,13.5689048579052,69.5398563008427));
#143816=CARTESIAN_POINT('Ctrl Pts',(68.408638167092,13.5662238098117,69.5778701295916));
#143817=CARTESIAN_POINT('Ctrl Pts',(68.3935024629306,13.5650265176363,69.5948461994463));
#143818=CARTESIAN_POINT('Ctrl Pts',(68.3786729461382,13.5637921386554,69.6122571171597));
#143819=CARTESIAN_POINT('Ctrl Pts',(68.3641820136269,13.5625209630308,69.630097615198));
#143820=CARTESIAN_POINT('Ctrl Pts',(68.3594486557417,13.5621057427432,69.6359250843411));
#143821=CARTESIAN_POINT('Ctrl Pts',(68.3547515554537,13.561686753605,69.6417982348309));
#143822=CARTESIAN_POINT('Ctrl Pts',(68.3500918920114,13.5612639147922,69.6477168369388));
#143823=CARTESIAN_POINT('Ctrl Pts',(68.3183422079409,13.5583828056981,69.6880445879435));
#143824=CARTESIAN_POINT('Ctrl Pts',(68.2883282544299,13.5553225520827,69.7304857583872));
#143825=CARTESIAN_POINT('Ctrl Pts',(68.2603193199432,13.5520755798442,69.7749137039889));
#143826=CARTESIAN_POINT('Ctrl Pts',(68.2328820724945,13.5488948811708,69.8184348360651));
#143827=CARTESIAN_POINT('Ctrl Pts',(68.2073688978383,13.5455349757244,69.8638627496069));
#143828=CARTESIAN_POINT('Ctrl Pts',(68.1840604240437,13.5419938709497,69.9110378480984));
#143829=CARTESIAN_POINT('Ctrl Pts',(68.1613768188838,13.5385476984011,69.95694824605));
#143830=CARTESIAN_POINT('Ctrl Pts',(68.1407814228562,13.5349298863568,70.0045135978539));
#143831=CARTESIAN_POINT('Ctrl Pts',(68.1225576898816,13.5311439178348,70.0535446151893));
#143832=CARTESIAN_POINT('Ctrl Pts',(68.1131060521354,13.5291803463185,70.0789742796179));
#143833=CARTESIAN_POINT('Ctrl Pts',(68.1042927727855,13.5271716324888,70.104797479399));
#143834=CARTESIAN_POINT('Ctrl Pts',(68.0961599336273,13.5251188862045,70.1309828875299));
#143835=CARTESIAN_POINT('Ctrl Pts',(68.091806425645,13.5240200513253,70.1449999338651));
#143836=CARTESIAN_POINT('Ctrl Pts',(68.0876479307248,13.5229086059803,70.1591207069769));
#143837=CARTESIAN_POINT('Ctrl Pts',(68.0836890907593,13.5217849930833,70.1733409057962));
#143838=CARTESIAN_POINT('Ctrl Pts',(68.0693978664713,13.5177288038804,70.2246751482821));
#143839=CARTESIAN_POINT('Ctrl Pts',(68.057713180962,13.5135202722556,70.2772924424713));
#143840=CARTESIAN_POINT('Ctrl Pts',(68.0488547159004,13.5091425519104,70.3309393260326));
#143841=CARTESIAN_POINT('Ctrl Pts',(68.0396975073969,13.5046171970444,70.3863954005243));
#143842=CARTESIAN_POINT('Ctrl Pts',(68.033560798574,13.4999109806522,70.4429520930334));
#143843=CARTESIAN_POINT('Ctrl Pts',(68.0306832804395,13.4950139845556,70.5002711676494));
#143844=CARTESIAN_POINT('Ctrl Pts',(68.0278057623051,13.4901169884591,70.5575902422654));
#143845=CARTESIAN_POINT('Ctrl Pts',(68.028187870028,13.4850291992576,70.6156716572521));
#143846=CARTESIAN_POINT('Ctrl Pts',(68.0320577126148,13.4797498060016,70.6741175007522));
#143847=CARTESIAN_POINT('Ctrl Pts',(68.0356152869072,13.4748964215795,70.7278471875989));
#143848=CARTESIAN_POINT('Ctrl Pts',(68.0421212736795,13.469880918388,70.7818841101077));
#143849=CARTESIAN_POINT('Ctrl Pts',(68.0516611136484,13.4647404820328,70.8358748421131));
#143850=CARTESIAN_POINT('Origin',(69.4419825833591,13.59506528922,70.083010104271));
#143851=CARTESIAN_POINT('Origin',(86.5648503253491,13.59506522122,67.063786802906));
#143852=CARTESIAN_POINT('',(86.010255170479,13.5950708837,66.1461463384425));
#143853=CARTESIAN_POINT('',(86.0102549463391,13.5950708837,66.146145068228));
#143854=CARTESIAN_POINT('Origin',(86.1839250991447,13.5950984680028,67.1309524517065));
#143855=CARTESIAN_POINT('Ctrl Pts',(88.6593324780691,14.84336710374,63.884495094759));
#143856=CARTESIAN_POINT('Ctrl Pts',(88.6758192267691,14.84102992348,63.945364550575));
#143857=CARTESIAN_POINT('Ctrl Pts',(88.7703803079691,14.82406732012,64.343280741328));
#143858=CARTESIAN_POINT('Ctrl Pts',(88.7916617756691,14.77049785957,65.102043024085));
#143859=CARTESIAN_POINT('Ctrl Pts',(88.4834074127691,14.66322007682,66.063510160615));
#143860=CARTESIAN_POINT('Ctrl Pts',(87.9165820708691,14.55516355775,66.832622048277));
#143861=CARTESIAN_POINT('Ctrl Pts',(87.1896027922191,14.47674597442,67.36402324018));
#143862=CARTESIAN_POINT('Ctrl Pts',(86.523410283589,14.45075628501,67.604169553547));
#143863=CARTESIAN_POINT('Ctrl Pts',(86.1167247268192,14.45343250308,67.662585942143));
#143864=CARTESIAN_POINT('Ctrl Pts',(85.9893418468191,14.4559869198,67.672805629135));
#143865=CARTESIAN_POINT('Ctrl Pts',(87.7659216997691,15.40269777024,64.163723845293));
#143866=CARTESIAN_POINT('Ctrl Pts',(87.7773647030691,15.4002869873,64.20866780167));
#143867=CARTESIAN_POINT('Ctrl Pts',(87.8419823874691,15.38277416046,64.50249998336));
#143868=CARTESIAN_POINT('Ctrl Pts',(87.840895988169,15.32713368737,65.060818615117));
#143869=CARTESIAN_POINT('Ctrl Pts',(87.5862445180691,15.21768960789,65.737276187674));
#143870=CARTESIAN_POINT('Ctrl Pts',(87.1681234221592,15.11051345271,66.238286033849));
#143871=CARTESIAN_POINT('Ctrl Pts',(86.6807204492591,15.0351865187,66.555863273335));
#143872=CARTESIAN_POINT('Ctrl Pts',(86.2648695496191,15.01090882485,66.69410425116));
#143873=CARTESIAN_POINT('Ctrl Pts',(86.0139094660691,15.01327826998,66.731297190963));
#143874=CARTESIAN_POINT('Ctrl Pts',(85.9350444544391,15.01568051436,66.738612051129));
#143875=CARTESIAN_POINT('Ctrl Pts',(86.9332803389491,14.72899156245,64.368226172776));
#143876=CARTESIAN_POINT('Ctrl Pts',(86.9399959780591,14.72666943294,64.394312291263));
#143877=CARTESIAN_POINT('Ctrl Pts',(86.9780279391791,14.70981934282,64.564854256711));
#143878=CARTESIAN_POINT('Ctrl Pts',(86.9790987592991,14.65667337628,64.889105458825));
#143879=CARTESIAN_POINT('Ctrl Pts',(86.8340345043091,14.54983857184,65.285119497221));
#143880=CARTESIAN_POINT('Ctrl Pts',(86.5913101296991,14.44160203029,65.5826856115101));
#143881=CARTESIAN_POINT('Ctrl Pts',(86.3034141674891,14.36255245106,65.774586384496));
#143882=CARTESIAN_POINT('Ctrl Pts',(86.0543471845591,14.33621268175,65.858780684233));
#143883=CARTESIAN_POINT('Ctrl Pts',(85.9036912609991,14.33895163073,65.880969539341));
#143884=CARTESIAN_POINT('Ctrl Pts',(85.8563785120091,14.34153716464,65.885238584742));
#143885=CARTESIAN_POINT('Ctrl Pts',(87.2326575734091,13.68901688165,64.234896062448));
#143886=CARTESIAN_POINT('Ctrl Pts',(87.241044301839,13.68683160307,64.263453882858));
#143887=CARTESIAN_POINT('Ctrl Pts',(87.2900525363391,13.67100455445,64.450120590002));
#143888=CARTESIAN_POINT('Ctrl Pts',(87.315030254419,13.62170926292,64.807824093329));
#143889=CARTESIAN_POINT('Ctrl Pts',(87.1945462053492,13.51890229723,65.288770118133));
#143890=CARTESIAN_POINT('Ctrl Pts',(86.9282513347491,13.40902887753,65.70929487038));
#143891=CARTESIAN_POINT('Ctrl Pts',(86.543113884849,13.32423279229,66.025357899537));
#143892=CARTESIAN_POINT('Ctrl Pts',(86.162694386879,13.29470987542,66.17289886931));
#143893=CARTESIAN_POINT('Ctrl Pts',(85.9278732541291,13.29801921346,66.205606769103));
#143894=CARTESIAN_POINT('Ctrl Pts',(85.8545530515491,13.30088768445,66.210607657589));
#143895=CARTESIAN_POINT('',(87.2268072287975,13.97255211819,64.4085086937024));
#143896=CARTESIAN_POINT('Ctrl Pts',(87.2268072287975,13.97255211819,64.4085086937024));
#143897=CARTESIAN_POINT('Ctrl Pts',(87.2312812396292,13.9698592700985,64.4338829742751));
#143898=CARTESIAN_POINT('Ctrl Pts',(87.2354272871341,13.9665880921402,64.4612020199036));
#143899=CARTESIAN_POINT('Ctrl Pts',(87.2389350555738,13.9627385843149,64.4904691407583));
#143900=CARTESIAN_POINT('Ctrl Pts',(87.2423151679509,13.9590291692638,64.5186711612585));
#143901=CARTESIAN_POINT('Ctrl Pts',(87.2451022399931,13.9547827520096,64.5486825826784));
#143902=CARTESIAN_POINT('Ctrl Pts',(87.2469812637975,13.9499993325526,64.5804766593118));
#143903=CARTESIAN_POINT('Ctrl Pts',(87.2488177885167,13.9453241027575,64.6115516289473));
#143904=CARTESIAN_POINT('Ctrl Pts',(87.2497865220104,13.9401358874976,64.644330080219));
#143905=CARTESIAN_POINT('Ctrl Pts',(87.2495621407118,13.9344346867727,64.6787501211913));
#143906=CARTESIAN_POINT('Ctrl Pts',(87.2493461835623,13.9289475313605,64.7118778995703));
#143907=CARTESIAN_POINT('Ctrl Pts',(87.2480245505996,13.9229851863581,64.7465266782797));
#143908=CARTESIAN_POINT('Ctrl Pts',(87.2452840225134,13.9165476517654,64.7826002641726));
#143909=CARTESIAN_POINT('Ctrl Pts',(87.2426391201109,13.9103347430945,64.8174151286769));
#143910=CARTESIAN_POINT('Ctrl Pts',(87.238672141117,13.9036792280069,64.8535573775341));
#143911=CARTESIAN_POINT('Ctrl Pts',(87.2330862628216,13.8965811065027,64.8908970380363));
#143912=CARTESIAN_POINT('Ctrl Pts',(87.227475282113,13.8894510867063,64.9284044994698));
#143913=CARTESIAN_POINT('Ctrl Pts',(87.2202303287225,13.8818744734913,64.9671207126452));
#143914=CARTESIAN_POINT('Ctrl Pts',(87.2110418621861,13.8738512668577,65.0068627398523));
#143915=CARTESIAN_POINT('Ctrl Pts',(87.2023231880501,13.8662382746477,65.0445728173009));
#143916=CARTESIAN_POINT('Ctrl Pts',(87.1918541218471,13.8582231888616,65.0832064522933));
#143917=CARTESIAN_POINT('Ctrl Pts',(87.1793699426723,13.8498060094996,65.1225585398391));
#143918=CARTESIAN_POINT('Ctrl Pts',(87.1671491162136,13.8415663898326,65.1610804983878));
#143919=CARTESIAN_POINT('Ctrl Pts',(87.152996760082,13.8329414619205,65.200291035028));
#143920=CARTESIAN_POINT('Ctrl Pts',(87.1366720319832,13.8239312257634,65.2399488099957));
#143921=CARTESIAN_POINT('Ctrl Pts',(87.1208093365176,13.8151760029279,65.2784841658893));
#143922=CARTESIAN_POINT('Ctrl Pts',(87.1028949803302,13.806056973669,65.3174417675221));
#143923=CARTESIAN_POINT('Ctrl Pts',(87.0827227812748,13.7965741379866,65.3565529957343));
#143924=CARTESIAN_POINT('Ctrl Pts',(87.0778123620077,13.7942657779058,65.3660736497813));
#143925=CARTESIAN_POINT('Ctrl Pts',(87.0727682435476,13.7919358601946,65.3756031840621));
#143926=CARTESIAN_POINT('Ctrl Pts',(87.0675876448807,13.7895843848528,65.3851372898738));
#143927=CARTESIAN_POINT('Ctrl Pts',(87.0518679418159,13.782449206756,65.4140670182677));
#143928=CARTESIAN_POINT('Ctrl Pts',(87.0348909798187,13.7751155426953,65.4430399321384));
#143929=CARTESIAN_POINT('Ctrl Pts',(87.0165845281435,13.7675833926708,65.4719258986537));
#143930=CARTESIAN_POINT('Ctrl Pts',(87.0074313023059,13.7638173176586,65.4863688819112));
#143931=CARTESIAN_POINT('Ctrl Pts',(86.9979458392243,13.7600016211554,65.5007898979865));
#143932=CARTESIAN_POINT('Ctrl Pts',(86.9881200266237,13.7561363031612,65.5151712902311));
#143933=CARTESIAN_POINT('Ctrl Pts',(86.9832071203233,13.7542036441641,65.5223619863535));
#143934=CARTESIAN_POINT('Ctrl Pts',(86.9782091268413,13.7522585797943,65.529542776657));
#143935=CARTESIAN_POINT('Ctrl Pts',(86.9731251124026,13.7503011100517,65.5367113457746));
#143936=CARTESIAN_POINT('Ctrl Pts',(86.9700355107765,13.7491115379582,65.5410677501612));
#143937=CARTESIAN_POINT('Ctrl Pts',(86.9665039298293,13.747760364286,65.5459898821353));
#143938=CARTESIAN_POINT('Ctrl Pts',(86.9632751770817,13.7465338567315,65.5504355297153));
#143939=CARTESIAN_POINT('Ctrl Pts',(86.9611909388439,13.7457421163464,65.5533053030929));
#143940=CARTESIAN_POINT('Ctrl Pts',(86.9592340192321,13.7450023245288,65.5559773238831));
#143941=CARTESIAN_POINT('Ctrl Pts',(86.9576140827913,13.7443914847058,65.5581780686928));
#143942=CARTESIAN_POINT('Ctrl Pts',(86.9276120553036,13.7330784277883,65.5989369556538));
#143943=CARTESIAN_POINT('Ctrl Pts',(86.8960454693322,13.7224082080239,65.6374984887618));
#143944=CARTESIAN_POINT('Ctrl Pts',(86.86326398763,13.7123808254125,65.6738297509258));
#143945=CARTESIAN_POINT('Ctrl Pts',(86.8296033654357,13.7020845264,65.7111353523215));
#143946=CARTESIAN_POINT('Ctrl Pts',(86.7946622475351,13.6924660063563,65.7460897243064));
#143947=CARTESIAN_POINT('Ctrl Pts',(86.7587956819623,13.6835252652814,65.7787070560654));
#143948=CARTESIAN_POINT('Ctrl Pts',(86.7223633854806,13.6744435000105,65.8118388678826));
#143949=CARTESIAN_POINT('Ctrl Pts',(86.6849765503329,13.6660610638373,65.842559747867));
#143950=CARTESIAN_POINT('Ctrl Pts',(86.6469774815292,13.6583779567619,65.8709299052986));
#143951=CARTESIAN_POINT('Ctrl Pts',(86.6080887922948,13.6505149755675,65.8999642545766));
#143952=CARTESIAN_POINT('Ctrl Pts',(86.5685591778603,13.6433844516553,65.9265369400317));
#143953=CARTESIAN_POINT('Ctrl Pts',(86.5287195432174,13.6369863850254,65.9507532985586));
#143954=CARTESIAN_POINT('Ctrl Pts',(86.5187484575909,13.6353850733974,65.9568141820632));
#143955=CARTESIAN_POINT('Ctrl Pts',(86.5087577674021,13.6338296431522,65.9627276422958));
#143956=CARTESIAN_POINT('Ctrl Pts',(86.4987522872098,13.6323200942899,65.9684956696234));
#143957=CARTESIAN_POINT('Ctrl Pts',(86.457246068366,13.6260579595165,65.9924234571914));
#143958=CARTESIAN_POINT('Ctrl Pts',(86.4154889093146,13.620585388071,66.0138460386652));
#143959=CARTESIAN_POINT('Ctrl Pts',(86.3737965186916,13.6159023799535,66.0329262200579));
#143960=CARTESIAN_POINT('Ctrl Pts',(86.3313585325839,13.6111356244266,66.0523476171228));
#143961=CARTESIAN_POINT('Ctrl Pts',(86.2889877557992,13.6071869246566,66.0693426394481));
#143962=CARTESIAN_POINT('Ctrl Pts',(86.2469691935481,13.6040562806436,66.0841107946872));
#143963=CARTESIAN_POINT('Ctrl Pts',(86.2036516610332,13.6008288552735,66.0993354956402));
#143964=CARTESIAN_POINT('Ctrl Pts',(86.1607085767477,13.5984708465459,66.1121940545044));
#143965=CARTESIAN_POINT('Ctrl Pts',(86.1183997985764,13.5969822544608,66.1229259772511));
#143966=CARTESIAN_POINT('Ctrl Pts',(86.0818331447479,13.5956956932831,66.1322013692844));
#143967=CARTESIAN_POINT('Ctrl Pts',(86.0457393733944,13.5950585696962,66.1398887501012));
#143968=CARTESIAN_POINT('Ctrl Pts',(86.0102558429037,13.5950708837,66.1461501490856));
#143969=CARTESIAN_POINT('Origin',(88.2116008665994,13.9725941882181,64.234862063316));
#143970=CARTESIAN_POINT('Origin',(88.0541760202691,-0.499074165591386,63.341979795825));
#143971=CARTESIAN_POINT('',(87.1036300406178,13.9995834170875,63.709936145709));
#143972=CARTESIAN_POINT('Origin',(87.0693682672991,-0.499074165591386,63.515627973492));
#143973=CARTESIAN_POINT('Origin',(88.088437795226,13.9995833743814,63.5362879772457));
#143974=CARTESIAN_POINT('Origin',(88.0778048294691,9.5,63.475985431442));
#143975=CARTESIAN_POINT('',(86.3873398105787,11.4325417365447,59.6476527159751));
#143976=CARTESIAN_POINT('Ctrl Pts',(86.3873923039748,11.4323977449269,59.6479500913008));
#143977=CARTESIAN_POINT('Ctrl Pts',(86.4137108606564,11.7502480376137,59.7972100433247));
#143978=CARTESIAN_POINT('Ctrl Pts',(86.4760319983401,12.3203221675509,60.1506507663566));
#143979=CARTESIAN_POINT('Ctrl Pts',(86.6035424971191,13.05672232746,60.87379879423));
#143980=CARTESIAN_POINT('Ctrl Pts',(86.7559255690891,13.60185460728,61.7380059407));
#143981=CARTESIAN_POINT('Ctrl Pts',(86.9268053206991,13.93453843381,62.70711391189));
#143982=CARTESIAN_POINT('Ctrl Pts',(87.0436770949691,14.00347098775,63.369924833184));
#143983=CARTESIAN_POINT('Ctrl Pts',(87.1036300406291,13.99958341709,63.709936145707));
#143984=CARTESIAN_POINT('',(87.2158423658651,11.8669336587046,58.5875534023177));
#143985=CARTESIAN_POINT('Ctrl Pts',(87.2158423505991,11.86693347431,58.58755331574));
#143986=CARTESIAN_POINT('Ctrl Pts',(86.9577709596166,11.8673938453636,58.6322628228547));
#143987=CARTESIAN_POINT('Ctrl Pts',(86.7183367978951,11.8209912942895,58.7733653215963));
#143988=CARTESIAN_POINT('Ctrl Pts',(86.4118284068604,11.6615314736288,59.1669451161913));
#143989=CARTESIAN_POINT('Ctrl Pts',(86.3465703878581,11.5494863410242,59.4169490701672));
#143990=CARTESIAN_POINT('Ctrl Pts',(86.3873396949891,11.4325417044808,59.6476527211807));
#143991=CARTESIAN_POINT('Origin',(88.0778048294691,9.5,63.475985431442));
#143992=CARTESIAN_POINT('Origin',(58.0359414686091,9.5,68.773176492713));
#143993=CARTESIAN_POINT('',(91.0401366110177,11.8600632412174,57.9099602235744));
#143994=CARTESIAN_POINT('Ctrl Pts',(91.0790830817097,12.2828346383176,58.1314725547239));
#143995=CARTESIAN_POINT('Ctrl Pts',(91.0655561192021,12.1563659248288,58.0571151382804));
#143996=CARTESIAN_POINT('Ctrl Pts',(91.0534674480175,12.0155874078506,57.9833514930887));
#143997=CARTESIAN_POINT('Ctrl Pts',(91.0401366110177,11.8600632412174,57.9099602235744));
#143998=CARTESIAN_POINT('Ctrl Pts',(87.2158423505991,11.86693347431,58.58755331574));
#143999=CARTESIAN_POINT('Ctrl Pts',(88.4907931887827,11.8652382567572,58.3629426652979));
#144000=CARTESIAN_POINT('Ctrl Pts',(89.7656022238009,11.8639324281498,58.1375278091412));
#144001=CARTESIAN_POINT('Ctrl Pts',(91.0401366110177,11.8600632412174,57.9099602235744));
#144002=CARTESIAN_POINT('Origin',(91.9465816191691,-0.0433423696914158,
83.0870666032));
#144003=CARTESIAN_POINT('',(90.9047766966899,10.0691253898985,57.142294634787));
#144004=CARTESIAN_POINT('',(90.6242545431152,4.0210988023396,55.5521021866124));
#144005=CARTESIAN_POINT('Ctrl Pts',(90.904778401325,10.0691210019042,57.1423041413024));
#144006=CARTESIAN_POINT('Ctrl Pts',(90.8376715128848,9.09973890145265,56.7649981889273));
#144007=CARTESIAN_POINT('Ctrl Pts',(90.7811184881318,8.10415089350686,56.4431269592421));
#144008=CARTESIAN_POINT('Ctrl Pts',(90.6876392936001,6.08161709929453,55.9116332521325));
#144009=CARTESIAN_POINT('Ctrl Pts',(90.6508535215351,5.05587121367757,55.7027270401013));
#144010=CARTESIAN_POINT('Ctrl Pts',(90.6242545431152,4.0210988023396,55.5521021866125));
#144011=CARTESIAN_POINT('',(90.9921937685691,11.26993034099,57.63983708294));
#144012=CARTESIAN_POINT('Ctrl Pts',(90.9921937685691,11.26993034099,57.63983708294));
#144013=CARTESIAN_POINT('Ctrl Pts',(90.9607404151601,10.8632738684627,57.4621582006354));
#144014=CARTESIAN_POINT('Ctrl Pts',(90.9324253490825,10.4675402739369,57.2966575608245));
#144015=CARTESIAN_POINT('Ctrl Pts',(90.9047784163434,10.0691212184121,57.1423042252401));
#144016=CARTESIAN_POINT('Ctrl Pts',(91.0401366110177,11.8600632412174,57.9099602235744));
#144017=CARTESIAN_POINT('Ctrl Pts',(91.0254325534448,11.6817810703298,57.8215495147345));
#144018=CARTESIAN_POINT('Ctrl Pts',(91.008241628779,11.4857992440152,57.7340837415959));
#144019=CARTESIAN_POINT('Ctrl Pts',(90.9921937685691,11.26993034099,57.63983708294));
#144020=CARTESIAN_POINT('',(87.0625519269491,9.81028963511501,57.71791233337));
#144021=CARTESIAN_POINT('Origin',(91.5481551204691,-0.0433423696914658,
83.15731994474));
#144022=CARTESIAN_POINT('Ctrl Pts',(87.0625519269491,9.81028963511501,57.71791233337));
#144023=CARTESIAN_POINT('Ctrl Pts',(87.9398460791424,9.01004234588953,57.2538665845636));
#144024=CARTESIAN_POINT('Ctrl Pts',(88.6726439433507,8.12875357581062,56.8262866069459));
#144025=CARTESIAN_POINT('Ctrl Pts',(89.8570639140029,6.19929588766557,56.0883896079714));
#144026=CARTESIAN_POINT('Ctrl Pts',(90.3086910869141,5.15099973035466,55.778101303947));
#144027=CARTESIAN_POINT('Ctrl Pts',(90.6242545337037,4.02109881283824,55.5521021898692));
#144028=CARTESIAN_POINT('Ctrl Pts',(83.5527963632191,7.79551024574101,56.39696245495));
#144029=CARTESIAN_POINT('Ctrl Pts',(84.6832114812291,8.33549466069001,57.18456946643));
#144030=CARTESIAN_POINT('Ctrl Pts',(85.9062799740191,9.11477790243301,57.67842771583));
#144031=CARTESIAN_POINT('Ctrl Pts',(87.0598604213891,10.03501468075,57.80394780523));
#144032=CARTESIAN_POINT('Ctrl Pts',(83.9461301143991,7.49859304613501,56.27865761436));
#144033=CARTESIAN_POINT('Ctrl Pts',(85.1013709827991,8.01223740062101,57.02294274994));
#144034=CARTESIAN_POINT('Ctrl Pts',(86.3505790285991,8.74968408384501,57.47095990997));
#144035=CARTESIAN_POINT('Ctrl Pts',(87.5310943091691,9.61958516366902,57.5556017672));
#144036=CARTESIAN_POINT('Ctrl Pts',(84.6734906132591,6.86959461361001,56.04876303691));
#144037=CARTESIAN_POINT('Ctrl Pts',(85.8693472222591,7.32712499929101,56.71036553051));
#144038=CARTESIAN_POINT('Ctrl Pts',(87.1601981332091,7.97782666496401,57.07216083468));
#144039=CARTESIAN_POINT('Ctrl Pts',(88.3840197380691,8.74413048764801,57.08058953316));
#144040=CARTESIAN_POINT('Ctrl Pts',(85.6006910643591,5.80441907889401,55.7287923738));
#144041=CARTESIAN_POINT('Ctrl Pts',(86.8339936590691,6.17114924616401,56.28135323536));
#144042=CARTESIAN_POINT('Ctrl Pts',(88.1602935371691,6.68693631322101,56.53299296536));
#144043=CARTESIAN_POINT('Ctrl Pts',(89.4222061602691,7.29363942440101,56.44631864302));
#144044=CARTESIAN_POINT('Ctrl Pts',(86.3890436286191,4.56793334804501,55.43379604209));
#144045=CARTESIAN_POINT('Ctrl Pts',(87.6400403009691,4.83930736953001,55.89394630833));
#144046=CARTESIAN_POINT('Ctrl Pts',(88.9796858299691,5.21750983688301,56.05603070301));
#144047=CARTESIAN_POINT('Ctrl Pts',(90.2577115618691,5.66224725175901,55.89495734691));
#144048=CARTESIAN_POINT('Ctrl Pts',(86.7846654732391,3.65544465457401,55.27474745921));
#144049=CARTESIAN_POINT('Ctrl Pts',(88.0375966273691,3.86480378841501,55.68903466726));
#144050=CARTESIAN_POINT('Ctrl Pts',(89.3757879463691,4.15550040108601,55.80860463891));
#144051=CARTESIAN_POINT('Ctrl Pts',(90.6540092174691,4.49744425651901,55.61381970811));
#144052=CARTESIAN_POINT('Ctrl Pts',(86.9516944429091,3.16130406753901,55.20620234028));
#144053=CARTESIAN_POINT('Ctrl Pts',(88.2044408468691,3.33962332755001,55.60142198926));
#144054=CARTESIAN_POINT('Ctrl Pts',(89.5408894909691,3.58684077310001,55.70363976371));
#144055=CARTESIAN_POINT('Ctrl Pts',(90.8181034903691,3.87767846552801,55.49540382885));
#144056=CARTESIAN_POINT('',(87.0452063053445,3.32468194401047,55.2706145694237));
#144057=CARTESIAN_POINT('Ctrl Pts',(87.045203902867,3.32467973942797,55.2706236824706));
#144058=CARTESIAN_POINT('Ctrl Pts',(87.0470012523809,3.86784541765893,55.4025787775118));
#144059=CARTESIAN_POINT('Ctrl Pts',(87.0490460696036,4.40136020801294,55.5629627912764));
#144060=CARTESIAN_POINT('Ctrl Pts',(87.0510069518472,4.9241759395484,55.741622912552));
#144061=CARTESIAN_POINT('Ctrl Pts',(87.0511357651415,4.9585204887604,55.7533593637665));
#144062=CARTESIAN_POINT('Ctrl Pts',(87.0512642162768,4.99281886767013,55.7651746825583));
#144063=CARTESIAN_POINT('Ctrl Pts',(87.0513922869735,5.02707185220943,55.7770659468569));
#144064=CARTESIAN_POINT('Ctrl Pts',(87.0531964624245,5.50960529212154,55.9445822303015));
#144065=CARTESIAN_POINT('Ctrl Pts',(87.0549245412221,5.98313101850152,56.1271703607983));
#144066=CARTESIAN_POINT('Ctrl Pts',(87.0565238510531,6.44982066766169,56.3166620251401));
#144067=CARTESIAN_POINT('Ctrl Pts',(87.0567662711181,6.5205605161276,56.3453847783557));
#144068=CARTESIAN_POINT('Ctrl Pts',(87.0570057326289,6.59114329985223,56.3742661462039));
#144069=CARTESIAN_POINT('Ctrl Pts',(87.0572418456943,6.66157985193077,56.403277172837));
#144070=CARTESIAN_POINT('Ctrl Pts',(87.058513573033,7.04095779438498,56.5595333107053));
#144071=CARTESIAN_POINT('Ctrl Pts',(87.0596934926687,7.41609585314038,56.7195520426998));
#144072=CARTESIAN_POINT('Ctrl Pts',(87.0607150048372,7.78868443971465,56.8788072211256));
#144073=CARTESIAN_POINT('Ctrl Pts',(87.061816906091,8.19059431738695,57.0505951705856));
#144074=CARTESIAN_POINT('Ctrl Pts',(87.0627344512309,8.58953771072732,57.2214945859138));
#144075=CARTESIAN_POINT('Ctrl Pts',(87.0630038488618,8.98798817633719,57.3865187845672));
#144076=CARTESIAN_POINT('Ctrl Pts',(87.0631892513137,9.26220622729475,57.50009027719));
#144077=CARTESIAN_POINT('Ctrl Pts',(87.0630676703773,9.53619078362226,57.6108791136097));
#144078=CARTESIAN_POINT('Ctrl Pts',(87.0624604019528,9.81049105390748,57.7173931076103));
#144079=CARTESIAN_POINT('Origin',(88.9840679110593,4.82687630561811,49.4062655211528));
#144080=CARTESIAN_POINT('Ctrl Pts',(86.2777587182191,3.35797480132401,55.0378852179));
#144081=CARTESIAN_POINT('Ctrl Pts',(87.6910580236691,3.55694831838901,55.61191127816));
#144082=CARTESIAN_POINT('Ctrl Pts',(89.2470251821691,3.86322784531101,55.79788947715));
#144083=CARTESIAN_POINT('Ctrl Pts',(90.7231331745691,4.23364950808901,55.56595754335));
#144084=CARTESIAN_POINT('Ctrl Pts',(86.7049180588991,2.24396285722701,54.88675785712));
#144085=CARTESIAN_POINT('Ctrl Pts',(88.1203558938691,2.36828606915101,55.40277505789));
#144086=CARTESIAN_POINT('Ctrl Pts',(89.6721739084691,2.55739749999101,55.53501604492));
#144087=CARTESIAN_POINT('Ctrl Pts',(91.1466488631691,2.78622655700001,55.26249917316));
#144088=CARTESIAN_POINT('Ctrl Pts',(86.9126052467991,1.05468974025801,54.80544650431));
#144089=CARTESIAN_POINT('Ctrl Pts',(88.3228401741691,1.11258841309801,55.294362315));
#144090=CARTESIAN_POINT('Ctrl Pts',(89.8650971183691,1.20112353795701,55.40385472609));
#144091=CARTESIAN_POINT('Ctrl Pts',(91.3314350643691,1.30850424140801,55.11623041902));
#144092=CARTESIAN_POINT('Ctrl Pts',(86.8937434252391,-0.150524780926486,
54.8128006371));
#144093=CARTESIAN_POINT('Ctrl Pts',(88.3044266143691,-0.158795700165486,
55.30418203856));
#144094=CARTESIAN_POINT('Ctrl Pts',(89.8475225660691,-0.171437606626586,
55.41575356859));
#144095=CARTESIAN_POINT('Ctrl Pts',(91.3145709684691,-0.186767340196186,
55.1295192676));
#144096=CARTESIAN_POINT('',(91.1670701462358,2.74307740674274E-14,55.1562792695813));
#144097=CARTESIAN_POINT('Ctrl Pts',(90.6242676274951,4.02108764649613,55.5521764045675));
#144098=CARTESIAN_POINT('Ctrl Pts',(90.6813389532947,3.8179674433382,55.5116429418745));
#144099=CARTESIAN_POINT('Ctrl Pts',(90.7332711723362,3.61452700426379,55.4743452737089));
#144100=CARTESIAN_POINT('Ctrl Pts',(90.7804179111772,3.41093104822288,55.440220608944));
#144101=CARTESIAN_POINT('Ctrl Pts',(90.8278289816426,3.20619361662901,55.4059046217613));
#144102=CARTESIAN_POINT('Ctrl Pts',(90.8704007345699,3.00129904715451,55.374797431572));
#144103=CARTESIAN_POINT('Ctrl Pts',(90.9084408089441,2.79640895953868,55.346841452405));
#144104=CARTESIAN_POINT('Ctrl Pts',(90.9217531255787,2.72470663596276,55.3370581159467));
#144105=CARTESIAN_POINT('Ctrl Pts',(90.9345099925611,2.65300480010805,55.3276607516866));
#144106=CARTESIAN_POINT('Ctrl Pts',(90.9467231118361,2.58131016892631,55.3186470337802));
#144107=CARTESIAN_POINT('Ctrl Pts',(90.9795215444716,2.38877364502865,55.2944406199317));
#144108=CARTESIAN_POINT('Ctrl Pts',(91.0084013120712,2.19628946790016,55.2730008323369));
#144109=CARTESIAN_POINT('Ctrl Pts',(91.0335604077023,2.0039904930509,55.254286091841));
#144110=CARTESIAN_POINT('Ctrl Pts',(91.0605575797341,1.79764251529882,55.2342040874594));
#144111=CARTESIAN_POINT('Ctrl Pts',(91.0832710805389,1.59150787532994,55.2172598837242));
#144112=CARTESIAN_POINT('Ctrl Pts',(91.1018956986807,1.38574194395299,55.2034051674291));
#144113=CARTESIAN_POINT('Ctrl Pts',(91.1205387383242,1.17977249068807,55.1895367475145));
#144114=CARTESIAN_POINT('Ctrl Pts',(91.1350847496725,0.974172664288115,
55.1787639986015));
#144115=CARTESIAN_POINT('Ctrl Pts',(91.1456782134625,0.769086615773664,
55.1710404532243));
#144116=CARTESIAN_POINT('Ctrl Pts',(91.1562761152521,0.563914649017109,
55.1633136721642));
#144117=CARTESIAN_POINT('Ctrl Pts',(91.1629180943347,0.359257095879952,
55.1586386921846));
#144118=CARTESIAN_POINT('Ctrl Pts',(91.165698781784,0.155243665858008,55.1569701398367));
#144119=CARTESIAN_POINT('Ctrl Pts',(91.1664046750334,0.103453701808425,
55.1565465683781));
#144120=CARTESIAN_POINT('Ctrl Pts',(91.1668614876952,0.0517051643952373,
55.1563167434454));
#144121=CARTESIAN_POINT('Ctrl Pts',(91.1670702628135,2.73247007625336E-14,
55.156279930759));
#144122=CARTESIAN_POINT('',(87.0379664172709,2.17389847372088E-10,54.8607146728376));
#144123=CARTESIAN_POINT('Ctrl Pts',(87.0379678287862,4.10407994795547E-10,
54.8607103703767));
#144124=CARTESIAN_POINT('Ctrl Pts',(87.0379693004997,0.20239753568915,54.8607199332154));
#144125=CARTESIAN_POINT('Ctrl Pts',(87.0380265697462,0.407113829529953,
54.865362440369));
#144126=CARTESIAN_POINT('Ctrl Pts',(87.0381782738253,0.613853290402161,
54.8748935232933));
#144127=CARTESIAN_POINT('Ctrl Pts',(87.0382727664481,0.742626056552804,
54.8808301930873));
#144128=CARTESIAN_POINT('Ctrl Pts',(87.0384036832572,0.872182872546045,
54.8886637295171));
#144129=CARTESIAN_POINT('Ctrl Pts',(87.0385782393398,1.00244245311521,54.8984581722552));
#144130=CARTESIAN_POINT('Ctrl Pts',(87.038856657565,1.21020743434017,54.9140803798709));
#144131=CARTESIAN_POINT('Ctrl Pts',(87.0392469253613,1.41976219000755,54.9346923733824));
#144132=CARTESIAN_POINT('Ctrl Pts',(87.03974221153,1.63084475620316,54.9604067657937));
#144133=CARTESIAN_POINT('Ctrl Pts',(87.0402076100815,1.82918972676854,54.9845694453454));
#144134=CARTESIAN_POINT('Ctrl Pts',(87.0407656988976,2.02888353522731,55.0132373241063));
#144135=CARTESIAN_POINT('Ctrl Pts',(87.0413993099936,2.22967027819263,55.0464953442303));
#144136=CARTESIAN_POINT('Ctrl Pts',(87.0420220231652,2.42700354829937,55.0791813362008));
#144137=CARTESIAN_POINT('Ctrl Pts',(87.0427179229967,2.62539230935319,55.1163025646978));
#144138=CARTESIAN_POINT('Ctrl Pts',(87.0434324375699,2.82460332828506,55.1577725266321));
#144139=CARTESIAN_POINT('Ctrl Pts',(87.0440284707663,2.9907810170511,55.1923659063779));
#144140=CARTESIAN_POINT('Ctrl Pts',(87.044637213594,3.15753036322419,55.2299849453235));
#144141=CARTESIAN_POINT('Ctrl Pts',(87.0452197681563,3.32469429787419,55.2705635024578));
#144142=CARTESIAN_POINT('Origin',(89.5099641414739,-2.03747057816781E-10,
48.9689653069594));
#144143=CARTESIAN_POINT('Ctrl Pts',(86.8937713403091,0.150278927427014,
54.81280807796));
#144144=CARTESIAN_POINT('Ctrl Pts',(88.3043999218691,0.158534897272514,
55.3042706166));
#144145=CARTESIAN_POINT('Ctrl Pts',(89.8475194425691,0.171158442280014,
55.41552889153));
#144146=CARTESIAN_POINT('Ctrl Pts',(91.3145776951691,0.186460507929914,
55.12953401502));
#144147=CARTESIAN_POINT('Ctrl Pts',(86.9126943758391,-1.06234500207499,
54.80543698782));
#144148=CARTESIAN_POINT('Ctrl Pts',(88.3228790529691,-1.12065140134899,
55.29442473537));
#144149=CARTESIAN_POINT('Ctrl Pts',(89.8651634112691,-1.20984047105699,
55.40359516778));
#144150=CARTESIAN_POINT('Ctrl Pts',(91.3315154389691,-1.31797588386699,
55.11620079281));
#144151=CARTESIAN_POINT('Ctrl Pts',(86.7024783203091,-2.25075885387899,
54.88765019828));
#144152=CARTESIAN_POINT('Ctrl Pts',(88.1178555459691,-2.37550823105599,
55.40408429379));
#144153=CARTESIAN_POINT('Ctrl Pts',(89.6697334134691,-2.56535408039399,
55.53630712185));
#144154=CARTESIAN_POINT('Ctrl Pts',(91.1442381655691,-2.79499085550699,
55.26426627484));
#144155=CARTESIAN_POINT('Ctrl Pts',(86.2773845990691,-3.35901852522699,
55.03803802306));
#144156=CARTESIAN_POINT('Ctrl Pts',(87.6906204733691,-3.55803150344899,
55.61220513576));
#144157=CARTESIAN_POINT('Ctrl Pts',(89.2466200909691,-3.86449453312799,
55.79788968037));
#144158=CARTESIAN_POINT('Ctrl Pts',(90.7227405050691,-4.23499951536299,
55.56626117546));
#144159=CARTESIAN_POINT('',(90.6242675720478,-4.0209956755633,55.5521118754408));
#144160=CARTESIAN_POINT('Ctrl Pts',(91.1670701073691,2.7354895961722E-14,
55.15627904919));
#144161=CARTESIAN_POINT('Ctrl Pts',(91.165849317076,-0.34243594626333,55.1564952164306));
#144162=CARTESIAN_POINT('Ctrl Pts',(91.1540382483519,-0.685319034794855,
55.1651207635041));
#144163=CARTESIAN_POINT('Ctrl Pts',(91.1196950287164,-1.19945881862615,
55.1907739782479));
#144164=CARTESIAN_POINT('Ctrl Pts',(91.105470345645,-1.37080633281857,55.2014442692401));
#144165=CARTESIAN_POINT('Ctrl Pts',(91.0798226281247,-1.62765967198077,
55.220642109171));
#144166=CARTESIAN_POINT('Ctrl Pts',(91.0659205480108,-1.75604424626546,
55.2310391461268));
#144167=CARTESIAN_POINT('Ctrl Pts',(91.0503689410442,-1.88434237146833,
55.2426360874994));
#144168=CARTESIAN_POINT('Ctrl Pts',(91.0396307218966,-1.96985259603912,
55.250634346356));
#144169=CARTESIAN_POINT('Ctrl Pts',(91.0337889985745,-2.01473568195959,
55.2549805002222));
#144170=CARTESIAN_POINT('Ctrl Pts',(90.9410678105965,-2.7048171237868,55.3238766186337));
#144171=CARTESIAN_POINT('Ctrl Pts',(90.8097152049346,-3.3619013328331,55.4205634794744));
#144172=CARTESIAN_POINT('Ctrl Pts',(90.6242620411691,-4.02100037299999,
55.55208048089));
#144173=CARTESIAN_POINT('',(87.0451990682794,-3.32463143800401,55.2706077778965));
#144174=CARTESIAN_POINT('Ctrl Pts',(87.0452086535362,-3.32464023403444,
55.2705714208367));
#144175=CARTESIAN_POINT('Ctrl Pts',(87.044512655429,-3.12434940334929,55.2219520465534));
#144176=CARTESIAN_POINT('Ctrl Pts',(87.0437782589915,-2.92464886642339,
55.1775771565754));
#144177=CARTESIAN_POINT('Ctrl Pts',(87.0430717007898,-2.72580575381143,
55.1375605048055));
#144178=CARTESIAN_POINT('Ctrl Pts',(87.0424604951936,-2.55379724423082,
55.1029442460931));
#144179=CARTESIAN_POINT('Ctrl Pts',(87.0418699116625,-2.38242948815377,
55.071588697763));
#144180=CARTESIAN_POINT('Ctrl Pts',(87.0413346239677,-2.21185108387118,
55.0435494536918));
#144181=CARTESIAN_POINT('Ctrl Pts',(87.0407234368002,-2.01708603929369,
55.0115344712302));
#144182=CARTESIAN_POINT('Ctrl Pts',(87.0401843291019,-1.82335088020513,
54.9838418574831));
#144183=CARTESIAN_POINT('Ctrl Pts',(87.039732739701,-1.63088300680562,54.9603934382341));
#144184=CARTESIAN_POINT('Ctrl Pts',(87.0392228290388,-1.41355855107868,
54.9339167340397));
#144185=CARTESIAN_POINT('Ctrl Pts',(87.0388247135594,-1.1978503828135,54.9128513309689));
#144186=CARTESIAN_POINT('Ctrl Pts',(87.0385455377253,-0.984048864472286,
54.8970736810246));
#144187=CARTESIAN_POINT('Ctrl Pts',(87.0382733538861,-0.775602032849812,
54.8816911843666));
#144188=CARTESIAN_POINT('Ctrl Pts',(87.0381138462719,-0.568968001308234,
54.8713330126585));
#144189=CARTESIAN_POINT('Ctrl Pts',(87.0380333744037,-0.364473437435225,
54.865729131077));
#144190=CARTESIAN_POINT('Ctrl Pts',(87.0379852570288,-0.242197891955986,
54.8623783443167));
#144191=CARTESIAN_POINT('Ctrl Pts',(87.0379651969979,-0.120686245134875,
54.8607276135635));
#144192=CARTESIAN_POINT('Ctrl Pts',(87.0379642136838,4.26840621093993E-10,
54.8607213896952));
#144193=CARTESIAN_POINT('Origin',(88.9855508168953,-4.82568011021053,49.4111666499231));
#144194=CARTESIAN_POINT('Ctrl Pts',(86.9516806969691,-3.16128829937699,
55.20619343277));
#144195=CARTESIAN_POINT('Ctrl Pts',(88.2046044567691,-3.33963640945299,
55.60147925581));
#144196=CARTESIAN_POINT('Ctrl Pts',(89.5412550807691,-3.58690525771299,
55.70367918435));
#144197=CARTESIAN_POINT('Ctrl Pts',(90.8186331109691,-3.87780431688299,
55.49533239395));
#144198=CARTESIAN_POINT('Ctrl Pts',(86.3310017513891,-4.99858829213699,
55.46112141282));
#144199=CARTESIAN_POINT('Ctrl Pts',(87.5848676480691,-5.29218632210199,
55.92705497751));
#144200=CARTESIAN_POINT('Ctrl Pts',(88.9282678155691,-5.70086660722399,
56.09343319582));
#144201=CARTESIAN_POINT('Ctrl Pts',(90.2096509505691,-6.18149989797999,
55.93471566337));
#144202=CARTESIAN_POINT('Ctrl Pts',(85.1490259917191,-6.59074061544199,
55.91688020941));
#144203=CARTESIAN_POINT('Ctrl Pts',(86.3803940981591,-7.02390396003999,
56.52876345794));
#144204=CARTESIAN_POINT('Ctrl Pts',(87.7097804104691,-7.63353048324999,
56.8365779079));
#144205=CARTESIAN_POINT('Ctrl Pts',(88.9728619095691,-8.34964142880199,
56.79608157395));
#144206=CARTESIAN_POINT('Ctrl Pts',(83.5523400802591,-7.79584216569499,
56.39708965395));
#144207=CARTESIAN_POINT('Ctrl Pts',(84.6828934797891,-8.33593481762399,
57.18486396867));
#144208=CARTESIAN_POINT('Ctrl Pts',(85.9061266288191,-9.11541493494999,
57.67880573437));
#144209=CARTESIAN_POINT('Ctrl Pts',(87.0598268116091,-10.03588562153,57.80428409672));
#144210=CARTESIAN_POINT('',(87.0625766316463,-9.81041847342618,57.7173854406919));
#144211=CARTESIAN_POINT('Ctrl Pts',(87.0625766316463,-9.81041847342618,
57.7173854406918));
#144212=CARTESIAN_POINT('Ctrl Pts',(87.0628390720482,-9.72800334949134,
57.6853973399913));
#144213=CARTESIAN_POINT('Ctrl Pts',(87.0630165460847,-9.64183968033886,
57.6515805060854));
#144214=CARTESIAN_POINT('Ctrl Pts',(87.0631680142214,-9.5518831048575,57.6158526863386));
#144215=CARTESIAN_POINT('Ctrl Pts',(87.0633173044982,-9.46321995533027,
57.580638573223));
#144216=CARTESIAN_POINT('Ctrl Pts',(87.0634412649436,-9.37087237149314,
57.543567861564));
#144217=CARTESIAN_POINT('Ctrl Pts',(87.0635591572122,-9.27480601330731,
57.5045950508041));
#144218=CARTESIAN_POINT('Ctrl Pts',(87.063676277597,-9.17936863662741,57.4658774092592));
#144219=CARTESIAN_POINT('Ctrl Pts',(87.0637873718588,-9.08026122963494,
57.4252823285718));
#144220=CARTESIAN_POINT('Ctrl Pts',(87.0638750591467,-8.9774553211851,57.3828008206487));
#144221=CARTESIAN_POINT('Ctrl Pts',(87.0639619897901,-8.87553651420938,
57.3406858812318));
#144222=CARTESIAN_POINT('Ctrl Pts',(87.0640258614301,-8.76998300272115,
57.2967168269121));
#144223=CARTESIAN_POINT('Ctrl Pts',(87.0640146935108,-8.66076881904943,
57.2509220047819));
#144224=CARTESIAN_POINT('Ctrl Pts',(87.0640067257105,-8.58284948796222,
57.218249491124));
#144225=CARTESIAN_POINT('Ctrl Pts',(87.0639598370757,-8.50306686636715,
57.184648402424));
#144226=CARTESIAN_POINT('Ctrl Pts',(87.063844289737,-8.42141094988714,57.1501411036244));
#144227=CARTESIAN_POINT('Ctrl Pts',(87.0636971541048,-8.31743196586373,
57.1062002108483));
#144228=CARTESIAN_POINT('Ctrl Pts',(87.0634755557133,-8.21039512883709,
57.0607768776444));
#144229=CARTESIAN_POINT('Ctrl Pts',(87.0632118349515,-8.10023332471427,
57.0139242727969));
#144230=CARTESIAN_POINT('Ctrl Pts',(87.0629538134131,-7.99245220816343,
56.9680841914367));
#144231=CARTESIAN_POINT('Ctrl Pts',(87.0626555217958,-7.88168000204142,
56.9208760258635));
#144232=CARTESIAN_POINT('Ctrl Pts',(87.0623152977027,-7.76783902226488,
56.8723843235867));
#144233=CARTESIAN_POINT('Ctrl Pts',(87.0620908174656,-7.69272661651815,
56.8403894442039));
#144234=CARTESIAN_POINT('Ctrl Pts',(87.0618474375089,-7.61627795303887,
56.8078365028245));
#144235=CARTESIAN_POINT('Ctrl Pts',(87.0615765299235,-7.53846614864338,
56.7747580743624));
#144236=CARTESIAN_POINT('Ctrl Pts',(87.0611942931426,-7.42867766273656,
56.728086099522));
#144237=CARTESIAN_POINT('Ctrl Pts',(87.0607724680966,-7.31617500558751,
56.6803657943976));
#144238=CARTESIAN_POINT('Ctrl Pts',(87.0603299026845,-7.20087200964981,
56.6317176985142));
#144239=CARTESIAN_POINT('Ctrl Pts',(87.0601349919148,-7.15009127741691,
56.6102925316257));
#144240=CARTESIAN_POINT('Ctrl Pts',(87.0599356548905,-7.09876703602993,
56.5886877983236));
#144241=CARTESIAN_POINT('Ctrl Pts',(87.0597314860299,-7.04689015678793,
56.5669156204394));
#144242=CARTESIAN_POINT('Ctrl Pts',(87.0593976081587,-6.96205576063497,
56.5313115210655));
#144243=CARTESIAN_POINT('Ctrl Pts',(87.0590537502245,-6.87574472053487,
56.4952595532075));
#144244=CARTESIAN_POINT('Ctrl Pts',(87.0587059254545,-6.78791548485091,
56.4588226097982));
#144245=CARTESIAN_POINT('Ctrl Pts',(87.0585320130695,-6.74400086700893,
56.4406041380935));
#144246=CARTESIAN_POINT('Ctrl Pts',(87.0583570948179,-6.699706629326,56.4222895954189));
#144247=CARTESIAN_POINT('Ctrl Pts',(87.0581820490815,-6.65502710214539,
56.4038879243479));
#144248=CARTESIAN_POINT('Ctrl Pts',(87.0580945262132,-6.63268733855508,
56.3946870888124));
#144249=CARTESIAN_POINT('Ctrl Pts',(87.0580069704471,-6.61025124788037,
56.3854644828236));
#144250=CARTESIAN_POINT('Ctrl Pts',(87.057919492524,-6.58771809232852,56.3762212956712));
#144251=CARTESIAN_POINT('Ctrl Pts',(87.0578487179328,-6.56948749407615,
56.3687430340865));
#144252=CARTESIAN_POINT('Ctrl Pts',(87.0577762649015,-6.55023610058555,
56.3608598848097));
#144253=CARTESIAN_POINT('Ctrl Pts',(87.0577058929201,-6.53228718790687,
56.3535227476336));
#144254=CARTESIAN_POINT('Ctrl Pts',(87.0576892846071,-6.52805111050587,
56.3517911284801));
#144255=CARTESIAN_POINT('Ctrl Pts',(87.0576729901796,-6.52388748793224,
56.3500898405514));
#144256=CARTESIAN_POINT('Ctrl Pts',(87.0576574112025,-6.51982669637165,
56.3484312386392));
#144257=CARTESIAN_POINT('Ctrl Pts',(87.0571374689694,-6.38429937495421,
56.2930760520697));
#144258=CARTESIAN_POINT('Ctrl Pts',(87.0566006156764,-6.2515905165016,56.2396059531338));
#144259=CARTESIAN_POINT('Ctrl Pts',(87.05604921051,-6.12167918640636,56.1881084907986));
#144260=CARTESIAN_POINT('Ctrl Pts',(87.0554872516434,-5.98928139932232,
56.1356253852171));
#144261=CARTESIAN_POINT('Ctrl Pts',(87.0549099356614,-5.85978891486309,
56.0851907730958));
#144262=CARTESIAN_POINT('Ctrl Pts',(87.0543251722186,-5.73321454309557,
56.0368560060033));
#144263=CARTESIAN_POINT('Ctrl Pts',(87.0537357786718,-5.6056379669076,55.9881385285993));
#144264=CARTESIAN_POINT('Ctrl Pts',(87.0531385664979,-5.48102569214467,
55.9415538436113));
#144265=CARTESIAN_POINT('Ctrl Pts',(87.052550870209,-5.35943007569011,55.8971192626733));
#144266=CARTESIAN_POINT('Ctrl Pts',(87.0519558777,-5.23632485570613,55.8521330286235));
#144267=CARTESIAN_POINT('Ctrl Pts',(87.0513703909122,-5.11631150324506,
55.8093502210095));
#144268=CARTESIAN_POINT('Ctrl Pts',(87.0508256785423,-4.99948723236905,
55.7687590932993));
#144269=CARTESIAN_POINT('Ctrl Pts',(87.0503358700086,-4.89443816795456,
55.7322593149784));
#144270=CARTESIAN_POINT('Ctrl Pts',(87.0498791272192,-4.79196827286971,
55.6975310760738));
#144271=CARTESIAN_POINT('Ctrl Pts',(87.0494893659084,-4.6921783257891,55.6645495917059));
#144272=CARTESIAN_POINT('Ctrl Pts',(87.0490528360166,-4.58041429584728,
55.6276105641358));
#144273=CARTESIAN_POINT('Ctrl Pts',(87.0486704434854,-4.47206232451012,
55.5928728915689));
#144274=CARTESIAN_POINT('Ctrl Pts',(87.0483243200076,-4.36712983835204,
55.5602093885637));
#144275=CARTESIAN_POINT('Ctrl Pts',(87.0479620947937,-4.25731587116184,
55.5260263726202));
#144276=CARTESIAN_POINT('Ctrl Pts',(87.047639371313,-4.15124699665592,55.4941147704494));
#144277=CARTESIAN_POINT('Ctrl Pts',(87.0473383877036,-4.0489891864447,55.4643215436082));
#144278=CARTESIAN_POINT('Ctrl Pts',(87.0470281082852,-3.94357316747328,
55.4336081598636));
#144279=CARTESIAN_POINT('Ctrl Pts',(87.0467408565464,-3.84220755551895,
55.4051457763424));
#144280=CARTESIAN_POINT('Ctrl Pts',(87.0464623874826,-3.74502133901434,
55.3787629182717));
#144281=CARTESIAN_POINT('Ctrl Pts',(87.0461680367163,-3.64229237903069,
55.3508753878329));
#144282=CARTESIAN_POINT('Ctrl Pts',(87.0458836085151,-3.5442333332799,55.3253110722094));
#144283=CARTESIAN_POINT('Ctrl Pts',(87.0455979336287,-3.45105532541971,
55.3018673545319));
#144284=CARTESIAN_POINT('Ctrl Pts',(87.0454654881388,-3.40785584417653,
55.2909983043629));
#144285=CARTESIAN_POINT('Ctrl Pts',(87.0453328410789,-3.36570630287924,
55.2805850943015));
#144286=CARTESIAN_POINT('Ctrl Pts',(87.0451990682794,-3.32463143800401,
55.2706077778965));
#144287=CARTESIAN_POINT('Ctrl Pts',(90.6242675720478,-4.0209956755633,55.5521118754408));
#144288=CARTESIAN_POINT('Ctrl Pts',(90.5688797519172,-4.21918219490549,
55.5916472433144));
#144289=CARTESIAN_POINT('Ctrl Pts',(90.5092334210679,-4.4148115362535,55.6339688670712));
#144290=CARTESIAN_POINT('Ctrl Pts',(90.4453817395859,-4.60789992207962,
55.6788299742543));
#144291=CARTESIAN_POINT('Ctrl Pts',(90.3803286655751,-4.80462133586623,
55.7245351594281));
#144292=CARTESIAN_POINT('Ctrl Pts',(90.3109105403745,-4.99870563338229,
55.7728765859279));
#144293=CARTESIAN_POINT('Ctrl Pts',(90.2371438374155,-5.19016628571155,
55.8236299825407));
#144294=CARTESIAN_POINT('Ctrl Pts',(90.1616401667213,-5.38613521836696,
55.8755784578114));
#144295=CARTESIAN_POINT('Ctrl Pts',(90.0815807831541,-5.57935587985819,
55.9300541196797));
#144296=CARTESIAN_POINT('Ctrl Pts',(89.9969412499602,-5.76983317571853,
55.9868500877407));
#144297=CARTESIAN_POINT('Ctrl Pts',(89.9114467241532,-5.96223459231502,
56.0442197845465));
#144298=CARTESIAN_POINT('Ctrl Pts',(89.8212790150361,-6.15183730756892,
56.1039572727477));
#144299=CARTESIAN_POINT('Ctrl Pts',(89.7263703623101,-6.33863102978564,
56.1658780736405));
#144300=CARTESIAN_POINT('Ctrl Pts',(89.6305117548475,-6.52729439798418,
56.228418648984));
#144301=CARTESIAN_POINT('Ctrl Pts',(89.5298167828039,-6.71309263142337,
56.2931868387061));
#144302=CARTESIAN_POINT('Ctrl Pts',(89.424172972098,-6.89599393591638,56.3600160628481));
#144303=CARTESIAN_POINT('Ctrl Pts',(89.372389864718,-6.98564611551143,56.3927735416511));
#144304=CARTESIAN_POINT('Ctrl Pts',(89.3194170895394,-7.07460191252195,
56.4260265319146));
#144305=CARTESIAN_POINT('Ctrl Pts',(89.265237764927,-7.16285534378127,56.4597570269004));
#144306=CARTESIAN_POINT('Ctrl Pts',(89.1514748157839,-7.3481653431933,56.5305825791401));
#144307=CARTESIAN_POINT('Ctrl Pts',(89.0324076176265,-7.53045736360164,
56.6035308814627));
#144308=CARTESIAN_POINT('Ctrl Pts',(88.9081095276437,-7.70971421697662,
56.6784254559144));
#144309=CARTESIAN_POINT('Ctrl Pts',(88.7848087492422,-7.88753279454283,
56.7527191102194));
#144310=CARTESIAN_POINT('Ctrl Pts',(88.6563608772338,-8.06236500249708,
56.8289279758922));
#144311=CARTESIAN_POINT('Ctrl Pts',(88.5227985537957,-8.23420622355589,
56.9069108044424));
#144312=CARTESIAN_POINT('Ctrl Pts',(88.3916483918356,-8.40294395881794,
56.983485247977));
#144313=CARTESIAN_POINT('Ctrl Pts',(88.2555670078433,-8.56879807427274,
57.0617702627864));
#144314=CARTESIAN_POINT('Ctrl Pts',(88.1145450617424,-8.73177155843689,
57.141660937297));
#144315=CARTESIAN_POINT('Ctrl Pts',(87.9754900721468,-8.89247190878235,
57.2204373066495));
#144316=CARTESIAN_POINT('Ctrl Pts',(87.8316316013172,-9.05037172662669,
57.3007749486453));
#144317=CARTESIAN_POINT('Ctrl Pts',(87.6829183415991,-9.20547662654759,
57.3826001342298));
#144318=CARTESIAN_POINT('Ctrl Pts',(87.537851788522,-9.35677808574178,57.4624188245747));
#144319=CARTESIAN_POINT('Ctrl Pts',(87.3881657871141,-9.50542030776213,
57.5436531350847));
#144320=CARTESIAN_POINT('Ctrl Pts',(87.2337694243479,-9.65140681675671,
57.6262586182279));
#144321=CARTESIAN_POINT('Ctrl Pts',(87.1773368748085,-9.70476552776076,
57.6564512855692));
#144322=CARTESIAN_POINT('Ctrl Pts',(87.1202746136925,-9.75776941491483,
57.6868273584235));
#144323=CARTESIAN_POINT('Ctrl Pts',(87.0625766316463,-9.81041847342618,
57.7173854406918));
#144324=CARTESIAN_POINT('Origin',(91.9461506873691,0.0433429899084442,83.08714534325));
#144325=CARTESIAN_POINT('Origin',(91.5481555916691,0.0433429899084342,83.15732261681));
#144326=CARTESIAN_POINT('',(90.9924243507979,-11.2698537367303,57.6400054152702));
#144327=CARTESIAN_POINT('Ctrl Pts',(90.9924243507979,-11.2698537367303,
57.6400054152702));
#144328=CARTESIAN_POINT('Ctrl Pts',(91.0087196669506,-11.4929559013193,
57.7372219051933));
#144329=CARTESIAN_POINT('Ctrl Pts',(91.0264213003634,-11.6946801922847,
57.8273475410391));
#144330=CARTESIAN_POINT('Ctrl Pts',(91.0413458950691,-11.874941516,57.91633991463));
#144331=CARTESIAN_POINT('',(90.9047353709724,-10.0689627465674,57.1426963510668));
#144332=CARTESIAN_POINT('Ctrl Pts',(90.9045946917496,-10.0692831548029,
57.1418989990502));
#144333=CARTESIAN_POINT('Ctrl Pts',(90.9324261720231,-10.4675541238281,
57.2966628248043));
#144334=CARTESIAN_POINT('Ctrl Pts',(90.9607405811956,-10.8632766047505,
57.4621592417098));
#144335=CARTESIAN_POINT('Ctrl Pts',(90.9923722612255,-11.2699867077158,
57.6397093617342));
#144336=CARTESIAN_POINT('Ctrl Pts',(90.6242620415567,-4.02100038809876,
55.5520804830879));
#144337=CARTESIAN_POINT('Ctrl Pts',(90.6508298361238,-5.05591292129145,
55.7027332878991));
#144338=CARTESIAN_POINT('Ctrl Pts',(90.6876273743442,-6.08235086745013,
55.9118120415735));
#144339=CARTESIAN_POINT('Ctrl Pts',(90.7811137180524,-8.10404684266629,
56.4431103566449));
#144340=CARTESIAN_POINT('Ctrl Pts',(90.8376673001883,-9.09977064310684,
56.7650116874898));
#144341=CARTESIAN_POINT('Ctrl Pts',(90.9047434407505,-10.0689443669993,
57.1427420895467));
#144342=CARTESIAN_POINT('Ctrl Pts',(90.7138133970691,-10.19657068826,57.22715772731));
#144343=CARTESIAN_POINT('Ctrl Pts',(90.6626401866691,-9.35597025367699,
56.89396444657));
#144344=CARTESIAN_POINT('Ctrl Pts',(90.5763427137691,-7.68274033475999,
56.32754975961));
#144345=CARTESIAN_POINT('Ctrl Pts',(90.4541100393691,-4.24096410950499,
55.51544965917));
#144346=CARTESIAN_POINT('Ctrl Pts',(90.4199971140691,-1.61565261237899,
55.278532208));
#144347=CARTESIAN_POINT('Ctrl Pts',(90.4235408013691,0.151366721048514,
55.2878082705));
#144348=CARTESIAN_POINT('Ctrl Pts',(92.7962304970691,-10.33573356652,56.91274505515));
#144349=CARTESIAN_POINT('Ctrl Pts',(92.6626615303691,-9.48934028449099,
56.58708866282));
#144350=CARTESIAN_POINT('Ctrl Pts',(92.4384562628691,-7.79709517031399,
56.02944513539));
#144351=CARTESIAN_POINT('Ctrl Pts',(92.1038555437691,-4.30231560357699,
55.22999031531));
#144352=CARTESIAN_POINT('Ctrl Pts',(91.9893535601691,-1.63094673070299,
55.00159014612));
#144353=CARTESIAN_POINT('Ctrl Pts',(91.9738408428691,0.152837241252914,
55.0144585082));
#144354=CARTESIAN_POINT('Ctrl Pts',(95.7917187514691,-10.46442002935,56.51480537428));
#144355=CARTESIAN_POINT('Ctrl Pts',(95.5385368179691,-9.61788303082499,
56.19345931582));
#144356=CARTESIAN_POINT('Ctrl Pts',(95.1142808849691,-7.90799621978299,
55.63550595397));
#144357=CARTESIAN_POINT('Ctrl Pts',(94.4716188046691,-4.36724739891599,
54.83183905851));
#144358=CARTESIAN_POINT('Ctrl Pts',(94.2410150211691,-1.65095915302099,
54.60377902895));
#144359=CARTESIAN_POINT('Ctrl Pts',(94.1980369484691,0.154734101969314,
54.62230769129));
#144360=CARTESIAN_POINT('Ctrl Pts',(98.8683031516691,-10.53264157621,56.06075913389));
#144361=CARTESIAN_POINT('Ctrl Pts',(98.4877770766691,-9.70318322055799,
55.75728931457));
#144362=CARTESIAN_POINT('Ctrl Pts',(97.8443279361691,-7.98735677313499,
55.21668635057));
#144363=CARTESIAN_POINT('Ctrl Pts',(96.8545601533691,-4.42828578380799,
54.43258140482));
#144364=CARTESIAN_POINT('Ctrl Pts',(96.4917933988691,-1.67262404030799,
54.20606631111));
#144365=CARTESIAN_POINT('Ctrl Pts',(96.4222845185691,0.156770965735314,
54.23015027228));
#144366=CARTESIAN_POINT('Ctrl Pts',(99.8158998763691,-10.54389419866,55.88918321301));
#144367=CARTESIAN_POINT('Ctrl Pts',(99.3961224694691,-9.72294815639999,
55.59736775867));
#144368=CARTESIAN_POINT('Ctrl Pts',(98.6828965672691,-8.00820666453199,
55.07186546666));
#144369=CARTESIAN_POINT('Ctrl Pts',(97.5798863617691,-4.44890047093699,
54.30829590648));
#144370=CARTESIAN_POINT('Ctrl Pts',(97.1727004419691,-1.68039152780799,
54.0858613594));
#144371=CARTESIAN_POINT('Ctrl Pts',(97.0962919792691,0.157498942840914,
54.11131090037));
#144372=CARTESIAN_POINT('',(96.9599167740691,3.35717732455102E-13,54.13484467945));
#144373=CARTESIAN_POINT('',(91.1670701073691,2.7354895961722E-14,55.15627904919));
#144374=CARTESIAN_POINT('',(96.602194994137,-10.3347552344798,56.3300847780142));
#144375=CARTESIAN_POINT('Ctrl Pts',(90.9045946917494,-10.0692831548015,
57.1418989990485));
#144376=CARTESIAN_POINT('Ctrl Pts',(92.790213969345,-10.1923684393204,56.8585600051375));
#144377=CARTESIAN_POINT('Ctrl Pts',(94.6808936658549,-10.2756779228702,
56.6037222733635));
#144378=CARTESIAN_POINT('Ctrl Pts',(96.602194994137,-10.3347552344798,56.3300847780142));
#144379=CARTESIAN_POINT('Ctrl Pts',(96.9599167578601,6.36803545775495E-13,
54.134844587524));
#144380=CARTESIAN_POINT('Ctrl Pts',(96.9599171426822,-0.277060945827445,
54.134843612205));
#144381=CARTESIAN_POINT('Ctrl Pts',(96.9591759725721,-0.56015552509148,
54.1397203553601));
#144382=CARTESIAN_POINT('Ctrl Pts',(96.9575927400265,-0.849076263937013,
54.1499931425902));
#144383=CARTESIAN_POINT('Ctrl Pts',(96.9566606021444,-1.01918012288742,
54.1560413091462));
#144384=CARTESIAN_POINT('Ctrl Pts',(96.9554366094299,-1.19130261050792,
54.1639598075232));
#144385=CARTESIAN_POINT('Ctrl Pts',(96.9539006071702,-1.36539298195192,
54.1738529901787));
#144386=CARTESIAN_POINT('Ctrl Pts',(96.9511742972054,-1.67439273208784,
54.1914127836539));
#144387=CARTESIAN_POINT('Ctrl Pts',(96.9474649896664,-1.98959457399915,
54.2151936749478));
#144388=CARTESIAN_POINT('Ctrl Pts',(96.9426532817427,-2.31074252617866,
54.24581600169));
#144389=CARTESIAN_POINT('Ctrl Pts',(96.9404448505482,-2.45813990916418,
54.2598707412332));
#144390=CARTESIAN_POINT('Ctrl Pts',(96.9380042152572,-2.60678916580932,
54.2753665899201));
#144391=CARTESIAN_POINT('Ctrl Pts',(96.9353199592136,-2.75666185664168,
54.2923630781649));
#144392=CARTESIAN_POINT('Ctrl Pts',(96.9296516014349,-3.07314881581515,
54.3282546528831));
#144393=CARTESIAN_POINT('Ctrl Pts',(96.9228968211612,-3.39509477480875,
54.3708380894919));
#144394=CARTESIAN_POINT('Ctrl Pts',(96.9149435292017,-3.72219497430077,
54.4206994698898));
#144395=CARTESIAN_POINT('Ctrl Pts',(96.9125976699976,-3.81867464807259,
54.4354063081065));
#144396=CARTESIAN_POINT('Ctrl Pts',(96.9101475494493,-3.91560238986618,
54.4507462954679));
#144397=CARTESIAN_POINT('Ctrl Pts',(96.9075903110946,-4.01296950428391,
54.4667344125127));
#144398=CARTESIAN_POINT('Ctrl Pts',(96.8994999337026,-4.32101145890927,
54.5173162835551));
#144399=CARTESIAN_POINT('Ctrl Pts',(96.8903373787788,-4.6334550620318,54.574385330324));
#144400=CARTESIAN_POINT('Ctrl Pts',(96.8800083495169,-4.94995790029281,
54.6384369908349));
#144401=CARTESIAN_POINT('Ctrl Pts',(96.8776910512548,-5.02096471598414,
54.6528068602415));
#144402=CARTESIAN_POINT('Ctrl Pts',(96.8753150437641,-5.09217563446697,
54.6675281773576));
#144403=CARTESIAN_POINT('Ctrl Pts',(96.8728792659521,-5.16358642425807,
54.6826065310305));
#144404=CARTESIAN_POINT('Ctrl Pts',(96.8630108022917,-5.45290459628258,
54.7436959229071));
#144405=CARTESIAN_POINT('Ctrl Pts',(96.8521608407434,-5.74550708452013,
54.8106478289228));
#144406=CARTESIAN_POINT('Ctrl Pts',(96.8402839376195,-6.04105560289267,
54.8837055006886));
#144407=CARTESIAN_POINT('Ctrl Pts',(96.8378379451746,-6.10192243286345,
54.8987513852354));
#144408=CARTESIAN_POINT('Ctrl Pts',(96.8353484135449,-6.16291405982723,
54.9140561536033));
#144409=CARTESIAN_POINT('Ctrl Pts',(96.8328149727655,-6.22402728514366,
54.9296217986156));
#144410=CARTESIAN_POINT('Ctrl Pts',(96.81901609602,-6.55689232407346,55.0144031042355));
#144411=CARTESIAN_POINT('Ctrl Pts',(96.8039139414176,-6.89336720567203,
55.1069268719829));
#144412=CARTESIAN_POINT('Ctrl Pts',(96.7874496467217,-7.23312623612149,
55.2075115883376));
#144413=CARTESIAN_POINT('Ctrl Pts',(96.786035072685,-7.26231754446941,55.2161535940153));
#144414=CARTESIAN_POINT('Ctrl Pts',(96.784610448577,-7.29153307619233,55.2248550796922));
#144415=CARTESIAN_POINT('Ctrl Pts',(96.7831757399513,-7.32077261352518,
55.2336162332069));
#144416=CARTESIAN_POINT('Ctrl Pts',(96.7803261873095,-7.37884684501412,
55.2510172355393));
#144417=CARTESIAN_POINT('Ctrl Pts',(96.7774368533627,-7.43701577347718,
55.2686536150049));
#144418=CARTESIAN_POINT('Ctrl Pts',(96.7745072371656,-7.49527846640879,
55.2865280332663));
#144419=CARTESIAN_POINT('Ctrl Pts',(96.7590394015428,-7.8028947876485,55.3809016798179));
#144420=CARTESIAN_POINT('Ctrl Pts',(96.742448658216,-8.11312489114606,55.4819107935465));
#144421=CARTESIAN_POINT('Ctrl Pts',(96.7246611171326,-8.42583162785647,
55.5899487265824));
#144422=CARTESIAN_POINT('Ctrl Pts',(96.7067169276187,-8.74129225951466,
55.6989381105564));
#144423=CARTESIAN_POINT('Ctrl Pts',(96.6875554159446,-9.05927574423186,
55.8150773272328));
#144424=CARTESIAN_POINT('Ctrl Pts',(96.6670513754222,-9.37946266624096,
55.9390253826691));
#144425=CARTESIAN_POINT('Ctrl Pts',(96.6645609067954,-9.41835331723715,
55.9540804028285));
#144426=CARTESIAN_POINT('Ctrl Pts',(96.662050621889,-9.45727644122763,55.9692506796209));
#144427=CARTESIAN_POINT('Ctrl Pts',(96.6595202881283,-9.49623143702847,
55.9845374374691));
#144428=CARTESIAN_POINT('Ctrl Pts',(96.6414623973248,-9.7742362881439,56.0936323751597));
#144429=CARTESIAN_POINT('Ctrl Pts',(96.6223838211085,-10.0538674463473,
56.2086575718103));
#144430=CARTESIAN_POINT('Ctrl Pts',(96.6021951000051,-10.3347534605419,
56.3300838067384));
#144431=CARTESIAN_POINT('Ctrl Pts',(96.6696289028691,0.160268731304714,
54.21733794602));
#144432=CARTESIAN_POINT('Ctrl Pts',(96.670308400869,-0.346230314545186,
54.21384224945));
#144433=CARTESIAN_POINT('Ctrl Pts',(96.6654264806691,-1.31612458106799,
54.23895742649));
#144434=CARTESIAN_POINT('Ctrl Pts',(96.6422624601691,-2.70059882064599,
54.35812538629));
#144435=CARTESIAN_POINT('Ctrl Pts',(96.608028791469,-3.95977777602399,54.53424146526));
#144436=CARTESIAN_POINT('Ctrl Pts',(96.5658452623691,-5.10903817364999,
54.75125582648));
#144437=CARTESIAN_POINT('Ctrl Pts',(96.5158510367691,-6.20578639454099,
55.00845253674));
#144438=CARTESIAN_POINT('Ctrl Pts',(96.4572022184691,-7.28729934218798,
55.31017304474));
#144439=CARTESIAN_POINT('Ctrl Pts',(96.3889045551691,-8.37105043441599,
55.6615323096));
#144440=CARTESIAN_POINT('Ctrl Pts',(96.3136363712691,-9.41723706373098,
56.04875161508));
#144441=CARTESIAN_POINT('Ctrl Pts',(96.258897993869,-10.09227685666,56.33035474907));
#144442=CARTESIAN_POINT('Ctrl Pts',(96.2311574648692,-10.41546419882,56.47306668683));
#144443=CARTESIAN_POINT('Ctrl Pts',(98.1128935683692,0.166136603669114,
53.6477629649701));
#144444=CARTESIAN_POINT('Ctrl Pts',(98.1135980223691,-0.358956357238386,
53.64413888123));
#144445=CARTESIAN_POINT('Ctrl Pts',(98.108536711269,-1.36355315035499,53.67017693973));
#144446=CARTESIAN_POINT('Ctrl Pts',(98.0845692883691,-2.79580825471999,
53.7934780261801));
#144447=CARTESIAN_POINT('Ctrl Pts',(98.0491810976691,-4.09738494468499,
53.97553357625));
#144448=CARTESIAN_POINT('Ctrl Pts',(98.0055962418691,-5.284787566009,54.1997571019299));
#144449=CARTESIAN_POINT('Ctrl Pts',(97.9539701807691,-6.41729306682898,
54.4653488368801));
#144450=CARTESIAN_POINT('Ctrl Pts',(97.893484104969,-7.53261697524899,54.7765211682));
#144451=CARTESIAN_POINT('Ctrl Pts',(97.8231219679691,-8.64911747269499,
55.1385011759801));
#144452=CARTESIAN_POINT('Ctrl Pts',(97.7455474807691,-9.72739355825898,
55.53758532437));
#144453=CARTESIAN_POINT('Ctrl Pts',(97.6890592547692,-10.42404175222,55.82819060393));
#144454=CARTESIAN_POINT('Ctrl Pts',(97.660409458769,-10.75782222324,55.97558029138));
#144455=CARTESIAN_POINT('Ctrl Pts',(99.2004280885691,0.159957130493114,
54.75442165969));
#144456=CARTESIAN_POINT('Ctrl Pts',(99.2011062613691,-0.345554525266686,
54.75093278085));
#144457=CARTESIAN_POINT('Ctrl Pts',(99.1962338672691,-1.31360598833699,
54.7759989502401));
#144458=CARTESIAN_POINT('Ctrl Pts',(99.1731125097691,-2.69554292728499,
54.89494742919));
#144459=CARTESIAN_POINT('Ctrl Pts',(99.1389401494691,-3.95247044164899,
55.0707481052501));
#144460=CARTESIAN_POINT('Ctrl Pts',(99.0968310347691,-5.09970537806498,
55.28737963921));
#144461=CARTESIAN_POINT('Ctrl Pts',(99.0469234643691,-6.19455478508299,
55.54413054964));
#144462=CARTESIAN_POINT('Ctrl Pts',(98.9883722097691,-7.27427227397399,
55.8453491387801));
#144463=CARTESIAN_POINT('Ctrl Pts',(98.9201841758691,-8.35628427908298,
56.1961444118));
#144464=CARTESIAN_POINT('Ctrl Pts',(98.8450384632691,-9.40076686645699,
56.58273366018));
#144465=CARTESIAN_POINT('Ctrl Pts',(98.7903930078691,-10.07465919146,56.8638587544801));
#144466=CARTESIAN_POINT('Ctrl Pts',(98.7627007634691,-10.39728400817,57.00632229035));
#144467=CARTESIAN_POINT('Ctrl Pts',(98.6057368794691,0.149267584137414,
56.18749216758));
#144468=CARTESIAN_POINT('Ctrl Pts',(98.6063695895691,-0.322371399450786,
56.18423717261));
#144469=CARTESIAN_POINT('Ctrl Pts',(98.6018239931692,-1.22720501392999,
56.20762212203));
#144470=CARTESIAN_POINT('Ctrl Pts',(98.5801661998691,-2.52209919915899,
56.31904125369));
#144471=CARTESIAN_POINT('Ctrl Pts',(98.5480970407691,-3.70179044778499,
56.48402195143));
#144472=CARTESIAN_POINT('Ctrl Pts',(98.5085407331691,-4.77954141403098,
56.68752049734));
#144473=CARTESIAN_POINT('Ctrl Pts',(98.461605889769,-5.80925152052899,56.9289781294));
#144474=CARTESIAN_POINT('Ctrl Pts',(98.4064015806692,-6.82737533285799,
57.21297826229));
#144475=CARTESIAN_POINT('Ctrl Pts',(98.3419744134691,-7.84972750498899,
57.54442564961));
#144476=CARTESIAN_POINT('Ctrl Pts',(98.2710301106691,-8.835752493285,57.90940062617));
#144477=CARTESIAN_POINT('Ctrl Pts',(98.2195723673692,-9.47028063478298,
58.17412644551));
#144478=CARTESIAN_POINT('Ctrl Pts',(98.1935365413691,-9.77360787053599,
58.30806849027));
#144479=CARTESIAN_POINT('Origin',(96.8148132210691,-9.75846282474099,57.69855282308));
#144480=CARTESIAN_POINT('Origin',(97.2203890703691,1.08526369006055E-7,
55.61205637088));
#144481=CARTESIAN_POINT('Ctrl Pts',(96.2311597944691,10.41560961071,56.47305462378));
#144482=CARTESIAN_POINT('Ctrl Pts',(96.2425456644691,10.28294688966,56.41447969266));
#144483=CARTESIAN_POINT('Ctrl Pts',(96.2665237450691,9.99701257139901,56.29112377728));
#144484=CARTESIAN_POINT('Ctrl Pts',(96.3029830043691,9.53999273052302,56.10355808445));
#144485=CARTESIAN_POINT('Ctrl Pts',(96.341615819269,9.02742880050502,55.90481047335));
#144486=CARTESIAN_POINT('Ctrl Pts',(96.3817550230691,8.45983449326603,55.69831320138));
#144487=CARTESIAN_POINT('Ctrl Pts',(96.4230873061691,7.83124748153802,55.48567809967));
#144488=CARTESIAN_POINT('Ctrl Pts',(96.465123940069,7.13529453258901,55.26941944543));
#144489=CARTESIAN_POINT('Ctrl Pts',(96.5071095016691,6.36519388110002,55.05342353344));
#144490=CARTESIAN_POINT('Ctrl Pts',(96.5479785345691,5.51425300235401,54.84317163521));
#144491=CARTESIAN_POINT('Ctrl Pts',(96.5862074329692,4.57747980015701,54.64650198403));
#144492=CARTESIAN_POINT('Ctrl Pts',(96.6201253331691,3.54799753503601,54.47201038533));
#144493=CARTESIAN_POINT('Ctrl Pts',(96.6478026904691,2.41338163155501,54.32962343617));
#144494=CARTESIAN_POINT('Ctrl Pts',(96.6664221526691,1.16626940880601,54.23383508485));
#144495=CARTESIAN_POINT('Ctrl Pts',(96.6702378408692,0.293677663957814,
54.21420516889));
#144496=CARTESIAN_POINT('Ctrl Pts',(96.6696289293692,-0.160237368166786,
54.21733773116));
#144497=CARTESIAN_POINT('Ctrl Pts',(97.6604144928692,10.75793837742,55.97555520529));
#144498=CARTESIAN_POINT('Ctrl Pts',(97.6721750711691,10.62090973503,55.9150525767801));
#144499=CARTESIAN_POINT('Ctrl Pts',(97.6969333406691,10.32566953004,55.78768295773));
#144500=CARTESIAN_POINT('Ctrl Pts',(97.7345529493691,9.854100032395,55.59414781434));
#144501=CARTESIAN_POINT('Ctrl Pts',(97.7743875562691,9.32558631739701,55.38921755005));
#144502=CARTESIAN_POINT('Ctrl Pts',(97.815752058769,8.74066062569102,55.17641669437));
#144503=CARTESIAN_POINT('Ctrl Pts',(97.8583357654691,8.09304235429201,54.95734360863));
#144504=CARTESIAN_POINT('Ctrl Pts',(97.9016574024691,7.37582286052101,54.7344742188501));
#144505=CARTESIAN_POINT('Ctrl Pts',(97.9449558647691,6.58165855423801,54.5117240523701));
#144506=CARTESIAN_POINT('Ctrl Pts',(97.9871389566692,5.70338735783601,54.2947119403101));
#144507=CARTESIAN_POINT('Ctrl Pts',(98.0266336670691,4.73562596871401,54.09153028349));
#144508=CARTESIAN_POINT('Ctrl Pts',(98.0616832237691,3.67181175629301,53.91121684539));
#144509=CARTESIAN_POINT('Ctrl Pts',(98.0903010919691,2.49871342897601,53.76399141175));
#144510=CARTESIAN_POINT('Ctrl Pts',(98.109568905869,1.20836539597901,53.66486759685));
#144511=CARTESIAN_POINT('Ctrl Pts',(98.1135250776691,0.304474695687914,
53.64451495891));
#144512=CARTESIAN_POINT('Ctrl Pts',(98.1128937887691,-0.166104368673886,
53.64776264251));
#144513=CARTESIAN_POINT('Ctrl Pts',(98.7627032108691,10.39743093721,57.0063110524));
#144514=CARTESIAN_POINT('Ctrl Pts',(98.7740691828691,10.26500005954,56.9478384877199));
#144515=CARTESIAN_POINT('Ctrl Pts',(98.7980058330692,9.97955991148701,56.82469571192));
#144516=CARTESIAN_POINT('Ctrl Pts',(98.8344034743691,9.52331270056701,56.63744701464));
#144517=CARTESIAN_POINT('Ctrl Pts',(98.8729724705691,9.01159575146801,56.43902772077));
#144518=CARTESIAN_POINT('Ctrl Pts',(98.9130466074691,8.44492179218101,56.2328651878));
#144519=CARTESIAN_POINT('Ctrl Pts',(98.9543124361691,7.81734539682401,56.02057196215));
#144520=CARTESIAN_POINT('Ctrl Pts',(98.9962808325691,7.12252176452102,55.80466435759));
#144521=CARTESIAN_POINT('Ctrl Pts',(99.0381966752691,6.35369896451901,55.58902711656));
#144522=CARTESIAN_POINT('Ctrl Pts',(99.0789959277691,5.50420940675301,55.3791342057501));
#144523=CARTESIAN_POINT('Ctrl Pts',(99.1171576077691,4.56908176925101,55.1828103613901));
#144524=CARTESIAN_POINT('Ctrl Pts',(99.1510154135691,3.54142263242401,55.00862791964));
#144525=CARTESIAN_POINT('Ctrl Pts',(99.1786428269691,2.40885025985901,54.86649790837));
#144526=CARTESIAN_POINT('Ctrl Pts',(99.1972278598691,1.16403398695201,54.77088668006));
#144527=CARTESIAN_POINT('Ctrl Pts',(99.2010360879692,0.293104309528914,
54.75129514278));
#144528=CARTESIAN_POINT('Ctrl Pts',(99.2004283647692,-0.159925813027386,
54.75442159177));
#144529=CARTESIAN_POINT('Ctrl Pts',(98.1935340747691,9.77380813262502,58.30808090183));
#144530=CARTESIAN_POINT('Ctrl Pts',(98.2042174378691,9.64933068563601,58.25312003751));
#144531=CARTESIAN_POINT('Ctrl Pts',(98.2267328124692,9.38084313911702,58.13728905489));
#144532=CARTESIAN_POINT('Ctrl Pts',(98.261016636769,8.95110114377703,57.96091494911));
#144533=CARTESIAN_POINT('Ctrl Pts',(98.297396319569,8.468440034004,57.77375863954));
#144534=CARTESIAN_POINT('Ctrl Pts',(98.335238320969,7.93333878387603,57.57907939087));
#144535=CARTESIAN_POINT('Ctrl Pts',(98.3742244223691,7.34043177270501,57.37851428755));
#144536=CARTESIAN_POINT('Ctrl Pts',(98.4138519189691,6.68434955980702,57.17464950802));
#144537=CARTESIAN_POINT('Ctrl Pts',(98.453376041069,5.95936369479301,56.97131654153));
#144538=CARTESIAN_POINT('Ctrl Pts',(98.4917814626692,5.15966197551602,56.77373876143));
#144539=CARTESIAN_POINT('Ctrl Pts',(98.5276372037691,4.28098574355801,56.58927788512));
#144540=CARTESIAN_POINT('Ctrl Pts',(98.5594334625691,3.31586936487401,56.42570113055));
#144541=CARTESIAN_POINT('Ctrl Pts',(98.585347540569,2.25340070375301,56.29238542167));
#144542=CARTESIAN_POINT('Ctrl Pts',(98.6027514664691,1.08734742089201,56.2028504316));
#144543=CARTESIAN_POINT('Ctrl Pts',(98.6063037745691,0.273435278283314,
56.18457548221));
#144544=CARTESIAN_POINT('Ctrl Pts',(98.605736816469,-0.149237855524086,
56.18749221385));
#144545=CARTESIAN_POINT('',(96.6024042671263,10.3348601566812,56.3300319325398));
#144546=CARTESIAN_POINT('Origin',(96.8148145050691,9.75862245206801,57.69854621723));
#144547=CARTESIAN_POINT('Ctrl Pts',(96.6024043659547,10.3348592664372,56.3300312921791));
#144548=CARTESIAN_POINT('Ctrl Pts',(96.6084219835484,10.2511412529389,56.2938461676181));
#144549=CARTESIAN_POINT('Ctrl Pts',(96.6144624575879,10.1658560418771,56.2575059362147));
#144550=CARTESIAN_POINT('Ctrl Pts',(96.6205180308355,10.0789934768286,56.221050733991));
#144551=CARTESIAN_POINT('Ctrl Pts',(96.6309956957853,9.9286993897054,56.157974064127));
#144552=CARTESIAN_POINT('Ctrl Pts',(96.6415186109792,9.77368272111521,56.0945529558029));
#144553=CARTESIAN_POINT('Ctrl Pts',(96.6520454633506,9.61389022100475,56.0310011592772));
#144554=CARTESIAN_POINT('Ctrl Pts',(96.6630026090245,9.44756607780156,55.9648516334932));
#144555=CARTESIAN_POINT('Ctrl Pts',(96.6739640081778,9.27606786512193,55.8985605793858));
#144556=CARTESIAN_POINT('Ctrl Pts',(96.6848822592359,9.09932968087413,55.8323732675094));
#144557=CARTESIAN_POINT('Ctrl Pts',(96.6930210020023,8.96758453131361,55.783035557386));
#144558=CARTESIAN_POINT('Ctrl Pts',(96.7011357766724,8.83292802143723,55.7337554546973));
#144559=CARTESIAN_POINT('Ctrl Pts',(96.7092052910968,8.69532473815957,55.6846430982255));
#144560=CARTESIAN_POINT('Ctrl Pts',(96.7124201954733,8.64050342248117,55.6650766755812));
#144561=CARTESIAN_POINT('Ctrl Pts',(96.7156279109387,8.58521438368289,55.6455369040242));
#144562=CARTESIAN_POINT('Ctrl Pts',(96.7188270717432,8.52945538252802,55.6260308482034));
#144563=CARTESIAN_POINT('Ctrl Pts',(96.7305350870968,8.32539335454058,55.554644251844));
#144564=CARTESIAN_POINT('Ctrl Pts',(96.7421288191065,8.11503747979796,55.4837077123816));
#144565=CARTESIAN_POINT('Ctrl Pts',(96.7535336198707,7.89825013892825,55.413607184542));
#144566=CARTESIAN_POINT('Ctrl Pts',(96.7646799253056,7.68637638806486,55.3450955190947));
#144567=CARTESIAN_POINT('Ctrl Pts',(96.7756460513596,7.46835904462709,55.2773809341928));
#144568=CARTESIAN_POINT('Ctrl Pts',(96.7863456394669,7.24407857810092,55.210909559299));
#144569=CARTESIAN_POINT('Ctrl Pts',(96.7870529629367,7.22925194775016,55.2065153000944));
#144570=CARTESIAN_POINT('Ctrl Pts',(96.7877591190464,7.21439794543156,55.2021264870342));
#144571=CARTESIAN_POINT('Ctrl Pts',(96.7884640817421,7.19951653632829,55.1977432546116));
#144572=CARTESIAN_POINT('Ctrl Pts',(96.7918518676576,7.12800207396804,55.1766790860286));
#144573=CARTESIAN_POINT('Ctrl Pts',(96.7952120997352,7.05585467210436,55.1557437612974));
#144574=CARTESIAN_POINT('Ctrl Pts',(96.7985416990093,6.98307159402205,55.1349531713329));
#144575=CARTESIAN_POINT('Ctrl Pts',(96.8005529259795,6.93910735762018,55.122394724559));
#144576=CARTESIAN_POINT('Ctrl Pts',(96.8025529812833,6.89491116477672,55.1098890893669));
#144577=CARTESIAN_POINT('Ctrl Pts',(96.8045411626626,6.85048244849461,55.0974398546943));
#144578=CARTESIAN_POINT('Ctrl Pts',(96.8055352533523,6.82826809035355,55.091215237358));
#144579=CARTESIAN_POINT('Ctrl Pts',(96.8065263756882,6.80599560113382,55.0850047209203));
#144580=CARTESIAN_POINT('Ctrl Pts',(96.8075144421586,6.78366490678631,55.078808758257));
#144581=CARTESIAN_POINT('Ctrl Pts',(96.8083790003203,6.76412554923223,55.0733872909267));
#144582=CARTESIAN_POINT('Ctrl Pts',(96.8092412188429,6.74454162836447,55.0679769663772));
#144583=CARTESIAN_POINT('Ctrl Pts',(96.8101010386112,6.72491309569946,55.06257809058));
#144584=CARTESIAN_POINT('Ctrl Pts',(96.8102238700067,6.72210901960446,55.0618068226089));
#144585=CARTESIAN_POINT('Ctrl Pts',(96.8102881861003,6.72064067545679,55.0614029734022));
#144586=CARTESIAN_POINT('Ctrl Pts',(96.8104693857455,6.71649813595896,55.0602649885249));
#144587=CARTESIAN_POINT('Ctrl Pts',(96.8146869362856,6.62007758461498,55.0337775816222));
#144588=CARTESIAN_POINT('Ctrl Pts',(96.8188309109694,6.52337416078276,55.0077816168893));
#144589=CARTESIAN_POINT('Ctrl Pts',(96.8228991985691,6.42639016931002,54.9822874190042));
#144590=CARTESIAN_POINT('Ctrl Pts',(96.8347505673355,6.14386514638222,54.9080200194814));
#144591=CARTESIAN_POINT('Ctrl Pts',(96.8459597618218,5.85895886716469,54.8380099622278));
#144592=CARTESIAN_POINT('Ctrl Pts',(96.8564654327478,5.57175606730921,54.772560755726));
#144593=CARTESIAN_POINT('Ctrl Pts',(96.8678570598177,5.26033310228057,54.7015921371824));
#144594=CARTESIAN_POINT('Ctrl Pts',(96.8784214633711,4.9462092729796,54.6359862154016));
#144595=CARTESIAN_POINT('Ctrl Pts',(96.8880960192383,4.62968227709694,54.5760520609986));
#144596=CARTESIAN_POINT('Ctrl Pts',(96.8985101039455,4.2889597682312,54.5115365039669));
#144597=CARTESIAN_POINT('Ctrl Pts',(96.9078930631961,3.9454530461053,54.453593113036));
#144598=CARTESIAN_POINT('Ctrl Pts',(96.916182680695,3.59934808772723,54.4025288115359));
#144599=CARTESIAN_POINT('Ctrl Pts',(96.9251664910279,3.224259454056,54.3471882605979));
#144600=CARTESIAN_POINT('Ctrl Pts',(96.9328662348363,2.84611874664824,54.2999268110739));
#144601=CARTESIAN_POINT('Ctrl Pts',(96.9391924031706,2.465241900983,54.2611926479285));
#144602=CARTESIAN_POINT('Ctrl Pts',(96.9461055728112,2.04902372481488,54.2188643653793));
#144603=CARTESIAN_POINT('Ctrl Pts',(96.9513785461808,1.62953797927088,54.1867186023368));
#144604=CARTESIAN_POINT('Ctrl Pts',(96.9548785263097,1.20715853147687,54.1654288564663));
#144605=CARTESIAN_POINT('Ctrl Pts',(96.9581927427499,0.807197143619323,
54.1452690775045));
#144606=CARTESIAN_POINT('Ctrl Pts',(96.9599172393264,0.40464045421033,54.134843246294));
#144607=CARTESIAN_POINT('Ctrl Pts',(96.9599167505116,-6.53612581251083E-14,
54.134844545849));
#144608=CARTESIAN_POINT('Ctrl Pts',(99.8229747619691,10.54405187355,55.88748381909));
#144609=CARTESIAN_POINT('Ctrl Pts',(99.6011503882691,10.11099294518,55.73360189522));
#144610=CARTESIAN_POINT('Ctrl Pts',(99.2102368780691,9.25605213789501,55.45271235202));
#144611=CARTESIAN_POINT('Ctrl Pts',(98.7021511514691,7.94604321926101,55.08505245608));
#144612=CARTESIAN_POINT('Ctrl Pts',(98.2701917582691,6.66238207832301,54.78216749588));
#144613=CARTESIAN_POINT('Ctrl Pts',(97.7799388929691,4.91797092981301,54.44745221876));
#144614=CARTESIAN_POINT('Ctrl Pts',(97.3195994411691,2.63983322288901,54.16192812077));
#144615=CARTESIAN_POINT('Ctrl Pts',(97.1410285879691,0.789227954741114,
54.0973421985));
#144616=CARTESIAN_POINT('Ctrl Pts',(97.1017087564691,-0.155244189994386,
54.11034113544));
#144617=CARTESIAN_POINT('Ctrl Pts',(99.4111077309691,10.53918164393,55.96185987267));
#144618=CARTESIAN_POINT('Ctrl Pts',(99.1983162588691,10.10413395607,55.80530734332));
#144619=CARTESIAN_POINT('Ctrl Pts',(98.8236902496691,9.24752851307401,55.52032811987));
#144620=CARTESIAN_POINT('Ctrl Pts',(98.3374458072691,7.93709116282101,55.14813869173));
#144621=CARTESIAN_POINT('Ctrl Pts',(97.9244713730691,6.65312626074601,54.84160399721));
#144622=CARTESIAN_POINT('Ctrl Pts',(97.4562446747691,4.90972638740901,54.50320205192));
#144623=CARTESIAN_POINT('Ctrl Pts',(97.0170970717691,2.63464759459801,54.21479821838));
#144624=CARTESIAN_POINT('Ctrl Pts',(96.8467105044691,0.787641994762214,
54.14926657865));
#144625=CARTESIAN_POINT('Ctrl Pts',(96.8089517314691,-0.154932922945286,
54.1619595982));
#144626=CARTESIAN_POINT('Ctrl Pts',(98.4777090344691,10.52329010473,56.11845317377));
#144627=CARTESIAN_POINT('Ctrl Pts',(98.2852261383691,10.08453122649,55.95714161523));
#144628=CARTESIAN_POINT('Ctrl Pts',(97.9470076983691,9.22517756954501,55.6650077805));
#144629=CARTESIAN_POINT('Ctrl Pts',(97.5092800778691,7.91480618950201,55.28511132683));
#144630=CARTESIAN_POINT('Ctrl Pts',(97.1383378946691,6.63111996167601,54.97247109813));
#144631=CARTESIAN_POINT('Ctrl Pts',(96.7186546373691,4.89091160154701,54.62808485806));
#144632=CARTESIAN_POINT('Ctrl Pts',(96.3258627810691,2.62326937253201,54.33521804603));
#144633=CARTESIAN_POINT('Ctrl Pts',(96.1735151682691,0.784230533506414,
54.26805760886));
#144634=CARTESIAN_POINT('Ctrl Pts',(96.1394690336691,-0.154262148337386,
54.27999958306));
#144635=CARTESIAN_POINT('Ctrl Pts',(95.4083885479691,10.44883596239,56.56563465392));
#144636=CARTESIAN_POINT('Ctrl Pts',(95.2828062625691,10.00197988592,56.3957398526));
#144637=CARTESIAN_POINT('Ctrl Pts',(95.0630081160691,9.13858690468502,56.09214344177));
#144638=CARTESIAN_POINT('Ctrl Pts',(94.7806758719691,7.83336858220501,55.70203084944));
#144639=CARTESIAN_POINT('Ctrl Pts',(94.5431290615691,6.55548841998301,55.38187058097));
#144640=CARTESIAN_POINT('Ctrl Pts',(94.2760893890691,4.83002811735801,55.03105620878));
#144641=CARTESIAN_POINT('Ctrl Pts',(94.0284201829691,2.58855410828601,54.73379249893));
#144642=CARTESIAN_POINT('Ctrl Pts',(93.9343732761691,0.774119276983114,
54.66327669956));
#144643=CARTESIAN_POINT('Ctrl Pts',(93.9140860931691,-0.152268583664686,
54.67235913534));
#144644=CARTESIAN_POINT('Ctrl Pts',(92.8064875484691,10.33635977521,56.9112474595));
#144645=CARTESIAN_POINT('Ctrl Pts',(92.7357330084691,9.88956369225401,56.7393789277));
#144646=CARTESIAN_POINT('Ctrl Pts',(92.6117114470691,9.03084370884002,56.43423816251));
#144647=CARTESIAN_POINT('Ctrl Pts',(92.4529045945691,7.73795351776001,56.04452333574));
#144648=CARTESIAN_POINT('Ctrl Pts',(92.3202486007691,6.47365310299701,55.7253050736));
#144649=CARTESIAN_POINT('Ctrl Pts',(92.1720133995691,4.76915259221901,55.37615663976));
#144650=CARTESIAN_POINT('Ctrl Pts',(92.0369115993691,2.55748337778701,55.07951654561));
#144651=CARTESIAN_POINT('Ctrl Pts',(91.9894945383691,0.765968439024214,
55.00654446214));
#144652=CARTESIAN_POINT('Ctrl Pts',(91.9814512487691,-0.150644741938386,
55.01310502597));
#144653=CARTESIAN_POINT('Ctrl Pts',(90.7164576703691,10.19678286554,57.22677077382));
#144654=CARTESIAN_POINT('Ctrl Pts',(90.6893899738691,9.75304619127001,57.05089591696));
#144655=CARTESIAN_POINT('Ctrl Pts',(90.6417223165691,8.90227290514001,56.73991954444));
#144656=CARTESIAN_POINT('Ctrl Pts',(90.5814051064691,7.62527961729201,56.34394113065));
#144657=CARTESIAN_POINT('Ctrl Pts',(90.5323570494691,6.37927852091801,56.01957703094));
#144658=CARTESIAN_POINT('Ctrl Pts',(90.4788919205691,4.70104472127001,55.66451641314));
#144659=CARTESIAN_POINT('Ctrl Pts',(90.4337583071691,2.52566132230601,55.3604051064));
#144660=CARTESIAN_POINT('Ctrl Pts',(90.4237131106691,0.758799367497314,
55.28274489739));
#144661=CARTESIAN_POINT('Ctrl Pts',(90.4255048500691,-0.149192139117986,
55.28745041171));
#144662=CARTESIAN_POINT('Ctrl Pts',(96.6024042105574,10.3348592504771,56.3300313412501));
#144663=CARTESIAN_POINT('Ctrl Pts',(94.6805165943852,10.2762753587676,56.6036838964873));
#144664=CARTESIAN_POINT('Ctrl Pts',(92.790310713495,10.192372964693,56.8585465176481));
#144665=CARTESIAN_POINT('Ctrl Pts',(90.9047040108584,10.0692900874229,57.1418824909803));
#144666=CARTESIAN_POINT('Ctrl Pts',(97.4033426433691,11.67390399386,56.81447980514));
#144667=CARTESIAN_POINT('Ctrl Pts',(97.2044197352691,11.15857038581,56.59946163497));
#144668=CARTESIAN_POINT('Ctrl Pts',(97.0199546676691,10.69792038896,56.41485272246));
#144669=CARTESIAN_POINT('Ctrl Pts',(96.8505358648691,10.20340241203,56.23655459461));
#144670=CARTESIAN_POINT('Ctrl Pts',(95.1818404305691,11.63097278493,57.12775727934));
#144671=CARTESIAN_POINT('Ctrl Pts',(95.0391297258691,11.10781492551,56.90710660012));
#144672=CARTESIAN_POINT('Ctrl Pts',(94.9074321944691,10.63959524128,56.71574595965));
#144673=CARTESIAN_POINT('Ctrl Pts',(94.7862029432691,10.14192491651,56.53272828161));
#144674=CARTESIAN_POINT('Ctrl Pts',(93.0043471674691,11.54190049326,57.40548638152));
#144675=CARTESIAN_POINT('Ctrl Pts',(92.9159773486691,11.02450742992,57.18494785266));
#144676=CARTESIAN_POINT('Ctrl Pts',(92.8351915464691,10.54867530012,56.98933837901));
#144677=CARTESIAN_POINT('Ctrl Pts',(92.7597699884691,10.05314564258,56.80529830028));
#144678=CARTESIAN_POINT('Ctrl Pts',(90.8330907240691,11.394827307,57.7243208529));
#144679=CARTESIAN_POINT('Ctrl Pts',(90.7978936089691,10.8933807422,57.50281317575));
#144680=CARTESIAN_POINT('Ctrl Pts',(90.7679564434691,10.40883217466,57.29914644491));
#144681=CARTESIAN_POINT('Ctrl Pts',(90.7377901915691,9.91924603277401,57.11183124642));
#144682=CARTESIAN_POINT('',(96.5107425399285,11.5157870618668,56.8740840772352));
#144683=CARTESIAN_POINT('Ctrl Pts',(96.5107425395691,11.51578706178,56.87408407794));
#144684=CARTESIAN_POINT('Ctrl Pts',(94.6510436680464,11.468268482461,57.1317517447984));
#144685=CARTESIAN_POINT('Ctrl Pts',(92.819127139777,11.3889026395626,57.3718290827166));
#144686=CARTESIAN_POINT('Ctrl Pts',(90.9921937685691,11.26993034099,57.63983708294));
#144687=CARTESIAN_POINT('Ctrl Pts',(96.5107387539899,11.5157988299523,56.8740589380757));
#144688=CARTESIAN_POINT('Ctrl Pts',(96.5207205591766,11.392698487589,56.8149316120969));
#144689=CARTESIAN_POINT('Ctrl Pts',(96.5307034778743,11.2688057038616,56.7558085326091));
#144690=CARTESIAN_POINT('Ctrl Pts',(96.5406385265741,11.1438449346926,56.6969417202444));
#144691=CARTESIAN_POINT('Ctrl Pts',(96.5530657379208,10.9875383140187,56.6233084305987));
#144692=CARTESIAN_POINT('Ctrl Pts',(96.5654180277,10.8295608937585,56.5500762210146));
#144693=CARTESIAN_POINT('Ctrl Pts',(96.5775455007843,10.6697694503403,56.4780162762873));
#144694=CARTESIAN_POINT('Ctrl Pts',(96.58595630413,10.5589488038983,56.4280403233424));
#144695=CARTESIAN_POINT('Ctrl Pts',(96.5942589709957,10.4472556926979,56.3786282277779));
#144696=CARTESIAN_POINT('Ctrl Pts',(96.6024044181752,10.3348599160687,56.3300325143648));
#144697=CARTESIAN_POINT('Ctrl Pts',(96.1920310780691,11.59801716752,56.99776218657));
#144698=CARTESIAN_POINT('Ctrl Pts',(96.1943841679691,11.57301298649,56.98565664926));
#144699=CARTESIAN_POINT('Ctrl Pts',(96.2102167272692,11.40463464678,56.90420559885));
#144700=CARTESIAN_POINT('Ctrl Pts',(96.2404380922691,11.08085053798,56.7487309300401));
#144701=CARTESIAN_POINT('Ctrl Pts',(96.2821887412691,10.61938261741,56.53394353332));
#144702=CARTESIAN_POINT('Ctrl Pts',(96.309676275269,10.29835023287,56.39253313524));
#144703=CARTESIAN_POINT('Ctrl Pts',(96.3230502473691,10.13650208273,56.32373035667));
#144704=CARTESIAN_POINT('Ctrl Pts',(97.5959005388692,11.92723780495,56.59071945719));
#144705=CARTESIAN_POINT('Ctrl Pts',(97.5982687932691,11.90207219424,56.57853590535));
#144706=CARTESIAN_POINT('Ctrl Pts',(97.6142156663691,11.73247787192,56.49649676485));
#144707=CARTESIAN_POINT('Ctrl Pts',(97.6448186696691,11.40462228168,56.33905874716));
#144708=CARTESIAN_POINT('Ctrl Pts',(97.6875832150691,10.93200877884,56.11905533097));
#144709=CARTESIAN_POINT('Ctrl Pts',(97.7160179626691,10.59995097196,55.97277196594));
#144710=CARTESIAN_POINT('Ctrl Pts',(97.7298770894691,10.43223240023,55.90147329555));
#144711=CARTESIAN_POINT('Ctrl Pts',(98.6373592863691,11.5387915904,57.5954048691));
#144712=CARTESIAN_POINT('Ctrl Pts',(98.6397096481691,11.51381644996,57.58331336632));
#144713=CARTESIAN_POINT('Ctrl Pts',(98.6555216428691,11.34565686104,57.50196811114));
#144714=CARTESIAN_POINT('Ctrl Pts',(98.6856743525691,11.02260519672,57.34684664155));
#144715=CARTESIAN_POINT('Ctrl Pts',(98.7272426052691,10.56314232525,57.13299758747));
#144716=CARTESIAN_POINT('Ctrl Pts',(98.7545597390691,10.24409337348,56.99246381815));
#144717=CARTESIAN_POINT('Ctrl Pts',(98.7678464336691,10.08330129051,56.92411004131));
#144718=CARTESIAN_POINT('Ctrl Pts',(98.0919591842691,10.88937663559,58.83060487635));
#144719=CARTESIAN_POINT('Ctrl Pts',(98.0942796327691,10.86471992855,58.81866726368));
#144720=CARTESIAN_POINT('Ctrl Pts',(98.109866134269,10.69895896597,58.73848206487));
#144721=CARTESIAN_POINT('Ctrl Pts',(98.139266030869,10.38393863577,58.58723346345));
#144722=CARTESIAN_POINT('Ctrl Pts',(98.1788342886691,9.94646134776901,58.38367343947));
#144723=CARTESIAN_POINT('Ctrl Pts',(98.204282965369,9.64916095408402,58.25275200076));
#144724=CARTESIAN_POINT('Ctrl Pts',(98.2166126522691,9.49994876354401,58.1893215771));
#144725=CARTESIAN_POINT('Origin',(96.7134309613668,10.8856837889288,58.2201165235725));
#144726=CARTESIAN_POINT('Ctrl Pts',(96.095757050069,12.56332359615,57.55926050678));
#144727=CARTESIAN_POINT('Ctrl Pts',(96.102715496369,12.51478413356,57.5234625825));
#144728=CARTESIAN_POINT('Ctrl Pts',(96.1154032364691,12.42239695131,57.45819014398));
#144729=CARTESIAN_POINT('Ctrl Pts',(96.1329310601691,12.28520907105,57.36801775808));
#144730=CARTESIAN_POINT('Ctrl Pts',(96.1492921242691,12.14940768661,57.28384780045));
#144731=CARTESIAN_POINT('Ctrl Pts',(96.1657574770691,12.0034808127,57.19914132621));
#144732=CARTESIAN_POINT('Ctrl Pts',(96.1813456845691,11.8528395076,57.11894735106));
#144733=CARTESIAN_POINT('Ctrl Pts',(96.195164363669,11.71115093,57.04785676469));
#144734=CARTESIAN_POINT('Ctrl Pts',(96.2081771592692,11.57434490033,56.98091206873));
#144735=CARTESIAN_POINT('Ctrl Pts',(96.2204772585692,11.44332796521,56.91763385951));
#144736=CARTESIAN_POINT('Ctrl Pts',(96.228403107169,11.35848918082,56.8768591065301));
#144737=CARTESIAN_POINT('Ctrl Pts',(96.232252508769,11.31727201741,56.85705575105));
#144738=CARTESIAN_POINT('Ctrl Pts',(97.4808568854692,13.00157661483,57.2381820055001));
#144739=CARTESIAN_POINT('Ctrl Pts',(97.4891197811691,12.94386767406,57.19567330404));
#144740=CARTESIAN_POINT('Ctrl Pts',(97.5038887926691,12.83627687729,57.11969370597));
#144741=CARTESIAN_POINT('Ctrl Pts',(97.5237380737692,12.68084622952,57.01757851685));
#144742=CARTESIAN_POINT('Ctrl Pts',(97.5420178020692,12.52915975172,56.92353793651));
#144743=CARTESIAN_POINT('Ctrl Pts',(97.5609169829691,12.36171395817,56.82631056443));
#144744=CARTESIAN_POINT('Ctrl Pts',(97.5787431504691,12.18934898555,56.73460334054));
#144745=CARTESIAN_POINT('Ctrl Pts',(97.5935031851692,12.03787995816,56.6586699236201));
#144746=CARTESIAN_POINT('Ctrl Pts',(97.6069668917692,11.89634010197,56.58940550347));
#144747=CARTESIAN_POINT('Ctrl Pts',(97.6194660408691,11.76319375133,56.52510327666));
#144748=CARTESIAN_POINT('Ctrl Pts',(97.6274325288691,11.67792065658,56.4841194534901));
#144749=CARTESIAN_POINT('Ctrl Pts',(97.6312875136692,11.63664378591,56.4642873747));
#144750=CARTESIAN_POINT('Ctrl Pts',(98.5264853577691,12.47205724986,58.15468209609));
#144751=CARTESIAN_POINT('Ctrl Pts',(98.5331721520691,12.42542733435,58.1202816935401));
#144752=CARTESIAN_POINT('Ctrl Pts',(98.545426466569,12.33620631021,58.05723902479));
#144753=CARTESIAN_POINT('Ctrl Pts',(98.5624708459691,12.20281749274,57.96955373189));
#144754=CARTESIAN_POINT('Ctrl Pts',(98.5784323475691,12.07032418462,57.88743933493));
#144755=CARTESIAN_POINT('Ctrl Pts',(98.5943908547691,11.92887863335,57.80534034209));
#144756=CARTESIAN_POINT('Ctrl Pts',(98.6095130062692,11.7827612897,57.72754400507));
#144757=CARTESIAN_POINT('Ctrl Pts',(98.6231356477691,11.64310949422,57.65746193988));
#144758=CARTESIAN_POINT('Ctrl Pts',(98.6360545410691,11.5072892856,57.5910003273));
#144759=CARTESIAN_POINT('Ctrl Pts',(98.6483131880692,11.37671580202,57.52793537011));
#144760=CARTESIAN_POINT('Ctrl Pts',(98.6562305735691,11.29196746291,57.48720415607));
#144761=CARTESIAN_POINT('Ctrl Pts',(98.6600788123691,11.25076273356,57.4674067822201));
#144762=CARTESIAN_POINT('Ctrl Pts',(98.0125191480691,11.59265124379,59.23931483098));
#144763=CARTESIAN_POINT('Ctrl Pts',(98.0165884117691,11.56442096011,59.21838038874));
#144764=CARTESIAN_POINT('Ctrl Pts',(98.0246664116691,11.50570776901,59.17682288956));
#144765=CARTESIAN_POINT('Ctrl Pts',(98.0370525149691,11.40892520096,59.11310222996));
#144766=CARTESIAN_POINT('Ctrl Pts',(98.0491639918691,11.30830719299,59.05079439342));
#144767=CARTESIAN_POINT('Ctrl Pts',(98.0602387379691,11.21004187408,58.99382004842));
#144768=CARTESIAN_POINT('Ctrl Pts',(98.0708701605691,11.10751561337,58.9391263933));
#144769=CARTESIAN_POINT('Ctrl Pts',(98.0826038618691,10.98748943577,58.87876203478));
#144770=CARTESIAN_POINT('Ctrl Pts',(98.0946179494691,10.86116820446,58.81695522043));
#144771=CARTESIAN_POINT('Ctrl Pts',(98.1064771796691,10.7348676425,58.75594507446));
#144772=CARTESIAN_POINT('Ctrl Pts',(98.1143130175691,10.65099079798,58.71563338423));
#144773=CARTESIAN_POINT('Ctrl Pts',(98.1181500529691,10.60990587824,58.69589364708));
#144774=CARTESIAN_POINT('Ctrl Pts',(96.4483997728069,12.4478951511663,57.3802413623125));
#144775=CARTESIAN_POINT('Ctrl Pts',(96.4503965593856,12.4174690215184,57.360275428893));
#144776=CARTESIAN_POINT('Ctrl Pts',(96.4523301450555,12.3874581010196,57.341020297604));
#144777=CARTESIAN_POINT('Ctrl Pts',(96.4542318291937,12.3577640171988,57.3223117132754));
#144778=CARTESIAN_POINT('Ctrl Pts',(96.4561788230357,12.3273624393641,57.3031573764695));
#144779=CARTESIAN_POINT('Ctrl Pts',(96.4580925317787,12.2972901160016,57.2845751437417));
#144780=CARTESIAN_POINT('Ctrl Pts',(96.4600178933175,12.267172905776,57.2663306183736));
#144781=CARTESIAN_POINT('Ctrl Pts',(96.4611390891504,12.2496347499947,57.2557062834612));
#144782=CARTESIAN_POINT('Ctrl Pts',(96.4622641396932,12.2320822382948,57.2451969710702));
#144783=CARTESIAN_POINT('Ctrl Pts',(96.4634011392841,12.2144484575392,57.2347604468922));
#144784=CARTESIAN_POINT('Ctrl Pts',(96.4638851130955,12.2069424846703,57.2303180491777));
#144785=CARTESIAN_POINT('Ctrl Pts',(96.4643712419676,12.1994218714392,57.2258888910985));
#144786=CARTESIAN_POINT('Ctrl Pts',(96.4648589255827,12.1918906230061,57.2214760169925));
#144787=CARTESIAN_POINT('Ctrl Pts',(96.4670040447873,12.1587637654514,57.2020656027413));
#144788=CARTESIAN_POINT('Ctrl Pts',(96.4691787247034,12.1254343605685,57.1829729329922));
#144789=CARTESIAN_POINT('Ctrl Pts',(96.4713360069344,12.0922182879089,57.1644361287263));
#144790=CARTESIAN_POINT('Ctrl Pts',(96.4719225310154,12.083187468384,57.1593963235811));
#144791=CARTESIAN_POINT('Ctrl Pts',(96.4725078065675,12.0741647991286,57.1543974169163));
#144792=CARTESIAN_POINT('Ctrl Pts',(96.4730909725966,12.0651561275595,57.1494437735876));
#144793=CARTESIAN_POINT('Ctrl Pts',(96.4749397057767,12.0365971422826,57.1337399014011));
#144794=CARTESIAN_POINT('Ctrl Pts',(96.4767669938174,12.0081829116634,57.1184921654224));
#144795=CARTESIAN_POINT('Ctrl Pts',(96.4785488707318,11.9803414777681,57.103821944266));
#144796=CARTESIAN_POINT('Ctrl Pts',(96.4800041754786,11.9576026619836,57.0918403969921));
#144797=CARTESIAN_POINT('Ctrl Pts',(96.4814292548088,11.9352449100542,57.0802437418831));
#144798=CARTESIAN_POINT('Ctrl Pts',(96.482812617572,11.913476986101,57.0690901595441));
#144799=CARTESIAN_POINT('Ctrl Pts',(96.4847631184953,11.8827848517605,57.0533639355705));
#144800=CARTESIAN_POINT('Ctrl Pts',(96.4866314864273,11.8532585032914,57.0385144148399));
#144801=CARTESIAN_POINT('Ctrl Pts',(96.4884731621611,11.8245853546652,57.0242540861522));
#144802=CARTESIAN_POINT('Ctrl Pts',(96.489733386178,11.8049648591179,57.014496011824));
#144803=CARTESIAN_POINT('Ctrl Pts',(96.4909809648059,11.7857447070329,57.0050145855083));
#144804=CARTESIAN_POINT('Ctrl Pts',(96.4922318608456,11.7668349910155,56.9957270555952));
#144805=CARTESIAN_POINT('Ctrl Pts',(96.4934096768903,11.7490300206445,56.9869821228436));
#144806=CARTESIAN_POINT('Ctrl Pts',(96.4945903601356,11.7315006612338,56.9784094735593));
#144807=CARTESIAN_POINT('Ctrl Pts',(96.495778605489,11.7142162265952,56.9699844976127));
#144808=CARTESIAN_POINT('Ctrl Pts',(96.4978222701042,11.6844887066305,56.955494371329));
#144809=CARTESIAN_POINT('Ctrl Pts',(96.499888464771,11.6554845981431,56.9414402003286));
#144810=CARTESIAN_POINT('Ctrl Pts',(96.5019986356943,11.6270641292994,56.9277098101259));
#144811=CARTESIAN_POINT('Ctrl Pts',(96.5048277488586,11.588960712341,56.9093014303847));
#144812=CARTESIAN_POINT('Ctrl Pts',(96.5077358157164,11.5519073988749,56.891475448813));
#144813=CARTESIAN_POINT('Ctrl Pts',(96.5107462434937,11.5157755464754,56.8741086777739));
#144814=CARTESIAN_POINT('Ctrl Pts',(97.3598553272691,12.59304662146,57.34302211945));
#144815=CARTESIAN_POINT('Ctrl Pts',(97.2905909335691,12.48457249915,57.27739215867));
#144816=CARTESIAN_POINT('Ctrl Pts',(97.1823916103691,12.29078220396,57.16980269553));
#144817=CARTESIAN_POINT('Ctrl Pts',(97.0407277756691,12.03891918979,57.04853971653));
#144818=CARTESIAN_POINT('Ctrl Pts',(96.9065972293691,11.77555579319,56.93603687571));
#144819=CARTESIAN_POINT('Ctrl Pts',(96.8118741496691,11.52347507691,56.83220141859));
#144820=CARTESIAN_POINT('Ctrl Pts',(96.7553526290691,11.35053149358,56.75991005414));
#144821=CARTESIAN_POINT('Ctrl Pts',(96.4155772962691,12.57897283386,57.47256425052));
#144822=CARTESIAN_POINT('Ctrl Pts',(96.3548004162691,12.47093811279,57.4066316253));
#144823=CARTESIAN_POINT('Ctrl Pts',(96.2601630177691,12.27776084815,57.2986569495));
#144824=CARTESIAN_POINT('Ctrl Pts',(96.1360036193691,12.02333015192,57.17498429364));
#144825=CARTESIAN_POINT('Ctrl Pts',(96.0179323943691,11.75617400365,57.05956940227));
#144826=CARTESIAN_POINT('Ctrl Pts',(95.9345062497691,11.50262773359,56.95458058277));
#144827=CARTESIAN_POINT('Ctrl Pts',(95.8848951356691,11.3292765712,56.88185866928));
#144828=CARTESIAN_POINT('Ctrl Pts',(94.2594273773691,12.53398823169,57.75933364546));
#144829=CARTESIAN_POINT('Ctrl Pts',(94.2182042994691,12.4271741912,57.6935704398));
#144830=CARTESIAN_POINT('Ctrl Pts',(94.1547707708691,12.23637559016,57.58613155241));
#144831=CARTESIAN_POINT('Ctrl Pts',(94.0707455882691,11.97320006148,57.45632676081));
#144832=CARTESIAN_POINT('Ctrl Pts',(93.9893028835691,11.69394466693,57.33289395567));
#144833=CARTESIAN_POINT('Ctrl Pts',(93.9314988904691,11.4384415765,57.2258100722));
#144834=CARTESIAN_POINT('Ctrl Pts',(93.8975579673691,11.26636189084,57.15304096365));
#144835=CARTESIAN_POINT('Ctrl Pts',(92.1249207086691,12.45611361649,58.0505002254));
#144836=CARTESIAN_POINT('Ctrl Pts',(92.1032618890691,12.35145474945,57.98614284192));
#144837=CARTESIAN_POINT('Ctrl Pts',(92.0710528306691,12.16481527354,57.88111746708));
#144838=CARTESIAN_POINT('Ctrl Pts',(92.0271469727691,11.8851148392,57.74207150913));
#144839=CARTESIAN_POINT('Ctrl Pts',(91.9820262412691,11.58554660934,57.60607342512));
#144840=CARTESIAN_POINT('Ctrl Pts',(91.9492978565691,11.33112885221,57.49706203015));
#144841=CARTESIAN_POINT('Ctrl Pts',(91.9306629864691,11.16481243865,57.42570847496));
#144842=CARTESIAN_POINT('Ctrl Pts',(90.9201693766691,12.4015395951,58.23050592227));
#144843=CARTESIAN_POINT('Ctrl Pts',(90.9095559520691,12.29862098453,58.16703117139));
#144844=CARTESIAN_POINT('Ctrl Pts',(90.8950120714691,12.11470097399,58.0633845424));
#144845=CARTESIAN_POINT('Ctrl Pts',(90.8739785056691,11.82255160128,57.91735245787));
#144846=CARTESIAN_POINT('Ctrl Pts',(90.8494994559691,11.50865392223,57.77212231743));
#144847=CARTESIAN_POINT('Ctrl Pts',(90.8307945255691,11.25577205409,57.6615810195));
#144848=CARTESIAN_POINT('Ctrl Pts',(90.8206727756691,11.09390799359,57.59118585437));
#144849=CARTESIAN_POINT('Ctrl Pts',(96.3228725566692,-10.13609008452,56.32369383094));
#144850=CARTESIAN_POINT('Ctrl Pts',(96.3073991073691,-10.32332545426,56.40329742928));
#144851=CARTESIAN_POINT('Ctrl Pts',(96.2766341738692,-10.6804967028,56.56156850188));
#144852=CARTESIAN_POINT('Ctrl Pts',(96.2323525649691,-11.16575807496,56.7893764936));
#144853=CARTESIAN_POINT('Ctrl Pts',(96.2043598232691,-11.46454615057,56.93338594698));
#144854=CARTESIAN_POINT('Ctrl Pts',(96.1917988812692,-11.59798170647,56.99800606902));
#144855=CARTESIAN_POINT('Ctrl Pts',(97.7297501322691,-10.43195556948,55.90123229366));
#144856=CARTESIAN_POINT('Ctrl Pts',(97.7137150971691,-10.6259862983,55.98372498668));
#144857=CARTESIAN_POINT('Ctrl Pts',(97.6818999404691,-10.99529135564,56.14739896205));
#144858=CARTESIAN_POINT('Ctrl Pts',(97.6366458245691,-11.49114086689,56.3802100435801));
#144859=CARTESIAN_POINT('Ctrl Pts',(97.6083601074691,-11.79304779847,56.52572671727));
#144860=CARTESIAN_POINT('Ctrl Pts',(97.5957180332691,-11.92734449924,56.59076422634));
#144861=CARTESIAN_POINT('Ctrl Pts',(98.7678990136691,-10.08298790648,56.92386767886));
#144862=CARTESIAN_POINT('Ctrl Pts',(98.7525263582691,-10.26900363965,57.00295274013));
#144863=CARTESIAN_POINT('Ctrl Pts',(98.7219499196691,-10.62399710232,57.16025409535));
#144864=CARTESIAN_POINT('Ctrl Pts',(98.6778428571691,-11.10735810665,57.38716412844));
#144865=CARTESIAN_POINT('Ctrl Pts',(98.6499026988691,-11.40558640745,57.53090306468));
#144866=CARTESIAN_POINT('Ctrl Pts',(98.6373563185692,-11.53886740437,57.59544827376));
#144867=CARTESIAN_POINT('Ctrl Pts',(98.2166477117691,-9.49950866349698,
58.18916950595));
#144868=CARTESIAN_POINT('Ctrl Pts',(98.2023825655691,-9.67212320196098,
58.2625569551));
#144869=CARTESIAN_POINT('Ctrl Pts',(98.1738772823691,-10.00318746055,58.40920319245));
#144870=CARTESIAN_POINT('Ctrl Pts',(98.1316881104691,-10.46566749127,58.62624658273));
#144871=CARTESIAN_POINT('Ctrl Pts',(98.1043257318692,-10.75774506542,58.76701311493));
#144872=CARTESIAN_POINT('Ctrl Pts',(98.0919393532691,-10.88932779005,58.83073519093));
#144873=CARTESIAN_POINT('',(96.5106393256908,-11.5155612869847,56.8741302054996));
#144874=CARTESIAN_POINT('Ctrl Pts',(96.6021949941369,-10.33475523448,56.3300847780136));
#144875=CARTESIAN_POINT('Ctrl Pts',(96.5948822022228,-10.435748834368,56.3737520728817));
#144876=CARTESIAN_POINT('Ctrl Pts',(96.5874571230913,-10.5359169900225,
56.4179778623221));
#144877=CARTESIAN_POINT('Ctrl Pts',(96.5799409457604,-10.635428958833,56.4626894439106));
#144878=CARTESIAN_POINT('Ctrl Pts',(96.5741108888598,-10.7126171909511,
56.4973707790231));
#144879=CARTESIAN_POINT('Ctrl Pts',(96.5682259870746,-10.7894129763387,
56.5323441573885));
#144880=CARTESIAN_POINT('Ctrl Pts',(96.5622983146813,-10.8658798203598,
56.567554048647));
#144881=CARTESIAN_POINT('Ctrl Pts',(96.556828481434,-10.9364405494262,56.600044412665));
#144882=CARTESIAN_POINT('Ctrl Pts',(96.5513222058239,-11.0067221225276,
56.6327362197256));
#144883=CARTESIAN_POINT('Ctrl Pts',(96.5457914507374,-11.0767403757038,
56.6655656323231));
#144884=CARTESIAN_POINT('Ctrl Pts',(96.5405297524791,-11.1433524232494,
56.6967979795132));
#144885=CARTESIAN_POINT('Ctrl Pts',(96.5352458876006,-11.2097266735917,
56.7281548929787));
#144886=CARTESIAN_POINT('Ctrl Pts',(96.5299527321305,-11.2758345850683,
56.7595617552571));
#144887=CARTESIAN_POINT('Ctrl Pts',(96.5248807987823,-11.3391795827159,
56.7896559992396));
#144888=CARTESIAN_POINT('Ctrl Pts',(96.519800335829,-11.4022802633477,56.8197960704493));
#144889=CARTESIAN_POINT('Ctrl Pts',(96.5147251649627,-11.4650665900728,
56.8498979075562));
#144890=CARTESIAN_POINT('Ctrl Pts',(96.5133627229575,-11.4819217327144,
56.8579788191922));
#144891=CARTESIAN_POINT('Ctrl Pts',(96.5120006766485,-11.4987539524958,
56.8660568709375));
#144892=CARTESIAN_POINT('Ctrl Pts',(96.5106393253565,-11.5155612875649,
56.8741302042353));
#144893=CARTESIAN_POINT('Origin',(96.7134217792691,-10.8854245001,58.22016396893));
#144894=CARTESIAN_POINT('Ctrl Pts',(96.2319806560691,-11.31915553447,56.85809517453));
#144895=CARTESIAN_POINT('Ctrl Pts',(96.2313075516691,-11.32636229438,56.8615579791));
#144896=CARTESIAN_POINT('Ctrl Pts',(96.2269271353691,-11.3732593077,56.88409315519));
#144897=CARTESIAN_POINT('Ctrl Pts',(96.2187625258692,-11.46060590276,56.92609622013));
#144898=CARTESIAN_POINT('Ctrl Pts',(96.2073028932692,-11.58253166397,56.98505062475));
#144899=CARTESIAN_POINT('Ctrl Pts',(96.1954645381691,-11.70692018984,57.04595337828));
#144900=CARTESIAN_POINT('Ctrl Pts',(96.1829463911691,-11.83547271731,57.11035333984));
#144901=CARTESIAN_POINT('Ctrl Pts',(96.1687179031691,-11.97470333685,57.18355220011));
#144902=CARTESIAN_POINT('Ctrl Pts',(96.1529902214692,-12.11658703733,57.2644637043));
#144903=CARTESIAN_POINT('Ctrl Pts',(96.1369908001691,-12.25127581358,57.34677318043));
#144904=CARTESIAN_POINT('Ctrl Pts',(96.1203673447691,-12.38344363953,57.43229301775));
#144905=CARTESIAN_POINT('Ctrl Pts',(96.1071896113692,-12.48167452487,57.50008624114));
#144906=CARTESIAN_POINT('Ctrl Pts',(96.0993554236692,-12.53698100232,57.5403894418501));
#144907=CARTESIAN_POINT('Ctrl Pts',(96.0978863429691,-12.54724815652,57.54794716878));
#144908=CARTESIAN_POINT('Ctrl Pts',(97.6310403542691,-11.63858287431,56.46525177409));
#144909=CARTESIAN_POINT('Ctrl Pts',(97.6303662018692,-11.64580085354,56.46871997001));
#144910=CARTESIAN_POINT('Ctrl Pts',(97.6259760867691,-11.69280167865,56.4913050417201));
#144911=CARTESIAN_POINT('Ctrl Pts',(97.6177567136691,-11.78073412854,56.53358983964));
#144912=CARTESIAN_POINT('Ctrl Pts',(97.6060926281691,-11.90484126191,56.5935960578001));
#144913=CARTESIAN_POINT('Ctrl Pts',(97.5938327508691,-12.03366062773,56.6566673441101));
#144914=CARTESIAN_POINT('Ctrl Pts',(97.5804970871691,-12.17067970326,56.7252730443601));
#144915=CARTESIAN_POINT('Ctrl Pts',(97.5643968403691,-12.32833263289,56.8081012202001));
#144916=CARTESIAN_POINT('Ctrl Pts',(97.5462329964691,-12.49217228257,56.9015456297601));
#144917=CARTESIAN_POINT('Ctrl Pts',(97.5283143898692,-12.6429610529,56.99372840947));
#144918=CARTESIAN_POINT('Ctrl Pts',(97.5095746503691,-12.79199140804,57.09013553031));
#144919=CARTESIAN_POINT('Ctrl Pts',(97.4944008867691,-12.90518115369,57.16819738757));
#144920=CARTESIAN_POINT('Ctrl Pts',(97.4850324848691,-12.9713358854,57.21639339649));
#144921=CARTESIAN_POINT('Ctrl Pts',(97.4832630223691,-12.98370914531,57.2254964466401));
#144922=CARTESIAN_POINT('Ctrl Pts',(98.6598999117692,-11.25268497975,57.4683762086));
#144923=CARTESIAN_POINT('Ctrl Pts',(98.6592270254691,-11.259889405,57.47183789127));
#144924=CARTESIAN_POINT('Ctrl Pts',(98.6548486273692,-11.30676481583,57.49436268444));
#144925=CARTESIAN_POINT('Ctrl Pts',(98.6466954137691,-11.39398949866,57.5363071227601));
#144926=CARTESIAN_POINT('Ctrl Pts',(98.6352783263692,-11.51546133186,57.59504265246));
#144927=CARTESIAN_POINT('Ctrl Pts',(98.6235276870692,-11.63892783149,57.65549414976));
#144928=CARTESIAN_POINT('Ctrl Pts',(98.6111796595691,-11.7657185306,57.71901892705));
#144929=CARTESIAN_POINT('Ctrl Pts',(98.5973406711692,-11.9011155986,57.79021399533));
#144930=CARTESIAN_POINT('Ctrl Pts',(98.5821199374691,-12.03843042241,57.86851749115));
#144931=CARTESIAN_POINT('Ctrl Pts',(98.5665198849691,-12.16976890454,57.94877240313));
#144932=CARTESIAN_POINT('Ctrl Pts',(98.5503368132692,-12.29842775824,58.03202667427));
#144933=CARTESIAN_POINT('Ctrl Pts',(98.5375744394691,-12.39354581128,58.0976830680801));
#144934=CARTESIAN_POINT('Ctrl Pts',(98.5300595107692,-12.44659484427,58.1363438316));
#144935=CARTESIAN_POINT('Ctrl Pts',(98.5286529374691,-12.45642373287,58.14357998778));
#144936=CARTESIAN_POINT('Ctrl Pts',(98.1179556775691,-10.61177639351,58.6968958282));
#144937=CARTESIAN_POINT('Ctrl Pts',(98.117284893969,-10.61895830798,58.70034669351));
#144938=CARTESIAN_POINT('Ctrl Pts',(98.1129259557691,-10.66562542773,58.72277137462));
#144939=CARTESIAN_POINT('Ctrl Pts',(98.1048826215691,-10.75167463385,58.76415053543));
#144940=CARTESIAN_POINT('Ctrl Pts',(98.093875754469,-10.86876969659,58.82077567492));
#144941=CARTESIAN_POINT('Ctrl Pts',(98.082970869869,-10.98334602619,58.87687616307));
#144942=CARTESIAN_POINT('Ctrl Pts',(98.072263132669,-11.09314918956,58.93196242022));
#144943=CARTESIAN_POINT('Ctrl Pts',(98.062179696969,-11.19158318259,58.98383694122));
#144944=CARTESIAN_POINT('Ctrl Pts',(98.0518469520691,-11.28484493202,59.03699404015));
#144945=CARTESIAN_POINT('Ctrl Pts',(98.0400976106691,-11.38387990358,59.09743885998));
#144946=CARTESIAN_POINT('Ctrl Pts',(98.028160714769,-11.47870527343,59.15884855924));
#144947=CARTESIAN_POINT('Ctrl Pts',(98.0194032357691,-11.5438094209,59.20390165835));
#144948=CARTESIAN_POINT('Ctrl Pts',(98.014966600369,-11.57509219147,59.22672605496));
#144949=CARTESIAN_POINT('Ctrl Pts',(98.0141627222692,-11.58069532646,59.23086162834));
#144950=CARTESIAN_POINT('',(96.4484068068018,-12.4473571364169,57.3800828637172));
#144951=CARTESIAN_POINT('Ctrl Pts',(96.4484069697816,-12.447356425455,57.3800839617248));
#144952=CARTESIAN_POINT('Ctrl Pts',(96.4893190913068,-12.4538771542219,
57.378233981164));
#144953=CARTESIAN_POINT('Ctrl Pts',(96.5312830311879,-12.4596052833508,
57.3777807178534));
#144954=CARTESIAN_POINT('Ctrl Pts',(96.5741400434367,-12.4644013848093,
57.3789024988894));
#144955=CARTESIAN_POINT('Ctrl Pts',(96.6157010964277,-12.4690524562772,
57.3799903582299));
#144956=CARTESIAN_POINT('Ctrl Pts',(96.6581018844681,-12.4728266228935,
57.3825600077121));
#144957=CARTESIAN_POINT('Ctrl Pts',(96.7011513468475,-12.4756001614079,
57.3867599081895));
#144958=CARTESIAN_POINT('Ctrl Pts',(96.7435267318481,-12.478330271283,57.3908940457572));
#144959=CARTESIAN_POINT('Ctrl Pts',(96.7865304254406,-12.4800904383511,
57.3966083483396));
#144960=CARTESIAN_POINT('Ctrl Pts',(96.8299370827375,-12.4807719117444,
57.404022119513));
#144961=CARTESIAN_POINT('Ctrl Pts',(96.8737937555444,-12.4814604502659,
57.4115127524449));
#144962=CARTESIAN_POINT('Ctrl Pts',(96.9180615393185,-12.4810473177835,
57.4207389690825));
#144963=CARTESIAN_POINT('Ctrl Pts',(96.9624667943407,-12.4794367139336,
57.4317912123836));
#144964=CARTESIAN_POINT('Ctrl Pts',(97.0068720493629,-12.4778261100836,
57.4428434556847));
#144965=CARTESIAN_POINT('Ctrl Pts',(97.0514142010242,-12.4750175693876,
57.4557223128417));
#144966=CARTESIAN_POINT('Ctrl Pts',(97.0957849195706,-12.470938813128,57.4704761434959));
#144967=CARTESIAN_POINT('Ctrl Pts',(97.1377011296428,-12.4670856863405,
57.4844138187315));
#144968=CARTESIAN_POINT('Ctrl Pts',(97.1794634177598,-12.4620989057031,
57.5000247223907));
#144969=CARTESIAN_POINT('Ctrl Pts',(97.2207917445358,-12.4559422742179,
57.5173087968349));
#144970=CARTESIAN_POINT('Ctrl Pts',(97.2617036898199,-12.4498476705862,
57.5344187348147));
#144971=CARTESIAN_POINT('Ctrl Pts',(97.3021896319551,-12.4426064948674,
57.5531684176607));
#144972=CARTESIAN_POINT('Ctrl Pts',(97.3419691595277,-12.434210692175,57.5735154359813));
#144973=CARTESIAN_POINT('Ctrl Pts',(97.3814382133613,-12.4258804175673,
57.5937036486236));
#144974=CARTESIAN_POINT('Ctrl Pts',(97.4202110615909,-12.4164133950479,
57.6154643206232));
#144975=CARTESIAN_POINT('Ctrl Pts',(97.4580164616892,-12.4058304019727,
57.638713508724));
#144976=CARTESIAN_POINT('Ctrl Pts',(97.4955830607536,-12.3953142572759,
57.6618158413454));
#144977=CARTESIAN_POINT('Ctrl Pts',(97.5321936397794,-12.3836962334291,
57.6863877413472));
#144978=CARTESIAN_POINT('Ctrl Pts',(97.5675961378212,-12.3710253925851,
57.7123065004887));
#144979=CARTESIAN_POINT('Ctrl Pts',(97.6029196551025,-12.3583828195952,
57.7381674364984));
#144980=CARTESIAN_POINT('Ctrl Pts',(97.6370397771934,-12.3446922587843,
57.7653688874088));
#144981=CARTESIAN_POINT('Ctrl Pts',(97.6697311107884,-12.3300298030798,
57.7937527192353));
#144982=CARTESIAN_POINT('Ctrl Pts',(97.7024160707833,-12.3153702060115,
57.8221310172651));
#144983=CARTESIAN_POINT('Ctrl Pts',(97.7336722081264,-12.2997393319065,
57.851690761331));
#144984=CARTESIAN_POINT('Ctrl Pts',(97.7633089944017,-12.2832377915447,
57.882243760512));
#144985=CARTESIAN_POINT('Ctrl Pts',(97.7930004653707,-12.2667058031555,
57.9128531349486));
#144986=CARTESIAN_POINT('Ctrl Pts',(97.8210661605585,-12.24930025847,57.94445885743));
#144987=CARTESIAN_POINT('Ctrl Pts',(97.8473571927605,-12.2311427286913,
57.9768493419059));
#144988=CARTESIAN_POINT('Ctrl Pts',(97.8738603842561,-12.2128386740951,
58.0095012060892));
#144989=CARTESIAN_POINT('Ctrl Pts',(97.898559852216,-12.1937708354519,58.042949909243));
#144990=CARTESIAN_POINT('Ctrl Pts',(97.9213521725345,-12.1740790873495,
58.0769652049586));
#144991=CARTESIAN_POINT('Ctrl Pts',(97.9442669650766,-12.1542815276342,
58.1111632784186));
#144992=CARTESIAN_POINT('Ctrl Pts',(97.9652539912341,-12.1338537746444,
58.1459333767709));
#144993=CARTESIAN_POINT('Ctrl Pts',(97.9842603705065,-12.1129471224486,
58.1810379229406));
#144994=CARTESIAN_POINT('Ctrl Pts',(98.0035173027979,-12.0917648667436,
58.2166052374207));
#144995=CARTESIAN_POINT('Ctrl Pts',(98.0207411070807,-12.0700914563442,
58.2525152097198));
#144996=CARTESIAN_POINT('Ctrl Pts',(98.0359302430688,-12.0480868126932,
58.2885272816885));
#144997=CARTESIAN_POINT('Ctrl Pts',(98.0481980866499,-12.030314272729,58.3176132327453));
#144998=CARTESIAN_POINT('Ctrl Pts',(98.0591397681909,-12.0123257910484,
58.3467658050509));
#144999=CARTESIAN_POINT('Ctrl Pts',(98.0687781393095,-11.9942038529267,
58.3758655187164));
#145000=CARTESIAN_POINT('Ctrl Pts',(98.0809676575064,-11.9712852817514,
58.4126675348335));
#145001=CARTESIAN_POINT('Ctrl Pts',(98.0910715461646,-11.9481538719064,
58.449383929842));
#145002=CARTESIAN_POINT('Ctrl Pts',(98.099178380364,-11.9249674616475,58.485794544027));
#145003=CARTESIAN_POINT('Ctrl Pts',(98.1077036599592,-11.9005842529365,
58.524084542136));
#145004=CARTESIAN_POINT('Ctrl Pts',(98.1140208053483,-11.876140710328,58.5620357186189));
#145005=CARTESIAN_POINT('Ctrl Pts',(98.118278757214,-11.851802770553,58.5994274744218));
#145006=CARTESIAN_POINT('Ctrl Pts',(98.1224939549306,-11.8277092083423,
58.636443779127));
#145007=CARTESIAN_POINT('Ctrl Pts',(98.1246919997929,-11.8037193227494,
58.6729117391277));
#145008=CARTESIAN_POINT('Ctrl Pts',(98.1250506186695,-11.7799723843313,
58.7086564524736));
#145009=CARTESIAN_POINT('Ctrl Pts',(98.1254196683622,-11.7555347406445,
58.7454408392881));
#145010=CARTESIAN_POINT('Ctrl Pts',(98.1238414891517,-11.7313546018995,
58.7814591122462));
#145011=CARTESIAN_POINT('Ctrl Pts',(98.1205327574654,-11.7075573331155,
58.8165648437517));
#145012=CARTESIAN_POINT('Ctrl Pts',(98.1173132273221,-11.6844016252964,
58.8507241445059));
#145013=CARTESIAN_POINT('Ctrl Pts',(98.1124559595994,-11.6616082826077,
58.8840198016753));
#145014=CARTESIAN_POINT('Ctrl Pts',(98.1061703789843,-11.63926799201,58.9163561174313));
#145015=CARTESIAN_POINT('Ctrl Pts',(96.5106393247643,-11.5155613004658,
56.8741302153513));
#145016=CARTESIAN_POINT('Ctrl Pts',(96.5066749286283,-11.5631862216957,
56.8970227527718));
#145017=CARTESIAN_POINT('Ctrl Pts',(96.5030313220881,-11.6080902015577,
56.918671656639));
#145018=CARTESIAN_POINT('Ctrl Pts',(96.4996983376335,-11.6502777389037,
56.9391304643533));
#145019=CARTESIAN_POINT('Ctrl Pts',(96.4963653531789,-11.6924652762497,
56.9595892720676));
#145020=CARTESIAN_POINT('Ctrl Pts',(96.4933429523757,-11.7319365505139,
56.9788582111886));
#145021=CARTESIAN_POINT('Ctrl Pts',(96.4906224361774,-11.7687490610692,
56.9969987578413));
#145022=CARTESIAN_POINT('Ctrl Pts',(96.4899581736939,-11.7777374911698,
57.0014280953984));
#145023=CARTESIAN_POINT('Ctrl Pts',(96.4893117294717,-11.7865742664474,
57.0057934108544));
#145024=CARTESIAN_POINT('Ctrl Pts',(96.4886826702735,-11.7952521909895,
57.0100916153233));
#145025=CARTESIAN_POINT('Ctrl Pts',(96.4867353898755,-11.8221150878399,
57.0233968961805));
#145026=CARTESIAN_POINT('Ctrl Pts',(96.4849547223737,-11.8474563107511,
57.0360607843061));
#145027=CARTESIAN_POINT('Ctrl Pts',(96.4833381269162,-11.8713352449221,
57.0481183769609));
#145028=CARTESIAN_POINT('Ctrl Pts',(96.4822687126468,-11.8871316971652,
57.0560947458044));
#145029=CARTESIAN_POINT('Ctrl Pts',(96.481271504146,-11.9022829407061,57.0638029876073));
#145030=CARTESIAN_POINT('Ctrl Pts',(96.4803555906446,-11.9167127980408,
57.0711991016382));
#145031=CARTESIAN_POINT('Ctrl Pts',(96.4798976338939,-11.9239277267081,
57.0748971586537));
#145032=CARTESIAN_POINT('Ctrl Pts',(96.47946022252,-11.9309599342884,57.0785158470131));
#145033=CARTESIAN_POINT('Ctrl Pts',(96.4790447553625,-11.9377979344283,
57.0820479225602));
#145034=CARTESIAN_POINT('Ctrl Pts',(96.4787394115283,-11.9428234608584,
57.0846437895757));
#145035=CARTESIAN_POINT('Ctrl Pts',(96.4784827063687,-11.9470974167123,
57.0868576939403));
#145036=CARTESIAN_POINT('Ctrl Pts',(96.4781940917681,-11.9520431752827,
57.0894262281173));
#145037=CARTESIAN_POINT('Ctrl Pts',(96.4780900019015,-11.9538268804346,
57.090352578965));
#145038=CARTESIAN_POINT('Ctrl Pts',(96.477981737352,-11.9556975042579,57.0913249890787));
#145039=CARTESIAN_POINT('Ctrl Pts',(96.4778654307572,-11.9577201783725,
57.0923778281301));
#145040=CARTESIAN_POINT('Ctrl Pts',(96.4770494692035,-11.9719104684157,
57.0997641349011));
#145041=CARTESIAN_POINT('Ctrl Pts',(96.4761923774212,-11.9868735820673,
57.1076221122303));
#145042=CARTESIAN_POINT('Ctrl Pts',(96.4752940421185,-12.002493003654,57.1159265339759));
#145043=CARTESIAN_POINT('Ctrl Pts',(96.4748697035453,-12.0098710094506,
57.1198492190405));
#145044=CARTESIAN_POINT('Ctrl Pts',(96.4744361763087,-12.0173960951725,
57.1238718803706));
#145045=CARTESIAN_POINT('Ctrl Pts',(96.4739935249068,-12.0250595572787,
57.1279938365111));
#145046=CARTESIAN_POINT('Ctrl Pts',(96.472933032369,-12.0434194773924,57.1378691101673));
#145047=CARTESIAN_POINT('Ctrl Pts',(96.4718199186621,-12.0625706369947,
57.1483134352813));
#145048=CARTESIAN_POINT('Ctrl Pts',(96.4706592173138,-12.0823880798194,
57.1592984892521));
#145049=CARTESIAN_POINT('Ctrl Pts',(96.4694477493664,-12.1030722952861,
57.1707640060321));
#145050=CARTESIAN_POINT('Ctrl Pts',(96.4681844326933,-12.1244823456784,
57.1828188137631));
#145051=CARTESIAN_POINT('Ctrl Pts',(96.4668787205247,-12.146531406365,57.1954486131704));
#145052=CARTESIAN_POINT('Ctrl Pts',(96.4663072983083,-12.1561807942083,
57.2009758251726));
#145053=CARTESIAN_POINT('Ctrl Pts',(96.4657278037075,-12.1659532578178,
57.206613363283));
#145054=CARTESIAN_POINT('Ctrl Pts',(96.465141233958,-12.1758444703791,57.2123607911272));
#145055=CARTESIAN_POINT('Ctrl Pts',(96.4639672349064,-12.1956413899699,
57.2238640690296));
#145056=CARTESIAN_POINT('Ctrl Pts',(96.4627716846492,-12.2156634952071,
57.2356621888345));
#145057=CARTESIAN_POINT('Ctrl Pts',(96.4615437003296,-12.2361742041662,
57.2479153418891));
#145058=CARTESIAN_POINT('Ctrl Pts',(96.4600634931821,-12.2608977267049,
57.2626852411802));
#145059=CARTESIAN_POINT('Ctrl Pts',(96.4585362478738,-12.2863371469124,
57.2781186113081));
#145060=CARTESIAN_POINT('Ctrl Pts',(96.4569321323794,-12.3126258335614,
57.294351191593));
#145061=CARTESIAN_POINT('Ctrl Pts',(96.4556292751448,-12.3339774168546,
57.3075352389607));
#145062=CARTESIAN_POINT('Ctrl Pts',(96.4542757135791,-12.355889621406,57.321247095118));
#145063=CARTESIAN_POINT('Ctrl Pts',(96.4528558209465,-12.3784018160607,
57.3355555749792));
#145064=CARTESIAN_POINT('Ctrl Pts',(96.4514434113654,-12.4007953680047,
57.349788646962));
#145065=CARTESIAN_POINT('Ctrl Pts',(96.4499653524067,-12.4237840599592,
57.3646127482254));
#145066=CARTESIAN_POINT('Ctrl Pts',(96.4484067536389,-12.447357368126,57.3800825052753));
#145067=CARTESIAN_POINT('Ctrl Pts',(90.9278844222691,-12.40246332161,58.22971617592));
#145068=CARTESIAN_POINT('Ctrl Pts',(90.9171817651691,-12.29937061118,58.16611616086));
#145069=CARTESIAN_POINT('Ctrl Pts',(90.9025093010691,-12.11530240729,58.06236938668));
#145070=CARTESIAN_POINT('Ctrl Pts',(90.8813150710691,-11.82300855506,57.91626489308));
#145071=CARTESIAN_POINT('Ctrl Pts',(90.8566702536691,-11.50876591956,57.77089205131));
#145072=CARTESIAN_POINT('Ctrl Pts',(90.8378431748691,-11.25540710816,57.660165762));
#145073=CARTESIAN_POINT('Ctrl Pts',(90.8276461323691,-11.0930235466,57.58955284956));
#145074=CARTESIAN_POINT('Ctrl Pts',(93.0012603032691,-12.49640477047,57.92011916884));
#145075=CARTESIAN_POINT('Ctrl Pts',(92.9715256168691,-12.39034853487,57.85501455448));
#145076=CARTESIAN_POINT('Ctrl Pts',(92.9264209346691,-12.20156124715,57.74887203586));
#145077=CARTESIAN_POINT('Ctrl Pts',(92.8658417595691,-11.93067689713,57.61478182321));
#145078=CARTESIAN_POINT('Ctrl Pts',(92.8056300846691,-11.64110581084,57.48530032852));
#145079=CARTESIAN_POINT('Ctrl Pts',(92.7626282873691,-11.38507271696,57.37719145258));
#145080=CARTESIAN_POINT('Ctrl Pts',(92.7377365505691,-11.21498097297,57.30490731823));
#145081=CARTESIAN_POINT('Ctrl Pts',(95.0799851341691,-12.55698062284,57.65477957029));
#145082=CARTESIAN_POINT('Ctrl Pts',(95.0311505215691,-12.44946610374,57.5884392369));
#145083=CARTESIAN_POINT('Ctrl Pts',(94.9556138692691,-12.25709808174,57.47998237856));
#145084=CARTESIAN_POINT('Ctrl Pts',(94.8560974936691,-11.99852059974,57.35274250657));
#145085=CARTESIAN_POINT('Ctrl Pts',(94.7605596055691,-11.72521941751,57.23289934619));
#145086=CARTESIAN_POINT('Ctrl Pts',(94.6929890760691,-11.46925250975,57.12614789029));
#145087=CARTESIAN_POINT('Ctrl Pts',(94.6530499956691,-11.29502925224,57.05268887033));
#145088=CARTESIAN_POINT('Ctrl Pts',(97.1903838030691,-12.59070340104,57.36655831744));
#145089=CARTESIAN_POINT('Ctrl Pts',(97.1225479932691,-12.48219631072,57.30079562324));
#145090=CARTESIAN_POINT('Ctrl Pts',(97.0166594629691,-12.28831915113,57.19301649588));
#145091=CARTESIAN_POINT('Ctrl Pts',(96.8780171988691,-12.03579204712,57.07122310877));
#145092=CARTESIAN_POINT('Ctrl Pts',(96.7465770377691,-11.77136893742,56.9580407289));
#145093=CARTESIAN_POINT('Ctrl Pts',(96.6537324103691,-11.51851036624,56.85379357844));
#145094=CARTESIAN_POINT('Ctrl Pts',(96.5983080857691,-11.34492571889,56.78118190673));
#145095=CARTESIAN_POINT('Ctrl Pts',(90.9923722612358,-11.2699867077028,
57.6397093617629));
#145096=CARTESIAN_POINT('Ctrl Pts',(92.8191441570593,-11.3889082784922,
57.3718321147041));
#145097=CARTESIAN_POINT('Ctrl Pts',(94.6514920487796,-11.4676844930577,
57.1318009631947));
#145098=CARTESIAN_POINT('Ctrl Pts',(96.5106393247643,-11.5155613004658,
56.8741302153513));
#145099=CARTESIAN_POINT('Ctrl Pts',(91.0788478348321,-12.2836022595699,
58.1301370595523));
#145100=CARTESIAN_POINT('Ctrl Pts',(92.2850753424178,-12.3359375090943,
57.9484854194747));
#145101=CARTESIAN_POINT('Ctrl Pts',(93.4933486351873,-12.3773001586785,
57.7816267963501));
#145102=CARTESIAN_POINT('Ctrl Pts',(94.7090794812645,-12.4088635897447,
57.6162793126818));
#145103=CARTESIAN_POINT('Ctrl Pts',(95.2869785032647,-12.4238673021232,
57.5376812007639));
#145104=CARTESIAN_POINT('Ctrl Pts',(95.866561870591,-12.4366566914144,57.4594245164494));
#145105=CARTESIAN_POINT('Ctrl Pts',(96.4484067536153,-12.4473573684819,
57.3800825055088));
#145106=CARTESIAN_POINT('Ctrl Pts',(91.7196664240691,-14.99486169804,63.073579399731));
#145107=CARTESIAN_POINT('Ctrl Pts',(91.6086219852691,-15.02536569563,62.38693020624));
#145108=CARTESIAN_POINT('Ctrl Pts',(91.3904040401691,-14.82128093489,61.04174493848));
#145109=CARTESIAN_POINT('Ctrl Pts',(91.1055790545691,-13.80539132818,59.26782647843));
#145110=CARTESIAN_POINT('Ctrl Pts',(90.9674151548691,-12.74459813474,58.4019492402));
#145111=CARTESIAN_POINT('Ctrl Pts',(90.9189065908691,-12.15226092818,58.08327559231));
#145112=CARTESIAN_POINT('Ctrl Pts',(94.5341587467691,-14.99518185508,62.57017586031));
#145113=CARTESIAN_POINT('Ctrl Pts',(94.3058556568691,-15.02368077332,61.93133855973));
#145114=CARTESIAN_POINT('Ctrl Pts',(93.8619238271691,-14.84035203637,60.68236085645));
#145115=CARTESIAN_POINT('Ctrl Pts',(93.2453658119691,-13.87785869838,58.97788256701));
#145116=CARTESIAN_POINT('Ctrl Pts',(92.9143512058691,-12.83695860105,58.12194824018));
#145117=CARTESIAN_POINT('Ctrl Pts',(92.7770364957691,-12.23327460907,57.79774621738));
#145118=CARTESIAN_POINT('Ctrl Pts',(97.3508737698691,-14.99520415789,62.08198995714));
#145119=CARTESIAN_POINT('Ctrl Pts',(97.0060920033691,-15.01646079956,61.49512945037));
#145120=CARTESIAN_POINT('Ctrl Pts',(96.3371921958691,-14.84261766533,60.34754264612));
#145121=CARTESIAN_POINT('Ctrl Pts',(95.3895471494691,-13.92370897909,58.72466409135));
#145122=CARTESIAN_POINT('Ctrl Pts',(94.8658120496691,-12.90001659179,57.87944249812));
#145123=CARTESIAN_POINT('Ctrl Pts',(94.6396504020691,-12.28798925498,57.54917879558));
#145124=CARTESIAN_POINT('Ctrl Pts',(100.153009715269,-14.99408560257,61.51961813125));
#145125=CARTESIAN_POINT('Ctrl Pts',(99.6992618204691,-15.00733180495,60.98982798051));
#145126=CARTESIAN_POINT('Ctrl Pts',(98.8190522278691,-14.83552964287,59.95248048231));
#145127=CARTESIAN_POINT('Ctrl Pts',(97.5553693844691,-13.94727437632,58.43815492047));
#145128=CARTESIAN_POINT('Ctrl Pts',(96.8420798112691,-12.93817712032,57.6191720668));
#145129=CARTESIAN_POINT('Ctrl Pts',(96.5270565421691,-12.32101949327,57.28901682961));
#145130=CARTESIAN_POINT('',(95.9754284248432,-14.9956419886409,61.9303999844587));
#145131=CARTESIAN_POINT('Origin',(98.8105231949682,-12.3613099371181,62.2951126343007));
#145132=CARTESIAN_POINT('Ctrl Pts',(96.4484067501759,-12.4473573835336,
57.3800824823133));
#145133=CARTESIAN_POINT('Ctrl Pts',(96.4428162056186,-12.5283681372492,
57.4332801275737));
#145134=CARTESIAN_POINT('Ctrl Pts',(96.4368593228261,-12.6103539483408,
57.4900322201445));
#145135=CARTESIAN_POINT('Ctrl Pts',(96.4305324801312,-12.692936721428,57.5506122478589));
#145136=CARTESIAN_POINT('Ctrl Pts',(96.4244080470619,-12.7728774898076,
57.6092541871269));
#145137=CARTESIAN_POINT('Ctrl Pts',(96.4179369598139,-12.853377918145,57.6714834137224));
#145138=CARTESIAN_POINT('Ctrl Pts',(96.4110862810531,-12.9340584971688,
57.7375404927103));
#145139=CARTESIAN_POINT('Ctrl Pts',(96.404572653096,-13.0107696222229,57.8003475883988));
#145140=CARTESIAN_POINT('Ctrl Pts',(96.3977157598507,-13.0876437966098,
57.8666154103833));
#145141=CARTESIAN_POINT('Ctrl Pts',(96.390460874326,-13.1643180271825,57.9365394324825));
#145142=CARTESIAN_POINT('Ctrl Pts',(96.3865098506456,-13.2060749507934,
57.9746201804411));
#145143=CARTESIAN_POINT('Ctrl Pts',(96.3824403273612,-13.2477719091297,
58.0137851031057));
#145144=CARTESIAN_POINT('Ctrl Pts',(96.3782400812873,-13.2893449453626,
58.0540638211877));
#145145=CARTESIAN_POINT('Ctrl Pts',(96.3708527587521,-13.3624629060766,
58.1249053567887));
#145146=CARTESIAN_POINT('Ctrl Pts',(96.3630604453054,-13.4352201280504,
58.1992131566058));
#145147=CARTESIAN_POINT('Ctrl Pts',(96.3548763444432,-13.5072188387596,
58.2771077118593));
#145148=CARTESIAN_POINT('Ctrl Pts',(96.3471245472971,-13.5754144059446,
58.3508876910257));
#145149=CARTESIAN_POINT('Ctrl Pts',(96.3390210681869,-13.6429296388791,
58.4278856448029));
#145150=CARTESIAN_POINT('Ctrl Pts',(96.3305652270021,-13.7093879100516,
58.5081822841182));
#145151=CARTESIAN_POINT('Ctrl Pts',(96.3243339046578,-13.7583626839465,
58.5673549000412));
#145152=CARTESIAN_POINT('Ctrl Pts',(96.3179109801911,-13.8067627338357,
58.6283184846363));
#145153=CARTESIAN_POINT('Ctrl Pts',(96.311292573197,-13.8544217822592,58.6910964484846));
#145154=CARTESIAN_POINT('Ctrl Pts',(96.3012126802154,-13.9270069387988,
58.7867078482902));
#145155=CARTESIAN_POINT('Ctrl Pts',(96.2906794509788,-13.9978731788578,
58.886529385776));
#145156=CARTESIAN_POINT('Ctrl Pts',(96.2796863362393,-14.0665428342779,
58.9906502113008));
#145157=CARTESIAN_POINT('Ctrl Pts',(96.2782723638938,-14.0753753622774,
59.0040425911105));
#145158=CARTESIAN_POINT('Ctrl Pts',(96.2768507738921,-14.0841715045556,
59.0175060445161));
#145159=CARTESIAN_POINT('Ctrl Pts',(96.2754215448577,-14.0929302031139,
59.0310407123128));
#145160=CARTESIAN_POINT('Ctrl Pts',(96.2648460395679,-14.1577397337775,
59.1311897768977));
#145161=CARTESIAN_POINT('Ctrl Pts',(96.2538646209972,-14.2204403323873,
59.2351481203322));
#145162=CARTESIAN_POINT('Ctrl Pts',(96.2424880512788,-14.2805792843769,
59.342886235106));
#145163=CARTESIAN_POINT('Ctrl Pts',(96.2313797913637,-14.3392998940383,
59.4480834088842));
#145164=CARTESIAN_POINT('Ctrl Pts',(96.2198944628484,-14.3955784719746,
59.5568842666274));
#145165=CARTESIAN_POINT('Ctrl Pts',(96.2080501970947,-14.448974966694,59.6692175922599));
#145166=CARTESIAN_POINT('Ctrl Pts',(96.1966034480307,-14.5005793707712,
59.7777807921056));
#145167=CARTESIAN_POINT('Ctrl Pts',(96.1848211929471,-14.5494920202302,
59.8896433046505));
#145168=CARTESIAN_POINT('Ctrl Pts',(96.1727317296069,-14.595295785503,60.0046990841294));
#145169=CARTESIAN_POINT('Ctrl Pts',(96.1614756943887,-14.6379419130047,
60.1118231035683));
#145170=CARTESIAN_POINT('Ctrl Pts',(96.1499532633247,-14.6778929586248,
60.2217150214299));
#145171=CARTESIAN_POINT('Ctrl Pts',(96.1382000098369,-14.7147945678952,
60.334254885635));
#145172=CARTESIAN_POINT('Ctrl Pts',(96.1381781684374,-14.7148631431872,
60.3344640216106));
#145173=CARTESIAN_POINT('Ctrl Pts',(96.1381563262449,-14.7149317079431,
60.3346731667205));
#145174=CARTESIAN_POINT('Ctrl Pts',(96.1381344832597,-14.7150002621608,
60.3348823209644));
#145175=CARTESIAN_POINT('Ctrl Pts',(96.1265419877911,-14.7513833137882,
60.4458845307021));
#145176=CARTESIAN_POINT('Ctrl Pts',(96.1147289493766,-14.784784785401,60.5594202667816));
#145177=CARTESIAN_POINT('Ctrl Pts',(96.1027197551907,-14.8149038052703,
60.6753933684173));
#145178=CARTESIAN_POINT('Ctrl Pts',(96.0911665365054,-14.8438792400707,
60.7869631027453));
#145179=CARTESIAN_POINT('Ctrl Pts',(96.0794317393021,-14.8698167501967,
60.9007887087091));
#145180=CARTESIAN_POINT('Ctrl Pts',(96.0675444498865,-14.8924386342188,
61.0167379648425));
#145181=CARTESIAN_POINT('Ctrl Pts',(96.0558646668671,-14.9146656270705,
61.1306631924994));
#145182=CARTESIAN_POINT('Ctrl Pts',(96.0440376212459,-14.9336917478691,
61.2466387514315));
#145183=CARTESIAN_POINT('Ctrl Pts',(96.0320988027607,-14.9492438342748,
61.3644912538338));
#145184=CARTESIAN_POINT('Ctrl Pts',(96.0204085402785,-14.9644721395256,
61.4798901678028));
#145185=CARTESIAN_POINT('Ctrl Pts',(96.0086110796642,-14.9763695368615,
61.5970887700541));
#145186=CARTESIAN_POINT('Ctrl Pts',(95.9967479481211,-14.9846702418281,
61.7158760293545));
#145187=CARTESIAN_POINT('Ctrl Pts',(95.9896612697387,-14.9896288335989,
61.78683596936));
#145188=CARTESIAN_POINT('Ctrl Pts',(95.9825513164671,-14.9933037637515,
61.8583618898565));
#145189=CARTESIAN_POINT('Ctrl Pts',(95.9754284498954,-14.9956367981312,
61.9304001540396));
#145190=CARTESIAN_POINT('Ctrl Pts',(96.1768270765691,-12.21821914294,57.31259750763));
#145191=CARTESIAN_POINT('Ctrl Pts',(96.1765540719691,-12.22049670601,57.31400198718));
#145192=CARTESIAN_POINT('Ctrl Pts',(96.125013223869,-12.64979361445,57.57915534127));
#145193=CARTESIAN_POINT('Ctrl Pts',(96.0004379081691,-13.43109859674,58.22003658354));
#145194=CARTESIAN_POINT('Ctrl Pts',(95.760653910069,-14.28932658605,59.45361215821));
#145195=CARTESIAN_POINT('Ctrl Pts',(95.508664051869,-14.73991191643,60.74998112612));
#145196=CARTESIAN_POINT('Ctrl Pts',(95.3400117127691,-14.82639922299,61.61761786439));
#145197=CARTESIAN_POINT('Ctrl Pts',(95.2660621166691,-14.82530888696,61.99805365762));
#145198=CARTESIAN_POINT('Ctrl Pts',(97.5558858534691,-12.58079776334,56.99230719877));
#145199=CARTESIAN_POINT('Ctrl Pts',(97.5555797012692,-12.58335181252,56.99388220715));
#145200=CARTESIAN_POINT('Ctrl Pts',(97.4977808113692,-13.06476520039,57.2912302344301));
#145201=CARTESIAN_POINT('Ctrl Pts',(97.3580539159691,-13.94156754952,58.01005920855));
#145202=CARTESIAN_POINT('Ctrl Pts',(97.0882075430691,-14.90739617189,59.39829152191));
#145203=CARTESIAN_POINT('Ctrl Pts',(96.8057546118691,-15.41176909157,60.8513786323701));
#145204=CARTESIAN_POINT('Ctrl Pts',(96.6172881371691,-15.50847663767,61.82094975328));
#145205=CARTESIAN_POINT('Ctrl Pts',(96.5345613751691,-15.50723744476,62.2465399249501));
#145206=CARTESIAN_POINT('Ctrl Pts',(98.5620168036692,-12.11465513185,57.94428625613));
#145207=CARTESIAN_POINT('Ctrl Pts',(98.5617532670691,-12.11685372168,57.9456420272201));
#145208=CARTESIAN_POINT('Ctrl Pts',(98.5119999151691,-12.53126450239,58.2015995564401));
#145209=CARTESIAN_POINT('Ctrl Pts',(98.3917523736692,-13.28529239276,58.82021644193));
#145210=CARTESIAN_POINT('Ctrl Pts',(98.1605551479692,-14.11278621153,60.00961712239));
#145211=CARTESIAN_POINT('Ctrl Pts',(97.9172665143691,-14.54800809194,61.2612223934401));
#145212=CARTESIAN_POINT('Ctrl Pts',(97.7542737240691,-14.63157617232,62.0997434229));
#145213=CARTESIAN_POINT('Ctrl Pts',(97.682831166269,-14.63052835456,62.46728168636));
#145214=CARTESIAN_POINT('Ctrl Pts',(98.0436849069692,-11.35329989804,59.07897747768));
#145215=CARTESIAN_POINT('Ctrl Pts',(98.043490974869,-11.3549179127,59.0799751663801));
#145216=CARTESIAN_POINT('Ctrl Pts',(98.0068784773692,-11.6598926921,59.26832919789));
#145217=CARTESIAN_POINT('Ctrl Pts',(97.9184467516692,-12.21339188063,59.72326871723));
#145218=CARTESIAN_POINT('Ctrl Pts',(97.7503755488691,-12.81494213701,60.58791578338));
#145219=CARTESIAN_POINT('Ctrl Pts',(97.5710543385692,-13.13721896131,61.51043883242));
#145220=CARTESIAN_POINT('Ctrl Pts',(97.449667961469,-13.19932622623,62.13491448977));
#145221=CARTESIAN_POINT('Ctrl Pts',(97.3966560026691,-13.19859098334,62.40763601439));
#145222=CARTESIAN_POINT('Origin',(95.9826151700641,-13.4964585873305,61.979706126618));
#145223=CARTESIAN_POINT('Ctrl Pts',(95.682105874569,-14.96190022504,61.8692911014));
#145224=CARTESIAN_POINT('Ctrl Pts',(95.664293696769,-14.96450789965,61.95534281803));
#145225=CARTESIAN_POINT('Ctrl Pts',(95.6496298637692,-14.9654665309,62.04260905828));
#145226=CARTESIAN_POINT('Ctrl Pts',(95.6382530725691,-14.96464552087,62.13064087233));
#145227=CARTESIAN_POINT('Ctrl Pts',(96.8346494067691,-15.21462566969,62.08646545812));
#145228=CARTESIAN_POINT('Ctrl Pts',(96.8206261241691,-15.21734286754,62.15227511246));
#145229=CARTESIAN_POINT('Ctrl Pts',(96.8091979606691,-15.21834430824,62.21938009097));
#145230=CARTESIAN_POINT('Ctrl Pts',(96.8005323646691,-15.21748720413,62.2873715029101));
#145231=CARTESIAN_POINT('Ctrl Pts',(97.6665770469691,-14.37138217867,62.2768002444601));
#145232=CARTESIAN_POINT('Ctrl Pts',(97.6586537487692,-14.3737339414,62.31431226909));
#145233=CARTESIAN_POINT('Ctrl Pts',(97.6521769500692,-14.37459254412,62.35249859934));
#145234=CARTESIAN_POINT('Ctrl Pts',(97.6472313728691,-14.37385587149,62.39113761776));
#145235=CARTESIAN_POINT('Ctrl Pts',(97.4238295483692,-13.19648568652,62.26777600234));
#145236=CARTESIAN_POINT('Ctrl Pts',(97.418788297569,-13.19832828617,62.29458380256));
#145237=CARTESIAN_POINT('Ctrl Pts',(97.4144906416691,-13.19898787182,62.32130596198));
#145238=CARTESIAN_POINT('Ctrl Pts',(97.4109020818691,-13.19841899715,62.34788560615));
#145239=CARTESIAN_POINT('Ctrl Pts',(90.8406504123691,-11.39533572462,57.72321044074));
#145240=CARTESIAN_POINT('Ctrl Pts',(90.8052024597691,-10.89290348004,57.50129529369));
#145241=CARTESIAN_POINT('Ctrl Pts',(90.7750420804691,-10.40751804626,57.29731207447));
#145242=CARTESIAN_POINT('Ctrl Pts',(90.7446611131691,-9.91698402361699,
57.10972154207));
#145243=CARTESIAN_POINT('Ctrl Pts',(92.9567503555691,-11.53858517108,57.4125624132));
#145244=CARTESIAN_POINT('Ctrl Pts',(92.8693838873691,-11.02060249956,57.19158992276));
#145245=CARTESIAN_POINT('Ctrl Pts',(92.7895817403691,-10.54376807816,56.9954777013));
#145246=CARTESIAN_POINT('Ctrl Pts',(92.7150350010691,-10.04738352125,56.81106258288));
#145247=CARTESIAN_POINT('Ctrl Pts',(95.0797166483691,-11.62590813736,57.14090192696));
#145248=CARTESIAN_POINT('Ctrl Pts',(94.9392588749691,-11.10213102618,56.91987534728));
#145249=CARTESIAN_POINT('Ctrl Pts',(94.8096789677691,-10.63281944271,56.72802165784));
#145250=CARTESIAN_POINT('Ctrl Pts',(94.6903690477691,-10.13427439673,56.54465061292));
#145251=CARTESIAN_POINT('Ctrl Pts',(97.2420359135691,-11.67063354251,56.83720086782));
#145252=CARTESIAN_POINT('Ctrl Pts',(97.0468268665691,-11.15380442011,56.6213857415));
#145253=CARTESIAN_POINT('Ctrl Pts',(96.8658778707691,-10.69185373956,56.43600362222));
#145254=CARTESIAN_POINT('Ctrl Pts',(96.6996976194691,-10.19607748941,56.25706068473));
#145255=CARTESIAN_POINT('Origin',(91.5481555916691,0.0433429899084342,83.15732261681));
#145256=CARTESIAN_POINT('',(86.2399318207952,-9.45371065428624,58.8116592805523));
#145257=CARTESIAN_POINT('Ctrl Pts',(87.0626987426128,-9.81003033307946,
57.7183966791295));
#145258=CARTESIAN_POINT('Ctrl Pts',(87.0192701258182,-9.8100014211504,57.7260378243172));
#145259=CARTESIAN_POINT('Ctrl Pts',(86.9763075420885,-9.8089355749407,57.7363696650627));
#145260=CARTESIAN_POINT('Ctrl Pts',(86.9341886174092,-9.80684024658477,
57.7493037322963));
#145261=CARTESIAN_POINT('Ctrl Pts',(86.8920820972307,-9.80474553532679,
57.7622339903005));
#145262=CARTESIAN_POINT('Ctrl Pts',(86.8508191937219,-9.80162196779496,
57.7777648091818));
#145263=CARTESIAN_POINT('Ctrl Pts',(86.8107626708517,-9.79749540496822,
57.7957613018672));
#145264=CARTESIAN_POINT('Ctrl Pts',(86.770702975838,-9.79336851535201,57.8137592197251));
#145265=CARTESIAN_POINT('Ctrl Pts',(86.7318502861524,-9.78823851310647,
57.8342230140293));
#145266=CARTESIAN_POINT('Ctrl Pts',(86.6945462489452,-9.78214922936584,
57.8569736609505));
#145267=CARTESIAN_POINT('Ctrl Pts',(86.6572512799027,-9.77606142585717,
57.879718777462));
#145268=CARTESIAN_POINT('Ctrl Pts',(86.6215046120629,-9.76901487191784,
57.9047493908735));
#145269=CARTESIAN_POINT('Ctrl Pts',(86.587620182679,-9.76107052191038,57.9318457730919));
#145270=CARTESIAN_POINT('Ctrl Pts',(86.5537279197534,-9.75312433529542,
57.9589484195632));
#145271=CARTESIAN_POINT('Ctrl Pts',(86.5216991222089,-9.74428002199653,
57.9881174996962));
#145272=CARTESIAN_POINT('Ctrl Pts',(86.4918147021235,-9.7346146247997,58.0190962830994));
#145273=CARTESIAN_POINT('Ctrl Pts',(86.4639209041257,-9.72559304645865,
58.0480115481104));
#145274=CARTESIAN_POINT('Ctrl Pts',(86.4378952152105,-9.71585634607102,
58.078502889963));
#145275=CARTESIAN_POINT('Ctrl Pts',(86.413935969951,-9.7054786939897,58.1103361914022));
#145276=CARTESIAN_POINT('Ctrl Pts',(86.3881332862203,-9.6943025792323,58.1446187658424));
#145277=CARTESIAN_POINT('Ctrl Pts',(86.3647255207292,-9.68238195554693,
58.1804608615058));
#145278=CARTESIAN_POINT('Ctrl Pts',(86.3439192905833,-9.66982318943558,
58.2175466712203));
#145279=CARTESIAN_POINT('Ctrl Pts',(86.3231146153295,-9.6572653618665,58.2546297094365));
#145280=CARTESIAN_POINT('Ctrl Pts',(86.3049113029344,-9.64406961852703,
58.29295588904));
#145281=CARTESIAN_POINT('Ctrl Pts',(86.2894700249156,-9.63035355780913,
58.3321875341742));
#145282=CARTESIAN_POINT('Ctrl Pts',(86.2740248074335,-9.61663399777479,
58.3714291883004));
#145283=CARTESIAN_POINT('Ctrl Pts',(86.2613431970179,-9.60239399767873,
58.411576361447));
#145284=CARTESIAN_POINT('Ctrl Pts',(86.251537209766,-9.58776045017598,58.4522751389188));
#145285=CARTESIAN_POINT('Ctrl Pts',(86.2417330684947,-9.57312965744369,
58.4929662548314));
#145286=CARTESIAN_POINT('Ctrl Pts',(86.2348035684838,-9.55810561832479,
58.5342083427317));
#145287=CARTESIAN_POINT('Ctrl Pts',(86.2308099331657,-9.54282213213603,
58.5756379736388));
#145288=CARTESIAN_POINT('Ctrl Pts',(86.2268156286862,-9.5275360850929,58.6170745463686));
#145289=CARTESIAN_POINT('Ctrl Pts',(86.225758215939,-9.51199066333907,58.6586982928197));
#145290=CARTESIAN_POINT('Ctrl Pts',(86.2276471137534,-9.49632437130441,
58.7001423158925));
#145291=CARTESIAN_POINT('Ctrl Pts',(86.2293520725841,-9.48218364715038,
58.7375505613668));
#145292=CARTESIAN_POINT('Ctrl Pts',(86.2334567965308,-9.46794459032098,
58.7748121163149));
#145293=CARTESIAN_POINT('Ctrl Pts',(86.2399318207952,-9.45371065428624,
58.8116592805523));
#145294=CARTESIAN_POINT('Origin',(90.5633478388691,0.0433429899084242,83.33097079443));
#145295=CARTESIAN_POINT('Origin',(84.8686633886791,111.0724296188,51.03481040504));
#145296=CARTESIAN_POINT('',(85.8121822997791,-3.09682809692899,56.38577205054));
#145297=CARTESIAN_POINT('Ctrl Pts',(86.2399316748491,-9.45371065431499,
58.81165930621));
#145298=CARTESIAN_POINT('Ctrl Pts',(86.2050308571491,-8.92719465950899,
58.61372693326));
#145299=CARTESIAN_POINT('Ctrl Pts',(86.1286442510291,-7.86795581398499,
58.18051696283));
#145300=CARTESIAN_POINT('Ctrl Pts',(85.9950408985391,-6.11431423260199,
57.42281469856));
#145301=CARTESIAN_POINT('Ctrl Pts',(85.8853720513791,-4.53306565801299,
56.80085176037));
#145302=CARTESIAN_POINT('Ctrl Pts',(85.8329578397391,-3.56074610599299,
56.5035959926));
#145303=CARTESIAN_POINT('Ctrl Pts',(85.8121822997791,-3.09682809692899,
56.38577205054));
#145304=CARTESIAN_POINT('',(85.7414326542391,-3.07748116878498E-13,55.9845308734));
#145305=CARTESIAN_POINT('Ctrl Pts',(85.8121822996917,-3.09682809692899,
56.3857720505554));
#145306=CARTESIAN_POINT('Ctrl Pts',(85.8042550696392,-2.91956454869101,
56.340814494886));
#145307=CARTESIAN_POINT('Ctrl Pts',(85.7970341308756,-2.74414917508697,
56.2998625139189));
#145308=CARTESIAN_POINT('Ctrl Pts',(85.7905101366221,-2.57080491642329,
56.2628631023544));
#145309=CARTESIAN_POINT('Ctrl Pts',(85.7839861423686,-2.39746065775961,
56.2258636907898));
#145310=CARTESIAN_POINT('Ctrl Pts',(85.7781590605377,-2.22618751960296,
56.1928166717312));
#145311=CARTESIAN_POINT('Ctrl Pts',(85.7730109343456,-2.0571911640259,56.1636201991709));
#145312=CARTESIAN_POINT('Ctrl Pts',(85.7725980204189,-2.04363653343167,
56.161278448079));
#145313=CARTESIAN_POINT('Ctrl Pts',(85.7721894698494,-2.03009654045611,
56.1589614427568));
#145314=CARTESIAN_POINT('Ctrl Pts',(85.7717852626336,-2.01657131006667,
56.1566690697222));
#145315=CARTESIAN_POINT('Ctrl Pts',(85.7674981318306,-1.87311906688457,
56.1323555427397));
#145316=CARTESIAN_POINT('Ctrl Pts',(85.7637062630122,-1.73132285554557,
56.1108507779212));
#145317=CARTESIAN_POINT('Ctrl Pts',(85.7603785874086,-1.59087479019068,
56.0919785903473));
#145318=CARTESIAN_POINT('Ctrl Pts',(85.7570556544217,-1.45062689198,56.0731332994906));
#145319=CARTESIAN_POINT('Ctrl Pts',(85.7541955755858,-1.31172299355045,
56.0569129905777));
#145320=CARTESIAN_POINT('Ctrl Pts',(85.7517759592566,-1.17384006401943,
56.0431906681962));
#145321=CARTESIAN_POINT('Ctrl Pts',(85.7506934950497,-1.11215535220779,
56.0370517102819));
#145322=CARTESIAN_POINT('Ctrl Pts',(85.7496993006597,-1.0506747851408,56.0314133550991));
#145323=CARTESIAN_POINT('Ctrl Pts',(85.7487919406473,-0.989368607252711,
56.0262674607562));
#145324=CARTESIAN_POINT('Ctrl Pts',(85.7484214945406,-0.964339253293176,
56.0241665564854));
#145325=CARTESIAN_POINT('Ctrl Pts',(85.7480653344121,-0.93933926649891,
56.0221466717985));
#145326=CARTESIAN_POINT('Ctrl Pts',(85.7477234313339,-0.914369143509711,
56.0202076428128));
#145327=CARTESIAN_POINT('Ctrl Pts',(85.7445918678451,-0.685662441327941,
56.0024476612164));
#145328=CARTESIAN_POINT('Ctrl Pts',(85.7426566455784,-0.459465001269848,
55.9914724733907));
#145329=CARTESIAN_POINT('Ctrl Pts',(85.7418573532768,-0.236281071834248,
55.9869394614726));
#145330=CARTESIAN_POINT('Ctrl Pts',(85.7415739067142,-0.157135160499135,
55.9853319561281));
#145331=CARTESIAN_POINT('Ctrl Pts',(85.7414332766001,-0.0783677830622838,
55.9845344027693));
#145332=CARTESIAN_POINT('Ctrl Pts',(85.7414326542756,-3.07551343926051E-13,
55.9845308733936));
#145333=CARTESIAN_POINT('',(85.8121820990868,3.09687523453428,56.3857703184204));
#145334=CARTESIAN_POINT('Ctrl Pts',(85.7414326542187,-3.07700181072834E-13,
55.9845308734036));
#145335=CARTESIAN_POINT('Ctrl Pts',(85.7414342469354,0.217224571779936,
55.9845399061576));
#145336=CARTESIAN_POINT('Ctrl Pts',(85.7425133790675,0.437429466837711,
55.9906599649905));
#145337=CARTESIAN_POINT('Ctrl Pts',(85.7447232224476,0.660115966676029,
56.0031926097539));
#145338=CARTESIAN_POINT('Ctrl Pts',(85.7456168491695,0.75016696696471,56.0082606188071));
#145339=CARTESIAN_POINT('Ctrl Pts',(85.7466953170994,0.840623293120425,
56.0143769162074));
#145340=CARTESIAN_POINT('Ctrl Pts',(85.7479618986746,0.931450000602351,
56.021560058383));
#145341=CARTESIAN_POINT('Ctrl Pts',(85.7482352910711,0.951055000164376,
56.0231105439517));
#145342=CARTESIAN_POINT('Ctrl Pts',(85.7485174474739,0.970677252051475,
56.0247107325998));
#145343=CARTESIAN_POINT('Ctrl Pts',(85.7488083786006,0.990316494777137,
56.0263606850092));
#145344=CARTESIAN_POINT('Ctrl Pts',(85.750804498331,1.12506412505384,56.037681242545));
#145345=CARTESIAN_POINT('Ctrl Pts',(85.7532186801139,1.26060419693265,56.0513727400778));
#145346=CARTESIAN_POINT('Ctrl Pts',(85.7560682381979,1.39727469347661,56.0675333839879));
#145347=CARTESIAN_POINT('Ctrl Pts',(85.7589245668126,1.53426991819143,56.0837324254781));
#145348=CARTESIAN_POINT('Ctrl Pts',(85.7622183598749,1.67240122844942,56.1024124570235));
#145349=CARTESIAN_POINT('Ctrl Pts',(85.765975812552,1.81199514782755,56.123722035509));
#145350=CARTESIAN_POINT('Ctrl Pts',(85.7678064767031,1.88000653902479,56.1341042504728));
#145351=CARTESIAN_POINT('Ctrl Pts',(85.7697473312333,1.94836487803584,56.1451113863991));
#145352=CARTESIAN_POINT('Ctrl Pts',(85.7718021388295,2.01710641374184,56.1567647793634));
#145353=CARTESIAN_POINT('Ctrl Pts',(85.7723664816671,2.03598593968704,56.1599653266389));
#145354=CARTESIAN_POINT('Ctrl Pts',(85.772939283409,2.05489449159769,56.1632138465122));
#145355=CARTESIAN_POINT('Ctrl Pts',(85.7735205983484,2.07383170835384,56.1665106470066));
#145356=CARTESIAN_POINT('Ctrl Pts',(85.7786559456038,2.24112344215451,56.1956346454168));
#145357=CARTESIAN_POINT('Ctrl Pts',(85.7844563508405,2.41065351637206,56.2285303729545));
#145358=CARTESIAN_POINT('Ctrl Pts',(85.7909391303511,2.58220810972347,56.2652960441803));
#145359=CARTESIAN_POINT('Ctrl Pts',(85.7973499416829,2.75185820028397,56.3016535635632));
#145360=CARTESIAN_POINT('Ctrl Pts',(85.8044280722384,2.92348806511701,56.3417956397942));
#145361=CARTESIAN_POINT('Ctrl Pts',(85.8121819977014,3.09687523453422,56.3857703362983));
#145362=CARTESIAN_POINT('',(86.2399778829169,9.45364604184037,58.8119255183517));
#145363=CARTESIAN_POINT('Ctrl Pts',(85.8121821021391,3.09687523453501,56.38577031788));
#145364=CARTESIAN_POINT('Ctrl Pts',(85.8156355274938,3.1740050849032,56.4053562795853));
#145365=CARTESIAN_POINT('Ctrl Pts',(85.822202833005,3.31500708348416,56.4426013199344));
#145366=CARTESIAN_POINT('Ctrl Pts',(85.829686486828,3.46655241282912,56.4850432298054));
#145367=CARTESIAN_POINT('Ctrl Pts',(85.8341872722727,3.55573178407053,56.5105684524717));
#145368=CARTESIAN_POINT('Ctrl Pts',(85.8354069598104,3.5797232594888,56.5174856442303));
#145369=CARTESIAN_POINT('Ctrl Pts',(85.8430146168074,3.7284293012332,56.5606308110469));
#145370=CARTESIAN_POINT('Ctrl Pts',(85.8495034720024,3.85058241988637,56.5974309375446));
#145371=CARTESIAN_POINT('Ctrl Pts',(85.8581126207165,4.00637430763456,56.6462558461291));
#145372=CARTESIAN_POINT('Ctrl Pts',(85.8603552199655,4.04638499592307,56.6589742584787));
#145373=CARTESIAN_POINT('Ctrl Pts',(85.8783041873205,4.3623958073411,56.7607679107204));
#145374=CARTESIAN_POINT('Ctrl Pts',(85.8963538313168,4.65690735461759,56.8631325285659));
#145375=CARTESIAN_POINT('Ctrl Pts',(85.9172071280309,4.97600702371672,56.9813974511006));
#145376=CARTESIAN_POINT('Ctrl Pts',(85.9179810042478,4.98782294542579,56.9857863212208));
#145377=CARTESIAN_POINT('Ctrl Pts',(85.9354066199147,5.25345961164944,57.0846118985475));
#145378=CARTESIAN_POINT('Ctrl Pts',(85.9545355436378,5.53172004014412,57.1930974158877));
#145379=CARTESIAN_POINT('Ctrl Pts',(85.9762431292321,5.83552461324838,57.3162072514163));
#145380=CARTESIAN_POINT('Ctrl Pts',(85.9766657534864,5.84143542331735,57.3186040726661));
#145381=CARTESIAN_POINT('Ctrl Pts',(85.9932700223378,6.07355818889181,57.4127715607314));
#145382=CARTESIAN_POINT('Ctrl Pts',(86.0125400581796,6.33673275251046,57.5220573646636));
#145383=CARTESIAN_POINT('Ctrl Pts',(86.0349080414051,6.63690299677357,57.6489125012727));
#145384=CARTESIAN_POINT('Ctrl Pts',(86.0352247765358,6.64115272418706,57.650708795461));
#145385=CARTESIAN_POINT('Ctrl Pts',(86.0394882418842,6.69835306693705,57.6748881089797));
#145386=CARTESIAN_POINT('Ctrl Pts',(86.0580652377802,6.94590676687942,57.7802434880673));
#145387=CARTESIAN_POINT('Ctrl Pts',(86.09124831534,7.38771230747788,57.9684340725516));
#145388=CARTESIAN_POINT('Ctrl Pts',(86.0916010803591,7.39240906229862,57.970434702391));
#145389=CARTESIAN_POINT('Ctrl Pts',(86.112649716,7.67265227052037,58.0898074470287));
#145390=CARTESIAN_POINT('Ctrl Pts',(86.1300138532744,7.90547540138447,58.1882843630672));
#145391=CARTESIAN_POINT('Ctrl Pts',(86.1443085918483,8.09917346504611,58.2693538540572));
#145392=CARTESIAN_POINT('Ctrl Pts',(86.1446022539483,8.10315349725212,58.2710192945862));
#145393=CARTESIAN_POINT('Ctrl Pts',(86.1828731263993,8.62218252871381,58.4880641977383));
#145394=CARTESIAN_POINT('Ctrl Pts',(86.2144528885248,9.06971500218893,58.6671619285489));
#145395=CARTESIAN_POINT('Ctrl Pts',(86.2399778829169,9.45364604184037,58.8119255183517));
#145396=CARTESIAN_POINT('Origin',(90.5633473677691,-0.0433423696915958,
83.33096812237));
#145397=CARTESIAN_POINT('',(87.2268073772291,-13.97255334344,64.408496138118));
#145398=CARTESIAN_POINT('Origin',(85.7495940118791,-15.20679038041,64.668971957449));
#145399=CARTESIAN_POINT('',(86.0102742699191,-13.59507145206,66.146140280904));
#145400=CARTESIAN_POINT('Origin',(87.4872779078691,111.0724296188,65.885711320467));
#145401=CARTESIAN_POINT('',(69.2683344771691,-3.46410161513799,69.098202607305));
#145402=CARTESIAN_POINT('',(69.2686179994291,13.59506703911,69.098152483414));
#145403=CARTESIAN_POINT('Origin',(69.5288067436691,15.14946593626,70.575414236823));
#145404=CARTESIAN_POINT('',(68.051595113123,15.14946593626,70.8358864974945));
#145405=CARTESIAN_POINT('Origin',(67.7911228476491,111.0724296188,69.358674873805));
#145406=CARTESIAN_POINT('Origin',(74.4243048522391,1.4210854715202E-14,
66.665926000619));
#145407=CARTESIAN_POINT('Origin',(74.0770084968991,1.4210854715202E-14,
64.696310494595));
#145408=CARTESIAN_POINT('',(64.805817992169,1.27380650104997,66.3310715238674));
#145409=CARTESIAN_POINT('',(64.805817992169,-1.27380650104994,66.3310715238674));
#145410=CARTESIAN_POINT('Origin',(74.0770084968991,1.4210854715202E-14,
64.696310494595));
#145411=CARTESIAN_POINT('',(64.8058179921691,-1.27380650101999,66.331071523868));
#145412=CARTESIAN_POINT('Origin',(66.2853705616391,-11.87963525096,66.577899792436));
#145413=CARTESIAN_POINT('',(66.0249519193982,-6.80058507386928,65.1006787085175));
#145414=CARTESIAN_POINT('',(66.0248982949952,-5.12347538298166,65.100688162132));
#145415=CARTESIAN_POINT('',(66.0248749202791,-6.80071698562199,65.100691123259));
#145416=CARTESIAN_POINT('',(64.8081589327399,-6.16441400339199,66.8383720624473));
#145417=CARTESIAN_POINT('Ctrl Pts',(64.8081589327399,-6.16441400339199,
66.8383720624473));
#145418=CARTESIAN_POINT('Ctrl Pts',(64.8018782379671,-6.16444558364484,
66.802752472863));
#145419=CARTESIAN_POINT('Ctrl Pts',(64.7966397238661,-6.16496886332639,
66.7654979979585));
#145420=CARTESIAN_POINT('Ctrl Pts',(64.7927790828751,-6.16617417900185,
66.726798004383));
#145421=CARTESIAN_POINT('Ctrl Pts',(64.7890472955959,-6.16733926576218,
66.6893896713979));
#145422=CARTESIAN_POINT('Ctrl Pts',(64.7866035704855,-6.16914162068152,
66.6506309119591));
#145423=CARTESIAN_POINT('Ctrl Pts',(64.7857300260124,-6.17175315117691,
66.6107367214207));
#145424=CARTESIAN_POINT('Ctrl Pts',(64.7848703921967,-6.17432309465844,
66.5714778212829));
#145425=CARTESIAN_POINT('Ctrl Pts',(64.7855319205551,-6.17767664766678,
66.531119607349));
#145426=CARTESIAN_POINT('Ctrl Pts',(64.7879536899489,-6.18197763514565,
66.4899071087765));
#145427=CARTESIAN_POINT('Ctrl Pts',(64.7903316449724,-6.18620080965898,
66.4494402219379));
#145428=CARTESIAN_POINT('Ctrl Pts',(64.7944071927674,-6.19133744700491,
66.408150068017));
#145429=CARTESIAN_POINT('Ctrl Pts',(64.8003699641285,-6.19754264031923,
66.3663029460676));
#145430=CARTESIAN_POINT('Ctrl Pts',(64.802891495943,-6.20016668732857,66.3486066697974));
#145431=CARTESIAN_POINT('Ctrl Pts',(64.805750019028,-6.20298182077583,66.3308111840328));
#145432=CARTESIAN_POINT('Ctrl Pts',(64.8089575523694,-6.20599976913376,
66.3129382366224));
#145433=CARTESIAN_POINT('Ctrl Pts',(64.8175795013529,-6.21411210780888,
66.264895200321));
#145434=CARTESIAN_POINT('Ctrl Pts',(64.8287186518659,-6.22341884736779,
66.2163193093983));
#145435=CARTESIAN_POINT('Ctrl Pts',(64.8426026562989,-6.23382808779138,
66.1675087943377));
#145436=CARTESIAN_POINT('Ctrl Pts',(64.844338156853,-6.23512924284433,66.1614074799551));
#145437=CARTESIAN_POINT('Ctrl Pts',(64.8461166196411,-6.23644769982519,
66.155302198922));
#145438=CARTESIAN_POINT('Ctrl Pts',(64.8479385087963,-6.23778316422518,
66.1491934903362));
#145439=CARTESIAN_POINT('Ctrl Pts',(64.8492890733101,-6.23877314257979,
66.1446651110888));
#145440=CARTESIAN_POINT('Ctrl Pts',(64.8508084707658,-6.23987842321675,
66.139666922722));
#145441=CARTESIAN_POINT('Ctrl Pts',(64.8520035489644,-6.24073954596106,
66.1357923315445));
#145442=CARTESIAN_POINT('Ctrl Pts',(64.8524206114576,-6.24104006353311,
66.1344401634116));
#145443=CARTESIAN_POINT('Ctrl Pts',(64.8527976450016,-6.24131084525289,
66.1332246742856));
#145444=CARTESIAN_POINT('Ctrl Pts',(64.8531123985251,-6.24153661316581,
66.132213182593));
#145445=CARTESIAN_POINT('Ctrl Pts',(64.8555457363169,-6.24328200933677,
66.1243934100468));
#145446=CARTESIAN_POINT('Ctrl Pts',(64.8581071814899,-6.24508366804847,
66.1163875900722));
#145447=CARTESIAN_POINT('Ctrl Pts',(64.860805733643,-6.24694729562907,66.1082030276649));
#145448=CARTESIAN_POINT('Ctrl Pts',(64.866202837949,-6.25067455079026,66.0918339028505));
#145449=CARTESIAN_POINT('Ctrl Pts',(64.8721481952012,-6.25464968142705,
66.0747497098203));
#145450=CARTESIAN_POINT('Ctrl Pts',(64.8787136065186,-6.25890835103562,
66.0570195656937));
#145451=CARTESIAN_POINT('Ctrl Pts',(64.8890331042377,-6.26560211768438,
66.0291513677959));
#145452=CARTESIAN_POINT('Ctrl Pts',(64.9008837340019,-6.27302883205694,
65.9996869371169));
#145453=CARTESIAN_POINT('Ctrl Pts',(64.9145547240413,-6.28129575024242,
65.9689137996651));
#145454=CARTESIAN_POINT('Ctrl Pts',(64.9277534687516,-6.28927709924174,
65.939203677429));
#145455=CARTESIAN_POINT('Ctrl Pts',(64.9426498964942,-6.29804160729299,
65.9082737349583));
#145456=CARTESIAN_POINT('Ctrl Pts',(64.9594971235488,-6.30768579498066,
65.8764301735881));
#145457=CARTESIAN_POINT('Ctrl Pts',(64.9696076707388,-6.31347357325478,
65.8573198577546));
#145458=CARTESIAN_POINT('Ctrl Pts',(64.9804206152209,-6.31957817474758,
65.8378814163225));
#145459=CARTESIAN_POINT('Ctrl Pts',(64.9919872957414,-6.32602046158861,
65.8181895006169));
#145460=CARTESIAN_POINT('Ctrl Pts',(65.010333486147,-6.33623872782528,65.7869556790943));
#145461=CARTESIAN_POINT('Ctrl Pts',(65.0305763187481,-6.34730016361858,
65.7550828730331));
#145462=CARTESIAN_POINT('Ctrl Pts',(65.0529182172327,-6.35923156460288,
65.7228786121327));
#145463=CARTESIAN_POINT('Ctrl Pts',(65.0615104126933,-6.36382011509899,
65.7104935722262));
#145464=CARTESIAN_POINT('Ctrl Pts',(65.0704128213947,-6.36853733343909,
65.6980599905497));
#145465=CARTESIAN_POINT('Ctrl Pts',(65.0796359212282,-6.373384743733,65.6855971661296));
#145466=CARTESIAN_POINT('Ctrl Pts',(65.0879372988571,-6.377747721918,65.6743798299085));
#145467=CARTESIAN_POINT('Ctrl Pts',(65.096924391596,-6.38244554878342,65.6625720000334));
#145468=CARTESIAN_POINT('Ctrl Pts',(65.106284192454,-6.38730345565473,65.6506698673355));
#145469=CARTESIAN_POINT('Ctrl Pts',(65.1149591713286,-6.39180592746183,
65.6396385696313));
#145470=CARTESIAN_POINT('Ctrl Pts',(65.1239539050347,-6.39644591130927,
65.6285262888787));
#145471=CARTESIAN_POINT('Ctrl Pts',(65.1329773043374,-6.40108426173598,
65.6176968032063));
#145472=CARTESIAN_POINT('Ctrl Pts',(65.1336896313987,-6.40145042335839,
65.6168418996999));
#145473=CARTESIAN_POINT('Ctrl Pts',(65.1344021162251,-6.40181657480153,
65.6159887414984));
#145474=CARTESIAN_POINT('Ctrl Pts',(65.1351146049841,-6.40218264761172,
65.6151374987312));
#145475=CARTESIAN_POINT('Ctrl Pts',(65.1545904777191,-6.41218924402872,
65.59186878664));
#145476=CARTESIAN_POINT('Ctrl Pts',(65.174534446433,-6.42233208182421,65.5694744033257));
#145477=CARTESIAN_POINT('Ctrl Pts',(65.1948880277455,-6.43256527208665,
65.5479251115468));
#145478=CARTESIAN_POINT('Ctrl Pts',(65.2282806527171,-6.44935411526127,
65.5125707722916));
#145479=CARTESIAN_POINT('Ctrl Pts',(65.2627791595159,-6.46636865768246,
65.4794863823339));
#145480=CARTESIAN_POINT('Ctrl Pts',(65.2981340375824,-6.48349628267055,
65.4485796227903));
#145481=CARTESIAN_POINT('Ctrl Pts',(65.3349584684363,-6.50133583060725,
65.4163881999382));
#145482=CARTESIAN_POINT('Ctrl Pts',(65.3727120202401,-6.51929805721341,
65.3865585271715));
#145483=CARTESIAN_POINT('Ctrl Pts',(65.4111687378838,-6.53725571101636,
65.3589776573745));
#145484=CARTESIAN_POINT('Ctrl Pts',(65.4258093262544,-6.54409224396922,
65.3484775370746));
#145485=CARTESIAN_POINT('Ctrl Pts',(65.4405523805545,-6.55092811416381,
65.3383033134471));
#145486=CARTESIAN_POINT('Ctrl Pts',(65.4553873823056,-6.55775630023164,
65.3284487441658));
#145487=CARTESIAN_POINT('Ctrl Pts',(65.5009941420158,-6.57874796888649,
65.2981531647785));
#145488=CARTESIAN_POINT('Ctrl Pts',(65.5474757338804,-6.59965827117149,
65.2708737574508));
#145489=CARTESIAN_POINT('Ctrl Pts',(65.5944928291456,-6.62040649357933,
65.2464765093496));
#145490=CARTESIAN_POINT('Ctrl Pts',(65.641450338879,-6.64112842142649,65.2221101802788));
#145491=CARTESIAN_POINT('Ctrl Pts',(65.6889424427869,-6.66168867994912,
65.2006179488416));
#145492=CARTESIAN_POINT('Ctrl Pts',(65.7366880486402,-6.68200686211981,
65.181852694402));
#145493=CARTESIAN_POINT('Ctrl Pts',(65.786825709474,-6.70334298527137,65.162147300665));
#145494=CARTESIAN_POINT('Ctrl Pts',(65.837243007763,-6.72441216840512,65.1454483117514));
#145495=CARTESIAN_POINT('Ctrl Pts',(65.8876737008058,-6.74512130373806,
65.1315812912464));
#145496=CARTESIAN_POINT('Ctrl Pts',(65.9334751418892,-6.76392945775325,
65.1189871846748));
#145497=CARTESIAN_POINT('Ctrl Pts',(65.9792887073989,-6.78244063083012,
65.1087286556775));
#145498=CARTESIAN_POINT('Ctrl Pts',(66.0249519193982,-6.80058507386928,
65.1006787085175));
#145499=CARTESIAN_POINT('',(64.8081615004591,6.16441400309888,66.8383716061749));
#145500=CARTESIAN_POINT('',(64.8081632946491,-6.16441400339199,66.838371293325));
#145501=CARTESIAN_POINT('',(66.0248982951649,6.80073525439801,65.1006881629131));
#145502=CARTESIAN_POINT('Ctrl Pts',(64.8081589321389,6.16441400309901,66.8383720590391));
#145503=CARTESIAN_POINT('Ctrl Pts',(64.7987827821794,6.16441838682887,66.7851972702575));
#145504=CARTESIAN_POINT('Ctrl Pts',(64.7921811970201,6.16585112404424,66.7309524641975));
#145505=CARTESIAN_POINT('Ctrl Pts',(64.7885778066817,6.16871221474511,66.6759377886771));
#145506=CARTESIAN_POINT('Ctrl Pts',(64.785040627147,6.17152073409038,66.6219339850137));
#145507=CARTESIAN_POINT('Ctrl Pts',(64.7843928677463,6.17570559836315,66.567188560321));
#145508=CARTESIAN_POINT('Ctrl Pts',(64.786817703994,6.18126680756346,66.5120261797856));
#145509=CARTESIAN_POINT('Ctrl Pts',(64.7891026366133,6.18650715660429,66.4600464542408));
#145510=CARTESIAN_POINT('Ctrl Pts',(64.7941159419607,6.19296961269943,66.407696948985));
#145511=CARTESIAN_POINT('Ctrl Pts',(64.8019823066183,6.20065417584886,66.3552806448622));
#145512=CARTESIAN_POINT('Ctrl Pts',(64.8101411712435,6.20862447892643,66.3009153124495));
#145513=CARTESIAN_POINT('Ctrl Pts',(64.8213698492503,6.21790946351572,66.246478174084));
#145514=CARTESIAN_POINT('Ctrl Pts',(64.8357695591531,6.22850912961671,66.1923392477849));
#145515=CARTESIAN_POINT('Ctrl Pts',(64.8499503796991,6.23894767065946,66.1390232849235));
#145516=CARTESIAN_POINT('Ctrl Pts',(64.8672068571494,6.25066122816447,66.085996883417));
#145517=CARTESIAN_POINT('Ctrl Pts',(64.8875930217995,6.26364980213172,66.0336407097191));
#145518=CARTESIAN_POINT('Ctrl Pts',(64.8935435202088,6.26744102476029,66.0183585154636));
#145519=CARTESIAN_POINT('Ctrl Pts',(64.8997603692193,6.2713408778002,66.0031335845166));
#145520=CARTESIAN_POINT('Ctrl Pts',(64.9062441577029,6.27534936125144,65.9879757617626));
#145521=CARTESIAN_POINT('Ctrl Pts',(64.9147863329762,6.28063040462715,65.9680058353756));
#145522=CARTESIAN_POINT('Ctrl Pts',(64.9237918809422,6.28609999981175,65.9481523759262));
#145523=CARTESIAN_POINT('Ctrl Pts',(64.9332611821828,6.29175814680523,65.9284383032111));
#145524=CARTESIAN_POINT('Ctrl Pts',(64.9379958328031,6.29458722030197,65.9185812668535));
#145525=CARTESIAN_POINT('Ctrl Pts',(64.942846410463,6.29746343175093,65.90875907166));
#145526=CARTESIAN_POINT('Ctrl Pts',(64.9478128497735,6.30038678115212,65.8989746364514));
#145527=CARTESIAN_POINT('Ctrl Pts',(64.9502960694287,6.30184845585272,65.894082418847));
#145528=CARTESIAN_POINT('Ctrl Pts',(64.9528082537229,6.30332191504137,65.8891996408788));
#145529=CARTESIAN_POINT('Ctrl Pts',(64.9553493886184,6.30480715871807,65.8843266677285));
#145530=CARTESIAN_POINT('Ctrl Pts',(64.9571933289268,6.30588490578621,65.8807906603997));
#145531=CARTESIAN_POINT('Ctrl Pts',(64.9594293287966,6.30718965479531,65.876547760901));
#145532=CARTESIAN_POINT('Ctrl Pts',(64.9612383475702,6.30824075099125,65.8731488579457));
#145533=CARTESIAN_POINT('Ctrl Pts',(64.9619223383106,6.30863817089411,65.8718637313441));
#145534=CARTESIAN_POINT('Ctrl Pts',(64.9625447294431,6.30899932861105,65.8706989672381));
#145535=CARTESIAN_POINT('Ctrl Pts',(64.9630596273281,6.30929824321235,65.8697375278373));
#145536=CARTESIAN_POINT('Ctrl Pts',(64.9746693744909,6.31603807075048,65.848059310308));
#145537=CARTESIAN_POINT('Ctrl Pts',(64.9876834635193,6.32365695723595,65.8250329634241));
#145538=CARTESIAN_POINT('Ctrl Pts',(65.0023383654708,6.33215490266875,65.80083584166));
#145539=CARTESIAN_POINT('Ctrl Pts',(65.0166474478898,6.34045231755374,65.7772097122753));
#145540=CARTESIAN_POINT('Ctrl Pts',(65.0325214116991,6.34958779363933,65.7524671037607));
#145541=CARTESIAN_POINT('Ctrl Pts',(65.0501936356578,6.35956133092553,65.7268193253099));
#145542=CARTESIAN_POINT('Ctrl Pts',(65.0674105003129,6.36927788057936,65.7018324118733));
#145543=CARTESIAN_POINT('Ctrl Pts',(65.0863347707334,6.37978985929114,65.6759861648845));
#145544=CARTESIAN_POINT('Ctrl Pts',(65.1071861193518,6.39109726706087,65.6495241034221));
#145545=CARTESIAN_POINT('Ctrl Pts',(65.1274779738104,6.40210126862294,65.6237720856654));
#145546=CARTESIAN_POINT('Ctrl Pts',(65.1495955070102,6.41385858521217,65.5974367512891));
#145547=CARTESIAN_POINT('Ctrl Pts',(65.1737357905544,6.42636921682857,65.5707909920993));
#145548=CARTESIAN_POINT('Ctrl Pts',(65.1972228978337,6.4385413417486,65.5448662011383));
#145549=CARTESIAN_POINT('Ctrl Pts',(65.2226253937009,6.45142656752832,65.5186475517802));
#145550=CARTESIAN_POINT('Ctrl Pts',(65.2501105477758,6.46502489416772,65.4924336696594));
#145551=CARTESIAN_POINT('Ctrl Pts',(65.2765224236187,6.4780922145798,65.4672434233886));
#145552=CARTESIAN_POINT('Ctrl Pts',(65.3048580009356,6.4918180309331,65.4420577603538));
#145553=CARTESIAN_POINT('Ctrl Pts',(65.3352442528554,6.50620234322766,65.4171844968716));
#145554=CARTESIAN_POINT('Ctrl Pts',(65.364957714832,6.5202681687053,65.3928619588152));
#145555=CARTESIAN_POINT('Ctrl Pts',(65.3966325957644,6.53496365308086,65.3688382857725));
#145556=CARTESIAN_POINT('Ctrl Pts',(65.4303588502056,6.55028879635433,65.3454408789985));
#145557=CARTESIAN_POINT('Ctrl Pts',(65.4630069700259,6.56512403738972,65.3227914222919));
#145558=CARTESIAN_POINT('Ctrl Pts',(65.4975778418086,6.58054932388348,65.3007291172199));
#145559=CARTESIAN_POINT('Ctrl Pts',(65.5341187593121,6.59656465583564,65.2795852198071));
#145560=CARTESIAN_POINT('Ctrl Pts',(65.5552586448087,6.60582994819253,65.2673529169315));
#145561=CARTESIAN_POINT('Ctrl Pts',(65.5770572174507,6.61529272451413,65.255428621325));
#145562=CARTESIAN_POINT('Ctrl Pts',(65.5995172355066,6.62495298480042,65.2438813461494));
#145563=CARTESIAN_POINT('Ctrl Pts',(65.6367046710099,6.64094764274979,65.2247623254182));
#145564=CARTESIAN_POINT('Ctrl Pts',(65.6757078881928,6.65748368305192,65.2066757042188));
#145565=CARTESIAN_POINT('Ctrl Pts',(65.7165057812049,6.6745611057068,65.1899542381791));
#145566=CARTESIAN_POINT('Ctrl Pts',(65.7565231187389,6.69131179884646,65.1735526914037));
#145567=CARTESIAN_POINT('Ctrl Pts',(65.7982674702529,6.70858335678332,65.1584649442466));
#145568=CARTESIAN_POINT('Ctrl Pts',(65.8416731700358,6.72637577951738,65.1450241437196));
#145569=CARTESIAN_POINT('Ctrl Pts',(65.8839311284249,6.7436977317794,65.1319387472803));
#145570=CARTESIAN_POINT('Ctrl Pts',(65.927763957186,6.76151336741847,65.120414793424));
#145571=CARTESIAN_POINT('Ctrl Pts',(65.9730632002797,6.77982268643461,65.1107719479587));
#145572=CARTESIAN_POINT('Ctrl Pts',(65.9901363495624,6.78672341402914,65.1071375883337));
#145573=CARTESIAN_POINT('Ctrl Pts',(66.007417292501,6.79369427001695,65.1037705353322));
#145574=CARTESIAN_POINT('Ctrl Pts',(66.0248982951649,6.80073525439801,65.1006881629131));
#145575=CARTESIAN_POINT('',(66.0248982950042,5.12347538298277,65.1006881621786));
#145576=CARTESIAN_POINT('',(66.0248982951391,5.12347538298101,65.100688162917));
#145577=CARTESIAN_POINT('Ctrl Pts',(66.0248982951388,5.12347538298986,65.1006881629177));
#145578=CARTESIAN_POINT('Ctrl Pts',(65.5457633364347,4.36379356331096,65.1851725835393));
#145579=CARTESIAN_POINT('Ctrl Pts',(65.2016180936169,3.51046595110393,65.471515880299));
#145580=CARTESIAN_POINT('Ctrl Pts',(64.9003152941216,2.17972224640472,65.9694338758958));
#145581=CARTESIAN_POINT('Ctrl Pts',(64.8358888771522,1.72400278119682,66.1508188509989));
#145582=CARTESIAN_POINT('Ctrl Pts',(64.8058179921649,1.27380650105203,66.3310715238719));
#145583=CARTESIAN_POINT('Ctrl Pts',(64.8058179921649,-1.27380650105201,
66.3310715238719));
#145584=CARTESIAN_POINT('Ctrl Pts',(64.8358888771522,-1.72400278119679,
66.1508188509989));
#145585=CARTESIAN_POINT('Ctrl Pts',(64.9003152941216,-2.17972224640469,
65.9694338758958));
#145586=CARTESIAN_POINT('Ctrl Pts',(65.2016180936169,-3.5104659511039,65.471515880299));
#145587=CARTESIAN_POINT('Ctrl Pts',(65.5457633364338,-4.36379356331136,
65.185172583538));
#145588=CARTESIAN_POINT('Ctrl Pts',(66.0248982951388,-5.12347538298983,
65.1006881629177));
#145589=CARTESIAN_POINT('Origin',(71.6139524734691,1.4210854715202E-14,
50.72762564822));
#145590=CARTESIAN_POINT('',(83.2590339728491,-3.72445119722915E-6,62.06184505375));
#145591=CARTESIAN_POINT('Origin',(73.9033603192391,1.4210854715202E-14,
63.711502741582));
#145592=CARTESIAN_POINT('Origin',(73.9033603192391,1.4210854715202E-14,
63.711502741582));
#145593=CARTESIAN_POINT('Origin',(73.9033603192391,1.4210854715202E-14,
63.711502741582));
#145594=CARTESIAN_POINT('',(83.2590347531395,-6.98291828557661,62.0618512036248));
#145595=CARTESIAN_POINT('',(83.2590347341691,-6.98291575896899,62.06184938817));
#145596=CARTESIAN_POINT('',(81.0965926396278,-7.61327390186262,62.4431418050118));
#145597=CARTESIAN_POINT('Origin',(82.7666300963491,-9.38083151964699,62.14866914261));
#145598=CARTESIAN_POINT('',(67.5092874005591,-8.31611745004299,64.838950313787));
#145599=CARTESIAN_POINT('Origin',(73.9033603192391,1.4210854715202E-14,
63.711502741607));
#145600=CARTESIAN_POINT('',(66.2209546742975,-7.02799158729797,65.0661181389945));
#145601=CARTESIAN_POINT('Ctrl Pts',(66.2209546733633,-7.02799158729799,
65.0661181336967));
#145602=CARTESIAN_POINT('Ctrl Pts',(66.3246656027716,-7.14505369148099,
65.0478310986477));
#145603=CARTESIAN_POINT('Ctrl Pts',(66.4234442496545,-7.25629879530099,
65.0304137580844));
#145604=CARTESIAN_POINT('Ctrl Pts',(66.5178883954126,-7.36052989680883,
65.0137607070173));
#145605=CARTESIAN_POINT('Ctrl Pts',(66.6123325411707,-7.46476099831666,
64.9971076559501));
#145606=CARTESIAN_POINT('Ctrl Pts',(66.702442185804,-7.56197809751232,64.9812188943793));
#145607=CARTESIAN_POINT('Ctrl Pts',(66.7896495528575,-7.65283723712582,
64.9658418826512));
#145608=CARTESIAN_POINT('Ctrl Pts',(66.876856919911,-7.74369637673932,64.9504648709231));
#145609=CARTESIAN_POINT('Ctrl Pts',(66.9611620093849,-7.82819755677066,
64.9355996090378));
#145610=CARTESIAN_POINT('Ctrl Pts',(67.0429998000091,-7.90686402925032,
64.9211693985092));
#145611=CARTESIAN_POINT('Ctrl Pts',(67.1248375906334,-7.98553050172999,
64.9067391879805));
#145612=CARTESIAN_POINT('Ctrl Pts',(67.2042080824082,-8.05836226665799,
64.8927440288086));
#145613=CARTESIAN_POINT('Ctrl Pts',(67.2818820035575,-8.12639721364099,
64.8790480208125));
#145614=CARTESIAN_POINT('Ctrl Pts',(67.3595559247068,-8.19443216062399,
64.8653520128165));
#145615=CARTESIAN_POINT('Ctrl Pts',(67.4355332752307,-8.25767028966199,
64.8519551559964));
#145616=CARTESIAN_POINT('Ctrl Pts',(67.5092874005549,-8.31611745004299,
64.8389503137632));
#145617=CARTESIAN_POINT('Origin',(73.9033603209991,1.4210854715202E-14,
63.711502751597));
#145618=CARTESIAN_POINT('Origin',(73.9033603192391,1.4210854715202E-14,
63.711502741582));
#145619=CARTESIAN_POINT('',(66.2208875197039,7.02805194586377,65.0661299774239));
#145620=CARTESIAN_POINT('Origin',(73.9033603203091,1.4210854715202E-14,
63.711502747645));
#145621=CARTESIAN_POINT('',(67.5092801231572,8.31611453423868,64.8389516048533));
#145622=CARTESIAN_POINT('Ctrl Pts',(66.2208657833691,7.02807183034301,65.066133808363));
#145623=CARTESIAN_POINT('Ctrl Pts',(66.4309100471391,7.26505475676601,65.029097337517));
#145624=CARTESIAN_POINT('Ctrl Pts',(66.8419704590391,7.72821672095301,64.956616290815));
#145625=CARTESIAN_POINT('Ctrl Pts',(67.2799358526991,8.13398401787701,64.879391187598));
#145626=CARTESIAN_POINT('Ctrl Pts',(67.5092801218091,8.31611453424001,64.838951597214));
#145627=CARTESIAN_POINT('',(81.0965921351133,7.61327336788956,62.4431418939603));
#145628=CARTESIAN_POINT('Origin',(73.9033603192391,1.4210854715202E-14,
63.711502741594));
#145629=CARTESIAN_POINT('',(83.2590339201892,6.98291692033359,62.0618459037933));
#145630=CARTESIAN_POINT('Origin',(82.7666300963491,9.38083151964701,62.14866914259));
#145631=CARTESIAN_POINT('',(83.2590339728491,-8.07105361845785E-10,62.06184505375));
#145632=CARTESIAN_POINT('Origin',(74.0770084968991,1.4210854715202E-14,
64.696310494594));
#145633=CARTESIAN_POINT('',(65.6628224406878,-7.69741850331449,66.1799585170539));
#145634=CARTESIAN_POINT('Origin',(66.3946016642385,-7.02812664320015,66.0509721790387));
#145635=CARTESIAN_POINT('',(65.4482167555244,-7.44842431834834,66.2177992895134));
#145636=CARTESIAN_POINT('Origin',(74.0770084968991,1.4210854715202E-14,
64.696310494594));
#145637=CARTESIAN_POINT('Origin',(66.1985464660391,-6.80073524628799,66.085495917122));
#145638=CARTESIAN_POINT('Ctrl Pts',(65.1021721393592,-6.87149439123999,
66.825730951951));
#145639=CARTESIAN_POINT('Ctrl Pts',(65.0984324276291,-6.86890400994998,
66.81588333904));
#145640=CARTESIAN_POINT('Ctrl Pts',(65.0923058811291,-6.86568651314798,
66.795286809766));
#145641=CARTESIAN_POINT('Ctrl Pts',(65.0880224526391,-6.86745667141899,
66.7631974852071));
#145642=CARTESIAN_POINT('Ctrl Pts',(65.0892419555591,-6.87754968651898,
66.72582778172));
#145643=CARTESIAN_POINT('Ctrl Pts',(65.0975331340091,-6.89813731240698,
66.682874279271));
#145644=CARTESIAN_POINT('Ctrl Pts',(65.1141392786591,-6.93040430719099,
66.635952050429));
#145645=CARTESIAN_POINT('Ctrl Pts',(65.1393962274192,-6.97394855130398,
66.5877397397371));
#145646=CARTESIAN_POINT('Ctrl Pts',(65.1730883139991,-7.02767577688599,
66.540401613751));
#145647=CARTESIAN_POINT('Ctrl Pts',(65.2156473534191,-7.09157262362899,
66.494759786697));
#145648=CARTESIAN_POINT('Ctrl Pts',(65.2686593298991,-7.16704019306199,
66.451322347829));
#145649=CARTESIAN_POINT('Ctrl Pts',(65.3339085497291,-7.255260014411,66.411786713305));
#145650=CARTESIAN_POINT('Ctrl Pts',(65.4124751097891,-7.35606512702098,
66.3792619117831));
#145651=CARTESIAN_POINT('Ctrl Pts',(65.4996859213891,-7.46199868601399,
66.359128467309));
#145652=CARTESIAN_POINT('Ctrl Pts',(65.5607994574491,-7.53227090791299,
66.355726537549));
#145653=CARTESIAN_POINT('Ctrl Pts',(65.5903804255091,-7.56541214625599,
66.356593540049));
#145654=CARTESIAN_POINT('Ctrl Pts',(64.5846873418391,-6.30826130801998,
67.129516993943));
#145655=CARTESIAN_POINT('Ctrl Pts',(64.5644558003891,-6.29438263574299,
67.070569230962));
#145656=CARTESIAN_POINT('Ctrl Pts',(64.5270818293391,-6.27495791837099,
66.936568367789));
#145657=CARTESIAN_POINT('Ctrl Pts',(64.4965238099191,-6.286222366815,66.718086212213));
#145658=CARTESIAN_POINT('Ctrl Pts',(64.4976343803391,-6.34198098713299,
66.5003543309391));
#145659=CARTESIAN_POINT('Ctrl Pts',(64.5265729662991,-6.42999665028198,
66.309045559806));
#145660=CARTESIAN_POINT('Ctrl Pts',(64.5750030295691,-6.53664105447099,
66.1491720266271));
#145661=CARTESIAN_POINT('Ctrl Pts',(64.6365600582891,-6.65313100744599,
66.01733044383));
#145662=CARTESIAN_POINT('Ctrl Pts',(64.7080223585791,-6.77577809653398,
65.907554455012));
#145663=CARTESIAN_POINT('Ctrl Pts',(64.7897203452091,-6.90580213921598,
65.813630090375));
#145664=CARTESIAN_POINT('Ctrl Pts',(64.8846591549891,-7.04714751738299,
65.731602763897));
#145665=CARTESIAN_POINT('Ctrl Pts',(64.9965114148391,-7.20324351350999,
65.661153574081));
#145666=CARTESIAN_POINT('Ctrl Pts',(65.1287226451391,-7.376030976721,65.604985997049));
#145667=CARTESIAN_POINT('Ctrl Pts',(65.2766685793991,-7.55657323556499,
65.57041707536));
#145668=CARTESIAN_POINT('Ctrl Pts',(65.3842659312291,-7.67917213547799,
65.564613257377));
#145669=CARTESIAN_POINT('Ctrl Pts',(65.4380564282991,-7.73843473867099,
65.5665426449911));
#145670=CARTESIAN_POINT('Ctrl Pts',(64.8058317116991,-5.52201624219599,
67.230640282151));
#145671=CARTESIAN_POINT('Ctrl Pts',(64.7749331788191,-5.50098256085199,
67.139286972566));
#145672=CARTESIAN_POINT('Ctrl Pts',(64.7172313694291,-5.47125424467599,
66.930476149142));
#145673=CARTESIAN_POINT('Ctrl Pts',(64.6691975511091,-5.48856163605999,
66.589141421244));
#145674=CARTESIAN_POINT('Ctrl Pts',(64.6694234445891,-5.573288773669,66.252648819473));
#145675=CARTESIAN_POINT('Ctrl Pts',(64.7105157551291,-5.70372966028198,
65.96379370785));
#145676=CARTESIAN_POINT('Ctrl Pts',(64.7778773578891,-5.85658577094199,
65.729818042446));
#145677=CARTESIAN_POINT('Ctrl Pts',(64.8607965267891,-6.01766835912799,
65.543296669127));
#145678=CARTESIAN_POINT('Ctrl Pts',(64.9541226473491,-6.18167532475599,
65.392893794028));
#145679=CARTESIAN_POINT('Ctrl Pts',(65.0580897008191,-6.35062629697198,
65.267762114542));
#145680=CARTESIAN_POINT('Ctrl Pts',(65.1765251610991,-6.53002757612,65.161024986461));
#145681=CARTESIAN_POINT('Ctrl Pts',(65.3142335534391,-6.72469234998399,
65.071054169118));
#145682=CARTESIAN_POINT('Ctrl Pts',(65.4761613813492,-6.93793738304699,
65.000296079579));
#145683=CARTESIAN_POINT('Ctrl Pts',(65.6580540847291,-7.16032441324298,
64.957284899351));
#145684=CARTESIAN_POINT('Ctrl Pts',(65.7921103656691,-7.31251780163099,
64.950635666937));
#145685=CARTESIAN_POINT('Ctrl Pts',(65.8598469333291,-7.38667276704598,
64.953620573712));
#145686=CARTESIAN_POINT('Ctrl Pts',(65.5578261387191,-5.25148611811499,
67.034089097041));
#145687=CARTESIAN_POINT('Ctrl Pts',(65.5321077652491,-5.23415329278699,
66.95747190315));
#145688=CARTESIAN_POINT('Ctrl Pts',(65.4840969924091,-5.20970588176098,
66.782734178228));
#145689=CARTESIAN_POINT('Ctrl Pts',(65.4438057846191,-5.22392714208799,
66.497514891794));
#145690=CARTESIAN_POINT('Ctrl Pts',(65.4432024666191,-5.29370795646599,
66.2154462285421));
#145691=CARTESIAN_POINT('Ctrl Pts',(65.4765356265291,-5.40171007433599,
65.971504655737));
#145692=CARTESIAN_POINT('Ctrl Pts',(65.5321490119791,-5.52919337005599,
65.771899666165));
#145693=CARTESIAN_POINT('Ctrl Pts',(65.6014213006191,-5.66461792108999,
65.61102310247));
#145694=CARTESIAN_POINT('Ctrl Pts',(65.6801624072491,-5.80356455863799,
65.479975844625));
#145695=CARTESIAN_POINT('Ctrl Pts',(65.7686054516391,-5.94766788378599,
65.370033317402));
#145696=CARTESIAN_POINT('Ctrl Pts',(65.8700307916591,-6.10154723232999,
65.275682893811));
#145697=CARTESIAN_POINT('Ctrl Pts',(65.9885549385691,-6.26923558293999,
65.195924179394));
#145698=CARTESIAN_POINT('Ctrl Pts',(66.1283506701291,-6.45340096160299,
65.133336548868));
#145699=CARTESIAN_POINT('Ctrl Pts',(66.2855066543292,-6.64555302768198,
65.095808364164));
#145700=CARTESIAN_POINT('Ctrl Pts',(66.4011371417991,-6.77680282292298,
65.090664511393));
#145701=CARTESIAN_POINT('Ctrl Pts',(66.4594531070191,-6.84062883253698,
65.093706344424));
#145702=CARTESIAN_POINT('',(64.9957413110435,-6.75150108785322,66.8052962244274));
#145703=CARTESIAN_POINT('Origin',(65.7929813465701,-6.16441562760705,66.6647005262893));
#145704=CARTESIAN_POINT('Ctrl Pts',(64.9957412482689,-6.75150113408116,
66.8052962354967));
#145705=CARTESIAN_POINT('Ctrl Pts',(64.9936068689243,-6.75150289354447,
66.7931850942144));
#145706=CARTESIAN_POINT('Ctrl Pts',(64.9919613219775,-6.75218103920743,
66.7810210222568));
#145707=CARTESIAN_POINT('Ctrl Pts',(64.990806008816,-6.75354673203848,66.7687616839126));
#145708=CARTESIAN_POINT('Ctrl Pts',(64.9903420903241,-6.75409512894045,
66.7638389201582));
#145709=CARTESIAN_POINT('Ctrl Pts',(64.9899575702403,-6.75475486043816,
66.7589008141091));
#145710=CARTESIAN_POINT('Ctrl Pts',(64.9896539598328,-6.75552852608416,
66.7539448192927));
#145711=CARTESIAN_POINT('Ctrl Pts',(64.9893478909668,-6.75630845641968,
66.7489486937441));
#145712=CARTESIAN_POINT('Ctrl Pts',(64.9891240499354,-6.75720417922191,
66.7439343836253));
#145713=CARTESIAN_POINT('Ctrl Pts',(64.9889836964078,-6.75821773879896,
66.7388992431453));
#145714=CARTESIAN_POINT('Ctrl Pts',(64.9886052261716,-6.76095085238226,
66.7253217375389));
#145715=CARTESIAN_POINT('Ctrl Pts',(64.9888244029213,-6.76452830191135,
66.7115917024379));
#145716=CARTESIAN_POINT('Ctrl Pts',(64.9896557162724,-6.76892729155128,
66.6978610038703));
#145717=CARTESIAN_POINT('Ctrl Pts',(64.9899520038508,-6.77049513114639,
66.6929672590232));
#145718=CARTESIAN_POINT('Ctrl Pts',(64.9903257678605,-6.77216693305507,
66.6880734760077));
#145719=CARTESIAN_POINT('Ctrl Pts',(64.9907767352693,-6.77394038232406,
66.6831866144325));
#145720=CARTESIAN_POINT('Ctrl Pts',(64.9911543157406,-6.77542523421738,
66.679095002798));
#145721=CARTESIAN_POINT('Ctrl Pts',(64.9915860087853,-6.77698133095018,
66.6750082448231));
#145722=CARTESIAN_POINT('Ctrl Pts',(64.9920709510125,-6.77860638547479,
66.6709299942178));
#145723=CARTESIAN_POINT('Ctrl Pts',(64.9942163426786,-6.78579565099697,
66.6528877525432));
#145724=CARTESIAN_POINT('Ctrl Pts',(64.9974229200744,-6.79435931348434,
66.6350163464812));
#145725=CARTESIAN_POINT('Ctrl Pts',(65.0016435135698,-6.80419766155188,
66.6173706480389));
#145726=CARTESIAN_POINT('Ctrl Pts',(65.0019806050124,-6.80498343325606,
66.6159613168746));
#145727=CARTESIAN_POINT('Ctrl Pts',(65.0023241818192,-6.80577735725546,
66.6145534283434));
#145728=CARTESIAN_POINT('Ctrl Pts',(65.0026742287018,-6.80657939339643,
66.6131470124946));
#145729=CARTESIAN_POINT('Ctrl Pts',(65.0034351778336,-6.80832289901075,
66.6100896765428));
#145730=CARTESIAN_POINT('Ctrl Pts',(65.004226700411,-6.81010473762457,66.6070392992945));
#145731=CARTESIAN_POINT('Ctrl Pts',(65.0050485723587,-6.81192444442103,
66.6039959761068));
#145732=CARTESIAN_POINT('Ctrl Pts',(65.0104135833997,-6.8238031161308,66.5841297882549));
#145733=CARTESIAN_POINT('Ctrl Pts',(65.017069095402,-6.83729073382415,66.564569670163));
#145734=CARTESIAN_POINT('Ctrl Pts',(65.0249308931841,-6.85218801398523,
66.5455059081924));
#145735=CARTESIAN_POINT('Ctrl Pts',(65.0257641556693,-6.85376695878043,
66.5434853630046));
#145736=CARTESIAN_POINT('Ctrl Pts',(65.0266109458093,-6.85536170153071,
66.5414704078398));
#145737=CARTESIAN_POINT('Ctrl Pts',(65.0274711486299,-6.85697199978835,
66.5394612146089));
#145738=CARTESIAN_POINT('Ctrl Pts',(65.034734709266,-6.87056937328712,66.5224955682377));
#145739=CARTESIAN_POINT('Ctrl Pts',(65.0429553072957,-6.88527632463471,
66.5059424169631));
#145740=CARTESIAN_POINT('Ctrl Pts',(65.0520130228369,-6.9008714845568,66.4899416996529));
#145741=CARTESIAN_POINT('Ctrl Pts',(65.0535496605724,-6.90351719705656,
66.4872271845082));
#145742=CARTESIAN_POINT('Ctrl Pts',(65.0551103163824,-6.90618838620459,
66.4845285292667));
#145743=CARTESIAN_POINT('Ctrl Pts',(65.0566943166813,-6.90888387134211,
66.4818463664612));
#145744=CARTESIAN_POINT('Ctrl Pts',(65.0573117932484,-6.90993462803117,
66.4808008030969));
#145745=CARTESIAN_POINT('Ctrl Pts',(65.0579328170036,-6.91098907647978,
66.4797577457591));
#145746=CARTESIAN_POINT('Ctrl Pts',(65.0585573503357,-6.91204715324597,
66.4787172235966));
#145747=CARTESIAN_POINT('Ctrl Pts',(65.0675938222681,-6.92735663395535,
66.4636617432355));
#145748=CARTESIAN_POINT('Ctrl Pts',(65.0773692007275,-6.94343040892352,
66.4491422646466));
#145749=CARTESIAN_POINT('Ctrl Pts',(65.0878742964325,-6.96024444379511,
66.4351010898323));
#145750=CARTESIAN_POINT('Ctrl Pts',(65.0907837768044,-6.96490124139173,
66.431212260671));
#145751=CARTESIAN_POINT('Ctrl Pts',(65.0937494246626,-6.96961500088883,
66.4273602900493));
#145752=CARTESIAN_POINT('Ctrl Pts',(65.0967714585411,-6.97438556823907,
66.4235443627965));
#145753=CARTESIAN_POINT('Ctrl Pts',(65.0969296794135,-6.97463533490569,
66.4233445770352));
#145754=CARTESIAN_POINT('Ctrl Pts',(65.0970880548828,-6.97488525731564,
66.4231448901174));
#145755=CARTESIAN_POINT('Ctrl Pts',(65.0972465850298,-6.97513533553087,
66.4229453018999));
#145756=CARTESIAN_POINT('Ctrl Pts',(65.1056308360837,-6.98836132805345,
66.4123895952783));
#145757=CARTESIAN_POINT('Ctrl Pts',(65.11444874283,-7.00202418757555,66.4021137805335));
#145758=CARTESIAN_POINT('Ctrl Pts',(65.1238002910885,-7.01625762713036,
66.3920320193054));
#145759=CARTESIAN_POINT('Ctrl Pts',(65.1301969814149,-7.02599365186076,
66.3851358452454));
#145760=CARTESIAN_POINT('Ctrl Pts',(65.1368440523132,-7.03599724609615,
66.3783311899346));
#145761=CARTESIAN_POINT('Ctrl Pts',(65.1437809996806,-7.0463159938978,66.3716013649534));
#145762=CARTESIAN_POINT('Ctrl Pts',(65.1443196991528,-7.04711731235965,
66.3710787498933));
#145763=CARTESIAN_POINT('Ctrl Pts',(65.1448601355016,-7.0479205171145,66.3705565810029));
#145764=CARTESIAN_POINT('Ctrl Pts',(65.1454023195242,-7.04872561738837,
66.3700348626769));
#145765=CARTESIAN_POINT('Ctrl Pts',(65.157176549479,-7.06620941507775,66.3587050718933));
#145766=CARTESIAN_POINT('Ctrl Pts',(65.1697742873168,-7.08458819847325,
66.3475839151916));
#145767=CARTESIAN_POINT('Ctrl Pts',(65.1833198536002,-7.10396819551667,
66.3367353431686));
#145768=CARTESIAN_POINT('Ctrl Pts',(65.1889252349162,-7.11198796162014,
66.332246023073));
#145769=CARTESIAN_POINT('Ctrl Pts',(65.1946930184249,-7.12017901613353,
66.3278039355833));
#145770=CARTESIAN_POINT('Ctrl Pts',(65.2006322564015,-7.12854790835301,
66.323416097461));
#145771=CARTESIAN_POINT('Ctrl Pts',(65.2021783884733,-7.13072654014328,
66.322273833542));
#145772=CARTESIAN_POINT('Ctrl Pts',(65.2037360963087,-7.13291718540268,
66.3211351618697));
#145773=CARTESIAN_POINT('Ctrl Pts',(65.2053053865769,-7.13511973984414,
66.3200003169949));
#145774=CARTESIAN_POINT('Ctrl Pts',(65.2199248637306,-7.15563869353206,
66.3094281245488));
#145775=CARTESIAN_POINT('Ctrl Pts',(65.2355518767617,-7.17719463681946,
66.2991875114242));
#145776=CARTESIAN_POINT('Ctrl Pts',(65.2521863781437,-7.19970040895401,
66.2894705284383));
#145777=CARTESIAN_POINT('Ctrl Pts',(65.2579637656283,-7.20751696824105,
66.286095688724));
#145778=CARTESIAN_POINT('Ctrl Pts',(65.2638624291241,-7.21544772945101,
66.2827840693087));
#145779=CARTESIAN_POINT('Ctrl Pts',(65.2698815295365,-7.22348782013174,
66.2795438864646));
#145780=CARTESIAN_POINT('Ctrl Pts',(65.2728140576992,-7.22740498228831,
66.2779652573022));
#145781=CARTESIAN_POINT('Ctrl Pts',(65.2757752682902,-7.23134816203923,
66.2764038098071));
#145782=CARTESIAN_POINT('Ctrl Pts',(65.2787654844822,-7.23531735155886,
66.2748602419139));
#145783=CARTESIAN_POINT('Ctrl Pts',(65.2953143393923,-7.25728417176686,
66.266317621759));
#145784=CARTESIAN_POINT('Ctrl Pts',(65.3127524129375,-7.28004996710753,
66.2583195996746));
#145785=CARTESIAN_POINT('Ctrl Pts',(65.331133299115,-7.30361038858351,66.2510082076709));
#145786=CARTESIAN_POINT('Ctrl Pts',(65.3379826757077,-7.31238984555927,
66.2482837211164));
#145787=CARTESIAN_POINT('Ctrl Pts',(65.3449628620906,-7.32127934330882,
66.2456549583717));
#145788=CARTESIAN_POINT('Ctrl Pts',(65.352076172117,-7.33027746437928,66.2431306889924));
#145789=CARTESIAN_POINT('Ctrl Pts',(65.3567887585433,-7.33623874303322,
66.2414583539515));
#145790=CARTESIAN_POINT('Ctrl Pts',(65.3615598154622,-7.34224766988668,
66.2398322314557));
#145791=CARTESIAN_POINT('Ctrl Pts',(65.3663903157263,-7.34830410595062,
66.2382550148849));
#145792=CARTESIAN_POINT('Ctrl Pts',(65.3837209722507,-7.37003312105212,
66.2325963465985));
#145793=CARTESIAN_POINT('Ctrl Pts',(65.4018176405439,-7.39237575559042,
66.2275642249406));
#145794=CARTESIAN_POINT('Ctrl Pts',(65.4207235793857,-7.41532150571302,
66.2233112864293));
#145795=CARTESIAN_POINT('Ctrl Pts',(65.4297043454721,-7.42622127727429,
66.2212910405019));
#145796=CARTESIAN_POINT('Ctrl Pts',(65.4388675593786,-7.43725674442328,
66.2194471739687));
#145797=CARTESIAN_POINT('Ctrl Pts',(65.4482167623584,-7.44842431244937,
66.2177992883089));
#145798=CARTESIAN_POINT('Origin',(77.1089102519491,1.4210854715202E-14,
81.89107979688));
#145799=CARTESIAN_POINT('',(65.0614528323817,-6.75160559577343,67.1773204194393));
#145800=CARTESIAN_POINT('Ctrl Pts',(65.6628233895018,-7.69741763536957,
66.1799583497825));
#145801=CARTESIAN_POINT('Ctrl Pts',(65.6127075559676,-7.63232133342805,
66.2334606385732));
#145802=CARTESIAN_POINT('Ctrl Pts',(65.5649450822481,-7.56794231263672,
66.2888414104336));
#145803=CARTESIAN_POINT('Ctrl Pts',(65.5194507398504,-7.50436891431119,
66.3461211498897));
#145804=CARTESIAN_POINT('Ctrl Pts',(65.5035580018977,-7.48216054054206,
66.3661309322318));
#145805=CARTESIAN_POINT('Ctrl Pts',(65.4879424060478,-7.46005074136449,
66.3863723088932));
#145806=CARTESIAN_POINT('Ctrl Pts',(65.472601424378,-7.43804417092933,66.4068456354934));
#145807=CARTESIAN_POINT('Ctrl Pts',(65.4692867937749,-7.43328934797185,
66.4112691799808));
#145808=CARTESIAN_POINT('Ctrl Pts',(65.4659849791221,-7.42853931851314,
66.4157036512151));
#145809=CARTESIAN_POINT('Ctrl Pts',(65.4626959189898,-7.4237941090516,66.420148940823));
#145810=CARTESIAN_POINT('Ctrl Pts',(65.4365856047165,-7.38612410444588,
66.4554380216017));
#145811=CARTESIAN_POINT('Ctrl Pts',(65.4112792364022,-7.34875798046335,
66.4914096876316));
#145812=CARTESIAN_POINT('Ctrl Pts',(65.3867600614493,-7.31171561938907,
66.5280685818853));
#145813=CARTESIAN_POINT('Ctrl Pts',(65.3729561601058,-7.29086136557404,
66.5487069500447));
#145814=CARTESIAN_POINT('Ctrl Pts',(65.3592361678855,-7.26985646092619,
66.5698166149439));
#145815=CARTESIAN_POINT('Ctrl Pts',(65.3458495281046,-7.24908536245234,
66.591022713179));
#145816=CARTESIAN_POINT('Ctrl Pts',(65.3324628883238,-7.22831426397849,
66.612228811414));
#145817=CARTESIAN_POINT('Ctrl Pts',(65.3194096074541,-7.20777716874016,
66.6335313515063));
#145818=CARTESIAN_POINT('Ctrl Pts',(65.3069059172977,-7.18784778724475,
66.6545146388941));
#145819=CARTESIAN_POINT('Ctrl Pts',(65.2686650771674,-7.12689647750146,
66.7186891768395));
#145820=CARTESIAN_POINT('Ctrl Pts',(65.2332616977372,-7.06794612605696,
66.7838861851928));
#145821=CARTESIAN_POINT('Ctrl Pts',(65.200445601414,-7.01101868563781,66.8499281049124));
#145822=CARTESIAN_POINT('Ctrl Pts',(65.1773957807998,-6.9710332078783,66.8963155358718));
#145823=CARTESIAN_POINT('Ctrl Pts',(65.1556242548341,-6.93204598359059,
66.9431219028185));
#145824=CARTESIAN_POINT('Ctrl Pts',(65.1351143718149,-6.8941175358365,66.9904058935751));
#145825=CARTESIAN_POINT('Ctrl Pts',(65.1129261116537,-6.85308530442445,
67.0415592564385));
#145826=CARTESIAN_POINT('Ctrl Pts',(65.0922142864307,-6.81329230333574,
67.0932711865362));
#145827=CARTESIAN_POINT('Ctrl Pts',(65.0729367663882,-6.77479600626462,
67.1455623671584));
#145828=CARTESIAN_POINT('Ctrl Pts',(65.0690422793673,-6.76701889961564,
67.1561263465393));
#145829=CARTESIAN_POINT('Ctrl Pts',(65.0652062714112,-6.75929465525485,
67.1667138179077));
#145830=CARTESIAN_POINT('Ctrl Pts',(65.0614283108073,-6.75162365816252,
67.1773247406763));
#145831=CARTESIAN_POINT('',(65.0614295862717,-6.75162271773899,67.1773245146892));
#145832=CARTESIAN_POINT('Origin',(77.1089102519491,1.4210854715202E-14,
81.89107979688));
#145833=CARTESIAN_POINT('',(64.9957413410401,6.7515010657631,66.8052962191372));
#145834=CARTESIAN_POINT('',(65.0614282834239,6.75162228554997,67.1773189309182));
#145835=CARTESIAN_POINT('',(65.6628212128545,7.69739984953404,66.1799651776145));
#145836=CARTESIAN_POINT('Ctrl Pts',(65.0614282834239,6.75162228554997,67.1773189309182));
#145837=CARTESIAN_POINT('Ctrl Pts',(65.0936086814867,6.81696027379672,67.086937637008));
#145838=CARTESIAN_POINT('Ctrl Pts',(65.1299716419799,6.88614028642303,66.9982120934198));
#145839=CARTESIAN_POINT('Ctrl Pts',(65.1707899936982,6.95892998196222,66.9110941930759));
#145840=CARTESIAN_POINT('Ctrl Pts',(65.1911991695574,6.99532482973182,66.8675352429039));
#145841=CARTESIAN_POINT('Ctrl Pts',(65.2127225848764,7.03262146593794,66.8243781344839));
#145842=CARTESIAN_POINT('Ctrl Pts',(65.2353966066073,7.07078698935139,66.7816164553411));
#145843=CARTESIAN_POINT('Ctrl Pts',(65.2515080065354,7.09790613118162,66.7512314392885));
#145844=CARTESIAN_POINT('Ctrl Pts',(65.2678894704613,7.12496058509741,66.721572719888));
#145845=CARTESIAN_POINT('Ctrl Pts',(65.2852160836108,7.15301162432833,66.6915154711413));
#145846=CARTESIAN_POINT('Ctrl Pts',(65.2922736955954,7.16443759367097,66.6792723168012));
#145847=CARTESIAN_POINT('Ctrl Pts',(65.2994885686195,7.17602855145341,66.6669629614903));
#145848=CARTESIAN_POINT('Ctrl Pts',(65.3069082509523,7.18785463689311,66.654511047652));
#145849=CARTESIAN_POINT('Ctrl Pts',(65.3692579692799,7.287232624119,66.5498740449287));
#145850=CARTESIAN_POINT('Ctrl Pts',(65.4373698278873,7.38919787124566,66.4504117121515));
#145851=CARTESIAN_POINT('Ctrl Pts',(65.5115870550174,7.49335931066728,66.3560635289208));
#145852=CARTESIAN_POINT('Ctrl Pts',(65.5594279581965,7.5605024461771,66.2952460816299));
#145853=CARTESIAN_POINT('Ctrl Pts',(65.6098058991986,7.62855713753377,66.2365536262945));
#145854=CARTESIAN_POINT('Ctrl Pts',(65.662813434262,7.69740712101228,66.1799698427528));
#145855=CARTESIAN_POINT('',(65.4482167089465,7.44842435396614,66.2177992977254));
#145856=CARTESIAN_POINT('Origin',(74.0770084968991,1.4210854715202E-14,
64.696310494594));
#145857=CARTESIAN_POINT('Ctrl Pts',(64.9957413309291,6.75150107320901,66.80529622092));
#145858=CARTESIAN_POINT('Ctrl Pts',(64.9939147746393,6.75150118167963,66.7949374485334));
#145859=CARTESIAN_POINT('Ctrl Pts',(64.9894338048507,6.7530267160936,66.7631516371945));
#145860=CARTESIAN_POINT('Ctrl Pts',(64.9875165633987,6.76373848476411,66.7075258057507));
#145861=CARTESIAN_POINT('Ctrl Pts',(64.9953306241186,6.79090605225776,66.63784977939));
#145862=CARTESIAN_POINT('Ctrl Pts',(65.0150684046813,6.83452434266292,66.5653197541562));
#145863=CARTESIAN_POINT('Ctrl Pts',(65.0481757788599,6.89549721919369,66.4921639904142));
#145864=CARTESIAN_POINT('Ctrl Pts',(65.0958776509467,6.97417184586988,66.4206746812155));
#145865=CARTESIAN_POINT('Ctrl Pts',(65.1594070364026,7.07061581212493,66.3532950647828));
#145866=CARTESIAN_POINT('Ctrl Pts',(65.2401133825063,7.1846757117932,66.2929751276064));
#145867=CARTESIAN_POINT('Ctrl Pts',(65.3374029752483,7.31312989194673,66.2447445995378));
#145868=CARTESIAN_POINT('Ctrl Pts',(65.410159366793,7.40296747944908,66.2245011702614));
#145869=CARTESIAN_POINT('Ctrl Pts',(65.4482167191791,7.44842434513301,66.217799295921));
#145870=CARTESIAN_POINT('Origin',(65.9936985527191,-6.16441400296899,67.803130872521));
#145871=CARTESIAN_POINT('Ctrl Pts',(65.0614295956489,-6.75162271329526,
67.1773245130358));
#145872=CARTESIAN_POINT('Ctrl Pts',(65.0357806317137,-6.71568906787898,
67.1819829434292));
#145873=CARTESIAN_POINT('Ctrl Pts',(65.0124824624939,-6.67801772235096,
67.1861703445779));
#145874=CARTESIAN_POINT('Ctrl Pts',(64.9917449493442,-6.6389415340824,67.1898735572973));
#145875=CARTESIAN_POINT('Ctrl Pts',(64.9710061590129,-6.59986293919032,
67.1935769980901));
#145876=CARTESIAN_POINT('Ctrl Pts',(64.9528285550174,-6.55937973262129,
67.1967961529284));
#145877=CARTESIAN_POINT('Ctrl Pts',(64.9373768558342,-6.51784954555001,
67.1995258269408));
#145878=CARTESIAN_POINT('Ctrl Pts',(64.9311493087832,-6.50111150328317,
67.2006259760664));
#145879=CARTESIAN_POINT('Ctrl Pts',(64.9253640162319,-6.48420364016903,
67.2016467094416));
#145880=CARTESIAN_POINT('Ctrl Pts',(64.9200295766639,-6.46715026990716,
67.2025880722727));
#145881=CARTESIAN_POINT('',(64.8738238573791,-6.16438935871099,67.210776354606));
#145882=CARTESIAN_POINT('Origin',(67.8574209319491,111.0724296188,84.13159620183));
#145883=CARTESIAN_POINT('',(65.1554501449391,-13.43008249787,68.807974748468));
#145884=CARTESIAN_POINT('Origin',(64.9111938245191,0.499074165591614,67.422711970997));
#145885=CARTESIAN_POINT('',(65.1554596847291,6.92820316569601,68.807986718554));
#145886=CARTESIAN_POINT('',(64.8738236000791,6.16438877351401,67.210774895336));
#145887=CARTESIAN_POINT('Ctrl Pts',(65.1269899167215,6.68586918419113,68.6465524198017));
#145888=CARTESIAN_POINT('Ctrl Pts',(65.1258607393499,6.6788598129293,68.640148532931));
#145889=CARTESIAN_POINT('Ctrl Pts',(65.124702511399,6.67185299366292,68.6335798904187));
#145890=CARTESIAN_POINT('Ctrl Pts',(65.1235144956525,6.66484982371274,68.6268423120024));
#145891=CARTESIAN_POINT('Ctrl Pts',(65.120473486417,6.64692354238209,68.6095958754548));
#145892=CARTESIAN_POINT('Ctrl Pts',(65.117237346027,6.62901914992627,68.5912427894659));
#145893=CARTESIAN_POINT('Ctrl Pts',(65.1137875519203,6.61115996404497,68.5716780151953));
#145894=CARTESIAN_POINT('Ctrl Pts',(65.1102351559665,6.59276962024424,68.5515313563492));
#145895=CARTESIAN_POINT('Ctrl Pts',(65.106456074087,6.57442649737051,68.530099099943));
#145896=CARTESIAN_POINT('Ctrl Pts',(65.1024308862485,6.55619573439959,68.5072711131346));
#145897=CARTESIAN_POINT('Ctrl Pts',(65.09832758876,6.53761119948784,68.4840001442517));
#145898=CARTESIAN_POINT('Ctrl Pts',(65.09396848797,6.51914372357155,68.4592784487402));
#145899=CARTESIAN_POINT('Ctrl Pts',(65.0893316050564,6.50087699663407,68.4329813787262));
#145900=CARTESIAN_POINT('Ctrl Pts',(65.0846447485376,6.48241340162472,68.4064008943114));
#145901=CARTESIAN_POINT('Ctrl Pts',(65.0796740241207,6.46415513437845,68.3782105212977));
#145902=CARTESIAN_POINT('Ctrl Pts',(65.0743965924953,6.44621207552659,68.3482807294666));
#145903=CARTESIAN_POINT('Ctrl Pts',(65.0690851709034,6.42815345213261,68.318158171022));
#145904=CARTESIAN_POINT('Ctrl Pts',(65.0634629542406,6.41041440358812,68.2862730103171));
#145905=CARTESIAN_POINT('Ctrl Pts',(65.0575092298989,6.39313250902638,68.2525077772224));
#145906=CARTESIAN_POINT('Ctrl Pts',(65.0527301358131,6.37926021744024,68.2254042002801));
#145907=CARTESIAN_POINT('Ctrl Pts',(65.047737608407,6.3656837258347,68.1970901834972));
#145908=CARTESIAN_POINT('Ctrl Pts',(65.0425198259768,6.3524726480596,68.16749868105));
#145909=CARTESIAN_POINT('Ctrl Pts',(65.0411986195115,6.34912744123976,68.1600057499295));
#145910=CARTESIAN_POINT('Ctrl Pts',(65.0398532109862,6.34578094414381,68.1523755620387));
#145911=CARTESIAN_POINT('Ctrl Pts',(65.0384839951051,6.3424383158584,68.1446103558303));
#145912=CARTESIAN_POINT('Ctrl Pts',(65.0330448194473,6.32915980904687,68.1137632694282));
#145913=CARTESIAN_POINT('Ctrl Pts',(65.0272294990806,6.31594506631054,68.0807829588119));
#145914=CARTESIAN_POINT('Ctrl Pts',(65.0210597275564,6.30310947651882,68.0457924531821));
#145915=CARTESIAN_POINT('Ctrl Pts',(65.0197620560254,6.300409801273,68.0384329937868));
#145916=CARTESIAN_POINT('Ctrl Pts',(65.0184487265847,6.29772676799765,68.0309847338614));
#145917=CARTESIAN_POINT('Ctrl Pts',(65.0171199775613,6.29506309001698,68.0234490250218));
#145918=CARTESIAN_POINT('Ctrl Pts',(65.0111943844742,6.28318434425673,67.9898433226514));
#145919=CARTESIAN_POINT('Ctrl Pts',(65.0049615477093,6.27169277400508,67.9544951524432));
#145920=CARTESIAN_POINT('Ctrl Pts',(64.9984504770749,6.26082766944341,67.9175690374176));
#145921=CARTESIAN_POINT('Ctrl Pts',(64.9967188376108,6.25793806112909,67.907748422403));
#145922=CARTESIAN_POINT('Ctrl Pts',(64.9949675588263,6.25509260064891,67.8978164271211));
#145923=CARTESIAN_POINT('Ctrl Pts',(64.9931972748634,6.25229542027833,67.8877766479843));
#145924=CARTESIAN_POINT('Ctrl Pts',(64.9865434827275,6.24178193366082,67.8500411180529));
#145925=CARTESIAN_POINT('Ctrl Pts',(64.9796207498768,6.23195352672873,67.8107803476211));
#145926=CARTESIAN_POINT('Ctrl Pts',(64.9724629900716,6.22299781395229,67.7701866722689));
#145927=CARTESIAN_POINT('Ctrl Pts',(64.9705097863249,6.22055398624287,67.7591095027427));
#145928=CARTESIAN_POINT('Ctrl Pts',(64.9685391158548,6.21817491653994,67.7479332744464));
#145929=CARTESIAN_POINT('Ctrl Pts',(64.9665517437151,6.21586389941347,67.7366623262435));
#145930=CARTESIAN_POINT('Ctrl Pts',(64.9594137719853,6.20756350383758,67.6961808743631));
#145931=CARTESIAN_POINT('Ctrl Pts',(64.9520599251814,6.20014425028192,67.6544751336973));
#145932=CARTESIAN_POINT('Ctrl Pts',(64.9445307639359,6.19372173806413,67.6117751362589));
#145933=CARTESIAN_POINT('Ctrl Pts',(64.9420607517207,6.1916147724788,67.5977670001828));
#145934=CARTESIAN_POINT('Ctrl Pts',(64.9395719148494,6.18961474102989,67.5836521042657));
#145935=CARTESIAN_POINT('Ctrl Pts',(64.9370658072044,6.18772473138426,67.5694392610461));
#145936=CARTESIAN_POINT('Ctrl Pts',(64.9290840161445,6.18170517267833,67.5241722729452));
#145937=CARTESIAN_POINT('Ctrl Pts',(64.9209269430576,6.17680556358816,67.4779112124193));
#145938=CARTESIAN_POINT('Ctrl Pts',(64.9126296391413,6.17308359635863,67.4308548650867));
#145939=CARTESIAN_POINT('Ctrl Pts',(64.9099778113126,6.17189405137193,67.4158156026189));
#145940=CARTESIAN_POINT('Ctrl Pts',(64.9073116720097,6.17082440163475,67.4006951759143));
#145941=CARTESIAN_POINT('Ctrl Pts',(64.9046323987211,6.16987543159412,67.3855002628188));
#145942=CARTESIAN_POINT('Ctrl Pts',(64.89575649588,6.16673168141535,67.3351625190385));
#145943=CARTESIAN_POINT('Ctrl Pts',(64.886736281088,6.16491611625309,67.2840063433688));
#145944=CARTESIAN_POINT('Ctrl Pts',(64.8776208551351,6.16448731723589,67.2323101971345));
#145945=CARTESIAN_POINT('Ctrl Pts',(64.8763568863287,6.16442785884253,67.2251418742725));
#145946=CARTESIAN_POINT('Ctrl Pts',(64.8750910900749,6.16439498447354,67.2179631874115));
#145947=CARTESIAN_POINT('Ctrl Pts',(64.8738236001678,6.16438877351401,67.2107748953204));
#145948=CARTESIAN_POINT('',(64.8738236000791,6.16438877351401,67.210774895336));
#145949=CARTESIAN_POINT('Origin',(65.9862249718391,6.16441400296901,67.760746089178));
#145950=CARTESIAN_POINT('Origin',(65.8588926025934,6.16441457066984,67.038621762377));
#145951=CARTESIAN_POINT('Origin',(65.7929806594911,6.16441569484309,66.6647268826104));
#145952=CARTESIAN_POINT('Ctrl Pts',(65.2148209050525,5.35492257705576,66.7666660125659));
#145953=CARTESIAN_POINT('Ctrl Pts',(65.2067722047426,5.35492482391508,66.7210106884506));
#145954=CARTESIAN_POINT('Ctrl Pts',(65.1864417669287,5.36110944695451,66.5810340695068));
#145955=CARTESIAN_POINT('Ctrl Pts',(65.1750536527964,5.40441097153357,66.3436679578443));
#145956=CARTESIAN_POINT('Ctrl Pts',(65.1976263796561,5.5026709611402,66.0785753213486));
#145957=CARTESIAN_POINT('Ctrl Pts',(65.2514687636523,5.6366770529586,65.8445384223639));
#145958=CARTESIAN_POINT('Ctrl Pts',(65.3294129760629,5.79388364819421,65.6465729402952));
#145959=CARTESIAN_POINT('Ctrl Pts',(65.4269859006806,5.96721711211323,65.481370283013));
#145960=CARTESIAN_POINT('Ctrl Pts',(65.5434369630249,6.15480444083051,65.3440105246222));
#145961=CARTESIAN_POINT('Ctrl Pts',(65.6810291451864,6.35793052064432,65.2315827919279));
#145962=CARTESIAN_POINT('Ctrl Pts',(65.8411083711151,6.57500738265653,65.1465990105339));
#145963=CARTESIAN_POINT('Ctrl Pts',(65.9609957865493,6.72440924846806,65.1119429840824));
#145964=CARTESIAN_POINT('Ctrl Pts',(66.024898044746,6.80073525449069,65.1006867422596));
#145965=CARTESIAN_POINT('Ctrl Pts',(64.7478165014519,5.69883052261465,66.8490114890303));
#145966=CARTESIAN_POINT('Ctrl Pts',(64.7397678016923,5.69883277272402,66.8033561572532));
#145967=CARTESIAN_POINT('Ctrl Pts',(64.719492874681,5.70509510400391,66.6633697271873));
#145968=CARTESIAN_POINT('Ctrl Pts',(64.7084945927605,5.7489422686341,66.425934839464));
#145969=CARTESIAN_POINT('Ctrl Pts',(64.7320602908078,5.84858612855244,66.160667075277));
#145970=CARTESIAN_POINT('Ctrl Pts',(64.7875095659817,5.98481406017563,65.9263468057011));
#145971=CARTESIAN_POINT('Ctrl Pts',(64.8677266075285,6.14512650416259,65.7279805382333));
#145972=CARTESIAN_POINT('Ctrl Pts',(64.9682788441699,6.32246750877359,65.5622525302054));
#145973=CARTESIAN_POINT('Ctrl Pts',(65.0884553317283,6.5149675127728,65.4242358662292));
#145974=CARTESIAN_POINT('Ctrl Pts',(65.2305600206851,6.72390358841762,65.3110124480889));
#145975=CARTESIAN_POINT('Ctrl Pts',(65.3958656909537,6.9475236623724,65.2251070982072));
#145976=CARTESIAN_POINT('Ctrl Pts',(65.5195237655255,7.10150168396956,65.1897862015458));
#145977=CARTESIAN_POINT('Ctrl Pts',(65.5853645199204,7.18014318571723,65.1781881505423));
#145978=CARTESIAN_POINT('Ctrl Pts',(64.6570714587516,6.27731354668077,66.8650128591567));
#145979=CARTESIAN_POINT('Ctrl Pts',(64.6516000319702,6.27731489253399,66.8339775578073));
#145980=CARTESIAN_POINT('Ctrl Pts',(64.6378901917127,6.28164735941406,66.7388053795214));
#145981=CARTESIAN_POINT('Ctrl Pts',(64.6308148861991,6.31199535826295,66.5766500360433));
#145982=CARTESIAN_POINT('Ctrl Pts',(64.6482673217965,6.38219167007379,66.3923267568599));
#145983=CARTESIAN_POINT('Ctrl Pts',(64.689589956481,6.48097961696787,66.2249050521873));
#145984=CARTESIAN_POINT('Ctrl Pts',(64.7512349038882,6.60143060796609,66.078236838856));
#145985=CARTESIAN_POINT('Ctrl Pts',(64.8311297980253,6.73956249720055,65.9513263032596));
#145986=CARTESIAN_POINT('Ctrl Pts',(64.9293853272694,6.8943095462238,65.8422964628036));
#145987=CARTESIAN_POINT('Ctrl Pts',(65.0479270422314,7.06635306504569,65.7506568750857));
#145988=CARTESIAN_POINT('Ctrl Pts',(65.1872242958992,7.2532642842925,65.6799752747044));
#145989=CARTESIAN_POINT('Ctrl Pts',(65.2913599872053,7.38256988089626,65.6506242928727));
#145990=CARTESIAN_POINT('Ctrl Pts',(65.3464951967837,7.44842499426927,65.6409115118738));
#145991=CARTESIAN_POINT('Ctrl Pts',(64.9957431297417,6.75150352764831,66.8052967130971));
#145992=CARTESIAN_POINT('Ctrl Pts',(64.993916514239,6.75150359144112,66.7949372501368));
#145993=CARTESIAN_POINT('Ctrl Pts',(64.9894355913503,6.7530291115906,66.7631517609198));
#145994=CARTESIAN_POINT('Ctrl Pts',(64.9875183761111,6.7637407804721,66.7075264708465));
#145995=CARTESIAN_POINT('Ctrl Pts',(64.99533238785,6.79090812929874,66.6378510271096));
#145996=CARTESIAN_POINT('Ctrl Pts',(65.0150700587209,6.83452613933823,66.5653214841042));
#145997=CARTESIAN_POINT('Ctrl Pts',(65.0481772878749,6.89549871360824,66.4921660939439));
#145998=CARTESIAN_POINT('Ctrl Pts',(65.0958789963607,6.97417303812965,66.4206770663893));
#145999=CARTESIAN_POINT('Ctrl Pts',(65.1594082053423,7.07061670809534,66.3532976616181));
#146000=CARTESIAN_POINT('Ctrl Pts',(65.2401143591712,7.18467631309772,66.2929778836045));
#146001=CARTESIAN_POINT('Ctrl Pts',(65.3374037384352,7.31313019617951,66.2447474696296));
#146002=CARTESIAN_POINT('Ctrl Pts',(65.4101599705141,7.40296758311013,66.2245040866366));
#146003=CARTESIAN_POINT('Ctrl Pts',(65.4482167677065,7.44842452942846,66.2177992873806));
#146004=CARTESIAN_POINT('Origin',(66.19854598009,6.80073540805928,66.0854943910165));
#146005=CARTESIAN_POINT('Origin',(74.0770084968991,1.4210854715202E-14,
64.696310494594));
#146006=CARTESIAN_POINT('Ctrl Pts',(66.2208657833691,7.02807183034301,65.066133808363));
#146007=CARTESIAN_POINT('Ctrl Pts',(65.7922441264735,7.4201337906415,65.1417542799438));
#146008=CARTESIAN_POINT('Ctrl Pts',(65.5610416355161,7.69728092662338,65.6031233574458));
#146009=CARTESIAN_POINT('Ctrl Pts',(65.6628292019748,7.69739218035355,66.1799637693547));
#146010=CARTESIAN_POINT('Ctrl Pts',(66.3469292448691,6.71669427049301,65.089883295194));
#146011=CARTESIAN_POINT('Ctrl Pts',(66.4172621304691,6.79578693974001,65.077481709831));
#146012=CARTESIAN_POINT('Ctrl Pts',(66.7042933355591,7.12081872370401,65.026870364069));
#146013=CARTESIAN_POINT('Ctrl Pts',(67.1737243974691,7.637641242897,64.9440970022721));
#146014=CARTESIAN_POINT('Ctrl Pts',(67.5996249658591,8.01039274550502,64.8689992409641));
#146015=CARTESIAN_POINT('Ctrl Pts',(67.8135694122091,8.17107382160801,64.8312750627));
#146016=CARTESIAN_POINT('Ctrl Pts',(65.6590187149691,7.304104680347,64.933907788844));
#146017=CARTESIAN_POINT('Ctrl Pts',(65.7282021697291,7.38185342331901,64.9217088791509));
#146018=CARTESIAN_POINT('Ctrl Pts',(66.0154107300992,7.70671666045502,64.871066260868));
#146019=CARTESIAN_POINT('Ctrl Pts',(66.5149459070591,8.25911872987902,64.782984731357));
#146020=CARTESIAN_POINT('Ctrl Pts',(67.0067799852291,8.69061703812601,64.696261113344));
#146021=CARTESIAN_POINT('Ctrl Pts',(67.2535719696491,8.87601922441701,64.652745027867));
#146022=CARTESIAN_POINT('Ctrl Pts',(65.2973419556991,7.73916500145001,65.656703935734));
#146023=CARTESIAN_POINT('Ctrl Pts',(65.3656740946791,7.81591837732301,65.6446551359809));
#146024=CARTESIAN_POINT('Ctrl Pts',(65.6530140116592,8.140656781741,65.593989355983));
#146025=CARTESIAN_POINT('Ctrl Pts',(66.1748455349991,8.71941053014201,65.501976379035));
#146026=CARTESIAN_POINT('Ctrl Pts',(66.7155126836291,9.19441914004002,65.406642173149));
#146027=CARTESIAN_POINT('Ctrl Pts',(66.9866329063991,9.39813079779402,65.358836362857));
#146028=CARTESIAN_POINT('Ctrl Pts',(65.6490951182391,7.55611768221601,66.484476132488));
#146029=CARTESIAN_POINT('Ctrl Pts',(65.7177854398991,7.63328984893302,66.472364175465));
#146030=CARTESIAN_POINT('Ctrl Pts',(66.0050700898891,7.95808077548001,66.421708140529));
#146031=CARTESIAN_POINT('Ctrl Pts',(66.5175206464091,8.52574731606101,66.331349281135));
#146032=CARTESIAN_POINT('Ctrl Pts',(67.0376417645191,8.98244939766902,66.239637894777));
#146033=CARTESIAN_POINT('Ctrl Pts',(67.2985261220691,9.17845752672701,66.193636943696));
#146034=CARTESIAN_POINT('',(67.0545200752973,9.08847803716292,65.7314839970685));
#146035=CARTESIAN_POINT('Ctrl Pts',(65.6628302778855,7.69739278665024,66.1799667264387));
#146036=CARTESIAN_POINT('Ctrl Pts',(65.8925920723134,7.96901192097917,66.0738323942691));
#146037=CARTESIAN_POINT('Ctrl Pts',(66.1235380564785,8.22889166321445,65.9816475253631));
#146038=CARTESIAN_POINT('Ctrl Pts',(66.5910239409522,8.69801793251633,65.8306234162482));
#146039=CARTESIAN_POINT('Ctrl Pts',(66.8277216597037,8.90785102579189,65.7715384074934));
#146040=CARTESIAN_POINT('Ctrl Pts',(67.0545035221437,9.08849832361973,65.7314815782556));
#146041=CARTESIAN_POINT('Ctrl Pts',(67.5092801258532,8.31611453423606,64.8389516201314));
#146042=CARTESIAN_POINT('Ctrl Pts',(67.4857251216335,8.34676180112001,64.8431135225438));
#146043=CARTESIAN_POINT('Ctrl Pts',(67.4625360504388,8.37744483878468,64.8495177543901));
#146044=CARTESIAN_POINT('Ctrl Pts',(67.4398979647076,8.40792091496171,64.8581222512767));
#146045=CARTESIAN_POINT('Ctrl Pts',(67.4164854557802,8.43943954308423,64.8670210982271));
#146046=CARTESIAN_POINT('Ctrl Pts',(67.3936625517779,8.47073630068296,64.8782726210766));
#146047=CARTESIAN_POINT('Ctrl Pts',(67.3716088947925,8.50156426811195,64.8917847097676));
#146048=CARTESIAN_POINT('Ctrl Pts',(67.3479088056494,8.53469372036818,64.9063055534854));
#146049=CARTESIAN_POINT('Ctrl Pts',(67.3250973264477,8.56728134404552,64.9234363998483));
#146050=CARTESIAN_POINT('Ctrl Pts',(67.303364532704,8.59905323088256,64.9430221214877));
#146051=CARTESIAN_POINT('Ctrl Pts',(67.2803811050845,8.63265346056626,64.9637349217372));
#146052=CARTESIAN_POINT('Ctrl Pts',(67.2586038660606,8.66534146643593,64.9871924753379));
#146053=CARTESIAN_POINT('Ctrl Pts',(67.2382220938984,8.69683126854594,65.0131798314819));
#146054=CARTESIAN_POINT('Ctrl Pts',(67.2157747527014,8.73151237117853,65.041800848611));
#146055=CARTESIAN_POINT('Ctrl Pts',(67.1950196746371,8.76474056465054,65.0734903266037));
#146056=CARTESIAN_POINT('Ctrl Pts',(67.1761723506734,8.79617468174395,65.1079321649017));
#146057=CARTESIAN_POINT('Ctrl Pts',(67.1724545513139,8.80237533604492,65.114726118495));
#146058=CARTESIAN_POINT('Ctrl Pts',(67.1688108901592,8.80850628147018,65.1216270832089));
#146059=CARTESIAN_POINT('Ctrl Pts',(67.1652428932428,8.81456503217954,65.1286325013422));
#146060=CARTESIAN_POINT('Ctrl Pts',(67.1485433751963,8.84292218023257,65.1614203958617));
#146061=CARTESIAN_POINT('Ctrl Pts',(67.1335316836684,8.86964762216346,65.1964438190701));
#146062=CARTESIAN_POINT('Ctrl Pts',(67.1203440833421,8.89449767307029,65.2333741365688));
#146063=CARTESIAN_POINT('Ctrl Pts',(67.107445608841,8.91880290981096,65.2694947913344));
#146064=CARTESIAN_POINT('Ctrl Pts',(67.0962919734964,8.94131432017231,65.3074398519547));
#146065=CARTESIAN_POINT('Ctrl Pts',(67.0869839112616,8.96183111467034,65.3468720680325));
#146066=CARTESIAN_POINT('Ctrl Pts',(67.0780132010575,8.98160431913696,65.3848751425944));
#146067=CARTESIAN_POINT('Ctrl Pts',(67.0707567941787,8.9995248045942,65.4242597030815));
#146068=CARTESIAN_POINT('Ctrl Pts',(67.0652801409245,9.01543717558087,65.4646929574987));
#146069=CARTESIAN_POINT('Ctrl Pts',(67.0599874736179,9.03081497690973,65.5037678731116));
#146070=CARTESIAN_POINT('Ctrl Pts',(67.056357246951,9.04431699425133,65.5438221960967));
#146071=CARTESIAN_POINT('Ctrl Pts',(67.0544223752917,9.05582913806265,65.5845248385036));
#146072=CARTESIAN_POINT('Ctrl Pts',(67.0525682421163,9.06686090218874,65.6235290376954));
#146073=CARTESIAN_POINT('Ctrl Pts',(67.0522711608951,9.07606503075263,65.6631282571404));
#146074=CARTESIAN_POINT('Ctrl Pts',(67.0535320899779,9.08337060870084,65.703004933018));
#146075=CARTESIAN_POINT('Ctrl Pts',(67.0538320909252,9.08510875586153,65.7124924138779));
#146076=CARTESIAN_POINT('Ctrl Pts',(67.0542201467146,9.08673958372169,65.7219954934958));
#146077=CARTESIAN_POINT('Ctrl Pts',(67.0546960008595,9.08826243435977,65.7315097040137));
#146078=CARTESIAN_POINT('Origin',(74.0770084968991,1.4210854715202E-14,
64.696310494594));
#146079=CARTESIAN_POINT('Origin',(74.0422787428291,1.4210854715202E-14,
64.499348271719));
#146080=CARTESIAN_POINT('Origin',(81.2702407042791,7.61327378225101,63.427949577933));
#146081=CARTESIAN_POINT('Origin',(82.9402782740091,9.38083151964701,63.133476895592));
#146082=CARTESIAN_POINT('Ctrl Pts',(83.2590337349668,6.9829169115756,62.061845095692));
#146083=CARTESIAN_POINT('Ctrl Pts',(83.2524681440442,7.01494834582241,62.0630028256722));
#146084=CARTESIAN_POINT('Ctrl Pts',(83.2460602430039,7.04755385579359,62.0657666515928));
#146085=CARTESIAN_POINT('Ctrl Pts',(83.2398870046894,7.08049337601265,62.0702775505784));
#146086=CARTESIAN_POINT('Ctrl Pts',(83.2337573121717,7.11320054206366,62.0747566298479));
#146087=CARTESIAN_POINT('Ctrl Pts',(83.2278591570096,7.14623651559213,62.080958589238));
#146088=CARTESIAN_POINT('Ctrl Pts',(83.2222654955408,7.17934027904419,62.0889773710341));
#146089=CARTESIAN_POINT('Ctrl Pts',(83.2167138008256,7.21219567968504,62.0969359914775));
#146090=CARTESIAN_POINT('Ctrl Pts',(83.2114622148937,7.24511726789558,62.1066845109911));
#146091=CARTESIAN_POINT('Ctrl Pts',(83.2065771533963,7.27783234147448,62.118266712207));
#146092=CARTESIAN_POINT('Ctrl Pts',(83.2053707477099,7.28591159509624,62.1211270310412));
#146093=CARTESIAN_POINT('Ctrl Pts',(83.2041866654247,7.29397819403508,62.1240989435197));
#146094=CARTESIAN_POINT('Ctrl Pts',(83.2030258423652,7.30202793164075,62.1271826320233));
#146095=CARTESIAN_POINT('Ctrl Pts',(83.19860460872,7.33268701481915,62.1389274946462));
#146096=CARTESIAN_POINT('Ctrl Pts',(83.1945222541898,7.36309703825039,62.1522961884262));
#146097=CARTESIAN_POINT('Ctrl Pts',(83.1908277125425,7.39300060942899,62.1672570785533));
#146098=CARTESIAN_POINT('Ctrl Pts',(83.1871429333242,7.42282516363598,62.1821784361368));
#146099=CARTESIAN_POINT('Ctrl Pts',(83.1838440400959,7.45214526961887,62.1986834628478));
#146100=CARTESIAN_POINT('Ctrl Pts',(83.1809688698346,7.48071466530648,62.2166909562356));
#146101=CARTESIAN_POINT('Ctrl Pts',(83.1780985493129,7.50923587110803,62.2346680751952));
#146102=CARTESIAN_POINT('Ctrl Pts',(83.1756506115634,7.53700825892937,62.2541423288748));
#146103=CARTESIAN_POINT('Ctrl Pts',(83.1736504501174,7.56380570618642,62.2749861383518));
#146104=CARTESIAN_POINT('Ctrl Pts',(83.1726807704526,7.57679712731737,62.2850912317322));
#146105=CARTESIAN_POINT('Ctrl Pts',(83.1718161401716,7.5895597503054,62.2955175369264));
#146106=CARTESIAN_POINT('Ctrl Pts',(83.1710583345944,7.60207007330836,62.3062468954608));
#146107=CARTESIAN_POINT('Ctrl Pts',(83.1694945364883,7.6278862193032,62.3283878654653));
#146108=CARTESIAN_POINT('Ctrl Pts',(83.1683868692723,7.65261988916478,62.3518166476268));
#146109=CARTESIAN_POINT('Ctrl Pts',(83.1677401427287,7.67609101314316,62.3763440729722));
#146110=CARTESIAN_POINT('Ctrl Pts',(83.1670929160326,7.69958028874797,62.4008904668451));
#146111=CARTESIAN_POINT('Ctrl Pts',(83.1669073340634,7.72180464093114,62.4265366428937));
#146112=CARTESIAN_POINT('Ctrl Pts',(83.1671743331004,7.74262337818449,62.4530620968364));
#146113=CARTESIAN_POINT('Ctrl Pts',(83.1674422460852,7.76351337877165,62.4796783484224));
#146114=CARTESIAN_POINT('Ctrl Pts',(83.168165798699,7.78298781481648,62.5071792800384));
#146115=CARTESIAN_POINT('Ctrl Pts',(83.1693222591529,7.80095017263617,62.5353199757027));
#146116=CARTESIAN_POINT('Ctrl Pts',(83.1698800666457,7.80961414185904,62.5488933675476));
#146117=CARTESIAN_POINT('Ctrl Pts',(83.1705383935998,7.81792703037044,62.5626153323347));
#146118=CARTESIAN_POINT('Ctrl Pts',(83.1712936299296,7.82588204732521,62.5764572343032));
#146119=CARTESIAN_POINT('Ctrl Pts',(83.1729608242511,7.84344285388512,62.6070134184412));
#146120=CARTESIAN_POINT('Ctrl Pts',(83.1751006289793,7.85925388829909,62.6381492155685));
#146121=CARTESIAN_POINT('Ctrl Pts',(83.17766709906,7.87330063587728,62.6695823984758));
#146122=CARTESIAN_POINT('Ctrl Pts',(83.1802465167818,7.88741824819954,62.701174159335));
#146123=CARTESIAN_POINT('Ctrl Pts',(83.1832567722595,7.89975384871325,62.7330656671778));
#146124=CARTESIAN_POINT('Ctrl Pts',(83.1866415987951,7.91034406890545,62.764977860896));
#146125=CARTESIAN_POINT('Ctrl Pts',(83.1900590807601,7.92103645923368,62.7971979304766));
#146126=CARTESIAN_POINT('Ctrl Pts',(83.193858237161,7.92994985743764,62.8294384796007));
#146127=CARTESIAN_POINT('Ctrl Pts',(83.1979736594296,7.93717160592385,62.8614294256434));
#146128=CARTESIAN_POINT('Ctrl Pts',(83.1989615480552,7.93890515420172,62.8691087085104));
#146129=CARTESIAN_POINT('Ctrl Pts',(83.1999676331307,7.94054143931416,62.8767737085479));
#146130=CARTESIAN_POINT('Ctrl Pts',(83.2009909626463,7.94208206232058,62.884420892197));
#146131=CARTESIAN_POINT('Ctrl Pts',(83.242348512759,6.67578265849103,62.10784857529));
#146132=CARTESIAN_POINT('Ctrl Pts',(83.334216228839,6.69096397737702,62.09800920288));
#146133=CARTESIAN_POINT('Ctrl Pts',(83.5256285431791,6.73684934210602,62.05584375918));
#146134=CARTESIAN_POINT('Ctrl Pts',(83.7924340751291,6.85036777994202,61.93083026476));
#146135=CARTESIAN_POINT('Ctrl Pts',(84.0221202772992,7.00517611130302,61.75968809345));
#146136=CARTESIAN_POINT('Ctrl Pts',(84.200186923649,7.18247783205801,61.57459024573));
#146137=CARTESIAN_POINT('Ctrl Pts',(84.2989069319091,7.32373971183602,61.43963697091));
#146138=CARTESIAN_POINT('Ctrl Pts',(84.3428871274891,7.40063711210602,61.37092003534));
#146139=CARTESIAN_POINT('Ctrl Pts',(84.3463939118291,7.40686952189903,61.36538012251));
#146140=CARTESIAN_POINT('Ctrl Pts',(83.0958792419792,7.42621601280802,61.89557920747));
#146141=CARTESIAN_POINT('Ctrl Pts',(83.1362882878291,7.43291182363202,61.89126897542));
#146142=CARTESIAN_POINT('Ctrl Pts',(83.2238974325991,7.45354780331802,61.87244519502));
#146143=CARTESIAN_POINT('Ctrl Pts',(83.3610746157191,7.51102643264402,61.8092817005701));
#146144=CARTESIAN_POINT('Ctrl Pts',(83.4921444347992,7.59854355671501,61.7124454520401));
#146145=CARTESIAN_POINT('Ctrl Pts',(83.6020881389591,7.70731505400102,61.59874227206));
#146146=CARTESIAN_POINT('Ctrl Pts',(83.6669013461292,7.79960598128501,61.51044916098));
#146147=CARTESIAN_POINT('Ctrl Pts',(83.6965467594992,7.85143798067902,61.46412926414));
#146148=CARTESIAN_POINT('Ctrl Pts',(83.6989158545292,7.85564850803701,61.46038646796));
#146149=CARTESIAN_POINT('Ctrl Pts',(83.0522723709792,8.02658218017502,62.41261250749));
#146150=CARTESIAN_POINT('Ctrl Pts',(83.1010403436091,8.03463924435402,62.40738738284));
#146151=CARTESIAN_POINT('Ctrl Pts',(83.2022866993591,8.05894910171303,62.38503344276));
#146152=CARTESIAN_POINT('Ctrl Pts',(83.3418023981191,8.11840394021002,62.31954363205));
#146153=CARTESIAN_POINT('Ctrl Pts',(83.4605211614992,8.198508337366,62.23099651645));
#146154=CARTESIAN_POINT('Ctrl Pts',(83.5516689143291,8.28933933996001,62.13618749888));
#146155=CARTESIAN_POINT('Ctrl Pts',(83.6017886106891,8.36110570925201,62.06763936861));
#146156=CARTESIAN_POINT('Ctrl Pts',(83.6240347796191,8.40000231746901,62.0328808413001));
#146157=CARTESIAN_POINT('Ctrl Pts',(83.6258080231391,8.40315379574102,62.03007954256));
#146158=CARTESIAN_POINT('Ctrl Pts',(83.1506552483792,7.93818769792802,63.195027498728));
#146159=CARTESIAN_POINT('Ctrl Pts',(83.2600994900291,7.95623135848103,63.183264358631));
#146160=CARTESIAN_POINT('Ctrl Pts',(83.480187110879,8.00984187819102,63.133675959378));
#146161=CARTESIAN_POINT('Ctrl Pts',(83.7519098984791,8.12751574075102,63.003770861248));
#146162=CARTESIAN_POINT('Ctrl Pts',(83.955625225199,8.266737144798,62.85005845822));
#146163=CARTESIAN_POINT('Ctrl Pts',(84.0941691519691,8.406314936159,62.704689841));
#146164=CARTESIAN_POINT('Ctrl Pts',(84.161992745499,8.50441931165102,62.61125483392));
#146165=CARTESIAN_POINT('Ctrl Pts',(84.1904143637091,8.55411713956403,62.56684828082));
#146166=CARTESIAN_POINT('Ctrl Pts',(84.1926682360992,8.55812266020902,62.56328807835));
#146167=CARTESIAN_POINT('',(83.867026488919,7.66994743046555,61.7007979888644));
#146168=CARTESIAN_POINT('Ctrl Pts',(83.2590342120925,6.98291585998354,62.0618450115583));
#146169=CARTESIAN_POINT('Ctrl Pts',(83.2985801165605,6.99966990543866,62.0548719917187));
#146170=CARTESIAN_POINT('Ctrl Pts',(83.3371733496626,7.01917008559866,62.0456086668951));
#146171=CARTESIAN_POINT('Ctrl Pts',(83.3745860713862,7.04141640046354,62.0343059151991));
#146172=CARTESIAN_POINT('Ctrl Pts',(83.4125223967804,7.06397406001513,62.0228449776774));
#146173=CARTESIAN_POINT('Ctrl Pts',(83.4492449461013,7.08935525832009,62.0092876911224));
#146174=CARTESIAN_POINT('Ctrl Pts',(83.4845685636801,7.11755999537844,61.9939086752094));
#146175=CARTESIAN_POINT('Ctrl Pts',(83.5206198762617,7.14634577276098,61.978212839169));
#146176=CARTESIAN_POINT('Ctrl Pts',(83.5552140688648,7.17807262153736,61.9606199922247));
#146177=CARTESIAN_POINT('Ctrl Pts',(83.5882081719665,7.21274054170755,61.9414270608567));
#146178=CARTESIAN_POINT('Ctrl Pts',(83.5958566796105,7.22077706422198,61.9369778633191));
#146179=CARTESIAN_POINT('Ctrl Pts',(83.603419423539,7.2289716337605,61.9324426815318));
#146180=CARTESIAN_POINT('Ctrl Pts',(83.6108950178491,7.2373242503231,61.9278252043225));
#146181=CARTESIAN_POINT('Ctrl Pts',(83.644056689583,7.27437638518764,61.9073421153394));
#146182=CARTESIAN_POINT('Ctrl Pts',(83.6754993164493,7.31453857244295,61.8852402508517));
#146183=CARTESIAN_POINT('Ctrl Pts',(83.7051350131012,7.35781081208902,61.8618372159296));
#146184=CARTESIAN_POINT('Ctrl Pts',(83.7361099877997,7.40303858398611,61.8373765655493));
#146185=CARTESIAN_POINT('Ctrl Pts',(83.7651110757759,7.45166385493483,61.8114950975671));
#146186=CARTESIAN_POINT('Ctrl Pts',(83.7920957448294,7.50368662493516,61.784540690884));
#146187=CARTESIAN_POINT('Ctrl Pts',(83.8190804138829,7.55570939493549,61.7575862842009));
#146188=CARTESIAN_POINT('Ctrl Pts',(83.8440491912441,7.61112966398742,61.7295593489844));
#146189=CARTESIAN_POINT('Ctrl Pts',(83.867011027257,7.66994743209099,61.7007856446916));
#146190=CARTESIAN_POINT('Ctrl Pts',(83.8670140452191,7.66994743515001,61.70078805062));
#146191=CARTESIAN_POINT('Ctrl Pts',(83.7214305777816,7.96200600407947,61.8832377455994));
#146192=CARTESIAN_POINT('Ctrl Pts',(83.7447899946214,8.21344901265172,62.1589320257208));
#146193=CARTESIAN_POINT('Ctrl Pts',(83.9303991623891,8.35407161789501,62.45142897117));
#146194=CARTESIAN_POINT('Ctrl Pts',(83.923859788829,7.37500816633501,61.67980641543));
#146195=CARTESIAN_POINT('Ctrl Pts',(83.9474802174891,7.38948776532201,61.65713017491));
#146196=CARTESIAN_POINT('Ctrl Pts',(84.0969682792491,7.48649501079001,61.50740188505));
#146197=CARTESIAN_POINT('Ctrl Pts',(84.3516500303791,7.72224899427102,61.17584896249));
#146198=CARTESIAN_POINT('Ctrl Pts',(84.6144842408191,8.16135276122401,60.63977389717));
#146199=CARTESIAN_POINT('Ctrl Pts',(84.7190477994991,8.56508431282901,60.20675032062));
#146200=CARTESIAN_POINT('Ctrl Pts',(84.7401260464792,8.81729927669401,59.95524756863));
#146201=CARTESIAN_POINT('Ctrl Pts',(84.7426394798291,8.86307976508602,59.91006480899));
#146202=CARTESIAN_POINT('Ctrl Pts',(83.5705122279591,7.87114698302502,61.85476420882));
#146203=CARTESIAN_POINT('Ctrl Pts',(83.5866454972991,7.88005369856502,61.83276215457));
#146204=CARTESIAN_POINT('Ctrl Pts',(83.6891686261191,7.94042075304802,61.6872892090601));
#146205=CARTESIAN_POINT('Ctrl Pts',(83.8676830517891,8.09595590885602,61.36311992254));
#146206=CARTESIAN_POINT('Ctrl Pts',(84.0543623951891,8.40203920228501,60.83553875239));
#146207=CARTESIAN_POINT('Ctrl Pts',(84.1282774583391,8.69307089532703,60.40662520731));
#146208=CARTESIAN_POINT('Ctrl Pts',(84.1420710017191,8.87760775573002,60.15662647416));
#146209=CARTESIAN_POINT('Ctrl Pts',(84.1436085530091,8.91117885085303,60.11169514057));
#146210=CARTESIAN_POINT('Ctrl Pts',(83.6270194382592,8.28666180430202,62.32998012357));
#146211=CARTESIAN_POINT('Ctrl Pts',(83.6393529195991,8.29846705592401,62.30586584266));
#146212=CARTESIAN_POINT('Ctrl Pts',(83.7156644082391,8.37619228209003,62.1476760354101));
#146213=CARTESIAN_POINT('Ctrl Pts',(83.8268510679491,8.54776921997102,61.8093361559901));
#146214=CARTESIAN_POINT('Ctrl Pts',(83.9072499723091,8.83518363827502,61.27924397807));
#146215=CARTESIAN_POINT('Ctrl Pts',(83.9054400779791,9.08060190236402,60.85810918613));
#146216=CARTESIAN_POINT('Ctrl Pts',(83.8814528874491,9.22856801730202,60.61571769384));
#146217=CARTESIAN_POINT('Ctrl Pts',(83.8764274466691,9.25527854442902,60.57228534855));
#146218=CARTESIAN_POINT('Ctrl Pts',(84.0561521783491,8.34779461768502,62.79236264607));
#146219=CARTESIAN_POINT('Ctrl Pts',(84.0708766974291,8.36906015182102,62.76474134613));
#146220=CARTESIAN_POINT('Ctrl Pts',(84.1589991300091,8.50670564499601,62.58524085521));
#146221=CARTESIAN_POINT('Ctrl Pts',(84.2560558454591,8.78001599820902,62.22051231515));
#146222=CARTESIAN_POINT('Ctrl Pts',(84.270070601449,9.175412951701,61.67855858024));
#146223=CARTESIAN_POINT('Ctrl Pts',(84.1973499601592,9.472356192965,61.26374630513));
#146224=CARTESIAN_POINT('Ctrl Pts',(84.1299774848391,9.63895321041302,61.030053317));
#146225=CARTESIAN_POINT('Ctrl Pts',(84.1171259072791,9.668672015192,60.98837992798));
#146226=CARTESIAN_POINT('',(84.0701935481991,9.38083151964701,60.90338912307));
#146227=CARTESIAN_POINT('Ctrl Pts',(83.867026488919,7.66994743046555,61.7007979888644));
#146228=CARTESIAN_POINT('Ctrl Pts',(83.884582223782,7.71471713563798,61.678837513214));
#146229=CARTESIAN_POINT('Ctrl Pts',(83.9016620036984,7.76247170792999,61.6555494980752));
#146230=CARTESIAN_POINT('Ctrl Pts',(83.9180456775371,7.81324485204552,61.6309189637823));
#146231=CARTESIAN_POINT('Ctrl Pts',(83.9330478039022,7.85973656882848,61.6083653905399));
#146232=CARTESIAN_POINT('Ctrl Pts',(83.9474668456226,7.90875951572417,61.584686124707));
#146233=CARTESIAN_POINT('Ctrl Pts',(83.9611283868236,7.96029842515161,61.5598856861656));
#146234=CARTESIAN_POINT('Ctrl Pts',(83.9654983093753,7.97678419636026,61.5519527601451));
#146235=CARTESIAN_POINT('Ctrl Pts',(83.9697906548141,7.99352703929664,61.5439052536026));
#146236=CARTESIAN_POINT('Ctrl Pts',(83.9739995139489,8.01052537813633,61.5357437222096));
#146237=CARTESIAN_POINT('Ctrl Pts',(83.9840684003346,8.05119063611737,61.5162188272922));
#146238=CARTESIAN_POINT('Ctrl Pts',(83.9936614914402,8.09332906917797,61.4960360616513));
#146239=CARTESIAN_POINT('Ctrl Pts',(84.0026899628803,8.13694385455923,61.4752245468069));
#146240=CARTESIAN_POINT('Ctrl Pts',(84.0078901294678,8.16206484554452,61.463237651257));
#146241=CARTESIAN_POINT('Ctrl Pts',(84.0129031535625,8.18767518208293,61.4510425428714));
#146242=CARTESIAN_POINT('Ctrl Pts',(84.0177140596479,8.21377418741589,61.4386368596428));
#146243=CARTESIAN_POINT('Ctrl Pts',(84.0242958335317,8.24948009159392,61.4216647133494));
#146244=CARTESIAN_POINT('Ctrl Pts',(84.0304965944768,8.28610154671648,61.404304876692));
#146245=CARTESIAN_POINT('Ctrl Pts',(84.0362709480598,8.32363855283814,61.3865709028769));
#146246=CARTESIAN_POINT('Ctrl Pts',(84.0391581248513,8.34240705589897,61.3777039159694));
#146247=CARTESIAN_POINT('Ctrl Pts',(84.0419387065085,8.36140444671648,61.3687434010195));
#146248=CARTESIAN_POINT('Ctrl Pts',(84.0446069334968,8.38063072531699,61.3596915411556));
#146249=CARTESIAN_POINT('Ctrl Pts',(84.045941046991,8.39024386461724,61.3551656112237));
#146250=CARTESIAN_POINT('Ctrl Pts',(84.0472470726545,8.3999142258631,61.3506168455892));
#146251=CARTESIAN_POINT('Ctrl Pts',(84.048524291865,8.40964180905692,61.3460455336731));
#146252=CARTESIAN_POINT('Ctrl Pts',(84.0491629014703,8.41450560065383,61.3437598777151));
#146253=CARTESIAN_POINT('Ctrl Pts',(84.0497943095174,8.41938369773772,61.3414685852175));
#146254=CARTESIAN_POINT('Ctrl Pts',(84.0504184260876,8.42427610030878,61.339171694199));
#146255=CARTESIAN_POINT('Ctrl Pts',(84.0510425426579,8.42916850287983,61.3368748031805));
#146256=CARTESIAN_POINT('Ctrl Pts',(84.0518355651505,8.43549793372503,61.3339050293409));
#146257=CARTESIAN_POINT('Ctrl Pts',(84.0522688115884,8.43899622448362,61.3322642642359));
#146258=CARTESIAN_POINT('Ctrl Pts',(84.0573240123512,8.47981493772962,61.3131195089983));
#146259=CARTESIAN_POINT('Ctrl Pts',(84.0621702402961,8.52350054174341,61.2924539443833));
#146260=CARTESIAN_POINT('Ctrl Pts',(84.0665105235108,8.57016855648445,61.2704338298668));
#146261=CARTESIAN_POINT('Ctrl Pts',(84.0704464936509,8.61248927691592,61.2504649686352));
#146262=CARTESIAN_POINT('Ctrl Pts',(84.0739658923583,8.65726283209245,61.2293828862379));
#146263=CARTESIAN_POINT('Ctrl Pts',(84.0768640731261,8.7045331478027,61.2073213444561));
#146264=CARTESIAN_POINT('Ctrl Pts',(84.0771617817812,8.7093888773934,61.2050551255905));
#146265=CARTESIAN_POINT('Ctrl Pts',(84.077452954973,8.71427091126197,61.2027785750419));
#146266=CARTESIAN_POINT('Ctrl Pts',(84.0777373852218,8.71917926764842,61.2004918392959));
#146267=CARTESIAN_POINT('Ctrl Pts',(84.0804044531795,8.76520433036884,61.1790493954613));
#146268=CARTESIAN_POINT('Ctrl Pts',(84.0824780972373,8.81354674953817,61.1567137657027));
#146269=CARTESIAN_POINT('Ctrl Pts',(84.0837834793078,8.8642306082537,61.1335396096708));
#146270=CARTESIAN_POINT('Ctrl Pts',(84.0850466303684,8.91327477036905,61.1111151713166));
#146271=CARTESIAN_POINT('Ctrl Pts',(84.0855909918429,8.96451147248083,61.087905989582));
#146272=CARTESIAN_POINT('Ctrl Pts',(84.0852600172611,9.01792742128314,61.0639311405896));
#146273=CARTESIAN_POINT('Ctrl Pts',(84.0849366685859,9.07011262592673,61.0405086903847));
#146274=CARTESIAN_POINT('Ctrl Pts',(84.0837786226198,9.12437776788739,61.0163556535295));
#146275=CARTESIAN_POINT('Ctrl Pts',(84.0816318863806,9.18067552376136,60.9914557007812));
#146276=CARTESIAN_POINT('Ctrl Pts',(84.0795194919131,9.23607267310616,60.9669540775874));
#146277=CARTESIAN_POINT('Ctrl Pts',(84.0764506397482,9.29343763867521,60.9417291457114));
#146278=CARTESIAN_POINT('Ctrl Pts',(84.072258679203,9.35269346002768,60.9157310279044));
#146279=CARTESIAN_POINT('Ctrl Pts',(84.0715984568464,9.36202609033123,60.911636395233));
#146280=CARTESIAN_POINT('Ctrl Pts',(84.0709103193938,9.37140556504035,60.9075225163887));
#146281=CARTESIAN_POINT('Ctrl Pts',(84.070193548197,9.38083151964701,60.9033891230704));
#146282=CARTESIAN_POINT('Ctrl Pts',(83.9304072607132,8.35406389118647,62.4514275465134));
#146283=CARTESIAN_POINT('Ctrl Pts',(83.9919651482484,8.44374030577409,62.3149821809302));
#146284=CARTESIAN_POINT('Ctrl Pts',(84.0355872880004,8.53794851523683,62.1709248993271));
#146285=CARTESIAN_POINT('Ctrl Pts',(84.0658026794286,8.63442789447643,62.0238615241773));
#146286=CARTESIAN_POINT('Ctrl Pts',(84.0883721371628,8.7064933938474,61.9140121900202));
#146287=CARTESIAN_POINT('Ctrl Pts',(84.1034614695384,8.77982608633684,61.802485617024));
#146288=CARTESIAN_POINT('Ctrl Pts',(84.111900980885,8.85387175171245,61.6903694643091));
#146289=CARTESIAN_POINT('Ctrl Pts',(84.1168352776888,8.89716374753911,61.6248189423331));
#146290=CARTESIAN_POINT('Ctrl Pts',(84.119496399077,8.94069937035746,61.5590669038891));
#146291=CARTESIAN_POINT('Ctrl Pts',(84.1200502816288,8.98436778258147,61.4933307421339));
#146292=CARTESIAN_POINT('Ctrl Pts',(84.121712032341,9.11538114432835,61.2961100258022));
#146293=CARTESIAN_POINT('Ctrl Pts',(84.1044062545909,9.24758975113299,61.0990322197026));
#146294=CARTESIAN_POINT('Ctrl Pts',(84.070193548197,9.38083151964701,60.9033891230704));
#146295=CARTESIAN_POINT('Origin',(82.9247768442291,9.38083151964701,63.045563918654));
#146296=CARTESIAN_POINT('',(84.0701935481991,9.38083151964701,60.90338912307));
#146297=CARTESIAN_POINT('Origin',(84.5911380811991,111.0724296188,63.857812382104));
#146298=CARTESIAN_POINT('',(84.330665814698,13.1050084134069,62.3806007525954));
#146299=CARTESIAN_POINT('',(84.3306658146991,13.10501209624,62.3806007526));
#146300=CARTESIAN_POINT('',(84.0366017122669,11.5683493747171,60.7128624132734));
#146301=CARTESIAN_POINT('Ctrl Pts',(84.3306655653021,13.105011407238,62.3805993381869));
#146302=CARTESIAN_POINT('Ctrl Pts',(84.2899365191375,12.9924913368189,62.149613439143));
#146303=CARTESIAN_POINT('Ctrl Pts',(84.251904294216,12.8600934104913,61.9339219733862));
#146304=CARTESIAN_POINT('Ctrl Pts',(84.2161389657171,12.7062180549234,61.731086716098));
#146305=CARTESIAN_POINT('Ctrl Pts',(84.1803735642168,12.5523423852767,61.5282510447979));
#146306=CARTESIAN_POINT('Ctrl Pts',(84.1468750683932,12.3769891987133,61.3382716344487));
#146307=CARTESIAN_POINT('Ctrl Pts',(84.1167829985401,12.1867580683441,61.1676110257763));
#146308=CARTESIAN_POINT('Ctrl Pts',(84.086690928687,11.996526937975,60.996950417104));
#146309=CARTESIAN_POINT('Ctrl Pts',(84.0600052848046,11.7914178638,60.8456086101085));
#146310=CARTESIAN_POINT('Ctrl Pts',(84.0365986439827,11.56834937513,60.7128629535571));
#146311=CARTESIAN_POINT('',(83.740534258072,9.21680318446827,59.0338374816974));
#146312=CARTESIAN_POINT('Ctrl Pts',(84.0366011831691,11.56834937513,60.71286250583));
#146313=CARTESIAN_POINT('Ctrl Pts',(84.0167422397526,11.3787529588475,60.6002516892439));
#146314=CARTESIAN_POINT('Ctrl Pts',(83.9799695099432,11.0446386484641,60.3917031752184));
#146315=CARTESIAN_POINT('Ctrl Pts',(83.9396547409223,10.7064633197752,60.1630667586076));
#146316=CARTESIAN_POINT('Ctrl Pts',(83.9157502918788,10.5122257397148,60.0274978913397));
#146317=CARTESIAN_POINT('Ctrl Pts',(83.9098596338177,10.4648391987288,59.9940903093718));
#146318=CARTESIAN_POINT('Ctrl Pts',(83.8533537997807,10.0150112533668,59.6736298000958));
#146319=CARTESIAN_POINT('Ctrl Pts',(83.7990070452368,9.6156595428362,59.3654140390955));
#146320=CARTESIAN_POINT('Ctrl Pts',(83.7405348394891,9.21680318431901,59.03383737954));
#146321=CARTESIAN_POINT('',(83.6360715663934,8.5371408778779,58.4413608714745));
#146322=CARTESIAN_POINT('Ctrl Pts',(83.740540996078,9.21680318437712,59.0338362937156));
#146323=CARTESIAN_POINT('Ctrl Pts',(83.727194557133,9.12572250911644,58.9581448314892));
#146324=CARTESIAN_POINT('Ctrl Pts',(83.7136768037681,9.0352116665213,58.8814821806832));
#146325=CARTESIAN_POINT('Ctrl Pts',(83.6999874765571,8.94527466677724,58.8038461597189));
#146326=CARTESIAN_POINT('Ctrl Pts',(83.6963779326866,8.92156045926676,58.7833754222396));
#146327=CARTESIAN_POINT('Ctrl Pts',(83.6927564621468,8.89788616303864,58.7628370117057));
#146328=CARTESIAN_POINT('Ctrl Pts',(83.6891230432056,8.87425175631427,58.7422308289417));
#146329=CARTESIAN_POINT('Ctrl Pts',(83.6717100607189,8.76098501855649,58.6434767063383));
#146330=CARTESIAN_POINT('Ctrl Pts',(83.6540227449861,8.64863571554548,58.5431668919965));
#146331=CARTESIAN_POINT('Ctrl Pts',(83.6360740268018,8.5371330073123,58.4413748701116));
#146332=CARTESIAN_POINT('',(83.6360659838734,-8.53719636731526,58.4413293403224));
#146333=CARTESIAN_POINT('',(83.6360730593091,8.53712703774001,58.44136942158));
#146334=CARTESIAN_POINT('',(83.7405267536393,-9.2167985425004,59.0338347984847));
#146335=CARTESIAN_POINT('Ctrl Pts',(83.6360729920622,-8.53720311761702,
58.4413691055294));
#146336=CARTESIAN_POINT('Ctrl Pts',(83.6540184616861,-8.64860998521598,
58.5431429211518));
#146337=CARTESIAN_POINT('Ctrl Pts',(83.6717001000893,-8.76092172492552,
58.6434204755692));
#146338=CARTESIAN_POINT('Ctrl Pts',(83.6891112932783,-8.874175396646,58.7421642589597));
#146339=CARTESIAN_POINT('Ctrl Pts',(83.7065246051586,-8.98744284970651,
58.8409200580459));
#146340=CARTESIAN_POINT('Ctrl Pts',(83.7236674060021,-9.101652464031,58.9381417128067));
#146341=CARTESIAN_POINT('Ctrl Pts',(83.7405402591061,-9.21679854220001,
59.0338324178608));
#146342=CARTESIAN_POINT('',(84.0366041203994,-11.56837406741,60.7128837058028));
#146343=CARTESIAN_POINT('Ctrl Pts',(83.7405343424891,-9.21679854219999,
59.03383346112));
#146344=CARTESIAN_POINT('Ctrl Pts',(83.7697426624094,-9.41601561043767,
59.1994474768037));
#146345=CARTESIAN_POINT('Ctrl Pts',(83.8190639716081,-9.76498641488459,
59.4791625209821));
#146346=CARTESIAN_POINT('Ctrl Pts',(83.8652652117883,-10.1145538556358,
59.7411827744601));
#146347=CARTESIAN_POINT('Ctrl Pts',(83.8909018219276,-10.3144527939354,
59.8865752154596));
#146348=CARTESIAN_POINT('Ctrl Pts',(83.8974093805898,-10.365729764731,59.923481414591));
#146349=CARTESIAN_POINT('Ctrl Pts',(83.9524868765521,-10.8041110086998,
60.2358414161119));
#146350=CARTESIAN_POINT('Ctrl Pts',(83.9968446284176,-11.1887561005569,
60.4874067278259));
#146351=CARTESIAN_POINT('Ctrl Pts',(84.0366050016191,-11.56837406741,60.71288355042));
#146352=CARTESIAN_POINT('',(84.330665789694,-13.1050131369444,62.3806006107895));
#146353=CARTESIAN_POINT('Ctrl Pts',(84.0366023579599,-11.56837406741,60.7128840165684));
#146354=CARTESIAN_POINT('Ctrl Pts',(84.0600599759165,-11.79192430949,60.8459187788173));
#146355=CARTESIAN_POINT('Ctrl Pts',(84.0867960216265,-11.99729070149,60.9975464287807));
#146356=CARTESIAN_POINT('Ctrl Pts',(84.1169120167458,-12.1875766534583,
61.1683427243805));
#146357=CARTESIAN_POINT('Ctrl Pts',(84.1470280118651,-12.3778626054267,
61.3391390199804));
#146358=CARTESIAN_POINT('Ctrl Pts',(84.1805239563937,-12.5530681173634,
61.5291039612167));
#146359=CARTESIAN_POINT('Ctrl Pts',(84.216268215619,-12.7067726588867,61.7318197287167));
#146360=CARTESIAN_POINT('Ctrl Pts',(84.2520124748443,-12.86047720041,61.9345354962168));
#146361=CARTESIAN_POINT('Ctrl Pts',(84.2900050487662,-12.99268077152,62.1500020899805));
#146362=CARTESIAN_POINT('Ctrl Pts',(84.3306658146978,-13.10501209624,62.3806007525802));
#146363=CARTESIAN_POINT('',(84.3306658146583,-9.38083151966199,62.3806007523748));
#146364=CARTESIAN_POINT('',(84.3306658146191,-9.38083151966199,62.38060075216));
#146365=CARTESIAN_POINT('',(84.0701935481991,-9.38083151964699,60.90338912307));
#146366=CARTESIAN_POINT('',(84.3306658146191,-9.38083151966199,62.38060075216));
#146367=CARTESIAN_POINT('',(84.0701935481991,-9.38083151964699,60.90338912307));
#146368=CARTESIAN_POINT('Origin',(83.0853857951891,-11.87956405717,61.07703730073));
#146369=CARTESIAN_POINT('',(83.8670110335795,-7.66994744389929,61.7007856367688));
#146370=CARTESIAN_POINT('Ctrl Pts',(83.8670110335795,-7.66994744389929,
61.7007856367688));
#146371=CARTESIAN_POINT('Ctrl Pts',(83.8877308381727,-7.72304817206258,
61.67482144373));
#146372=CARTESIAN_POINT('Ctrl Pts',(83.9066801507776,-7.77708798385845,
61.648427071772));
#146373=CARTESIAN_POINT('Ctrl Pts',(83.9239978184073,-7.83191890481131,
61.6217664761134));
#146374=CARTESIAN_POINT('Ctrl Pts',(83.942232338449,-7.88965274913706,61.593694383713));
#146375=CARTESIAN_POINT('Ctrl Pts',(83.9586585766351,-7.94826368775387,
61.5653269014276));
#146376=CARTESIAN_POINT('Ctrl Pts',(83.9734288711074,-8.00757897719989,
61.5367975592492));
#146377=CARTESIAN_POINT('Ctrl Pts',(83.9886134799562,-8.06855809110232,
61.5074679543107));
#146378=CARTESIAN_POINT('Ctrl Pts',(84.0020485456467,-8.13028162484728,
61.477966711392));
#146379=CARTESIAN_POINT('Ctrl Pts',(84.0138793093052,-8.19256188677082,
61.4483859162442));
#146380=CARTESIAN_POINT('Ctrl Pts',(84.0261862036942,-8.25734862650568,
61.4176146378776));
#146381=CARTESIAN_POINT('Ctrl Pts',(84.0367576686922,-8.32273780734182,
61.3867566809908));
#146382=CARTESIAN_POINT('Ctrl Pts',(84.045726040153,-8.388518152353,61.3558680987108));
#146383=CARTESIAN_POINT('Ctrl Pts',(84.0509005473253,-8.42647162791296,
61.3380462242216));
#146384=CARTESIAN_POINT('Ctrl Pts',(84.0555407617356,-8.46455532113187,
61.3202133320056));
#146385=CARTESIAN_POINT('Ctrl Pts',(84.0596665974345,-8.5027286514264,61.3023746442309));
#146386=CARTESIAN_POINT('Ctrl Pts',(84.0679871904554,-8.57971299322025,
61.2663992754013));
#146387=CARTESIAN_POINT('Ctrl Pts',(84.0742039804002,-8.65709134161381,
61.2304615370746));
#146388=CARTESIAN_POINT('Ctrl Pts',(84.078445246042,-8.73478433456591,61.1946507654007));
#146389=CARTESIAN_POINT('Ctrl Pts',(84.0827823726163,-8.81423334173372,
61.1580305999612));
#146390=CARTESIAN_POINT('Ctrl Pts',(84.0850540629707,-8.89401137736572,
61.1215421469891));
#146391=CARTESIAN_POINT('Ctrl Pts',(84.0853520837786,-8.97403357566445,
61.0852483715776));
#146392=CARTESIAN_POINT('Ctrl Pts',(84.0856564729272,-9.05576575058707,
61.0481790425214));
#146393=CARTESIAN_POINT('Ctrl Pts',(84.0839021793659,-9.13775263458298,
61.0113116213905));
#146394=CARTESIAN_POINT('Ctrl Pts',(84.0801352228852,-9.21990380433592,
60.9746968097292));
#146395=CARTESIAN_POINT('Ctrl Pts',(84.0776783196428,-9.27348485215759,
60.95081571369));
#146396=CARTESIAN_POINT('Ctrl Pts',(84.0743641506513,-9.32713578672443,
60.9270417849153));
#146397=CARTESIAN_POINT('Ctrl Pts',(84.0701935482024,-9.38083151964699,
60.9033891230694));
#146398=CARTESIAN_POINT('Ctrl Pts',(83.2590363734724,-6.9829160281516,62.0618549710651));
#146399=CARTESIAN_POINT('Ctrl Pts',(83.282289361152,-6.99276570574769,62.0577559880571));
#146400=CARTESIAN_POINT('Ctrl Pts',(83.3067925291477,-7.00454606434442,
62.0525868755333));
#146401=CARTESIAN_POINT('Ctrl Pts',(83.3323113975882,-7.01851063662673,
62.046084087642));
#146402=CARTESIAN_POINT('Ctrl Pts',(83.3578302660286,-7.03247520890904,
62.0395812997506));
#146403=CARTESIAN_POINT('Ctrl Pts',(83.3843643714203,-7.0486240708107,62.0317442661474));
#146404=CARTESIAN_POINT('Ctrl Pts',(83.4116337788324,-7.06724343137114,
62.0223229982725));
#146405=CARTESIAN_POINT('Ctrl Pts',(83.436142258631,-7.08397764987694,62.0138555992601));
#146406=CARTESIAN_POINT('Ctrl Pts',(83.4612451921201,-7.10270815720052,
62.0041068565072));
#146407=CARTESIAN_POINT('Ctrl Pts',(83.4866821771397,-7.12365747172556,
61.9929546294659));
#146408=CARTESIAN_POINT('Ctrl Pts',(83.5121191621594,-7.14460678625059,
61.9818024024245));
#146409=CARTESIAN_POINT('Ctrl Pts',(83.5378901428163,-7.16777501729968,
61.9692463862192));
#146410=CARTESIAN_POINT('Ctrl Pts',(83.5636960707018,-7.19340099565594,
61.9552021971918));
#146411=CARTESIAN_POINT('Ctrl Pts',(83.5864308247299,-7.21597721602059,
61.9428294127494));
#146412=CARTESIAN_POINT('Ctrl Pts',(83.6091922328673,-7.24046130049242,
61.9293019787599));
#146413=CARTESIAN_POINT('Ctrl Pts',(83.6317511913142,-7.26702562691842,
61.9145891050788));
#146414=CARTESIAN_POINT('Ctrl Pts',(83.6541863104381,-7.29344412621307,
61.8999569989702));
#146415=CARTESIAN_POINT('Ctrl Pts',(83.6764207471435,-7.32192008762135,
61.8841506374782));
#146416=CARTESIAN_POINT('Ctrl Pts',(83.6982293579439,-7.35263870495623,
61.8672313618185));
#146417=CARTESIAN_POINT('Ctrl Pts',(83.7195548675035,-7.38267684785449,
61.8506868795439));
#146418=CARTESIAN_POINT('Ctrl Pts',(83.7404731816077,-7.41485975670852,
61.8330781446068));
#146419=CARTESIAN_POINT('Ctrl Pts',(83.7607573278311,-7.44936440703707,
61.8145090737762));
#146420=CARTESIAN_POINT('Ctrl Pts',(83.7696671104134,-7.46452052596472,
61.806352635638));
#146421=CARTESIAN_POINT('Ctrl Pts',(83.778454322578,-7.48012461781848,61.7980115321834));
#146422=CARTESIAN_POINT('Ctrl Pts',(83.7870987073549,-7.49619158640237,
61.7894976170954));
#146423=CARTESIAN_POINT('Ctrl Pts',(83.8052065587327,-7.5298479178492,61.7716630674965));
#146424=CARTESIAN_POINT('Ctrl Pts',(83.8226877130566,-7.56553553137317,
61.7530667791856));
#146425=CARTESIAN_POINT('Ctrl Pts',(83.8393888914259,-7.60341084157583,
61.7338939949398));
#146426=CARTESIAN_POINT('Ctrl Pts',(83.8488547931309,-7.62487782764677,
61.7230272352976));
#146427=CARTESIAN_POINT('Ctrl Pts',(83.8580700758562,-7.64704755743563,
61.7119761780314));
#146428=CARTESIAN_POINT('Ctrl Pts',(83.8670064350194,-7.669947443743,61.7007819662909));
#146429=CARTESIAN_POINT('Ctrl Pts',(83.1513105236491,-7.93829473335598,
63.194966112929));
#146430=CARTESIAN_POINT('Ctrl Pts',(83.264872395859,-7.957053728333,63.182689563492));
#146431=CARTESIAN_POINT('Ctrl Pts',(83.5018558838091,-8.01558777810299,
63.1281192597161));
#146432=CARTESIAN_POINT('Ctrl Pts',(83.793035941679,-8.14822056533799,62.98049002751));
#146433=CARTESIAN_POINT('Ctrl Pts',(84.007518739009,-8.31001055232898,62.80322092744));
#146434=CARTESIAN_POINT('Ctrl Pts',(84.1262881301092,-8.44906746979797,
62.6628219159601));
#146435=CARTESIAN_POINT('Ctrl Pts',(84.1780214029591,-8.53201891951698,
62.5865012713));
#146436=CARTESIAN_POINT('Ctrl Pts',(84.1930532967891,-8.55878077391199,
62.56272764659));
#146437=CARTESIAN_POINT('Ctrl Pts',(83.0525582468391,-8.02666120745799,
62.41257219589));
#146438=CARTESIAN_POINT('Ctrl Pts',(83.1031659906391,-8.03504796986499,
62.40712679656));
#146439=CARTESIAN_POINT('Ctrl Pts',(83.2123457583091,-8.06157435232,62.38250638988));
#146440=CARTESIAN_POINT('Ctrl Pts',(83.3637640416291,-8.12919594766799,
62.30742514836));
#146441=CARTESIAN_POINT('Ctrl Pts',(83.4927183665891,-8.22488484773499,
62.20236174747));
#146442=CARTESIAN_POINT('Ctrl Pts',(83.5748180822491,-8.31962531502999,
62.1063728352201));
#146443=CARTESIAN_POINT('Ctrl Pts',(83.6142389534991,-8.38260961938299,
62.04833795058));
#146444=CARTESIAN_POINT('Ctrl Pts',(83.6260728217892,-8.40367762948599,
62.02962298588));
#146445=CARTESIAN_POINT('Ctrl Pts',(83.0961181729091,-7.42626321265199,
61.89553186311));
#146446=CARTESIAN_POINT('Ctrl Pts',(83.1380603031291,-7.43324549126899,
61.89104875086));
#146447=CARTESIAN_POINT('Ctrl Pts',(83.2327226191091,-7.45574602055999,
61.8702911395001));
#146448=CARTESIAN_POINT('Ctrl Pts',(83.3835527426891,-7.52175173551999,
61.79719441311));
#146449=CARTESIAN_POINT('Ctrl Pts',(83.5294730142391,-7.62865565051299,
61.67962372064));
#146450=CARTESIAN_POINT('Ctrl Pts',(83.6316464408291,-7.74551728364799,
61.56096647174));
#146451=CARTESIAN_POINT('Ctrl Pts',(83.6834667115091,-7.82815871933699,
61.48476057679));
#146452=CARTESIAN_POINT('Ctrl Pts',(83.6992824959991,-7.85631560981899,
61.45974886626));
#146453=CARTESIAN_POINT('Ctrl Pts',(83.2429027023891,-6.67585548217199,
62.10780057242));
#146454=CARTESIAN_POINT('Ctrl Pts',(83.3382436431191,-6.69166131028399,
62.09754739579));
#146455=CARTESIAN_POINT('Ctrl Pts',(83.544701711279,-6.74173031670498,62.05109927843));
#146456=CARTESIAN_POINT('Ctrl Pts',(83.8346450628892,-6.87096543964799,
61.90764282796));
#146457=CARTESIAN_POINT('Ctrl Pts',(84.0848016584592,-7.05633690953499,
61.7040750128));
#146458=CARTESIAN_POINT('Ctrl Pts',(84.2457794526591,-7.24190735349899,
61.51601195481));
#146459=CARTESIAN_POINT('Ctrl Pts',(84.3235845789591,-7.36619127664198,
61.4014836598));
#146460=CARTESIAN_POINT('Ctrl Pts',(84.3469891311591,-7.40785871185899,
61.36447005234));
#146461=CARTESIAN_POINT('',(83.2009909607981,-7.94208206191376,62.8844208924415));
#146462=CARTESIAN_POINT('Ctrl Pts',(83.2009862869082,-7.94210140073919,
62.8844176222466));
#146463=CARTESIAN_POINT('Ctrl Pts',(83.1968609444218,-7.93589258748885,
62.8535949750669));
#146464=CARTESIAN_POINT('Ctrl Pts',(83.1930177536416,-7.92812896197403,
62.8224913291405));
#146465=CARTESIAN_POINT('Ctrl Pts',(83.1895151218238,-7.91871788470194,
62.791331832236));
#146466=CARTESIAN_POINT('Ctrl Pts',(83.1860613434666,-7.90943806978235,
62.7606069368919));
#146467=CARTESIAN_POINT('Ctrl Pts',(83.1829389107385,-7.8985558891018,62.7298283228265));
#146468=CARTESIAN_POINT('Ctrl Pts',(83.1802003270392,-7.88602364173719,
62.6992405351296));
#146469=CARTESIAN_POINT('Ctrl Pts',(83.1775058788668,-7.87369336641399,
62.6691457059375));
#146470=CARTESIAN_POINT('Ctrl Pts',(83.1751832107692,-7.85976544420628,
62.6392363428651));
#146471=CARTESIAN_POINT('Ctrl Pts',(83.1732757839844,-7.84424106305769,
62.6097634807669));
#146472=CARTESIAN_POINT('Ctrl Pts',(83.1725527987444,-7.83835674890296,
62.5985921768699));
#146473=CARTESIAN_POINT('Ctrl Pts',(83.1718893871919,-7.83224358151196,
62.5874837139982));
#146474=CARTESIAN_POINT('Ctrl Pts',(83.1712875738902,-7.82590353889161,
62.5764520960335));
#146475=CARTESIAN_POINT('Ctrl Pts',(83.1697259221037,-7.80945169434663,
62.5478260323457));
#146476=CARTESIAN_POINT('Ctrl Pts',(83.1685797522826,-7.79146864491412,
62.5197178703259));
#146477=CARTESIAN_POINT('Ctrl Pts',(83.1678774334007,-7.77202362631577,
62.4923718004139));
#146478=CARTESIAN_POINT('Ctrl Pts',(83.1671796572841,-7.7527043827144,62.4652026113747));
#146479=CARTESIAN_POINT('Ctrl Pts',(83.1669201223469,-7.73194218273304,
62.438786525598));
#146480=CARTESIAN_POINT('Ctrl Pts',(83.1671144478248,-7.70985343530854,
62.4133520640267));
#146481=CARTESIAN_POINT('Ctrl Pts',(83.1673079982892,-7.68785278275714,
62.3880190407859));
#146482=CARTESIAN_POINT('Ctrl Pts',(83.1679518517265,-7.66453652820068,
62.3636606057523));
#146483=CARTESIAN_POINT('Ctrl Pts',(83.1690480192404,-7.64006390061212,
62.3404795080263));
#146484=CARTESIAN_POINT('Ctrl Pts',(83.1701512360192,-7.61543389376028,
62.3171493366436));
#146485=CARTESIAN_POINT('Ctrl Pts',(83.1717126130741,-7.58963314283984,
62.2950124109263));
#146486=CARTESIAN_POINT('Ctrl Pts',(83.1737200409363,-7.56286188520676,
62.274240623076));
#146487=CARTESIAN_POINT('Ctrl Pts',(83.1757178816941,-7.53621848215234,
62.2535680374456));
#146488=CARTESIAN_POINT('Ctrl Pts',(83.1781574363581,-7.50861459563722,
62.2342480221177));
#146489=CARTESIAN_POINT('Ctrl Pts',(83.1810134084009,-7.48027493168117,
62.216407035279));
#146490=CARTESIAN_POINT('Ctrl Pts',(83.1838931323914,-7.4516995783667,62.1984176722723));
#146491=CARTESIAN_POINT('Ctrl Pts',(83.1871961048047,-7.4223769946218,62.1819323415515));
#146492=CARTESIAN_POINT('Ctrl Pts',(83.1908843299669,-7.39255325226539,
62.1670311076611));
#146493=CARTESIAN_POINT('Ctrl Pts',(83.1945643726918,-7.36279567476835,
62.1521629326013));
#146494=CARTESIAN_POINT('Ctrl Pts',(83.1986277702836,-7.33254001686404,
62.1388717827871));
#146495=CARTESIAN_POINT('Ctrl Pts',(83.2030272346504,-7.30203343974707,
62.1271862973236));
#146496=CARTESIAN_POINT('Ctrl Pts',(83.2075236494605,-7.27085459302483,
62.1152433002858));
#146497=CARTESIAN_POINT('Ctrl Pts',(83.2123707521351,-7.23941441702322,
62.1049774188593));
#146498=CARTESIAN_POINT('Ctrl Pts',(83.217510289309,-7.20796636671036,62.096367038009));
#146499=CARTESIAN_POINT('Ctrl Pts',(83.2227040839583,-7.17618632311442,
62.0876657584042));
#146500=CARTESIAN_POINT('Ctrl Pts',(83.2281962897528,-7.14439897464933,
62.0806546693344));
#146501=CARTESIAN_POINT('Ctrl Pts',(83.2339228693355,-7.11284321740108,
62.0752629920924));
#146502=CARTESIAN_POINT('Ctrl Pts',(83.2397622659586,-7.08066579287576,
62.0697650955865));
#146503=CARTESIAN_POINT('Ctrl Pts',(83.245845131012,-7.04872979197433,62.0659504563783));
#146504=CARTESIAN_POINT('Ctrl Pts',(83.2521030588475,-7.01725456501231,
62.0637017729808));
#146505=CARTESIAN_POINT('Ctrl Pts',(83.2543914510472,-7.00574473847601,
62.0628794768979));
#146506=CARTESIAN_POINT('Ctrl Pts',(83.2567032652368,-6.99429616000662,
62.062266226382));
#146507=CARTESIAN_POINT('Ctrl Pts',(83.2590352295789,-6.98291823983333,
62.0618551727003));
#146508=CARTESIAN_POINT('',(83.9305070695251,-8.35425122912034,62.451223254077));
#146509=CARTESIAN_POINT('Ctrl Pts',(83.9304978963085,-8.3542226563704,62.4512190361288));
#146510=CARTESIAN_POINT('Ctrl Pts',(83.9171890192848,-8.34413946079924,
62.4302377284297));
#146511=CARTESIAN_POINT('Ctrl Pts',(83.9042062657205,-8.33297575049901,
62.4084312846382));
#146512=CARTESIAN_POINT('Ctrl Pts',(83.8917600544071,-8.32062588453196,
62.3858523588766));
#146513=CARTESIAN_POINT('Ctrl Pts',(83.8797850045273,-8.30874353276729,
62.3641281766803));
#146514=CARTESIAN_POINT('Ctrl Pts',(83.8683071406987,-8.29576258438283,
62.3416887413461));
#146515=CARTESIAN_POINT('Ctrl Pts',(83.8575356795425,-8.28160799316187,
62.3186183448306));
#146516=CARTESIAN_POINT('Ctrl Pts',(83.8480119751002,-8.26909305750599,
62.2982204030292));
#146517=CARTESIAN_POINT('Ctrl Pts',(83.8390410731563,-8.2556605856278,62.2773296366975));
#146518=CARTESIAN_POINT('Ctrl Pts',(83.8307772578393,-8.24127725732503,
62.2560312206357));
#146519=CARTESIAN_POINT('Ctrl Pts',(83.82186485708,-8.22576505367934,62.2330611986542));
#146520=CARTESIAN_POINT('Ctrl Pts',(83.8137756270682,-8.20914632687142,
62.2096168110415));
#146521=CARTESIAN_POINT('Ctrl Pts',(83.8067059121274,-8.19140860833201,
62.185842001208));
#146522=CARTESIAN_POINT('Ctrl Pts',(83.8029369618848,-8.1819524167948,62.1731673635399));
#146523=CARTESIAN_POINT('Ctrl Pts',(83.7994577864604,-8.17217878861295,
62.1603994365102));
#146524=CARTESIAN_POINT('Ctrl Pts',(83.7962975892537,-8.16209030713504,
62.1475641665206));
#146525=CARTESIAN_POINT('Ctrl Pts',(83.7917535760363,-8.14758418926295,
62.1291084713005));
#146526=CARTESIAN_POINT('Ctrl Pts',(83.7878694125071,-8.13242640488484,
62.1105131109079));
#146527=CARTESIAN_POINT('Ctrl Pts',(83.7847278327247,-8.116637410475,62.0918650260291));
#146528=CARTESIAN_POINT('Ctrl Pts',(83.7831570428335,-8.10874291327008,
62.0825409835898));
#146529=CARTESIAN_POINT('Ctrl Pts',(83.78177180665,-8.10069085666175,62.0732039349876));
#146530=CARTESIAN_POINT('Ctrl Pts',(83.7805817563341,-8.09248530304138,
62.0638657206417));
#146531=CARTESIAN_POINT('Ctrl Pts',(83.7799240917833,-8.08795061936961,
62.0587050879681));
#146532=CARTESIAN_POINT('Ctrl Pts',(83.7792933688352,-8.08311536214206,
62.0532586758234));
#146533=CARTESIAN_POINT('Ctrl Pts',(83.778749465815,-8.07839873268998,62.0480028192095));
#146534=CARTESIAN_POINT('Ctrl Pts',(83.7783091711006,-8.07458057588619,
62.0437481528436));
#146535=CARTESIAN_POINT('Ctrl Pts',(83.7779247392201,-8.07084079598696,
62.0396181897044));
#146536=CARTESIAN_POINT('Ctrl Pts',(83.7776061937308,-8.0674132493151,62.035859999865));
#146537=CARTESIAN_POINT('Ctrl Pts',(83.7754984072372,-8.04473348512597,
62.0109923999474));
#146538=CARTESIAN_POINT('Ctrl Pts',(83.7748802107319,-8.02137383895631,
61.98661819215));
#146539=CARTESIAN_POINT('Ctrl Pts',(83.7757452476007,-7.9975176531896,61.9629193749232));
#146540=CARTESIAN_POINT('Ctrl Pts',(83.7766127091347,-7.97359459944707,
61.9391541308186));
#146541=CARTESIAN_POINT('Ctrl Pts',(83.7789715750591,-7.94917288402073,
61.9160686262253));
#146542=CARTESIAN_POINT('Ctrl Pts',(83.7827704559858,-7.92444881313273,
61.8938221111338));
#146543=CARTESIAN_POINT('Ctrl Pts',(83.7866067112694,-7.89948150054621,
61.8713567291679));
#146544=CARTESIAN_POINT('Ctrl Pts',(83.7919111255218,-7.87420655012517,
61.8497473758364));
#146545=CARTESIAN_POINT('Ctrl Pts',(83.7985885813855,-7.84882739185262,
61.8291255942874));
#146546=CARTESIAN_POINT('Ctrl Pts',(83.8053127266468,-7.82327078012543,
61.808359623308));
#146547=CARTESIAN_POINT('Ctrl Pts',(83.8134286419699,-7.79760916121798,
61.7885953306014));
#146548=CARTESIAN_POINT('Ctrl Pts',(83.8228032789842,-7.77204117685951,
61.7699289893133));
#146549=CARTESIAN_POINT('Ctrl Pts',(83.8323126753202,-7.74610565568599,
61.7509943215301));
#146550=CARTESIAN_POINT('Ctrl Pts',(83.8431165916147,-7.72026707691074,
61.7331894893711));
#146551=CARTESIAN_POINT('Ctrl Pts',(83.8550483663382,-7.69471378481215,
61.7165732848687));
#146552=CARTESIAN_POINT('Ctrl Pts',(83.8589179758298,-7.68642656317606,
61.7111844618188));
#146553=CARTESIAN_POINT('Ctrl Pts',(83.862906037903,-7.67816916362773,61.7059203292459));
#146554=CARTESIAN_POINT('Ctrl Pts',(83.8670064351955,-7.66994744419446,
61.7007819660702));
#146555=CARTESIAN_POINT('Ctrl Pts',(83.2009909607981,-7.94208206191376,
62.8844208924415));
#146556=CARTESIAN_POINT('Ctrl Pts',(83.2281670225282,-7.94783420853062,
62.8796179614531));
#146557=CARTESIAN_POINT('Ctrl Pts',(83.2557799101056,-7.95432167821131,
62.8736428485721));
#146558=CARTESIAN_POINT('Ctrl Pts',(83.2837135173524,-7.96165657404679,
62.866504562709));
#146559=CARTESIAN_POINT('Ctrl Pts',(83.3074796736338,-7.96789716729324,
62.8604312469391));
#146560=CARTESIAN_POINT('Ctrl Pts',(83.3314783642032,-7.9747513011514,62.8535164195537));
#146561=CARTESIAN_POINT('Ctrl Pts',(83.3556339282506,-7.98228535354528,
62.8457291378132));
#146562=CARTESIAN_POINT('Ctrl Pts',(83.3777271527932,-7.98917616805606,
62.8386067140217));
#146563=CARTESIAN_POINT('Ctrl Pts',(83.3999519971398,-7.99663580775826,
62.8307546185476));
#146564=CARTESIAN_POINT('Ctrl Pts',(83.4222414954207,-8.00471164959767,
62.8221119623137));
#146565=CARTESIAN_POINT('Ctrl Pts',(83.4497231308661,-8.01466868580137,
62.8114560774255));
#146566=CARTESIAN_POINT('Ctrl Pts',(83.4772986038528,-8.02556596420315,
62.7996349070896));
#146567=CARTESIAN_POINT('Ctrl Pts',(83.5048073038998,-8.03749391859776,
62.7866175289148));
#146568=CARTESIAN_POINT('Ctrl Pts',(83.5149872747595,-8.04190802133417,
62.7818002700016));
#146569=CARTESIAN_POINT('Ctrl Pts',(83.5251579439255,-8.04646318982533,
62.7768187441885));
#146570=CARTESIAN_POINT('Ctrl Pts',(83.5353104485783,-8.05116368426297,
62.7716696637962));
#146571=CARTESIAN_POINT('Ctrl Pts',(83.5541039408197,-8.05986485789111,
62.7621381042734));
#146572=CARTESIAN_POINT('Ctrl Pts',(83.5728350316721,-8.06906427407646,
62.7520359380708));
#146573=CARTESIAN_POINT('Ctrl Pts',(83.5914414113032,-8.07878738133277,
62.7413522091509));
#146574=CARTESIAN_POINT('Ctrl Pts',(83.6007446011188,-8.08364893496093,
62.7360103446909));
#146575=CARTESIAN_POINT('Ctrl Pts',(83.6100166058091,-8.08864142410212,
62.7305230886088));
#146576=CARTESIAN_POINT('Ctrl Pts',(83.6192489219252,-8.09376770771874,
62.724889277636));
#146577=CARTESIAN_POINT('Ctrl Pts',(83.6238650799833,-8.09633084952704,
62.7220723721496));
#146578=CARTESIAN_POINT('Ctrl Pts',(83.6284713157787,-8.09892744021904,
62.7192188279071));
#146579=CARTESIAN_POINT('Ctrl Pts',(83.6330665448275,-8.1015578272724,62.7163285084698));
#146580=CARTESIAN_POINT('Ctrl Pts',(83.6353641593519,-8.10287302079907,
62.7148833487512));
#146581=CARTESIAN_POINT('Ctrl Pts',(83.6376590221754,-8.10419666343821,
62.713428995233));
#146582=CARTESIAN_POINT('Ctrl Pts',(83.6399509952151,-8.10552879729796,
62.7119654317475));
#146583=CARTESIAN_POINT('Ctrl Pts',(83.6415565080225,-8.10646194875131,
62.7109402146616));
#146584=CARTESIAN_POINT('Ctrl Pts',(83.6437083400293,-8.10772030426501,
62.7095596759605));
#146585=CARTESIAN_POINT('Ctrl Pts',(83.6452547229997,-8.10862970828445,
62.7085597546232));
#146586=CARTESIAN_POINT('Ctrl Pts',(83.6459159014145,-8.10901853713185,
62.7081322237867));
#146587=CARTESIAN_POINT('Ctrl Pts',(83.6464667190264,-8.10934333658453,
62.7077748921016));
#146588=CARTESIAN_POINT('Ctrl Pts',(83.6468181061104,-8.10955071426685,
62.7075470955155));
#146589=CARTESIAN_POINT('Ctrl Pts',(83.6609113500737,-8.11786810669007,
62.6984107526942));
#146590=CARTESIAN_POINT('Ctrl Pts',(83.6761493632529,-8.12725369277389,
62.6881873915792));
#146591=CARTESIAN_POINT('Ctrl Pts',(83.6923132574621,-8.13783350053357,
62.6767294536937));
#146592=CARTESIAN_POINT('Ctrl Pts',(83.7079130162838,-8.14804406287054,
62.6656714088133));
#146593=CARTESIAN_POINT('Ctrl Pts',(83.7243749174002,-8.15936730271737,
62.6534622780592));
#146594=CARTESIAN_POINT('Ctrl Pts',(83.741461207875,-8.17193021827758,62.6399908037421));
#146595=CARTESIAN_POINT('Ctrl Pts',(83.7576258179059,-8.18381545639761,
62.6272460169671));
#146596=CARTESIAN_POINT('Ctrl Pts',(83.7743487743116,-8.19681056643385,
62.6133706978287));
#146597=CARTESIAN_POINT('Ctrl Pts',(83.791396945696,-8.21103063117005,62.5983031779341));
#146598=CARTESIAN_POINT('Ctrl Pts',(83.8079720798566,-8.22485613042504,
62.5836537379392));
#146599=CARTESIAN_POINT('Ctrl Pts',(83.8248541767592,-8.23983981935114,
62.5678767447202));
#146600=CARTESIAN_POINT('Ctrl Pts',(83.8418047246299,-8.25609055218577,
62.5509566094758));
#146601=CARTESIAN_POINT('Ctrl Pts',(83.8581533560038,-8.27176421906046,
62.5346373107714));
#146602=CARTESIAN_POINT('Ctrl Pts',(83.8745651391945,-8.28861678574483,
62.5172543098411));
#146603=CARTESIAN_POINT('Ctrl Pts',(83.8908103573094,-8.30674512902824,
62.4988387136964));
#146604=CARTESIAN_POINT('Ctrl Pts',(83.9042019757953,-8.32168908701729,
62.4836579610579));
#146605=CARTESIAN_POINT('Ctrl Pts',(83.917479982152,-8.33750004403912,62.4677762256421));
#146606=CARTESIAN_POINT('Ctrl Pts',(83.9305111742816,-8.35423003346305,
62.4512372195408));
#146607=CARTESIAN_POINT('Origin',(82.8534541851791,-9.38083151964699,62.64107301909));
#146608=CARTESIAN_POINT('Origin',(82.8534541851791,-9.38083151964699,62.64107301909));
#146609=CARTESIAN_POINT('',(83.1139265222929,-9.38083161253521,64.1182846361553));
#146610=CARTESIAN_POINT('Origin',(82.8534541851791,-9.38083151964699,62.64107301909));
#146611=CARTESIAN_POINT('',(81.9035260552726,-8.32029685773108,63.1131988274128));
#146612=CARTESIAN_POINT('Origin',(82.8534541851791,-9.38083151964699,62.64107301909));
#146613=CARTESIAN_POINT('Origin',(82.9055487652491,-9.38083151964699,62.93651606395));
#146614=CARTESIAN_POINT('Origin',(82.9402782740091,-9.38083151964699,63.133476895592));
#146615=CARTESIAN_POINT('Origin',(81.2702407042791,-7.61327378225099,63.427949577933));
#146616=CARTESIAN_POINT('Origin',(74.0770084968991,1.4210854715202E-14,
64.696310494594));
#146617=CARTESIAN_POINT('',(67.0545019141992,-9.08849701091377,65.731481543374));
#146618=CARTESIAN_POINT('Ctrl Pts',(67.0545019147976,-9.08849701139183,
65.7314815432678));
#146619=CARTESIAN_POINT('Ctrl Pts',(67.05231832276,-9.08149629921886,65.6877553753418));
#146620=CARTESIAN_POINT('Ctrl Pts',(67.0519935097677,-9.07221722874611,
65.6443013928565));
#146621=CARTESIAN_POINT('Ctrl Pts',(67.0535297172201,-9.06074116961122,
65.6015030780834));
#146622=CARTESIAN_POINT('Ctrl Pts',(67.0551227184189,-9.04884083939825,
65.5571225052427));
#146623=CARTESIAN_POINT('Ctrl Pts',(67.0587170898111,-9.03457794627075,
65.5134475618804));
#146624=CARTESIAN_POINT('Ctrl Pts',(67.0642780735054,-9.01808724623876,
65.4708926217762));
#146625=CARTESIAN_POINT('Ctrl Pts',(67.0696412490677,-9.00218313209702,
65.4298513910583));
#146626=CARTESIAN_POINT('Ctrl Pts',(67.0768333564601,-8.98420728490995,
65.3898522398811));
#146627=CARTESIAN_POINT('Ctrl Pts',(67.085790362286,-8.9643178708117,65.3512482201939));
#146628=CARTESIAN_POINT('Ctrl Pts',(67.094746074706,-8.9444313287763,65.3126497749882));
#146629=CARTESIAN_POINT('Ctrl Pts',(67.1054660812389,-8.92263198011543,
65.2754464602497));
#146630=CARTESIAN_POINT('Ctrl Pts',(67.1178552704815,-8.89911169370504,
65.2399665586183));
#146631=CARTESIAN_POINT('Ctrl Pts',(67.1302446240882,-8.87559109525728,
65.2044861862845));
#146632=CARTESIAN_POINT('Ctrl Pts',(67.1443030751752,-8.85034975810816,
65.170729642724));
#146633=CARTESIAN_POINT('Ctrl Pts',(67.159906081631,-8.8236099380638,65.1389948090526));
#146634=CARTESIAN_POINT('Ctrl Pts',(67.1616370485728,-8.82064347485965,
65.1354742088309));
#146635=CARTESIAN_POINT('Ctrl Pts',(67.16338699617,-8.81765859794769,65.1319784562168));
#146636=CARTESIAN_POINT('Ctrl Pts',(67.1651557332315,-8.81465563169097,
65.1285079318638));
#146637=CARTESIAN_POINT('Ctrl Pts',(67.1810999456227,-8.7875855075655,65.0972230232154));
#146638=CARTESIAN_POINT('Ctrl Pts',(67.1985731460612,-8.75904344674962,
65.067991317463));
#146639=CARTESIAN_POINT('Ctrl Pts',(67.2174209748346,-8.72928110048734,
65.0410707466328));
#146640=CARTESIAN_POINT('Ctrl Pts',(67.2369656124516,-8.69841843299819,
65.0131549157091));
#146641=CARTESIAN_POINT('Ctrl Pts',(67.2579883376272,-8.66624379144337,
64.9877248586781));
#146642=CARTESIAN_POINT('Ctrl Pts',(67.2802895307771,-8.6330621782672,64.965021818082));
#146643=CARTESIAN_POINT('Ctrl Pts',(67.3017974531902,-8.60106086080673,
64.943126342248));
#146644=CARTESIAN_POINT('Ctrl Pts',(67.3244941408036,-8.56812339116989,
64.9237672910116));
#146645=CARTESIAN_POINT('Ctrl Pts',(67.3481791255317,-8.5345402554752,64.9071155221357));
#146646=CARTESIAN_POINT('Ctrl Pts',(67.3718606906226,-8.50096196851232,
64.8904661574415));
#146647=CARTESIAN_POINT('Ctrl Pts',(67.3965300201918,-8.46673855222839,
64.8765234658199));
#146648=CARTESIAN_POINT('Ctrl Pts',(67.4219693026433,-8.43217175319865,
64.8654104757455));
#146649=CARTESIAN_POINT('Ctrl Pts',(67.4474089232091,-8.39760449474063,
64.8542973379681));
#146650=CARTESIAN_POINT('Ctrl Pts',(67.4736182520635,-8.36269420470903,
64.8460140928845));
#146651=CARTESIAN_POINT('Ctrl Pts',(67.5003658828917,-8.32774869419913,
64.8406338471304));
#146652=CARTESIAN_POINT('Ctrl Pts',(67.5033332164201,-8.32387190280511,
64.8400369724494));
#146653=CARTESIAN_POINT('Ctrl Pts',(67.5063071636439,-8.31999468080688,
64.8394757742891));
#146654=CARTESIAN_POINT('Ctrl Pts',(67.5092874005591,-8.31611745004299,
64.8389503137869));
#146655=CARTESIAN_POINT('Origin',(74.0422786883791,1.4210854715202E-14,
64.499347962919));
#146656=CARTESIAN_POINT('Origin',(73.9901844080691,1.4210854715202E-14,
64.203906618088));
#146657=CARTESIAN_POINT('',(66.3719565885174,-10.2467348102415,67.0703602807809));
#146658=CARTESIAN_POINT('Origin',(74.2506566745691,1.4210854715202E-14,
65.681118247606));
#146659=CARTESIAN_POINT('Ctrl Pts',(66.3719377767423,-10.2467141764814,
67.0703489624824));
#146660=CARTESIAN_POINT('Ctrl Pts',(66.4084017164395,-10.199381809132,67.0639183297397));
#146661=CARTESIAN_POINT('Ctrl Pts',(66.4442296537897,-10.1520433256366,
67.0539284012353));
#146662=CARTESIAN_POINT('Ctrl Pts',(66.4791651716259,-10.1050413196356,
67.0404508581616));
#146663=CARTESIAN_POINT('Ctrl Pts',(66.5140986365642,-10.0580420755894,
67.0269741070618));
#146664=CARTESIAN_POINT('Ctrl Pts',(66.5481395450799,-10.0113795967587,
67.0100102452616));
#146665=CARTESIAN_POINT('Ctrl Pts',(66.5810442303557,-9.96539144021289,
66.9896812286782));
#146666=CARTESIAN_POINT('Ctrl Pts',(66.6139549715822,-9.91939481976567,
66.969348470636));
#146667=CARTESIAN_POINT('Ctrl Pts',(66.6457288424415,-9.87407309027168,
66.9456494588101));
#146668=CARTESIAN_POINT('Ctrl Pts',(66.6761382860771,-9.82975415389626,
66.9187547716618));
#146669=CARTESIAN_POINT('Ctrl Pts',(66.7065433412699,-9.78544161326815,
66.8918639657354));
#146670=CARTESIAN_POINT('Ctrl Pts',(66.7355841521626,-9.74213188408042,
66.8617785948035));
#146671=CARTESIAN_POINT('Ctrl Pts',(66.7630527981812,-9.70013817434927,
66.8287152352373));
#146672=CARTESIAN_POINT('Ctrl Pts',(66.790524079827,-9.65814043530542,66.7956487032289));
#146673=CARTESIAN_POINT('Ctrl Pts',(66.8164227032188,-9.61745926028037,
66.7596038403276));
#146674=CARTESIAN_POINT('Ctrl Pts',(66.8405632538059,-9.57838888827831,
66.7208402393864));
#146675=CARTESIAN_POINT('Ctrl Pts',(66.8573825149536,-9.55116768686174,
66.6938327722244));
#146676=CARTESIAN_POINT('Ctrl Pts',(66.8733488394468,-9.52472800867184,
66.6655064724249));
#146677=CARTESIAN_POINT('Ctrl Pts',(66.8884067047024,-9.49916279037104,
66.6359604921911));
#146678=CARTESIAN_POINT('Ctrl Pts',(66.9100174794419,-9.46247205337188,
66.5935566379629));
#146679=CARTESIAN_POINT('Ctrl Pts',(66.929755988921,-9.42758391409385,66.5486391633832));
#146680=CARTESIAN_POINT('Ctrl Pts',(66.9474800086736,-9.39474983739101,
66.501531784445));
#146681=CARTESIAN_POINT('Ctrl Pts',(66.9652029887504,-9.36191768670704,
66.4544271687855));
#146682=CARTESIAN_POINT('Ctrl Pts',(66.9809115925191,-9.33113958549307,
66.4051332333531));
#146683=CARTESIAN_POINT('Ctrl Pts',(66.9944926518804,-9.30263735104727,
66.3540051939298));
#146684=CARTESIAN_POINT('Ctrl Pts',(67.0080762112771,-9.27412986983884,
66.3028677427291));
#146685=CARTESIAN_POINT('Ctrl Pts',(67.0195313475018,-9.2478992925461,66.2498958669422));
#146686=CARTESIAN_POINT('Ctrl Pts',(67.0287755137373,-9.22413473587621,
66.1954714264602));
#146687=CARTESIAN_POINT('Ctrl Pts',(67.0380183454304,-9.20037360999825,
66.1410548430123));
#146688=CARTESIAN_POINT('Ctrl Pts',(67.0450507819468,-9.17907795707956,
66.0851864930388));
#146689=CARTESIAN_POINT('Ctrl Pts',(67.0498221747758,-9.16040127550207,
66.0282690003933));
#146690=CARTESIAN_POINT('Ctrl Pts',(67.0545940249536,-9.14172280372224,
65.9713460520768));
#146691=CARTESIAN_POINT('Ctrl Pts',(67.0571043642474,-9.12566393580531,
65.9133741554404));
#146692=CARTESIAN_POINT('Ctrl Pts',(67.0573351324854,-9.11234045373913,
65.85477117363));
#146693=CARTESIAN_POINT('Ctrl Pts',(67.0574959471453,-9.10305576509771,
65.8139327173717));
#146694=CARTESIAN_POINT('Ctrl Pts',(67.0565504325796,-9.09509865285608,
65.7727881131849));
#146695=CARTESIAN_POINT('Ctrl Pts',(67.0545019148004,-9.0884970113884,65.7314815432682));
#146696=CARTESIAN_POINT('Ctrl Pts',(66.3062970743491,-10.66489088643,67.041769621825));
#146697=CARTESIAN_POINT('Ctrl Pts',(66.2504617153091,-10.58427361457,67.053542835718));
#146698=CARTESIAN_POINT('Ctrl Pts',(66.0547528912291,-10.2876201762,67.106528502032));
#146699=CARTESIAN_POINT('Ctrl Pts',(65.7753967212292,-9.779459606408,67.246161639635));
#146700=CARTESIAN_POINT('Ctrl Pts',(65.5119315184691,-9.16743128369398,
67.4698540222511));
#146701=CARTESIAN_POINT('Ctrl Pts',(65.3288460021691,-8.62877957219299,
67.705374609763));
#146702=CARTESIAN_POINT('Ctrl Pts',(65.2062279860991,-8.16440041052299,
67.942334778192));
#146703=CARTESIAN_POINT('Ctrl Pts',(65.1320446995391,-7.77960342737999,
68.174487400817));
#146704=CARTESIAN_POINT('Ctrl Pts',(65.0980975644191,-7.48390022505899,
68.396209689244));
#146705=CARTESIAN_POINT('Ctrl Pts',(65.0969663795691,-7.29264316256499,
68.598155241067));
#146706=CARTESIAN_POINT('Ctrl Pts',(65.1139303495591,-7.22517886813799,
68.749749824733));
#146707=CARTESIAN_POINT('Ctrl Pts',(65.1293731629891,-7.22766901996699,
68.835084325791));
#146708=CARTESIAN_POINT('Ctrl Pts',(65.1353202143191,-7.23318211597299,
68.864201267989));
#146709=CARTESIAN_POINT('Ctrl Pts',(66.9228783679491,-9.857884207097,67.18800044511));
#146710=CARTESIAN_POINT('Ctrl Pts',(66.8813725186591,-9.78412567680498,
67.1771385985831));
#146711=CARTESIAN_POINT('Ctrl Pts',(66.7297181498991,-9.510843685412,67.145288462166));
#146712=CARTESIAN_POINT('Ctrl Pts',(66.4767641188491,-9.03120867882798,
67.138102774496));
#146713=CARTESIAN_POINT('Ctrl Pts',(66.1820507100991,-8.43327718432299,
67.201352307393));
#146714=CARTESIAN_POINT('Ctrl Pts',(65.9284768389591,-7.88808399311499,
67.317910472815));
#146715=CARTESIAN_POINT('Ctrl Pts',(65.7113975443191,-7.39715233850599,
67.480135816037));
#146716=CARTESIAN_POINT('Ctrl Pts',(65.5295093985692,-6.96458385138599,
67.6891203028381));
#146717=CARTESIAN_POINT('Ctrl Pts',(65.3870747679392,-6.59986960464899,
67.9543145934371));
#146718=CARTESIAN_POINT('Ctrl Pts',(65.2999640064091,-6.32849541217299,
68.288796224779));
#146719=CARTESIAN_POINT('Ctrl Pts',(65.2986301726591,-6.21755287707399,
68.628674831736));
#146720=CARTESIAN_POINT('Ctrl Pts',(65.3361506337991,-6.222198461074,68.82847382208));
#146721=CARTESIAN_POINT('Ctrl Pts',(65.3527548091692,-6.23109205796199,
68.8946036571191));
#146722=CARTESIAN_POINT('Ctrl Pts',(67.3317483081991,-9.21987568814898,
66.4962091862191));
#146723=CARTESIAN_POINT('Ctrl Pts',(67.2730998070291,-9.15153958578098,
66.470222614952));
#146724=CARTESIAN_POINT('Ctrl Pts',(67.0554617533692,-8.89673474290699,
66.386577884774));
#146725=CARTESIAN_POINT('Ctrl Pts',(66.6734667414291,-8.43965165912399,
66.3162259117851));
#146726=CARTESIAN_POINT('Ctrl Pts',(66.2034070026591,-7.85286492552099,
66.349711667394));
#146727=CARTESIAN_POINT('Ctrl Pts',(65.7813830547891,-7.30250012931199,
66.48266933916));
#146728=CARTESIAN_POINT('Ctrl Pts',(65.4063407259891,-6.79057643445299,
66.704345376687));
#146729=CARTESIAN_POINT('Ctrl Pts',(65.0805829419992,-6.32024044517699,
67.019393916489));
#146730=CARTESIAN_POINT('Ctrl Pts',(64.8157501610991,-5.90096700411599,
67.448562171506));
#146731=CARTESIAN_POINT('Ctrl Pts',(64.6458675632491,-5.56625329692299,
68.021190828507));
#146732=CARTESIAN_POINT('Ctrl Pts',(64.6364193785091,-5.42093745532399,
68.624674676515));
#146733=CARTESIAN_POINT('Ctrl Pts',(64.7035612536991,-5.42728709471999,
68.980959567861));
#146734=CARTESIAN_POINT('Ctrl Pts',(64.7336316140092,-5.438853269687,69.098531485314));
#146735=CARTESIAN_POINT('Ctrl Pts',(67.2323151506591,-9.21991446919998,
65.474984814013));
#146736=CARTESIAN_POINT('Ctrl Pts',(67.1376547180191,-9.15157803723199,
65.452503202276));
#146737=CARTESIAN_POINT('Ctrl Pts',(66.7925045216491,-8.896772071233,65.388183277361));
#146738=CARTESIAN_POINT('Ctrl Pts',(66.2208933601991,-8.43968761664299,
65.384755954266));
#146739=CARTESIAN_POINT('Ctrl Pts',(65.5602997427191,-7.85290020560999,
65.541038647212));
#146740=CARTESIAN_POINT('Ctrl Pts',(64.9957046052491,-7.30253572375499,
65.813701215149));
#146741=CARTESIAN_POINT('Ctrl Pts',(64.5153282640591,-6.79061330488699,
66.185306688001));
#146742=CARTESIAN_POINT('Ctrl Pts',(64.1153057006891,-6.32027961129199,
66.657675625535));
#146743=CARTESIAN_POINT('Ctrl Pts',(63.8041484102192,-5.90100948658499,
67.250769932652));
#146744=CARTESIAN_POINT('Ctrl Pts',(63.6155536603191,-5.56629962945499,
67.992076363979));
#146745=CARTESIAN_POINT('Ctrl Pts',(63.6141400609291,-5.42098587722199,
68.740690180875));
#146746=CARTESIAN_POINT('Ctrl Pts',(63.6966701364891,-5.42733541303799,
69.180437561794));
#146747=CARTESIAN_POINT('Ctrl Pts',(63.7331157142191,-5.43890142555399,
69.32606171939));
#146748=CARTESIAN_POINT('Ctrl Pts',(65.6628221245791,-7.69741879281999,
66.179958572744));
#146749=CARTESIAN_POINT('Ctrl Pts',(65.880635783277,-7.95491253744867,66.079322299056));
#146750=CARTESIAN_POINT('Ctrl Pts',(66.098391668443,-8.20085114340354,65.9933372157089));
#146751=CARTESIAN_POINT('Ctrl Pts',(66.5559400877547,-8.66510116739808,
65.8421362758434));
#146752=CARTESIAN_POINT('Ctrl Pts',(66.7955834923,-8.88331642583493,65.7770795900716));
#146753=CARTESIAN_POINT('Ctrl Pts',(67.0545019147991,-9.08849701138999,
65.731481543268));
#146754=CARTESIAN_POINT('Ctrl Pts',(66.3719249731476,-10.2467348134123,
67.0703693338527));
#146755=CARTESIAN_POINT('Ctrl Pts',(66.3587699159923,-10.2258771100607,
67.0726860040253));
#146756=CARTESIAN_POINT('Ctrl Pts',(66.3456963439005,-10.204931303275,67.0751687775537));
#146757=CARTESIAN_POINT('Ctrl Pts',(66.3327087066816,-10.1839044520611,
67.0778129159232));
#146758=CARTESIAN_POINT('Ctrl Pts',(66.2013322819353,-9.97120737024384,
67.1045596936215));
#146759=CARTESIAN_POINT('Ctrl Pts',(66.0787482680444,-9.75021642292389,
67.1478203956863));
#146760=CARTESIAN_POINT('Ctrl Pts',(65.9657693900773,-9.52542421822077,
67.2039202363711));
#146761=CARTESIAN_POINT('Ctrl Pts',(65.9267523303586,-9.44779261988124,
67.2232942191331));
#146762=CARTESIAN_POINT('Ctrl Pts',(65.8888808777626,-9.36970777215893,
67.2441991958904));
#146763=CARTESIAN_POINT('Ctrl Pts',(65.8521738661728,-9.29135080903652,
67.2665615746551));
#146764=CARTESIAN_POINT('Ctrl Pts',(65.795534694387,-9.17044547507714,67.3010668791606));
#146765=CARTESIAN_POINT('Ctrl Pts',(65.7416673787108,-9.04889180086284,
67.3390422948992));
#146766=CARTESIAN_POINT('Ctrl Pts',(65.6906372195148,-8.92735669390233,
67.3802192562758));
#146767=CARTESIAN_POINT('Ctrl Pts',(65.615348862804,-8.74804746520514,67.4409705023081));
#146768=CARTESIAN_POINT('Ctrl Pts',(65.5462361893532,-8.56877865507418,
67.5086905980588));
#146769=CARTESIAN_POINT('Ctrl Pts',(65.4836031430187,-8.39215335319471,
67.5833304387398));
#146770=CARTESIAN_POINT('Ctrl Pts',(65.4273219721058,-8.23344035128313,
67.6504007454888));
#146771=CARTESIAN_POINT('Ctrl Pts',(65.3762728187147,-8.07686186894069,
67.7230584414322));
#146772=CARTESIAN_POINT('Ctrl Pts',(65.3310788970486,-7.925489868639,67.8019493212137));
#146773=CARTESIAN_POINT('Ctrl Pts',(65.290241741339,-7.78871037001386,67.8732349946612));
#146774=CARTESIAN_POINT('Ctrl Pts',(65.2541853212793,-7.65618191234247,
67.9496099938284));
#146775=CARTESIAN_POINT('Ctrl Pts',(65.2240011710327,-7.53224655616877,
68.0320923495727));
#146776=CARTESIAN_POINT('Ctrl Pts',(65.196700477153,-7.42015059878312,68.1066952628982));
#146777=CARTESIAN_POINT('Ctrl Pts',(65.1742036921384,-7.315084379016,68.1862944018207));
#146778=CARTESIAN_POINT('Ctrl Pts',(65.1582250830977,-7.2235599576371,68.271795733124));
#146779=CARTESIAN_POINT('Ctrl Pts',(65.1480055899892,-7.16502337343489,
68.3264801092046));
#146780=CARTESIAN_POINT('Ctrl Pts',(65.140452382556,-7.11202611388141,68.3835788078871));
#146781=CARTESIAN_POINT('Ctrl Pts',(65.1363083340697,-7.0676644135367,68.4428285860919));
#146782=CARTESIAN_POINT('Ctrl Pts',(65.1345887505014,-7.0492564119832,68.4674144338111));
#146783=CARTESIAN_POINT('Ctrl Pts',(65.1334561730655,-7.03233529570783,
68.4923707145794));
#146784=CARTESIAN_POINT('Ctrl Pts',(65.1329636891759,-7.01712232415006,
68.5176785935998));
#146785=CARTESIAN_POINT('Ctrl Pts',(65.1314613787278,-6.9707155145032,68.5948796795156));
#146786=CARTESIAN_POINT('Ctrl Pts',(65.1359154341253,-6.94020380920389,
68.6753525626475));
#146787=CARTESIAN_POINT('Ctrl Pts',(65.1471893670695,-6.93113776553883,
68.7557374140826));
#146788=CARTESIAN_POINT('Ctrl Pts',(65.1496362012979,-6.92917011981428,
68.7731837131618));
#146789=CARTESIAN_POINT('Ctrl Pts',(65.1524042774959,-6.92821264454784,
68.7906258645289));
#146790=CARTESIAN_POINT('Ctrl Pts',(65.1554789178604,-6.92824180418985,
68.8080164594658));
#146791=CARTESIAN_POINT('Ctrl Pts',(65.0995290409545,-6.72702913922128,
68.2204986910971));
#146792=CARTESIAN_POINT('Ctrl Pts',(65.0988514463376,-6.72473836951761,
68.2093410230739));
#146793=CARTESIAN_POINT('Ctrl Pts',(65.0981431109678,-6.72240545263861,
68.1975201313493));
#146794=CARTESIAN_POINT('Ctrl Pts',(65.0974068849537,-6.72006496510622,
68.185017239628));
#146795=CARTESIAN_POINT('Ctrl Pts',(65.095956155403,-6.71545304653674,68.1603803561993));
#146796=CARTESIAN_POINT('Ctrl Pts',(65.0943969051797,-6.71080899338494,
68.1330953877451));
#146797=CARTESIAN_POINT('Ctrl Pts',(65.0927528773071,-6.70642531220498,
68.1030094464778));
#146798=CARTESIAN_POINT('Ctrl Pts',(65.092564261298,-6.70592238128561,68.099557746986));
#146799=CARTESIAN_POINT('Ctrl Pts',(65.0923745342892,-6.70542293357853,
68.0960691845815));
#146800=CARTESIAN_POINT('Ctrl Pts',(65.0921837359439,-6.70492745545278,
68.0925435338524));
#146801=CARTESIAN_POINT('Ctrl Pts',(65.0905324080161,-6.70063917472585,
68.0620296134879));
#146802=CARTESIAN_POINT('Ctrl Pts',(65.0888002238557,-6.6966448016099,68.0287347627108));
#146803=CARTESIAN_POINT('Ctrl Pts',(65.0870164722665,-6.69326342402229,
67.992527598533));
#146804=CARTESIAN_POINT('Ctrl Pts',(65.0858004314016,-6.69095823009796,
67.967844009458));
#146805=CARTESIAN_POINT('Ctrl Pts',(65.0845601918433,-6.68893784615693,
67.9418052937458));
#146806=CARTESIAN_POINT('Ctrl Pts',(65.0833114663123,-6.68733036335121,
67.914406116581));
#146807=CARTESIAN_POINT('Ctrl Pts',(65.0828758257721,-6.68676956383172,
67.9048474168961));
#146808=CARTESIAN_POINT('Ctrl Pts',(65.0824392146896,-6.68625922884587,
67.8951235016651));
#146809=CARTESIAN_POINT('Ctrl Pts',(65.0820025323917,-6.68580556870411,
67.8852355166209));
#146810=CARTESIAN_POINT('Ctrl Pts',(65.0812623939487,-6.68503665429501,
67.8684762435933));
#146811=CARTESIAN_POINT('Ctrl Pts',(65.0805220832648,-6.68443058742722,
67.8512457977658));
#146812=CARTESIAN_POINT('Ctrl Pts',(65.0797840166927,-6.68401364421596,
67.833538954931));
#146813=CARTESIAN_POINT('Ctrl Pts',(65.0789318710392,-6.68353225627798,
67.8130952582115));
#146814=CARTESIAN_POINT('Ctrl Pts',(65.0780775318777,-6.68329142394815,
67.7920156087582));
#146815=CARTESIAN_POINT('Ctrl Pts',(65.0772270244056,-6.68333895508708,
67.7703021843689));
#146816=CARTESIAN_POINT('Ctrl Pts',(65.0756899091387,-6.68342485772956,
67.7310596883076));
#146817=CARTESIAN_POINT('Ctrl Pts',(65.0741648682245,-6.68445235162658,
67.6897441658871));
#146818=CARTESIAN_POINT('Ctrl Pts',(65.0726921564383,-6.68669839222721,
67.6463985424324));
#146819=CARTESIAN_POINT('Ctrl Pts',(65.0712383938668,-6.6889155332793,67.6036106421764));
#146820=CARTESIAN_POINT('Ctrl Pts',(65.0698366208069,-6.69232153309281,
67.558849859444));
#146821=CARTESIAN_POINT('Ctrl Pts',(65.0685138680218,-6.69715122989116,
67.5121000321052));
#146822=CARTESIAN_POINT('Ctrl Pts',(65.0673678998273,-6.70133544252872,
67.4715982725699));
#146823=CARTESIAN_POINT('Ctrl Pts',(65.0662802825402,-6.70658810797603,
67.4295981517366));
#146824=CARTESIAN_POINT('Ctrl Pts',(65.0652803514322,-6.71304062012262,
67.3861644948326));
#146825=CARTESIAN_POINT('Ctrl Pts',(65.0651262182528,-6.71403523485581,
67.3794694659676));
#146826=CARTESIAN_POINT('Ctrl Pts',(65.0649741827216,-6.71505834890559,
67.3727404754684));
#146827=CARTESIAN_POINT('Ctrl Pts',(65.0648243687283,-6.71611043536287,
67.3659778759423));
#146828=CARTESIAN_POINT('Ctrl Pts',(65.0640048900083,-6.72186532143319,
67.3289866291271));
#146829=CARTESIAN_POINT('Ctrl Pts',(65.0632512908526,-6.7284869270308,67.2909859159469));
#146830=CARTESIAN_POINT('Ctrl Pts',(65.0625891014791,-6.73607132014469,
67.2520668980457));
#146831=CARTESIAN_POINT('Ctrl Pts',(65.0623372359469,-6.73895606472791,
67.237263943559));
#146832=CARTESIAN_POINT('Ctrl Pts',(65.062098671377,-6.74198011486308,67.2223286428493));
#146833=CARTESIAN_POINT('Ctrl Pts',(65.0618751224679,-6.74514886085747,
67.2072680328656));
#146834=CARTESIAN_POINT('Ctrl Pts',(65.0617277540022,-6.7472377694431,67.1973397402365));
#146835=CARTESIAN_POINT('Ctrl Pts',(65.0615869183904,-6.74938956300479,
67.1873570366761));
#146836=CARTESIAN_POINT('Ctrl Pts',(65.0614528323817,-6.75160559577343,
67.1773204194393));
#146837=CARTESIAN_POINT('Ctrl Pts',(65.2414845310557,-7.08609081947666,
68.1857750435771));
#146838=CARTESIAN_POINT('Ctrl Pts',(65.2409930225825,-7.08307946957817,
68.1829875467368));
#146839=CARTESIAN_POINT('Ctrl Pts',(65.2390270370096,-7.07130660341053,
68.1718378108095));
#146840=CARTESIAN_POINT('Ctrl Pts',(65.2350498086539,-7.04943590107549,
68.149281891156));
#146841=CARTESIAN_POINT('Ctrl Pts',(65.2289662965972,-7.01998916036024,
68.1147805561278));
#146842=CARTESIAN_POINT('Ctrl Pts',(65.2215006476313,-6.98832976483916,
68.0724407641344));
#146843=CARTESIAN_POINT('Ctrl Pts',(65.2124609423225,-6.95501062438879,
68.0211740455227));
#146844=CARTESIAN_POINT('Ctrl Pts',(65.2016910752082,-6.92085388141908,
67.9600950946355));
#146845=CARTESIAN_POINT('Ctrl Pts',(65.1890769486371,-6.88686554625872,
67.8885568277298));
#146846=CARTESIAN_POINT('Ctrl Pts',(65.174545294336,-6.85408467185527,67.8061437209722));
#146847=CARTESIAN_POINT('Ctrl Pts',(65.158112543083,-6.8238577244596,67.7129489575022));
#146848=CARTESIAN_POINT('Ctrl Pts',(65.1395177520264,-6.79716341683066,
67.6074926570354));
#146849=CARTESIAN_POINT('Ctrl Pts',(65.1184916003832,-6.77532627398624,
67.4882474255094));
#146850=CARTESIAN_POINT('Ctrl Pts',(65.0946850953443,-6.75993711427478,
67.3532340262738));
#146851=CARTESIAN_POINT('Ctrl Pts',(65.0754454868457,-6.75486817113625,
67.2441207843846));
#146852=CARTESIAN_POINT('Ctrl Pts',(65.0642368910678,-6.75456867256639,
67.1805536789273));
#146853=CARTESIAN_POINT('Ctrl Pts',(65.061993565123,-6.75461306050176,67.1678311452813));
#146854=CARTESIAN_POINT('Ctrl Pts',(65.1897746446634,-7.02642538409721,
68.2593549473257));
#146855=CARTESIAN_POINT('Ctrl Pts',(65.1892024303291,-7.02291951297361,
68.2561097468352));
#146856=CARTESIAN_POINT('Ctrl Pts',(65.1869252802611,-7.00928483992008,
68.2431953208314));
#146857=CARTESIAN_POINT('Ctrl Pts',(65.1823929989191,-6.98437727076367,
68.2174915299371));
#146858=CARTESIAN_POINT('Ctrl Pts',(65.1755690707742,-6.95136155253651,
68.1787910901047));
#146859=CARTESIAN_POINT('Ctrl Pts',(65.1673123831504,-6.91636344682656,
68.1319650938863));
#146860=CARTESIAN_POINT('Ctrl Pts',(65.1574350184448,-6.87997139936304,
68.0759477730928));
#146861=CARTESIAN_POINT('Ctrl Pts',(65.1457914940052,-6.84305859113378,
68.0099140652061));
#146862=CARTESIAN_POINT('Ctrl Pts',(65.1322865151918,-6.80668404378828,
67.9333235241955));
#146863=CARTESIAN_POINT('Ctrl Pts',(65.1168576306764,-6.77189004270382,
67.845821972033));
#146864=CARTESIAN_POINT('Ctrl Pts',(65.0994927393792,-6.73995596016165,
67.7473407796801));
#146865=CARTESIAN_POINT('Ctrl Pts',(65.0799361853932,-6.71188987072493,
67.636430050595));
#146866=CARTESIAN_POINT('Ctrl Pts',(65.0579186559581,-6.68903360033692,
67.5115624362205));
#146867=CARTESIAN_POINT('Ctrl Pts',(65.0331151814423,-6.67301084343169,
67.370894942116));
#146868=CARTESIAN_POINT('Ctrl Pts',(65.013150050025,-6.66775695913348,67.2576670552906));
#146869=CARTESIAN_POINT('Ctrl Pts',(65.0015330056641,-6.66744694909317,
67.1917835228098));
#146870=CARTESIAN_POINT('Ctrl Pts',(64.9992085127703,-6.66749296220202,
67.1786006685223));
#146871=CARTESIAN_POINT('Ctrl Pts',(65.1535738069259,-6.96027158061405,
68.3372101679681));
#146872=CARTESIAN_POINT('Ctrl Pts',(65.1529121103036,-6.95621741113752,
68.3334574904581));
#146873=CARTESIAN_POINT('Ctrl Pts',(65.1502899578951,-6.94051846743772,
68.3185864716667));
#146874=CARTESIAN_POINT('Ctrl Pts',(65.1451422638615,-6.91224378481554,
68.2893924916179));
#146875=CARTESIAN_POINT('Ctrl Pts',(65.1374974024557,-6.87527097760616,
68.2460363117872));
#146876=CARTESIAN_POINT('Ctrl Pts',(65.1283636540082,-6.83657109085138,
68.1942362552807));
#146877=CARTESIAN_POINT('Ctrl Pts',(65.1175575379276,-6.79677197050921,
68.1329517240636));
#146878=CARTESIAN_POINT('Ctrl Pts',(65.1049453495612,-6.75680338637883,
68.0614244499476));
#146879=CARTESIAN_POINT('Ctrl Pts',(65.0904526420255,-6.71778313619111,
67.9792322210226));
#146880=CARTESIAN_POINT('Ctrl Pts',(65.0740289572397,-6.68075708926638,
67.886088876167));
#146881=CARTESIAN_POINT('Ctrl Pts',(65.055630559543,-6.64693022772616,67.7817463777627));
#146882=CARTESIAN_POINT('Ctrl Pts',(65.0350076549065,-6.61734318091172,
67.6647880736179));
#146883=CARTESIAN_POINT('Ctrl Pts',(65.011890939465,-6.59335695709566,67.533686665629));
#146884=CARTESIAN_POINT('Ctrl Pts',(64.9859820791854,-6.5766317019353,67.3867502173394));
#146885=CARTESIAN_POINT('Ctrl Pts',(64.9652125272479,-6.57117276489505,
67.268960235043));
#146886=CARTESIAN_POINT('Ctrl Pts',(64.9531426172181,-6.57085110030559,
67.2005083737279));
#146887=CARTESIAN_POINT('Ctrl Pts',(64.9507281308072,-6.57089891531876,
67.1868151408426));
#146888=CARTESIAN_POINT('Ctrl Pts',(65.1342438570207,-6.88922545630012,
68.4173762199009));
#146889=CARTESIAN_POINT('Ctrl Pts',(65.133486060561,-6.88458243975978,68.4130785355508));
#146890=CARTESIAN_POINT('Ctrl Pts',(65.1304933916005,-6.86666656489,68.3961062266279));
#146891=CARTESIAN_POINT('Ctrl Pts',(65.1246847728085,-6.83477575818617,
68.3631639449019));
#146892=CARTESIAN_POINT('Ctrl Pts',(65.1161582670608,-6.79355322048586,
68.3148077157122));
#146893=CARTESIAN_POINT('Ctrl Pts',(65.1060825958666,-6.75087779215306,
68.2576657485828));
#146894=CARTESIAN_POINT('Ctrl Pts',(65.0942790437781,-6.70741963316853,
68.1907244770599));
#146895=CARTESIAN_POINT('Ctrl Pts',(65.0806265551699,-6.66416928709678,
68.1132973669754));
#146896=CARTESIAN_POINT('Ctrl Pts',(65.0650730726838,-6.62230767446081,
68.0250891843942));
#146897=CARTESIAN_POINT('Ctrl Pts',(65.0475810184328,-6.58288451356995,
67.9258868152054));
#146898=CARTESIAN_POINT('Ctrl Pts',(65.0280726826782,-6.5470248949559,67.8152495452771));
#146899=CARTESIAN_POINT('Ctrl Pts',(65.0063045667778,-6.51580441028536,
67.6917964253113));
#146900=CARTESIAN_POINT('Ctrl Pts',(64.9820073764202,-6.49060466876522,
67.5540002113891));
#146901=CARTESIAN_POINT('Ctrl Pts',(64.9549113829709,-6.47312496298017,
67.4003311963398));
#146902=CARTESIAN_POINT('Ctrl Pts',(64.9332779206116,-6.46744580878183,
67.2776417345743));
#146903=CARTESIAN_POINT('Ctrl Pts',(64.9207216538056,-6.46711162774576,
67.2064316069159));
#146904=CARTESIAN_POINT('Ctrl Pts',(64.9182105185209,-6.46716137792081,
67.1921902510292));
#146905=CARTESIAN_POINT('Origin',(66.6326669169691,-15.387431115,68.54751529846));
#146906=CARTESIAN_POINT('',(66.3723475853491,-13.10500468188,67.070279796935));
#146907=CARTESIAN_POINT('Origin',(64.8949830209491,111.0724296188,67.330775935442));
#146908=CARTESIAN_POINT('',(83.1139264516123,-13.1050132065526,64.118284648618));
#146909=CARTESIAN_POINT('',(83.1139264526491,-9.38083151849399,64.118284648434));
#146910=CARTESIAN_POINT('',(83.1139264515391,-13.10501209623,64.118284648628));
#146911=CARTESIAN_POINT('Origin',(64.8949830209491,111.0724296188,67.330775935442));
#146912=CARTESIAN_POINT('',(66.37195527291,10.2467337056388,67.0703617289055));
#146913=CARTESIAN_POINT('',(66.372346455996,13.1050047578536,67.0702791546134));
#146914=CARTESIAN_POINT('',(66.3720475457991,10.24677906507,67.0703345259));
#146915=CARTESIAN_POINT('',(83.1139264516833,13.1050084134076,64.1182846486046));
#146916=CARTESIAN_POINT('',(66.3723465844291,13.10500475785,67.070279883));
#146917=CARTESIAN_POINT('',(83.1139264516891,13.10501209624,64.118284648603));
#146918=CARTESIAN_POINT('Origin',(74.2506566745691,1.4210854715202E-14,
65.681118247606));
#146919=CARTESIAN_POINT('Origin',(83.3948788947791,-13.10501209624,62.54560523476));
#146920=CARTESIAN_POINT('Origin',(82.8534541851791,-13.10501209624,62.64107301909));
#146921=CARTESIAN_POINT('Origin',(82.8534541851791,-13.10501209624,62.64107301909));
#146922=CARTESIAN_POINT('Origin',(82.8534541851791,-13.10501431796,62.64107301909));
#146923=CARTESIAN_POINT('Origin',(82.8534541851791,-13.10501209624,62.64107301909));
#146924=CARTESIAN_POINT('Origin',(83.1537660643691,-9.5,64.344226319777));
#146925=CARTESIAN_POINT('Ctrl Pts',(82.3363233957455,-12.343665452965,59.7087760102195));
#146926=CARTESIAN_POINT('Ctrl Pts',(82.5103580067827,-12.3443368485801,
59.6774248403774));
#146927=CARTESIAN_POINT('Ctrl Pts',(82.7030337161479,-12.3276047655723,
59.6714205660576));
#146928=CARTESIAN_POINT('Ctrl Pts',(83.0885922050506,-12.2518831267182,
59.7305332382176));
#146929=CARTESIAN_POINT('Ctrl Pts',(83.2804190043815,-12.1926335983454,
59.7962739132679));
#146930=CARTESIAN_POINT('Ctrl Pts',(83.6124903709299,-12.0410881150009,
59.9924860734914));
#146931=CARTESIAN_POINT('Ctrl Pts',(83.7516096696434,-11.9493050886816,
60.1222919943206));
#146932=CARTESIAN_POINT('Ctrl Pts',(83.9504113602448,-11.7582926728204,
60.4084317135998));
#146933=CARTESIAN_POINT('Ctrl Pts',(84.0104131841654,-11.6596554556486,
60.563712095989));
#146934=CARTESIAN_POINT('Ctrl Pts',(84.0366050016191,-11.56837406741,60.71288355042));
#146935=CARTESIAN_POINT('Ctrl Pts',(82.0553296437291,-10.06961035349,58.06788670299));
#146936=CARTESIAN_POINT('Ctrl Pts',(82.0508297110692,-10.32189652016,58.28772795841));
#146937=CARTESIAN_POINT('Ctrl Pts',(82.044185238899,-10.85545409583,58.73637934571));
#146938=CARTESIAN_POINT('Ctrl Pts',(82.0434349722091,-11.65068683102,59.33916327135));
#146939=CARTESIAN_POINT('Ctrl Pts',(82.0448098099991,-12.20048376736,59.70692633614));
#146940=CARTESIAN_POINT('Ctrl Pts',(82.0452134587591,-12.45553486127,59.86597852961));
#146941=CARTESIAN_POINT('Ctrl Pts',(83.2289392944191,-10.06541382727,57.8659223213401));
#146942=CARTESIAN_POINT('Ctrl Pts',(83.2201513675491,-10.3397788344,58.06049300364));
#146943=CARTESIAN_POINT('Ctrl Pts',(83.2017243183791,-10.91461113645,58.45747334811));
#146944=CARTESIAN_POINT('Ctrl Pts',(83.1784930097592,-11.75261430238,58.9905418745401));
#146945=CARTESIAN_POINT('Ctrl Pts',(83.1625683469792,-12.32074716019,59.313379833));
#146946=CARTESIAN_POINT('Ctrl Pts',(83.1546752474691,-12.58190616187,59.45208388284));
#146947=CARTESIAN_POINT('Ctrl Pts',(84.0014320878491,-9.416662390436,58.49880899002));
#146948=CARTESIAN_POINT('Ctrl Pts',(84.0197603423191,-9.71427756945499,
58.68408877132));
#146949=CARTESIAN_POINT('Ctrl Pts',(84.0535870702291,-10.3409287432,59.06357280994));
#146950=CARTESIAN_POINT('Ctrl Pts',(84.0914425043691,-11.25380191593,59.57276536302));
#146951=CARTESIAN_POINT('Ctrl Pts',(84.1097895903591,-11.87370493252,59.88080283618));
#146952=CARTESIAN_POINT('Ctrl Pts',(84.1164333695691,-12.1590724314,60.01281199009));
#146953=CARTESIAN_POINT('Ctrl Pts',(83.6792160484492,-8.70584534846799,
59.39830177706));
#146954=CARTESIAN_POINT('Ctrl Pts',(83.7317180692091,-9.00700658342599,
59.59861227705));
#146955=CARTESIAN_POINT('Ctrl Pts',(83.834918244039,-9.64949457496699,60.01048401614));
#146956=CARTESIAN_POINT('Ctrl Pts',(83.9625807365691,-10.60211439156,60.56307735249));
#146957=CARTESIAN_POINT('Ctrl Pts',(84.0359995174791,-11.26073934252,60.8997277557));
#146958=CARTESIAN_POINT('Ctrl Pts',(84.0669616904391,-11.5666800367,61.04470635445));
#146959=CARTESIAN_POINT('',(82.3525647217089,-10.1664213136743,58.1365952838437));
#146960=CARTESIAN_POINT('Ctrl Pts',(82.3525700953787,-10.166478497124,58.1365255250151));
#146961=CARTESIAN_POINT('Ctrl Pts',(82.3951531597494,-10.1611675921044,
58.135452276721));
#146962=CARTESIAN_POINT('Ctrl Pts',(82.4382846388827,-10.1545975757461,
58.1357792398753));
#146963=CARTESIAN_POINT('Ctrl Pts',(82.4817296150921,-10.1467003204195,
58.1376346901912));
#146964=CARTESIAN_POINT('Ctrl Pts',(82.5246216655268,-10.1389035737455,
58.1394665261243));
#146965=CARTESIAN_POINT('Ctrl Pts',(82.5678188296875,-10.1298128164637,
58.1427886782012));
#146966=CARTESIAN_POINT('Ctrl Pts',(82.6110610457748,-10.1193888719939,
58.147698859281));
#146967=CARTESIAN_POINT('Ctrl Pts',(82.6536135361689,-10.1091311924147,
58.1525307215707));
#146968=CARTESIAN_POINT('Ctrl Pts',(82.6962090421351,-10.0975822925618,
58.158900732393));
#146969=CARTESIAN_POINT('Ctrl Pts',(82.7385745301759,-10.0847346980979,
58.1668705743677));
#146970=CARTESIAN_POINT('Ctrl Pts',(82.770926444484,-10.0749237813735,58.172956651893));
#146971=CARTESIAN_POINT('Ctrl Pts',(82.8031436173484,-10.0643561291815,
58.1799750588118));
#146972=CARTESIAN_POINT('Ctrl Pts',(82.8350979729569,-10.0530414423116,
58.1879387605769));
#146973=CARTESIAN_POINT('Ctrl Pts',(82.8762053001496,-10.0384857885866,
58.1981835765931));
#146974=CARTESIAN_POINT('Ctrl Pts',(82.9168777867966,-10.0226925608224,
58.2099942907058));
#146975=CARTESIAN_POINT('Ctrl Pts',(82.9568372896724,-10.0057091209681,
58.2233628773243));
#146976=CARTESIAN_POINT('Ctrl Pts',(82.9965729684327,-9.98882081001011,
58.2366565828292));
#146977=CARTESIAN_POINT('Ctrl Pts',(83.0356028553504,-9.97075565883965,
58.2514908027958));
#146978=CARTESIAN_POINT('Ctrl Pts',(83.0736579528351,-9.95159249143506,
58.2678180795554));
#146979=CARTESIAN_POINT('Ctrl Pts',(83.1115465711695,-9.93251315689487,
58.2840739295853));
#146980=CARTESIAN_POINT('Ctrl Pts',(83.1484681595522,-9.912345594257,58.301809691031));
#146981=CARTESIAN_POINT('Ctrl Pts',(83.1841731300037,-9.89119758550829,
58.3209396729932));
#146982=CARTESIAN_POINT('Ctrl Pts',(83.2163800673443,-9.87212145733807,
58.3381954814308));
#146983=CARTESIAN_POINT('Ctrl Pts',(83.2475969420267,-9.85224812681749,
58.3565850795893));
#146984=CARTESIAN_POINT('Ctrl Pts',(83.2776590840935,-9.83167513719697,
58.3760201451493));
#146985=CARTESIAN_POINT('Ctrl Pts',(83.3109913998323,-9.80886420828183,
58.3975693661001));
#146986=CARTESIAN_POINT('Ctrl Pts',(83.3429030393085,-9.78519311877206,
58.4204040341745));
#146987=CARTESIAN_POINT('Ctrl Pts',(83.3732035467558,-9.7608150923811,58.4443733288806));
#146988=CARTESIAN_POINT('Ctrl Pts',(83.40356420074,-9.73638867558394,58.4683902026601));
#146989=CARTESIAN_POINT('Ctrl Pts',(83.4323068914428,-9.71125298127848,
58.4935457242152));
#146990=CARTESIAN_POINT('Ctrl Pts',(83.4592833428956,-9.68557718695221,
58.5196624506196));
#146991=CARTESIAN_POINT('Ctrl Pts',(83.4864770128165,-9.65969464724576,
58.5459894728559));
#146992=CARTESIAN_POINT('Ctrl Pts',(83.5118756015812,-9.63326378255559,
58.5732926811178));
#146993=CARTESIAN_POINT('Ctrl Pts',(83.5353766794126,-9.60646576177959,
58.6013721221683));
#146994=CARTESIAN_POINT('Ctrl Pts',(83.5564064501732,-9.58248574529688,
58.626498808383));
#146995=CARTESIAN_POINT('Ctrl Pts',(83.5759174780459,-9.558212083325,58.6522465149794));
#146996=CARTESIAN_POINT('Ctrl Pts',(83.5938712055915,-9.53377483715701,
58.6784655241524));
#146997=CARTESIAN_POINT('Ctrl Pts',(83.6143253646157,-9.5059341941504,58.7083360778702));
#146998=CARTESIAN_POINT('Ctrl Pts',(83.6327573590749,-9.47788182466822,
58.738817802516));
#146999=CARTESIAN_POINT('Ctrl Pts',(83.6491609908517,-9.4498040488955,58.7696891456885));
#147000=CARTESIAN_POINT('Ctrl Pts',(83.6657208741947,-9.42145882037187,
58.800854551529));
#147001=CARTESIAN_POINT('Ctrl Pts',(83.6802138906995,-9.39308814599666,
58.8324164399566));
#147002=CARTESIAN_POINT('Ctrl Pts',(83.6926849067531,-9.36486944317266,
58.8641550268704));
#147003=CARTESIAN_POINT('Ctrl Pts',(83.7053978734835,-9.33610326817695,
58.8965093753666));
#147004=CARTESIAN_POINT('Ctrl Pts',(83.716010056729,-9.3074954147027,58.9290467923253));
#147005=CARTESIAN_POINT('Ctrl Pts',(83.7246162927773,-9.27921253917801,
58.9615517347137));
#147006=CARTESIAN_POINT('Ctrl Pts',(83.7310073805458,-9.25820935743756,
58.9856902708343));
#147007=CARTESIAN_POINT('Ctrl Pts',(83.7362932957204,-9.23738494648499,
59.0098112489987));
#147008=CARTESIAN_POINT('Ctrl Pts',(83.7405267536393,-9.2167985425004,59.0338347984847));
#147009=CARTESIAN_POINT('Ctrl Pts',(82.3525700823783,-10.1664785168028,
58.1365255401533));
#147010=CARTESIAN_POINT('Ctrl Pts',(82.3488876921889,-10.3859560294258,
58.3162559244322));
#147011=CARTESIAN_POINT('Ctrl Pts',(82.3460217722092,-10.6066582564664,
58.4916352097824));
#147012=CARTESIAN_POINT('Ctrl Pts',(82.3439687240532,-10.829866174788,58.6621421225721));
#147013=CARTESIAN_POINT('Ctrl Pts',(82.3415371907178,-11.0942230981875,
58.8640824624238));
#147014=CARTESIAN_POINT('Ctrl Pts',(82.3402450190165,-11.3620941909475,
59.0591873596057));
#147015=CARTESIAN_POINT('Ctrl Pts',(82.339146797498,-11.6336159214709,59.2457463654941));
#147016=CARTESIAN_POINT('Ctrl Pts',(82.3390437206752,-11.6591003950567,
59.2632564117383));
#147017=CARTESIAN_POINT('Ctrl Pts',(82.3389423585988,-11.6846170092359,
59.2806912063098));
#147018=CARTESIAN_POINT('Ctrl Pts',(82.3388419338635,-11.7101658660261,
59.2980493546135));
#147019=CARTESIAN_POINT('Ctrl Pts',(82.3380197652076,-11.9193321553656,
59.4401590192575));
#147020=CARTESIAN_POINT('Ctrl Pts',(82.3372600244892,-12.130659856514,59.5771301339812));
#147021=CARTESIAN_POINT('Ctrl Pts',(82.3361472036304,-12.3441228986193,
59.7080238558997));
#147022=CARTESIAN_POINT('Ctrl Pts',(62.3774191338491,-11.93682814514,62.997303880638));
#147023=CARTESIAN_POINT('Ctrl Pts',(62.8594167896691,-11.31836793413,62.63949114694));
#147024=CARTESIAN_POINT('Ctrl Pts',(63.7016296262191,-10.28886737917,61.77926831279));
#147025=CARTESIAN_POINT('Ctrl Pts',(64.4353443697491,-9.50098361185099,
60.52921910213));
#147026=CARTESIAN_POINT('Ctrl Pts',(64.7094707273291,-9.22984173748599,
59.95551214223));
#147027=CARTESIAN_POINT('Ctrl Pts',(63.2468805636391,-12.17561401984,62.96400152021));
#147028=CARTESIAN_POINT('Ctrl Pts',(63.6737193233791,-11.57121353012,62.58432057163));
#147029=CARTESIAN_POINT('Ctrl Pts',(64.4147249566291,-10.57536035644,61.70772610609));
#147030=CARTESIAN_POINT('Ctrl Pts',(65.0622360532691,-9.81899150863899,
60.48721794767));
#147031=CARTESIAN_POINT('Ctrl Pts',(65.3060138057191,-9.55843720322299,
59.93191843234));
#147032=CARTESIAN_POINT('Ctrl Pts',(64.9762859395291,-12.57208772501,62.89914697212));
#147033=CARTESIAN_POINT('Ctrl Pts',(65.3033337930391,-12.00439019394,62.48973876938));
#147034=CARTESIAN_POINT('Ctrl Pts',(65.8640127693391,-11.0832288162,61.60122473724));
#147035=CARTESIAN_POINT('Ctrl Pts',(66.3552140056091,-10.38653655991,60.44446305748));
#147036=CARTESIAN_POINT('Ctrl Pts',(66.5422504654091,-10.14466666957,59.92552707855));
#147037=CARTESIAN_POINT('Ctrl Pts',(67.2900608069791,-12.92642311826,62.76588968559));
#147038=CARTESIAN_POINT('Ctrl Pts',(67.5005502484191,-12.40978705063,62.34387880989));
#147039=CARTESIAN_POINT('Ctrl Pts',(67.8553038215491,-11.57897812252,61.47239442111));
#147040=CARTESIAN_POINT('Ctrl Pts',(68.1616279566091,-10.94422799439,60.39769057588));
#147041=CARTESIAN_POINT('Ctrl Pts',(68.2781957858191,-10.72029903218,59.92119556699));
#147042=CARTESIAN_POINT('Ctrl Pts',(69.1793814374391,-13.12660404221,62.60480660922));
#147043=CARTESIAN_POINT('Ctrl Pts',(69.3025957496291,-12.64231047897,62.18346776903));
#147044=CARTESIAN_POINT('Ctrl Pts',(69.5039001954291,-11.86638416497,61.33529575915));
#147045=CARTESIAN_POINT('Ctrl Pts',(69.6676543241791,-11.26766155885,60.31872861861));
#147046=CARTESIAN_POINT('Ctrl Pts',(69.7281187264291,-11.05395501206,59.87083582562));
#147047=CARTESIAN_POINT('Ctrl Pts',(70.6290331937791,-13.2354548215,62.4487226016));
#147048=CARTESIAN_POINT('Ctrl Pts',(70.6877066225591,-12.77011721816,62.03193358429));
#147049=CARTESIAN_POINT('Ctrl Pts',(70.7757857175191,-12.02562572997,61.20384952745));
#147050=CARTESIAN_POINT('Ctrl Pts',(70.8324235385491,-11.44701084757,60.22578653053));
#147051=CARTESIAN_POINT('Ctrl Pts',(70.8500678830391,-11.23893116136,59.79623434573));
#147052=CARTESIAN_POINT('Ctrl Pts',(72.1029034837291,-13.30219283541,62.25362486817));
#147053=CARTESIAN_POINT('Ctrl Pts',(72.0972809910691,-12.84940037151,61.84484177145));
#147054=CARTESIAN_POINT('Ctrl Pts',(72.0725811599691,-12.12531389286,61.03819560464));
#147055=CARTESIAN_POINT('Ctrl Pts',(72.0209865447691,-11.55943931721,60.09237908051));
#147056=CARTESIAN_POINT('Ctrl Pts',(71.9948866285191,-11.35486963736,59.67756847178));
#147057=CARTESIAN_POINT('Ctrl Pts',(73.5959843581491,-13.32506131179,62.01408346482));
#147058=CARTESIAN_POINT('Ctrl Pts',(73.5261098994091,-12.87698220968,61.61585739229));
#147059=CARTESIAN_POINT('Ctrl Pts',(73.3882074986691,-12.16043554427,60.83032202918));
#147060=CARTESIAN_POINT('Ctrl Pts',(73.2263446677791,-11.59915063933,59.90895273874));
#147061=CARTESIAN_POINT('Ctrl Pts',(73.1553017064691,-11.39582011201,59.50465582683));
#147062=CARTESIAN_POINT('Ctrl Pts',(75.0808070354991,-13.30270992682,61.72903176202));
#147063=CARTESIAN_POINT('Ctrl Pts',(74.9469689190791,-12.85001089683,61.34282758741));
#147064=CARTESIAN_POINT('Ctrl Pts',(74.6955188142491,-12.1260767583,60.57617067235));
#147065=CARTESIAN_POINT('Ctrl Pts',(74.4217256775691,-11.56029813203,59.66963151356));
#147066=CARTESIAN_POINT('Ctrl Pts',(74.3048733948091,-11.3557551519,59.27087592838));
#147067=CARTESIAN_POINT('Ctrl Pts',(76.5328601007591,-13.2364944323,61.40866159641));
#147068=CARTESIAN_POINT('Ctrl Pts',(76.3358699248491,-12.77133451632,61.03688416139));
#147069=CARTESIAN_POINT('Ctrl Pts',(75.9711298326091,-12.02713706143,60.28864044243));
#147070=CARTESIAN_POINT('Ctrl Pts',(75.5846252539191,-11.44871074133,59.388898241));
#147071=CARTESIAN_POINT('Ctrl Pts',(75.4216320368191,-11.24068411792,58.99129878541));
#147072=CARTESIAN_POINT('Ctrl Pts',(77.9498391600291,-13.12798216966,61.05954876707));
#147073=CARTESIAN_POINT('Ctrl Pts',(77.6905880595291,-12.64391742949,60.7055511469));
#147074=CARTESIAN_POINT('Ctrl Pts',(77.2125004260691,-11.86837549639,59.97715614722));
#147075=CARTESIAN_POINT('Ctrl Pts',(76.7121050136191,-11.26990259162,59.07792972341));
#147076=CARTESIAN_POINT('Ctrl Pts',(76.5025735472391,-11.05626656671,58.67777561906));
#147077=CARTESIAN_POINT('Ctrl Pts',(79.7859365961591,-12.92767443376,60.56353474153));
#147078=CARTESIAN_POINT('Ctrl Pts',(79.4441950016891,-12.41122585012,60.23879024504));
#147079=CARTESIAN_POINT('Ctrl Pts',(78.8135085271691,-11.58074421675,59.54101492748));
#147080=CARTESIAN_POINT('Ctrl Pts',(78.1588401911891,-10.94621534765,58.63594665383));
#147081=CARTESIAN_POINT('Ctrl Pts',(77.8866345956591,-10.72235004384,58.22811289685));
#147082=CARTESIAN_POINT('Ctrl Pts',(82.0128595054191,-12.5725402543,59.89542135394));
#147083=CARTESIAN_POINT('Ctrl Pts',(81.5655827020591,-12.0048890977,59.6224962674));
#147084=CARTESIAN_POINT('Ctrl Pts',(80.7349790983591,-11.08381973837,58.97925604537));
#147085=CARTESIAN_POINT('Ctrl Pts',(79.8779241817091,-10.38719737489,58.0602712301));
#147086=CARTESIAN_POINT('Ctrl Pts',(79.5247423704091,-10.14534841056,57.63662074318));
#147087=CARTESIAN_POINT('Ctrl Pts',(83.6613481708691,-12.17565886824,59.36439714515));
#147088=CARTESIAN_POINT('Ctrl Pts',(83.1304065130891,-11.57125651121,59.15359310812));
#147089=CARTESIAN_POINT('Ctrl Pts',(82.1343014018491,-10.57540150418,58.58329052728));
#147090=CARTESIAN_POINT('Ctrl Pts',(81.1084241173391,-9.81903260043799,
57.65784452337));
#147091=CARTESIAN_POINT('Ctrl Pts',(80.6894326096791,-9.55847843356399,
57.21940958338));
#147092=CARTESIAN_POINT('Ctrl Pts',(84.4900685407791,-11.93678967047,59.098228309));
#147093=CARTESIAN_POINT('Ctrl Pts',(83.9147510912491,-11.31832804455,58.92685361738));
#147094=CARTESIAN_POINT('Ctrl Pts',(82.8290997230891,-10.28882373832,58.4065707627));
#147095=CARTESIAN_POINT('Ctrl Pts',(81.7120752713391,-9.50093629271799,
57.48285528109));
#147096=CARTESIAN_POINT('Ctrl Pts',(81.2582553288491,-9.22979318182899,
57.03750320808));
#147097=CARTESIAN_POINT('',(64.4192382040804,-9.75938259365387,60.7790388614543));
#147098=CARTESIAN_POINT('Ctrl Pts',(62.670809092837,-11.8749841815823,62.918604792603));
#147099=CARTESIAN_POINT('Ctrl Pts',(62.8226759631422,-11.6771183294842,
62.7956341012768));
#147100=CARTESIAN_POINT('Ctrl Pts',(62.9747638129586,-11.4821292443563,
62.6583787294019));
#147101=CARTESIAN_POINT('Ctrl Pts',(63.1257819325367,-11.2918678559167,
62.5071312698821));
#147102=CARTESIAN_POINT('Ctrl Pts',(63.2686085750815,-11.1119265654766,
62.3640877271803));
#147103=CARTESIAN_POINT('Ctrl Pts',(63.4104791030648,-10.9362130860917,
62.2085281972315));
#147104=CARTESIAN_POINT('Ctrl Pts',(63.5502962427671,-10.7663115879761,
62.0406536860054));
#147105=CARTESIAN_POINT('Ctrl Pts',(63.5583151170356,-10.7565672980105,
62.031025648976));
#147106=CARTESIAN_POINT('Ctrl Pts',(63.56632723384,-10.7468421329298,62.0213570921456));
#147107=CARTESIAN_POINT('Ctrl Pts',(63.5743323848798,-10.7371363944787,
62.0116480491215));
#147108=CARTESIAN_POINT('Ctrl Pts',(63.7064941004239,-10.576898687788,61.8513557853052));
#147109=CARTESIAN_POINT('Ctrl Pts',(63.8366793388084,-10.4220504821042,
61.6801213857542));
#147110=CARTESIAN_POINT('Ctrl Pts',(63.9638878042343,-10.274013906201,61.4982248136155));
#147111=CARTESIAN_POINT('Ctrl Pts',(64.1207829204576,-10.091430021521,61.2738790223918));
#147112=CARTESIAN_POINT('Ctrl Pts',(64.2731491329682,-9.91920894240649,
61.0333138935713));
#147113=CARTESIAN_POINT('Ctrl Pts',(64.4192367794444,-9.75938555497426,
60.7790363314927));
#147114=CARTESIAN_POINT('',(81.8125095647161,-9.7594394284026,57.7121067929141));
#147115=CARTESIAN_POINT('Origin',(81.9839346339093,-12.2832340267788,54.5148848282765));
#147116=CARTESIAN_POINT('Ctrl Pts',(64.4192213382197,-9.75941427061367,
60.779009237256));
#147117=CARTESIAN_POINT('Ctrl Pts',(64.5917519527215,-9.83352394633715,
60.7599201369048));
#147118=CARTESIAN_POINT('Ctrl Pts',(64.7636436728503,-9.90338401441579,
60.7407900832214));
#147119=CARTESIAN_POINT('Ctrl Pts',(64.9346888991107,-9.96953429478545,
60.7216255705971));
#147120=CARTESIAN_POINT('Ctrl Pts',(65.1120846075897,-10.0381405699141,
60.7017495274652));
#147121=CARTESIAN_POINT('Ctrl Pts',(65.2885702109627,-10.1027569733337,
60.6818363413983));
#147122=CARTESIAN_POINT('Ctrl Pts',(65.4639649804991,-10.163959985253,60.6618886487032));
#147123=CARTESIAN_POINT('Ctrl Pts',(65.6217577290577,-10.2190208715972,
60.6439428384256));
#147124=CARTESIAN_POINT('Ctrl Pts',(65.7786685868604,-10.2713189031568,
60.6259689958084));
#147125=CARTESIAN_POINT('Ctrl Pts',(65.9345948041783,-10.3212524718176,
60.6079667941811));
#147126=CARTESIAN_POINT('Ctrl Pts',(66.1617756184333,-10.3940045014771,
60.5817380117839));
#147127=CARTESIAN_POINT('Ctrl Pts',(66.3868666255169,-10.4617357625455,
60.5554485392112));
#147128=CARTESIAN_POINT('Ctrl Pts',(66.6097177236863,-10.5249661998724,
60.5290770483234));
#147129=CARTESIAN_POINT('Ctrl Pts',(66.6556411171841,-10.5379962287942,
60.5236426198502));
#147130=CARTESIAN_POINT('Ctrl Pts',(66.7014695395411,-10.5508350301772,
60.5182047170576));
#147131=CARTESIAN_POINT('Ctrl Pts',(66.7472018955564,-10.5634869991576,
60.5127631675472));
#147132=CARTESIAN_POINT('Ctrl Pts',(66.9802171685718,-10.627951248609,60.4850374115337));
#147133=CARTESIAN_POINT('Ctrl Pts',(67.2107340791529,-10.6875669815364,
60.457215529793));
#147134=CARTESIAN_POINT('Ctrl Pts',(67.4386303704974,-10.74289155313,60.4292758802627));
#147135=CARTESIAN_POINT('Ctrl Pts',(67.5998059025019,-10.782018856198,60.4095160682424));
#147136=CARTESIAN_POINT('Ctrl Pts',(67.7596715637253,-10.8189990303699,
60.3896974299897));
#147137=CARTESIAN_POINT('Ctrl Pts',(67.9181936648736,-10.8540169049373,
60.3698135497309));
#147138=CARTESIAN_POINT('Ctrl Pts',(68.1914973421711,-10.9143902776157,
60.3355322882897));
#147139=CARTESIAN_POINT('Ctrl Pts',(68.4608051825333,-10.9689305948752,
60.3010566373054));
#147140=CARTESIAN_POINT('Ctrl Pts',(68.7259000127629,-11.0181836739645,
60.2663757344958));
#147141=CARTESIAN_POINT('Ctrl Pts',(69.0001300308213,-11.0691340178712,
60.2304997251617));
#147142=CARTESIAN_POINT('Ctrl Pts',(69.2698521901208,-11.1144268899995,
60.1944041771647));
#147143=CARTESIAN_POINT('Ctrl Pts',(69.5348702087699,-11.1546321440666,
60.1580854692593));
#147144=CARTESIAN_POINT('Ctrl Pts',(69.7478446792571,-11.1869419950699,
60.1288989346063));
#147145=CARTESIAN_POINT('Ctrl Pts',(69.9577821379011,-11.2159655707178,
60.0995684697029));
#147146=CARTESIAN_POINT('Ctrl Pts',(70.164597028615,-11.2419808637392,60.0700952271198));
#147147=CARTESIAN_POINT('Ctrl Pts',(70.4576205793241,-11.2788403640756,
60.0283363665135));
#147148=CARTESIAN_POINT('Ctrl Pts',(70.7443728961861,-11.3096600624236,
59.9862909687595));
#147149=CARTESIAN_POINT('Ctrl Pts',(71.0245712394748,-11.3350228063679,
59.9439827482278));
#147150=CARTESIAN_POINT('Ctrl Pts',(71.3047695827635,-11.3603855503121,
59.9016745276962));
#147151=CARTESIAN_POINT('Ctrl Pts',(71.5784145540188,-11.3802916869536,
59.8591036487755));
#147152=CARTESIAN_POINT('Ctrl Pts',(71.8452775886959,-11.3952984906318,
59.816295698531));
#147153=CARTESIAN_POINT('Ctrl Pts',(71.9953031740864,-11.4037350450215,
59.7922298409177));
#147154=CARTESIAN_POINT('Ctrl Pts',(72.1431862617957,-11.4106226810622,
59.7680890736475));
#147155=CARTESIAN_POINT('Ctrl Pts',(72.2888927362891,-11.4160562736744,
59.7438779705844));
#147156=CARTESIAN_POINT('Ctrl Pts',(72.3617459735358,-11.4187730699805,
59.7317724190528));
#147157=CARTESIAN_POINT('Ctrl Pts',(72.4340550627953,-11.4211263104244,
59.719649306186));
#147158=CARTESIAN_POINT('Ctrl Pts',(72.5058162028691,-11.4231275454711,
59.7075091748962));
#147159=CARTESIAN_POINT('Ctrl Pts',(72.541696772906,-11.4241281629944,59.7014391092512));
#147160=CARTESIAN_POINT('Ctrl Pts',(72.5774403560181,-11.4250407762218,
59.6953647904832));
#147161=CARTESIAN_POINT('Ctrl Pts',(72.6130464884757,-11.4258668097512,
59.6892862902963));
#147162=CARTESIAN_POINT('Ctrl Pts',(72.6308495547045,-11.4262798265159,
59.6862470402029));
#147163=CARTESIAN_POINT('Ctrl Pts',(72.6486182582896,-11.4266711981716,
59.6832067448475));
#147164=CARTESIAN_POINT('Ctrl Pts',(72.6663525427507,-11.4270411015404,
59.6801654131775));
#147165=CARTESIAN_POINT('Ctrl Pts',(72.6752196849812,-11.4272260532248,
59.6786447473425));
#147166=CARTESIAN_POINT('Ctrl Pts',(72.684078222432,-11.4274056378258,59.6771238224347));
#147167=CARTESIAN_POINT('Ctrl Pts',(72.6929281481366,-11.4275798773662,
59.6756026395695));
#147168=CARTESIAN_POINT('Ctrl Pts',(72.6964426804789,-11.4276490723539,
59.6749985388621));
#147169=CARTESIAN_POINT('Ctrl Pts',(72.6997502454414,-11.4277134482094,
59.6744298198451));
#147170=CARTESIAN_POINT('Ctrl Pts',(72.7030957980396,-11.4277778278489,
59.6738542816511));
#147171=CARTESIAN_POINT('Ctrl Pts',(72.7081746641268,-11.4278755622465,
59.6729805600971));
#147172=CARTESIAN_POINT('Ctrl Pts',(72.7133410737757,-11.4279734137452,
59.6720911235426));
#147173=CARTESIAN_POINT('Ctrl Pts',(72.7194520827137,-11.428086583983,59.6710383182928));
#147174=CARTESIAN_POINT('Ctrl Pts',(72.9810700988372,-11.4329315078579,
59.6259667395027));
#147175=CARTESIAN_POINT('Ctrl Pts',(73.2479207672801,-11.4334108481625,
59.5785889245677));
#147176=CARTESIAN_POINT('Ctrl Pts',(73.519805288403,-11.4291105759769,59.5289406205662));
#147177=CARTESIAN_POINT('Ctrl Pts',(73.7881294221,-11.4248666167985,59.479942471993));
#147178=CARTESIAN_POINT('Ctrl Pts',(74.0613566957298,-11.4159672194884,
59.4287328216431));
#147179=CARTESIAN_POINT('Ctrl Pts',(74.3392563577797,-11.4019861630037,
59.3753589727235));
#147180=CARTESIAN_POINT('Ctrl Pts',(74.6123805523945,-11.388245358988,59.3229023076376));
#147181=CARTESIAN_POINT('Ctrl Pts',(74.8900180959707,-11.3695958349094,
59.2683550418568));
#147182=CARTESIAN_POINT('Ctrl Pts',(75.1719082682765,-11.3456084272083,
59.2117763741919));
#147183=CARTESIAN_POINT('Ctrl Pts',(75.2718400877254,-11.3371047419758,
59.1917188845835));
#147184=CARTESIAN_POINT('Ctrl Pts',(75.3723059570812,-11.3279300071673,
59.1714062426861));
#147185=CARTESIAN_POINT('Ctrl Pts',(75.4732929209364,-11.3180644214381,
59.1508415889956));
#147186=CARTESIAN_POINT('Ctrl Pts',(75.7652124079432,-11.2895463175644,
59.0913960632897));
#147187=CARTESIAN_POINT('Ctrl Pts',(76.0614882663886,-11.2552580782005,
59.0298433493103));
#147188=CARTESIAN_POINT('Ctrl Pts',(76.3619250156597,-11.2146421120415,
58.9662470746486));
#147189=CARTESIAN_POINT('Ctrl Pts',(76.6471518824436,-11.1760823659484,
58.9058704189801));
#147190=CARTESIAN_POINT('Ctrl Pts',(76.9361293595584,-11.1318188885074,
58.8436516267443));
#147191=CARTESIAN_POINT('Ctrl Pts',(77.2286584914008,-11.0813483885709,
58.7796645919439));
#147192=CARTESIAN_POINT('Ctrl Pts',(77.4808729255173,-11.0378334452869,
58.7244958855955));
#147193=CARTESIAN_POINT('Ctrl Pts',(77.7357273295204,-10.989703883753,58.6680128402438));
#147194=CARTESIAN_POINT('Ctrl Pts',(77.9930700490635,-10.9366243447965,
58.610277964424));
#147195=CARTESIAN_POINT('Ctrl Pts',(78.2338867509886,-10.8869534641363,
58.556250703013));
#147196=CARTESIAN_POINT('Ctrl Pts',(78.4768827703228,-10.832950409161,58.501127128419));
#147197=CARTESIAN_POINT('Ctrl Pts',(78.7219624690903,-10.7740694948733,
58.4449636970163));
#147198=CARTESIAN_POINT('Ctrl Pts',(78.9234244085341,-10.7256678392149,
58.3987958835535));
#147199=CARTESIAN_POINT('Ctrl Pts',(79.126294167326,-10.6739692719136,58.3519255825824));
#147200=CARTESIAN_POINT('Ctrl Pts',(79.3305018595802,-10.6186523159379,
58.3043932560179));
#147201=CARTESIAN_POINT('Ctrl Pts',(79.5640892996969,-10.555376804625,58.2500223635092));
#147202=CARTESIAN_POINT('Ctrl Pts',(79.799427858751,-10.4873682963686,58.1947861358713));
#147203=CARTESIAN_POINT('Ctrl Pts',(80.03638006309,-10.4141215949237,58.138760307174));
#147204=CARTESIAN_POINT('Ctrl Pts',(80.0775805354926,-10.4013856986281,
58.1290187197703));
#147205=CARTESIAN_POINT('Ctrl Pts',(80.118829689162,-10.3884913809975,58.1192533088284));
#147206=CARTESIAN_POINT('Ctrl Pts',(80.1601266628084,-10.3754359204086,
58.1094645360177));
#147207=CARTESIAN_POINT('Ctrl Pts',(80.3413664727616,-10.318139489531,58.0665046005249));
#147208=CARTESIAN_POINT('Ctrl Pts',(80.5235305056401,-10.2577417309642,
58.0230937615654));
#147209=CARTESIAN_POINT('Ctrl Pts',(80.7064782053457,-10.1936443957154,
57.9792858696897));
#147210=CARTESIAN_POINT('Ctrl Pts',(80.8895041300135,-10.1295196536633,
57.9354592463914));
#147211=CARTESIAN_POINT('Ctrl Pts',(81.0733151387544,-10.0616917875014,
57.89123506624));
#147212=CARTESIAN_POINT('Ctrl Pts',(81.2577249642791,-9.98953601001032,
57.8466803522544));
#147213=CARTESIAN_POINT('Ctrl Pts',(81.4299851561752,-9.92213413464029,
57.8050610754117));
#147214=CARTESIAN_POINT('Ctrl Pts',(81.6027680171716,-9.85095528252832,
57.7631533837741));
#147215=CARTESIAN_POINT('Ctrl Pts',(81.7758764615611,-9.77547488249053,
57.7210242487723));
#147216=CARTESIAN_POINT('Ctrl Pts',(81.7880859230404,-9.77015119628938,
57.7180528509715));
#147217=CARTESIAN_POINT('Ctrl Pts',(81.8002969836653,-9.76480610695126,
57.7150803570125));
#147218=CARTESIAN_POINT('Ctrl Pts',(81.8125095647161,-9.7594394284026,57.7121067929141));
#147219=CARTESIAN_POINT('Ctrl Pts',(64.2331132192591,-10.03116309748,61.45331963667));
#147220=CARTESIAN_POINT('Ctrl Pts',(64.8063721520591,-10.24997839378,61.35223861989));
#147221=CARTESIAN_POINT('Ctrl Pts',(66.0434889198791,-10.63841202821,61.13410155544));
#147222=CARTESIAN_POINT('Ctrl Pts',(68.0303682092991,-11.08801271264,60.7837611293));
#147223=CARTESIAN_POINT('Ctrl Pts',(70.2942220615191,-11.4211637098,60.38458261477));
#147224=CARTESIAN_POINT('Ctrl Pts',(72.8294884823191,-11.58264132366,59.9375467415));
#147225=CARTESIAN_POINT('Ctrl Pts',(75.4730113240291,-11.49327715213,59.47142234039));
#147226=CARTESIAN_POINT('Ctrl Pts',(77.9968724871491,-11.16992495207,59.02639752177));
#147227=CARTESIAN_POINT('Ctrl Pts',(80.2177679758191,-10.69349944306,58.63479372578));
#147228=CARTESIAN_POINT('Ctrl Pts',(81.5864419160991,-10.2722145784,58.39345958232));
#147229=CARTESIAN_POINT('Ctrl Pts',(82.2177997746791,-10.03126774286,58.28213415737));
#147230=CARTESIAN_POINT('Ctrl Pts',(64.1715173750991,-9.822263906076,60.65197132249));
#147231=CARTESIAN_POINT('Ctrl Pts',(64.7364200849891,-10.03788724212,60.55236373326));
#147232=CARTESIAN_POINT('Ctrl Pts',(65.9600066241391,-10.4222368381,60.33661241318));
#147233=CARTESIAN_POINT('Ctrl Pts',(67.9308405009391,-10.86825461979,59.9891012262));
#147234=CARTESIAN_POINT('Ctrl Pts',(70.1779537377492,-11.19894289262,59.59287453385));
#147235=CARTESIAN_POINT('Ctrl Pts',(72.6937925515491,-11.35916309554,59.14926427186));
#147236=CARTESIAN_POINT('Ctrl Pts',(75.3164862035391,-11.2705174991,58.68681261888));
#147237=CARTESIAN_POINT('Ctrl Pts',(77.8218404664591,-10.94955206463,58.2450510661));
#147238=CARTESIAN_POINT('Ctrl Pts',(80.0252868599591,-10.47682216277,57.8565240163801));
#147239=CARTESIAN_POINT('Ctrl Pts',(81.3794504710091,-10.05980091539,57.61774843546));
#147240=CARTESIAN_POINT('Ctrl Pts',(82.0016116056192,-9.82236568198599,
57.50804464108));
#147241=CARTESIAN_POINT('Ctrl Pts',(64.3417810494792,-9.15894490746699,
60.18227954555));
#147242=CARTESIAN_POINT('Ctrl Pts',(64.8801501889191,-9.36443279080099,
60.08735054068));
#147243=CARTESIAN_POINT('Ctrl Pts',(66.0607741025291,-9.73581431216599,
59.8791746906401));
#147244=CARTESIAN_POINT('Ctrl Pts',(67.9806588733992,-10.17045527885,59.54064720569));
#147245=CARTESIAN_POINT('Ctrl Pts',(70.1746155222091,-10.49332364665,59.153793454));
#147246=CARTESIAN_POINT('Ctrl Pts',(72.6287657256591,-10.6495511842,58.72106055842));
#147247=CARTESIAN_POINT('Ctrl Pts',(75.1853203123391,-10.56318728404,58.27027100713));
#147248=CARTESIAN_POINT('Ctrl Pts',(77.6319094913791,-10.24980056232,57.83887132416));
#147249=CARTESIAN_POINT('Ctrl Pts',(79.7799496563691,-9.78880534654499,
57.4601138874301));
#147250=CARTESIAN_POINT('Ctrl Pts',(81.0880385219991,-9.38532239160899,
57.22946252725));
#147251=CARTESIAN_POINT('Ctrl Pts',(81.6809972375691,-9.15903757193999,
57.12490790725));
#147252=CARTESIAN_POINT('Ctrl Pts',(64.6524871507491,-8.39735190850099,
60.29642878604));
#147253=CARTESIAN_POINT('Ctrl Pts',(65.1603916396291,-8.59120272152199,
60.20687152102));
#147254=CARTESIAN_POINT('Ctrl Pts',(66.2916878016091,-8.94769488368699,
60.0073934845));
#147255=CARTESIAN_POINT('Ctrl Pts',(68.1530751037291,-9.36927350378199,
59.67918068158));
#147256=CARTESIAN_POINT('Ctrl Pts',(70.2859997523291,-9.68316340882398,
59.30308851822));
#147257=CARTESIAN_POINT('Ctrl Pts',(72.6693218717691,-9.83480674783699,
58.88284452484));
#147258=CARTESIAN_POINT('Ctrl Pts',(75.1499385624891,-9.75106258857898,
58.44544487347));
#147259=CARTESIAN_POINT('Ctrl Pts',(77.5290563189391,-9.44637740348698,
58.02594222273));
#147260=CARTESIAN_POINT('Ctrl Pts',(79.6134815477891,-8.99885542575598,
57.65840181561));
#147261=CARTESIAN_POINT('Ctrl Pts',(80.8686694659091,-8.61091652845699,
57.43707831978));
#147262=CARTESIAN_POINT('Ctrl Pts',(81.4280992791691,-8.39743411163299,
57.33843574989));
#147263=CARTESIAN_POINT('',(81.3676320540161,-8.73787997306191,57.3182172534742));
#147264=CARTESIAN_POINT('Origin',(81.6276298114341,-8.73683444149237,58.7943917882984));
#147265=CARTESIAN_POINT('',(64.7026106475202,-8.73788137707176,60.2567101732879));
#147266=CARTESIAN_POINT('Ctrl Pts',(64.7026106495657,-8.73788137707563,
60.2567101848969));
#147267=CARTESIAN_POINT('Ctrl Pts',(64.8615289588377,-8.79636287531833,
60.2286885992441));
#147268=CARTESIAN_POINT('Ctrl Pts',(65.0242194072014,-8.85311144898981,
60.2000018670068));
#147269=CARTESIAN_POINT('Ctrl Pts',(65.1906746728955,-8.9081752454954,60.1706512945918));
#147270=CARTESIAN_POINT('Ctrl Pts',(65.3484303793116,-8.96036120716788,
60.1428346901381));
#147271=CARTESIAN_POINT('Ctrl Pts',(65.5095676690178,-9.01103369452827,
60.1144218212214));
#147272=CARTESIAN_POINT('Ctrl Pts',(65.6740443346344,-9.06026075602945,
60.0854201373193));
#147273=CARTESIAN_POINT('Ctrl Pts',(65.8254175891191,-9.1055660306726,60.0587289391403));
#147274=CARTESIAN_POINT('Ctrl Pts',(65.9796191823325,-9.14964703194275,
60.031539034199));
#147275=CARTESIAN_POINT('Ctrl Pts',(66.1365862032439,-9.19258130032827,
60.0038615123292));
#147276=CARTESIAN_POINT('Ctrl Pts',(66.1994474557214,-9.20977536994396,
59.9927773770751));
#147277=CARTESIAN_POINT('Ctrl Pts',(66.2627518288678,-9.226785877604,59.9816151080364));
#147278=CARTESIAN_POINT('Ctrl Pts',(66.3265033459271,-9.24360804472882,
59.9703739955178));
#147279=CARTESIAN_POINT('Ctrl Pts',(66.5717190342031,-9.3083133173261,59.927135853582));
#147280=CARTESIAN_POINT('Ctrl Pts',(66.8234929969238,-9.37029807677882,
59.8827413125373));
#147281=CARTESIAN_POINT('Ctrl Pts',(67.0820950773821,-9.4293459458507,59.8371427899164));
#147282=CARTESIAN_POINT('Ctrl Pts',(67.3236004841906,-9.48449004838888,
59.7945588720458));
#147283=CARTESIAN_POINT('Ctrl Pts',(67.5710612273839,-9.53707216271436,
59.7509248662921));
#147284=CARTESIAN_POINT('Ctrl Pts',(67.8246519491363,-9.58691921072333,
59.7062099778814));
#147285=CARTESIAN_POINT('Ctrl Pts',(67.8916055025385,-9.60007993272353,
59.6944042594056));
#147286=CARTESIAN_POINT('Ctrl Pts',(67.9589860937402,-9.61305004355902,
59.6825232425739));
#147287=CARTESIAN_POINT('Ctrl Pts',(68.0267963286315,-9.62582647639699,
59.6705664681337));
#147288=CARTESIAN_POINT('Ctrl Pts',(68.0758505082094,-9.63506899608155,
59.6619168924245));
#147289=CARTESIAN_POINT('Ctrl Pts',(68.125129516931,-9.64421016985909,59.6532276733608));
#147290=CARTESIAN_POINT('Ctrl Pts',(68.1746351227241,-9.65324707650833,
59.6444984993631));
#147291=CARTESIAN_POINT('Ctrl Pts',(68.4597847662522,-9.70529917582814,
59.5942189236698));
#147292=CARTESIAN_POINT('Ctrl Pts',(68.7524450534309,-9.75392338446086,
59.5426150331964));
#147293=CARTESIAN_POINT('Ctrl Pts',(69.0526690215057,-9.79862110545472,
59.4896774592567));
#147294=CARTESIAN_POINT('Ctrl Pts',(69.3443409468083,-9.84204558759224,
59.4382478408593));
#147295=CARTESIAN_POINT('Ctrl Pts',(69.6431520356423,-9.88176400622764,
59.3855593785784));
#147296=CARTESIAN_POINT('Ctrl Pts',(69.9491160079193,-9.91728452785944,
59.3316096557762));
#147297=CARTESIAN_POINT('Ctrl Pts',(70.021529525791,-9.92569128865828,59.3188411942243));
#147298=CARTESIAN_POINT('Ctrl Pts',(70.0943435402784,-9.93386275391163,
59.3060021142891));
#147299=CARTESIAN_POINT('Ctrl Pts',(70.1675579135585,-9.941792116299,59.29309244248));
#147300=CARTESIAN_POINT('Ctrl Pts',(70.1976472393991,-9.94505089128939,
59.2877868815067));
#147301=CARTESIAN_POINT('Ctrl Pts',(70.2278041846103,-9.94826877393099,
59.2824693977986));
#147302=CARTESIAN_POINT('Ctrl Pts',(70.2580287970341,-9.95144511113433,
59.2771399831468));
#147303=CARTESIAN_POINT('Ctrl Pts',(70.457293110271,-9.97238601328903,59.2420043084309));
#147304=CARTESIAN_POINT('Ctrl Pts',(70.659489612735,-9.99147794137391,59.2063516429878));
#147305=CARTESIAN_POINT('Ctrl Pts',(70.8649999857744,-10.0084667689348,
59.1701146740796));
#147306=CARTESIAN_POINT('Ctrl Pts',(71.0666836824957,-10.0251392584777,
59.1345524504346));
#147307=CARTESIAN_POINT('Ctrl Pts',(71.2715591381151,-10.039786381797,59.0984274494948));
#147308=CARTESIAN_POINT('Ctrl Pts',(71.4799768039724,-10.0521198835458,
59.061677815081));
#147309=CARTESIAN_POINT('Ctrl Pts',(71.6822225627885,-10.0640881512538,
59.0260164537101));
#147310=CARTESIAN_POINT('Ctrl Pts',(71.8878039703601,-10.073877845892,58.9897668731155));
#147311=CARTESIAN_POINT('Ctrl Pts',(72.0970295004326,-10.0811786262709,
58.9528746912693));
#147312=CARTESIAN_POINT('Ctrl Pts',(72.2571003275373,-10.0867641872365,
58.9246498276029));
#147313=CARTESIAN_POINT('Ctrl Pts',(72.4193039333546,-10.0908920360261,
58.8960488701054));
#147314=CARTESIAN_POINT('Ctrl Pts',(72.5837728363951,-10.0934033137685,
58.8670485590694));
#147315=CARTESIAN_POINT('Ctrl Pts',(72.5889778711876,-10.09348278951,58.8661307708119));
#147316=CARTESIAN_POINT('Ctrl Pts',(72.5941851743727,-10.0935606446403,
58.8652125826667));
#147317=CARTESIAN_POINT('Ctrl Pts',(72.5993947501158,-10.0936368748965,
58.8642939939051));
#147318=CARTESIAN_POINT('Ctrl Pts',(72.7565181226876,-10.0959360170016,
58.8365889040207));
#147319=CARTESIAN_POINT('Ctrl Pts',(72.9157167769922,-10.0969060819709,
58.8085179695934));
#147320=CARTESIAN_POINT('Ctrl Pts',(73.0762555072849,-10.0964561144708,
58.7802107415833));
#147321=CARTESIAN_POINT('Ctrl Pts',(73.2361228133097,-10.0960080288785,
58.752021903446));
#147322=CARTESIAN_POINT('Ctrl Pts',(73.3973188990355,-10.0941517228034,
58.7235987642996));
#147323=CARTESIAN_POINT('Ctrl Pts',(73.5591156265634,-10.0908491089493,
58.695069677654));
#147324=CARTESIAN_POINT('Ctrl Pts',(73.7212252509706,-10.0875401082073,
58.6664854189273));
#147325=CARTESIAN_POINT('Ctrl Pts',(73.8839377243019,-10.0827791874739,
58.6377948239968));
#147326=CARTESIAN_POINT('Ctrl Pts',(74.0465202638102,-10.0765805590394,
58.6091271032536));
#147327=CARTESIAN_POINT('Ctrl Pts',(74.2098916585598,-10.0703518546783,
58.58032028589));
#147328=CARTESIAN_POINT('Ctrl Pts',(74.3731317315009,-10.0626714977316,
58.5515365876632));
#147329=CARTESIAN_POINT('Ctrl Pts',(74.5354983984075,-10.0536067189506,
58.5229068885933));
#147330=CARTESIAN_POINT('Ctrl Pts',(74.6999245212776,-10.0444269626741,
58.4939140509211));
#147331=CARTESIAN_POINT('Ctrl Pts',(74.8634548104611,-10.0338274966925,
58.4650791673765));
#147332=CARTESIAN_POINT('Ctrl Pts',(75.0253219776175,-10.0219315564534,
58.4365375853093));
#147333=CARTESIAN_POINT('Ctrl Pts',(75.0712160880304,-10.0185587069473,
58.4284452059728));
#147334=CARTESIAN_POINT('Ctrl Pts',(75.1169765291583,-10.0150819570383,
58.4203764001192));
#147335=CARTESIAN_POINT('Ctrl Pts',(75.1625858832791,-10.011504868184,58.4123342404151));
#147336=CARTESIAN_POINT('Ctrl Pts',(75.1858092673094,-10.0096834850538,
58.4082393312272));
#147337=CARTESIAN_POINT('Ctrl Pts',(75.2089936066737,-10.0078333411188,
58.4041513080727));
#147338=CARTESIAN_POINT('Ctrl Pts',(75.2321388545488,-10.0059548274891,
58.4000701788148));
#147339=CARTESIAN_POINT('Ctrl Pts',(75.5062487793658,-9.98370752935837,
58.3517372320221));
#147340=CARTESIAN_POINT('Ctrl Pts',(75.7748719275291,-9.95748323024815,
58.3043718338795));
#147341=CARTESIAN_POINT('Ctrl Pts',(76.0379123704695,-9.9278821710273,58.2579907107122));
#147342=CARTESIAN_POINT('Ctrl Pts',(76.3079786025199,-9.89749046989149,
58.2103707514693));
#147343=CARTESIAN_POINT('Ctrl Pts',(76.5721601181975,-9.86353936051064,
58.1637883594333));
#147344=CARTESIAN_POINT('Ctrl Pts',(76.8304008668996,-9.82665083638614,
58.1182535083477));
#147345=CARTESIAN_POINT('Ctrl Pts',(77.0672365918304,-9.79281992319151,
58.0764929437557));
#147346=CARTESIAN_POINT('Ctrl Pts',(77.2990762891904,-9.75651805774799,
58.0356133378304));
#147347=CARTESIAN_POINT('Ctrl Pts',(77.5259085168275,-9.71820412518583,
57.9956166960039));
#147348=CARTESIAN_POINT('Ctrl Pts',(77.5722835992516,-9.71037097114477,
57.98743951774));
#147349=CARTESIAN_POINT('Ctrl Pts',(77.6184484777247,-9.70245252846947,
57.979299404357));
#147350=CARTESIAN_POINT('Ctrl Pts',(77.6644058729966,-9.69445110924848,
57.9711958759488));
#147351=CARTESIAN_POINT('Ctrl Pts',(77.9366797519281,-9.64704682457646,
57.9231866469732));
#147352=CARTESIAN_POINT('Ctrl Pts',(78.2016673585848,-9.59673221438433,
57.8764621844258));
#147353=CARTESIAN_POINT('Ctrl Pts',(78.4598486734758,-9.54366743699993,
57.8309378514623));
#147354=CARTESIAN_POINT('Ctrl Pts',(78.7237453817438,-9.48942795773075,
57.7844057404137));
#147355=CARTESIAN_POINT('Ctrl Pts',(78.9805321306992,-9.43231602864913,
57.7391273064302));
#147356=CARTESIAN_POINT('Ctrl Pts',(79.2307594684004,-9.3724652090838,57.6950054752351));
#147357=CARTESIAN_POINT('Ctrl Pts',(79.3496677215687,-9.3440240464571,57.674038741855));
#147358=CARTESIAN_POINT('Ctrl Pts',(79.4670952051025,-9.31496378084444,
57.6533331082674));
#147359=CARTESIAN_POINT('Ctrl Pts',(79.5831029172942,-9.28529511169891,
57.6328778186374));
#147360=CARTESIAN_POINT('Ctrl Pts',(79.6454199770665,-9.26935768656075,
57.621889639641));
#147361=CARTESIAN_POINT('Ctrl Pts',(79.7073248346892,-9.2532431425775,57.6109741429906));
#147362=CARTESIAN_POINT('Ctrl Pts',(79.768819522112,-9.23695668243318,57.6001309705432));
#147363=CARTESIAN_POINT('Ctrl Pts',(79.9384711523821,-9.19202557324938,
57.5702168111239));
#147364=CARTESIAN_POINT('Ctrl Pts',(80.1049977223805,-9.14578298969952,
57.5408536853916));
#147365=CARTESIAN_POINT('Ctrl Pts',(80.2682871329044,-9.09815175589844,
57.5120613640152));
#147366=CARTESIAN_POINT('Ctrl Pts',(80.4355213763116,-9.04936982128483,
57.482573462345));
#147367=CARTESIAN_POINT('Ctrl Pts',(80.5993602988871,-8.99913154808042,
57.4536842539922));
#147368=CARTESIAN_POINT('Ctrl Pts',(80.7597247279027,-8.94739041898081,
57.4254076950173));
#147369=CARTESIAN_POINT('Ctrl Pts',(80.9258767490569,-8.8937819396599,57.3961106279944));
#147370=CARTESIAN_POINT('Ctrl Pts',(81.0882990124221,-8.83856036728512,
57.3674712197974));
#147371=CARTESIAN_POINT('Ctrl Pts',(81.246945842003,-8.78170943534271,57.3394975102689));
#147372=CARTESIAN_POINT('Ctrl Pts',(81.2874202232777,-8.76720548148913,
57.3323607865908));
#147373=CARTESIAN_POINT('Ctrl Pts',(81.3276490768491,-8.75259564200151,
57.3252673552758));
#147374=CARTESIAN_POINT('Ctrl Pts',(81.36763205815,-8.73787997306976,57.3182172769027));
#147375=CARTESIAN_POINT('Origin',(64.963008146268,-8.7384120949578,61.7339660696974));
#147376=CARTESIAN_POINT('Ctrl Pts',(61.3161921152491,-8.63494495661699,
61.56839581797));
#147377=CARTESIAN_POINT('Ctrl Pts',(61.6689613460491,-8.80141153096799,
61.50619308462));
#147378=CARTESIAN_POINT('Ctrl Pts',(62.3879498808491,-9.12917633459899,
61.3794160071101));
#147379=CARTESIAN_POINT('Ctrl Pts',(63.4646091717291,-9.58075322763798,
61.1895719251));
#147380=CARTESIAN_POINT('Ctrl Pts',(64.1905860164991,-9.85765191546899,
61.06156262));
#147381=CARTESIAN_POINT('Ctrl Pts',(64.5445578719791,-9.98587197454498,
60.99914783146));
#147382=CARTESIAN_POINT('Ctrl Pts',(61.3635047997591,-8.32363710783399,
61.00358429971));
#147383=CARTESIAN_POINT('Ctrl Pts',(61.7136157253391,-8.48884930107399,
60.94185029729));
#147384=CARTESIAN_POINT('Ctrl Pts',(62.4267246286491,-8.813927159173,60.81610995745));
#147385=CARTESIAN_POINT('Ctrl Pts',(63.4936241370291,-9.26140270324298,
60.6279867884201));
#147386=CARTESIAN_POINT('Ctrl Pts',(64.2125417155791,-9.53560504453799,
60.50122222242));
#147387=CARTESIAN_POINT('Ctrl Pts',(64.5629831003891,-9.66254624807698,
60.43942995112));
#147388=CARTESIAN_POINT('Ctrl Pts',(61.5659552580091,-7.78462977649199,
60.70922393812));
#147389=CARTESIAN_POINT('Ctrl Pts',(61.9114635177491,-7.94767009832599,
60.64830150987));
#147390=CARTESIAN_POINT('Ctrl Pts',(62.6143922585991,-8.26809570192399,
60.52435620734));
#147391=CARTESIAN_POINT('Ctrl Pts',(63.6643933998191,-8.70847005284398,
60.33921267637));
#147392=CARTESIAN_POINT('Ctrl Pts',(64.3710883625392,-8.97800386246999,
60.21460328731));
#147393=CARTESIAN_POINT('Ctrl Pts',(64.7154169892491,-9.10273081888299,
60.15388886019));
#147394=CARTESIAN_POINT('Ctrl Pts',(61.8513779092791,-7.21005775654899,
60.7902425591001));
#147395=CARTESIAN_POINT('Ctrl Pts',(62.1919798108591,-7.37078290293399,
60.73018525417));
#147396=CARTESIAN_POINT('Ctrl Pts',(62.8840566835191,-7.68624928777699,
60.60815342879));
#147397=CARTESIAN_POINT('Ctrl Pts',(63.9160444724591,-8.119053895848,60.42618613784));
#147398=CARTESIAN_POINT('Ctrl Pts',(64.6097103488191,-8.38361113555599,
60.30387412824));
#147399=CARTESIAN_POINT('Ctrl Pts',(64.9475228864791,-8.50597774477099,
60.24430866343));
#147400=CARTESIAN_POINT('',(61.8556180259586,-7.547638577278,60.7587117050873));
#147401=CARTESIAN_POINT('Ctrl Pts',(61.8556180259591,-7.54763857727799,
60.75871170509));
#147402=CARTESIAN_POINT('Ctrl Pts',(62.1807441003591,-7.69967237513199,
60.70138320604));
#147403=CARTESIAN_POINT('Ctrl Pts',(62.8258076996291,-7.98759295852699,
60.58764109685));
#147404=CARTESIAN_POINT('Ctrl Pts',(63.7736235103591,-8.38552632889799,
60.42051556228));
#147405=CARTESIAN_POINT('Ctrl Pts',(64.3947998691991,-8.62477639321799,
60.31098549452));
#147406=CARTESIAN_POINT('Ctrl Pts',(64.7026106434291,-8.73788137706399,
60.25671015007));
#147407=CARTESIAN_POINT('',(61.5370694839504,-8.36456075042586,61.1190591594443));
#147408=CARTESIAN_POINT('Ctrl Pts',(61.537069464754,-8.36456080303529,61.1190590948193));
#147409=CARTESIAN_POINT('Ctrl Pts',(61.572528837482,-8.25039306980219,61.0155853898407));
#147410=CARTESIAN_POINT('Ctrl Pts',(61.619097823721,-8.11839868372747,60.9296178865568));
#147411=CARTESIAN_POINT('Ctrl Pts',(61.72823931643,-7.83865781611668,60.8067047653259));
#147412=CARTESIAN_POINT('Ctrl Pts',(61.7906680935864,-7.69127956002283,
60.7699199295052));
#147413=CARTESIAN_POINT('Ctrl Pts',(61.8556180259591,-7.54763857727799,
60.75871170509));
#147414=CARTESIAN_POINT('Ctrl Pts',(61.5375998153948,-8.36381223691337,
61.1200821961353));
#147415=CARTESIAN_POINT('Ctrl Pts',(61.7638676019835,-8.48785590553016,
61.0935564776125));
#147416=CARTESIAN_POINT('Ctrl Pts',(61.9904255296258,-8.60865722923069,
61.0669821445775));
#147417=CARTESIAN_POINT('Ctrl Pts',(62.2172365718248,-8.72616597744292,
61.0403576980771));
#147418=CARTESIAN_POINT('Ctrl Pts',(62.4543428442658,-8.84900859126664,
61.0125247354297));
#147419=CARTESIAN_POINT('Ctrl Pts',(62.6917262477102,-8.96825216347004,
60.9846367825683));
#147420=CARTESIAN_POINT('Ctrl Pts',(62.92930835593,-9.08381469527325,60.9566563455559));
#147421=CARTESIAN_POINT('Ctrl Pts',(63.1774284872662,-9.20450303659402,
60.9274348281683));
#147422=CARTESIAN_POINT('Ctrl Pts',(63.42576597902,-9.32117554294915,60.8981120121884));
#147423=CARTESIAN_POINT('Ctrl Pts',(63.6741838693174,-9.43372663307082,
60.8686121173679));
#147424=CARTESIAN_POINT('Ctrl Pts',(63.9226017596147,-9.54627772319248,
60.8391122225473));
#147425=CARTESIAN_POINT('Ctrl Pts',(64.1711003449158,-9.65470638105591,
60.8094345145158));
#147426=CARTESIAN_POINT('Ctrl Pts',(64.4194894281585,-9.75891075203393,
60.7794801263297));
#147427=CARTESIAN_POINT('Ctrl Pts',(59.3595940627791,-9.91651499671599,
62.64129792143));
#147428=CARTESIAN_POINT('Ctrl Pts',(61.9983506403891,-7.63333700038399,
61.37410443204));
#147429=CARTESIAN_POINT('Ctrl Pts',(63.8659696541791,-6.480223454794,58.3422073918001));
#147430=CARTESIAN_POINT('Ctrl Pts',(64.2231073245191,-6.94208487257399,
54.61475371526));
#147431=CARTESIAN_POINT('Ctrl Pts',(60.3806855157591,-10.72894715554,62.78026368079));
#147432=CARTESIAN_POINT('Ctrl Pts',(62.7316376310391,-8.36267113991899,
61.44466582565));
#147433=CARTESIAN_POINT('Ctrl Pts',(64.4149724654791,-7.13948508442198,
58.48833863363));
#147434=CARTESIAN_POINT('Ctrl Pts',(64.8063219458291,-7.53992389692399,
54.8938706937));
#147435=CARTESIAN_POINT('Ctrl Pts',(61.5100324248391,-11.44895486624,62.90864202214));
#147436=CARTESIAN_POINT('Ctrl Pts',(63.5792248770391,-9.04876204197899,
61.51862151364));
#147437=CARTESIAN_POINT('Ctrl Pts',(65.0678444367891,-7.77042731743899,
58.6411780333901));
#147438=CARTESIAN_POINT('Ctrl Pts',(65.4595128993991,-8.081181454842,55.1748163377));
#147439=CARTESIAN_POINT('Ctrl Pts',(62.7519440770891,-12.07793713058,63.001930692665));
#147440=CARTESIAN_POINT('Ctrl Pts',(64.5506391796491,-9.66794220213098,
61.5739182200701));
#147441=CARTESIAN_POINT('Ctrl Pts',(65.8341505913691,-8.345140508031,58.7751971799));
#147442=CARTESIAN_POINT('Ctrl Pts',(66.1846613547391,-8.56004330716699,
55.4275781765));
#147443=CARTESIAN_POINT('',(59.6330689813191,-9.92669794294899,62.60067797587));
#147444=CARTESIAN_POINT('Origin',(59.0283126277726,-11.8776332136077,56.407512485888));
#147445=CARTESIAN_POINT('Ctrl Pts',(62.6710204155491,-11.87440155793,62.91980324276));
#147446=CARTESIAN_POINT('Ctrl Pts',(61.5797032381311,-11.3041158507879,
62.8377246971986));
#147447=CARTESIAN_POINT('Ctrl Pts',(60.5660753810985,-10.656617993369,62.7258066167314));
#147448=CARTESIAN_POINT('Ctrl Pts',(59.6330689813191,-9.92669794294899,
62.60067797587));
#147449=CARTESIAN_POINT('Origin',(48.9523887185591,1.4210854715202E-14,
90.52409909588));
#147450=CARTESIAN_POINT('',(59.6330698027491,9.92669722269101,62.60067754791));
#147451=CARTESIAN_POINT('Ctrl Pts',(59.6330689813191,-9.92669794294899,
62.60067797587));
#147452=CARTESIAN_POINT('Ctrl Pts',(58.8256240021749,-9.29268345738896,
62.4965871587399));
#147453=CARTESIAN_POINT('Ctrl Pts',(58.1121214390089,-8.59697796096149,
62.3761470806078));
#147454=CARTESIAN_POINT('Ctrl Pts',(57.1869930364504,-7.45620088899646,
62.1948494800253));
#147455=CARTESIAN_POINT('Ctrl Pts',(56.9028114774077,-7.0597600374091,62.1343504064346));
#147456=CARTESIAN_POINT('Ctrl Pts',(56.5133433337057,-6.44066295576373,
62.0464075659451));
#147457=CARTESIAN_POINT('Ctrl Pts',(56.3278109528225,-6.12500857788751,
62.0031412305677));
#147458=CARTESIAN_POINT('Ctrl Pts',(56.1275782079375,-5.74606076495384,
61.9545711474323));
#147459=CARTESIAN_POINT('Ctrl Pts',(56.0315325883226,-5.55391891982303,
61.9308498620689));
#147460=CARTESIAN_POINT('Ctrl Pts',(55.9912441373022,-5.47100113770906,
61.920813777626));
#147461=CARTESIAN_POINT('Ctrl Pts',(55.9645795676856,-5.4155957217327,61.9141530327728));
#147462=CARTESIAN_POINT('Ctrl Pts',(55.9504938767487,-5.38602774362974,
61.9106239994492));
#147463=CARTESIAN_POINT('Ctrl Pts',(55.5450166264099,-4.52711198014621,
61.8087787806478));
#147464=CARTESIAN_POINT('Ctrl Pts',(55.2489854890233,-3.66087265800569,
61.726882166269));
#147465=CARTESIAN_POINT('Ctrl Pts',(54.8540101262023,-1.86737516575817,
61.6125178560279));
#147466=CARTESIAN_POINT('Ctrl Pts',(54.7550696578738,-0.939068762628913,
61.5800655192276));
#147467=CARTESIAN_POINT('Ctrl Pts',(54.7571025726164,0.965762057650877,
61.5806459286186));
#147468=CARTESIAN_POINT('Ctrl Pts',(54.8576920430293,1.89157838449658,61.6136107485148));
#147469=CARTESIAN_POINT('Ctrl Pts',(55.1557894049005,3.23393920163968,61.6998972699383));
#147470=CARTESIAN_POINT('Ctrl Pts',(55.2796908290689,3.67369113242594,61.7347999542579));
#147471=CARTESIAN_POINT('Ctrl Pts',(55.5020817713188,4.32117592818264,61.7948638456308));
#147472=CARTESIAN_POINT('Ctrl Pts',(55.6224120031278,4.64188471197103,61.8268235931936));
#147473=CARTESIAN_POINT('Ctrl Pts',(55.778725961735,5.01062902444841,61.8671595443865));
#147474=CARTESIAN_POINT('Ctrl Pts',(55.8608580366601,5.19363538838132,61.8880497823729));
#147475=CARTESIAN_POINT('Ctrl Pts',(55.896908547343,5.27177278704354,61.8971532233772));
#147476=CARTESIAN_POINT('Ctrl Pts',(55.9211312595259,5.3237989424665,61.9032551490484));
#147477=CARTESIAN_POINT('Ctrl Pts',(55.93249072425,5.34799379679885,61.9061103997539));
#147478=CARTESIAN_POINT('Ctrl Pts',(56.7870303300843,7.15064334101463,62.1203429205986));
#147479=CARTESIAN_POINT('Ctrl Pts',(58.0232520392425,8.66387025801734,62.3909057621657));
#147480=CARTESIAN_POINT('Ctrl Pts',(59.6330698027491,9.92669722269101,62.60067754791));
#147481=CARTESIAN_POINT('Ctrl Pts',(59.6330698027491,9.92669722269101,62.60067754791));
#147482=CARTESIAN_POINT('Ctrl Pts',(60.5660767630722,10.6566178221567,62.7258062817894));
#147483=CARTESIAN_POINT('Ctrl Pts',(61.5797045052489,11.304115765727,62.8377244443988));
#147484=CARTESIAN_POINT('Ctrl Pts',(62.6710208743191,11.87440113975,62.91980295862));
#147485=CARTESIAN_POINT('Ctrl Pts',(-3.58430183424491,-12.77734752092,56.71623037308));
#147486=CARTESIAN_POINT('Ctrl Pts',(-2.82654579637091,-13.56823877579,56.66356760301));
#147487=CARTESIAN_POINT('Ctrl Pts',(-1.22510960093091,-14.96301005098,56.57763219321));
#147488=CARTESIAN_POINT('Ctrl Pts',(1.36103340034909,-16.52464473566,56.54069563469));
#147489=CARTESIAN_POINT('Ctrl Pts',(3.87584585923909,-17.55452762874,56.60358098145));
#147490=CARTESIAN_POINT('Ctrl Pts',(6.19710063835909,-18.15797232338,56.74716429009));
#147491=CARTESIAN_POINT('Ctrl Pts',(8.31505282592909,-18.45204200109,56.94959224141));
#147492=CARTESIAN_POINT('Ctrl Pts',(10.3190076082391,-18.5227178858,57.20308600798));
#147493=CARTESIAN_POINT('Ctrl Pts',(12.2966611152891,-18.39728886114,57.51358361024));
#147494=CARTESIAN_POINT('Ctrl Pts',(14.2762842352891,-18.07077538528,57.88694259276));
#147495=CARTESIAN_POINT('Ctrl Pts',(16.1913087147191,-17.5550687573,58.30881641828));
#147496=CARTESIAN_POINT('Ctrl Pts',(18.0106355730791,-16.87094604643,58.76532096745));
#147497=CARTESIAN_POINT('Ctrl Pts',(19.7936798013391,-16.00018983021,59.26535024511));
#147498=CARTESIAN_POINT('Ctrl Pts',(21.6152587953191,-14.87219739396,59.8316118168));
#147499=CARTESIAN_POINT('Ctrl Pts',(23.5037332083091,-13.38226243744,60.48072054854));
#147500=CARTESIAN_POINT('Ctrl Pts',(25.4089773760291,-11.42609024385,61.20195839564));
#147501=CARTESIAN_POINT('Ctrl Pts',(27.1843832993891,-8.93696435445999,
61.93748494782));
#147502=CARTESIAN_POINT('Ctrl Pts',(28.5837262234791,-5.98779183204199,
62.56306222481));
#147503=CARTESIAN_POINT('Ctrl Pts',(29.4131721215591,-2.80038937228799,
62.95281639517));
#147504=CARTESIAN_POINT('Ctrl Pts',(29.5612752799991,-0.620166171525686,
63.023935917286));
#147505=CARTESIAN_POINT('Ctrl Pts',(29.5343220504091,0.444915684091514,
63.011087634094));
#147506=CARTESIAN_POINT('Ctrl Pts',(29.5338703742191,0.461774656562614,
63.0108722771));
#147507=CARTESIAN_POINT('Ctrl Pts',(-3.72288960953291,-12.85329830414,55.62299833527));
#147508=CARTESIAN_POINT('Ctrl Pts',(-2.94901860386991,-13.64890746123,55.56862071173));
#147509=CARTESIAN_POINT('Ctrl Pts',(-1.31349980804092,-15.05199668853,55.47970165767));
#147510=CARTESIAN_POINT('Ctrl Pts',(1.32767713553909,-16.6228801163,55.44051598947));
#147511=CARTESIAN_POINT('Ctrl Pts',(3.89588111527909,-17.65877088157,55.5036943663299));
#147512=CARTESIAN_POINT('Ctrl Pts',(6.26621663463909,-18.26566107639,55.64967374489));
#147513=CARTESIAN_POINT('Ctrl Pts',(8.42872386496909,-18.56136755362,55.8560400985301));
#147514=CARTESIAN_POINT('Ctrl Pts',(10.4746065168291,-18.63242271852,56.11476044379));
#147515=CARTESIAN_POINT('Ctrl Pts',(12.4933994745791,-18.50631935278,56.431858726));
#147516=CARTESIAN_POINT('Ctrl Pts',(14.5139561217791,-18.17810478474,56.81330363737));
#147517=CARTESIAN_POINT('Ctrl Pts',(16.4683569012591,-17.65977495691,57.24442226139));
#147518=CARTESIAN_POINT('Ctrl Pts',(18.3249224039791,-16.97222998037,57.71101147142));
#147519=CARTESIAN_POINT('Ctrl Pts',(20.1443477633591,-16.09715278017,58.22215868751));
#147520=CARTESIAN_POINT('Ctrl Pts',(22.0030374225591,-14.96355146807,58.80109378072));
#147521=CARTESIAN_POINT('Ctrl Pts',(23.9300250610891,-13.46607983077,59.4648497644901));
#147522=CARTESIAN_POINT('Ctrl Pts',(25.8743271231091,-11.49961504094,60.20254853862));
#147523=CARTESIAN_POINT('Ctrl Pts',(27.6865453689491,-8.99647741870398,
60.9551385269801));
#147524=CARTESIAN_POINT('Ctrl Pts',(29.1154374711391,-6.02908615362698,
61.59554524518));
#147525=CARTESIAN_POINT('Ctrl Pts',(29.9627342908991,-2.82017517727099,
61.99473019848));
#147526=CARTESIAN_POINT('Ctrl Pts',(30.1140601046791,-0.624535642130786,
62.06759020103));
#147527=CARTESIAN_POINT('Ctrl Pts',(30.0865221951591,0.448052485067714,
62.05442854821));
#147528=CARTESIAN_POINT('Ctrl Pts',(30.0860607192791,0.465030265795814,
62.05420793871));
#147529=CARTESIAN_POINT('Ctrl Pts',(-3.17320105054691,-12.28484166745,54.85174559045));
#147530=CARTESIAN_POINT('Ctrl Pts',(-2.42508695642091,-13.04513949903,54.80503919576));
#147531=CARTESIAN_POINT('Ctrl Pts',(-0.844253174050915,-14.3859726853,54.73047035947));
#147532=CARTESIAN_POINT('Ctrl Pts',(1.70866986857909,-15.8876335301,54.70700946437));
#147533=CARTESIAN_POINT('Ctrl Pts',(4.19228482572909,-16.87855813869,54.77837472681));
#147534=CARTESIAN_POINT('Ctrl Pts',(6.48653288913908,-17.45966035134,54.92597342556));
#147535=CARTESIAN_POINT('Ctrl Pts',(8.58186134395909,-17.74311613794,55.12908301981));
#147536=CARTESIAN_POINT('Ctrl Pts',(10.5664452653491,-17.81133256526,55.38081209437));
#147537=CARTESIAN_POINT('Ctrl Pts',(12.5270981927391,-17.69027633198,55.68738173201));
#147538=CARTESIAN_POINT('Ctrl Pts',(14.4918977503591,-17.37479365556,56.05469422228));
#147539=CARTESIAN_POINT('Ctrl Pts',(16.3945506037791,-16.87609727056,56.4687746378201));
#147540=CARTESIAN_POINT('Ctrl Pts',(18.2036342066391,-16.21416637664,56.91612646381));
#147541=CARTESIAN_POINT('Ctrl Pts',(19.9776601847591,-15.37142975168,57.40549259896));
#147542=CARTESIAN_POINT('Ctrl Pts',(21.7905301121891,-14.27980829232,57.95894164));
#147543=CARTESIAN_POINT('Ctrl Pts',(23.6696227303091,-12.83874523999,58.59230118133));
#147544=CARTESIAN_POINT('Ctrl Pts',(25.5636008457491,-10.94931579331,59.29438635056));
#147545=CARTESIAN_POINT('Ctrl Pts',(27.3248106085391,-8.55104953890899,
60.00792469414));
#147546=CARTESIAN_POINT('Ctrl Pts',(28.7082158942091,-5.72001717281198,
60.61198629947));
#147547=CARTESIAN_POINT('Ctrl Pts',(29.5252295808991,-2.67208753843899,
60.98663314509));
#147548=CARTESIAN_POINT('Ctrl Pts',(29.6707996220691,-0.591832166815786,
61.0548216514));
#147549=CARTESIAN_POINT('Ctrl Pts',(29.6442913120391,0.424574974273814,
61.04249344665));
#147550=CARTESIAN_POINT('Ctrl Pts',(29.6438471072391,0.440663529910414,
61.04228680651));
#147551=CARTESIAN_POINT('Ctrl Pts',(-2.38244347352091,-11.53445397631,55.02993629904));
#147552=CARTESIAN_POINT('Ctrl Pts',(-1.68100325115091,-12.24813930956,54.99404617299));
#147553=CARTESIAN_POINT('Ctrl Pts',(-0.199132288740913,-13.50679179131,
54.93948658306));
#147554=CARTESIAN_POINT('Ctrl Pts',(2.19404928560909,-14.91707579071,54.93693122039));
#147555=CARTESIAN_POINT('Ctrl Pts',(4.52391333623909,-15.8486431004,55.0177166612));
#147556=CARTESIAN_POINT('Ctrl Pts',(6.67880783080909,-16.3957040456,55.16484050833));
#147557=CARTESIAN_POINT('Ctrl Pts',(8.6498779854791,-16.6629883833,55.36014776661));
#147558=CARTESIAN_POINT('Ctrl Pts',(10.5198070717491,-16.72745755252,55.5983555735));
#147559=CARTESIAN_POINT('Ctrl Pts',(12.3703411755791,-16.61306375545,55.88583297768));
#147560=CARTESIAN_POINT('Ctrl Pts',(14.2280550377091,-16.31438773435,56.22829233863));
#147561=CARTESIAN_POINT('Ctrl Pts',(16.0299360351191,-15.84160835493,56.61291322706));
#147562=CARTESIAN_POINT('Ctrl Pts',(17.7454468009191,-15.21348917344,57.02735648449));
#147563=CARTESIAN_POINT('Ctrl Pts',(19.4292282283691,-14.41344352614,57.47976284219));
#147564=CARTESIAN_POINT('Ctrl Pts',(21.1506253523991,-13.37723731351,57.99030081481));
#147565=CARTESIAN_POINT('Ctrl Pts',(22.9343804115591,-12.01063606723,58.57294969782));
#147566=CARTESIAN_POINT('Ctrl Pts',(24.7295945359991,-10.22289665205,59.2163207090301));
#147567=CARTESIAN_POINT('Ctrl Pts',(26.3934737214891,-7.96306520251299,
59.86646337428));
#147568=CARTESIAN_POINT('Ctrl Pts',(27.6933626732391,-5.31203256334299,
60.41257442068));
#147569=CARTESIAN_POINT('Ctrl Pts',(28.4565964661691,-2.47660536052199,
60.74867761106));
#147570=CARTESIAN_POINT('Ctrl Pts',(28.5921150013391,-0.548662145128386,
60.80958320983));
#147571=CARTESIAN_POINT('Ctrl Pts',(28.5674129242191,0.393583630375914,
60.79855720673));
#147572=CARTESIAN_POINT('Ctrl Pts',(28.5669990101191,0.408498369893214,
60.79837239285));
#147573=CARTESIAN_POINT('',(25.6004794355172,-11.218697295749,60.475052154922));
#147574=CARTESIAN_POINT('',(25.5799831827151,-11.2436247403821,60.4681283373529));
#147575=CARTESIAN_POINT('Origin',(21.9145513802835,-0.849633245104839,64.0093316151609));
#147576=CARTESIAN_POINT('',(28.8585550967729,1.26413730018565E-6,60.8967821146319));
#147577=CARTESIAN_POINT('Origin',(28.2409971615791,4.54795488838455E-7,
62.26375785167));
#147578=CARTESIAN_POINT('Ctrl Pts',(24.9372765286891,-10.33197973489,59.27186775219));
#147579=CARTESIAN_POINT('Ctrl Pts',(25.0884729081682,-10.1544298226021,
59.3290195277117));
#147580=CARTESIAN_POINT('Ctrl Pts',(25.2354201309973,-9.9748009926422,59.3851860135425));
#147581=CARTESIAN_POINT('Ctrl Pts',(25.5208782555178,-9.61138944051975,
59.4953766986517));
#147582=CARTESIAN_POINT('Ctrl Pts',(25.6598691932805,-9.42681391865182,
59.5495917842428));
#147583=CARTESIAN_POINT('Ctrl Pts',(25.8594487747258,-9.15113148708486,
59.6281484626401));
#147584=CARTESIAN_POINT('Ctrl Pts',(25.9245460860465,-9.05934679202463,
59.6538934847045));
#147585=CARTESIAN_POINT('Ctrl Pts',(26.0518918830672,-8.87599629949502,
59.7044763172425));
#147586=CARTESIAN_POINT('Ctrl Pts',(26.1136416461275,-8.7852514273904,59.7291135015114));
#147587=CARTESIAN_POINT('Ctrl Pts',(26.2377099140975,-8.59835774438392,
59.7788244733545));
#147588=CARTESIAN_POINT('Ctrl Pts',(26.3309422684908,-8.45454220553908,
59.8163406575038));
#147589=CARTESIAN_POINT('Ctrl Pts',(26.4244444582738,-8.30525875180928,
59.8542091925063));
#147590=CARTESIAN_POINT('Ctrl Pts',(26.4868390017902,-8.20452135712609,
59.8795335075995));
#147591=CARTESIAN_POINT('Ctrl Pts',(26.5169758557494,-8.15534444186653,
59.8917905523518));
#147592=CARTESIAN_POINT('Ctrl Pts',(26.8081007315441,-7.67489638239888,
60.0104588863508));
#147593=CARTESIAN_POINT('Ctrl Pts',(27.0450450385791,-7.24149359007942,
60.1089036136706));
#147594=CARTESIAN_POINT('Ctrl Pts',(27.3681375817506,-6.58188262574454,
60.2449193946893));
#147595=CARTESIAN_POINT('Ctrl Pts',(27.4704472110256,-6.36042784165697,
60.2883182251975));
#147596=CARTESIAN_POINT('Ctrl Pts',(27.6643543418031,-5.9143493481966,60.3710792742253));
#147597=CARTESIAN_POINT('Ctrl Pts',(27.7564152946973,-5.6885104661461,60.4106417290895));
#147598=CARTESIAN_POINT('Ctrl Pts',(27.9280295321704,-5.2385244674707,60.4847886476882));
#147599=CARTESIAN_POINT('Ctrl Pts',(28.0492171779347,-4.89688936050973,
60.5374646811016));
#147600=CARTESIAN_POINT('Ctrl Pts',(28.1591754869717,-4.54903584161711,
60.5856085834238));
#147601=CARTESIAN_POINT('Ctrl Pts',(28.229991130401,-4.31575162637056,60.6166845351935));
#147602=CARTESIAN_POINT('Ctrl Pts',(28.2647375028393,-4.19632677709933,
60.6319696429302));
#147603=CARTESIAN_POINT('Ctrl Pts',(28.3617489734771,-3.84853026724173,
60.6747331281475));
#147604=CARTESIAN_POINT('Ctrl Pts',(28.4205039887194,-3.61803496350203,
60.7007531586585));
#147605=CARTESIAN_POINT('Ctrl Pts',(28.5262194626522,-3.15978242835333,
60.7477144820933));
#147606=CARTESIAN_POINT('Ctrl Pts',(28.573570911436,-2.92987058514986,60.7688305329133));
#147607=CARTESIAN_POINT('Ctrl Pts',(28.7770209552515,-1.80870266790406,
60.8597651208632));
#147608=CARTESIAN_POINT('Ctrl Pts',(28.8583068535147,-0.906823667388817,
60.8966776934278));
#147609=CARTESIAN_POINT('Ctrl Pts',(28.8585550967491,1.26413730024185E-6,
60.89678211462));
#147610=CARTESIAN_POINT('Origin',(27.8340462222691,-10.33198915989,80.111318784329));
#147611=CARTESIAN_POINT('',(25.5859599196424,-11.2434451392657,60.5013612007571));
#147612=CARTESIAN_POINT('Ctrl Pts',(25.5859731978904,-11.2434554550835,
60.5013588594437));
#147613=CARTESIAN_POINT('Ctrl Pts',(25.5617439507817,-11.2756175802506,
60.5056541712706));
#147614=CARTESIAN_POINT('Ctrl Pts',(25.5355170543215,-11.3077304797386,
60.5102892020757));
#147615=CARTESIAN_POINT('Ctrl Pts',(25.5071495594106,-11.3395024335167,
60.5152935580816));
#147616=CARTESIAN_POINT('Ctrl Pts',(25.4797518807739,-11.3701881807781,
60.5201268272181));
#147617=CARTESIAN_POINT('Ctrl Pts',(25.450357033342,-11.400555707154,60.5253046767574));
#147618=CARTESIAN_POINT('Ctrl Pts',(25.4188616887057,-11.430302309678,60.5308492906578));
#147619=CARTESIAN_POINT('Ctrl Pts',(25.3876284774293,-11.4598013334899,
60.536347757158));
#147620=CARTESIAN_POINT('Ctrl Pts',(25.3543290304519,-11.4886896256522,
60.5422070066329));
#147621=CARTESIAN_POINT('Ctrl Pts',(25.3188954936569,-11.5166339195595,
60.5484428698022));
#147622=CARTESIAN_POINT('Ctrl Pts',(25.2851308147859,-11.5432620858504,
60.5543850346674));
#147623=CARTESIAN_POINT('Ctrl Pts',(25.2494225844771,-11.569035071514,60.560670192729));
#147624=CARTESIAN_POINT('Ctrl Pts',(25.2117913961462,-11.5936084226505,
60.567294816086));
#147625=CARTESIAN_POINT('Ctrl Pts',(25.1746664986275,-11.6178511633954,
60.5738303116187));
#147626=CARTESIAN_POINT('Ctrl Pts',(25.1356698214058,-11.6409258437336,
60.5806962377468));
#147627=CARTESIAN_POINT('Ctrl Pts',(25.0948699814531,-11.662492632175,60.587880594608));
#147628=CARTESIAN_POINT('Ctrl Pts',(25.0547695127091,-11.6836897331148,
60.5949418006837));
#147629=CARTESIAN_POINT('Ctrl Pts',(25.0129270804413,-11.7034296793926,
60.6023106299535));
#147630=CARTESIAN_POINT('Ctrl Pts',(24.969457530366,-11.721388378979,60.6099669261679));
#147631=CARTESIAN_POINT('Ctrl Pts',(24.9583766179001,-11.7259662680479,
60.6119186083919));
#147632=CARTESIAN_POINT('Ctrl Pts',(24.9471902337381,-11.7304284263342,
60.6138889246517));
#147633=CARTESIAN_POINT('Ctrl Pts',(24.9359008166787,-11.7347695342002,
60.615877446481));
#147634=CARTESIAN_POINT('Ctrl Pts',(24.8950689026342,-11.7504705878782,
60.6230695939568));
#147635=CARTESIAN_POINT('Ctrl Pts',(24.8528848469115,-11.7645863342241,
60.6305006701846));
#147636=CARTESIAN_POINT('Ctrl Pts',(24.8095371872525,-11.7768605936715,
60.6381374890892));
#147637=CARTESIAN_POINT('Ctrl Pts',(24.7664707110653,-11.7890552336211,
60.6457247702041));
#147638=CARTESIAN_POINT('Ctrl Pts',(24.7222559707473,-11.7994316951804,
60.6535150818304));
#147639=CARTESIAN_POINT('Ctrl Pts',(24.6771182451751,-11.8077693443997,
60.6614687583141));
#147640=CARTESIAN_POINT('Ctrl Pts',(24.6323179488033,-11.8160446651282,
60.6693629767134));
#147641=CARTESIAN_POINT('Ctrl Pts',(24.5866088138828,-11.8223111141212,
60.6774180563243));
#147642=CARTESIAN_POINT('Ctrl Pts',(24.5402458485445,-11.8263901448243,
60.6855890881521));
#147643=CARTESIAN_POINT('Ctrl Pts',(24.5118636392179,-11.8288872220156,
60.6905911826916));
#147644=CARTESIAN_POINT('Ctrl Pts',(24.4832370623221,-11.8305653058195,
60.6956366147681));
#147645=CARTESIAN_POINT('Ctrl Pts',(24.4544300514047,-11.8313913716027,
60.700714123978));
#147646=CARTESIAN_POINT('Ctrl Pts',(24.4102349808851,-11.8326587032134,
60.7085039248094));
#147647=CARTESIAN_POINT('Ctrl Pts',(24.3656202037618,-11.8319176257155,
60.7163683549808));
#147648=CARTESIAN_POINT('Ctrl Pts',(24.3208617900099,-11.8290857387875,
60.724258732631));
#147649=CARTESIAN_POINT('Ctrl Pts',(24.2762129275026,-11.8262607832209,
60.7321297976958));
#147650=CARTESIAN_POINT('Ctrl Pts',(24.2314217272845,-11.8213550940037,
60.7400265781715));
#147651=CARTESIAN_POINT('Ctrl Pts',(24.1867724304541,-11.8143375855243,
60.7478989514316));
#147652=CARTESIAN_POINT('Ctrl Pts',(24.1421965809794,-11.8073316207304,
60.7557583747677));
#147653=CARTESIAN_POINT('Ctrl Pts',(24.0977627877234,-11.7982207526536,
60.763593361921));
#147654=CARTESIAN_POINT('Ctrl Pts',(24.0537549386197,-11.7870259624055,
60.7713538525533));
#147655=CARTESIAN_POINT('Ctrl Pts',(24.015060944415,-11.7771829194528,60.7781772803205));
#147656=CARTESIAN_POINT('Ctrl Pts',(23.9766965226053,-11.7657296368449,
60.784943066333));
#147657=CARTESIAN_POINT('Ctrl Pts',(23.938849578094,-11.7527133111511,60.791618075687));
#147658=CARTESIAN_POINT('Ctrl Pts',(23.8958012397551,-11.7379081214686,
60.7992104471397));
#147659=CARTESIAN_POINT('Ctrl Pts',(23.8534319854631,-11.7210830022974,
60.8066836786859));
#147660=CARTESIAN_POINT('Ctrl Pts',(23.8120016585327,-11.7023562910476,
60.8139918950497));
#147661=CARTESIAN_POINT('Ctrl Pts',(23.7705439333247,-11.6836171956418,
60.8213049444079));
#147662=CARTESIAN_POINT('Ctrl Pts',(23.7300269189893,-11.6629743125864,
60.828452664821));
#147663=CARTESIAN_POINT('Ctrl Pts',(23.6906856655416,-11.6405917607177,
60.8353935526258));
#147664=CARTESIAN_POINT('Ctrl Pts',(23.6512108294834,-11.6181332092444,
60.8423580081067));
#147665=CARTESIAN_POINT('Ctrl Pts',(23.61292023339,-11.5939235627926,60.8491141391936));
#147666=CARTESIAN_POINT('Ctrl Pts',(23.5760181235856,-11.5681689960332,
60.8556258731524));
#147667=CARTESIAN_POINT('Ctrl Pts',(23.5436778970136,-11.5455982398168,
60.8613326187212));
#147668=CARTESIAN_POINT('Ctrl Pts',(23.5124037313837,-11.5218417453141,
60.8668517195986));
#147669=CARTESIAN_POINT('Ctrl Pts',(23.4823083059907,-11.4970595304308,
60.8721632679438));
#147670=CARTESIAN_POINT('Ctrl Pts',(23.4457177470307,-11.4669288682786,
60.8786211438621));
#147671=CARTESIAN_POINT('Ctrl Pts',(23.4108755040482,-11.4352865540032,
60.8847711606764));
#147672=CARTESIAN_POINT('Ctrl Pts',(23.3779075667015,-11.4024230541389,
60.8905910114592));
#147673=CARTESIAN_POINT('Ctrl Pts',(23.3447898798322,-11.369410279136,60.8964372976198));
#147674=CARTESIAN_POINT('Ctrl Pts',(23.3135636764316,-11.3351657988586,
60.9019503917891));
#147675=CARTESIAN_POINT('Ctrl Pts',(23.2843063996213,-11.2999978236278,
60.9071165458509));
#147676=CARTESIAN_POINT('Ctrl Pts',(23.2547721708609,-11.264496945257,60.9123316031803));
#147677=CARTESIAN_POINT('Ctrl Pts',(23.2272443510674,-11.2280556116708,
60.9171931157136));
#147678=CARTESIAN_POINT('Ctrl Pts',(23.2017503470999,-11.1909957260633,
60.9216961554168));
#147679=CARTESIAN_POINT('Ctrl Pts',(23.1863525897707,-11.1686124579834,
60.9244158816976));
#147680=CARTESIAN_POINT('Ctrl Pts',(23.1716957239107,-11.1460036003936,
60.9270050212694));
#147681=CARTESIAN_POINT('Ctrl Pts',(23.1577767525345,-11.1232395308346,
60.9294640815484));
#147682=CARTESIAN_POINT('Ctrl Pts',(23.1327166558873,-11.0822544775707,
60.9338914409119));
#147683=CARTESIAN_POINT('Ctrl Pts',(23.1100497867108,-11.0407673431689,
60.9378969026038));
#147684=CARTESIAN_POINT('Ctrl Pts',(23.0896832982784,-10.9991169831627,
60.9414967508537));
#147685=CARTESIAN_POINT('Ctrl Pts',(23.0690722941755,-10.9569665779111,
60.9451398181057));
#147686=CARTESIAN_POINT('Ctrl Pts',(23.0508168200725,-10.9146493658429,
60.9483675477527));
#147687=CARTESIAN_POINT('Ctrl Pts',(23.0347783054181,-10.8724843186724,
60.9512042831912));
#147688=CARTESIAN_POINT('Ctrl Pts',(23.0184359877794,-10.8295205773937,
60.9540947523269));
#147689=CARTESIAN_POINT('Ctrl Pts',(23.0043949684957,-10.7867151439778,
60.9565793528));
#147690=CARTESIAN_POINT('Ctrl Pts',(22.9924714929908,-10.7443668699682,
60.9586903899386));
#147691=CARTESIAN_POINT('Ctrl Pts',(22.9895840444815,-10.7341115999663,
60.9592016092586));
#147692=CARTESIAN_POINT('Ctrl Pts',(22.9868206267988,-10.7238829530939,
60.9596909478518));
#147693=CARTESIAN_POINT('Ctrl Pts',(22.9841783578299,-10.7136848126932,
60.9601589125555));
#147694=CARTESIAN_POINT('Ctrl Pts',(22.9727445921569,-10.6695548815562,
60.9621839141084));
#147695=CARTESIAN_POINT('Ctrl Pts',(22.9635782890116,-10.6259943202261,
60.9638088760509));
#147696=CARTESIAN_POINT('Ctrl Pts',(22.9564244603178,-10.5832263381758,
60.9650802235541));
#147697=CARTESIAN_POINT('Ctrl Pts',(22.9490201628826,-10.5389609701676,
60.9663960832789));
#147698=CARTESIAN_POINT('Ctrl Pts',(22.9437711795339,-10.495544595905,60.9673332303685));
#147699=CARTESIAN_POINT('Ctrl Pts',(22.940391170487,-10.4531675797244,60.9679437773532));
#147700=CARTESIAN_POINT('Ctrl Pts',(22.9370852180643,-10.4117190518159,
60.9685409471403));
#147701=CARTESIAN_POINT('Ctrl Pts',(22.9355668160252,-10.3712642552272,
60.9688257461811));
#147702=CARTESIAN_POINT('Ctrl Pts',(22.9355719204515,-10.33193324195,60.9688462512761));
#147703=CARTESIAN_POINT('Ctrl Pts',(25.5859731981751,-11.2434554547056,
60.5013588593932));
#147704=CARTESIAN_POINT('Ctrl Pts',(25.5844441899389,-11.2434658445421,
60.4927332003613));
#147705=CARTESIAN_POINT('Ctrl Pts',(25.5814984568459,-11.2436306576258,
60.4767534011199));
#147706=CARTESIAN_POINT('Ctrl Pts',(25.5799825962517,-11.2436242846107,
60.468128440764));
#147707=CARTESIAN_POINT('Origin',(17.7894674803291,1.4210854715202E-14,
100.88908350184));
#147708=CARTESIAN_POINT('Ctrl Pts',(25.585946658962,-11.2434347939771,60.5013635109443));
#147709=CARTESIAN_POINT('Ctrl Pts',(25.5908280517064,-11.2352178056434,
60.4925865053532));
#147710=CARTESIAN_POINT('Ctrl Pts',(25.5956760553759,-11.2269748700148,
60.4838153871567));
#147711=CARTESIAN_POINT('Ctrl Pts',(25.6004962205391,-11.21871037585,60.47504917764));
#147712=CARTESIAN_POINT('Origin',(17.7894674803291,1.4210854715202E-14,
100.88908350184));
#147713=CARTESIAN_POINT('',(25.600494243824,11.2187561752663,60.4750587214126));
#147714=CARTESIAN_POINT('',(25.6004957464494,11.2187573377186,60.4750584567717));
#147715=CARTESIAN_POINT('',(25.5858158203339,11.2436003008624,60.5011154491916));
#147716=CARTESIAN_POINT('Ctrl Pts',(25.6004937437591,11.2187557868,60.4750588099));
#147717=CARTESIAN_POINT('Ctrl Pts',(25.5980190908531,11.2229268927494,60.4793882956317));
#147718=CARTESIAN_POINT('Ctrl Pts',(25.5932000195592,11.2311758344546,60.4882199299609));
#147719=CARTESIAN_POINT('Ctrl Pts',(25.5882867359841,11.2394404119784,60.4967919610514));
#147720=CARTESIAN_POINT('Ctrl Pts',(25.585824508856,11.2435868068197,60.5011009711373));
#147721=CARTESIAN_POINT('',(25.5799682824491,11.24364172947,60.46812340452));
#147722=CARTESIAN_POINT('Ctrl Pts',(17.4667653729091,-22.5257212764,77.256905072711));
#147723=CARTESIAN_POINT('Ctrl Pts',(17.4522156153291,-22.52947690984,77.201794509167));
#147724=CARTESIAN_POINT('Ctrl Pts',(17.2326821287691,-22.58361462996,76.351112313277));
#147725=CARTESIAN_POINT('Ctrl Pts',(16.9332603507591,-22.57430986834,74.585159968858));
#147726=CARTESIAN_POINT('Ctrl Pts',(16.9282178457291,-22.22368100432,72.0018522533659));
#147727=CARTESIAN_POINT('Ctrl Pts',(17.3279784679891,-21.55585890438,69.568778249818));
#147728=CARTESIAN_POINT('Ctrl Pts',(18.0359271396891,-20.63613602496,67.425763312453));
#147729=CARTESIAN_POINT('Ctrl Pts',(18.9494515331591,-19.52905542686,65.598121631019));
#147730=CARTESIAN_POINT('Ctrl Pts',(20.0049202231791,-18.26930231769,64.050828430023));
#147731=CARTESIAN_POINT('Ctrl Pts',(21.1756845328891,-16.86079661466,62.74165530726));
#147732=CARTESIAN_POINT('Ctrl Pts',(22.4532806921391,-15.29024780344,61.65009812484));
#147733=CARTESIAN_POINT('Ctrl Pts',(23.8321876788191,-13.5386198194,60.78746444366));
#147734=CARTESIAN_POINT('Ctrl Pts',(24.9093942416691,-12.10874261238,60.35716873393));
#147735=CARTESIAN_POINT('Ctrl Pts',(25.5188775489791,-11.26992181782,60.2071336687));
#147736=CARTESIAN_POINT('Ctrl Pts',(25.6673509880891,-11.06368060085,60.17641247788));
#147737=CARTESIAN_POINT('Ctrl Pts',(18.7773649827691,-17.75527490826,76.717063290409));
#147738=CARTESIAN_POINT('Ctrl Pts',(18.7654556117691,-17.75828882524,76.674914380299));
#147739=CARTESIAN_POINT('Ctrl Pts',(18.5862635620091,-17.80174165801,76.0240512343981));
#147740=CARTESIAN_POINT('Ctrl Pts',(18.3577568645891,-17.79425534819,74.665378823862));
#147741=CARTESIAN_POINT('Ctrl Pts',(18.4246335003491,-17.51291935268,72.6770817004958));
#147742=CARTESIAN_POINT('Ctrl Pts',(18.8714641952291,-16.98119012651,70.822183427483));
#147743=CARTESIAN_POINT('Ctrl Pts',(19.6142963879091,-16.25801796827,69.218239633607));
#147744=CARTESIAN_POINT('Ctrl Pts',(20.5621683937491,-15.40160733776,67.8849620187121));
#147745=CARTESIAN_POINT('Ctrl Pts',(21.6579870981791,-14.44562122449,66.791899033372));
#147746=CARTESIAN_POINT('Ctrl Pts',(22.8780955574091,-13.40004445027,65.903735017982));
#147747=CARTESIAN_POINT('Ctrl Pts',(24.2153171433191,-12.26374841242,65.203217298719));
#147748=CARTESIAN_POINT('Ctrl Pts',(25.6646851711591,-11.03571934281,64.698047871997));
#147749=CARTESIAN_POINT('Ctrl Pts',(26.8015432713391,-10.07428690511,64.495800893793));
#147750=CARTESIAN_POINT('Ctrl Pts',(27.4463952672191,-9.53132694979998,
64.453831767256));
#147751=CARTESIAN_POINT('Ctrl Pts',(27.6035705906891,-9.399240458337,64.448068196782));
#147752=CARTESIAN_POINT('Ctrl Pts',(22.6527444970191,-14.84009533989,75.599270274124));
#147753=CARTESIAN_POINT('Ctrl Pts',(22.6450480694791,-14.8417831418,75.575183427031));
#147754=CARTESIAN_POINT('Ctrl Pts',(22.5298127564291,-14.866114563,75.203116801731));
#147755=CARTESIAN_POINT('Ctrl Pts',(22.4006621202491,-14.86192846848,74.422696506464));
#147756=CARTESIAN_POINT('Ctrl Pts',(22.5181198569391,-14.70436463479,73.2633823361753));
#147757=CARTESIAN_POINT('Ctrl Pts',(22.9377195244991,-14.4052238805,72.1556566073007));
#147758=CARTESIAN_POINT('Ctrl Pts',(23.6141508774891,-13.99538058674,71.163675788398));
#147759=CARTESIAN_POINT('Ctrl Pts',(24.4918032145691,-13.50533859052,70.299994638951));
#147760=CARTESIAN_POINT('Ctrl Pts',(25.5329266094991,-12.95204779512,69.5496905418731));
#147761=CARTESIAN_POINT('Ctrl Pts',(26.7219181594991,-12.33886835717,68.8939981611091));
#147762=CARTESIAN_POINT('Ctrl Pts',(28.0550484564891,-11.66205659809,68.32348737336));
#147763=CARTESIAN_POINT('Ctrl Pts',(29.5302626991891,-10.91639130965,67.842821810496));
#147764=CARTESIAN_POINT('Ctrl Pts',(30.7112123601191,-10.3172835446,67.571237827604));
#147765=CARTESIAN_POINT('Ctrl Pts',(31.3905930089891,-9.97074480891598,
67.457066442736));
#147766=CARTESIAN_POINT('Ctrl Pts',(31.5567731140791,-9.88587105497599,
67.431705971039));
#147767=CARTESIAN_POINT('Ctrl Pts',(27.4727097388691,-14.99894242272,74.370845864195));
#147768=CARTESIAN_POINT('Ctrl Pts',(27.4690374908891,-14.99927412475,74.362370216541));
#147769=CARTESIAN_POINT('Ctrl Pts',(27.4146355861491,-15.00404176909,74.231520094978));
#147770=CARTESIAN_POINT('Ctrl Pts',(27.3717438376491,-15.00325792021,73.9585721062895));
#147771=CARTESIAN_POINT('Ctrl Pts',(27.4972980083791,-14.97219965841,73.5156372957745));
#147772=CARTESIAN_POINT('Ctrl Pts',(27.8267501244891,-14.90490385564,73.0117077491551));
#147773=CARTESIAN_POINT('Ctrl Pts',(28.3632567205591,-14.79417301808,72.4487361234403));
#147774=CARTESIAN_POINT('Ctrl Pts',(29.0954791031191,-14.63302923949,71.833557915698));
#147775=CARTESIAN_POINT('Ctrl Pts',(30.0097285339691,-14.41300577028,71.171242909551));
#147776=CARTESIAN_POINT('Ctrl Pts',(31.1001512767791,-14.12091813026,70.4622944187711));
#147777=CARTESIAN_POINT('Ctrl Pts',(32.3671840294791,-13.73672387177,69.7064055545461));
#147778=CARTESIAN_POINT('Ctrl Pts',(33.8128240385791,-13.23052362994,68.90703904439));
#147779=CARTESIAN_POINT('Ctrl Pts',(35.0038717625891,-12.73614203142,68.297720297344));
#147780=CARTESIAN_POINT('Ctrl Pts',(35.7025055078291,-12.40446635354,67.961264321001));
#147781=CARTESIAN_POINT('Ctrl Pts',(35.8742286296091,-12.32012494619,67.879945375125));
#147782=CARTESIAN_POINT('',(28.2952879006395,-10.3188826735431,64.2104019363119));
#147783=CARTESIAN_POINT('',(26.0141520549875,-12.1870332282214,64.6126277311938));
#147784=CARTESIAN_POINT('Ctrl Pts',(28.2952879006395,-10.3188826735431,
64.2104019363119));
#147785=CARTESIAN_POINT('Ctrl Pts',(27.9287930576915,-10.6438766835605,
64.2750248654141));
#147786=CARTESIAN_POINT('Ctrl Pts',(27.5458477659422,-10.9632373020545,
64.3425484525577));
#147787=CARTESIAN_POINT('Ctrl Pts',(26.7888573507576,-11.5772327263092,
64.4760262868924));
#147788=CARTESIAN_POINT('Ctrl Pts',(26.3839963435794,-11.8964640257404,
64.5474142058218));
#147789=CARTESIAN_POINT('Ctrl Pts',(26.0141587646837,-12.1870420332971,
64.612626549461));
#147790=CARTESIAN_POINT('Ctrl Pts',(25.6004488369058,-11.2186736973405,
60.4750575395639));
#147791=CARTESIAN_POINT('Ctrl Pts',(25.6771414538508,-11.1557830040577,
60.6337815308351));
#147792=CARTESIAN_POINT('Ctrl Pts',(25.7584151174531,-11.0953949289909,
60.7932143542437));
#147793=CARTESIAN_POINT('Ctrl Pts',(25.844310928499,-11.037781455913,60.9529979077714));
#147794=CARTESIAN_POINT('Ctrl Pts',(25.9295618292542,-10.9806005478371,
61.1115817979316));
#147795=CARTESIAN_POINT('Ctrl Pts',(26.0193659247053,-10.9261530587674,
61.2705108944446));
#147796=CARTESIAN_POINT('Ctrl Pts',(26.113720684445,-10.8746965781389,61.4294088726265));
#147797=CARTESIAN_POINT('Ctrl Pts',(26.2086156080668,-10.8229455184938,
61.5892165129072));
#147798=CARTESIAN_POINT('Ctrl Pts',(26.3081136900117,-10.7742201760057,
61.7489923872755));
#147799=CARTESIAN_POINT('Ctrl Pts',(26.4121655715204,-10.7287689378137,
61.9083312146541));
#147800=CARTESIAN_POINT('Ctrl Pts',(26.5162174530291,-10.6833176996217,
62.0676700420328));
#147801=CARTESIAN_POINT('Ctrl Pts',(26.6248232672778,-10.6411409234484,
62.2265714462408));
#147802=CARTESIAN_POINT('Ctrl Pts',(26.7378842407237,-10.6024679594409,
62.3846128012655));
#147803=CARTESIAN_POINT('Ctrl Pts',(26.8508360347518,-10.5638323406955,
62.5425015407359));
#147804=CARTESIAN_POINT('Ctrl Pts',(26.9682348811087,-10.528693532743,62.6995312136569));
#147805=CARTESIAN_POINT('Ctrl Pts',(27.0899297391689,-10.4972591991273,
62.8552717178284));
#147806=CARTESIAN_POINT('Ctrl Pts',(27.2075046724398,-10.466889060765,63.005739697145));
#147807=CARTESIAN_POINT('Ctrl Pts',(27.3290893789845,-10.43997694453,63.1550038764423));
#147808=CARTESIAN_POINT('Ctrl Pts',(27.4545028264304,-10.416683963319,63.3026721539028));
#147809=CARTESIAN_POINT('Ctrl Pts',(27.5794141640008,-10.3934842387413,
63.4497492212345));
#147810=CARTESIAN_POINT('Ctrl Pts',(27.7081235256901,-10.373874942025,63.5952427264035));
#147811=CARTESIAN_POINT('Ctrl Pts',(27.8404094539594,-10.3579861278288,
63.7387672788158));
#147812=CARTESIAN_POINT('Ctrl Pts',(27.9721230978152,-10.342166050503,63.8816709272108));
#147813=CARTESIAN_POINT('Ctrl Pts',(28.1073822405416,-10.330034502476,64.022622210721));
#147814=CARTESIAN_POINT('Ctrl Pts',(28.2459282980801,-10.3216880682509,
64.1612488914306));
#147815=CARTESIAN_POINT('Ctrl Pts',(28.2623353354503,-10.3206996586153,
64.1776654764373));
#147816=CARTESIAN_POINT('Ctrl Pts',(28.2787884243379,-10.319764293024,64.1940494748701));
#147817=CARTESIAN_POINT('Ctrl Pts',(28.2952871000938,-10.3188821006174,
64.2104002803598));
#147818=CARTESIAN_POINT('Ctrl Pts',(26.0141520557349,-12.1870332282901,
64.6126277283268));
#147819=CARTESIAN_POINT('Ctrl Pts',(26.0012422809462,-12.1388602075693,
64.4661526914882));
#147820=CARTESIAN_POINT('Ctrl Pts',(25.9872836532194,-12.087933236017,64.3090583874833));
#147821=CARTESIAN_POINT('Ctrl Pts',(25.9645184990504,-12.0084297043005,
64.057478451471));
#147822=CARTESIAN_POINT('Ctrl Pts',(25.9566253013141,-11.9814136956279,
63.9709621319751));
#147823=CARTESIAN_POINT('Ctrl Pts',(25.944299540303,-11.9402823435069,63.8371998866629));
#147824=CARTESIAN_POINT('Ctrl Pts',(25.9380151379575,-11.9195652713876,
63.7693217847163));
#147825=CARTESIAN_POINT('Ctrl Pts',(25.9304640520936,-11.895171370767,63.6883847335085));
#147826=CARTESIAN_POINT('Ctrl Pts',(25.9263591770947,-11.8820491146581,
63.6445577240038));
#147827=CARTESIAN_POINT('Ctrl Pts',(25.9244272053296,-11.8759114862136,
63.6239777222435));
#147828=CARTESIAN_POINT('Ctrl Pts',(25.9233191909306,-11.8724010161351,
63.6121865158046));
#147829=CARTESIAN_POINT('Ctrl Pts',(25.9231709220948,-11.8719313157875,
63.6106087420972));
#147830=CARTESIAN_POINT('Ctrl Pts',(25.8707006041343,-11.7059929720678,
63.0526023350243));
#147831=CARTESIAN_POINT('Ctrl Pts',(25.8210422190118,-11.581613044566,62.5685125411034));
#147832=CARTESIAN_POINT('Ctrl Pts',(25.687446953851,-11.3093598897932,61.3232443887802));
#147833=CARTESIAN_POINT('Ctrl Pts',(25.6201332141581,-11.2608219841326,
60.7717569482344));
#147834=CARTESIAN_POINT('Ctrl Pts',(25.5859466416791,-11.24343482307,60.50136354202));
#147835=CARTESIAN_POINT('Ctrl Pts',(28.1799730489391,-14.15117801268,74.301595852087));
#147836=CARTESIAN_POINT('Ctrl Pts',(28.1735718783691,-14.15291478505,74.2652930097969));
#147837=CARTESIAN_POINT('Ctrl Pts',(28.1587242848691,-14.15609086467,74.181088122743));
#147838=CARTESIAN_POINT('Ctrl Pts',(28.1345641629891,-14.15802842506,74.044069262757));
#147839=CARTESIAN_POINT('Ctrl Pts',(28.1065660850191,-14.1557638184,73.8852842721588));
#147840=CARTESIAN_POINT('Ctrl Pts',(28.0757500096891,-14.14785693146,73.7105176244119));
#147841=CARTESIAN_POINT('Ctrl Pts',(28.0418954916191,-14.13302748591,73.5185191115803));
#147842=CARTESIAN_POINT('Ctrl Pts',(28.0048627881991,-14.11015935491,73.3084962139256));
#147843=CARTESIAN_POINT('Ctrl Pts',(27.9645715192991,-14.07834643848,73.0799930731187));
#147844=CARTESIAN_POINT('Ctrl Pts',(27.9208888531191,-14.036930053,72.8322563625702));
#147845=CARTESIAN_POINT('Ctrl Pts',(27.8735693541391,-13.98520775603,72.5638941483318));
#147846=CARTESIAN_POINT('Ctrl Pts',(27.8223275617791,-13.92248791285,72.2732875029045));
#147847=CARTESIAN_POINT('Ctrl Pts',(27.7669353440791,-13.84821962507,71.9591426257));
#147848=CARTESIAN_POINT('Ctrl Pts',(27.7071659871591,-13.76186996469,71.620173758449));
#147849=CARTESIAN_POINT('Ctrl Pts',(27.6427331848091,-13.66295161782,71.2547571778699));
#147850=CARTESIAN_POINT('Ctrl Pts',(27.5731736312291,-13.55077370827,70.860265346269));
#147851=CARTESIAN_POINT('Ctrl Pts',(27.4979482253291,-13.42445216333,70.433640869453));
#147852=CARTESIAN_POINT('Ctrl Pts',(27.4168343894691,-13.28392357974,69.97362144678));
#147853=CARTESIAN_POINT('Ctrl Pts',(27.3294747454891,-13.12902729583,69.478180286149));
#147854=CARTESIAN_POINT('Ctrl Pts',(27.2352897672591,-12.95931585803,68.944030731412));
#147855=CARTESIAN_POINT('Ctrl Pts',(27.1330543177591,-12.77375947438,68.36422468536));
#147856=CARTESIAN_POINT('Ctrl Pts',(27.0215516935991,-12.57148328781,67.731861880101));
#147857=CARTESIAN_POINT('Ctrl Pts',(26.8998844749991,-12.35307312972,67.041852795234));
#147858=CARTESIAN_POINT('Ctrl Pts',(26.7675133818891,-12.12114868892,66.2911390213841));
#147859=CARTESIAN_POINT('Ctrl Pts',(26.6238265063091,-11.87925312292,65.4762502561861));
#147860=CARTESIAN_POINT('Ctrl Pts',(26.4673150737591,-11.63288870712,64.588629814245));
#147861=CARTESIAN_POINT('Ctrl Pts',(26.2960779423591,-11.39104634332,63.617495784079));
#147862=CARTESIAN_POINT('Ctrl Pts',(26.1146351892191,-11.17902244978,62.5884827969));
#147863=CARTESIAN_POINT('Ctrl Pts',(25.9376619630691,-11.03545945137,61.5848177569));
#147864=CARTESIAN_POINT('Ctrl Pts',(25.8044546378291,-10.98673841047,60.8293614750201));
#147865=CARTESIAN_POINT('Ctrl Pts',(25.7335896270191,-10.98615918857,60.42746602756));
#147866=CARTESIAN_POINT('Ctrl Pts',(25.7147102194091,-10.98797446009,60.3203955863901));
#147867=CARTESIAN_POINT('Ctrl Pts',(27.1734273383791,-16.2916628133,74.5810090502221));
#147868=CARTESIAN_POINT('Ctrl Pts',(27.1646108851991,-16.29406243743,74.531008459631));
#147869=CARTESIAN_POINT('Ctrl Pts',(27.1440760525391,-16.29846019828,74.414549636477));
#147870=CARTESIAN_POINT('Ctrl Pts',(27.1104807962291,-16.30115793748,74.224021470152));
#147871=CARTESIAN_POINT('Ctrl Pts',(27.0715520564091,-16.29800450584,74.003245615733));
#147872=CARTESIAN_POINT('Ctrl Pts',(27.0290761160691,-16.28707212928,73.7623525874979));
#147873=CARTESIAN_POINT('Ctrl Pts',(26.9836467347891,-16.26711075281,73.5047097634025));
#147874=CARTESIAN_POINT('Ctrl Pts',(26.9353870206991,-16.23724121735,73.231015324247));
#147875=CARTESIAN_POINT('Ctrl Pts',(26.8847204870791,-16.19715982767,72.9436711332555));
#147876=CARTESIAN_POINT('Ctrl Pts',(26.8316423236691,-16.14677063562,72.6426499101076));
#147877=CARTESIAN_POINT('Ctrl Pts',(26.7758815320691,-16.08576509839,72.3264147464796));
#147878=CARTESIAN_POINT('Ctrl Pts',(26.7171808327491,-16.01386768581,71.9935065376213));
#147879=CARTESIAN_POINT('Ctrl Pts',(26.6552374104291,-15.93077840098,71.642207932743));
#147880=CARTESIAN_POINT('Ctrl Pts',(26.5897379537191,-15.83611958068,71.2707420546911));
#147881=CARTESIAN_POINT('Ctrl Pts',(26.5204490164191,-15.72972144342,70.877784964302));
#147882=CARTESIAN_POINT('Ctrl Pts',(26.4467441668391,-15.61084028714,70.45978399085));
#147883=CARTESIAN_POINT('Ctrl Pts',(26.3680895688091,-15.47874470736,70.0137115990481));
#147884=CARTESIAN_POINT('Ctrl Pts',(26.2843664547391,-15.33368482781,69.5388942243469));
#147885=CARTESIAN_POINT('Ctrl Pts',(26.1950217273191,-15.17526161349,69.032195096033));
#147886=CARTESIAN_POINT('Ctrl Pts',(26.0996654749091,-15.00343453373,68.491402915343));
#147887=CARTESIAN_POINT('Ctrl Pts',(25.9971340390191,-14.81733951027,67.9099182470231));
#147888=CARTESIAN_POINT('Ctrl Pts',(25.8861065416291,-14.61592784221,67.2802500196189));
#147889=CARTESIAN_POINT('Ctrl Pts',(25.7662123528591,-14.40070911901,66.600296286566));
#147890=CARTESIAN_POINT('Ctrl Pts',(25.6369459663191,-14.17424139564,65.867190178725));
#147891=CARTESIAN_POINT('Ctrl Pts',(25.4982315426691,-13.940759467,65.080501589758));
#147892=CARTESIAN_POINT('Ctrl Pts',(25.3495581035291,-13.70681104471,64.2373326172561));
#147893=CARTESIAN_POINT('Ctrl Pts',(25.1899312459191,-13.48155823901,63.3320437218209));
#147894=CARTESIAN_POINT('Ctrl Pts',(25.0263288417991,-13.29087482736,62.4042083816401));
#147895=CARTESIAN_POINT('Ctrl Pts',(24.8740404427791,-13.16819509687,61.54053795295));
#147896=CARTESIAN_POINT('Ctrl Pts',(24.7660208233591,-13.12950137129,60.9279282491701));
#147897=CARTESIAN_POINT('Ctrl Pts',(24.7113232798591,-13.12914167291,60.61772306514));
#147898=CARTESIAN_POINT('Ctrl Pts',(24.6969486285791,-13.13052501539,60.53620036667));
#147899=CARTESIAN_POINT('Ctrl Pts',(24.9455852428891,-15.52840338343,74.937490541193));
#147900=CARTESIAN_POINT('Ctrl Pts',(24.9376300372391,-15.53056664622,74.89237432799));
#147901=CARTESIAN_POINT('Ctrl Pts',(24.9191231745591,-15.53452877692,74.787416694133));
#147902=CARTESIAN_POINT('Ctrl Pts',(24.8888923221091,-15.53695544966,74.6159690102469));
#147903=CARTESIAN_POINT('Ctrl Pts',(24.8538612650591,-15.53411895745,74.417298013271));
#147904=CARTESIAN_POINT('Ctrl Pts',(24.8155430285791,-15.52426541755,74.1999844953681));
#147905=CARTESIAN_POINT('Ctrl Pts',(24.7742410410091,-15.50613399786,73.9657492841528));
#147906=CARTESIAN_POINT('Ctrl Pts',(24.7299846824891,-15.47876104073,73.7147590026961));
#147907=CARTESIAN_POINT('Ctrl Pts',(24.6830177867491,-15.44162804395,73.4483965007143));
#147908=CARTESIAN_POINT('Ctrl Pts',(24.6332898932691,-15.39443839773,73.1663756024908));
#147909=CARTESIAN_POINT('Ctrl Pts',(24.5805391189291,-15.33674310157,72.8672110950277));
#147910=CARTESIAN_POINT('Ctrl Pts',(24.5244981353291,-15.26811824966,72.5493868835785));
#147911=CARTESIAN_POINT('Ctrl Pts',(24.4648907579491,-15.18817437804,72.2113366479453));
#147912=CARTESIAN_POINT('Ctrl Pts',(24.4014345545691,-15.0964784588,71.851458635375));
#147913=CARTESIAN_POINT('Ctrl Pts',(24.3338772300291,-14.99274748392,71.468322008935));
#147914=CARTESIAN_POINT('Ctrl Pts',(24.2616505204791,-14.87625658814,71.05870398415));
#147915=CARTESIAN_POINT('Ctrl Pts',(24.1842187123691,-14.74621992816,70.61956637857));
#147916=CARTESIAN_POINT('Ctrl Pts',(24.1014260212591,-14.60277582948,70.150025694656));
#147917=CARTESIAN_POINT('Ctrl Pts',(24.0127891398591,-14.44561025683,69.647340960648));
#147918=CARTESIAN_POINT('Ctrl Pts',(23.9178505433291,-14.27453757798,69.108917424153));
#147919=CARTESIAN_POINT('Ctrl Pts',(23.8154246510091,-14.08863462405,68.5280313231649));
#147920=CARTESIAN_POINT('Ctrl Pts',(23.7042277317191,-13.88691468382,67.897402256442));
#147921=CARTESIAN_POINT('Ctrl Pts',(23.5837013115391,-13.67055795077,67.213862960861));
#147922=CARTESIAN_POINT('Ctrl Pts',(23.4533278409591,-13.44214445744,66.4744782673861));
#147923=CARTESIAN_POINT('Ctrl Pts',(23.3128403279491,-13.20566237292,65.677733988967));
#147924=CARTESIAN_POINT('Ctrl Pts',(23.1613719974891,-12.96728662458,64.818714400188));
#147925=CARTESIAN_POINT('Ctrl Pts',(22.9976051193791,-12.73611827271,63.889946281738));
#147926=CARTESIAN_POINT('Ctrl Pts',(22.8276411589291,-12.53782521859,62.9260327628401));
#147927=CARTESIAN_POINT('Ctrl Pts',(22.6665505824491,-12.40769888014,62.0124427051201));
#147928=CARTESIAN_POINT('Ctrl Pts',(22.5495494678191,-12.36542958935,61.34889641084));
#147929=CARTESIAN_POINT('Ctrl Pts',(22.4890868883391,-12.36499161272,61.00599608308));
#147930=CARTESIAN_POINT('Ctrl Pts',(22.4731059197691,-12.36652897355,60.91536350656));
#147931=CARTESIAN_POINT('Ctrl Pts',(25.3958369987791,-13.19733209216,74.747091056725));
#147932=CARTESIAN_POINT('Ctrl Pts',(25.3905121299191,-13.19877348358,74.716892224767));
#147933=CARTESIAN_POINT('Ctrl Pts',(25.3781988921391,-13.20140515586,74.6470603831829));
#147934=CARTESIAN_POINT('Ctrl Pts',(25.3582432684491,-13.20300396427,74.533886417376));
#147935=CARTESIAN_POINT('Ctrl Pts',(25.3351161277591,-13.20113543707,74.40272588482));
#147936=CARTESIAN_POINT('Ctrl Pts',(25.3094959382791,-13.19457677317,74.25742657001));
#147937=CARTESIAN_POINT('Ctrl Pts',(25.2807994274291,-13.18203422608,74.0946805697331));
#147938=CARTESIAN_POINT('Ctrl Pts',(25.2487697206791,-13.16228607101,73.9130310761299));
#147939=CARTESIAN_POINT('Ctrl Pts',(25.2131018921891,-13.13415776355,73.7107487688747));
#147940=CARTESIAN_POINT('Ctrl Pts',(25.1736060610091,-13.09673985306,73.4867567795944));
#147941=CARTESIAN_POINT('Ctrl Pts',(25.1300481830191,-13.04915436699,73.2397277780308));
#147942=CARTESIAN_POINT('Ctrl Pts',(25.0821302395191,-12.99052424551,72.9679716162406));
#147943=CARTESIAN_POINT('Ctrl Pts',(25.0296573790591,-12.92018678314,72.6703832366873));
#147944=CARTESIAN_POINT('Ctrl Pts',(24.9724414774691,-12.83753986258,72.345895734205));
#147945=CARTESIAN_POINT('Ctrl Pts',(24.9101726729691,-12.74195467067,71.9927517952847));
#147946=CARTESIAN_POINT('Ctrl Pts',(24.8424603521591,-12.63276387159,71.6087361413429));
#147947=CARTESIAN_POINT('Ctrl Pts',(24.7687630678091,-12.50901536037,71.190778072421));
#147948=CARTESIAN_POINT('Ctrl Pts',(24.6888119822491,-12.37050601941,70.737352934449));
#147949=CARTESIAN_POINT('Ctrl Pts',(24.6023369340291,-12.21718141131,70.246928565596));
#147950=CARTESIAN_POINT('Ctrl Pts',(24.5086739006791,-12.04841274893,69.715739107405));
#147951=CARTESIAN_POINT('Ctrl Pts',(24.4065703490691,-11.86309639472,69.1366810914259));
#147952=CARTESIAN_POINT('Ctrl Pts',(24.2948559982191,-11.66043496018,68.503117524501));
#147953=CARTESIAN_POINT('Ctrl Pts',(24.1723986795191,-11.44060263028,67.8086275592741));
#147954=CARTESIAN_POINT('Ctrl Pts',(24.0386440625791,-11.20624655919,67.0500674319299));
#147955=CARTESIAN_POINT('Ctrl Pts',(23.8927413558091,-10.96060169599,66.222612063574));
#147956=CARTESIAN_POINT('Ctrl Pts',(23.7327371453591,-10.70870444727,65.315183093782));
#147957=CARTESIAN_POINT('Ctrl Pts',(23.5563262270191,-10.45946942069,64.314707059819));
#147958=CARTESIAN_POINT('Ctrl Pts',(23.3669334318491,-10.23793575087,63.240607143819));
#147959=CARTESIAN_POINT('Ctrl Pts',(23.1789601174791,-10.08506672053,62.1745575034399));
#147960=CARTESIAN_POINT('Ctrl Pts',(23.0345286104791,-10.03187729293,61.35544572364));
#147961=CARTESIAN_POINT('Ctrl Pts',(22.9564590295991,-10.03120024663,60.9126911289));
#147962=CARTESIAN_POINT('Ctrl Pts',(22.9355722059791,-10.033207995,60.79423606582));
#147963=CARTESIAN_POINT('Ctrl Pts',(23.651525801475,-10.9473150473928,65.0292224863858));
#147964=CARTESIAN_POINT('Ctrl Pts',(23.6515257621658,-11.1312070918152,
65.0292224933171));
#147965=CARTESIAN_POINT('Ctrl Pts',(23.6828327230095,-11.3139663116835,
65.0237022314369));
#147966=CARTESIAN_POINT('Ctrl Pts',(23.807271208638,-11.6646282261749,65.0017603689821));
#147967=CARTESIAN_POINT('Ctrl Pts',(23.9012088684855,-11.8295758620756,
64.9851966250261));
#147968=CARTESIAN_POINT('Ctrl Pts',(24.1432300222825,-12.1167462245558,
64.9425217657095));
#147969=CARTESIAN_POINT('Ctrl Pts',(24.2894314553903,-12.2364947812159,
64.9167425084553));
#147970=CARTESIAN_POINT('Ctrl Pts',(24.6217353068813,-12.4156530859415,
64.8581483736441));
#147971=CARTESIAN_POINT('Ctrl Pts',(24.80507951085,-12.4718672970602,64.8258198437246));
#147972=CARTESIAN_POINT('Ctrl Pts',(25.1736178642303,-12.5072619289281,
64.7608365885978));
#147973=CARTESIAN_POINT('Ctrl Pts',(25.3543120349207,-12.4898627065513,
64.7289753310509));
#147974=CARTESIAN_POINT('Ctrl Pts',(25.7039070130317,-12.3869706731887,
64.6673323040898));
#147975=CARTESIAN_POINT('Ctrl Pts',(25.8687813243819,-12.3012676530536,
64.6382605145725));
#147976=CARTESIAN_POINT('Ctrl Pts',(26.0141453440937,-12.1870244234308,
64.6126289158731));
#147977=CARTESIAN_POINT('Ctrl Pts',(25.3886736533591,-11.44208510792,60.2115109699));
#147978=CARTESIAN_POINT('Ctrl Pts',(25.5981770475491,-11.17175375805,60.22632667139));
#147979=CARTESIAN_POINT('Ctrl Pts',(25.8078177068491,-10.88204468039,60.24561988886));
#147980=CARTESIAN_POINT('Ctrl Pts',(26.0168787184791,-10.57129328633,60.270855635));
#147981=CARTESIAN_POINT('Ctrl Pts',(27.3087836696091,-9.624602273718,64.44463626086));
#147982=CARTESIAN_POINT('Ctrl Pts',(27.5425179224791,-9.479512324536,64.50183542974));
#147983=CARTESIAN_POINT('Ctrl Pts',(27.7759878147791,-9.32787789472698,
64.56281239081));
#147984=CARTESIAN_POINT('Ctrl Pts',(28.0092438744591,-9.16583693103399,
64.625382279757));
#147985=CARTESIAN_POINT('Ctrl Pts',(31.2407814247091,-10.04443147536,67.489770329979));
#147986=CARTESIAN_POINT('Ctrl Pts',(31.5318184331991,-9.93037722233698,
67.468249475135));
#147987=CARTESIAN_POINT('Ctrl Pts',(31.8153253258691,-9.81435677539199,
67.4542319002));
#147988=CARTESIAN_POINT('Ctrl Pts',(32.0927104552091,-9.69360679656099,
67.4456953393931));
#147989=CARTESIAN_POINT('Ctrl Pts',(35.5328635075091,-12.52520554518,68.067674694392));
#147990=CARTESIAN_POINT('Ctrl Pts',(35.8902027012991,-12.3349434155,67.879400029176));
#147991=CARTESIAN_POINT('Ctrl Pts',(36.2289341849091,-12.1371151135,67.705214293035));
#147992=CARTESIAN_POINT('Ctrl Pts',(36.5518441070791,-11.93289063421,67.547001987805));
#147993=CARTESIAN_POINT('Ctrl Pts',(28.7123816359948,-9.91606170434255,
64.1368570572843));
#147994=CARTESIAN_POINT('Ctrl Pts',(28.6457638811355,-9.98626732421584,
64.1486035648602));
#147995=CARTESIAN_POINT('Ctrl Pts',(28.5777184993322,-10.0548652908716,
64.1606018015785));
#147996=CARTESIAN_POINT('Ctrl Pts',(28.4385393129266,-10.1892126190695,
64.1851428472949));
#147997=CARTESIAN_POINT('Ctrl Pts',(28.3676165512144,-10.2547579475351,
64.1976484437373));
#147998=CARTESIAN_POINT('Ctrl Pts',(28.295281579335,-10.3188753218672,64.2104030509284));
#147999=CARTESIAN_POINT('Ctrl Pts',(36.2511910984291,-0.816951121684487,
99.13095237507));
#148000=CARTESIAN_POINT('Ctrl Pts',(36.2200982088991,-1.45683196280799,
99.1098451401801));
#148001=CARTESIAN_POINT('Ctrl Pts',(36.0778630790891,-2.85039942836099,
99.0419676728901));
#148002=CARTESIAN_POINT('Ctrl Pts',(35.6275483510391,-4.94247000735899,
98.84599903898));
#148003=CARTESIAN_POINT('Ctrl Pts',(34.9397597871691,-7.05113172994599,
98.51977184372));
#148004=CARTESIAN_POINT('Ctrl Pts',(34.0734741662491,-9.09163743804897,
98.0649602571899));
#148005=CARTESIAN_POINT('Ctrl Pts',(33.0099168483791,-11.12983443612,97.44906592845));
#148006=CARTESIAN_POINT('Ctrl Pts',(31.7699785170891,-13.12298748389,96.6589115129399));
#148007=CARTESIAN_POINT('Ctrl Pts',(30.4746258290591,-14.92251334854,95.75721789378));
#148008=CARTESIAN_POINT('Ctrl Pts',(29.1968815731991,-16.50069944243,94.7947864407199));
#148009=CARTESIAN_POINT('Ctrl Pts',(27.9225293421991,-17.92619343051,93.76208048801));
#148010=CARTESIAN_POINT('Ctrl Pts',(26.5896727465691,-19.28349187111,92.5956876894801));
#148011=CARTESIAN_POINT('Ctrl Pts',(25.1814694175691,-20.58838494568,91.25117303266));
#148012=CARTESIAN_POINT('Ctrl Pts',(23.7249591534991,-21.81419974781,89.71266771848));
#148013=CARTESIAN_POINT('Ctrl Pts',(22.2142909846591,-22.9637208008,87.91364117654));
#148014=CARTESIAN_POINT('Ctrl Pts',(20.6065395382091,-24.05476593901,85.68623624305));
#148015=CARTESIAN_POINT('Ctrl Pts',(18.9416778012191,-25.02348229969,82.825890425796));
#148016=CARTESIAN_POINT('Ctrl Pts',(17.5339994345191,-25.65356630387,79.417420667109));
#148017=CARTESIAN_POINT('Ctrl Pts',(16.9242179391691,-25.78353110717,76.926255793732));
#148018=CARTESIAN_POINT('Ctrl Pts',(16.7312453442491,-25.77964745785,75.805602355198));
#148019=CARTESIAN_POINT('Ctrl Pts',(34.9680768531591,-0.377262712455286,
92.83793248162));
#148020=CARTESIAN_POINT('Ctrl Pts',(34.9401900659091,-0.768818210978587,
92.83356221903));
#148021=CARTESIAN_POINT('Ctrl Pts',(34.8109275223991,-1.62812620872499,
92.8325719567701));
#148022=CARTESIAN_POINT('Ctrl Pts',(34.3972755661991,-2.97122279462399,
92.8255990532501));
#148023=CARTESIAN_POINT('Ctrl Pts',(33.7599966114291,-4.39375486831299,
92.76261787049));
#148024=CARTESIAN_POINT('Ctrl Pts',(32.9521573659891,-5.82931930270299,
92.61621541888));
#148025=CARTESIAN_POINT('Ctrl Pts',(31.9551618598791,-7.31697565127499,
92.35621163472));
#148026=CARTESIAN_POINT('Ctrl Pts',(30.7878189799691,-8.81951599642399,
91.9596113594201));
#148027=CARTESIAN_POINT('Ctrl Pts',(29.5643467643691,-10.21287137887,91.45281600972));
#148028=CARTESIAN_POINT('Ctrl Pts',(28.3547145027491,-11.46125770319,90.86912642514));
#148029=CARTESIAN_POINT('Ctrl Pts',(27.1462246720591,-12.60932492795,90.2068010813201));
#148030=CARTESIAN_POINT('Ctrl Pts',(25.8804633212691,-13.72121825748,89.42218714027));
#148031=CARTESIAN_POINT('Ctrl Pts',(24.5415426038291,-14.80846467629,88.4770655865801));
#148032=CARTESIAN_POINT('Ctrl Pts',(23.1553900553591,-15.84725088264,87.34998754959));
#148033=CARTESIAN_POINT('Ctrl Pts',(21.7169286490991,-16.83785256507,85.9795861337301));
#148034=CARTESIAN_POINT('Ctrl Pts',(20.1864646779891,-17.79411649535,84.2176273015201));
#148035=CARTESIAN_POINT('Ctrl Pts',(18.6056376920291,-18.65837811088,81.868380902977));
#148036=CARTESIAN_POINT('Ctrl Pts',(17.2833457609491,-19.22934869733,78.9739891356611));
#148037=CARTESIAN_POINT('Ctrl Pts',(16.7318898964791,-19.34793907064,76.820460370021));
#148038=CARTESIAN_POINT('Ctrl Pts',(16.5654152065891,-19.34439445674,75.849914932886));
#148039=CARTESIAN_POINT('Ctrl Pts',(38.6686947048191,-0.267618408180286,
87.57152762521));
#148040=CARTESIAN_POINT('Ctrl Pts',(38.6331457099391,-0.640502714598286,
87.56228047755));
#148041=CARTESIAN_POINT('Ctrl Pts',(38.4681697649291,-1.45257130791499,
87.5371031361401));
#148042=CARTESIAN_POINT('Ctrl Pts',(37.9543196144491,-2.67152049410099,
87.46697907679));
#148043=CARTESIAN_POINT('Ctrl Pts',(37.1964789572891,-3.89993484531899,
87.33954011223));
#148044=CARTESIAN_POINT('Ctrl Pts',(36.2722354399091,-5.08847143352099,
87.1482156939501));
#148045=CARTESIAN_POINT('Ctrl Pts',(35.1711071623791,-6.27550574943099,
86.8740206795701));
#148046=CARTESIAN_POINT('Ctrl Pts',(33.9234036585391,-7.436166673543,86.50611895787));
#148047=CARTESIAN_POINT('Ctrl Pts',(32.6526782149891,-8.48396598041999,
86.07171874038));
#148048=CARTESIAN_POINT('Ctrl Pts',(31.4266015655591,-9.40280963542199,
85.5959755830301));
#148049=CARTESIAN_POINT('Ctrl Pts',(30.2282183070691,-10.23269364386,85.07485106796));
#148050=CARTESIAN_POINT('Ctrl Pts',(29.0009821455491,-11.02282107056,84.4750277186701));
#148051=CARTESIAN_POINT('Ctrl Pts',(27.7349646372491,-11.7823880216,83.77066674245));
#148052=CARTESIAN_POINT('Ctrl Pts',(26.4611997445191,-12.49587308951,82.949856613029));
#148053=CARTESIAN_POINT('Ctrl Pts',(25.1820693516891,-13.16490311603,81.9728674396441));
#148054=CARTESIAN_POINT('Ctrl Pts',(23.8728795301391,-13.79985263807,80.741966022882));
#148055=CARTESIAN_POINT('Ctrl Pts',(22.5850112147791,-14.36356654138,79.133191069062));
#148056=CARTESIAN_POINT('Ctrl Pts',(21.5697113092491,-14.73019815096,77.183930116823));
#148057=CARTESIAN_POINT('Ctrl Pts',(21.1758003549191,-14.80581932552,75.7409655371681));
#148058=CARTESIAN_POINT('Ctrl Pts',(21.0646250899491,-14.8035595922,75.088550558094));
#148059=CARTESIAN_POINT('Ctrl Pts',(45.0312706731691,-0.556809233210386,
86.63588923546));
#148060=CARTESIAN_POINT('Ctrl Pts',(44.9819984429591,-1.15239083593299,
86.6032111113799));
#148061=CARTESIAN_POINT('Ctrl Pts',(44.7550297579291,-2.43387817146999,
86.47794742155));
#148062=CARTESIAN_POINT('Ctrl Pts',(44.0669849657891,-4.23139684260399,
86.1321464635101));
#148063=CARTESIAN_POINT('Ctrl Pts',(43.0931519133991,-5.87949518942999,
85.65298684557));
#148064=CARTESIAN_POINT('Ctrl Pts',(41.9506857162891,-7.33390305288999,
85.0915934778799));
#148065=CARTESIAN_POINT('Ctrl Pts',(40.6400631633491,-8.65884473130499,
84.44202906066));
#148066=CARTESIAN_POINT('Ctrl Pts',(39.2094613534091,-9.84085525044999,
83.71996478425));
#148067=CARTESIAN_POINT('Ctrl Pts',(37.8019957376891,-10.82051536224,82.99003573172));
#148068=CARTESIAN_POINT('Ctrl Pts',(36.4852355554891,-11.6168290835,82.283717786993));
#148069=CARTESIAN_POINT('Ctrl Pts',(35.2348621603691,-12.28740211764,81.586024678646));
#148070=CARTESIAN_POINT('Ctrl Pts',(33.9934103628291,-12.88127932846,80.858065721516));
#148071=CARTESIAN_POINT('Ctrl Pts',(32.7581770629291,-13.40872065919,80.08477919832));
#148072=CARTESIAN_POINT('Ctrl Pts',(31.5683175582891,-13.86272653758,79.272924596943));
#148073=CARTESIAN_POINT('Ctrl Pts',(30.4356778789491,-14.24928723071,78.407307267481));
#148074=CARTESIAN_POINT('Ctrl Pts',(29.3529211006491,-14.57798235441,77.439888248051));
#148075=CARTESIAN_POINT('Ctrl Pts',(28.3831326036191,-14.83361972799,76.336383711929));
#148076=CARTESIAN_POINT('Ctrl Pts',(27.7038229907891,-14.97888942575,75.170329705841));
#148077=CARTESIAN_POINT('Ctrl Pts',(27.4678322792991,-15.00690558171,74.365048202755));
#148078=CARTESIAN_POINT('Ctrl Pts',(27.4060630052191,-15.00607043787,73.999190543978));
#148079=CARTESIAN_POINT('',(39.4126085609146,-0.605361527076818,89.303184116066));
#148080=CARTESIAN_POINT('Origin',(46.4982593122882,-1.66437591746992,96.9778062066542));
#148081=CARTESIAN_POINT('Ctrl Pts',(39.4126085609146,-0.605361527076818,
89.303184116066));
#148082=CARTESIAN_POINT('Ctrl Pts',(39.4099252318568,-0.683444947045363,
89.2948644632298));
#148083=CARTESIAN_POINT('Ctrl Pts',(39.4065580192006,-0.766708479631635,
89.2850814479826));
#148084=CARTESIAN_POINT('Ctrl Pts',(39.4024210385378,-0.855040525558286,
89.2733819496395));
#148085=CARTESIAN_POINT('Ctrl Pts',(39.398394517039,-0.941014067848123,
89.2619948329367));
#148086=CARTESIAN_POINT('Ctrl Pts',(39.3936386153616,-1.03178968344965,
89.2487913177301));
#148087=CARTESIAN_POINT('Ctrl Pts',(39.3880680095067,-1.12722013107941,
89.2333348457709));
#148088=CARTESIAN_POINT('Ctrl Pts',(39.3827970165748,-1.21751788827826,
89.2187096942936));
#148089=CARTESIAN_POINT('Ctrl Pts',(39.376796440701,-1.31198352671711,89.2020666380893));
#148090=CARTESIAN_POINT('Ctrl Pts',(39.3699907959889,-1.41044597584285,
89.18303073602));
#148091=CARTESIAN_POINT('Ctrl Pts',(39.3680156935601,-1.43902128804925,
89.1775062254112));
#148092=CARTESIAN_POINT('Ctrl Pts',(39.3659727708971,-1.46793290362972,
89.1717801833692));
#148093=CARTESIAN_POINT('Ctrl Pts',(39.3638601573462,-1.49717579541164,
89.165843500559));
#148094=CARTESIAN_POINT('Ctrl Pts',(39.3570424034594,-1.59154745132835,
89.1466848417087));
#148095=CARTESIAN_POINT('Ctrl Pts',(39.349498818428,-1.68937304753144,89.1253315940075));
#148096=CARTESIAN_POINT('Ctrl Pts',(39.3411664250101,-1.79045253825546,
89.1014834303828));
#148097=CARTESIAN_POINT('Ctrl Pts',(39.3332784622089,-1.88614068244171,
89.0789072727156));
#148098=CARTESIAN_POINT('Ctrl Pts',(39.3246835089933,-1.98474496992307,
89.0540948478411));
#148099=CARTESIAN_POINT('Ctrl Pts',(39.3153290594718,-2.08605049367797,
89.02680462528));
#148100=CARTESIAN_POINT('Ctrl Pts',(39.3125220352183,-2.1164496167415,89.0186155472978));
#148101=CARTESIAN_POINT('Ctrl Pts',(39.3096466338812,-2.14709164187481,
89.0102034744062));
#148102=CARTESIAN_POINT('Ctrl Pts',(39.3067014714057,-2.17796988374068,
89.0015622132242));
#148103=CARTESIAN_POINT('Ctrl Pts',(39.2953949077397,-2.29651234462463,
88.9683881623794));
#148104=CARTESIAN_POINT('Ctrl Pts',(39.2830597414625,-2.41853715928627,
88.931832687132));
#148105=CARTESIAN_POINT('Ctrl Pts',(39.2696208587223,-2.5438092321937,88.8915720104783));
#148106=CARTESIAN_POINT('Ctrl Pts',(39.2573429243572,-2.65825939287037,
88.8547893437193));
#148107=CARTESIAN_POINT('Ctrl Pts',(39.2441436631701,-2.77541978677909,
88.8149137769909));
#148108=CARTESIAN_POINT('Ctrl Pts',(39.2299712767101,-2.89509818012012,
88.771739172233));
#148109=CARTESIAN_POINT('Ctrl Pts',(39.2163617007677,-3.01002393291677,
88.730279107346));
#148110=CARTESIAN_POINT('Ctrl Pts',(39.2018546701449,-3.12727157407915,
88.6857764236995));
#148111=CARTESIAN_POINT('Ctrl Pts',(39.1864107197701,-3.24666035753036,
88.6380926390761));
#148112=CARTESIAN_POINT('Ctrl Pts',(39.1718165907419,-3.3594796341998,88.593032710207));
#148113=CARTESIAN_POINT('Ctrl Pts',(39.1563857726419,-3.47421079212239,
88.5451319765576));
#148114=CARTESIAN_POINT('Ctrl Pts',(39.1400916515551,-3.59069318020269,
88.4943174196277));
#148115=CARTESIAN_POINT('Ctrl Pts',(39.1242484391298,-3.7039521408009,88.4449090584498));
#148116=CARTESIAN_POINT('Ctrl Pts',(39.1075889810899,-3.81886668350723,
88.3927456112529));
#148117=CARTESIAN_POINT('Ctrl Pts',(39.0900961118598,-3.93528238987657,
88.3378061841039));
#148118=CARTESIAN_POINT('Ctrl Pts',(39.0698623223758,-4.06993902420666,
88.2742584156573));
#148119=CARTESIAN_POINT('Ctrl Pts',(39.0485138104168,-4.20660231927269,
88.2069983091697));
#148120=CARTESIAN_POINT('Ctrl Pts',(39.0260063500057,-4.34510209183181,
88.1359004735261));
#148121=CARTESIAN_POINT('Ctrl Pts',(39.0038129707741,-4.48166916424905,
88.0657947752304));
#148122=CARTESIAN_POINT('Ctrl Pts',(38.9804926658221,-4.62002153013926,
87.9919572692072));
#148123=CARTESIAN_POINT('Ctrl Pts',(38.956010639519,-4.76001118441306,87.9143169217427));
#148124=CARTESIAN_POINT('Ctrl Pts',(38.9329641196511,-4.89179252916653,
87.8412290250045));
#148125=CARTESIAN_POINT('Ctrl Pts',(38.9088880990889,-5.02502466824429,
87.7647711919074));
#148126=CARTESIAN_POINT('Ctrl Pts',(38.8837610666994,-5.15960032747597,
87.6849303671281));
#148127=CARTESIAN_POINT('Ctrl Pts',(38.8821959706719,-5.16798268741426,
87.6799572944723));
#148128=CARTESIAN_POINT('Ctrl Pts',(38.8806267996404,-5.17637026567736,
87.6749711124725));
#148129=CARTESIAN_POINT('Ctrl Pts',(38.8790535494728,-5.18476303873876,
87.669971824328));
#148130=CARTESIAN_POINT('Ctrl Pts',(38.8667928540052,-5.25016982321366,
87.6310112376653));
#148131=CARTESIAN_POINT('Ctrl Pts',(38.8542843732491,-5.31589201516666,
87.5912544160014));
#148132=CARTESIAN_POINT('Ctrl Pts',(38.8415264249196,-5.38191912340202,
87.5507045284967));
#148133=CARTESIAN_POINT('Ctrl Pts',(38.8351474507548,-5.4149326775197,87.5304295847443));
#148134=CARTESIAN_POINT('Ctrl Pts',(38.8287061320204,-5.4480224845055,87.5099564060667));
#148135=CARTESIAN_POINT('Ctrl Pts',(38.8222022899081,-5.4811873405972,87.4892856894754));
#148136=CARTESIAN_POINT('Ctrl Pts',(38.8189503688519,-5.49776976864305,
87.4789503311798));
#148137=CARTESIAN_POINT('Ctrl Pts',(38.8156828184417,-5.51437096051822,
87.4685655904894));
#148138=CARTESIAN_POINT('Ctrl Pts',(38.8123996220168,-5.53099077426008,
87.4581315703589));
#148139=CARTESIAN_POINT('Ctrl Pts',(38.8107580238043,-5.53930068113101,
87.4529145602937));
#148140=CARTESIAN_POINT('Ctrl Pts',(38.8091125141816,-5.54761524357118,
87.4476852305022));
#148141=CARTESIAN_POINT('Ctrl Pts',(38.8074630912624,-5.55593444431467,
87.4424435950278));
#148142=CARTESIAN_POINT('Ctrl Pts',(38.8066383798028,-5.56009404468641,
87.4398227772906));
#148143=CARTESIAN_POINT('Ctrl Pts',(38.805812690025,-5.5642548046405,87.4371988831411));
#148144=CARTESIAN_POINT('Ctrl Pts',(38.8049860217041,-5.5684167220486,87.4345719144101));
#148145=CARTESIAN_POINT('Ctrl Pts',(38.8041593533833,-5.5725786394567,87.4319449456791));
#148146=CARTESIAN_POINT('Ctrl Pts',(38.8035398266194,-5.57569581376081,
87.429976243687));
#148147=CARTESIAN_POINT('Ctrl Pts',(38.8025030809044,-5.58090594453013,
87.4266817863445));
#148148=CARTESIAN_POINT('Ctrl Pts',(38.7941338525687,-5.62296522043224,
87.4000869662815));
#148149=CARTESIAN_POINT('Ctrl Pts',(38.785795322314,-5.66453645375523,87.3735549895261));
#148150=CARTESIAN_POINT('Ctrl Pts',(38.7774907818068,-5.70562997173392,
87.3471006541145));
#148151=CARTESIAN_POINT('Ctrl Pts',(38.7517807423839,-5.83285145573393,
87.2652006374005));
#148152=CARTESIAN_POINT('Ctrl Pts',(38.7263971118217,-5.95549632462261,
87.1840477757184));
#148153=CARTESIAN_POINT('Ctrl Pts',(38.7014116402201,-6.07382542997955,
87.1039392551767));
#148154=CARTESIAN_POINT('Ctrl Pts',(38.6759210529494,-6.19454672093023,
87.0222112307251));
#148155=CARTESIAN_POINT('Ctrl Pts',(38.6508448633532,-6.31077597806947,
86.9415700268134));
#148156=CARTESIAN_POINT('Ctrl Pts',(38.6262499273492,-6.42276010232269,
86.8622868002747));
#148157=CARTESIAN_POINT('Ctrl Pts',(38.600834152501,-6.53848161865936,86.7803575513182));
#148158=CARTESIAN_POINT('Ctrl Pts',(38.5759322826389,-6.64966995204747,
86.6998783321325));
#148159=CARTESIAN_POINT('Ctrl Pts',(38.5516084311598,-6.75656543709959,
86.6211034109643));
#148160=CARTESIAN_POINT('Ctrl Pts',(38.5267820277867,-6.86566947569938,
86.5407009315176));
#148161=CARTESIAN_POINT('Ctrl Pts',(38.5025577418917,-6.97030138917467,
86.4620736868377));
#148162=CARTESIAN_POINT('Ctrl Pts',(38.4789941794526,-7.07068405749413,
86.3854485627193));
#148163=CARTESIAN_POINT('Ctrl Pts',(38.4546485284467,-7.17439848591595,
86.3062802054348));
#148164=CARTESIAN_POINT('Ctrl Pts',(38.431008169128,-7.27357690004313,86.2292489218633));
#148165=CARTESIAN_POINT('Ctrl Pts',(38.4081280055139,-7.36843108572141,
86.1545617683574));
#148166=CARTESIAN_POINT('Ctrl Pts',(38.3990610478215,-7.40601992918434,
86.1249647220937));
#148167=CARTESIAN_POINT('Ctrl Pts',(38.3901133666663,-7.4429293396309,86.0957353418035));
#148168=CARTESIAN_POINT('Ctrl Pts',(38.3812879877655,-7.47917110582456,
86.0668848138656));
#148169=CARTESIAN_POINT('Ctrl Pts',(38.3558773358293,-7.58352094923186,
85.983816343735));
#148170=CARTESIAN_POINT('Ctrl Pts',(38.3314812804312,-7.68233842547393,
85.9038911148172));
#148171=CARTESIAN_POINT('Ctrl Pts',(38.3081575920777,-7.7758529635305,85.8273073700796));
#148172=CARTESIAN_POINT('Ctrl Pts',(38.284046918763,-7.87252285737706,85.7481395462523));
#148173=CARTESIAN_POINT('Ctrl Pts',(38.2610821761243,-7.96352586312083,
85.6725423438921));
#148174=CARTESIAN_POINT('Ctrl Pts',(38.23931671923,-8.04907660758938,85.6006963800654));
#148175=CARTESIAN_POINT('Ctrl Pts',(38.2333882777533,-8.07237878701643,
85.5811270875876));
#148176=CARTESIAN_POINT('Ctrl Pts',(38.2275487544219,-8.09527625006559,
85.5618358942794));
#148177=CARTESIAN_POINT('Ctrl Pts',(38.2217991031176,-8.11777286689644,
85.5428260041036));
#148178=CARTESIAN_POINT('Ctrl Pts',(38.2114933540447,-8.15809609273672,
85.5087524320407));
#148179=CARTESIAN_POINT('Ctrl Pts',(38.2014763692145,-8.19713161021553,
85.4755827144277));
#148180=CARTESIAN_POINT('Ctrl Pts',(38.1917532454106,-8.23490019381938,
85.4433338928739));
#148181=CARTESIAN_POINT('Ctrl Pts',(38.1868916835087,-8.25378448562131,
85.4272094820971));
#148182=CARTESIAN_POINT('Ctrl Pts',(38.1821035743238,-8.27235201668672,
85.4113152672317));
#148183=CARTESIAN_POINT('Ctrl Pts',(38.1773895147866,-8.29060520596237,
85.3956532183678));
#148184=CARTESIAN_POINT('Ctrl Pts',(38.1750324850179,-8.29973180060019,
85.3878221939358));
#148185=CARTESIAN_POINT('Ctrl Pts',(38.1726939669064,-8.30877980817986,
85.3800492093379));
#148186=CARTESIAN_POINT('Ctrl Pts',(38.1703740314513,-8.31774952095548,
85.372334501168));
#148187=CARTESIAN_POINT('Ctrl Pts',(38.1692140637238,-8.32223437734328,
85.368477147083));
#148188=CARTESIAN_POINT('Ctrl Pts',(38.1680587416159,-8.32669965993112,
85.3646343620035));
#148189=CARTESIAN_POINT('Ctrl Pts',(38.1669080738451,-8.3311454045957,85.3608061749156));
#148190=CARTESIAN_POINT('Ctrl Pts',(38.1657574060743,-8.33559114926027,
85.3569779878277));
#148191=CARTESIAN_POINT('Ctrl Pts',(38.1650167285598,-8.33845237175655,
85.3545135513215));
#148192=CARTESIAN_POINT('Ctrl Pts',(38.1634700421177,-8.34442406028693,
85.3493654362194));
#148193=CARTESIAN_POINT('Ctrl Pts',(38.1209894227077,-8.50843986904196,
85.2079695382673));
#148194=CARTESIAN_POINT('Ctrl Pts',(38.0774939924553,-8.67347496440427,
85.0627533003965));
#148195=CARTESIAN_POINT('Ctrl Pts',(38.032998366253,-8.83954481212098,84.913779614927));
#148196=CARTESIAN_POINT('Ctrl Pts',(37.9948607039445,-8.9818849995149,84.786092725356));
#148197=CARTESIAN_POINT('Ctrl Pts',(37.955988367647,-9.12498584008693,84.6556458945396));
#148198=CARTESIAN_POINT('Ctrl Pts',(37.9163956452311,-9.26888020790597,
84.5224980340405));
#148199=CARTESIAN_POINT('Ctrl Pts',(37.8643469034322,-9.45804428503791,
84.3474613558498));
#148200=CARTESIAN_POINT('Ctrl Pts',(37.8110530695196,-9.64857949412737,
84.1677572350173));
#148201=CARTESIAN_POINT('Ctrl Pts',(37.7565315729619,-9.84047473256546,
83.9834084838153));
#148202=CARTESIAN_POINT('Ctrl Pts',(37.7036370545627,-10.0266436175219,
83.8045608910676));
#148203=CARTESIAN_POINT('Ctrl Pts',(37.6495870319644,-10.2140924789878,
83.6213416835189));
#148204=CARTESIAN_POINT('Ctrl Pts',(37.5944071466661,-10.4028513988054,
83.4337976900769));
#148205=CARTESIAN_POINT('Ctrl Pts',(37.5649595694911,-10.5035854403633,
83.3337120122845));
#148206=CARTESIAN_POINT('Ctrl Pts',(37.535190377774,-10.6046932838906,83.232395092593));
#148207=CARTESIAN_POINT('Ctrl Pts',(37.505104684855,-10.7061845463452,83.1298573144579));
#148208=CARTESIAN_POINT('Ctrl Pts',(39.6168697557491,-0.401447571728686,
89.09878183643));
#148209=CARTESIAN_POINT('Ctrl Pts',(39.6164986632191,-0.423699213959886,
89.0966772661));
#148210=CARTESIAN_POINT('Ctrl Pts',(39.6062991625191,-1.00745211277799,
89.03883302323));
#148211=CARTESIAN_POINT('Ctrl Pts',(39.5603644817491,-2.20004318169699,
88.77832450325));
#148212=CARTESIAN_POINT('Ctrl Pts',(39.4305948837391,-3.89800233267899,
88.04236454135));
#148213=CARTESIAN_POINT('Ctrl Pts',(39.2432936369891,-5.59810631869199,
86.98012638587));
#148214=CARTESIAN_POINT('Ctrl Pts',(39.0062523874891,-7.30762248550998,
85.6357986570799));
#148215=CARTESIAN_POINT('Ctrl Pts',(38.7409445539891,-8.95066677755598,
84.13116316432));
#148216=CARTESIAN_POINT('Ctrl Pts',(38.5531406949991,-10.01036398978,83.0660745532));
#148217=CARTESIAN_POINT('Ctrl Pts',(38.4618769343391,-10.51042279016,82.54849204656));
#148218=CARTESIAN_POINT('Ctrl Pts',(38.5589532493791,-0.521574169437586,
90.55113115247));
#148219=CARTESIAN_POINT('Ctrl Pts',(38.5585212780491,-0.547502548905586,
90.54868132133));
#148220=CARTESIAN_POINT('Ctrl Pts',(38.5466482255191,-1.22751162701999,
90.48134589437));
#148221=CARTESIAN_POINT('Ctrl Pts',(38.4932267806791,-2.60548887972399,
90.1783778255));
#148222=CARTESIAN_POINT('Ctrl Pts',(38.3476657190791,-4.50165028275699,
89.35286002319));
#148223=CARTESIAN_POINT('Ctrl Pts',(38.1451917885991,-6.335462567224,88.2045733022701));
#148224=CARTESIAN_POINT('Ctrl Pts',(37.8958275904891,-8.13206152847199,
86.79035865909));
#148225=CARTESIAN_POINT('Ctrl Pts',(37.6219025168191,-9.82769184312899,
85.2368523688499));
#148226=CARTESIAN_POINT('Ctrl Pts',(37.4302304055891,-10.90908042546,84.1498258091));
#148227=CARTESIAN_POINT('Ctrl Pts',(37.3374134759791,-11.41764050787,83.62343484366));
#148228=CARTESIAN_POINT('Ctrl Pts',(36.8542747409091,-0.438522368068186,
89.97657015498));
#148229=CARTESIAN_POINT('Ctrl Pts',(36.8538848592891,-0.461908765523086,
89.97435902645));
#148230=CARTESIAN_POINT('Ctrl Pts',(36.8431688485591,-1.07536930870899,
89.91358550959));
#148231=CARTESIAN_POINT('Ctrl Pts',(36.7949235200291,-2.32517630764799,
89.63997265504));
#148232=CARTESIAN_POINT('Ctrl Pts',(36.6602801862491,-4.08430682507998,
88.8763723640501));
#148233=CARTESIAN_POINT('Ctrl Pts',(36.4682961783991,-5.82567734180799,
87.78757695064));
#148234=CARTESIAN_POINT('Ctrl Pts',(36.2274516844991,-7.56206996171599,
86.42167995104));
#148235=CARTESIAN_POINT('Ctrl Pts',(35.9594843032291,-9.22134393241599,
84.9019614134));
#148236=CARTESIAN_POINT('Ctrl Pts',(35.7704865815491,-10.28773577467,83.83010207047));
#148237=CARTESIAN_POINT('Ctrl Pts',(35.6787434647391,-10.79041833453,83.30980100006));
#148238=CARTESIAN_POINT('Ctrl Pts',(36.9040323489391,-0.269278349005186,
88.1844214108399));
#148239=CARTESIAN_POINT('Ctrl Pts',(36.9037282382691,-0.287484663123986,
88.1826967135399));
#148240=CARTESIAN_POINT('Ctrl Pts',(36.8953700620491,-0.765331753880986,
88.1352951406999));
#148241=CARTESIAN_POINT('Ctrl Pts',(36.8576726892891,-1.75395177657199,
87.92150271593));
#148242=CARTESIAN_POINT('Ctrl Pts',(36.7452776403791,-3.23383900930099,
87.28407871843));
#148243=CARTESIAN_POINT('Ctrl Pts',(36.5746701305291,-4.78683051385399,
86.31651544951));
#148244=CARTESIAN_POINT('Ctrl Pts',(36.3511871984191,-6.40053388423998,
85.04908075965));
#148245=CARTESIAN_POINT('Ctrl Pts',(36.0953604786391,-7.98572043397698,
83.5982153347901));
#148246=CARTESIAN_POINT('Ctrl Pts',(35.9118126620491,-9.02155172821997,
82.55726393953));
#148247=CARTESIAN_POINT('Ctrl Pts',(35.8222577746591,-9.51225699775298,
82.049372934817));
#148248=CARTESIAN_POINT('',(35.848007777729,-9.62145567905125,82.3699746323318));
#148249=CARTESIAN_POINT('Ctrl Pts',(37.5051004487691,-10.70616518419,83.12983477216));
#148250=CARTESIAN_POINT('Ctrl Pts',(36.5978347423554,-10.7058101101168,
83.2902037073864));
#148251=CARTESIAN_POINT('Ctrl Pts',(35.9481946009574,-10.2251893971186,
82.9382716566004));
#148252=CARTESIAN_POINT('Ctrl Pts',(35.8480077820191,-9.62145570514599,
82.369974656902));
#148253=CARTESIAN_POINT('',(36.9231078832491,-0.454164387253686,88.46717031284));
#148254=CARTESIAN_POINT('Ctrl Pts',(36.9231078836017,-0.454164387253684,
88.4671703127778));
#148255=CARTESIAN_POINT('Ctrl Pts',(36.9204855400661,-0.579215517453633,
88.4522982635594));
#148256=CARTESIAN_POINT('Ctrl Pts',(36.9172067488959,-0.705401523346811,
88.4337033100507));
#148257=CARTESIAN_POINT('Ctrl Pts',(36.91324787678,-0.832819212190252,88.41125141964));
#148258=CARTESIAN_POINT('Ctrl Pts',(36.9093083236504,-0.959615112677564,
88.3889090926985));
#148259=CARTESIAN_POINT('Ctrl Pts',(36.9046952253662,-1.0876312092335,88.3627468944092));
#148260=CARTESIAN_POINT('Ctrl Pts',(36.8993790061486,-1.21692649295543,
88.3325971105308));
#148261=CARTESIAN_POINT('Ctrl Pts',(36.8941653038762,-1.34372847138129,
88.3030287292655));
#148262=CARTESIAN_POINT('Ctrl Pts',(36.8882752386231,-1.47176119273405,
88.2696245200025));
#148263=CARTESIAN_POINT('Ctrl Pts',(36.881676227213,-1.60103855818878,88.2321996896396));
#148264=CARTESIAN_POINT('Ctrl Pts',(36.8786089337181,-1.66112810758537,
88.214804214532));
#148265=CARTESIAN_POINT('Ctrl Pts',(36.8753884149429,-1.72148592772201,
88.1965397574779));
#148266=CARTESIAN_POINT('Ctrl Pts',(36.8720111362573,-1.78210985327536,
88.1773862624852));
#148267=CARTESIAN_POINT('Ctrl Pts',(36.8713476061124,-1.79402056774533,
88.1736231968658));
#148268=CARTESIAN_POINT('Ctrl Pts',(36.8706780245898,-1.80594154616967,
88.1698258118269));
#148269=CARTESIAN_POINT('Ctrl Pts',(36.8700023719187,-1.81787287878656,
88.1659939951173));
#148270=CARTESIAN_POINT('Ctrl Pts',(36.862917561535,-1.94298335764443,88.1258140387938));
#148271=CARTESIAN_POINT('Ctrl Pts',(36.8551789643605,-2.06925582542825,
88.0819262305807));
#148272=CARTESIAN_POINT('Ctrl Pts',(36.846783675606,-2.19653931916896,88.0343141627442));
#148273=CARTESIAN_POINT('Ctrl Pts',(36.8384573156836,-2.3227777621871,87.9870930098994));
#148274=CARTESIAN_POINT('Ctrl Pts',(36.8294849882894,-2.45001066457938,
87.9362084117139));
#148275=CARTESIAN_POINT('Ctrl Pts',(36.8198726336355,-2.57808496455812,
87.8816940519132));
#148276=CARTESIAN_POINT('Ctrl Pts',(36.8103596902718,-2.70483471588556,
87.8277434814267));
#148277=CARTESIAN_POINT('Ctrl Pts',(36.8002198826719,-2.83240851462995,
87.7702377975226));
#148278=CARTESIAN_POINT('Ctrl Pts',(36.7894677550147,-2.96065282739329,
87.7092594667506));
#148279=CARTESIAN_POINT('Ctrl Pts',(36.7808506229816,-3.06343231539864,
87.660389294802));
#148280=CARTESIAN_POINT('Ctrl Pts',(36.7718403631796,-3.16664236853377,
87.609289579579));
#148281=CARTESIAN_POINT('Ctrl Pts',(36.7624486466323,-3.27020175607686,
87.556026508269));
#148282=CARTESIAN_POINT('Ctrl Pts',(36.7613578466867,-3.28222965041635,
87.5498402743687));
#148283=CARTESIAN_POINT('Ctrl Pts',(36.7602618544229,-3.2942624067366,87.5436245932785));
#148284=CARTESIAN_POINT('Ctrl Pts',(36.7591606886614,-3.30629995569941,
87.5373795717616));
#148285=CARTESIAN_POINT('Ctrl Pts',(36.7454949420224,-3.45568899414377,
87.4598772693939));
#148286=CARTESIAN_POINT('Ctrl Pts',(36.7310316990482,-3.6058155140173,87.3778521356401));
#148287=CARTESIAN_POINT('Ctrl Pts',(36.7157841777847,-3.75665276525037,
87.2913791460365));
#148288=CARTESIAN_POINT('Ctrl Pts',(36.7008648563705,-3.90424327478115,
87.2067674702607));
#148289=CARTESIAN_POINT('Ctrl Pts',(36.6851946205673,-4.05251425759033,
87.1178971509139));
#148290=CARTESIAN_POINT('Ctrl Pts',(36.6687943330814,-4.20144801214735,
87.0248865006242));
#148291=CARTESIAN_POINT('Ctrl Pts',(36.6528740097125,-4.34602313225598,
86.9345978620479));
#148292=CARTESIAN_POINT('Ctrl Pts',(36.6362657192849,-4.49122280935251,
86.840407566456));
#148293=CARTESIAN_POINT('Ctrl Pts',(36.6189970158369,-4.63703770276595,
86.7424718825201));
#148294=CARTESIAN_POINT('Ctrl Pts',(36.6134116009886,-4.68420028640901,
86.7107954208286));
#148295=CARTESIAN_POINT('Ctrl Pts',(36.6077571665088,-4.7314272847846,86.6787275293833));
#148296=CARTESIAN_POINT('Ctrl Pts',(36.6020348484833,-4.77871854018616,
86.6462746511988));
#148297=CARTESIAN_POINT('Ctrl Pts',(36.5974580311413,-4.81654297372506,
86.6203182302154));
#148298=CARTESIAN_POINT('Ctrl Pts',(36.5928372138935,-4.85440937352727,
86.5941122733467));
#148299=CARTESIAN_POINT('Ctrl Pts',(36.5881730494456,-4.89231733944232,
86.5676604823064));
#148300=CARTESIAN_POINT('Ctrl Pts',(36.5685170244251,-5.05207155369143,
86.4561856249483));
#148301=CARTESIAN_POINT('Ctrl Pts',(36.5480905445439,-5.21256245260813,
86.3403413012061));
#148302=CARTESIAN_POINT('Ctrl Pts',(36.5269096847282,-5.37380385031308,
86.2202186747469));
#148303=CARTESIAN_POINT('Ctrl Pts',(36.5060987806526,-5.53222892322571,
86.1021941715726));
#148304=CARTESIAN_POINT('Ctrl Pts',(36.4845595894665,-5.6913784719199,85.980039345428));
#148305=CARTESIAN_POINT('Ctrl Pts',(36.4623154504218,-5.85128432563395,
85.8538865639369));
#148306=CARTESIAN_POINT('Ctrl Pts',(36.4400713113771,-6.011190179348,85.7277337824458));
#148307=CARTESIAN_POINT('Ctrl Pts',(36.4171221689588,-6.17185223853716,
85.5975827335966));
#148308=CARTESIAN_POINT('Ctrl Pts',(36.3935001965489,-6.33332230407614,
85.4636158709251));
#148309=CARTESIAN_POINT('Ctrl Pts',(36.3839537583239,-6.39857782038479,
85.4094753293783));
#148310=CARTESIAN_POINT('Ctrl Pts',(36.3742956241308,-6.46396357224032,
85.3547013272084));
#148311=CARTESIAN_POINT('Ctrl Pts',(36.3645278890673,-6.52948729328553,
85.2993057480396));
#148312=CARTESIAN_POINT('Ctrl Pts',(36.33721729842,-6.71269164019927,85.1444196893474));
#148313=CARTESIAN_POINT('Ctrl Pts',(36.3090494265076,-6.89697275943275,
84.9846717516336));
#148314=CARTESIAN_POINT('Ctrl Pts',(36.2800326420702,-7.08247408334454,
84.8201093911229));
#148315=CARTESIAN_POINT('Ctrl Pts',(36.2523166598315,-7.25965951234608,
84.662924246404));
#148316=CARTESIAN_POINT('Ctrl Pts',(36.2238261451942,-7.43795816874329,
84.5013465077463));
#148317=CARTESIAN_POINT('Ctrl Pts',(36.1945754362192,-7.61751897861946,
84.3354574934946));
#148318=CARTESIAN_POINT('Ctrl Pts',(36.1770708801192,-7.72497388757679,
84.2361842225859));
#148319=CARTESIAN_POINT('Ctrl Pts',(36.1592942197124,-7.83288126073805,
84.1353677724498));
#148320=CARTESIAN_POINT('Ctrl Pts',(36.1412498888878,-7.94127751027461,
84.0330332870971));
#148321=CARTESIAN_POINT('Ctrl Pts',(36.1254304032814,-8.03630862702806,
83.9433165259818));
#148322=CARTESIAN_POINT('Ctrl Pts',(36.1094026818148,-8.13170908607084,
83.8524187996686));
#148323=CARTESIAN_POINT('Ctrl Pts',(36.0931717062841,-8.22749574121146,
83.7603683628236));
#148324=CARTESIAN_POINT('Ctrl Pts',(36.0600954702211,-8.42269423751378,
83.572783705757));
#148325=CARTESIAN_POINT('Ctrl Pts',(36.0261748143884,-8.61949496237244,
83.380410108411));
#148326=CARTESIAN_POINT('Ctrl Pts',(35.9914249486467,-8.81798075492089,
83.1833338271658));
#148327=CARTESIAN_POINT('Ctrl Pts',(35.9576129973166,-9.01110932719348,
82.9915767228563));
#148328=CARTESIAN_POINT('Ctrl Pts',(35.9230159764349,-9.20583318997005,
82.795367266301));
#148329=CARTESIAN_POINT('Ctrl Pts',(35.8876549358059,-9.40225689693438,
82.5948248385148));
#148330=CARTESIAN_POINT('Ctrl Pts',(35.8745437364782,-9.4750870605519,82.5204675317842));
#148331=CARTESIAN_POINT('Ctrl Pts',(35.8613275731665,-9.54815120444581,
82.4455149448095));
#148332=CARTESIAN_POINT('Ctrl Pts',(35.84800778227,-9.62145570514599,82.3699746568577));
#148333=CARTESIAN_POINT('Ctrl Pts',(39.4126085609146,-0.605361527076818,
89.303184116066));
#148334=CARTESIAN_POINT('Ctrl Pts',(39.3830826694109,-0.607949740687352,
89.3300849028713));
#148335=CARTESIAN_POINT('Ctrl Pts',(39.3517747790665,-0.610432005932147,
89.3564534797));
#148336=CARTESIAN_POINT('Ctrl Pts',(39.3186428950151,-0.612776874303673,
89.3820233316278));
#148337=CARTESIAN_POINT('Ctrl Pts',(39.2863134838357,-0.615064948643988,
89.4069738673561));
#148338=CARTESIAN_POINT('Ctrl Pts',(39.2522468551104,-0.617222132514938,
89.4311634103301));
#148339=CARTESIAN_POINT('Ctrl Pts',(39.2164458244507,-0.619217002864159,
89.4543179667453));
#148340=CARTESIAN_POINT('Ctrl Pts',(39.181806346853,-0.621147150278882,
89.4767212809363));
#148341=CARTESIAN_POINT('Ctrl Pts',(39.145542886646,-0.622925266528472,
89.4981550600761));
#148342=CARTESIAN_POINT('Ctrl Pts',(39.1077034021859,-0.624521879320095,
89.5183542503743));
#148343=CARTESIAN_POINT('Ctrl Pts',(39.070516042106,-0.626090976141504,
89.5382053285181));
#148344=CARTESIAN_POINT('Ctrl Pts',(39.031806250036,-0.6274846871524,89.5568633344759));
#148345=CARTESIAN_POINT('Ctrl Pts',(38.9916684203604,-0.62867524175512,
89.574069494001));
#148346=CARTESIAN_POINT('Ctrl Pts',(38.9524709787942,-0.629837902886744,
89.5908725308871));
#148347=CARTESIAN_POINT('Ctrl Pts',(38.9119116024645,-0.630806730929495,
89.6062902404851));
#148348=CARTESIAN_POINT('Ctrl Pts',(38.8701272580662,-0.631557299395677,
89.6200848773503));
#148349=CARTESIAN_POINT('Ctrl Pts',(38.836450628922,-0.63216222969306,89.6312028421426));
#148350=CARTESIAN_POINT('Ctrl Pts',(38.801979225164,-0.632625389896376,
89.6412663788308));
#148351=CARTESIAN_POINT('Ctrl Pts',(38.766808573118,-0.632935279074347,
89.6501576115731));
#148352=CARTESIAN_POINT('Ctrl Pts',(38.7243785122306,-0.633309131019783,
89.6608840418402));
#148353=CARTESIAN_POINT('Ctrl Pts',(38.6809298997421,-0.633459689529876,
89.6699030852832));
#148354=CARTESIAN_POINT('Ctrl Pts',(38.6366711021073,-0.633369300936823,
89.6770286079621));
#148355=CARTESIAN_POINT('Ctrl Pts',(38.5928762441042,-0.633279859835633,
89.684079437867));
#148356=CARTESIAN_POINT('Ctrl Pts',(38.5482885036326,-0.632954428539797,
89.6892755904881));
#148357=CARTESIAN_POINT('Ctrl Pts',(38.503149051083,-0.632380513370048,
89.6924686713012));
#148358=CARTESIAN_POINT('Ctrl Pts',(38.4585245181781,-0.631813145027487,
89.6956253276575));
#148359=CARTESIAN_POINT('Ctrl Pts',(38.4133613629055,-0.6310028806348,89.6968238366789));
#148360=CARTESIAN_POINT('Ctrl Pts',(38.3679238893794,-0.629943047301416,
89.6959608290385));
#148361=CARTESIAN_POINT('Ctrl Pts',(38.361206822858,-0.629786371094542,
89.695833249768));
#148362=CARTESIAN_POINT('Ctrl Pts',(38.3544838081868,-0.62962425123485,
89.6956606977974));
#148363=CARTESIAN_POINT('Ctrl Pts',(38.3477557452501,-0.629456677211184,
89.6954429242308));
#148364=CARTESIAN_POINT('Ctrl Pts',(38.3027202313773,-0.62833498998285,
89.6939852172245));
#148365=CARTESIAN_POINT('Ctrl Pts',(38.2574572497619,-0.626968432168449,
89.6904973541722));
#148366=CARTESIAN_POINT('Ctrl Pts',(38.2122466402006,-0.625357297113154,
89.6849323266811));
#148367=CARTESIAN_POINT('Ctrl Pts',(38.1672370341778,-0.623753325063409,
89.6793920409537));
#148368=CARTESIAN_POINT('Ctrl Pts',(38.1222800998557,-0.621906940809301,
89.6717928435791));
#148369=CARTESIAN_POINT('Ctrl Pts',(38.0776608857395,-0.619824596328343,
89.6621387514638));
#148370=CARTESIAN_POINT('Ctrl Pts',(38.0331730893736,-0.617748385012941,
89.6525130937146));
#148371=CARTESIAN_POINT('Ctrl Pts',(37.9890218157171,-0.61543762055268,
89.6408446505096));
#148372=CARTESIAN_POINT('Ctrl Pts',(37.9454868331697,-0.61290473306776,
89.6271887923972));
#148373=CARTESIAN_POINT('Ctrl Pts',(37.9355265063314,-0.612325236173121,
89.6240644817372));
#148374=CARTESIAN_POINT('Ctrl Pts',(37.9255983994401,-0.611734136535927,
89.6208363517161));
#148375=CARTESIAN_POINT('Ctrl Pts',(37.9157057758992,-0.6111316252669,89.6175054371492));
#148376=CARTESIAN_POINT('Ctrl Pts',(37.8724267966282,-0.608495714518348,
89.6029331063716));
#148377=CARTESIAN_POINT('Ctrl Pts',(37.8298286826496,-0.605640984164935,
89.5863897887462));
#148378=CARTESIAN_POINT('Ctrl Pts',(37.7881725496278,-0.602586648415914,
89.567991787781));
#148379=CARTESIAN_POINT('Ctrl Pts',(37.7464396078346,-0.5995266808485,89.5495598631713));
#148380=CARTESIAN_POINT('Ctrl Pts',(37.7056527864113,-0.59626643688015,
89.5292668474361));
#148381=CARTESIAN_POINT('Ctrl Pts',(37.6660467507015,-0.592829880871123,
89.507273757858));
#148382=CARTESIAN_POINT('Ctrl Pts',(37.6262056706644,-0.589372930420163,
89.4851501490079));
#148383=CARTESIAN_POINT('Ctrl Pts',(37.5875599780202,-0.585737648835415,
89.4613068050183));
#148384=CARTESIAN_POINT('Ctrl Pts',(37.5503111464723,-0.58195202546577,
89.4359445295695));
#148385=CARTESIAN_POINT('Ctrl Pts',(37.541937453631,-0.581101001527752,
89.4302429841641));
#148386=CARTESIAN_POINT('Ctrl Pts',(37.5336341875282,-0.580242391247806,
89.4244648026186));
#148387=CARTESIAN_POINT('Ctrl Pts',(37.5254033402407,-0.579376530745491,
89.4186124714025));
#148388=CARTESIAN_POINT('Ctrl Pts',(37.4883253743076,-0.575476039691987,
89.3922491421023));
#148389=CARTESIAN_POINT('Ctrl Pts',(37.4527208525358,-0.571428301082649,
89.3643794486022));
#148390=CARTESIAN_POINT('Ctrl Pts',(37.4187425064932,-0.56726506356026,
89.3352448517187));
#148391=CARTESIAN_POINT('Ctrl Pts',(37.3844890561168,-0.563068118550058,
89.3058743677247));
#148392=CARTESIAN_POINT('Ctrl Pts',(37.3518883561261,-0.55875389246498,
89.2752191981415));
#148393=CARTESIAN_POINT('Ctrl Pts',(37.3210457848244,-0.554355573082808,
89.2435412610773));
#148394=CARTESIAN_POINT('Ctrl Pts',(37.2897623391319,-0.549894382600837,
89.2114105086147));
#148395=CARTESIAN_POINT('Ctrl Pts',(37.2602876182062,-0.545346770319937,
89.1782283273344));
#148396=CARTESIAN_POINT('Ctrl Pts',(37.2326783053699,-0.54074660372001,
89.1442709319909));
#148397=CARTESIAN_POINT('Ctrl Pts',(37.2288889262586,-0.540115230700122,
89.1396102783429));
#148398=CARTESIAN_POINT('Ctrl Pts',(37.2251346069408,-0.539482865285731,
89.1349350153405));
#148399=CARTESIAN_POINT('Ctrl Pts',(37.2214154186073,-0.538849592483184,
89.1302458487828));
#148400=CARTESIAN_POINT('Ctrl Pts',(37.193700854511,-0.534130584435423,
89.0953032227386));
#148401=CARTESIAN_POINT('Ctrl Pts',(37.1679412772532,-0.529361330935144,
89.0595897996328));
#148402=CARTESIAN_POINT('Ctrl Pts',(37.144136481793,-0.524575905972413,
89.0233898608578));
#148403=CARTESIAN_POINT('Ctrl Pts',(37.1199332686332,-0.519710387987728,
88.986584048516));
#148404=CARTESIAN_POINT('Ctrl Pts',(37.0977503832959,-0.514828222470887,
88.9492759630769));
#148405=CARTESIAN_POINT('Ctrl Pts',(37.0775381404591,-0.509961568520209,
88.9117425176981));
#148406=CARTESIAN_POINT('Ctrl Pts',(37.0567000583587,-0.50494422653606,
88.8730469101579));
#148407=CARTESIAN_POINT('Ctrl Pts',(37.0379560348227,-0.49994343426556,
88.834112388713));
#148408=CARTESIAN_POINT('Ctrl Pts',(37.021206637527,-0.494989533180578,
88.79520925528));
#148409=CARTESIAN_POINT('Ctrl Pts',(37.0041561906232,-0.489946591877963,
88.7556068863539));
#148410=CARTESIAN_POINT('Ctrl Pts',(36.9891719984924,-0.484952271510473,
88.7160374157217));
#148411=CARTESIAN_POINT('Ctrl Pts',(36.9761129012183,-0.480032883108771,
88.6767445821553));
#148412=CARTESIAN_POINT('Ctrl Pts',(36.962628390604,-0.474953240639975,
88.6361717446794));
#148413=CARTESIAN_POINT('Ctrl Pts',(36.9511957079229,-0.469953510914846,
88.5958941545307));
#148414=CARTESIAN_POINT('Ctrl Pts',(36.9416322998081,-0.465056243063057,
88.5561310553602));
#148415=CARTESIAN_POINT('Ctrl Pts',(36.9344242400316,-0.461365111303961,
88.526161112398));
#148416=CARTESIAN_POINT('Ctrl Pts',(36.9282774544592,-0.457732046663515,
88.4964823808057));
#148417=CARTESIAN_POINT('Ctrl Pts',(36.9231078836017,-0.454164387253685,
88.4671703127778));
#148418=CARTESIAN_POINT('Ctrl Pts',(39.6230428380891,0.194165912825814,
89.10440256372));
#148419=CARTESIAN_POINT('Ctrl Pts',(39.6230835571391,0.188318965759814,
89.1046334929299));
#148420=CARTESIAN_POINT('Ctrl Pts',(39.6238267343091,0.0765431320962642,
89.10884826011));
#148421=CARTESIAN_POINT('Ctrl Pts',(39.6239646769391,-0.140676791074186,
89.10963057164));
#148422=CARTESIAN_POINT('Ctrl Pts',(39.6205750423291,-0.456053684225086,
89.0904069985));
#148423=CARTESIAN_POINT('Ctrl Pts',(39.6159638777391,-0.665968720299886,
89.06425578459));
#148424=CARTESIAN_POINT('Ctrl Pts',(39.6130667616891,-0.771133841521687,
89.0478254230199));
#148425=CARTESIAN_POINT('Ctrl Pts',(39.6130033270391,-0.773426316473186,
89.04746566723));
#148426=CARTESIAN_POINT('Ctrl Pts',(38.5691068518391,0.244771599243314,
90.5717118808201));
#148427=CARTESIAN_POINT('Ctrl Pts',(38.5691581710291,0.237403022922614,
90.5720029264299));
#148428=CARTESIAN_POINT('Ctrl Pts',(38.5700948214891,0.0965319925331742,
90.57731493513));
#148429=CARTESIAN_POINT('Ctrl Pts',(38.5702688861991,-0.177441261231286,
90.5783021051901));
#148430=CARTESIAN_POINT('Ctrl Pts',(38.5659956750091,-0.574725948486886,
90.5540675202501));
#148431=CARTESIAN_POINT('Ctrl Pts',(38.5602096181291,-0.837927759919986,
90.5212531610201));
#148432=CARTESIAN_POINT('Ctrl Pts',(38.5565902006391,-0.969313074494586,
90.50072642442));
#148433=CARTESIAN_POINT('Ctrl Pts',(38.5565109568191,-0.972176888914785,
90.50027701038));
#148434=CARTESIAN_POINT('Ctrl Pts',(36.8563477221291,0.210105182233614,
89.99587069318));
#148435=CARTESIAN_POINT('Ctrl Pts',(36.8563917799091,0.203778967710814,
89.99612055725));
#148436=CARTESIAN_POINT('Ctrl Pts',(36.8571958953491,0.0828390220290842,
90.00068092251));
#148437=CARTESIAN_POINT('Ctrl Pts',(36.8573452153491,-0.152256493592886,
90.0015277583201));
#148438=CARTESIAN_POINT('Ctrl Pts',(36.8536772806891,-0.493431878756386,
89.98072586715));
#148439=CARTESIAN_POINT('Ctrl Pts',(36.8486960603491,-0.720130646629686,
89.95247596284));
#148440=CARTESIAN_POINT('Ctrl Pts',(36.8455714410691,-0.833554340264386,
89.93475536632));
#148441=CARTESIAN_POINT('Ctrl Pts',(36.8455030270091,-0.836026769967186,
89.93436737088));
#148442=CARTESIAN_POINT('Ctrl Pts',(36.9051284241591,0.139155051791214,
88.19062138055));
#148443=CARTESIAN_POINT('Ctrl Pts',(36.9051576203291,0.134962190291614,
88.19078696029));
#148444=CARTESIAN_POINT('Ctrl Pts',(36.9056904825591,0.0548142612602442,
88.19380897218));
#148445=CARTESIAN_POINT('Ctrl Pts',(36.9057891587191,-0.100712010394486,
88.1943685924501));
#148446=CARTESIAN_POINT('Ctrl Pts',(36.9033600151491,-0.327051117515386,
88.1805922347));
#148447=CARTESIAN_POINT('Ctrl Pts',(36.9000260160591,-0.479040817491986,
88.16168418626));
#148448=CARTESIAN_POINT('Ctrl Pts',(36.8979140770691,-0.555703303635986,
88.14970678509));
#148449=CARTESIAN_POINT('Ctrl Pts',(36.8978678277591,-0.557374704586886,
88.14944449221));
#148450=CARTESIAN_POINT('',(36.9278603430303,-1.00177063435092E-6,88.4941228548076));
#148451=CARTESIAN_POINT('Ctrl Pts',(36.9278603430291,-2.97267519524715E-6,
88.4941228548));
#148452=CARTESIAN_POINT('Ctrl Pts',(36.9278604219491,-0.0762479038749758,
88.49412330237));
#148453=CARTESIAN_POINT('Ctrl Pts',(36.9270606224491,-0.228190456260686,
88.4895874156));
#148454=CARTESIAN_POINT('Ctrl Pts',(36.9246749306291,-0.379014038241186,
88.47605748015));
#148455=CARTESIAN_POINT('Ctrl Pts',(36.9231078832491,-0.454164387253686,
88.46717031284));
#148456=CARTESIAN_POINT('',(39.4241793029232,-9.78010097509158E-7,89.3342949669387));
#148457=CARTESIAN_POINT('Origin',(38.4050719433491,9.69735768033255E-7,
88.23365042271));
#148458=CARTESIAN_POINT('Origin',(36.6903869784213,-0.361278919426404,81.9235440633504));
#148459=CARTESIAN_POINT('Ctrl Pts',(36.2786061953091,0.207874208027314,
99.1854858506699));
#148460=CARTESIAN_POINT('Ctrl Pts',(36.2804402733591,0.0518199014528942,
99.18628534125));
#148461=CARTESIAN_POINT('Ctrl Pts',(36.2798690360391,-0.330489837835886,
99.18604356481));
#148462=CARTESIAN_POINT('Ctrl Pts',(36.2628587211991,-0.832940233787786,
99.1786077462799));
#148463=CARTESIAN_POINT('Ctrl Pts',(36.2409501422491,-1.18047906866699,
99.16880011873));
#148464=CARTESIAN_POINT('Ctrl Pts',(36.2321464823691,-1.30088361809899,
99.16482121612));
#148465=CARTESIAN_POINT('Ctrl Pts',(34.9573762488691,0.103201196527414,
92.86118521246));
#148466=CARTESIAN_POINT('Ctrl Pts',(34.9589714992491,0.0257039272848542,
92.86073498844));
#148467=CARTESIAN_POINT('Ctrl Pts',(34.9584734757791,-0.163964725101886,
92.8608772735799));
#148468=CARTESIAN_POINT('Ctrl Pts',(34.9436819944391,-0.413997315175786,
92.86504889005));
#148469=CARTESIAN_POINT('Ctrl Pts',(34.9246064026991,-0.588616325050186,
92.8700772173199));
#148470=CARTESIAN_POINT('Ctrl Pts',(34.9169358794491,-0.649381969463186,
92.87203589546));
#148471=CARTESIAN_POINT('Ctrl Pts',(38.6633388710591,0.0807359298002742,
87.56791503177));
#148472=CARTESIAN_POINT('Ctrl Pts',(38.6653943621291,0.0201178049123542,
87.56771699648));
#148473=CARTESIAN_POINT('Ctrl Pts',(38.6647586993891,-0.128317194034386,
87.5677800351001));
#148474=CARTESIAN_POINT('Ctrl Pts',(38.6456800868891,-0.323682344850186,
87.56961385163));
#148475=CARTESIAN_POINT('Ctrl Pts',(38.6212145471391,-0.459440396730986,
87.57177962771));
#148476=CARTESIAN_POINT('Ctrl Pts',(38.6114058460491,-0.506574295099986,
87.57261479282));
#148477=CARTESIAN_POINT('Ctrl Pts',(45.0583801383591,0.154651878623914,
86.6452310386901));
#148478=CARTESIAN_POINT('Ctrl Pts',(45.0613045698591,0.0385858522600842,
86.6466279881101));
#148479=CARTESIAN_POINT('Ctrl Pts',(45.0604072521791,-0.246037484612986,
86.64619846919));
#148480=CARTESIAN_POINT('Ctrl Pts',(45.0332403204891,-0.618975576296886,
86.6332241827699));
#148481=CARTESIAN_POINT('Ctrl Pts',(44.9985624478491,-0.874449147389286,
86.6166349022499));
#148482=CARTESIAN_POINT('Ctrl Pts',(44.9846932436191,-0.962558808579585,
86.6099942916699));
#148483=CARTESIAN_POINT('Origin',(46.5579300163491,-6.05980869095053E-8,
97.03881113036));
#148484=CARTESIAN_POINT('Origin',(-15.5675364833309,-75.,72.98888938658));
#148485=CARTESIAN_POINT('',(-15.5675364833309,-86.22497216032,82.938763757646));
#148486=CARTESIAN_POINT('',(-15.5675364833309,-63.77502783969,82.938763757662));
#148487=CARTESIAN_POINT('Origin',(-15.5675364833309,-75.,72.98888938658));
#148488=CARTESIAN_POINT('',(-15.5675364833309,-63.77502783968,63.039015015514));
#148489=CARTESIAN_POINT('Ctrl Pts',(-15.5675364833309,-63.7750278396901,
82.938763757662));
#148490=CARTESIAN_POINT('Ctrl Pts',(-15.5675364833309,-62.6179303673713,
81.6333817569256));
#148491=CARTESIAN_POINT('Ctrl Pts',(-15.5675364831843,-61.6763643545582,
80.0979293949852));
#148492=CARTESIAN_POINT('Ctrl Pts',(-15.5675364831843,-60.3554402463129,
76.7331391278798));
#148493=CARTESIAN_POINT('Ctrl Pts',(-15.5675364833367,-60.0000151056028,
74.8473853384574));
#148494=CARTESIAN_POINT('Ctrl Pts',(-15.5675364833367,-59.9999845441923,
71.2120906405687));
#148495=CARTESIAN_POINT('Ctrl Pts',(-15.5675364832353,-60.3254915562694,
69.3197329090816));
#148496=CARTESIAN_POINT('Ctrl Pts',(-15.5675364832353,-61.7205672754213,
65.7681234014825));
#148497=CARTESIAN_POINT('Ctrl Pts',(-15.5675364833309,-62.6886244946971,
64.2646432845299));
#148498=CARTESIAN_POINT('Ctrl Pts',(-15.5675364833309,-63.7750278396796,
63.0390150155136));
#148499=CARTESIAN_POINT('',(-15.5675722559773,-86.2249610151766,63.0390024421084));
#148500=CARTESIAN_POINT('Origin',(-15.5675364833309,-75.,72.98888938658));
#148501=CARTESIAN_POINT('',(-15.5675362859867,-87.7888428218549,65.1501692217888));
#148502=CARTESIAN_POINT('Ctrl Pts',(-15.5675364833309,-86.22496630623,63.039008410399));
#148503=CARTESIAN_POINT('Ctrl Pts',(-15.5675364833309,-86.8043901271152,
63.6926858768345));
#148504=CARTESIAN_POINT('Ctrl Pts',(-15.5675364833309,-87.3248767325505,
64.3932124764954));
#148505=CARTESIAN_POINT('Ctrl Pts',(-15.5675364833309,-87.7888432730159,
65.1501689452555));
#148506=CARTESIAN_POINT('',(-15.5675362859827,-87.7888428219253,80.8276095513668));
#148507=CARTESIAN_POINT('Ctrl Pts',(-15.5675364833309,-87.78884383193,65.150169857118));
#148508=CARTESIAN_POINT('Ctrl Pts',(-15.5675364833309,-88.1384521311545,
65.7205578137845));
#148509=CARTESIAN_POINT('Ctrl Pts',(-15.5675364833309,-88.4562376776849,
66.3283180635497));
#148510=CARTESIAN_POINT('Ctrl Pts',(-15.5675364833309,-88.7331232623695,
66.9594691299437));
#148511=CARTESIAN_POINT('Ctrl Pts',(-15.5675364833309,-89.0100091596637,
67.5906209089204));
#148512=CARTESIAN_POINT('Ctrl Pts',(-15.5675364833309,-89.2459950027582,
68.2451635573432));
#148513=CARTESIAN_POINT('Ctrl Pts',(-15.5675364833309,-89.434356875338,
68.9085289128966));
#148514=CARTESIAN_POINT('Ctrl Pts',(-15.5675364833309,-89.6227187479178,
69.5718942684499));
#148515=CARTESIAN_POINT('Ctrl Pts',(-15.5675364833309,-89.763456649983,
70.2440823311337));
#148516=CARTESIAN_POINT('Ctrl Pts',(-15.5675364833309,-89.8578157866714,
70.9238061165624));
#148517=CARTESIAN_POINT('Ctrl Pts',(-15.5675364833309,-89.9049953550156,
71.2636680092768));
#148518=CARTESIAN_POINT('Ctrl Pts',(-15.5675364833309,-89.9405802320157,
71.6054138326774));
#148519=CARTESIAN_POINT('Ctrl Pts',(-15.5675364833309,-89.9643226891465,
71.9496920446505));
#148520=CARTESIAN_POINT('Ctrl Pts',(-15.5675364833309,-89.9880651462773,
72.2939702566235));
#148521=CARTESIAN_POINT('Ctrl Pts',(-15.5675364833309,-89.9999651835389,
72.6407808571691));
#148522=CARTESIAN_POINT('Ctrl Pts',(-15.5675364833309,-89.9999999415976,
72.9875657846074));
#148523=CARTESIAN_POINT('Ctrl Pts',(-15.5675364833309,-90.0000346996564,
73.3343507120457));
#148524=CARTESIAN_POINT('Ctrl Pts',(-15.5675364833309,-89.9882041785122,
73.6811099663768));
#148525=CARTESIAN_POINT('Ctrl Pts',(-15.5675364833309,-89.964544078123,
74.025310009284));
#148526=CARTESIAN_POINT('Ctrl Pts',(-15.5675364833309,-89.9408839777337,
74.3695100521911));
#148527=CARTESIAN_POINT('Ctrl Pts',(-15.5675364833309,-89.9053942980993,
74.7111508836743));
#148528=CARTESIAN_POINT('Ctrl Pts',(-15.5675364833309,-89.8582821639484,
75.0509875740311));
#148529=CARTESIAN_POINT('Ctrl Pts',(-15.5675364833309,-89.7640578956464,
75.7306609547447));
#148530=CARTESIAN_POINT('Ctrl Pts',(-15.5675364833309,-89.623343809278,
76.4031177709525));
#148531=CARTESIAN_POINT('Ctrl Pts',(-15.5675364833309,-89.4350795265403,
77.066692601835));
#148532=CARTESIAN_POINT('Ctrl Pts',(-15.5675364833309,-89.2468152438025,
77.7302674327175));
#148533=CARTESIAN_POINT('Ctrl Pts',(-15.5675364833309,-89.0110007646955,
78.3849602782747));
#148534=CARTESIAN_POINT('Ctrl Pts',(-15.5675364833309,-88.7341288890014,
79.016341571848));
#148535=CARTESIAN_POINT('Ctrl Pts',(-15.5675364833309,-88.4572573251297,
79.6477221543386));
#148536=CARTESIAN_POINT('Ctrl Pts',(-15.5675364833309,-88.1393284571513,
80.2557912373537));
#148537=CARTESIAN_POINT('Ctrl Pts',(-15.5675364833309,-87.78884383202,80.827608916005));
#148538=CARTESIAN_POINT('Ctrl Pts',(-15.5675364833309,-87.7888432730861,
80.8276098278998));
#148539=CARTESIAN_POINT('Ctrl Pts',(-15.5675364833309,-87.3288337727753,
81.578110400252));
#148540=CARTESIAN_POINT('Ctrl Pts',(-15.5675364833309,-86.8094297339697,
82.2794066895671));
#148541=CARTESIAN_POINT('Ctrl Pts',(-15.5675364833309,-86.22497216032,82.938763757646));
#148542=CARTESIAN_POINT('Ctrl Pts',(-11.5022227331779,-92.24059357535,82.170676098169));
#148543=CARTESIAN_POINT('Ctrl Pts',(-11.6900590068975,-90.08199127819,81.018814103239));
#148544=CARTESIAN_POINT('Ctrl Pts',(-13.340335337564,-88.3574125816099,
80.449317902351));
#148545=CARTESIAN_POINT('Ctrl Pts',(-15.7224335390679,-87.8306099166801,
80.7144498191781));
#148546=CARTESIAN_POINT('Ctrl Pts',(-11.2606355037699,-91.60559269606,83.19560543535));
#148547=CARTESIAN_POINT('Ctrl Pts',(-11.5151253257779,-89.4713091151301,
81.8775645334381));
#148548=CARTESIAN_POINT('Ctrl Pts',(-13.2736598773321,-87.7877285948101,
81.2333685902111));
#148549=CARTESIAN_POINT('Ctrl Pts',(-15.7260522384459,-87.33074482682,81.559964759865));
#148550=CARTESIAN_POINT('Ctrl Pts',(-10.9937695135339,-90.85061125929,84.14672603444));
#148551=CARTESIAN_POINT('Ctrl Pts',(-11.3301258891669,-88.76446201931,82.6491481018461));
#148552=CARTESIAN_POINT('Ctrl Pts',(-13.2094624536123,-87.14018413018,81.934204163023));
#148553=CARTESIAN_POINT('Ctrl Pts',(-15.7293652895189,-86.75795515826,82.345374479499));
#148554=CARTESIAN_POINT('Ctrl Pts',(-10.7185240592019,-89.96317024714,85.01999559162));
#148555=CARTESIAN_POINT('Ctrl Pts',(-11.1489392586529,-87.96379513296,83.3387148150201));
#148556=CARTESIAN_POINT('Ctrl Pts',(-13.1546927793304,-86.41956569116,82.5627311416799));
#148557=CARTESIAN_POINT('Ctrl Pts',(-15.7319333912539,-86.10357629771,83.0806217453801));
#148558=CARTESIAN_POINT('',(-11.4804365249865,-91.9999348338944,82.2509739592588));
#148559=CARTESIAN_POINT('Origin',(-16.3445396267105,-91.9999999945449,83.4087740069438));
#148560=CARTESIAN_POINT('',(-10.7897592617989,-89.96662731952,84.7813312827));
#148561=CARTESIAN_POINT('Ctrl Pts',(-10.7897592617989,-89.96662731952,84.7813312827));
#148562=CARTESIAN_POINT('Ctrl Pts',(-11.0308907230739,-90.74601077157,83.99976427574));
#148563=CARTESIAN_POINT('Ctrl Pts',(-11.2651526237029,-91.42091161506,83.15544542039));
#148564=CARTESIAN_POINT('Ctrl Pts',(-11.4804394903149,-91.99991170272,82.250961503044));
#148565=CARTESIAN_POINT('Origin',(-15.5675364833161,-89.9666295470565,86.2553885480345));
#148566=CARTESIAN_POINT('Ctrl Pts',(-14.1113299480839,-82.00270966797,86.25689542676));
#148567=CARTESIAN_POINT('Ctrl Pts',(-11.8626405705278,-82.36550259023,85.9811177666601));
#148568=CARTESIAN_POINT('Ctrl Pts',(-10.0162267657079,-83.30617916224,86.96615946002));
#148569=CARTESIAN_POINT('Ctrl Pts',(-9.30362299642891,-84.4520975419701,
88.8218429037501));
#148570=CARTESIAN_POINT('Ctrl Pts',(-14.6084235581879,-83.63151313314,85.3977275067));
#148571=CARTESIAN_POINT('Ctrl Pts',(-12.276179191861,-84.05626187835,85.01902796749));
#148572=CARTESIAN_POINT('Ctrl Pts',(-10.3874061607449,-85.22811992478,85.94969573067));
#148573=CARTESIAN_POINT('Ctrl Pts',(-9.74725467143191,-86.64761078011,87.79310189116));
#148574=CARTESIAN_POINT('Ctrl Pts',(-15.2202405060039,-85.09580522496,84.23630032922));
#148575=CARTESIAN_POINT('Ctrl Pts',(-12.769810936277,-85.4989458425199,
83.74870650635));
#148576=CARTESIAN_POINT('Ctrl Pts',(-10.8264676087449,-86.88819562728,84.6034677629701));
#148577=CARTESIAN_POINT('Ctrl Pts',(-10.2937231765359,-88.61774941448,86.4032922329));
#148578=CARTESIAN_POINT('Ctrl Pts',(-15.7858253484419,-86.2968668049501,
82.861956262163));
#148579=CARTESIAN_POINT('Ctrl Pts',(-13.2006025443896,-86.61561365093,82.351027486014));
#148580=CARTESIAN_POINT('Ctrl Pts',(-11.2038824748679,-88.19070270453,83.1115754237));
#148581=CARTESIAN_POINT('Ctrl Pts',(-10.7993506281129,-90.23051883621,84.76141092968));
#148582=CARTESIAN_POINT('',(-13.9923004473311,-82.1549149953847,86.172484981779));
#148583=CARTESIAN_POINT('Ctrl Pts',(-15.5675364833309,-86.2249721603224,
82.9387637576481));
#148584=CARTESIAN_POINT('Ctrl Pts',(-15.4656120592592,-86.0053159811617,
83.186569348349));
#148585=CARTESIAN_POINT('Ctrl Pts',(-15.3632750078612,-85.7773435514771,
83.4269937600978));
#148586=CARTESIAN_POINT('Ctrl Pts',(-15.2605270092227,-85.5416684370871,
83.6596025386694));
#148587=CARTESIAN_POINT('Ctrl Pts',(-15.2286260724226,-85.4684966281066,
83.7318223195185));
#148588=CARTESIAN_POINT('Ctrl Pts',(-15.1966858016408,-85.3945820821006,
83.8032886910187));
#148589=CARTESIAN_POINT('Ctrl Pts',(-15.164707060717,-85.3199424351608,
83.8739887164398));
#148590=CARTESIAN_POINT('Ctrl Pts',(-15.0972183933928,-85.1624212146251,
84.0231956694847));
#148591=CARTESIAN_POINT('Ctrl Pts',(-15.0295559702083,-85.0016705180204,
84.1689897085444));
#148592=CARTESIAN_POINT('Ctrl Pts',(-14.9617196972663,-84.8378521215638,
84.3112487193089));
#148593=CARTESIAN_POINT('Ctrl Pts',(-14.9278015607953,-84.7559429233355,
84.3823782246912));
#148594=CARTESIAN_POINT('Ctrl Pts',(-14.8938399616955,-84.6732667166982,
84.4526239646191));
#148595=CARTESIAN_POINT('Ctrl Pts',(-14.8598348933904,-84.5898433513543,
84.5219705847097));
#148596=CARTESIAN_POINT('Ctrl Pts',(-14.8428323592378,-84.5481316686824,
84.556643894755));
#148597=CARTESIAN_POINT('Ctrl Pts',(-14.8258189578757,-84.5062331934517,
84.591092423657));
#148598=CARTESIAN_POINT('Ctrl Pts',(-14.8087946891932,-84.4641503913645,
84.62531424654));
#148599=CARTESIAN_POINT('Ctrl Pts',(-14.800282554852,-84.4431089903209,
84.6424251579815));
#148600=CARTESIAN_POINT('Ctrl Pts',(-14.7917677036892,-84.4220215074326,
84.6594793928585));
#148601=CARTESIAN_POINT('Ctrl Pts',(-14.7832501357467,-84.4008882502899,
84.6764767101802));
#148602=CARTESIAN_POINT('Ctrl Pts',(-14.7789913517754,-84.3903216217185,
84.6849753688411));
#148603=CARTESIAN_POINT('Ctrl Pts',(-14.7747318886098,-84.3797435495776,
84.6934597981097));
#148604=CARTESIAN_POINT('Ctrl Pts',(-14.7704717462589,-84.369154072285,
84.7019299678404));
#148605=CARTESIAN_POINT('Ctrl Pts',(-14.766211603908,-84.3585645949924,
84.7104001375712));
#148606=CARTESIAN_POINT('Ctrl Pts',(-14.7614487457711,-84.3467135103602,
84.7198505336849));
#148607=CARTESIAN_POINT('Ctrl Pts',(-14.7576892816615,-84.3373514633523,
84.7272976682604));
#148608=CARTESIAN_POINT('Ctrl Pts',(-14.7244766462451,-84.2546433312974,
84.7930886848384));
#148609=CARTESIAN_POINT('Ctrl Pts',(-14.6899790214534,-84.1668123881177,
84.8615417050829));
#148610=CARTESIAN_POINT('Ctrl Pts',(-14.6541527336378,-84.0736496771072,
84.9323421676274));
#148611=CARTESIAN_POINT('Ctrl Pts',(-14.6190512769554,-83.9823718176266,
85.0017102077069));
#148612=CARTESIAN_POINT('Ctrl Pts',(-14.5826740707097,-83.8859755482417,
85.0733317188635));
#148613=CARTESIAN_POINT('Ctrl Pts',(-14.5450085622793,-83.7842556594628,
85.1468719738496));
#148614=CARTESIAN_POINT('Ctrl Pts',(-14.5085310419877,-83.6857440645948,
85.2180927340436));
#148615=CARTESIAN_POINT('Ctrl Pts',(-14.4708449976359,-83.5822391858921,
85.2911130827089));
#148616=CARTESIAN_POINT('Ctrl Pts',(-14.4319696764409,-83.4735492502824,
85.3655920748298));
#148617=CARTESIAN_POINT('Ctrl Pts',(-14.403554012694,-83.3941030471894,
85.4200320107907));
#148618=CARTESIAN_POINT('Ctrl Pts',(-14.3745035450076,-83.3118864615012,
85.4752505271231));
#148619=CARTESIAN_POINT('Ctrl Pts',(-14.3448377050704,-83.226823529824,
85.5311014069342));
#148620=CARTESIAN_POINT('Ctrl Pts',(-14.3254712279096,-83.1712926792887,
85.5675620225972));
#148621=CARTESIAN_POINT('Ctrl Pts',(-14.305834205992,-83.1145490552796,
85.6042917190634));
#148622=CARTESIAN_POINT('Ctrl Pts',(-14.2859266399296,-83.0565718014343,
85.6412469333113));
#148623=CARTESIAN_POINT('Ctrl Pts',(-14.2834381941718,-83.0493246447036,
85.6458663350923));
#148624=CARTESIAN_POINT('Ctrl Pts',(-14.2809455211633,-83.0420582113039,
85.6504892585988));
#148625=CARTESIAN_POINT('Ctrl Pts',(-14.2784486209066,-83.0347724632451,
85.6551156146363));
#148626=CARTESIAN_POINT('Ctrl Pts',(-14.2759517206499,-83.0274867151863,
85.6597419706738));
#148627=CARTESIAN_POINT('Ctrl Pts',(-14.2743733488263,-83.0228757247468,
85.6626637660008));
#148628=CARTESIAN_POINT('Ctrl Pts',(-14.2724657592636,-83.0172989205455,
85.6661941687955));
#148629=CARTESIAN_POINT('Ctrl Pts',(-14.2686505801383,-83.0061453121428,
85.6732549743849));
#148630=CARTESIAN_POINT('Ctrl Pts',(-14.2648485991046,-82.995009046459,
85.6802841527487));
#148631=CARTESIAN_POINT('Ctrl Pts',(-14.2610598161618,-82.9838902900655,
85.6872818862916));
#148632=CARTESIAN_POINT('Ctrl Pts',(-14.2534822502762,-82.9616527772784,
85.7012773533773));
#148633=CARTESIAN_POINT('Ctrl Pts',(-14.2459574767545,-82.9394853020566,
85.7151470420563));
#148634=CARTESIAN_POINT('Ctrl Pts',(-14.2384854955891,-82.9173892245883,
85.728892379904));
#148635=CARTESIAN_POINT('Ctrl Pts',(-14.2085975709273,-82.8290049147154,
85.7838737312947));
#148636=CARTESIAN_POINT('Ctrl Pts',(-14.1795543240126,-82.7417631278529,
85.8368657570438));
#148637=CARTESIAN_POINT('Ctrl Pts',(-14.1513557539548,-82.6557450291385,
85.8879604016492));
#148638=CARTESIAN_POINT('Ctrl Pts',(-14.1056922840827,-82.5164512688153,
85.9707007235795));
#148639=CARTESIAN_POINT('Ctrl Pts',(-14.0622424879955,-82.3803683376981,
86.0484660866791));
#148640=CARTESIAN_POINT('Ctrl Pts',(-14.021009930264,-82.247807422868,86.1216401981717));
#148641=CARTESIAN_POINT('Ctrl Pts',(-14.0113177916852,-82.216647610638,
86.138840528881));
#148642=CARTESIAN_POINT('Ctrl Pts',(-14.001748027803,-82.1856822216306,
86.1557871400861));
#148643=CARTESIAN_POINT('Ctrl Pts',(-13.9923004473314,-82.154914973001,
86.1724849405352));
#148644=CARTESIAN_POINT('',(-9.38953228746991,-84.5398910625,88.61388938658));
#148645=CARTESIAN_POINT('Ctrl Pts',(-9.38953228746955,-84.5398910625,88.6138893865798));
#148646=CARTESIAN_POINT('Ctrl Pts',(-9.46732490041307,-84.9199146414493,
88.4305627134663));
#148647=CARTESIAN_POINT('Ctrl Pts',(-9.5481939019438,-85.2933517189332,
88.2361911028148));
#148648=CARTESIAN_POINT('Ctrl Pts',(-9.63163192688313,-85.6602022949516,
88.0305923802988));
#148649=CARTESIAN_POINT('Ctrl Pts',(-9.71506995182247,-86.0270528709701,
87.8249936577829));
#148650=CARTESIAN_POINT('Ctrl Pts',(-9.80107708871513,-86.3873169455232,
87.6081675118582));
#148651=CARTESIAN_POINT('Ctrl Pts',(-9.88908546297492,-86.7409945186108,
87.3799276312666));
#148652=CARTESIAN_POINT('Ctrl Pts',(-9.93149206319931,-86.9114131131639,
87.2699508540234));
#148653=CARTESIAN_POINT('Ctrl Pts',(-9.97460623810215,-87.0812177182641,
87.1566792372891));
#148654=CARTESIAN_POINT('Ctrl Pts',(-10.017829253044,-87.2484237990849,
87.0414895539076));
#148655=CARTESIAN_POINT('Ctrl Pts',(-10.0344080496992,-87.312558048331,
86.9973069271257));
#148656=CARTESIAN_POINT('Ctrl Pts',(-10.0510033555079,-87.3763099990063,
86.9528423147313));
#148657=CARTESIAN_POINT('Ctrl Pts',(-10.0675832966058,-87.4395676628322,
86.9081741743193));
#148658=CARTESIAN_POINT('Ctrl Pts',(-10.1642601017378,-87.8084199285117,
86.6477164874846));
#148659=CARTESIAN_POINT('Ctrl Pts',(-10.2617137234065,-88.1657810428126,
86.3768586594466));
#148660=CARTESIAN_POINT('Ctrl Pts',(-10.359310849766,-88.5116510057349,
86.0954446257135));
#148661=CARTESIAN_POINT('Ctrl Pts',(-10.4558982141828,-88.8539425197962,
85.8169421652203));
#148662=CARTESIAN_POINT('Ctrl Pts',(-10.5526260811727,-89.1849794325178,
85.5281004989366));
#148663=CARTESIAN_POINT('Ctrl Pts',(-10.6488314986673,-89.5047617438996,
85.2287819496263));
#148664=CARTESIAN_POINT('Ctrl Pts',(-10.6959609636712,-89.6614178828744,
85.0821506739443));
#148665=CARTESIAN_POINT('Ctrl Pts',(-10.7429643021365,-89.8153730747478,
84.9330053285659));
#148666=CARTESIAN_POINT('Ctrl Pts',(-10.7897592617965,-89.96662731952,84.7813312826992));
#148667=CARTESIAN_POINT('Origin',(-13.9922814971304,-84.5398910366688,90.5670141989917));
#148668=CARTESIAN_POINT('Ctrl Pts',(-9.36316543113591,-84.79485741396,88.68507306022));
#148669=CARTESIAN_POINT('Ctrl Pts',(-9.52089785507191,-84.52189181462,88.25909049769));
#148670=CARTESIAN_POINT('Ctrl Pts',(-9.99271929691491,-83.97055140082,87.46229833598));
#148671=CARTESIAN_POINT('Ctrl Pts',(-11.1638051091349,-83.19637684992,86.55460492855));
#148672=CARTESIAN_POINT('Ctrl Pts',(-12.6378577027309,-82.58312137528,86.06242162813));
#148673=CARTESIAN_POINT('Ctrl Pts',(-13.6855439527239,-82.3368973288,86.05405719771));
#148674=CARTESIAN_POINT('Ctrl Pts',(-14.2037341389199,-82.25481693243,86.12140353019));
#148675=CARTESIAN_POINT('Ctrl Pts',(-9.24767657508891,-84.00598446336,88.94968435057));
#148676=CARTESIAN_POINT('Ctrl Pts',(-9.42115179510291,-83.75855212272,88.5312692084));
#148677=CARTESIAN_POINT('Ctrl Pts',(-9.91247134952491,-83.26101823161,87.75513773229));
#148678=CARTESIAN_POINT('Ctrl Pts',(-11.0704798546419,-82.56016909489,86.87706862434));
#148679=CARTESIAN_POINT('Ctrl Pts',(-12.5011304605773,-81.99370416917,86.3973053855));
#148680=CARTESIAN_POINT('Ctrl Pts',(-13.5150380396684,-81.75325243071,86.38291437305));
#148681=CARTESIAN_POINT('Ctrl Pts',(-14.0186219503769,-81.66825256106,86.44526609955));
#148682=CARTESIAN_POINT('Ctrl Pts',(-9.02110732129691,-82.43288905337,89.39524706291));
#148683=CARTESIAN_POINT('Ctrl Pts',(-9.21938651903491,-82.23328319354,88.99421222644));
#148684=CARTESIAN_POINT('Ctrl Pts',(-9.73855112510891,-81.83512480463,88.25989487262));
#148685=CARTESIAN_POINT('Ctrl Pts',(-10.8679585310409,-81.27152859285,87.43449506429));
#148686=CARTESIAN_POINT('Ctrl Pts',(-12.2214087371624,-80.80111226951,86.97204043525));
#148687=CARTESIAN_POINT('Ctrl Pts',(-13.1759013667958,-80.58377622138,86.94116396896));
#148688=CARTESIAN_POINT('Ctrl Pts',(-13.6534062038429,-80.50032404056,86.99087839766));
#148689=CARTESIAN_POINT('Ctrl Pts',(-8.63390385764391,-79.20559950703,90.01976900704));
#148690=CARTESIAN_POINT('Ctrl Pts',(-8.86287624956091,-79.09733565716,89.65283473253));
#148691=CARTESIAN_POINT('Ctrl Pts',(-9.41039510203091,-78.88383521299,88.99091950632));
#148692=CARTESIAN_POINT('Ctrl Pts',(-10.4863410151329,-78.5781942732,88.24450783708));
#148693=CARTESIAN_POINT('Ctrl Pts',(-11.722657985102,-78.30941010548,87.79963352364));
#148694=CARTESIAN_POINT('Ctrl Pts',(-12.5878203220956,-78.16912067339,87.73316725532));
#148695=CARTESIAN_POINT('Ctrl Pts',(-13.0250798682998,-78.10921981045,87.75627315149));
#148696=CARTESIAN_POINT('Ctrl Pts',(-8.43646722755891,-75.82295460461,90.27567271427));
#148697=CARTESIAN_POINT('Ctrl Pts',(-8.67457228700691,-75.80159547571,89.9271492125));
#148698=CARTESIAN_POINT('Ctrl Pts',(-9.22633231332491,-75.75956225844,89.30069277592));
#148699=CARTESIAN_POINT('Ctrl Pts',(-10.2725773694299,-75.69964845786,88.5884829841));
#148700=CARTESIAN_POINT('Ctrl Pts',(-11.4566903832199,-75.64722956981,88.14814037352));
#148701=CARTESIAN_POINT('Ctrl Pts',(-12.2830364939519,-75.62002220028,88.06199406937));
#148702=CARTESIAN_POINT('Ctrl Pts',(-12.7024212510196,-75.6084141972,88.07026937053));
#148703=CARTESIAN_POINT('Ctrl Pts',(-8.53644251351991,-72.45433594609,90.14553315307));
#148704=CARTESIAN_POINT('Ctrl Pts',(-8.76988752817891,-72.52017514507,89.78750600586));
#148705=CARTESIAN_POINT('Ctrl Pts',(-9.31940153097291,-72.64985744622,89.14272588511));
#148706=CARTESIAN_POINT('Ctrl Pts',(-10.3807195496249,-72.83504863245,88.41288548734));
#148707=CARTESIAN_POINT('Ctrl Pts',(-11.5914114362033,-72.99743164875,87.9703890705));
#148708=CARTESIAN_POINT('Ctrl Pts',(-12.4374024314272,-73.08191917965,87.89458815261));
#148709=CARTESIAN_POINT('Ctrl Pts',(-12.8657678794551,-73.11797934746,87.91059102918));
#148710=CARTESIAN_POINT('Ctrl Pts',(-8.80312062497391,-69.07786522395,89.75884753243));
#148711=CARTESIAN_POINT('Ctrl Pts',(-9.01991246902591,-69.23307671621,89.3769250268));
#148712=CARTESIAN_POINT('Ctrl Pts',(-9.55697366388591,-69.54076372218,88.68389914341));
#148713=CARTESIAN_POINT('Ctrl Pts',(-10.6566609744269,-69.97917371075,87.90432815956));
#148714=CARTESIAN_POINT('Ctrl Pts',(-11.9426748847926,-70.35617472473,87.45249436166));
#148715=CARTESIAN_POINT('Ctrl Pts',(-12.8456722144427,-70.54333343852,87.40161797299));
#148716=CARTESIAN_POINT('Ctrl Pts',(-13.3001072668109,-70.62003610521,87.4364636821));
#148717=CARTESIAN_POINT('Ctrl Pts',(-9.14077283870491,-66.72557398356,89.19463338426));
#148718=CARTESIAN_POINT('Ctrl Pts',(-9.32880949855591,-66.94937144786,88.78323786731));
#148719=CARTESIAN_POINT('Ctrl Pts',(-9.83816023021391,-67.39707941798,88.02624050682));
#148720=CARTESIAN_POINT('Ctrl Pts',(-10.9840980003949,-68.02992693744,87.17553264098));
#148721=CARTESIAN_POINT('Ctrl Pts',(-12.3746508960219,-68.55282376321,86.70717184876));
#148722=CARTESIAN_POINT('Ctrl Pts',(-13.3573195647358,-68.78769939384,86.6871470724));
#148723=CARTESIAN_POINT('Ctrl Pts',(-13.8473824995249,-68.87528428493,86.74485486738));
#148724=CARTESIAN_POINT('Ctrl Pts',(-9.36320138448591,-65.20481666306,88.68499094841));
#148725=CARTESIAN_POINT('Ctrl Pts',(-9.52093025095291,-65.47779132966,88.25900375063));
#148726=CARTESIAN_POINT('Ctrl Pts',(-9.99274691583291,-66.02915171764,87.46220423853));
#148727=CARTESIAN_POINT('Ctrl Pts',(-11.1638314564919,-66.80336097775,86.55450907384));
#148728=CARTESIAN_POINT('Ctrl Pts',(-12.63788868308,-67.41665312944,86.0623326859));
#148729=CARTESIAN_POINT('Ctrl Pts',(-13.6855831157219,-67.66289929178,86.05397688329));
#148730=CARTESIAN_POINT('Ctrl Pts',(-14.2037786680419,-67.74498930276,86.1213279171));
#148731=CARTESIAN_POINT('Ctrl Pts',(-9.38953228746991,-65.4601089375,88.61388938658));
#148732=CARTESIAN_POINT('Ctrl Pts',(-9.28328709691747,-66.2097609713885,
88.8642676240639));
#148733=CARTESIAN_POINT('Ctrl Pts',(-9.17708486958767,-66.9655883719527,
89.0795251225669));
#148734=CARTESIAN_POINT('Ctrl Pts',(-9.0302280749938,-68.1085925228124,
89.3540432573925));
#148735=CARTESIAN_POINT('Ctrl Pts',(-8.98330754389956,-68.4911377481012,
89.4374960493532));
#148736=CARTESIAN_POINT('Ctrl Pts',(-8.91715535501208,-69.0672713485378,
89.5511487398476));
#148737=CARTESIAN_POINT('Ctrl Pts',(-8.88513273745213,-69.3559170893819,
89.6050931419384));
#148738=CARTESIAN_POINT('Ctrl Pts',(-8.84983719738048,-69.6936835997954,
89.6630999929911));
#148739=CARTESIAN_POINT('Ctrl Pts',(-8.83273032605669,-69.8628201415259,
89.6908850775549));
#148740=CARTESIAN_POINT('Ctrl Pts',(-8.82551731869127,-69.9353615065227,
89.7025333452868));
#148741=CARTESIAN_POINT('Ctrl Pts',(-8.82073526432502,-69.9837344777835,
89.7102413212732));
#148742=CARTESIAN_POINT('Ctrl Pts',(-8.81853574016785,-70.0061031598871,
89.7137803985326));
#148743=CARTESIAN_POINT('Ctrl Pts',(-8.73463441113894,-70.8648417345999,
89.8485086409056));
#148744=CARTESIAN_POINT('Ctrl Pts',(-8.67003768437608,-71.6936986475477,
89.944358023184));
#148745=CARTESIAN_POINT('Ctrl Pts',(-8.60463652245025,-72.9311950958996,
90.0398919577533));
#148746=CARTESIAN_POINT('Ctrl Pts',(-8.58803785671435,-73.3427290918387,
90.0636744407946));
#148747=CARTESIAN_POINT('Ctrl Pts',(-8.57132975194435,-73.9585828554797,
90.0875200458021));
#148748=CARTESIAN_POINT('Ctrl Pts',(-8.56712264234536,-74.1636262383155,
90.0934954812812));
#148749=CARTESIAN_POINT('Ctrl Pts',(-8.56146522762817,-74.5732305938979,
90.1015227750632));
#148750=CARTESIAN_POINT('Ctrl Pts',(-8.56001530984221,-74.7765851842616,
90.1035740849179));
#148751=CARTESIAN_POINT('Ctrl Pts',(-8.55968148378128,-75.8042159346871,
90.1040468034545));
#148752=CARTESIAN_POINT('Ctrl Pts',(-8.58177592616641,-76.6283044763792,
90.0732381391729));
#148753=CARTESIAN_POINT('Ctrl Pts',(-8.64644160601739,-77.867413200945,
89.9788480269719));
#148754=CARTESIAN_POINT('Ctrl Pts',(-8.67320843583484,-78.2809454278049,
89.9393254017685));
#148755=CARTESIAN_POINT('Ctrl Pts',(-8.72052840036098,-78.9019877461016,
89.8675311439229));
#148756=CARTESIAN_POINT('Ctrl Pts',(-8.74597657546545,-79.2126948997517,
89.8285040402398));
#148757=CARTESIAN_POINT('Ctrl Pts',(-8.77860779189364,-79.5755120693882,
89.7773794891791));
#148758=CARTESIAN_POINT('Ctrl Pts',(-8.79563181834841,-79.7570020268009,
89.7504030045294));
#148759=CARTESIAN_POINT('Ctrl Pts',(-8.80307665120823,-79.8348008741052,
89.7385368699022));
#148760=CARTESIAN_POINT('Ctrl Pts',(-8.80807260339695,-79.8866706471935,
89.7305581866392));
#148761=CARTESIAN_POINT('Ctrl Pts',(-8.81073338330589,-79.9141085081485,
89.7263000880263));
#148762=CARTESIAN_POINT('Ctrl Pts',(-8.9656995991205,-81.5025605981437,
89.4778327793481));
#148763=CARTESIAN_POINT('Ctrl Pts',(-9.17644065973502,-83.0363422081069,
89.1160627640075));
#148764=CARTESIAN_POINT('Ctrl Pts',(-9.38953228746991,-84.5398910625,88.61388938658));
#148765=CARTESIAN_POINT('',(-13.9922632538745,-67.8450784104076,86.1724813495899));
#148766=CARTESIAN_POINT('Origin',(-13.9922817629778,-65.4601089375625,90.5670143866247));
#148767=CARTESIAN_POINT('Ctrl Pts',(-13.9922632538729,-67.8450784104129,
86.1724813495793));
#148768=CARTESIAN_POINT('Ctrl Pts',(-13.9285551321338,-68.0520701946722,
86.2848187148604));
#148769=CARTESIAN_POINT('Ctrl Pts',(-13.8647015765799,-68.2609196751036,
86.3918585032884));
#148770=CARTESIAN_POINT('Ctrl Pts',(-13.8013730345684,-68.4716504870294,
86.4937275061761));
#148771=CARTESIAN_POINT('Ctrl Pts',(-13.7378365702574,-68.6830731771134,
86.5959309686403));
#148772=CARTESIAN_POINT('Ctrl Pts',(-13.6748285726308,-68.8963899825192,
86.6929298523555));
#148773=CARTESIAN_POINT('Ctrl Pts',(-13.6130261144539,-69.1116541348552,
86.7848084560886));
#148774=CARTESIAN_POINT('Ctrl Pts',(-13.5511371715245,-69.3272195222469,
86.87681563235));
#148775=CARTESIAN_POINT('Ctrl Pts',(-13.4904571444066,-69.5447381338853,
86.9636883767891));
#148776=CARTESIAN_POINT('Ctrl Pts',(-13.431665952279,-69.7642865478471,
87.0454645258856));
#148777=CARTESIAN_POINT('Ctrl Pts',(-13.3830763120145,-69.9457385318768,
87.1130507326457));
#148778=CARTESIAN_POINT('Ctrl Pts',(-13.3357768712037,-70.1285775377871,
87.1771548238835));
#148779=CARTESIAN_POINT('Ctrl Pts',(-13.2901514710066,-70.3128555667207,
87.2377727484992));
#148780=CARTESIAN_POINT('Ctrl Pts',(-13.2637884073469,-70.4193342690851,
87.2727987252283));
#148781=CARTESIAN_POINT('Ctrl Pts',(-13.2379850419819,-70.5262944514629,
87.3066606384413));
#148782=CARTESIAN_POINT('Ctrl Pts',(-13.2128161545854,-70.6337472099288,
87.3393540680178));
#148783=CARTESIAN_POINT('Ctrl Pts',(-13.2096700436608,-70.647178804737,
87.3434407467149));
#148784=CARTESIAN_POINT('Ctrl Pts',(-13.2065338464545,-70.6606180964965,
87.347509164306));
#148785=CARTESIAN_POINT('Ctrl Pts',(-13.2034077096942,-70.6740651067791,
87.351559308973));
#148786=CARTESIAN_POINT('Ctrl Pts',(-13.2005271864215,-70.6864556159081,
87.3552912429432));
#148787=CARTESIAN_POINT('Ctrl Pts',(-13.1986999834587,-70.6943412175539,
87.3576538279662));
#148788=CARTESIAN_POINT('Ctrl Pts',(-13.1966065552207,-70.7033861337611,
87.3603579713991));
#148789=CARTESIAN_POINT('Ctrl Pts',(-13.1964280549407,-70.7041573663479,
87.3605885455125));
#148790=CARTESIAN_POINT('Ctrl Pts',(-13.1962476190816,-70.7049370361643,
87.3608215746784));
#148791=CARTESIAN_POINT('Ctrl Pts',(-13.1960644296178,-70.7057286591898,
87.3610581043308));
#148792=CARTESIAN_POINT('Ctrl Pts',(-13.1914012059293,-70.7258800105199,
87.3670791420875));
#148793=CARTESIAN_POINT('Ctrl Pts',(-13.1867535757959,-70.7460473567043,
87.3730587939704));
#148794=CARTESIAN_POINT('Ctrl Pts',(-13.1821220573804,-70.7662307481179,
87.3789970276582));
#148795=CARTESIAN_POINT('Ctrl Pts',(-13.1728590205494,-70.8065975309452,
87.3908734950339));
#148796=CARTESIAN_POINT('Ctrl Pts',(-13.1636604305903,-70.847028493799,
87.4025842960819));
#148797=CARTESIAN_POINT('Ctrl Pts',(-13.1545307665253,-70.8875252185154,
87.4141294598562));
#148798=CARTESIAN_POINT('Ctrl Pts',(-13.1180121102655,-71.0495121173814,
87.4603101149533));
#148799=CARTESIAN_POINT('Ctrl Pts',(-13.0825962683134,-71.2125513108651,
87.5038416280283));
#148800=CARTESIAN_POINT('Ctrl Pts',(-13.0485477116034,-71.3766762962778,
87.5446966585263));
#148801=CARTESIAN_POINT('Ctrl Pts',(-13.0031366647857,-71.5955721355358,
87.5991855967357));
#148802=CARTESIAN_POINT('Ctrl Pts',(-12.9601460521461,-71.8163441963887,
87.648893413177));
#148803=CARTESIAN_POINT('Ctrl Pts',(-12.9200620589948,-72.0385592644602,
87.6936460581433));
#148804=CARTESIAN_POINT('Ctrl Pts',(-12.9000372367978,-72.1495715882784,
87.7160032059183));
#148805=CARTESIAN_POINT('Ctrl Pts',(-12.8807378246369,-72.2609437584287,
87.7371244433808));
#148806=CARTESIAN_POINT('Ctrl Pts',(-12.8622244395765,-72.3726202435535,
87.7569927047253));
#148807=CARTESIAN_POINT('Ctrl Pts',(-12.8344384838983,-72.5402307510792,
87.7868121368456));
#148808=CARTESIAN_POINT('Ctrl Pts',(-12.8084219928603,-72.7085275052885,
87.8138085585889));
#148809=CARTESIAN_POINT('Ctrl Pts',(-12.7843726877417,-72.8773244673507,
87.8379381299538));
#148810=CARTESIAN_POINT('Ctrl Pts',(-12.7813665246019,-72.8984240876085,
87.8409543263744));
#148811=CARTESIAN_POINT('Ctrl Pts',(-12.7783910987421,-72.9195315229508,
87.8439257486868));
#148812=CARTESIAN_POINT('Ctrl Pts',(-12.7754467790334,-72.9406464143135,
87.8468523293632));
#148813=CARTESIAN_POINT('Ctrl Pts',(-12.7750787390698,-72.9432857757339,
87.8472181519478));
#148814=CARTESIAN_POINT('Ctrl Pts',(-12.7747111851399,-72.9459252721915,
87.8475831396505));
#148815=CARTESIAN_POINT('Ctrl Pts',(-12.7744712210636,-72.9476510013597,
87.8478215012301));
#148816=CARTESIAN_POINT('Ctrl Pts',(-12.7742312569873,-72.9493767305279,
87.8480598628097));
#148817=CARTESIAN_POINT('Ctrl Pts',(-12.7741183959124,-72.9501886470366,
87.8481717891691));
#148818=CARTESIAN_POINT('Ctrl Pts',(-12.7740743827478,-72.9505060053221,
87.8482155612684));
#148819=CARTESIAN_POINT('Ctrl Pts',(-12.7739863564187,-72.951140721893,
87.8483031054669));
#148820=CARTESIAN_POINT('Ctrl Pts',(-12.7738970129558,-72.9517866318275,
87.8483921520975));
#148821=CARTESIAN_POINT('Ctrl Pts',(-12.7738063561645,-72.9524437358476,
87.8484826967998));
#148822=CARTESIAN_POINT('Ctrl Pts',(-12.7736250425818,-72.9537579438877,
87.8486637862044));
#148823=CARTESIAN_POINT('Ctrl Pts',(-12.7734384756853,-72.9551169282491,
87.8488508680473));
#148824=CARTESIAN_POINT('Ctrl Pts',(-12.7732466858366,-72.9565206948447,
87.8490439056084));
#148825=CARTESIAN_POINT('Ctrl Pts',(-12.7724795264419,-72.962135761227,
87.8498160558532));
#148826=CARTESIAN_POINT('Ctrl Pts',(-12.7716287998118,-72.9684673368165,
87.8506835461686));
#148827=CARTESIAN_POINT('Ctrl Pts',(-12.7706965559355,-72.9755158673858,
87.8516436399744));
#148828=CARTESIAN_POINT('Ctrl Pts',(-12.7688320681828,-72.9896129285244,
87.853563827586));
#148829=CARTESIAN_POINT('Ctrl Pts',(-12.7666415114454,-73.0065777253166,
87.8558550511194));
#148830=CARTESIAN_POINT('Ctrl Pts',(-12.7641489210632,-73.0264146540014,
87.8584879313309));
#148831=CARTESIAN_POINT('Ctrl Pts',(-12.7603881731616,-73.0563440352818,
87.8624603444484));
#148832=CARTESIAN_POINT('Ctrl Pts',(-12.7559136899501,-73.0928109209032,
87.8672128776889));
#148833=CARTESIAN_POINT('Ctrl Pts',(-12.7508847748352,-73.1358347705,87.872601557847));
#148834=CARTESIAN_POINT('Ctrl Pts',(-12.7458602570049,-73.1788210000318,
87.8779855261419));
#148835=CARTESIAN_POINT('Ctrl Pts',(-12.740282276438,-73.2283528810644,
87.8840045407208));
#148836=CARTESIAN_POINT('Ctrl Pts',(-12.7343097190214,-73.2844532911088,
87.8904631118485));
#148837=CARTESIAN_POINT('Ctrl Pts',(-12.730411970744,-73.3210649569928,
87.8946780373371));
#148838=CARTESIAN_POINT('Ctrl Pts',(-12.726346172469,-73.3604742247497,
87.8990791121011));
#148839=CARTESIAN_POINT('Ctrl Pts',(-12.7221564858865,-73.4026877304981,
87.9036000278797));
#148840=CARTESIAN_POINT('Ctrl Pts',(-12.7157559134418,-73.4671771848689,
87.9105066182385));
#148841=CARTESIAN_POINT('Ctrl Pts',(-12.7090596196822,-73.5382113626362,
87.9176953668346));
#148842=CARTESIAN_POINT('Ctrl Pts',(-12.7023689986799,-73.6158148009317,
87.9248872218329));
#148843=CARTESIAN_POINT('Ctrl Pts',(-12.6957025587298,-73.6931377670874,
87.9320530842334));
#148844=CARTESIAN_POINT('Ctrl Pts',(-12.6890417506065,-73.7769828554256,
87.9392220142129));
#148845=CARTESIAN_POINT('Ctrl Pts',(-12.6826847123091,-73.8673696091889,
87.9460665399673));
#148846=CARTESIAN_POINT('Ctrl Pts',(-12.6784412431516,-73.9277048445438,
87.9506354182054));
#148847=CARTESIAN_POINT('Ctrl Pts',(-12.6743331298586,-73.9909548630671,
87.9550586877087));
#148848=CARTESIAN_POINT('Ctrl Pts',(-12.6704490504521,-74.057123363438,
87.9592261779894));
#148849=CARTESIAN_POINT('Ctrl Pts',(-12.6646823504542,-74.1553638603548,
87.9654136586451));
#148850=CARTESIAN_POINT('Ctrl Pts',(-12.6594351109689,-74.2600388012238,
87.9710396197401));
#148851=CARTESIAN_POINT('Ctrl Pts',(-12.6551289584109,-74.3711533682616,
87.9757019867879));
#148852=CARTESIAN_POINT('Ctrl Pts',(-12.6536321151853,-74.4097774264428,
87.9773226522049));
#148853=CARTESIAN_POINT('Ctrl Pts',(-12.6522489832399,-74.4491794557137,
87.9788264449859));
#148854=CARTESIAN_POINT('Ctrl Pts',(-12.6509972713499,-74.4893592249046,
87.9801950668338));
#148855=CARTESIAN_POINT('Ctrl Pts',(-12.6485709388204,-74.5672441453867,
87.9828480189523));
#148856=CARTESIAN_POINT('Ctrl Pts',(-12.6466421084436,-74.6480517625337,
87.9849937078946));
#148857=CARTESIAN_POINT('Ctrl Pts',(-12.6453635744747,-74.7317783140308,
87.9864910990931));
#148858=CARTESIAN_POINT('Ctrl Pts',(-12.6447243074902,-74.7736415897794,
87.9872397946923));
#148859=CARTESIAN_POINT('Ctrl Pts',(-12.6442478758437,-74.8162345453753,
87.9878262556343));
#148860=CARTESIAN_POINT('Ctrl Pts',(-12.6439550111987,-74.8595563603345,
87.9882318916392));
#148861=CARTESIAN_POINT('Ctrl Pts',(-12.6438085788762,-74.8812172678141,
87.9884347096417));
#148862=CARTESIAN_POINT('Ctrl Pts',(-12.643708038304,-74.9030603906,87.9885923114367));
#148863=CARTESIAN_POINT('Ctrl Pts',(-12.6436561075558,-74.9250855971942,
87.9887023131552));
#148864=CARTESIAN_POINT('Ctrl Pts',(-12.6436301421817,-74.9360982004913,
87.9887573140144));
#148865=CARTESIAN_POINT('Ctrl Pts',(-12.6436163292635,-74.9471563247771,
87.9888004142327));
#148866=CARTESIAN_POINT('Ctrl Pts',(-12.6436150126614,-74.9582599527134,
87.9888313120827));
#148867=CARTESIAN_POINT('Ctrl Pts',(-12.6436136960593,-74.9693635806496,
87.9888622099326));
#148868=CARTESIAN_POINT('Ctrl Pts',(-12.6436289425738,-74.9824075328569,
87.9888819529563));
#148869=CARTESIAN_POINT('Ctrl Pts',(-12.643648897583,-74.9917073296298,
87.9888870943004));
#148870=CARTESIAN_POINT('Ctrl Pts',(-12.6441957679959,-75.2465698379219,
87.9890279937067));
#148871=CARTESIAN_POINT('Ctrl Pts',(-12.6513772313359,-75.5018909548218,
87.9826693312941));
#148872=CARTESIAN_POINT('Ctrl Pts',(-12.6647090535987,-75.757165505727,
87.9697672112249));
#148873=CARTESIAN_POINT('Ctrl Pts',(-12.6780337951938,-76.0123044776953,
87.9568719436042));
#148874=CARTESIAN_POINT('Ctrl Pts',(-12.6975023644089,-76.2673965773429,
87.9374401515452));
#148875=CARTESIAN_POINT('Ctrl Pts',(-12.7226312983753,-76.5219356309839,
87.9114800442085));
#148876=CARTESIAN_POINT('Ctrl Pts',(-12.7310755095397,-76.6074697615364,
87.9027565293752));
#148877=CARTESIAN_POINT('Ctrl Pts',(-12.7401588878712,-76.6929414509161,
87.8932962737769));
#148878=CARTESIAN_POINT('Ctrl Pts',(-12.74986308835,-76.7783315551092,87.8831009091851));
#148879=CARTESIAN_POINT('Ctrl Pts',(-12.7782149982648,-77.027808320039,
87.8533140082358));
#148880=CARTESIAN_POINT('Ctrl Pts',(-12.8118641877124,-77.2765816129467,
87.8172492980099));
#148881=CARTESIAN_POINT('Ctrl Pts',(-12.8503429439184,-77.5241603024399,
87.7749847050739));
#148882=CARTESIAN_POINT('Ctrl Pts',(-12.8576532392744,-77.5711959533419,
87.7669551664939));
#148883=CARTESIAN_POINT('Ctrl Pts',(-12.8651378501164,-77.6181885118085,
87.7587020021747));
#148884=CARTESIAN_POINT('Ctrl Pts',(-12.872793569282,-77.6651346488302,
87.7502259555904));
#148885=CARTESIAN_POINT('Ctrl Pts',(-12.8967699000968,-77.8121614777091,
87.7236805073432));
#148886=CARTESIAN_POINT('Ctrl Pts',(-12.9224245115847,-77.9587328844472,
87.6949484881787));
#148887=CARTESIAN_POINT('Ctrl Pts',(-12.9496575490047,-78.1047475853005,
87.6640569301405));
#148888=CARTESIAN_POINT('Ctrl Pts',(-12.9632740677147,-78.1777549357272,
87.6486111511213));
#148889=CARTESIAN_POINT('Ctrl Pts',(-12.9772851929078,-78.2506231495068,
87.6326255837542));
#148890=CARTESIAN_POINT('Ctrl Pts',(-12.9916784029335,-78.3233398291162,
87.6161041720479));
#148891=CARTESIAN_POINT('Ctrl Pts',(-12.9988750079464,-78.3596981689209,
87.6078434661947));
#148892=CARTESIAN_POINT('Ctrl Pts',(-13.0061671341675,-78.3960186283675,
87.5994488049755));
#148893=CARTESIAN_POINT('Ctrl Pts',(-13.0135532117496,-78.4322996754754,
87.5909207157386));
#148894=CARTESIAN_POINT('Ctrl Pts',(-13.0204776594828,-78.4663131571391,
87.5829256320791));
#148895=CARTESIAN_POINT('Ctrl Pts',(-13.0274846816545,-78.5002919991374,
87.5748132779195));
#148896=CARTESIAN_POINT('Ctrl Pts',(-13.0345729827054,-78.53423494977,87.5665841055616));
#148897=CARTESIAN_POINT('Ctrl Pts',(-13.0350455361088,-78.5364978131455,
87.5660354940711));
#148898=CARTESIAN_POINT('Ctrl Pts',(-13.0358533538705,-78.5403615571573,
87.5650974156943));
#148899=CARTESIAN_POINT('Ctrl Pts',(-13.0359917262273,-78.5410230609782,
87.5649367136718));
#148900=CARTESIAN_POINT('Ctrl Pts',(-13.0404196416454,-78.5621911832477,
87.5597942489534));
#148901=CARTESIAN_POINT('Ctrl Pts',(-13.0461916289288,-78.5902495695812,
87.5529342151086));
#148902=CARTESIAN_POINT('Ctrl Pts',(-13.0534262917923,-78.6251519329629,
87.5442414421963));
#148903=CARTESIAN_POINT('Ctrl Pts',(-13.0604266942057,-78.6589241478486,
87.535830143754));
#148904=CARTESIAN_POINT('Ctrl Pts',(-13.0687965820832,-78.6991043297429,
87.5257025283007));
#148905=CARTESIAN_POINT('Ctrl Pts',(-13.0786434069086,-78.7456357479416,
87.5137030805226));
#148906=CARTESIAN_POINT('Ctrl Pts',(-13.0889845008086,-78.7945028470755,
87.5011013110768));
#148907=CARTESIAN_POINT('Ctrl Pts',(-13.1009545249819,-78.8503751368275,
87.4864354576878));
#148908=CARTESIAN_POINT('Ctrl Pts',(-13.1146779375454,-78.9131671994993,
87.4694668083806));
#148909=CARTESIAN_POINT('Ctrl Pts',(-13.1284013501089,-78.9759592621712,
87.4524981590734));
#148910=CARTESIAN_POINT('Ctrl Pts',(-13.1438781510625,-79.0456713500959,
87.4332265985393));
#148911=CARTESIAN_POINT('Ctrl Pts',(-13.161232798523,-79.1221945220809,
87.4113549289942));
#148912=CARTESIAN_POINT('Ctrl Pts',(-13.1783109482994,-79.1974985117185,
87.3898317232246));
#148913=CARTESIAN_POINT('Ctrl Pts',(-13.1972368930209,-79.2793960174767,
87.3657911402542));
#148914=CARTESIAN_POINT('Ctrl Pts',(-13.218151617703,-79.3677741621452,
87.338891089315));
#148915=CARTESIAN_POINT('Ctrl Pts',(-13.2390663423851,-79.4561523068137,
87.3119910383758));
#148916=CARTESIAN_POINT('Ctrl Pts',(-13.2619698470278,-79.5510114316163,
87.2822313862799));
#148917=CARTESIAN_POINT('Ctrl Pts',(-13.2870031166466,-79.6522076225808,
87.2492177220848));
#148918=CARTESIAN_POINT('Ctrl Pts',(-13.3106570500547,-79.7478278910742,
87.2180231148154));
#148919=CARTESIAN_POINT('Ctrl Pts',(-13.3362102523045,-79.8491089599361,
87.1839219451345));
#148920=CARTESIAN_POINT('Ctrl Pts',(-13.3637483455945,-79.9559219629347,
87.1465317573033));
#148921=CARTESIAN_POINT('Ctrl Pts',(-13.3653541795417,-79.9621505694112,
87.1443514163379));
#148922=CARTESIAN_POINT('Ctrl Pts',(-13.3669667629672,-79.9683979776324,
87.1421598797651));
#148923=CARTESIAN_POINT('Ctrl Pts',(-13.3685861128491,-79.974664158566,
87.1399570674823));
#148924=CARTESIAN_POINT('Ctrl Pts',(-13.3832807253308,-80.0315259285838,
87.1199678895857));
#148925=CARTESIAN_POINT('Ctrl Pts',(-13.3985319081437,-80.0899341144083,
87.0990503614809));
#148926=CARTESIAN_POINT('Ctrl Pts',(-13.4143477726808,-80.1498678263095,
87.0771419883593));
#148927=CARTESIAN_POINT('Ctrl Pts',(-13.4222557049493,-80.1798346822601,
87.0661878017985));
#148928=CARTESIAN_POINT('Ctrl Pts',(-13.4303048076488,-80.2101828977198,
87.0549858456473));
#148929=CARTESIAN_POINT('Ctrl Pts',(-13.438495672417,-80.2409097575134,
87.0435279416479));
#148930=CARTESIAN_POINT('Ctrl Pts',(-13.4425911048011,-80.2562731874102,
87.0377989896482));
#148931=CARTESIAN_POINT('Ctrl Pts',(-13.4467219777023,-80.2717312769617,
87.0320060469452));
#148932=CARTESIAN_POINT('Ctrl Pts',(-13.4508883493137,-80.2872836790015,
87.0261480683085));
#148933=CARTESIAN_POINT('Ctrl Pts',(-13.4529715351194,-80.2950598800215,
87.0232190789902));
#148934=CARTESIAN_POINT('Ctrl Pts',(-13.4550635956026,-80.3028596590685,
87.0202738304531));
#148935=CARTESIAN_POINT('Ctrl Pts',(-13.4571645363622,-80.310682972302,
87.0173121905769));
#148936=CARTESIAN_POINT('Ctrl Pts',(-13.4592654771218,-80.3185062855355,
87.0143505507008));
#148937=CARTESIAN_POINT('Ctrl Pts',(-13.4618074963136,-80.327958614595,
87.0107616557018));
#148938=CARTESIAN_POINT('Ctrl Pts',(-13.4634940045304,-80.3342234703738,
87.0083779638468));
#148939=CARTESIAN_POINT('Ctrl Pts',(-13.5025360795712,-80.4792526893253,
86.9531963315527));
#148940=CARTESIAN_POINT('Ctrl Pts',(-13.5406679976172,-80.6176638563657,
86.8979602069061));
#148941=CARTESIAN_POINT('Ctrl Pts',(-13.5776553922539,-80.7495778925329,
86.8432155722051));
#148942=CARTESIAN_POINT('Ctrl Pts',(-13.6150631201262,-80.8829910300608,
86.7878488069199));
#148943=CARTESIAN_POINT('Ctrl Pts',(-13.6513001635259,-81.0097589628704,
86.7329848246882));
#148944=CARTESIAN_POINT('Ctrl Pts',(-13.6861240747114,-81.1300193085492,
86.6791363995748));
#148945=CARTESIAN_POINT('Ctrl Pts',(-13.7120606592147,-81.2195883004261,
86.639030501622));
#148946=CARTESIAN_POINT('Ctrl Pts',(-13.7372133570588,-81.3055477211668,
86.5994868643739));
#148947=CARTESIAN_POINT('Ctrl Pts',(-13.7614820014301,-81.387956741055,
86.5606987233784));
#148948=CARTESIAN_POINT('Ctrl Pts',(-13.7942709972533,-81.4992983128203,
86.5082926567835));
#148949=CARTESIAN_POINT('Ctrl Pts',(-13.8254696763634,-81.6041576702389,
86.4572683615342));
#148950=CARTESIAN_POINT('Ctrl Pts',(-13.8550187233761,-81.7026898173829,
86.4080528929969));
#148951=CARTESIAN_POINT('Ctrl Pts',(-13.8847124905224,-81.8017045379744,
86.3585963855803));
#148952=CARTESIAN_POINT('Ctrl Pts',(-13.9127404274452,-81.8943302867114,
86.3109664100033));
#148953=CARTESIAN_POINT('Ctrl Pts',(-13.9390423429716,-81.9807195923339,
86.265543858743));
#148954=CARTESIAN_POINT('Ctrl Pts',(-13.957667695685,-82.0418950335774,
86.2333784813768));
#148955=CARTESIAN_POINT('Ctrl Pts',(-13.9754275217782,-82.0999430662178,
86.2023189351202));
#148956=CARTESIAN_POINT('Ctrl Pts',(-13.9923004473309,-82.154914972983,
86.1724849405017));
#148957=CARTESIAN_POINT('Origin',(-15.5675364833309,-75.,72.98888938658));
#148958=CARTESIAN_POINT('Ctrl Pts',(-13.9922632538729,-67.8450784104129,
86.1724813495793));
#148959=CARTESIAN_POINT('Ctrl Pts',(-14.0172702688094,-67.7636406775926,
86.1282839415892));
#148960=CARTESIAN_POINT('Ctrl Pts',(-14.0444973895826,-67.6769323819869,
86.0802539845106));
#148961=CARTESIAN_POINT('Ctrl Pts',(-14.0739446161924,-67.5851571089398,
86.0280651619461));
#148962=CARTESIAN_POINT('Ctrl Pts',(-14.1032441861568,-67.4938420228274,
85.9761380287613));
#148963=CARTESIAN_POINT('Ctrl Pts',(-14.1347416533126,-67.3975103985407,
85.9200933988725));
#148964=CARTESIAN_POINT('Ctrl Pts',(-14.1684370176596,-67.296401626475,
85.8595759300175));
#148965=CARTESIAN_POINT('Ctrl Pts',(-14.2017938107947,-67.196308795924,
85.7996665410326));
#148966=CARTESIAN_POINT('Ctrl Pts',(-14.2373045540593,-67.0915341169454,
85.7353734611614));
#148967=CARTESIAN_POINT('Ctrl Pts',(-14.2749692474532,-66.9823514351676,
85.6663225451827));
#148968=CARTESIAN_POINT('Ctrl Pts',(-14.3123575914211,-66.8739698370767,
85.5977782623207));
#148969=CARTESIAN_POINT('Ctrl Pts',(-14.3518683939993,-66.7612444428563,
85.5245454041851));
#148970=CARTESIAN_POINT('Ctrl Pts',(-14.3935016551879,-66.6444877606173,
85.4462332133163));
#148971=CARTESIAN_POINT('Ctrl Pts',(-14.4346033139423,-66.5292219088997,
85.3689209669655));
#148972=CARTESIAN_POINT('Ctrl Pts',(-14.4777735752965,-66.4100268721727,
85.2866579311862));
#148973=CARTESIAN_POINT('Ctrl Pts',(-14.5230124392504,-66.2872501238768,
85.1990486646613));
#148974=CARTESIAN_POINT('Ctrl Pts',(-14.544098664004,-66.2300228223309,
85.1582132297502));
#148975=CARTESIAN_POINT('Ctrl Pts',(-14.5656343076739,-66.1720180533392,
85.1162160408558));
#148976=CARTESIAN_POINT('Ctrl Pts',(-14.5876193702598,-66.1132747231402,
85.0730159108109));
#148977=CARTESIAN_POINT('Ctrl Pts',(-14.6338698573215,-65.9896950142947,
84.9821347933299));
#148978=CARTESIAN_POINT('Ctrl Pts',(-14.6821093158676,-65.8628433973624,
84.8859304129358));
#148979=CARTESIAN_POINT('Ctrl Pts',(-14.7323378288026,-65.7331185860723,
84.7840116352132));
#148980=CARTESIAN_POINT('Ctrl Pts',(-14.7818996441456,-65.6051156497544,
84.6834456549301));
#148981=CARTESIAN_POINT('Ctrl Pts',(-14.8333980617202,-65.4743151543327,
84.577315594984));
#148982=CARTESIAN_POINT('Ctrl Pts',(-14.8868331611732,-65.3411504316446,
84.465240070307));
#148983=CARTESIAN_POINT('Ctrl Pts',(-14.9391086331413,-65.2108755973263,
84.3555967645297));
#148984=CARTESIAN_POINT('Ctrl Pts',(-14.9932376408722,-65.0783380079684,
84.2402628757793));
#148985=CARTESIAN_POINT('Ctrl Pts',(-15.049220258939,-64.9439929085543,
84.1188813621743));
#148986=CARTESIAN_POINT('Ctrl Pts',(-15.1044918229534,-64.811354171412,
83.9990415559796));
#148987=CARTESIAN_POINT('Ctrl Pts',(-15.1615702096795,-64.676953472949,
83.8733064025776));
#148988=CARTESIAN_POINT('Ctrl Pts',(-15.2204554908848,-64.5412786150475,
83.7413378050537));
#148989=CARTESIAN_POINT('Ctrl Pts',(-15.2781110133641,-64.4084371874531,
83.6121252363886));
#148990=CARTESIAN_POINT('Ctrl Pts',(-15.3374987481049,-64.2743742884252,
83.4769365119666));
#148991=CARTESIAN_POINT('Ctrl Pts',(-15.3986187624717,-64.1395959885378,
83.335464892892));
#148992=CARTESIAN_POINT('Ctrl Pts',(-15.4535266119418,-64.0185163932739,
83.208372279369));
#148993=CARTESIAN_POINT('Ctrl Pts',(-15.5098325026146,-63.8968599934556,
83.0762089638245));
#148994=CARTESIAN_POINT('Ctrl Pts',(-15.5675364833309,-63.7750278396912,
82.9387637576609));
#148995=CARTESIAN_POINT('Ctrl Pts',(-15.7859374982489,-63.70265213093,82.861383624057));
#148996=CARTESIAN_POINT('Ctrl Pts',(-13.2002732600734,-63.38383560984,82.350395801635));
#148997=CARTESIAN_POINT('Ctrl Pts',(-11.2034697254109,-61.8083020344701,
83.11121227182));
#148998=CARTESIAN_POINT('Ctrl Pts',(-10.7994091717229,-59.76814774659,84.76133204249));
#148999=CARTESIAN_POINT('Ctrl Pts',(-15.2200740724999,-64.90402508323,84.23663134082));
#149000=CARTESIAN_POINT('Ctrl Pts',(-12.7693205181935,-64.50074857368,83.74901632495));
#149001=CARTESIAN_POINT('Ctrl Pts',(-10.8258933224599,-63.11114403357,84.60411552944));
#149002=CARTESIAN_POINT('Ctrl Pts',(-10.2935001377589,-61.38139141585,86.40429721953));
#149003=CARTESIAN_POINT('Ctrl Pts',(-14.6041660747459,-66.38156201951,85.4050021444));
#149004=CARTESIAN_POINT('Ctrl Pts',(-12.2722897776818,-65.95698671183,85.02702776225));
#149005=CARTESIAN_POINT('Ctrl Pts',(-10.3838362619619,-64.78669608641,85.95842638835));
#149006=CARTESIAN_POINT('Ctrl Pts',(-9.74335915314591,-63.36928148601,87.80238251478));
#149007=CARTESIAN_POINT('Ctrl Pts',(-14.1110631602059,-67.99782845316,86.2571636203899));
#149008=CARTESIAN_POINT('Ctrl Pts',(-11.8620763883513,-67.6350035382001,
85.98143506887));
#149009=CARTESIAN_POINT('Ctrl Pts',(-10.0155685768079,-66.69421658395,86.96682116639));
#149010=CARTESIAN_POINT('Ctrl Pts',(-9.30321403080591,-65.54825406424,88.82286146046));
#149011=CARTESIAN_POINT('Origin',(-15.5675402745283,-60.0333674837764,86.255392349124));
#149012=CARTESIAN_POINT('Ctrl Pts',(-10.7041478512819,-60.09386358317,85.0646713926));
#149013=CARTESIAN_POINT('Ctrl Pts',(-10.7993782800689,-60.52820765432,84.69634244083));
#149014=CARTESIAN_POINT('Ctrl Pts',(-11.1849148787739,-61.42183746252,83.9980255694));
#149015=CARTESIAN_POINT('Ctrl Pts',(-12.3843078552043,-62.66523363698,83.23440107119));
#149016=CARTESIAN_POINT('Ctrl Pts',(-14.0046199477159,-63.57750343473,82.906426537614));
#149017=CARTESIAN_POINT('Ctrl Pts',(-15.1626528546819,-63.86437128804,83.00677838687));
#149018=CARTESIAN_POINT('Ctrl Pts',(-15.7241364691869,-63.93250661788,83.12048790153));
#149019=CARTESIAN_POINT('Ctrl Pts',(-10.9677003684169,-59.23917692107,84.23345016192));
#149020=CARTESIAN_POINT('Ctrl Pts',(-11.0441856921629,-59.69432284707,83.89966200941));
#149021=CARTESIAN_POINT('Ctrl Pts',(-11.3853725838139,-60.62794654061,83.26859435449));
#149022=CARTESIAN_POINT('Ctrl Pts',(-12.4999814042177,-61.9296416061,82.572868554654));
#149023=CARTESIAN_POINT('Ctrl Pts',(-14.0404250630399,-62.89957197101,82.257638700836));
#149024=CARTESIAN_POINT('Ctrl Pts',(-15.1678421958949,-63.22153762943,82.32904067551));
#149025=CARTESIAN_POINT('Ctrl Pts',(-15.7218484252699,-63.30516960113,82.422318246836));
#149026=CARTESIAN_POINT('Ctrl Pts',(-11.3522936220239,-58.1404827969,82.865207710886));
#149027=CARTESIAN_POINT('Ctrl Pts',(-11.4036986376399,-58.61682481435,82.583952417586));
#149028=CARTESIAN_POINT('Ctrl Pts',(-11.6848368356737,-59.58954811194,82.054712944551));
#149029=CARTESIAN_POINT('Ctrl Pts',(-12.6807018187587,-60.95041422044,81.466427752057));
#149030=CARTESIAN_POINT('Ctrl Pts',(-14.1030936751929,-61.98838456191,81.183450354301));
#149031=CARTESIAN_POINT('Ctrl Pts',(-15.1787465752679,-62.36041090116,81.223135164807));
#149032=CARTESIAN_POINT('Ctrl Pts',(-15.7172649246479,-62.46838269082,81.291197010499));
#149033=CARTESIAN_POINT('Ctrl Pts',(-11.7927722579691,-57.0209055347,80.87660427494));
#149034=CARTESIAN_POINT('Ctrl Pts',(-11.8176818813139,-57.51258307741,80.664597756629));
#149035=CARTESIAN_POINT('Ctrl Pts',(-12.0347761979652,-58.51132096518,80.267386771243));
#149036=CARTESIAN_POINT('Ctrl Pts',(-12.900196635276,-59.91385972122,79.821483937711));
#149037=CARTESIAN_POINT('Ctrl Pts',(-14.1863686741569,-61.01129527968,79.593672952375));
#149038=CARTESIAN_POINT('Ctrl Pts',(-15.1950629340279,-61.43683394942,79.60664069943));
#149039=CARTESIAN_POINT('Ctrl Pts',(-15.7105937362879,-61.57320926475,79.649025591868));
#149040=CARTESIAN_POINT('Ctrl Pts',(-12.0661314106457,-56.37283617373,79.38235543526));
#149041=CARTESIAN_POINT('Ctrl Pts',(-12.0758434847391,-56.87031895131,79.218299414597));
#149042=CARTESIAN_POINT('Ctrl Pts',(-12.255568884686,-57.87753552957,78.911808500822));
#149043=CARTESIAN_POINT('Ctrl Pts',(-13.0422585423339,-59.29546209928,78.565409307254));
#149044=CARTESIAN_POINT('Ctrl Pts',(-14.2430805630429,-60.42240614723,78.381490093937));
#149045=CARTESIAN_POINT('Ctrl Pts',(-15.2068409041219,-60.87953638866,78.382502187017));
#149046=CARTESIAN_POINT('Ctrl Pts',(-15.7058387404459,-61.0336884742,78.410472854166));
#149047=CARTESIAN_POINT('Ctrl Pts',(-12.2840775879539,-55.88110902617,77.838409205923));
#149048=CARTESIAN_POINT('Ctrl Pts',(-12.2827124321547,-56.38084424398,77.718226582429));
#149049=CARTESIAN_POINT('Ctrl Pts',(-12.4345336551895,-57.3898254788,77.49440046578));
#149050=CARTESIAN_POINT('Ctrl Pts',(-13.1600193818496,-58.81285577353,77.240660890849));
#149051=CARTESIAN_POINT('Ctrl Pts',(-14.2920472090029,-59.95780874928,77.102673904364));
#149052=CARTESIAN_POINT('Ctrl Pts',(-15.2174560511349,-60.43844112167,77.099030649501));
#149053=CARTESIAN_POINT('Ctrl Pts',(-15.7015914388329,-60.60654655031,77.117122227125));
#149054=CARTESIAN_POINT('Ctrl Pts',(-12.4455223641938,-55.53147356832,76.248194310692));
#149055=CARTESIAN_POINT('Ctrl Pts',(-12.4364409723141,-56.03153659583,76.169508058991));
#149056=CARTESIAN_POINT('Ctrl Pts',(-12.5684953465771,-57.03906368194,76.023333781968));
#149057=CARTESIAN_POINT('Ctrl Pts',(-13.2494610073287,-58.46199397328,75.857320665731));
#149058=CARTESIAN_POINT('Ctrl Pts',(-14.3302328652499,-59.61727660643,75.76553819577));
#149059=CARTESIAN_POINT('Ctrl Pts',(-15.2259605578989,-60.11434751671,75.761106780194));
#149060=CARTESIAN_POINT('Ctrl Pts',(-15.6982072375269,-60.29264234043,75.771817510397));
#149061=CARTESIAN_POINT('Ctrl Pts',(-12.5457498999123,-55.32390979009,74.632044951833));
#149062=CARTESIAN_POINT('Ctrl Pts',(-12.5323125837539,-55.82305995791,74.593269618371));
#149063=CARTESIAN_POINT('Ctrl Pts',(-12.6528329390154,-56.82750771549,74.521337406159));
#149064=CARTESIAN_POINT('Ctrl Pts',(-13.3066685414211,-58.24764282185,74.439492266471));
#149065=CARTESIAN_POINT('Ctrl Pts',(-14.3552787532369,-59.40754337176,74.393701806354));
#149066=CARTESIAN_POINT('Ctrl Pts',(-15.2316755631149,-59.91449324558,74.390782624317));
#149067=CARTESIAN_POINT('Ctrl Pts',(-15.6959440082919,-60.09919481949,74.39565266482));
#149068=CARTESIAN_POINT('Ctrl Pts',(-12.5810013147727,-55.25465453146,73.0095737856597));
#149069=CARTESIAN_POINT('Ctrl Pts',(-12.5662393202892,-55.75295766122,73.0090978203629));
#149070=CARTESIAN_POINT('Ctrl Pts',(-12.6830375165281,-56.75533192764,73.0082135404681));
#149071=CARTESIAN_POINT('Ctrl Pts',(-13.3275136480566,-58.17334349545,73.0071997776312));
#149072=CARTESIAN_POINT('Ctrl Pts',(-14.3646256854699,-59.33424330126,73.0066206299221));
#149073=CARTESIAN_POINT('Ctrl Pts',(-15.2338545192429,-59.84467210232,73.0065694532389));
#149074=CARTESIAN_POINT('Ctrl Pts',(-15.6950847124779,-60.03173379517,73.0066211743601));
#149075=CARTESIAN_POINT('Ctrl Pts',(-12.5475045162963,-55.32017430335,71.387087839408));
#149076=CARTESIAN_POINT('Ctrl Pts',(-12.533981149037,-55.8193273013,71.424862343681));
#149077=CARTESIAN_POINT('Ctrl Pts',(-12.654283968606,-56.82375706032,71.494940544456));
#149078=CARTESIAN_POINT('Ctrl Pts',(-13.3076377377326,-58.24388402961,71.574696849883));
#149079=CARTESIAN_POINT('Ctrl Pts',(-14.3556951419789,-59.4038845339,71.619353265881));
#149080=CARTESIAN_POINT('Ctrl Pts',(-15.2317691498139,-59.91100278183,71.622241360802));
#149081=CARTESIAN_POINT('Ctrl Pts',(-15.6959068347219,-60.0958104599,71.61752019893));
#149082=CARTESIAN_POINT('Ctrl Pts',(-12.4158905694987,-55.59282803409,69.229401204407));
#149083=CARTESIAN_POINT('Ctrl Pts',(-12.4081109279248,-56.09315502217,69.320374998153));
#149084=CARTESIAN_POINT('Ctrl Pts',(-12.5435994725067,-57.10157402003,69.489396119942));
#149085=CARTESIAN_POINT('Ctrl Pts',(-13.2325997356449,-58.52529383771,69.681292799115));
#149086=CARTESIAN_POINT('Ctrl Pts',(-14.3228650735119,-59.67918060652,69.787209745794));
#149087=CARTESIAN_POINT('Ctrl Pts',(-15.2242815937599,-60.17332252705,69.792102588723));
#149088=CARTESIAN_POINT('Ctrl Pts',(-15.6988723085229,-60.34972220064,69.779595279849));
#149089=CARTESIAN_POINT('Ctrl Pts',(-12.0984815213225,-56.28453201346,66.598496595256));
#149090=CARTESIAN_POINT('Ctrl Pts',(-12.1059032952083,-56.78383432926,66.759784999304));
#149091=CARTESIAN_POINT('Ctrl Pts',(-12.2803121570357,-57.79442431143,67.060817730495));
#149092=CARTESIAN_POINT('Ctrl Pts',(-13.0569396205602,-59.21756273984,67.402062653449));
#149093=CARTESIAN_POINT('Ctrl Pts',(-14.2480069695899,-60.35063110239,67.586009442708));
#149094=CARTESIAN_POINT('Ctrl Pts',(-15.2076486671699,-60.8123315191,67.588584775643));
#149095=CARTESIAN_POINT('Ctrl Pts',(-15.7054941595619,-60.96870853934,67.562980380674));
#149096=CARTESIAN_POINT('Ctrl Pts',(-11.4801382308969,-57.77429967396,63.567629022451));
#149097=CARTESIAN_POINT('Ctrl Pts',(-11.5230945717649,-58.25793556693,63.831385556471));
#149098=CARTESIAN_POINT('Ctrl Pts',(-11.784103413135,-59.24408794518,64.326760510344));
#149099=CARTESIAN_POINT('Ctrl Pts',(-12.7404495534908,-60.62500522954,64.879476066085));
#149100=CARTESIAN_POINT('Ctrl Pts',(-14.1237202044219,-61.68566477043,65.151993286447));
#149101=CARTESIAN_POINT('Ctrl Pts',(-15.1823110544269,-62.07418257557,65.123079900673));
#149102=CARTESIAN_POINT('Ctrl Pts',(-15.7157641330979,-62.19013200718,65.063526526587));
#149103=CARTESIAN_POINT('Ctrl Pts',(-10.9713079387679,-59.2277623056,61.75592042875));
#149104=CARTESIAN_POINT('Ctrl Pts',(-11.0475501095339,-59.68314485839,62.08924479198));
#149105=CARTESIAN_POINT('Ctrl Pts',(-11.3881525214239,-60.61722479436,62.71941099542));
#149106=CARTESIAN_POINT('Ctrl Pts',(-12.5016155027438,-61.91961304936,63.414226922204));
#149107=CARTESIAN_POINT('Ctrl Pts',(-14.0409546878489,-62.89027630592,63.729283079577));
#149108=CARTESIAN_POINT('Ctrl Pts',(-15.1679259362799,-63.21272241284,63.65826525009));
#149109=CARTESIAN_POINT('Ctrl Pts',(-15.7218123616389,-63.29657498626,63.565259667224));
#149110=CARTESIAN_POINT('Ctrl Pts',(-10.7040595554379,-60.0941142792,60.91280126868));
#149111=CARTESIAN_POINT('Ctrl Pts',(-10.7992944412109,-60.52845915509,61.28113961178));
#149112=CARTESIAN_POINT('Ctrl Pts',(-11.1848427857719,-61.42209035945,61.97947395869));
#149113=CARTESIAN_POINT('Ctrl Pts',(-12.3842618607264,-62.66548448627,62.7431137798));
#149114=CARTESIAN_POINT('Ctrl Pts',(-14.0046020364749,-63.57774528311,63.071087750167));
#149115=CARTESIAN_POINT('Ctrl Pts',(-15.1626491571459,-63.86460259476,62.97072528602));
#149116=CARTESIAN_POINT('Ctrl Pts',(-15.7241379640389,-63.9327320353,62.85700885034));
#149117=CARTESIAN_POINT('Origin',(-15.5675364833322,-60.0333704528863,59.7223902251838));
#149118=CARTESIAN_POINT('Ctrl Pts',(-14.1109587916119,-67.99806761864,59.72048255862));
#149119=CARTESIAN_POINT('Ctrl Pts',(-11.8622349709499,-67.6352743646101,
59.9961606353001));
#149120=CARTESIAN_POINT('Ctrl Pts',(-10.0158495894229,-66.69465820612,59.0109757487901));
#149121=CARTESIAN_POINT('Ctrl Pts',(-9.30331679897591,-65.5488541427201,
57.15519830438));
#149122=CARTESIAN_POINT('Ctrl Pts',(-14.6029404122129,-66.3855391917801,
60.57083234018));
#149123=CARTESIAN_POINT('Ctrl Pts',(-12.2714944067202,-65.96131004996,60.94839266561));
#149124=CARTESIAN_POINT('Ctrl Pts',(-10.3832434550279,-64.79176598389,60.0170714877401));
#149125=CARTESIAN_POINT('Ctrl Pts',(-9.74244088945891,-63.37501002094,58.17348929348));
#149126=CARTESIAN_POINT('Ctrl Pts',(-15.2156776004529,-64.91333674655,61.73072156537));
#149127=CARTESIAN_POINT('Ctrl Pts',(-12.7662414190393,-64.50943479782,62.21808717786));
#149128=CARTESIAN_POINT('Ctrl Pts',(-10.8233228751789,-63.12150890318,61.36245727412));
#149129=CARTESIAN_POINT('Ctrl Pts',(-10.2896898327509,-61.39440175993,59.56133749228));
#149130=CARTESIAN_POINT('Ctrl Pts',(-15.7859912232719,-63.70246439342,63.116600358883));
#149131=CARTESIAN_POINT('Ctrl Pts',(-13.2006081304612,-63.38367271774,63.627536549936));
#149132=CARTESIAN_POINT('Ctrl Pts',(-11.2038952684519,-61.8083637843599,
62.8669303902801));
#149133=CARTESIAN_POINT('Ctrl Pts',(-10.7995805712549,-59.76836009227,61.21707043588));
#149134=CARTESIAN_POINT('',(-13.9922553804024,-67.8450769206476,59.8052980196146));
#149135=CARTESIAN_POINT('Origin',(-13.9922814999513,-65.4601089597576,55.4107645745232));
#149136=CARTESIAN_POINT('Ctrl Pts',(-15.5675364833309,-63.775027839677,
63.0390150155114));
#149137=CARTESIAN_POINT('Ctrl Pts',(-15.5486560109279,-63.8156900744696,
62.9931418279215));
#149138=CARTESIAN_POINT('Ctrl Pts',(-15.5276796743979,-63.8610333030251,
62.9425581622453));
#149139=CARTESIAN_POINT('Ctrl Pts',(-15.504601517406,-63.9112558109,62.8874513628923));
#149140=CARTESIAN_POINT('Ctrl Pts',(-15.4815962090432,-63.9613197861483,
62.8325185139455));
#149141=CARTESIAN_POINT('Ctrl Pts',(-15.4565020002374,-64.016232557767,
62.7730908821243));
#149142=CARTESIAN_POINT('Ctrl Pts',(-15.429319211093,-64.0762215379075,
62.7093948971326));
#149143=CARTESIAN_POINT('Ctrl Pts',(-15.4195418942773,-64.097798840412,
62.686484230319));
#149144=CARTESIAN_POINT('Ctrl Pts',(-15.4094944497678,-64.1200331503125,
62.6630217404487));
#149145=CARTESIAN_POINT('Ctrl Pts',(-15.3991772236595,-64.1429359253291,
62.6390193286406));
#149146=CARTESIAN_POINT('Ctrl Pts',(-15.3671474528508,-64.2140374624055,
62.5645039752888));
#149147=CARTESIAN_POINT('Ctrl Pts',(-15.3324052214448,-64.2918409859351,
62.4845101324438));
#149148=CARTESIAN_POINT('Ctrl Pts',(-15.2950981599505,-64.3763510127759,
62.3998250092134));
#149149=CARTESIAN_POINT('Ctrl Pts',(-15.2583555496539,-64.4595824134272,
62.3164211613588));
#149150=CARTESIAN_POINT('Ctrl Pts',(-15.2191246511704,-64.5493200493604,
62.228467495124));
#149151=CARTESIAN_POINT('Ctrl Pts',(-15.177580101105,-64.6455612701451,
62.1367522446501));
#149152=CARTESIAN_POINT('Ctrl Pts',(-15.1720477058737,-64.6583774992313,
62.1245387289529));
#149153=CARTESIAN_POINT('Ctrl Pts',(-15.1664743364701,-64.6713090363615,
62.1122585525923));
#149154=CARTESIAN_POINT('Ctrl Pts',(-15.1608604577245,-64.6843558498199,
62.0999136179658));
#149155=CARTESIAN_POINT('Ctrl Pts',(-15.1243743065958,-64.7691507000761,
62.0196804724232));
#149156=CARTESIAN_POINT('Ctrl Pts',(-15.0897314949321,-64.8506403030421,
61.9444417012586));
#149157=CARTESIAN_POINT('Ctrl Pts',(-15.0569457220555,-64.9285380674421,
61.8739305478222));
#149158=CARTESIAN_POINT('Ctrl Pts',(-15.0233657115331,-65.0083229106442,
61.8017112567521));
#149159=CARTESIAN_POINT('Ctrl Pts',(-14.9917334822288,-65.0843399044684,
61.7344511114654));
#149160=CARTESIAN_POINT('Ctrl Pts',(-14.9620434453303,-65.1563274476019,
61.671884384849));
#149161=CARTESIAN_POINT('Ctrl Pts',(-14.9487610463081,-65.1885324352816,
61.6438939774516));
#149162=CARTESIAN_POINT('Ctrl Pts',(-14.9358671186469,-65.2199315701482,
61.616843208052));
#149163=CARTESIAN_POINT('Ctrl Pts',(-14.9233601493996,-65.2505042236718,
61.5907098279098));
#149164=CARTESIAN_POINT('Ctrl Pts',(-14.8947732166026,-65.3203835345124,
61.5309772766328));
#149165=CARTESIAN_POINT('Ctrl Pts',(-14.8682163869933,-65.3859411515636,
61.47603640133));
#149166=CARTESIAN_POINT('Ctrl Pts',(-14.8436906166197,-65.44695781362,61.4256453742038));
#149167=CARTESIAN_POINT('Ctrl Pts',(-14.8391498514624,-65.4582545977317,
61.4163158478838));
#149168=CARTESIAN_POINT('Ctrl Pts',(-14.8346786770759,-65.4693958425011,
61.4071423621721));
#149169=CARTESIAN_POINT('Ctrl Pts',(-14.8302770628544,-65.4803803100542,
61.3981234958639));
#149170=CARTESIAN_POINT('Ctrl Pts',(-14.8161891644792,-65.5155374262401,
61.3692575240608));
#149171=CARTESIAN_POINT('Ctrl Pts',(-14.8028142414204,-65.5490881151195,
61.3419752144693));
#149172=CARTESIAN_POINT('Ctrl Pts',(-14.7901522947983,-65.5809946859591,
61.3162327255843));
#149173=CARTESIAN_POINT('Ctrl Pts',(-14.7838213214872,-65.5969479713789,
61.3033614811419));
#149174=CARTESIAN_POINT('Ctrl Pts',(-14.7776685923084,-65.6124902860436,
61.2908752655851));
#149175=CARTESIAN_POINT('Ctrl Pts',(-14.7716941073786,-65.627617355836,
61.2787689719339));
#149176=CARTESIAN_POINT('Ctrl Pts',(-14.7687068649137,-65.6351808907321,
61.2727158251082));
#149177=CARTESIAN_POINT('Ctrl Pts',(-14.7657641835125,-65.6426406181008,
61.2667576633422));
#149178=CARTESIAN_POINT('Ctrl Pts',(-14.7628660631932,-65.6499960269563,
61.260893874795));
#149179=CARTESIAN_POINT('Ctrl Pts',(-14.7614170030336,-65.6536737313841,
61.2579619805214));
#149180=CARTESIAN_POINT('Ctrl Pts',(-14.7599790831445,-65.657325356411,
61.2550536798404));
#149181=CARTESIAN_POINT('Ctrl Pts',(-14.7585523035282,-65.6609508397835,
61.2521688977952));
#149182=CARTESIAN_POINT('Ctrl Pts',(-14.75783891372,-65.6627635814697,61.2507265067726));
#149183=CARTESIAN_POINT('Ctrl Pts',(-14.75712830898,-65.6645697877565,61.249289995427));
#149184=CARTESIAN_POINT('Ctrl Pts',(-14.7564204893085,-65.6663694509628,
61.2478593544845));
#149185=CARTESIAN_POINT('Ctrl Pts',(-14.7557126696371,-65.6681691141691,
61.246428713542));
#149186=CARTESIAN_POINT('Ctrl Pts',(-14.7555273948954,-65.6686399307073,
61.2460541282831));
#149187=CARTESIAN_POINT('Ctrl Pts',(-14.7543053854998,-65.6717488037198,
61.2435850336611));
#149188=CARTESIAN_POINT('Ctrl Pts',(-14.7009716673493,-65.8074333226892,
61.1358231808213));
#149189=CARTESIAN_POINT('Ctrl Pts',(-14.6492741378672,-65.9416405763828,
61.0330309177387));
#149190=CARTESIAN_POINT('Ctrl Pts',(-14.5992805060834,-66.0740270455773,
60.9349368939584));
#149191=CARTESIAN_POINT('Ctrl Pts',(-14.5480365872424,-66.2097243582351,
60.834389643958));
#149192=CARTESIAN_POINT('Ctrl Pts',(-14.4985826667428,-66.3435087517832,
60.7387783956766));
#149193=CARTESIAN_POINT('Ctrl Pts',(-14.4509563393972,-66.4750525354945,
60.6478083689958));
#149194=CARTESIAN_POINT('Ctrl Pts',(-14.4013843434623,-66.6119702504397,
60.5531219624608));
#149195=CARTESIAN_POINT('Ctrl Pts',(-14.3537921692459,-66.7464605320466,
60.4634635300441));
#149196=CARTESIAN_POINT('Ctrl Pts',(-14.3081869089074,-66.8781987461111,
60.3785008789946));
#149197=CARTESIAN_POINT('Ctrl Pts',(-14.2614817556639,-67.0131141797742,
60.2914891262324));
#149198=CARTESIAN_POINT('Ctrl Pts',(-14.2168602310794,-67.1451433252664,
60.2094021511291));
#149199=CARTESIAN_POINT('Ctrl Pts',(-14.1742971125142,-67.2739825744216,
60.1318868147313));
#149200=CARTESIAN_POINT('Ctrl Pts',(-14.1301511161401,-67.4076132203373,
60.0514887641441));
#149201=CARTESIAN_POINT('Ctrl Pts',(-14.0882192053369,-67.5378123569951,
59.9760084098408));
#149202=CARTESIAN_POINT('Ctrl Pts',(-14.0484424922265,-67.6642878599627,
59.9050597858963));
#149203=CARTESIAN_POINT('Ctrl Pts',(-14.0292131234284,-67.7254302696874,
59.8707608921751));
#149204=CARTESIAN_POINT('Ctrl Pts',(-14.0104870165509,-67.7857031151876,
59.8375212431477));
#149205=CARTESIAN_POINT('Ctrl Pts',(-13.9922553803942,-67.84507700969,59.8052981836874));
#149206=CARTESIAN_POINT('Origin',(-15.5675364833309,-75.,72.98888938658));
#149207=CARTESIAN_POINT('',(-13.992324693093,-82.1549107482684,59.80529132868));
#149208=CARTESIAN_POINT('Ctrl Pts',(-13.9923246930889,-82.1549106597401,
59.8052914918042));
#149209=CARTESIAN_POINT('Ctrl Pts',(-14.0326498230923,-82.2862352156339,
59.8765630424347));
#149210=CARTESIAN_POINT('Ctrl Pts',(-14.0753636476136,-82.4216623800802,
59.9525976352346));
#149211=CARTESIAN_POINT('Ctrl Pts',(-14.1204661666528,-82.5608583504549,
60.0338355077126));
#149212=CARTESIAN_POINT('Ctrl Pts',(-14.164833681325,-82.6977859409637,
60.1137495031144));
#149213=CARTESIAN_POINT('Ctrl Pts',(-14.2115126710949,-82.8383606652471,
60.1986989265006));
#149214=CARTESIAN_POINT('Ctrl Pts',(-14.2605031359626,-82.9822165051163,
60.2891169608454));
#149215=CARTESIAN_POINT('Ctrl Pts',(-14.2838382988673,-83.0507379912303,
60.3321849245127));
#149216=CARTESIAN_POINT('Ctrl Pts',(-14.3076978920675,-83.1200031737454,
60.376493789032));
#149217=CARTESIAN_POINT('Ctrl Pts',(-14.3320819155632,-83.189968386651,
60.4220911537103));
#149218=CARTESIAN_POINT('Ctrl Pts',(-14.3821603647954,-83.3336587568286,
60.5157362944545));
#149219=CARTESIAN_POINT('Ctrl Pts',(-14.4344507817197,-83.4803050486517,
60.6148159552382));
#149220=CARTESIAN_POINT('Ctrl Pts',(-14.4889531663359,-83.629491646429,
60.7197462248017));
#149221=CARTESIAN_POINT('Ctrl Pts',(-14.5038961495022,-83.6703943121549,
60.7485150807473));
#149222=CARTESIAN_POINT('Ctrl Pts',(-14.5190054059185,-83.7114876322699,
60.7777237429279));
#149223=CARTESIAN_POINT('Ctrl Pts',(-14.5342809355846,-83.7527623504291,
60.807380808538));
#149224=CARTESIAN_POINT('Ctrl Pts',(-14.5697763505206,-83.8486715123008,
60.8762942847067));
#149225=CARTESIAN_POINT('Ctrl Pts',(-14.6061695545896,-83.9455607506708,
60.9476289427235));
#149226=CARTESIAN_POINT('Ctrl Pts',(-14.6434605477914,-84.0433074223558,
61.0214923903754));
#149227=CARTESIAN_POINT('Ctrl Pts',(-14.6621060443923,-84.0921807581983,
61.0584241142014));
#149228=CARTESIAN_POINT('Ctrl Pts',(-14.6809759882764,-84.1412684034276,
61.0959880996756));
#149229=CARTESIAN_POINT('Ctrl Pts',(-14.7000703794438,-84.1905540445187,
61.1341976421785));
#149230=CARTESIAN_POINT('Ctrl Pts',(-14.7096175750275,-84.2151968650643,
61.15330241343));
#149231=CARTESIAN_POINT('Ctrl Pts',(-14.719220882432,-84.2398891817751,
61.1725685777272));
#149232=CARTESIAN_POINT('Ctrl Pts',(-14.7288803016573,-84.2646289158787,
61.1919978023081));
#149233=CARTESIAN_POINT('Ctrl Pts',(-14.7337100112699,-84.2769987829305,
61.2017124145986));
#149234=CARTESIAN_POINT('Ctrl Pts',(-14.7385537488377,-84.2893805041449,
61.2114677921951));
#149235=CARTESIAN_POINT('Ctrl Pts',(-14.7434115143608,-84.3017738161273,
61.2212641429886));
#149236=CARTESIAN_POINT('Ctrl Pts',(-14.7470548385031,-84.3110688001141,
61.2286114060838));
#149237=CARTESIAN_POINT('Ctrl Pts',(-14.7507060533702,-84.3203703038928,
61.2359817166214));
#149238=CARTESIAN_POINT('Ctrl Pts',(-14.7543651589621,-84.3296782155313,
61.2433751622201));
#149239=CARTESIAN_POINT('Ctrl Pts',(-14.755584860826,-84.3327808527442,
61.2458396440863));
#149240=CARTESIAN_POINT('Ctrl Pts',(-14.7573339681262,-84.3372273399798,
61.2493753137917));
#149241=CARTESIAN_POINT('Ctrl Pts',(-14.7580268947955,-84.3389882589171,
61.2507763227265));
#149242=CARTESIAN_POINT('Ctrl Pts',(-14.7768365894209,-84.386788912201,
61.2888071150147));
#149243=CARTESIAN_POINT('Ctrl Pts',(-14.7977293784119,-84.4394960083863,
61.3312128540246));
#149244=CARTESIAN_POINT('Ctrl Pts',(-14.8207052617688,-84.4969374834265,
61.3781969681284));
#149245=CARTESIAN_POINT('Ctrl Pts',(-14.8436265989847,-84.5542425889202,
61.425069539095));
#149246=CARTESIAN_POINT('Ctrl Pts',(-14.8686211515223,-84.6162597920851,
61.4764989573845));
#149247=CARTESIAN_POINT('Ctrl Pts',(-14.8956889193815,-84.6827791928586,
61.532721305483));
#149248=CARTESIAN_POINT('Ctrl Pts',(-14.9054580666535,-84.7067870026634,
61.5530127606711));
#149249=CARTESIAN_POINT('Ctrl Pts',(-14.9154972693076,-84.7313808828853,
61.5739288477366));
#149250=CARTESIAN_POINT('Ctrl Pts',(-14.9258065273436,-84.7565496415734,
61.5954816833722));
#149251=CARTESIAN_POINT('Ctrl Pts',(-14.9613055287583,-84.8432159949767,
61.6696969314578));
#149252=CARTESIAN_POINT('Ctrl Pts',(-15.0001623842594,-84.9370814084717,
61.7517856729689));
#149253=CARTESIAN_POINT('Ctrl Pts',(-15.0421313229565,-85.0370242993539,
61.8417757146836));
#149254=CARTESIAN_POINT('Ctrl Pts',(-15.0799715589912,-85.1271352885374,
61.9229129682091));
#149255=CARTESIAN_POINT('Ctrl Pts',(-15.1203416923637,-85.2221854894093,
62.0104747748732));
#149256=CARTESIAN_POINT('Ctrl Pts',(-15.1630615839724,-85.3213168395165,
62.1044776570324));
#149257=CARTESIAN_POINT('Ctrl Pts',(-15.2011471370805,-85.4096942243133,
62.1882829202475));
#149258=CARTESIAN_POINT('Ctrl Pts',(-15.2372063400547,-85.4924235671457,
62.2687710769314));
#149259=CARTESIAN_POINT('Ctrl Pts',(-15.271239192895,-85.5697904373298,
62.3456037044735));
#149260=CARTESIAN_POINT('Ctrl Pts',(-15.3055305040041,-85.6477448605887,
62.4230198278512));
#149261=CARTESIAN_POINT('Ctrl Pts',(-15.3377645703823,-85.7202553698275,
62.4967248514297));
#149262=CARTESIAN_POINT('Ctrl Pts',(-15.3679413920297,-85.7875924641561,
62.5664209252565));
#149263=CARTESIAN_POINT('Ctrl Pts',(-15.3982064291167,-85.8551264039793,
62.6363207405465));
#149264=CARTESIAN_POINT('Ctrl Pts',(-15.4264021760685,-85.917456901521,
62.7021883246434));
#149265=CARTESIAN_POINT('Ctrl Pts',(-15.4525286328851,-85.9748308097405,
62.7637689130809));
#149266=CARTESIAN_POINT('Ctrl Pts',(-15.4787359078586,-86.0323821952792,
62.8255399915529));
#149267=CARTESIAN_POINT('Ctrl Pts',(-15.5028610708378,-86.0849465067054,
62.8829976855202));
#149268=CARTESIAN_POINT('Ctrl Pts',(-15.5249041218226,-86.1327430496248,
62.9359280223336));
#149269=CARTESIAN_POINT('Ctrl Pts',(-15.540118771326,-86.1657333851503,
62.9724618271717));
#149270=CARTESIAN_POINT('Ctrl Pts',(-15.554341482711,-86.1964516844456,
63.006839651937));
#149271=CARTESIAN_POINT('Ctrl Pts',(-15.5675722559773,-86.2249610151766,
63.0390024421084));
#149272=CARTESIAN_POINT('Ctrl Pts',(-13.9923246931012,-82.1549108584552,
59.8052911256458));
#149273=CARTESIAN_POINT('Ctrl Pts',(-13.8764053214032,-81.7772458110216,
59.6003274086972));
#149274=CARTESIAN_POINT('Ctrl Pts',(-13.759594104912,-81.3911404276565,
59.4119043240187));
#149275=CARTESIAN_POINT('Ctrl Pts',(-13.6461287874938,-80.998246292647,
59.2404767632645));
#149276=CARTESIAN_POINT('Ctrl Pts',(-13.5955968116095,-80.8232702082617,
59.1641312017921));
#149277=CARTESIAN_POINT('Ctrl Pts',(-13.5457287373038,-80.6469483273635,
59.091156658539));
#149278=CARTESIAN_POINT('Ctrl Pts',(-13.4969004303083,-80.4694293652599,
59.0215935397703));
#149279=CARTESIAN_POINT('Ctrl Pts',(-13.4891180900334,-80.4411360851249,
59.0105064492247));
#149280=CARTESIAN_POINT('Ctrl Pts',(-13.4813621647133,-80.4128123990875,
58.9995060170376));
#149281=CARTESIAN_POINT('Ctrl Pts',(-13.4736342771085,-80.3844581946216,
58.9885923464971));
#149282=CARTESIAN_POINT('Ctrl Pts',(-13.3910906411719,-80.0815993474981,
58.8720205103256));
#149283=CARTESIAN_POINT('Ctrl Pts',(-13.3117448569047,-79.7752576428201,
58.76534781653));
#149284=CARTESIAN_POINT('Ctrl Pts',(-13.2375806890342,-79.4653029779942,
58.6686969596962));
#149285=CARTESIAN_POINT('Ctrl Pts',(-13.200498605099,-79.3103256455813,
58.6203715312792));
#149286=CARTESIAN_POINT('Ctrl Pts',(-13.1647119249596,-79.1544451175713,
58.5745514140121));
#149287=CARTESIAN_POINT('Ctrl Pts',(-13.1304700378892,-78.9976463931186,
58.5312511229017));
#149288=CARTESIAN_POINT('Ctrl Pts',(-13.1133490943541,-78.9192470308923,
58.5096009773465));
#149289=CARTESIAN_POINT('Ctrl Pts',(-13.0966143490608,-78.8406181238311,
58.4885807747893));
#149290=CARTESIAN_POINT('Ctrl Pts',(-13.0802970349933,-78.7617578322529,
58.468192245756));
#149291=CARTESIAN_POINT('Ctrl Pts',(-13.0761874678022,-78.7418966182315,
58.4630573301907));
#149292=CARTESIAN_POINT('Ctrl Pts',(-13.0721043779967,-78.7220207273617,
58.4579624813401));
#149293=CARTESIAN_POINT('Ctrl Pts',(-13.0680482612186,-78.7021301359867,
58.4529077276365));
#149294=CARTESIAN_POINT('Ctrl Pts',(-13.0640518352002,-78.6825322591894,
58.4479273608663));
#149295=CARTESIAN_POINT('Ctrl Pts',(-13.0600815941711,-78.6629201113842,
58.4429859178198));
#149296=CARTESIAN_POINT('Ctrl Pts',(-13.0561378076375,-78.6432939594342,
58.4380834580874));
#149297=CARTESIAN_POINT('Ctrl Pts',(-13.0521645688367,-78.623521239036,
58.4331443866995));
#149298=CARTESIAN_POINT('Ctrl Pts',(-13.0482182337873,-78.6037342324225,
58.4282448649682));
#149299=CARTESIAN_POINT('Ctrl Pts',(-13.0442990168641,-78.5839332966098,
58.4233849750262));
#149300=CARTESIAN_POINT('Ctrl Pts',(-13.0423394084025,-78.5740328287034,
58.4209550300552));
#149301=CARTESIAN_POINT('Ctrl Pts',(-13.0403865794723,-78.5641288785112,
58.4185349929956));
#149302=CARTESIAN_POINT('Ctrl Pts',(-13.0384405700567,-78.5542214726372,
58.4161248695598));
#149303=CARTESIAN_POINT('Ctrl Pts',(-13.036981062995,-78.5467909182318,
58.4143172769829));
#149304=CARTESIAN_POINT('Ctrl Pts',(-13.0355253919102,-78.5393584200044,
58.4125152608217));
#149305=CARTESIAN_POINT('Ctrl Pts',(-13.034073571557,-78.5319239920785,
58.4107188242082));
#149306=CARTESIAN_POINT('Ctrl Pts',(-13.0335896314393,-78.5294458494366,
58.4101200120037));
#149307=CARTESIAN_POINT('Ctrl Pts',(-13.0328644451769,-78.5257275292609,
58.4092228702754));
#149308=CARTESIAN_POINT('Ctrl Pts',(-13.0326230353278,-78.5244889214428,
58.4089242475597));
#149309=CARTESIAN_POINT('Ctrl Pts',(-13.0200682121633,-78.460073562334,
58.3933939972347));
#149310=CARTESIAN_POINT('Ctrl Pts',(-13.0065976875759,-78.3901336774366,
58.3769827524417));
#149311=CARTESIAN_POINT('Ctrl Pts',(-12.9923806697727,-78.31460200394,58.3599205538385));
#149312=CARTESIAN_POINT('Ctrl Pts',(-12.9777555199851,-78.2369020211531,
58.3423685458343));
#149313=CARTESIAN_POINT('Ctrl Pts',(-12.9623398683733,-78.1532842847873,
58.3241273990271));
#149314=CARTESIAN_POINT('Ctrl Pts',(-12.9463600484581,-78.0636753035669,
58.3054893939602));
#149315=CARTESIAN_POINT('Ctrl Pts',(-12.9315695409071,-77.9807355507775,
58.2882385390605));
#149316=CARTESIAN_POINT('Ctrl Pts',(-12.9162959040133,-77.8926629407206,
58.2706480744648));
#149317=CARTESIAN_POINT('Ctrl Pts',(-12.9007554028391,-77.7994028167243,
58.2529831582825));
#149318=CARTESIAN_POINT('Ctrl Pts',(-12.8855314124791,-77.7080421062309,
58.2356780205231));
#149319=CARTESIAN_POINT('Ctrl Pts',(-12.8700511623901,-77.61170279788,58.218301470208));
#149320=CARTESIAN_POINT('Ctrl Pts',(-12.8545549880426,-77.510340523674,
58.2011336697347));
#149321=CARTESIAN_POINT('Ctrl Pts',(-12.8393842755942,-77.4111071335083,
58.1843264398654));
#149322=CARTESIAN_POINT('Ctrl Pts',(-12.8241981560509,-77.3070593267112,
58.1677193176427));
#149323=CARTESIAN_POINT('Ctrl Pts',(-12.8092601697167,-77.1981656687249,
58.1516045550749));
#149324=CARTESIAN_POINT('Ctrl Pts',(-12.7946393385933,-77.0915839817282,
58.1358319323916));
#149325=CARTESIAN_POINT('Ctrl Pts',(-12.7802560819789,-76.9803598142564,
58.1205310146299));
#149326=CARTESIAN_POINT('Ctrl Pts',(-12.7663963661219,-76.8644767830903,
58.1060037986954));
#149327=CARTESIAN_POINT('Ctrl Pts',(-12.7527924430809,-76.7507324715907,
58.0917446948572));
#149328=CARTESIAN_POINT('Ctrl Pts',(-12.7396927706292,-76.6324994663116,
58.0782310111901));
#149329=CARTESIAN_POINT('Ctrl Pts',(-12.7274076754917,-76.509778133224,
58.0657752664847));
#149330=CARTESIAN_POINT('Ctrl Pts',(-12.7155212989591,-76.3910397793613,
58.053723778897));
#149331=CARTESIAN_POINT('Ctrl Pts',(-12.7043974504569,-76.2680995647439,
58.042662743653));
#149332=CARTESIAN_POINT('Ctrl Pts',(-12.6943560376396,-76.1409753244791,
58.0328999684157));
#149333=CARTESIAN_POINT('Ctrl Pts',(-12.6844879597932,-76.0160455041525,
58.0233057183046));
#149334=CARTESIAN_POINT('Ctrl Pts',(-12.675665147966,-75.8870746813651,
58.0149652977699));
#149335=CARTESIAN_POINT('Ctrl Pts',(-12.6682306289814,-75.7540994155384,
58.0081946946424));
#149336=CARTESIAN_POINT('Ctrl Pts',(-12.6609684644375,-75.6242069150686,
58.0015810543955));
#149337=CARTESIAN_POINT('Ctrl Pts',(-12.655030899086,-75.4904933443661,
57.9964653146573));
#149338=CARTESIAN_POINT('Ctrl Pts',(-12.6507769180658,-75.3530140123066,
57.9931646932654));
#149339=CARTESIAN_POINT('Ctrl Pts',(-12.6500770198269,-75.3303948370138,
57.9926216492113));
#149340=CARTESIAN_POINT('Ctrl Pts',(-12.6494227846886,-75.3076737752469,
57.992127789802));
#149341=CARTESIAN_POINT('Ctrl Pts',(-12.6488159186004,-75.2848511344054,
57.9916845878715));
#149342=CARTESIAN_POINT('Ctrl Pts',(-12.647423216751,-75.2324752730287,
57.990667480209));
#149343=CARTESIAN_POINT('Ctrl Pts',(-12.6462799292659,-75.1795643997014,
57.9899171327559));
#149344=CARTESIAN_POINT('Ctrl Pts',(-12.6454073095658,-75.1261226027846,
57.9894516915813));
#149345=CARTESIAN_POINT('Ctrl Pts',(-12.6449709997158,-75.0994017043262,
57.989218970994));
#149346=CARTESIAN_POINT('Ctrl Pts',(-12.6446023568134,-75.0725480749185,
57.9890574844566));
#149347=CARTESIAN_POINT('Ctrl Pts',(-12.6443041376411,-75.0455622853593,
57.9889695458607));
#149348=CARTESIAN_POINT('Ctrl Pts',(-12.644155028055,-75.0320693905796,
57.9889255765627));
#149349=CARTESIAN_POINT('Ctrl Pts',(-12.6440235244015,-75.0185434557562,
57.988899994721));
#149350=CARTESIAN_POINT('Ctrl Pts',(-12.6439099743117,-75.004984554064,
57.9888930924322));
#149351=CARTESIAN_POINT('Ctrl Pts',(-12.6438586623979,-74.9988574501932,
57.9888899733713));
#149352=CARTESIAN_POINT('Ctrl Pts',(-12.6438110165178,-74.992723614377,
57.9888906687514));
#149353=CARTESIAN_POINT('Ctrl Pts',(-12.643767068976,-74.9865830535138,
57.9888952056554));
#149354=CARTESIAN_POINT('Ctrl Pts',(-12.6437623899226,-74.9859292737851,
57.9888956886953));
#149355=CARTESIAN_POINT('Ctrl Pts',(-12.6437577527925,-74.9852754178238,
57.9888962152815));
#149356=CARTESIAN_POINT('Ctrl Pts',(-12.6437531576071,-74.9846214856349,
57.9888967854431));
#149357=CARTESIAN_POINT('Ctrl Pts',(-12.6437292801042,-74.9812235231251,
57.9888997481169));
#149358=CARTESIAN_POINT('Ctrl Pts',(-12.6437065355134,-74.9778235025011,
57.9889038873485));
#149359=CARTESIAN_POINT('Ctrl Pts',(-12.6436849263517,-74.974421424422,
57.9889092072289));
#149360=CARTESIAN_POINT('Ctrl Pts',(-12.6436741217709,-74.9727203853825,
57.988911867169));
#149361=CARTESIAN_POINT('Ctrl Pts',(-12.6436636010473,-74.9710188319792,
57.9889148222714));
#149362=CARTESIAN_POINT('Ctrl Pts',(-12.6436533645937,-74.9693167643124,
57.9889180730478));
#149363=CARTESIAN_POINT('Ctrl Pts',(-12.64364312814,-74.9676146966457,57.9889213238242));
#149364=CARTESIAN_POINT('Ctrl Pts',(-12.6436266975925,-74.9647708441181,
57.9889274452835));
#149365=CARTESIAN_POINT('Ctrl Pts',(-12.6436235084189,-74.9642090186155,
57.9889287129107));
#149366=CARTESIAN_POINT('Ctrl Pts',(-12.6423924798547,-74.7473430452712,
57.9894180200292));
#149367=CARTESIAN_POINT('Ctrl Pts',(-12.6464722421314,-74.5272810364192,
57.9946990479728));
#149368=CARTESIAN_POINT('Ctrl Pts',(-12.6559493112579,-74.3042892424013,
58.0051451784453));
#149369=CARTESIAN_POINT('Ctrl Pts',(-12.6590427852643,-74.2315009880133,
58.0085549702968));
#149370=CARTESIAN_POINT('Ctrl Pts',(-12.6627110658457,-74.1584008772902,
58.0125150158115));
#149371=CARTESIAN_POINT('Ctrl Pts',(-12.6669563735319,-74.0849990552687,
58.0170380732945));
#149372=CARTESIAN_POINT('Ctrl Pts',(-12.6755819225541,-73.9358623940509,
58.0262279499616));
#149373=CARTESIAN_POINT('Ctrl Pts',(-12.6865899761586,-73.7854797682283,
58.037742148481));
#149374=CARTESIAN_POINT('Ctrl Pts',(-12.6999939404739,-73.6339417234719,
58.0516862103875));
#149375=CARTESIAN_POINT('Ctrl Pts',(-12.7016694360133,-73.6149994678774,
58.0534292181258));
#149376=CARTESIAN_POINT('Ctrl Pts',(-12.7033823676581,-73.596039158706,
58.0552101908171));
#149377=CARTESIAN_POINT('Ctrl Pts',(-12.7051327395031,-73.5770609952093,
58.0570293310643));
#149378=CARTESIAN_POINT('Ctrl Pts',(-12.7060079254256,-73.567571913461,
58.0579389011879));
#149379=CARTESIAN_POINT('Ctrl Pts',(-12.7068924713982,-73.5580783681313,
58.0588580131901));
#149380=CARTESIAN_POINT('Ctrl Pts',(-12.7077863807806,-73.5485803811959,
58.0597866926387));
#149381=CARTESIAN_POINT('Ctrl Pts',(-12.7083434951339,-73.5426609167027,
58.0603654768652));
#149382=CARTESIAN_POINT('Ctrl Pts',(-12.7094999600431,-73.5304270822779,
58.0615666407172));
#149383=CARTESIAN_POINT('Ctrl Pts',(-12.7107956448812,-73.5169414277841,
58.062914021425));
#149384=CARTESIAN_POINT('Ctrl Pts',(-12.7115789314904,-73.5087888799804,
58.0637285599879));
#149385=CARTESIAN_POINT('Ctrl Pts',(-12.7124127687112,-73.5001787991258,
58.0645961630611));
#149386=CARTESIAN_POINT('Ctrl Pts',(-12.7131886153166,-73.492228755033,
58.0654037341901));
#149387=CARTESIAN_POINT('Ctrl Pts',(-12.7256079849222,-73.3649683722766,
58.0783309343132));
#149388=CARTESIAN_POINT('Ctrl Pts',(-12.7394903373919,-73.2379099565758,
58.0928780348362));
#149389=CARTESIAN_POINT('Ctrl Pts',(-12.7547724123794,-73.111094650057,
58.1090308435863));
#149390=CARTESIAN_POINT('Ctrl Pts',(-12.8005432352705,-72.7312744398236,
58.1574095715472));
#149391=CARTESIAN_POINT('Ctrl Pts',(-12.8588680404003,-72.3536377877317,
58.2201931924962));
#149392=CARTESIAN_POINT('Ctrl Pts',(-12.9276269165322,-71.9805430020649,
58.2966226816471));
#149393=CARTESIAN_POINT('Ctrl Pts',(-12.9713073127522,-71.7435273761213,
58.3451759820618));
#149394=CARTESIAN_POINT('Ctrl Pts',(-13.0191991735993,-71.5083440691444,
58.3992359930534));
#149395=CARTESIAN_POINT('Ctrl Pts',(-13.070764446851,-71.2755883075958,
58.4586057913291));
#149396=CARTESIAN_POINT('Ctrl Pts',(-13.0726976055627,-71.2668623996393,
58.4608315381451));
#149397=CARTESIAN_POINT('Ctrl Pts',(-13.0746359275625,-71.2581399024908,
58.4630647475309));
#149398=CARTESIAN_POINT('Ctrl Pts',(-13.0765793755592,-71.2494208109103,
58.4653054191105));
#149399=CARTESIAN_POINT('Ctrl Pts',(-13.0824690904162,-71.2229971745143,
58.4720958846719));
#149400=CARTESIAN_POINT('Ctrl Pts',(-13.088563822919,-71.1959483931376,
58.4791276115216));
#149401=CARTESIAN_POINT('Ctrl Pts',(-13.094365672755,-71.1703746713447,
58.4858479438368));
#149402=CARTESIAN_POINT('Ctrl Pts',(-13.0974641278934,-71.1567171255727,
58.4894369109391));
#149403=CARTESIAN_POINT('Ctrl Pts',(-13.1004785546761,-71.1434799258363,
58.4929362950644));
#149404=CARTESIAN_POINT('Ctrl Pts',(-13.1033301380902,-71.1309808245413,
58.4962571597016));
#149405=CARTESIAN_POINT('Ctrl Pts',(-13.117605932808,-71.0684069565064,
58.5128823026352));
#149406=CARTESIAN_POINT('Ctrl Pts',(-13.1333784859781,-70.9996257008027,
58.5315864012066));
#149407=CARTESIAN_POINT('Ctrl Pts',(-13.1507809817488,-70.9247447921021,
58.5526325801446));
#149408=CARTESIAN_POINT('Ctrl Pts',(-13.168897069721,-70.8467933794233,
58.5745417611118));
#149409=CARTESIAN_POINT('Ctrl Pts',(-13.1887803485131,-70.7622317902181,
58.5989886469898));
#149410=CARTESIAN_POINT('Ctrl Pts',(-13.2105817144479,-70.6712004295549,
58.6263267340083));
#149411=CARTESIAN_POINT('Ctrl Pts',(-13.2311438855887,-70.5853433129532,
58.6521109176973));
#149412=CARTESIAN_POINT('Ctrl Pts',(-13.2534130327245,-70.4937312430357,
58.6804674325607));
#149413=CARTESIAN_POINT('Ctrl Pts',(-13.2775048114296,-70.3964964858422,
58.711740169317));
#149414=CARTESIAN_POINT('Ctrl Pts',(-13.3010877577409,-70.3013153833359,
58.7423524076643));
#149415=CARTESIAN_POINT('Ctrl Pts',(-13.3264179063024,-70.2007467197002,
58.7757591300533));
#149416=CARTESIAN_POINT('Ctrl Pts',(-13.3535821398449,-70.0949263892232,
58.8123256645947));
#149417=CARTESIAN_POINT('Ctrl Pts',(-13.379711247878,-69.9931384686179,
58.8474987877359));
#149418=CARTESIAN_POINT('Ctrl Pts',(-13.4075379091794,-69.8864916331328,
58.8855957367618));
#149419=CARTESIAN_POINT('Ctrl Pts',(-13.4371097624152,-69.7751159602277,
58.9269786558671));
#149420=CARTESIAN_POINT('Ctrl Pts',(-13.4452861747418,-69.7443213591059,
58.938420745992));
#149421=CARTESIAN_POINT('Ctrl Pts',(-13.4535957952498,-69.7131652949402,
58.9501142568892));
#149422=CARTESIAN_POINT('Ctrl Pts',(-13.4620391155253,-69.6816506263856,
58.9620673329486));
#149423=CARTESIAN_POINT('Ctrl Pts',(-13.46677738784,-69.6639650386489,58.968775230733));
#149424=CARTESIAN_POINT('Ctrl Pts',(-13.4715577617754,-69.6461665165836,
58.9755648770865));
#149425=CARTESIAN_POINT('Ctrl Pts',(-13.4763802887566,-69.6282555714961,
58.9824377406472));
#149426=CARTESIAN_POINT('Ctrl Pts',(-13.4787915522472,-69.6193000989524,
58.9858741724276));
#149427=CARTESIAN_POINT('Ctrl Pts',(-13.481213354,-69.6103165207718,58.9893314088175));
#149428=CARTESIAN_POINT('Ctrl Pts',(-13.4836456973389,-69.6013049011923,
58.9928096353972));
#149429=CARTESIAN_POINT('Ctrl Pts',(-13.4859012793976,-69.592948166714,
58.9960350951191));
#149430=CARTESIAN_POINT('Ctrl Pts',(-13.4893480346654,-69.5801931700439,
59.0009709140122));
#149431=CARTESIAN_POINT('Ctrl Pts',(-13.4925521253834,-69.568363122783,
59.0055695370881));
#149432=CARTESIAN_POINT('Ctrl Pts',(-13.4928032176347,-69.5674360475342,
59.0059299134702));
#149433=CARTESIAN_POINT('Ctrl Pts',(-13.4930528122557,-69.5665146428691,
59.0062881936137));
#149434=CARTESIAN_POINT('Ctrl Pts',(-13.4933002153033,-69.5656014654837,
59.0066433785788));
#149435=CARTESIAN_POINT('Ctrl Pts',(-13.506917884383,-69.5153379478529,
59.0261936281169));
#149436=CARTESIAN_POINT('Ctrl Pts',(-13.520340769412,-69.4661983742167,
59.0456237114897));
#149437=CARTESIAN_POINT('Ctrl Pts',(-13.533551277004,-69.4181692104236,
59.0649008672749));
#149438=CARTESIAN_POINT('Ctrl Pts',(-13.559972292188,-69.3221108828374,
59.1034551788453));
#149439=CARTESIAN_POINT('Ctrl Pts',(-13.5855437946768,-69.2304936374915,
59.1413963750281));
#149440=CARTESIAN_POINT('Ctrl Pts',(-13.6101573958495,-69.1432184685839,
59.1784781910238));
#149441=CARTESIAN_POINT('Ctrl Pts',(-13.6375278398563,-69.046168057024,
59.219713350449));
#149442=CARTESIAN_POINT('Ctrl Pts',(-13.6637136362959,-68.9544866600855,
59.2598853043287));
#149443=CARTESIAN_POINT('Ctrl Pts',(-13.6886091518112,-68.8680542840001,
59.2986865946742));
#149444=CARTESIAN_POINT('Ctrl Pts',(-13.7140937238119,-68.7795768186437,
59.338405968106));
#149445=CARTESIAN_POINT('Ctrl Pts',(-13.7382267357766,-68.6965997193151,
59.3766888995997));
#149446=CARTESIAN_POINT('Ctrl Pts',(-13.7609340346995,-68.6190114939214,
59.4132413986414));
#149447=CARTESIAN_POINT('Ctrl Pts',(-13.7843489555268,-68.5390054059721,
59.4509329741125));
#149448=CARTESIAN_POINT('Ctrl Pts',(-13.8062484159958,-68.4647292758614,
59.4867843745649));
#149449=CARTESIAN_POINT('Ctrl Pts',(-13.8265845753271,-68.3960790089942,
59.5205137508794));
#149450=CARTESIAN_POINT('Ctrl Pts',(-13.8365619932143,-68.3623975065314,
59.5370622090755));
#149451=CARTESIAN_POINT('Ctrl Pts',(-13.846163558071,-68.3300704921782,
59.5531004967338));
#149452=CARTESIAN_POINT('Ctrl Pts',(-13.8553858823851,-68.2990872092859,
59.5685989544768));
#149453=CARTESIAN_POINT('Ctrl Pts',(-13.8747444748846,-68.2340501614248,
59.6011317865045));
#149454=CARTESIAN_POINT('Ctrl Pts',(-13.8924309393971,-68.1749327207469,
59.6312830134023));
#149455=CARTESIAN_POINT('Ctrl Pts',(-13.9084295097878,-68.1216492241398,
59.6588125801309));
#149456=CARTESIAN_POINT('Ctrl Pts',(-13.9245519020274,-68.0679533368688,
59.6865552135129));
#149457=CARTESIAN_POINT('Ctrl Pts',(-13.9389606952694,-68.0201820868406,
59.7116353842495));
#149458=CARTESIAN_POINT('Ctrl Pts',(-13.9516539764714,-67.97826618418,59.7338551628796));
#149459=CARTESIAN_POINT('Ctrl Pts',(-13.9644135161547,-67.936131481982,
59.7561909279724));
#149460=CARTESIAN_POINT('Ctrl Pts',(-13.9754400180266,-67.8999134516241,
59.7756363162961));
#149461=CARTESIAN_POINT('Ctrl Pts',(-13.9847386240222,-67.8695596322964,
59.7920391320418));
#149462=CARTESIAN_POINT('Ctrl Pts',(-13.9873839818165,-67.8609242828058,
59.7967055644621));
#149463=CARTESIAN_POINT('Ctrl Pts',(-13.989889515867,-67.8527636585599,
59.8011260517909));
#149464=CARTESIAN_POINT('Ctrl Pts',(-13.9922553804113,-67.8450768092218,
59.8052978142969));
#149465=CARTESIAN_POINT('Ctrl Pts',(-14.2053627384179,-82.25455936809,59.85616341864));
#149466=CARTESIAN_POINT('Ctrl Pts',(-13.6866847824119,-82.3366282815,59.92373292204));
#149467=CARTESIAN_POINT('Ctrl Pts',(-12.6383817091255,-82.58289982254,59.91553905833));
#149468=CARTESIAN_POINT('Ctrl Pts',(-11.1637780911499,-83.19639241636,59.42315761485));
#149469=CARTESIAN_POINT('Ctrl Pts',(-9.99316319052391,-83.97026149908,58.51581872871));
#149470=CARTESIAN_POINT('Ctrl Pts',(-9.52143302578291,-84.52126777961,57.71959030244));
#149471=CARTESIAN_POINT('Ctrl Pts',(-9.36367665720391,-84.79397357294,57.29408547033));
#149472=CARTESIAN_POINT('Ctrl Pts',(-14.0202046372369,-81.66798572512,59.53231650414));
#149473=CARTESIAN_POINT('Ctrl Pts',(-13.5161419891421,-81.7529897771,59.59488219199));
#149474=CARTESIAN_POINT('Ctrl Pts',(-12.5016391850972,-81.9934997129,59.58065052531));
#149475=CARTESIAN_POINT('Ctrl Pts',(-11.0704533736609,-82.56018318755,59.10069440813));
#149476=CARTESIAN_POINT('Ctrl Pts',(-9.91290994947291,-83.2607556917,58.2229682051));
#149477=CARTESIAN_POINT('Ctrl Pts',(-9.42170896486991,-83.75798893721,57.44738812635));
#149478=CARTESIAN_POINT('Ctrl Pts',(-9.24823875588991,-84.00518323524,57.0294496165));
#149479=CARTESIAN_POINT('Ctrl Pts',(-13.6549069241899,-80.50006195024,58.98674389696));
#149480=CARTESIAN_POINT('Ctrl Pts',(-13.1769404748632,-80.58353896436,59.03665035665));
#149481=CARTESIAN_POINT('Ctrl Pts',(-12.2218902458404,-80.80094275264,59.00590868676));
#149482=CARTESIAN_POINT('Ctrl Pts',(-10.8679330721049,-81.27153994433,58.54326883773));
#149483=CARTESIAN_POINT('Ctrl Pts',(-9.73897835675991,-81.83491357831,57.71819138306));
#149484=CARTESIAN_POINT('Ctrl Pts',(-9.21997508227391,-82.23283245568,56.98439768797));
#149485=CARTESIAN_POINT('Ctrl Pts',(-9.02174978536891,-82.43224264183,56.58383055835));
#149486=CARTESIAN_POINT('Ctrl Pts',(-13.0264541098134,-78.10903159314,58.22143278291));
#149487=CARTESIAN_POINT('Ctrl Pts',(-12.5887620025533,-78.16896765775,58.24468551411));
#149488=CARTESIAN_POINT('Ctrl Pts',(-11.7230981427644,-78.30931348211,58.17830836715));
#149489=CARTESIAN_POINT('Ctrl Pts',(-10.4863172342789,-78.57820044195,57.73325733766));
#149490=CARTESIAN_POINT('Ctrl Pts',(-9.41080141879391,-78.88372055786,56.98713738772));
#149491=CARTESIAN_POINT('Ctrl Pts',(-8.86349672505391,-79.09709391693,56.32569316036));
#149492=CARTESIAN_POINT('Ctrl Pts',(-8.63464566340091,-79.20524884609,55.9591981337));
#149493=CARTESIAN_POINT('Ctrl Pts',(-12.703739323494,-75.60837772321,57.90748319535));
#149494=CARTESIAN_POINT('Ctrl Pts',(-12.2839358655288,-75.61999252453,57.91587997198));
#149495=CARTESIAN_POINT('Ctrl Pts',(-11.4571120723489,-75.64721072235,57.82979946692));
#149496=CARTESIAN_POINT('Ctrl Pts',(-10.2725544129919,-75.69964966516,57.38928272527));
#149497=CARTESIAN_POINT('Ctrl Pts',(-9.22672717125391,-75.7595397854,56.67735146262));
#149498=CARTESIAN_POINT('Ctrl Pts',(-8.67519748870391,-75.80154788321,56.05133853923));
#149499=CARTESIAN_POINT('Ctrl Pts',(-8.43723858833691,-75.82288542366,55.70323479651));
#149500=CARTESIAN_POINT('Ctrl Pts',(-12.8671141721127,-73.11809265367,58.06713723927));
#149501=CARTESIAN_POINT('Ctrl Pts',(-12.4383232178021,-73.08201133181,58.08327470442));
#149502=CARTESIAN_POINT('Ctrl Pts',(-11.5918425291893,-72.9974900293,58.00755176422));
#149503=CARTESIAN_POINT('Ctrl Pts',(-10.3806961735769,-72.83504489813,57.56487994748));
#149504=CARTESIAN_POINT('Ctrl Pts',(-9.31980220568191,-72.64992691269,56.83532487628));
#149505=CARTESIAN_POINT('Ctrl Pts',(-8.77051022514591,-72.52032197963,56.19100248932));
#149506=CARTESIAN_POINT('Ctrl Pts',(-8.53719879336891,-72.4545491955,55.83340513874));
#149507=CARTESIAN_POINT('Ctrl Pts',(-13.3015354916696,-70.62027701925,58.54120535384));
#149508=CARTESIAN_POINT('Ctrl Pts',(-12.8466551590814,-70.5435375917,58.57621796265));
#149509=CARTESIAN_POINT('Ctrl Pts',(-11.9431325981647,-70.35631033313,58.52545042363));
#149510=CARTESIAN_POINT('Ctrl Pts',(-10.6566364727679,-69.97916480861,58.07343649006));
#149511=CARTESIAN_POINT('Ctrl Pts',(-9.55738924270591,-69.54092805089,57.29417007323));
#149512=CARTESIAN_POINT('Ctrl Pts',(-9.02052118745191,-69.23342500244,56.60163811033));
#149513=CARTESIAN_POINT('Ctrl Pts',(-8.80382301199891,-69.07836783959,56.22016816974));
#149514=CARTESIAN_POINT('Ctrl Pts',(-13.8489227043029,-68.87555927534,59.23274232687));
#149515=CARTESIAN_POINT('Ctrl Pts',(-13.3583894250031,-68.78795581714,59.29065555428));
#149516=CARTESIAN_POINT('Ctrl Pts',(-12.3751455164616,-68.5530122456,59.2707797108));
#149517=CARTESIAN_POINT('Ctrl Pts',(-10.9840720246409,-68.02991414936,58.80223087688));
#149518=CARTESIAN_POINT('Ctrl Pts',(-9.83859395163391,-67.39731651073,57.95185518517));
#149519=CARTESIAN_POINT('Ctrl Pts',(-9.32938702250191,-66.94987820901,57.19539776513));
#149520=CARTESIAN_POINT('Ctrl Pts',(-9.14138216248191,-66.72629866191,56.78447782593));
#149521=CARTESIAN_POINT('Ctrl Pts',(-14.2054072809129,-67.7452469082,59.85623901085));
#149522=CARTESIAN_POINT('Ctrl Pts',(-13.6867239510529,-67.66316837402,59.92381322088));
#149523=CARTESIAN_POINT('Ctrl Pts',(-12.638412688455,-67.41687470616,59.91562799188));
#149524=CARTESIAN_POINT('Ctrl Pts',(-11.1638044367439,-66.80334542226,59.42325346353));
#149525=CARTESIAN_POINT('Ctrl Pts',(-9.99319080751391,-66.0294416455,58.51591282125));
#149526=CARTESIAN_POINT('Ctrl Pts',(-9.52146541439891,-65.47841540134,57.71967705271));
#149527=CARTESIAN_POINT('Ctrl Pts',(-9.36371259686991,-65.20570054798,57.29416759219));
#149528=CARTESIAN_POINT('',(-9.38953228746991,-84.5398910625,57.36388938658));
#149529=CARTESIAN_POINT('Ctrl Pts',(-9.38953228746991,-84.5398910625,57.36388938658));
#149530=CARTESIAN_POINT('Ctrl Pts',(-9.28299760588214,-83.7881949943336,
57.1128289322841));
#149531=CARTESIAN_POINT('Ctrl Pts',(-9.17640320159037,-83.0289015577622,
56.8968437256352));
#149532=CARTESIAN_POINT('Ctrl Pts',(-9.0288200623923,-81.878565350298,56.6211725879014));
#149533=CARTESIAN_POINT('Ctrl Pts',(-8.98163454409537,-81.4932206057088,
56.5373250438838));
#149534=CARTESIAN_POINT('Ctrl Pts',(-8.91505371442895,-80.912354475673,
56.4230638276863));
#149535=CARTESIAN_POINT('Ctrl Pts',(-8.88280899763094,-80.6212091573672,
56.3688110463283));
#149536=CARTESIAN_POINT('Ctrl Pts',(-8.84724153253191,-80.2802931760899,
56.3104368697372));
#149537=CARTESIAN_POINT('Ctrl Pts',(-8.82999560524952,-80.1095235746376,
56.2824661787593));
#149538=CARTESIAN_POINT('Ctrl Pts',(-8.82272235145397,-80.036269828841,
56.2707379426101));
#149539=CARTESIAN_POINT('Ctrl Pts',(-8.81789998947072,-79.9874191596997,
56.2629765596512));
#149540=CARTESIAN_POINT('Ctrl Pts',(-8.81564686072979,-79.9644706595696,
56.2593567797579));
#149541=CARTESIAN_POINT('Ctrl Pts',(-8.73217725899237,-79.108964570998,
56.1255245945277));
#149542=CARTESIAN_POINT('Ctrl Pts',(-8.66805506192752,-78.2811374986499,
56.03048087595));
#149543=CARTESIAN_POINT('Ctrl Pts',(-8.60339061485789,-77.0420287740733,
55.9360899191963));
#149544=CARTESIAN_POINT('Ctrl Pts',(-8.58704180991944,-76.629431179872,
55.912677597911));
#149545=CARTESIAN_POINT('Ctrl Pts',(-8.57070859794398,-76.0111927595564,
55.8893750942785));
#149546=CARTESIAN_POINT('Ctrl Pts',(-8.5666264756538,-75.805222947949,55.8835786701577));
#149547=CARTESIAN_POINT('Ctrl Pts',(-8.56121809111822,-75.3935026483962,
55.875906038777));
#149548=CARTESIAN_POINT('Ctrl Pts',(-8.55989222037363,-75.1863169678766,
55.8740303858725));
#149549=CARTESIAN_POINT('Ctrl Pts',(-8.5601738412577,-74.1652888001767,
55.8744291786204));
#149550=CARTESIAN_POINT('Ctrl Pts',(-8.58277625686303,-73.3443787169755,
55.9059564905164));
#149551=CARTESIAN_POINT('Ctrl Pts',(-8.64817866699291,-72.1068822686112,
56.0014895705712));
#149552=CARTESIAN_POINT('Ctrl Pts',(-8.6751867907122,-71.6933615652295,
56.0414040317809));
#149553=CARTESIAN_POINT('Ctrl Pts',(-8.72285528790025,-71.0715476792663,
56.1138062125568));
#149554=CARTESIAN_POINT('Ctrl Pts',(-8.74847436625131,-70.7602575285621,
56.1531423150808));
#149555=CARTESIAN_POINT('Ctrl Pts',(-8.78129743014174,-70.3964150725592,
56.2046369603786));
#149556=CARTESIAN_POINT('Ctrl Pts',(-8.79841527834946,-70.2143261911791,
56.2318009811849));
#149557=CARTESIAN_POINT('Ctrl Pts',(-8.80589984657586,-70.136252173435,
56.2437480312132));
#149558=CARTESIAN_POINT('Ctrl Pts',(-8.81092218104178,-70.0841948447782,
56.2517807797118));
#149559=CARTESIAN_POINT('Ctrl Pts',(-8.81362946612278,-70.0563216785734,
56.2561199096933));
#149560=CARTESIAN_POINT('Ctrl Pts',(-8.96727708076544,-68.4835727284964,
56.5028463120566));
#149561=CARTESIAN_POINT('Ctrl Pts',(-9.17702010416681,-66.959567194033,
56.8630815323802));
#149562=CARTESIAN_POINT('Ctrl Pts',(-9.38953228747191,-65.46010893749,57.36388938658));
#149563=CARTESIAN_POINT('Origin',(-13.9922814988585,-84.5398910375432,55.4107645734512));
#149564=CARTESIAN_POINT('Ctrl Pts',(-15.7857783725409,-86.29661480505,63.115509260726));
#149565=CARTESIAN_POINT('Ctrl Pts',(-13.2009589750593,-86.61530731379,63.626388245958));
#149566=CARTESIAN_POINT('Ctrl Pts',(-11.2043264355719,-88.19001512956,62.8661053606));
#149567=CARTESIAN_POINT('Ctrl Pts',(-10.7993789544399,-90.22954893502,61.21655661769));
#149568=CARTESIAN_POINT('Ctrl Pts',(-15.2179723740469,-85.09055880868,61.73606668887));
#149569=CARTESIAN_POINT('Ctrl Pts',(-12.7684152553155,-85.49389189082,62.22346223447));
#149570=CARTESIAN_POINT('Ctrl Pts',(-10.8253714758709,-86.8819838928,61.36857549732));
#149571=CARTESIAN_POINT('Ctrl Pts',(-10.2917538863009,-88.6099845115701,
59.56845212724));
#149572=CARTESIAN_POINT('Ctrl Pts',(-14.6117331505359,-83.64165090183,60.58580302674));
#149573=CARTESIAN_POINT('Ctrl Pts',(-12.2792545314831,-84.06648481616,60.9650212480601));
#149574=CARTESIAN_POINT('Ctrl Pts',(-10.3902588488939,-85.23953592222,60.03498149361));
#149575=CARTESIAN_POINT('Ctrl Pts',(-9.75033914806491,-86.66066443089,58.19212486272));
#149576=CARTESIAN_POINT('Ctrl Pts',(-14.1114447652699,-82.00287655395,59.72095409226));
#149577=CARTESIAN_POINT('Ctrl Pts',(-11.863059732406,-82.36563442235,59.99674441583));
#149578=CARTESIAN_POINT('Ctrl Pts',(-10.0167553446379,-83.30615659356,59.01200819548));
#149579=CARTESIAN_POINT('Ctrl Pts',(-9.30390833655991,-84.4519641217,57.1566590954));
#149580=CARTESIAN_POINT('',(-10.7897586692569,-89.96662969245,61.19644556989));
#149581=CARTESIAN_POINT('Ctrl Pts',(-10.7897586692559,-89.96662969245,61.1964455698903));
#149582=CARTESIAN_POINT('Ctrl Pts',(-10.6961214763189,-89.6639756404415,
60.8929443067986));
#149583=CARTESIAN_POINT('Ctrl Pts',(-10.6017810121018,-89.3511888436508,
60.5999837275916));
#149584=CARTESIAN_POINT('Ctrl Pts',(-10.5074125253993,-89.0282693020777,
60.3174330412154));
#149585=CARTESIAN_POINT('Ctrl Pts',(-10.480907523704,-88.9375718320227,
60.2380738538097));
#149586=CARTESIAN_POINT('Ctrl Pts',(-10.4544000117395,-88.8460750270309,
60.1595357621056));
#149587=CARTESIAN_POINT('Ctrl Pts',(-10.4279042498625,-88.7537788871023,
60.08181564452));
#149588=CARTESIAN_POINT('Ctrl Pts',(-10.367488574311,-88.54332509187,59.9045981170654));
#149589=CARTESIAN_POINT('Ctrl Pts',(-10.3071345456509,-88.3287152994673,
59.7316336299325));
#149590=CARTESIAN_POINT('Ctrl Pts',(-10.2470052765235,-88.1099495098942,
59.562883596963));
#149591=CARTESIAN_POINT('Ctrl Pts',(-10.2169406419597,-88.0005666151076,
59.4785085804783));
#149592=CARTESIAN_POINT('Ctrl Pts',(-10.186932093323,-87.8901447210284,
59.3951872149272));
#149593=CARTESIAN_POINT('Ctrl Pts',(-10.1569992127604,-87.7786838276566,
59.3129144044139));
#149594=CARTESIAN_POINT('Ctrl Pts',(-10.1270663321978,-87.6672229342848,
59.2306415939007));
#149595=CARTESIAN_POINT('Ctrl Pts',(-10.0974532876728,-87.5556544419064,
59.1500751344039));
#149596=CARTESIAN_POINT('Ctrl Pts',(-10.0674467345878,-87.4411841496634,
59.0692366916427));
#149597=CARTESIAN_POINT('Ctrl Pts',(-9.97973503412739,-87.1065777736358,
58.8329390650181));
#149598=CARTESIAN_POINT('Ctrl Pts',(-9.89342048644049,-86.7651177864549,
58.6072399120118));
#149599=CARTESIAN_POINT('Ctrl Pts',(-9.80904654297317,-86.4168041881208,
58.3919743536847));
#149600=CARTESIAN_POINT('Ctrl Pts',(-9.72420583947613,-86.0665637050301,
58.1755179376796));
#149601=CARTESIAN_POINT('Ctrl Pts',(-9.64132724870226,-85.7093935721399,
57.969610592813));
#149602=CARTESIAN_POINT('Ctrl Pts',(-9.56091049367537,-85.3452937894501,
57.7740847762417));
#149603=CARTESIAN_POINT('Ctrl Pts',(-9.50242505129663,-85.0804915495003,
57.6318828946213));
#149604=CARTESIAN_POINT('Ctrl Pts',(-9.44524065669213,-84.8120239738502,
57.4951721601973));
#149605=CARTESIAN_POINT('Ctrl Pts',(-9.38953228746956,-84.5398910625,57.3638893865801));
#149606=CARTESIAN_POINT('Origin',(-15.5675364833292,-89.9666295471007,59.7223902251639));
#149607=CARTESIAN_POINT('Ctrl Pts',(-10.7183277173439,-89.9625444980999,
60.95715572325));
#149608=CARTESIAN_POINT('Ctrl Pts',(-11.1488047984679,-87.96322629393,62.63856744174));
#149609=CARTESIAN_POINT('Ctrl Pts',(-13.154649703826,-86.4190502844,63.414597018712));
#149610=CARTESIAN_POINT('Ctrl Pts',(-15.7319351985739,-86.1031085662201,
62.89663151716));
#149611=CARTESIAN_POINT('Ctrl Pts',(-10.9910678176069,-90.84201858795,61.82247418517));
#149612=CARTESIAN_POINT('Ctrl Pts',(-11.3283473228529,-88.7567304712899,
63.321898809999));
#149613=CARTESIAN_POINT('Ctrl Pts',(-13.2089159040587,-87.13321591558,64.037450008722));
#149614=CARTESIAN_POINT('Ctrl Pts',(-15.7293910876889,-86.75161252055,63.625211302696));
#149615=CARTESIAN_POINT('Ctrl Pts',(-11.2584139392729,-91.59984702702,62.77268895686));
#149616=CARTESIAN_POINT('Ctrl Pts',(-11.5134937823499,-89.46571522909,64.092206053233));
#149617=CARTESIAN_POINT('Ctrl Pts',(-13.2730319217104,-87.78250254908,64.7371138262451));
#149618=CARTESIAN_POINT('Ctrl Pts',(-15.7260859252339,-87.32621487051,64.4100287288261));
#149619=CARTESIAN_POINT('Ctrl Pts',(-11.5024576829099,-92.24121677998,63.808093557901));
#149620=CARTESIAN_POINT('Ctrl Pts',(-11.6902236879807,-90.08258370556,64.959788823145));
#149621=CARTESIAN_POINT('Ctrl Pts',(-13.3403958339825,-88.3579608586,65.529213168241));
#149622=CARTESIAN_POINT('Ctrl Pts',(-15.7224300293869,-87.83109219926,65.264145083567));
#149623=CARTESIAN_POINT('',(-11.4804281687819,-92.,63.72676972225));
#149624=CARTESIAN_POINT('Ctrl Pts',(-11.4804281687818,-92.,63.72676972225));
#149625=CARTESIAN_POINT('Ctrl Pts',(-11.3791659077606,-91.7276039629617,
63.3013371498193));
#149626=CARTESIAN_POINT('Ctrl Pts',(-11.2743320050127,-91.4356124926206,
62.8917472513322));
#149627=CARTESIAN_POINT('Ctrl Pts',(-11.1672746427287,-91.1239902090124,
62.4978437851762));
#149628=CARTESIAN_POINT('Ctrl Pts',(-11.0628000093336,-90.8198857257414,
62.1134431298476));
#149629=CARTESIAN_POINT('Ctrl Pts',(-10.9562080540964,-90.4970861151506,
61.7439811046052));
#149630=CARTESIAN_POINT('Ctrl Pts',(-10.8487288878876,-90.1556011109963,
61.3893000120327));
#149631=CARTESIAN_POINT('Ctrl Pts',(-10.829099340904,-90.0932337130188,
61.3245225354629));
#149632=CARTESIAN_POINT('Ctrl Pts',(-10.8094401338748,-90.030243166608,
61.2602380564391));
#149633=CARTESIAN_POINT('Ctrl Pts',(-10.7897586692573,-89.9666296924501,
61.1964455698899));
#149634=CARTESIAN_POINT('Origin',(-16.3445396385588,-92.0000000217413,62.5690048024171));
#149635=CARTESIAN_POINT('Ctrl Pts',(-15.7267485954679,-87.66539271722,80.98689185542));
#149636=CARTESIAN_POINT('Ctrl Pts',(-15.1845473504709,-87.78122714385,80.916890805709));
#149637=CARTESIAN_POINT('Ctrl Pts',(-14.1051578442959,-88.17294061374,80.871443999723));
#149638=CARTESIAN_POINT('Ctrl Pts',(-12.6905091994459,-89.25086783016,81.140906685209));
#149639=CARTESIAN_POINT('Ctrl Pts',(-11.7187170051615,-90.65190210376,81.710977340828));
#149640=CARTESIAN_POINT('Ctrl Pts',(-11.4633133420439,-91.64600244116,82.225570496093));
#149641=CARTESIAN_POINT('Ctrl Pts',(-11.4262749611389,-92.13114394692,82.498924437511));
#149642=CARTESIAN_POINT('Ctrl Pts',(-15.7173836160999,-88.05182477781,80.364280814309));
#149643=CARTESIAN_POINT('Ctrl Pts',(-15.2062426832829,-88.16375596495,80.330470883294));
#149644=CARTESIAN_POINT('Ctrl Pts',(-14.2055189094499,-88.52846025707,80.340232470926));
#149645=CARTESIAN_POINT('Ctrl Pts',(-12.8992702355175,-89.49997920196,80.607597479859));
#149646=CARTESIAN_POINT('Ctrl Pts',(-11.9627692360111,-90.76949848147,81.092123199415));
#149647=CARTESIAN_POINT('Ctrl Pts',(-11.666429117173,-91.70187736404,81.517563967468));
#149648=CARTESIAN_POINT('Ctrl Pts',(-11.5979936627015,-92.16979066453,81.745905912518));
#149649=CARTESIAN_POINT('Ctrl Pts',(-15.7002372525439,-88.72433818278,79.089598686914));
#149650=CARTESIAN_POINT('Ctrl Pts',(-15.2467375145529,-88.82579237976,79.100193597181));
#149651=CARTESIAN_POINT('Ctrl Pts',(-14.3760944340769,-89.13993303906,79.168545711718));
#149652=CARTESIAN_POINT('Ctrl Pts',(-13.2334233980418,-89.94290089825,79.413180303588));
#149653=CARTESIAN_POINT('Ctrl Pts',(-12.3569948357183,-90.99911727509,79.774927745118));
#149654=CARTESIAN_POINT('Ctrl Pts',(-12.0079449977392,-91.80959370206,80.073791601054));
#149655=CARTESIAN_POINT('Ctrl Pts',(-11.8932536346062,-92.23267061772,80.234650779147));
#149656=CARTESIAN_POINT('Ctrl Pts',(-15.6808989474229,-89.45529670407,77.067422189446));
#149657=CARTESIAN_POINT('Ctrl Pts',(-15.2931912697469,-89.54407975723,77.094016900249));
#149658=CARTESIAN_POINT('Ctrl Pts',(-14.5550845677969,-89.80455656405,77.169706300882));
#149659=CARTESIAN_POINT('Ctrl Pts',(-13.5661328445162,-90.44243352221,77.349989108941));
#149660=CARTESIAN_POINT('Ctrl Pts',(-12.7529608600718,-91.28077188604,77.584104760901));
#149661=CARTESIAN_POINT('Ctrl Pts',(-12.3659618936567,-91.94231099482,77.767814371209));
#149662=CARTESIAN_POINT('Ctrl Pts',(-12.211902366606,-92.29761926682,77.866438532652));
#149663=CARTESIAN_POINT('Ctrl Pts',(-15.6717957676439,-89.80966909398,75.388028487314));
#149664=CARTESIAN_POINT('Ctrl Pts',(-15.3151695191169,-89.89025483975,75.409280511305));
#149665=CARTESIAN_POINT('Ctrl Pts',(-14.6374260128379,-90.12244382554,75.46239351056));
#149666=CARTESIAN_POINT('Ctrl Pts',(-13.7177800254399,-90.68309838254,75.574038621683));
#149667=CARTESIAN_POINT('Ctrl Pts',(-12.9367807162256,-91.42083563943,75.711139278103));
#149668=CARTESIAN_POINT('Ctrl Pts',(-12.538043838553,-92.0102950282,75.815680084024));
#149669=CARTESIAN_POINT('Ctrl Pts',(-12.3689260666087,-92.33083105141,75.871517394051));
#149670=CARTESIAN_POINT('Ctrl Pts',(-15.6681296739329,-89.95257099154,74.024855121973));
#149671=CARTESIAN_POINT('Ctrl Pts',(-15.3240385042369,-90.03019457712,74.034896853418));
#149672=CARTESIAN_POINT('Ctrl Pts',(-14.6702817192719,-90.25160971085,74.059201836835));
#149673=CARTESIAN_POINT('Ctrl Pts',(-13.7779625534719,-90.78190268908,74.10851169455));
#149674=CARTESIAN_POINT('Ctrl Pts',(-13.0100010368838,-91.47919202969,74.168024423489));
#149675=CARTESIAN_POINT('Ctrl Pts',(-12.6072846536751,-92.03865947839,74.213003982407));
#149676=CARTESIAN_POINT('Ctrl Pts',(-12.4326148349899,-92.34428896209,74.236998274081));
#149677=CARTESIAN_POINT('Ctrl Pts',(-15.6672248087549,-89.98827259123,72.9875954719413));
#149678=CARTESIAN_POINT('Ctrl Pts',(-15.3262299348879,-90.06524457197,72.9875820642177));
#149679=CARTESIAN_POINT('Ctrl Pts',(-14.6783497519689,-90.28411903404,72.987550292389));
#149680=CARTESIAN_POINT('Ctrl Pts',(-13.7927252045719,-90.8069898723,72.9874874147133));
#149681=CARTESIAN_POINT('Ctrl Pts',(-13.0280723074446,-91.49419544011,72.987412580105));
#149682=CARTESIAN_POINT('Ctrl Pts',(-12.6245704860005,-92.04598955855,72.9873565731651));
#149683=CARTESIAN_POINT('Ctrl Pts',(-12.4486600227693,-92.34772416774,72.9873268080765));
#149684=CARTESIAN_POINT('Ctrl Pts',(-15.6681350491459,-89.9523609443,71.950180627016));
#149685=CARTESIAN_POINT('Ctrl Pts',(-15.3240254973829,-90.02998927862,71.940116172401));
#149686=CARTESIAN_POINT('Ctrl Pts',(-14.6702336070009,-90.25142080795,71.915752744234));
#149687=CARTESIAN_POINT('Ctrl Pts',(-13.7778744577689,-90.78175855918,71.866316228017));
#149688=CARTESIAN_POINT('Ctrl Pts',(-13.0098937512633,-91.47910696723,71.806645169241));
#149689=CARTESIAN_POINT('Ctrl Pts',(-12.6071830844856,-92.03861806362,71.761543025199));
#149690=CARTESIAN_POINT('Ctrl Pts',(-12.432521388372,-92.34426923603,71.737482735481));
#149691=CARTESIAN_POINT('Ctrl Pts',(-15.6718111921509,-89.80907524214,70.586583011817));
#149692=CARTESIAN_POINT('Ctrl Pts',(-15.3151322403169,-89.8896753559,70.565323380961));
#149693=CARTESIAN_POINT('Ctrl Pts',(-14.6372871557079,-90.12191254573,70.512171532443));
#149694=CARTESIAN_POINT('Ctrl Pts',(-13.7175254777709,-90.68269626992,70.400398310495));
#149695=CARTESIAN_POINT('Ctrl Pts',(-12.9364726797289,-91.42060119049,70.26311038424));
#149696=CARTESIAN_POINT('Ctrl Pts',(-12.5377554772725,-92.01018118362,70.158412233547));
#149697=CARTESIAN_POINT('Ctrl Pts',(-12.3686629807924,-92.33077573351,70.102488458309));
#149698=CARTESIAN_POINT('Ctrl Pts',(-15.6809151702919,-89.45464488429,68.907864632705));
#149699=CARTESIAN_POINT('Ctrl Pts',(-15.2931521975629,-89.54343665812,68.881249937272));
#149700=CARTESIAN_POINT('Ctrl Pts',(-14.5549361924049,-89.80395622407,68.805510076319));
#149701=CARTESIAN_POINT('Ctrl Pts',(-13.5658570449471,-90.44197313346,68.625123720347));
#149702=CARTESIAN_POINT('Ctrl Pts',(-12.7526267697373,-91.28050410382,68.390888386043));
#149703=CARTESIAN_POINT('Ctrl Pts',(-12.3656508008458,-91.94218435098,68.207096911123));
#149704=CARTESIAN_POINT('Ctrl Pts',(-12.2116193557359,-92.29756107263,68.10843240078));
#149705=CARTESIAN_POINT('Ctrl Pts',(-15.7002706718129,-88.7231701863,66.886166124211));
#149706=CARTESIAN_POINT('Ctrl Pts',(-15.2466574582849,-88.82466182876,66.87569843402));
#149707=CARTESIAN_POINT('Ctrl Pts',(-14.3757812509549,-89.13891694147,66.807519820801));
#149708=CARTESIAN_POINT('Ctrl Pts',(-13.2328406129946,-89.94217161044,66.56288459358));
#149709=CARTESIAN_POINT('Ctrl Pts',(-12.3563117520386,-90.99872782708,66.200892463384));
#149710=CARTESIAN_POINT('Ctrl Pts',(-12.0073444264764,-91.80940442047,65.901727738338));
#149711=CARTESIAN_POINT('Ctrl Pts',(-11.8927308025875,-92.23255966739,65.740692166119));
#149712=CARTESIAN_POINT('Ctrl Pts',(-15.7174074004949,-88.05102698964,65.612205998375));
#149713=CARTESIAN_POINT('Ctrl Pts',(-15.2061864647479,-88.16296384459,65.646084060879));
#149714=CARTESIAN_POINT('Ctrl Pts',(-14.2052830448809,-88.52771792363,65.636424008647));
#149715=CARTESIAN_POINT('Ctrl Pts',(-12.8988133538895,-89.49944296408,65.369043826289));
#149716=CARTESIAN_POINT('Ctrl Pts',(-11.9622505755144,-90.76922838303,64.884337945583));
#149717=CARTESIAN_POINT('Ctrl Pts',(-11.6659998956679,-91.70174963819,64.458710962093));
#149718=CARTESIAN_POINT('Ctrl Pts',(-11.5976315022519,-92.16971281076,64.230273662566));
#149719=CARTESIAN_POINT('Ctrl Pts',(-15.7267394992299,-87.66571800126,64.991418639046));
#149720=CARTESIAN_POINT('Ctrl Pts',(-15.1845687552979,-87.78154939555,65.06139114091));
#149721=CARTESIAN_POINT('Ctrl Pts',(-14.1052496752619,-88.17324122689,65.106795438126));
#149722=CARTESIAN_POINT('Ctrl Pts',(-12.6906903787521,-89.25108309904,64.837337670906));
#149723=CARTESIAN_POINT('Ctrl Pts',(-11.7189249564791,-90.65200901472,64.267339208866));
#149724=CARTESIAN_POINT('Ctrl Pts',(-11.4634864352539,-91.64605309874,63.752821353271));
#149725=CARTESIAN_POINT('Ctrl Pts',(-11.4264214263539,-92.13117582295,63.479506114825));
#149726=CARTESIAN_POINT('',(-12.4950500697605,-92.2592915992045,72.9888916301979));
#149727=CARTESIAN_POINT('Ctrl Pts',(-12.4950500697605,-92.2592915992045,
72.9888916301979));
#149728=CARTESIAN_POINT('Ctrl Pts',(-12.4950499645961,-92.2592918029314,
72.6614778940476));
#149729=CARTESIAN_POINT('Ctrl Pts',(-12.491624737793,-92.25830728403,72.3313232059512));
#149730=CARTESIAN_POINT('Ctrl Pts',(-12.4845501034544,-92.2563257071442,
71.9984875391328));
#149731=CARTESIAN_POINT('Ctrl Pts',(-12.4775098513783,-92.2543537605931,
71.6672694319906));
#149732=CARTESIAN_POINT('Ctrl Pts',(-12.4668556073995,-92.2513942171472,
71.3333959665445));
#149733=CARTESIAN_POINT('Ctrl Pts',(-12.4523224890172,-92.2474120640036,
70.9969401667793));
#149734=CARTESIAN_POINT('Ctrl Pts',(-12.4379614328067,-92.2434770568269,
70.6644677733357));
#149735=CARTESIAN_POINT('Ctrl Pts',(-12.4198128355913,-92.2385431083273,
70.3294734603283));
#149736=CARTESIAN_POINT('Ctrl Pts',(-12.3975777779154,-92.2325586333523,
69.9920467993465));
#149737=CARTESIAN_POINT('Ctrl Pts',(-12.384491286254,-92.2290364575613,
69.7934536025296));
#149738=CARTESIAN_POINT('Ctrl Pts',(-12.369988449416,-92.2251500697599,
69.5940182420788));
#149739=CARTESIAN_POINT('Ctrl Pts',(-12.3540010848255,-92.2208870301984,
69.3937629526273));
#149740=CARTESIAN_POINT('Ctrl Pts',(-12.3376237210235,-92.2165199971327,
69.1886225925616));
#149741=CARTESIAN_POINT('Ctrl Pts',(-12.3196885500552,-92.2117576623272,
68.9826217608456));
#149742=CARTESIAN_POINT('Ctrl Pts',(-12.3001162617764,-92.2065859680532,
68.7757882374567));
#149743=CARTESIAN_POINT('Ctrl Pts',(-12.290330117637,-92.2040001209162,
68.6723714757622));
#149744=CARTESIAN_POINT('Ctrl Pts',(-12.2801346070993,-92.2013118947475,
68.5687465506039));
#149745=CARTESIAN_POINT('Ctrl Pts',(-12.2695192254143,-92.198519576097,
68.4649174124185));
#149746=CARTESIAN_POINT('Ctrl Pts',(-12.2642115345717,-92.1971234167717,
68.4130028433258));
#149747=CARTESIAN_POINT('Ctrl Pts',(-12.2587988707683,-92.1957012318768,
68.3610372214912));
#149748=CARTESIAN_POINT('Ctrl Pts',(-12.253279885861,-92.1942528057138,
68.3090210593462));
#149749=CARTESIAN_POINT('Ctrl Pts',(-12.2505203934074,-92.1935285926323,
68.2830129782737));
#149750=CARTESIAN_POINT('Ctrl Pts',(-12.247734320347,-92.1927978190947,
68.2569922621632));
#149751=CARTESIAN_POINT('Ctrl Pts',(-12.2449214958836,-92.1920604584762,
68.2309589769342));
#149752=CARTESIAN_POINT('Ctrl Pts',(-12.2421086714201,-92.1913230978577,
68.2049256917052));
#149753=CARTESIAN_POINT('Ctrl Pts',(-12.2390463837868,-92.1905208353914,
68.1768552411708));
#149754=CARTESIAN_POINT('Ctrl Pts',(-12.2364025960719,-92.1898285886005,
68.1528214804896));
#149755=CARTESIAN_POINT('Ctrl Pts',(-12.1941019926332,-92.1787526399455,
67.7682813095912));
#149756=CARTESIAN_POINT('Ctrl Pts',(-12.1466029853855,-92.1665260937355,
67.3874265867434));
#149757=CARTESIAN_POINT('Ctrl Pts',(-12.0939475661605,-92.1531019687639,
67.0104245935852));
#149758=CARTESIAN_POINT('Ctrl Pts',(-12.044461672975,-92.1404858919339,
66.6561157562667));
#149759=CARTESIAN_POINT('Ctrl Pts',(-11.990420891063,-92.1268113856426,
66.305209676447));
#149760=CARTESIAN_POINT('Ctrl Pts',(-11.9318247232044,-92.1120654825007,
65.9578628232496));
#149761=CARTESIAN_POINT('Ctrl Pts',(-11.8750461046509,-92.0977769711471,
65.6212900540016));
#149762=CARTESIAN_POINT('Ctrl Pts',(-11.8139898351115,-92.0824817906833,
65.2880590602539));
#149763=CARTESIAN_POINT('Ctrl Pts',(-11.7486284014674,-92.0662034766387,
64.9583306855135));
#149764=CARTESIAN_POINT('Ctrl Pts',(-11.6860810945097,-92.0506260229549,
64.642798716312));
#149765=CARTESIAN_POINT('Ctrl Pts',(-11.619590763227,-92.0341477884734,
64.330474329946));
#149766=CARTESIAN_POINT('Ctrl Pts',(-11.5491159559696,-92.0168306342924,
64.0215155315664));
#149767=CARTESIAN_POINT('Ctrl Pts',(-11.5266264088242,-92.0113044757893,
63.9229222365642));
#149768=CARTESIAN_POINT('Ctrl Pts',(-11.5037310060279,-92.0056932411832,
63.8246718023983));
#149769=CARTESIAN_POINT('Ctrl Pts',(-11.4804281687818,-92.,63.72676972225));
#149770=CARTESIAN_POINT('Ctrl Pts',(-11.4804394788205,-91.9999117027221,
82.2509615003081));
#149771=CARTESIAN_POINT('Ctrl Pts',(-11.5530700737656,-92.0176752428972,
81.9458308790911));
#149772=CARTESIAN_POINT('Ctrl Pts',(-11.6217432522474,-92.0346347091691,
81.6373099655569));
#149773=CARTESIAN_POINT('Ctrl Pts',(-11.6865041851513,-92.0507147503459,
81.3255602912215));
#149774=CARTESIAN_POINT('Ctrl Pts',(-11.7540919465117,-92.0674966887306,
81.000202677482));
#149775=CARTESIAN_POINT('Ctrl Pts',(-11.8174191484055,-92.0833212628977,
80.6713283984278));
#149776=CARTESIAN_POINT('Ctrl Pts',(-11.8765199305579,-92.0981530040061,
80.3391017829893));
#149777=CARTESIAN_POINT('Ctrl Pts',(-11.8914927191536,-92.1019105265977,
80.2549343879455));
#149778=CARTESIAN_POINT('Ctrl Pts',(-11.9061941332142,-92.1056045451107,
80.1705517335308));
#149779=CARTESIAN_POINT('Ctrl Pts',(-11.9206244884779,-92.109234899873,
80.0859562980525));
#149780=CARTESIAN_POINT('Ctrl Pts',(-11.980343758288,-92.1242589330027,
79.7358625170093));
#149781=CARTESIAN_POINT('Ctrl Pts',(-12.0354233298406,-92.1381898452128,
79.3821260864904));
#149782=CARTESIAN_POINT('Ctrl Pts',(-12.0858651976485,-92.1510401785318,
79.024909586593));
#149783=CARTESIAN_POINT('Ctrl Pts',(-12.0886225005406,-92.1517426160656,
79.0053830676297));
#149784=CARTESIAN_POINT('Ctrl Pts',(-12.0913659372046,-92.1524418329199,
78.9858461451773));
#149785=CARTESIAN_POINT('Ctrl Pts',(-12.0940955049538,-92.153137833817,
78.9662988441322));
#149786=CARTESIAN_POINT('Ctrl Pts',(-12.1204275305434,-92.1598521252785,
78.7777268508298));
#149787=CARTESIAN_POINT('Ctrl Pts',(-12.1454690953703,-92.1662669790196,
78.5881890941633));
#149788=CARTESIAN_POINT('Ctrl Pts',(-12.1692162275469,-92.1723876925774,
78.3977071808957));
#149789=CARTESIAN_POINT('Ctrl Pts',(-12.1810897936351,-92.1754480493563,
78.3024662242619));
#149790=CARTESIAN_POINT('Ctrl Pts',(-12.1926397203039,-92.1784348592657,
78.2069892242869));
#149791=CARTESIAN_POINT('Ctrl Pts',(-12.2038652288885,-92.1813489786785,
78.1112787478959));
#149792=CARTESIAN_POINT('Ctrl Pts',(-12.2094779831807,-92.182806038385,
78.0634235097003));
#149793=CARTESIAN_POINT('Ctrl Pts',(-12.2150096307703,-92.1842449246855,
78.0155099020937));
#149794=CARTESIAN_POINT('Ctrl Pts',(-12.2204600597818,-92.1856657446596,
77.9675382424531));
#149795=CARTESIAN_POINT('Ctrl Pts',(-12.2231852742876,-92.1863761546466,
77.9435524126328));
#149796=CARTESIAN_POINT('Ctrl Pts',(-12.2258901840184,-92.187082047999,
77.9195520697877));
#149797=CARTESIAN_POINT('Ctrl Pts',(-12.2285747738969,-92.1877834386385,
77.8955372531514));
#149798=CARTESIAN_POINT('Ctrl Pts',(-12.2312593637755,-92.188484829278,
77.8715224365152));
#149799=CARTESIAN_POINT('Ctrl Pts',(-12.2337037293511,-92.1891241280636,
77.84949293961));
#149800=CARTESIAN_POINT('Ctrl Pts',(-12.236567568283,-92.189874116359,77.8234494209454));
#149801=CARTESIAN_POINT('Ctrl Pts',(-12.2736228920444,-92.1995782441962,
77.4864713160506));
#149802=CARTESIAN_POINT('Ctrl Pts',(-12.3061816785662,-92.208175820577,
77.1515711996581));
#149803=CARTESIAN_POINT('Ctrl Pts',(-12.3345957999658,-92.2157260680699,
76.8188790499968));
#149804=CARTESIAN_POINT('Ctrl Pts',(-12.363731878687,-92.2234681552605,
76.4777337255931));
#149805=CARTESIAN_POINT('Ctrl Pts',(-12.3885100948304,-92.2301097342852,
76.1389096533919));
#149806=CARTESIAN_POINT('Ctrl Pts',(-12.409264189783,-92.2357117772265,
75.8025164120411));
#149807=CARTESIAN_POINT('Ctrl Pts',(-12.4301989546193,-92.2413625874327,
75.4631947785863));
#149808=CARTESIAN_POINT('Ctrl Pts',(-12.4470391638925,-92.2459562388365,
75.1263460665604));
#149809=CARTESIAN_POINT('Ctrl Pts',(-12.4600815069596,-92.2495426758459,
74.7920579531015));
#149810=CARTESIAN_POINT('Ctrl Pts',(-12.4732389077876,-92.2531607519104,
74.4548207957765));
#149811=CARTESIAN_POINT('Ctrl Pts',(-12.4825310889809,-92.2557541419737,
74.1201892216622));
#149812=CARTESIAN_POINT('Ctrl Pts',(-12.4882171413017,-92.2573542389111,
73.7882342603867));
#149813=CARTESIAN_POINT('Ctrl Pts',(-12.4928112169424,-92.2586470455806,
73.5200295173804));
#149814=CARTESIAN_POINT('Ctrl Pts',(-12.4950503743449,-92.2592910724911,
73.2535716056014));
#149815=CARTESIAN_POINT('Ctrl Pts',(-12.4950500697605,-92.2592915992045,
72.9888916301979));
#149816=CARTESIAN_POINT('Origin',(27.4324635166691,-92.,72.98888938658));
#149817=CARTESIAN_POINT('',(-9.38953228746991,-92.,57.36388938658));
#149818=CARTESIAN_POINT('Origin',(27.4324635166691,-92.,72.98888938658));
#149819=CARTESIAN_POINT('',(-8.92925733991791,-92.5,57.55920188658));
#149820=CARTESIAN_POINT('Origin',(-8.92925733991791,-92.,57.55920188658));
#149821=CARTESIAN_POINT('',(-8.92925733991791,-92.5,88.41857688658));
#149822=CARTESIAN_POINT('Origin',(27.4324635166691,-92.5,72.98888938658));
#149823=CARTESIAN_POINT('',(-9.38953228746991,-92.,88.61388938658));
#149824=CARTESIAN_POINT('Origin',(-8.92925733991791,-92.,88.41857688658));
#149825=CARTESIAN_POINT('Origin',(27.4324635166691,-92.,72.98888938658));
#149826=CARTESIAN_POINT('Origin',(27.4324635166691,25.,72.98888938658));
#149827=CARTESIAN_POINT('',(-9.38953228746991,-84.5398910625,88.61388938658));
#149828=CARTESIAN_POINT('Origin',(-2.02513312664091,-92.5,85.48888938658));
#149829=CARTESIAN_POINT('',(-9.38953228746991,84.5398910625,88.61388938658));
#149830=CARTESIAN_POINT('Ctrl Pts',(-9.38953228746991,84.5398910625,88.61388938658));
#149831=CARTESIAN_POINT('Ctrl Pts',(-9.28328709694071,83.7902390287746,
88.8642676240091));
#149832=CARTESIAN_POINT('Ctrl Pts',(-9.17708486962772,83.034411628292,89.079525122487));
#149833=CARTESIAN_POINT('Ctrl Pts',(-9.03022807503691,81.8914074774324,
89.3540432573144));
#149834=CARTESIAN_POINT('Ctrl Pts',(-8.9833075439401,81.5088622521231,89.4374960492821));
#149835=CARTESIAN_POINT('Ctrl Pts',(-8.91715535504234,80.9327286516253,
89.5511487397963));
#149836=CARTESIAN_POINT('Ctrl Pts',(-8.88513273747567,80.6440829107429,
89.6050931418994));
#149837=CARTESIAN_POINT('Ctrl Pts',(-8.84983719739325,80.3063164002716,
89.6630999929703));
#149838=CARTESIAN_POINT('Ctrl Pts',(-8.83273032606334,80.1371798585086,
89.6908850775441));
#149839=CARTESIAN_POINT('Ctrl Pts',(-8.82551731869513,80.0646384934973,
89.7025333452805));
#149840=CARTESIAN_POINT('Ctrl Pts',(-8.82073526432699,80.0162655222266,
89.71024132127));
#149841=CARTESIAN_POINT('Ctrl Pts',(-8.81853574016787,79.9938968401075,
89.7137803985326));
#149842=CARTESIAN_POINT('Ctrl Pts',(-8.73463441113909,79.1351582655722,
89.8485086409054));
#149843=CARTESIAN_POINT('Ctrl Pts',(-8.6700376843763,78.3063013527105,89.9443580231836));
#149844=CARTESIAN_POINT('Ctrl Pts',(-8.60463652245047,77.0688049043587,
90.039891957753));
#149845=CARTESIAN_POINT('Ctrl Pts',(-8.58803785671456,76.6572709083983,
90.0636744407943));
#149846=CARTESIAN_POINT('Ctrl Pts',(-8.57132975194452,76.0414171446928,
90.0875200458018));
#149847=CARTESIAN_POINT('Ctrl Pts',(-8.56712264234551,75.8363737618302,
90.093495481281));
#149848=CARTESIAN_POINT('Ctrl Pts',(-8.56146522762828,75.4267694061832,
90.101522775063));
#149849=CARTESIAN_POINT('Ctrl Pts',(-8.56001530984225,75.2234148157065,
90.1035740849179));
#149850=CARTESIAN_POINT('Ctrl Pts',(-8.5596814837813,74.195784065444,90.1040468034545));
#149851=CARTESIAN_POINT('Ctrl Pts',(-8.58177592616642,73.3716955238175,
90.0732381391729));
#149852=CARTESIAN_POINT('Ctrl Pts',(-8.64644160601741,72.132586799253,89.9788480269718));
#149853=CARTESIAN_POINT('Ctrl Pts',(-8.67320843583488,71.7190545723774,
89.9393254017685));
#149854=CARTESIAN_POINT('Ctrl Pts',(-8.72052840036103,71.0980122540328,
89.8675311439228));
#149855=CARTESIAN_POINT('Ctrl Pts',(-8.74597657546552,70.7873051003526,
89.8285040402397));
#149856=CARTESIAN_POINT('Ctrl Pts',(-8.77860779189372,70.4244879306706,
89.777379489179));
#149857=CARTESIAN_POINT('Ctrl Pts',(-8.7956318183485,70.2429979732323,89.7504030045292));
#149858=CARTESIAN_POINT('Ctrl Pts',(-8.80307665120833,70.1651991259165,
89.7385368699021));
#149859=CARTESIAN_POINT('Ctrl Pts',(-8.80807260339705,70.1133293528205,
89.7305581866391));
#149860=CARTESIAN_POINT('Ctrl Pts',(-8.81073338330673,70.0858914918537,
89.726300088025));
#149861=CARTESIAN_POINT('Ctrl Pts',(-8.96569959907365,68.4974394021023,
89.4778327794232));
#149862=CARTESIAN_POINT('Ctrl Pts',(-9.17644065970042,66.963657792137,89.116062764089));
#149863=CARTESIAN_POINT('Ctrl Pts',(-9.38953228746991,65.4601089375,88.61388938658));
#149864=CARTESIAN_POINT('',(1.23275780153909,-92.,92.79547180931));
#149865=CARTESIAN_POINT('Origin',(-2.02513312664091,-92.,85.48888938658));
#149866=CARTESIAN_POINT('',(1.23275780153909,-24.69194692623,92.79547180931));
#149867=CARTESIAN_POINT('',(1.23275780153909,-24.69194692623,92.79547180931));
#149868=CARTESIAN_POINT('',(1.23275780153909,24.69194692623,92.79547180931));
#149869=CARTESIAN_POINT('Ctrl Pts',(1.23275780153909,-24.69194692623,92.79547180931));
#149870=CARTESIAN_POINT('Ctrl Pts',(0.699306919210318,-24.1238270516451,
93.033329221926));
#149871=CARTESIAN_POINT('Ctrl Pts',(0.153641228329698,-23.4653479951291,
93.2064179486881));
#149872=CARTESIAN_POINT('Ctrl Pts',(-0.660308888464234,-22.3420906374582,
93.3764797028993));
#149873=CARTESIAN_POINT('Ctrl Pts',(-0.93091665494534,-21.9450817227518,
93.4182936546966));
#149874=CARTESIAN_POINT('Ctrl Pts',(-1.33337035782043,-21.315683657468,
93.4600658810012));
#149875=CARTESIAN_POINT('Ctrl Pts',(-1.46694860399934,-21.1002368535027,
93.4705009261982));
#149876=CARTESIAN_POINT('Ctrl Pts',(-1.66618741489872,-20.7685954742487,
93.4811094260117));
#149877=CARTESIAN_POINT('Ctrl Pts',(-1.76552499736201,-20.6006569912952,
93.4851528403169));
#149878=CARTESIAN_POINT('Ctrl Pts',(-1.88087013739072,-20.4010226228614,
93.4877069287156));
#149879=CARTESIAN_POINT('Ctrl Pts',(-1.93839884063816,-20.3002789040641,
93.4884486918558));
#149880=CARTESIAN_POINT('Ctrl Pts',(-1.96302245967253,-20.2569044814552,
93.4886524817677));
#149881=CARTESIAN_POINT('Ctrl Pts',(-1.97943111860132,-20.2279440790216,
93.4887630506161));
#149882=CARTESIAN_POINT('Ctrl Pts',(-1.98827002315454,-20.21231115855,93.4888080269244));
#149883=CARTESIAN_POINT('Ctrl Pts',(-2.4796105271812,-19.3417230633289,
93.4906078204203));
#149884=CARTESIAN_POINT('Ctrl Pts',(-2.94214572836347,-18.4235503155145,
93.4484191451384));
#149885=CARTESIAN_POINT('Ctrl Pts',(-3.59503988466488,-16.9548237203979,
93.336446286239));
#149886=CARTESIAN_POINT('Ctrl Pts',(-3.80591399159718,-16.4500036097931,
93.2910065179068));
#149887=CARTESIAN_POINT('Ctrl Pts',(-4.11145661580154,-15.6699065755372,
93.2127684219845));
#149888=CARTESIAN_POINT('Ctrl Pts',(-4.26154056320608,-15.2741413413221,
93.1711286684841));
#149889=CARTESIAN_POINT('Ctrl Pts',(-4.43184466783831,-14.8024109798352,
93.1185820511613));
#149890=CARTESIAN_POINT('Ctrl Pts',(-4.50379795258712,-14.5980970560045,
93.095258574056));
#149891=CARTESIAN_POINT('Ctrl Pts',(-4.55153628454621,-14.4614113803602,
93.0795361718871));
#149892=CARTESIAN_POINT('Ctrl Pts',(-4.5747411202905,-14.3944288506155,
93.0717748303771));
#149893=CARTESIAN_POINT('Ctrl Pts',(-4.98592652946738,-13.1973273465102,
92.932058176407));
#149894=CARTESIAN_POINT('Ctrl Pts',(-5.3198620500585,-12.0688920126009,
92.7858901900897));
#149895=CARTESIAN_POINT('Ctrl Pts',(-5.74715455760815,-10.3736116637277,
92.5721034394466));
#149896=CARTESIAN_POINT('Ctrl Pts',(-5.8773686152273,-9.80808032276836,
92.5016614623134));
#149897=CARTESIAN_POINT('Ctrl Pts',(-6.05539233988914,-8.95912647432705,
92.3998721882845));
#149898=CARTESIAN_POINT('Ctrl Pts',(-6.11185164605444,-8.67603238534623,
92.3665827064308));
#149899=CARTESIAN_POINT('Ctrl Pts',(-6.19235016148506,-8.2512270426244,
92.3178926520071));
#149900=CARTESIAN_POINT('Ctrl Pts',(-6.23155181248203,-8.03878331895086,
92.2938581923587));
#149901=CARTESIAN_POINT('Ctrl Pts',(-6.27548255450619,-7.79086046645125,
92.2664186269981));
#149902=CARTESIAN_POINT('Ctrl Pts',(-6.29853734869913,-7.65802540934062,
92.2518870126521));
#149903=CARTESIAN_POINT('Ctrl Pts',(-6.30916623139605,-7.59603047757618,
92.245152345545));
#149904=CARTESIAN_POINT('Ctrl Pts',(-6.31520813159063,-7.56060351939743,
92.2413155915439));
#149905=CARTESIAN_POINT('Ctrl Pts',(-6.31649962626153,-7.5530196494862,
92.2404949532742));
#149906=CARTESIAN_POINT('Ctrl Pts',(-6.53857587101954,-6.24625869247446,
92.0992622520935));
#149907=CARTESIAN_POINT('Ctrl Pts',(-6.69735300861218,-4.97029942653783,
91.9840774441894));
#149908=CARTESIAN_POINT('Ctrl Pts',(-6.90717880053878,-2.45972441701621,
91.8278748390932));
#149909=CARTESIAN_POINT('Ctrl Pts',(-6.95835699251618,-1.2259449036321,
91.7867701797679));
#149910=CARTESIAN_POINT('Ctrl Pts',(-6.95905409394932,1.2036155215881,91.7862240675702));
#149911=CARTESIAN_POINT('Ctrl Pts',(-6.9084204097403,2.43929636195716,91.8269083023811));
#149912=CARTESIAN_POINT('Ctrl Pts',(-6.75167133250576,4.32416856414915,
91.9436613581591));
#149913=CARTESIAN_POINT('Ctrl Pts',(-6.68586311304225,4.9576844551529,91.9917478371863));
#149914=CARTESIAN_POINT('Ctrl Pts',(-6.56554449137394,5.91579602706811,
92.0757746632258));
#149915=CARTESIAN_POINT('Ctrl Pts',(-6.52183275150553,6.23647284027476,
92.1057581128436));
#149916=CARTESIAN_POINT('Ctrl Pts',(-6.45066355615867,6.71944749393717,
92.1533845086149));
#149917=CARTESIAN_POINT('Ctrl Pts',(-6.41367824672563,6.96142467923148,
92.1778596656006));
#149918=CARTESIAN_POINT('Ctrl Pts',(-6.36803224803482,7.2445886477186,92.2074953644351));
#149919=CARTESIAN_POINT('Ctrl Pts',(-6.34457929391623,7.38638494503977,
92.2225732149781));
#149920=CARTESIAN_POINT('Ctrl Pts',(-6.33269459525855,7.45733667196975,
92.2301758281113));
#149921=CARTESIAN_POINT('Ctrl Pts',(-6.32756716935408,7.48775603599745,
92.2334475955992));
#149922=CARTESIAN_POINT('Ctrl Pts',(-6.32414132469903,7.50803816336209,
92.2356317589976));
#149923=CARTESIAN_POINT('Ctrl Pts',(-6.32220703604282,7.51946334166994,
92.2368638227256));
#149924=CARTESIAN_POINT('Ctrl Pts',(-6.12833274488395,8.66250345548086,
92.3602612590921));
#149925=CARTESIAN_POINT('Ctrl Pts',(-5.89275515319288,9.79454916349254,
92.4990711709164));
#149926=CARTESIAN_POINT('Ctrl Pts',(-5.46622706734526,11.4894172809252,
92.7127498288003));
#149927=CARTESIAN_POINT('Ctrl Pts',(-5.31185728563353,12.0538399126387,
92.7848056604388));
#149928=CARTESIAN_POINT('Ctrl Pts',(-5.06112989749341,12.8996737490626,
92.8909810572153));
#149929=CARTESIAN_POINT('Ctrl Pts',(-4.9743606690004,13.1814850093462,92.9260492732788));
#149930=CARTESIAN_POINT('Ctrl Pts',(-4.83933084495306,13.6040018719851,
92.9777219906298));
#149931=CARTESIAN_POINT('Ctrl Pts',(-4.77059724301506,13.8152102963579,
93.0033254222042));
#149932=CARTESIAN_POINT('Ctrl Pts',(-4.70002259590991,14.0263437103108,
93.0284914261226));
#149933=CARTESIAN_POINT('Ctrl Pts',(-4.65256250400756,14.1670826506304,
93.0451614472216));
#149934=CARTESIAN_POINT('Ctrl Pts',(-4.62813328271855,14.238883430196,93.0536110760009));
#149935=CARTESIAN_POINT('Ctrl Pts',(-4.22613512108353,15.4104071039695,
93.1905351366738));
#149936=CARTESIAN_POINT('Ctrl Pts',(-3.81812010120504,16.4516269765654,
93.2978637470464));
#149937=CARTESIAN_POINT('Ctrl Pts',(-3.16554630125634,17.9213708196141,
93.4102641728471));
#149938=CARTESIAN_POINT('Ctrl Pts',(-2.94130847507913,18.3959377729894,
93.4396164690059));
#149939=CARTESIAN_POINT('Ctrl Pts',(-2.59583390833896,19.0847667115912,
93.4693442746077));
#149940=CARTESIAN_POINT('Ctrl Pts',(-2.47915954494509,19.3105394425483,
93.4768697171106));
#149941=CARTESIAN_POINT('Ctrl Pts',(-2.30202538350384,19.6434431661185,
93.48431452321));
#149942=CARTESIAN_POINT('Ctrl Pts',(-2.21292800063565,19.8084561846873,
93.4870760871862));
#149943=CARTESIAN_POINT('Ctrl Pts',(-2.10808999070051,19.998453397389,93.4885580276519));
#149944=CARTESIAN_POINT('Ctrl Pts',(-2.05545313008902,20.0928225098327,
93.4888567453215));
#149945=CARTESIAN_POINT('Ctrl Pts',(-2.03284832541677,20.1331315236142,
93.4888892195676));
#149946=CARTESIAN_POINT('Ctrl Pts',(-2.01776826009236,20.1599742235681,
93.4888895497571));
#149947=CARTESIAN_POINT('Ctrl Pts',(-2.01088755578811,20.1722021291677,
93.4888809205938));
#149948=CARTESIAN_POINT('Ctrl Pts',(-1.47693698316475,21.1192411119197,
93.487381835435));
#149949=CARTESIAN_POINT('Ctrl Pts',(-0.936180877114922,21.960906935257,
93.4338723147665));
#149950=CARTESIAN_POINT('Ctrl Pts',(0.151417256604318,23.4626319241098,
93.2071274730942));
#149951=CARTESIAN_POINT('Ctrl Pts',(0.698240340815898,24.1226910896253,
93.0338047925655));
#149952=CARTESIAN_POINT('Ctrl Pts',(1.23275780153909,24.69194692623,92.79547180931));
#149953=CARTESIAN_POINT('',(1.23275780153909,92.,92.79547180931));
#149954=CARTESIAN_POINT('',(1.23275780153909,92.,92.79547180931));
#149955=CARTESIAN_POINT('',(-9.38953228746991,92.,88.61388938658));
#149956=CARTESIAN_POINT('Origin',(-2.02513312664091,92.,85.48888938658));
#149957=CARTESIAN_POINT('',(-9.38953228746991,92.,88.61388938658));
#149958=CARTESIAN_POINT('Origin',(27.4324635166691,25.,72.98888938658));
#149959=CARTESIAN_POINT('',(-11.4804281687819,92.,82.25100905091));
#149960=CARTESIAN_POINT('',(-10.7897586692519,89.96662969243,84.78133320328));
#149961=CARTESIAN_POINT('Ctrl Pts',(-11.4804281687818,92.,82.25100905091));
#149962=CARTESIAN_POINT('Ctrl Pts',(-11.3989064198707,91.7807060486943,
82.5935059199151));
#149963=CARTESIAN_POINT('Ctrl Pts',(-11.3150515968862,91.5487028907016,
82.9257444363946));
#149964=CARTESIAN_POINT('Ctrl Pts',(-11.2295974501764,91.3039859861016,
83.2477899999947));
#149965=CARTESIAN_POINT('Ctrl Pts',(-11.1430417623464,91.0561145741593,
83.5739868709863));
#149966=CARTESIAN_POINT('Ctrl Pts',(-11.0548453666189,90.7951995316041,
83.8897266165751));
#149967=CARTESIAN_POINT('Ctrl Pts',(-10.9657236454974,90.5212361406782,
84.1951029602733));
#149968=CARTESIAN_POINT('Ctrl Pts',(-10.9074027231312,90.3419555180385,
84.3949401022091));
#149969=CARTESIAN_POINT('Ctrl Pts',(-10.8486845747637,90.1570871426494,
84.5903397936053));
#149970=CARTESIAN_POINT('Ctrl Pts',(-10.7897586692526,89.96662969243,84.7813332032802));
#149971=CARTESIAN_POINT('Ctrl Pts',(-10.7897586692519,89.96662969243,84.78133320328));
#149972=CARTESIAN_POINT('Ctrl Pts',(-10.6704705500044,89.5814629807082,
85.1679754522423));
#149973=CARTESIAN_POINT('Ctrl Pts',(-10.5499815065516,89.1792964266136,
85.5377153276576));
#149974=CARTESIAN_POINT('Ctrl Pts',(-10.3694940364216,88.5505468319125,
86.0673753755885));
#149975=CARTESIAN_POINT('Ctrl Pts',(-10.2793088439709,88.229797093672,86.3259690138416));
#149976=CARTESIAN_POINT('Ctrl Pts',(-10.1895685665396,87.899484944097,86.5752917864897));
#149977=CARTESIAN_POINT('Ctrl Pts',(-10.1298784240562,87.6771518640837,
86.7394565083492));
#149978=CARTESIAN_POINT('Ctrl Pts',(-10.1003990762871,87.5660572424311,
86.8197121966598));
#149979=CARTESIAN_POINT('Ctrl Pts',(-9.83051731905192,86.5362238831801,
87.5472559457811));
#149980=CARTESIAN_POINT('Ctrl Pts',(-9.60025783789904,85.5656437994716,
88.1172919252206));
#149981=CARTESIAN_POINT('Ctrl Pts',(-9.38953228746991,84.5398910625,88.61388938658));
#149982=CARTESIAN_POINT('Origin',(27.4324635166691,92.,72.98888938658));
#149983=CARTESIAN_POINT('Origin',(27.4324635166691,92.,72.98888938658));
#149984=CARTESIAN_POINT('',(-11.4804365249865,91.9999348338944,63.7268048139011));
#149985=CARTESIAN_POINT('',(-12.4950500697606,92.2592915992044,72.9888871429622));
#149986=CARTESIAN_POINT('Ctrl Pts',(-11.4804394788206,91.9999117027221,
63.7268172728519));
#149987=CARTESIAN_POINT('Ctrl Pts',(-11.5530700739286,92.0176752429416,
64.031947894754));
#149988=CARTESIAN_POINT('Ctrl Pts',(-11.6217432526045,92.0346347092598,
64.3404688091952));
#149989=CARTESIAN_POINT('Ctrl Pts',(-11.6865041857173,92.0507147504843,
64.652218484662));
#149990=CARTESIAN_POINT('Ctrl Pts',(-11.7540919472641,92.0674966889109,
64.9775760994306));
#149991=CARTESIAN_POINT('Ctrl Pts',(-11.8174191493645,92.0833212631222,
65.3064503797548));
#149992=CARTESIAN_POINT('Ctrl Pts',(-11.8765199317249,92.0981530042764,
65.6386769967062));
#149993=CARTESIAN_POINT('Ctrl Pts',(-11.8914927197326,92.1019105267189,
65.7228443885322));
#149994=CARTESIAN_POINT('Ctrl Pts',(-11.9061941332286,92.1056045450884,
65.8072270397262));
#149995=CARTESIAN_POINT('Ctrl Pts',(-11.9206244879506,92.1092348997126,
65.8918224719814));
#149996=CARTESIAN_POINT('Ctrl Pts',(-11.9803437580264,92.1242589329019,
66.241916254385));
#149997=CARTESIAN_POINT('Ctrl Pts',(-12.035423329848,92.1381898451751,66.5956526865277));
#149998=CARTESIAN_POINT('Ctrl Pts',(-12.0858651979061,92.1510401785601,
66.952869188313));
#149999=CARTESIAN_POINT('Ctrl Pts',(-12.0886225006044,92.1517426160446,
66.9723957059099));
#150000=CARTESIAN_POINT('Ctrl Pts',(-12.0913659370766,92.1524418328501,
66.991932626995));
#150001=CARTESIAN_POINT('Ctrl Pts',(-12.094095504636,92.1531378336989,67.0114799266722));
#150002=CARTESIAN_POINT('Ctrl Pts',(-12.1204275302738,92.1598521251739,
67.2000519202346));
#150003=CARTESIAN_POINT('Ctrl Pts',(-12.1454690951536,92.1662669789315,
67.3895896772274));
#150004=CARTESIAN_POINT('Ctrl Pts',(-12.1692162273843,92.1723876925088,
67.5800715908876));
#150005=CARTESIAN_POINT('Ctrl Pts',(-12.1810897934996,92.1754480492974,
67.6753125477177));
#150006=CARTESIAN_POINT('Ctrl Pts',(-12.1926397201958,92.1784348592172,
67.7707895479056));
#150007=CARTESIAN_POINT('Ctrl Pts',(-12.2038652288077,92.1813489786412,
67.8665000245261));
#150008=CARTESIAN_POINT('Ctrl Pts',(-12.2094779831137,92.1828060383532,
67.9143552628363));
#150009=CARTESIAN_POINT('Ctrl Pts',(-12.2150096307169,92.1842449246595,
67.9622688705619));
#150010=CARTESIAN_POINT('Ctrl Pts',(-12.220460059742,92.1856657446395,68.0102405303256));
#150011=CARTESIAN_POINT('Ctrl Pts',(-12.2231852742546,92.1863761546295,
68.0342263602074));
#150012=CARTESIAN_POINT('Ctrl Pts',(-12.2258901839921,92.187082047985,68.058226703115));
#150013=CARTESIAN_POINT('Ctrl Pts',(-12.2285747738774,92.1877834386275,
68.0822415198149));
#150014=CARTESIAN_POINT('Ctrl Pts',(-12.2312593637628,92.18848482927,68.1062563365148));
#150015=CARTESIAN_POINT('Ctrl Pts',(-12.2337037293575,92.1891241280619,
68.1282858335971));
#150016=CARTESIAN_POINT('Ctrl Pts',(-12.2365675682838,92.1898741163572,
68.1543293522149));
#150017=CARTESIAN_POINT('Ctrl Pts',(-12.2736228920578,92.1995782442172,
68.4913074572907));
#150018=CARTESIAN_POINT('Ctrl Pts',(-12.3061816786017,92.2081758206156,
68.8262075739754));
#150019=CARTESIAN_POINT('Ctrl Pts',(-12.3345958000255,92.2157260681214,
69.1588997240404));
#150020=CARTESIAN_POINT('Ctrl Pts',(-12.3637318787694,92.2234681553245,
69.5000450488309));
#150021=CARTESIAN_POINT('Ctrl Pts',(-12.3885100949383,92.2301097343569,
69.8388691215366));
#150022=CARTESIAN_POINT('Ctrl Pts',(-12.4092641899117,92.2357117773015,
70.1752623635098));
#150023=CARTESIAN_POINT('Ctrl Pts',(-12.4301989547663,92.2413625875103,
70.5145839975501));
#150024=CARTESIAN_POINT('Ctrl Pts',(-12.4470391640537,92.2459562389126,
70.8514327102822));
#150025=CARTESIAN_POINT('Ctrl Pts',(-12.4600815071228,92.2495426759163,
71.185720824568));
#150026=CARTESIAN_POINT('Ctrl Pts',(-12.4732389079497,92.2531607519744,
71.5229579826459));
#150027=CARTESIAN_POINT('Ctrl Pts',(-12.4825310891311,92.2557541420275,
71.8575895576373));
#150028=CARTESIAN_POINT('Ctrl Pts',(-12.4882171414205,92.2573542389513,
72.1895445199136));
#150029=CARTESIAN_POINT('Ctrl Pts',(-12.4928112169792,92.2586470455938,
72.4577492604156));
#150030=CARTESIAN_POINT('Ctrl Pts',(-12.495050374345,92.2592910724909,72.7242071698142));
#150031=CARTESIAN_POINT('Ctrl Pts',(-12.4950500697606,92.2592915992044,
72.9888871429622));
#150032=CARTESIAN_POINT('Ctrl Pts',(-12.4950500697606,92.2592915992044,
72.9888871429622));
#150033=CARTESIAN_POINT('Ctrl Pts',(-12.4950499645961,92.2592918029315,
73.3163008749631));
#150034=CARTESIAN_POINT('Ctrl Pts',(-12.4916247378875,92.2583072840424,
73.6464555593212));
#150035=CARTESIAN_POINT('Ctrl Pts',(-12.4845501037104,92.2563257071815,
73.9792912228145));
#150036=CARTESIAN_POINT('Ctrl Pts',(-12.4775098517978,92.254353760656,74.3105093265076));
#150037=CARTESIAN_POINT('Ctrl Pts',(-12.4668556080519,92.2513942172489,
74.6443827889115));
#150038=CARTESIAN_POINT('Ctrl Pts',(-12.4523224899448,92.2474120641582,
74.9808385860427));
#150039=CARTESIAN_POINT('Ctrl Pts',(-12.4379614340165,92.2434770570366,
75.3133109766448));
#150040=CARTESIAN_POINT('Ctrl Pts',(-12.4198128371299,92.2385431086074,
75.6483052872056));
#150041=CARTESIAN_POINT('Ctrl Pts',(-12.3975777798044,92.2325586337195,
75.9857319461363));
#150042=CARTESIAN_POINT('Ctrl Pts',(-12.3844912877986,92.2290364578315,
76.1843251501014));
#150043=CARTESIAN_POINT('Ctrl Pts',(-12.3699884505046,92.2251500699082,
76.3837605179081));
#150044=CARTESIAN_POINT('Ctrl Pts',(-12.3540010853324,92.2208870301987,
76.5840158149206));
#150045=CARTESIAN_POINT('Ctrl Pts',(-12.3376237215031,92.2165199971329,
76.789156175612));
#150046=CARTESIAN_POINT('Ctrl Pts',(-12.3196885504839,92.2117576623274,
76.9951570081091));
#150047=CARTESIAN_POINT('Ctrl Pts',(-12.300116262123,92.2065859680533,77.2019905324337));
#150048=CARTESIAN_POINT('Ctrl Pts',(-12.2903301179426,92.2040001209163,
77.305407294596));
#150049=CARTESIAN_POINT('Ctrl Pts',(-12.2801346073562,92.2013118947475,
77.4090322202606));
#150050=CARTESIAN_POINT('Ctrl Pts',(-12.2695192256138,92.198519576097,77.5128613589908));
#150051=CARTESIAN_POINT('Ctrl Pts',(-12.2642115347425,92.1971234167717,
77.564775928356));
#150052=CARTESIAN_POINT('Ctrl Pts',(-12.2587988709082,92.1957012318767,
77.6167415504726));
#150053=CARTESIAN_POINT('Ctrl Pts',(-12.2532798859677,92.1942528057137,
77.6687577129092));
#150054=CARTESIAN_POINT('Ctrl Pts',(-12.2505203934975,92.1935285926322,
77.6947657941275));
#150055=CARTESIAN_POINT('Ctrl Pts',(-12.24773432042,92.1927978190946,77.7207865103862));
#150056=CARTESIAN_POINT('Ctrl Pts',(-12.2449214959388,92.1920604584761,
77.7468197957659));
#150057=CARTESIAN_POINT('Ctrl Pts',(-12.2421086714576,92.1913230978576,
77.7728530811455));
#150058=CARTESIAN_POINT('Ctrl Pts',(-12.2390463837698,92.1905208353823,
77.8009235321599));
#150059=CARTESIAN_POINT('Ctrl Pts',(-12.2364025960721,92.1898285886004,
77.8249572926695));
#150060=CARTESIAN_POINT('Ctrl Pts',(-12.194101992908,92.1787526400903,78.2094974608232));
#150061=CARTESIAN_POINT('Ctrl Pts',(-12.1466029859566,92.1665260939933,
78.5903521816213));
#150062=CARTESIAN_POINT('Ctrl Pts',(-12.0939475669821,92.1531019690993,
78.9673541734208));
#150063=CARTESIAN_POINT('Ctrl Pts',(-12.0444616746194,92.140485892492,79.3216630052577));
#150064=CARTESIAN_POINT('Ctrl Pts',(-11.9904208935979,92.1268113864172,
79.6725690802869));
#150065=CARTESIAN_POINT('Ctrl Pts',(-11.9318247266413,92.1120654834831,
80.0199159293835));
#150066=CARTESIAN_POINT('Ctrl Pts',(-11.8750461090089,92.0977769723428,
80.356488694378));
#150067=CARTESIAN_POINT('Ctrl Pts',(-11.8139898404085,92.0824817920859,
80.6897196845255));
#150068=CARTESIAN_POINT('Ctrl Pts',(-11.7486284076709,92.0662034782385,
81.0194480563154));
#150069=CARTESIAN_POINT('Ctrl Pts',(-11.6860811016712,92.0506260247658,
81.3349800222365));
#150070=CARTESIAN_POINT('Ctrl Pts',(-11.619590771328,92.0341477904893,81.6473044059264));
#150071=CARTESIAN_POINT('Ctrl Pts',(-11.5491159649485,92.0168306365032,
81.9562632022298));
#150072=CARTESIAN_POINT('Ctrl Pts',(-11.5266264149309,92.0113044772877,
82.0548565103891));
#150073=CARTESIAN_POINT('Ctrl Pts',(-11.5037310091423,92.0056932419443,
82.1531069576772));
#150074=CARTESIAN_POINT('Ctrl Pts',(-11.4804281687818,92.,82.25100905091));
#150075=CARTESIAN_POINT('',(-8.92925733991791,92.5,88.41857688658));
#150076=CARTESIAN_POINT('Origin',(-8.92925733991791,92.,88.41857688658));
#150077=CARTESIAN_POINT('',(-8.92925733991791,92.5,57.55920188658));
#150078=CARTESIAN_POINT('Origin',(27.4324635166691,92.5,72.98888938658));
#150079=CARTESIAN_POINT('',(-9.38953228746991,92.,57.36388938658));
#150080=CARTESIAN_POINT('Origin',(-8.92925733991791,92.,57.55920188658));
#150081=CARTESIAN_POINT('Origin',(27.4324635166691,92.,72.98888938658));
#150082=CARTESIAN_POINT('Origin',(27.4324635166691,25.,72.98888938658));
#150083=CARTESIAN_POINT('',(-9.38953228747191,84.53989106251,57.36388938659));
#150084=CARTESIAN_POINT('',(-10.7897592617979,89.96662731952,61.19644749046));
#150085=CARTESIAN_POINT('Ctrl Pts',(-9.38953228747346,84.53989106251,57.3638893865893));
#150086=CARTESIAN_POINT('Ctrl Pts',(-9.46407393605236,84.9040360028837,
57.5395548119466));
#150087=CARTESIAN_POINT('Ctrl Pts',(-9.54149202137624,85.2622843930189,
57.7254840535312));
#150088=CARTESIAN_POINT('Ctrl Pts',(-9.62133538212254,85.6146362329159,
57.9218396698004));
#150089=CARTESIAN_POINT('Ctrl Pts',(-9.65220762867145,85.7508766512999,
57.9977625635772));
#150090=CARTESIAN_POINT('Ctrl Pts',(-9.68344192114709,85.8862354995815,
58.0752443252074));
#150091=CARTESIAN_POINT('Ctrl Pts',(-9.71501009391432,86.0207127777606,
58.1542945370059));
#150092=CARTESIAN_POINT('Ctrl Pts',(-9.79703933318159,86.3701491835071,
58.3597048654899));
#150093=CARTESIAN_POINT('Ctrl Pts',(-9.88155117347576,86.7144627113139,
58.5762881726688));
#150094=CARTESIAN_POINT('Ctrl Pts',(-9.96752404023887,87.0518501318954,
58.8029480803737));
#150095=CARTESIAN_POINT('Ctrl Pts',(-10.000205282342,87.1801026886582,58.8891093030674));
#150096=CARTESIAN_POINT('Ctrl Pts',(-10.0330980015701,87.307354408076,58.9767262639575));
#150097=CARTESIAN_POINT('Ctrl Pts',(-10.0661476244504,87.4335062383448,
59.0657373552651));
#150098=CARTESIAN_POINT('Ctrl Pts',(-10.1635306433684,87.8052214049021,
59.3280147440303));
#150099=CARTESIAN_POINT('Ctrl Pts',(-10.261646774493,88.1651378511986,59.6006888927839));
#150100=CARTESIAN_POINT('Ctrl Pts',(-10.3598592983923,88.5132555772343,
59.8839156650425));
#150101=CARTESIAN_POINT('Ctrl Pts',(-10.4570454426319,88.8577352646674,
60.164182548006));
#150102=CARTESIAN_POINT('Ctrl Pts',(-10.5543259257963,89.19066155062,60.4547829485653));
#150103=CARTESIAN_POINT('Ctrl Pts',(-10.6510347955172,89.5120344350921,
60.7558539372034));
#150104=CARTESIAN_POINT('Ctrl Pts',(-10.6974344449989,89.6662249373226,
60.9003038556258));
#150105=CARTESIAN_POINT('Ctrl Pts',(-10.7437017885551,89.8177558987986,
61.0471638206023));
#150106=CARTESIAN_POINT('Ctrl Pts',(-10.7897592617964,89.96662731952,61.1964474904605));
#150107=CARTESIAN_POINT('Ctrl Pts',(-10.7897592617979,89.96662731952,61.19644749046));
#150108=CARTESIAN_POINT('Ctrl Pts',(-11.0308907230829,90.74601077155,61.97801449744));
#150109=CARTESIAN_POINT('Ctrl Pts',(-11.2651526236999,91.42091161506,62.82233335276));
#150110=CARTESIAN_POINT('Ctrl Pts',(-11.4804394903149,91.99991170272,63.726817270116));
#150111=CARTESIAN_POINT('',(-9.38953228747191,84.53989106251,57.36388938659));
#150112=CARTESIAN_POINT('Origin',(-2.02513312664091,25.,60.48888938658));
#150113=CARTESIAN_POINT('Ctrl Pts',(-9.38953228746991,65.4601089375,57.36388938658));
#150114=CARTESIAN_POINT('Ctrl Pts',(-9.28299760589922,66.2118050055448,
57.1128289323244));
#150115=CARTESIAN_POINT('Ctrl Pts',(-9.17640320161983,66.9710984420553,
56.8968437256938));
#150116=CARTESIAN_POINT('Ctrl Pts',(-9.02882006242401,68.1214346495195,
56.6211725879589));
#150117=CARTESIAN_POINT('Ctrl Pts',(-8.98163454412516,68.5067793941239,
56.537325043936));
#150118=CARTESIAN_POINT('Ctrl Pts',(-8.91505371445119,69.0876455242053,
56.423063827724));
#150119=CARTESIAN_POINT('Ctrl Pts',(-8.88280899764823,69.3787908425396,
56.368811046357));
#150120=CARTESIAN_POINT('Ctrl Pts',(-8.84724153254128,69.7197068238602,
56.3104368697525));
#150121=CARTESIAN_POINT('Ctrl Pts',(-8.82999560525437,69.8904764253365,
56.2824661787672));
#150122=CARTESIAN_POINT('Ctrl Pts',(-8.82272235145676,69.963730171144,56.2707379426146));
#150123=CARTESIAN_POINT('Ctrl Pts',(-8.81789998947213,70.0125808402926,
56.2629765596535));
#150124=CARTESIAN_POINT('Ctrl Pts',(-8.8156468607298,70.0355293404337,56.2593567797579));
#150125=CARTESIAN_POINT('Ctrl Pts',(-8.73217725899094,70.8910354288936,
56.1255245945254));
#150126=CARTESIAN_POINT('Ctrl Pts',(-8.66805506192528,71.7188625011877,
56.0304808759467));
#150127=CARTESIAN_POINT('Ctrl Pts',(-8.60339061485563,72.9579712257644,
55.936089919193));
#150128=CARTESIAN_POINT('Ctrl Pts',(-8.58704180991737,73.3705688199792,
55.912677597908));
#150129=CARTESIAN_POINT('Ctrl Pts',(-8.57070859794248,73.9888072403353,
55.8893750942764));
#150130=CARTESIAN_POINT('Ctrl Pts',(-8.56662647565255,74.1947770519598,
55.8835786701559));
#150131=CARTESIAN_POINT('Ctrl Pts',(-8.56121809111756,74.6064973515531,
55.8759060387761));
#150132=CARTESIAN_POINT('Ctrl Pts',(-8.5598922203733,74.8136830320495,55.874030385872));
#150133=CARTESIAN_POINT('Ctrl Pts',(-8.56017384125938,75.8347112001197,
55.8744291786228));
#150134=CARTESIAN_POINT('Ctrl Pts',(-8.58277625686546,76.6556212834695,
55.9059564905199));
#150135=CARTESIAN_POINT('Ctrl Pts',(-8.64817866699516,77.8931177318349,
56.0014895705745));
#150136=CARTESIAN_POINT('Ctrl Pts',(-8.67518679071417,78.3066384351802,
56.0414040317839));
#150137=CARTESIAN_POINT('Ctrl Pts',(-8.72285528790153,78.9284523210332,
56.1138062125588));
#150138=CARTESIAN_POINT('Ctrl Pts',(-8.74847436625218,79.2397424716684,
56.1531423150821));
#150139=CARTESIAN_POINT('Ctrl Pts',(-8.78129743014201,79.6035849275667,
56.204636960379));
#150140=CARTESIAN_POINT('Ctrl Pts',(-8.79841527834941,79.7856738088883,
56.2318009811848));
#150141=CARTESIAN_POINT('Ctrl Pts',(-8.80589984657566,79.8637478266061,
56.2437480312129));
#150142=CARTESIAN_POINT('Ctrl Pts',(-8.81092218104148,79.9158051552451,
56.2517807797114));
#150143=CARTESIAN_POINT('Ctrl Pts',(-8.81362946612071,79.9436783214225,
56.2561199096899));
#150144=CARTESIAN_POINT('Ctrl Pts',(-8.96727708087226,81.5164272720892,
56.5028463122281));
#150145=CARTESIAN_POINT('Ctrl Pts',(-9.1770201042476,83.0404328065509,56.863081532569));
#150146=CARTESIAN_POINT('Ctrl Pts',(-9.38953228747191,84.53989106251,57.36388938659));
#150147=CARTESIAN_POINT('',(1.23275780153909,92.,53.18230696385));
#150148=CARTESIAN_POINT('Origin',(-2.02513312664091,92.,60.48888938658));
#150149=CARTESIAN_POINT('',(1.23275780350218,24.13180332306,53.1823069610377));
#150150=CARTESIAN_POINT('',(1.23275780153909,92.,53.18230696385));
#150151=CARTESIAN_POINT('',(-2.42457387236482,16.9255393804567,52.4988701141421));
#150152=CARTESIAN_POINT('Ctrl Pts',(1.23275780212727,24.13180332306,53.1823069641211));
#150153=CARTESIAN_POINT('Ctrl Pts',(1.09525026227048,23.9222975650672,53.1209945008038));
#150154=CARTESIAN_POINT('Ctrl Pts',(0.957371605292284,23.7068349358274,
53.0640496456824));
#150155=CARTESIAN_POINT('Ctrl Pts',(0.819366193047706,23.4853492447597,
53.0113999264875));
#150156=CARTESIAN_POINT('Ctrl Pts',(0.678897420682025,23.2599100926654,
52.9578104237252));
#150157=CARTESIAN_POINT('Ctrl Pts',(0.538297793952373,23.0282309049978,
52.9086708304224));
#150158=CARTESIAN_POINT('Ctrl Pts',(0.397838434541305,22.7902825142855,
52.8638717634787));
#150159=CARTESIAN_POINT('Ctrl Pts',(0.256254933206571,22.5504297452335,
52.8187141550358));
#150160=CARTESIAN_POINT('Ctrl Pts',(0.114814424623342,22.3042070568793,
52.7779668212956));
#150161=CARTESIAN_POINT('Ctrl Pts',(-0.0261990531770868,22.0516254172157,
52.7414840959157));
#150162=CARTESIAN_POINT('Ctrl Pts',(-0.169023217529076,21.7958004976526,
52.7045329133272));
#150163=CARTESIAN_POINT('Ctrl Pts',(-0.311408876098802,21.5334522976639,
52.6719565200889));
#150164=CARTESIAN_POINT('Ctrl Pts',(-0.45306134541689,21.2646335721508,
52.6435694854777));
#150165=CARTESIAN_POINT('Ctrl Pts',(-0.516137561329358,21.1449316844717,
52.6309290653504));
#150166=CARTESIAN_POINT('Ctrl Pts',(-0.57906844504845,21.0239473502742,
52.6191188750192));
#150167=CARTESIAN_POINT('Ctrl Pts',(-0.641828334153602,20.9016877827935,
52.6081204724598));
#150168=CARTESIAN_POINT('Ctrl Pts',(-0.769429273692215,20.653114436018,
52.5857589527053));
#150169=CARTESIAN_POINT('Ctrl Pts',(-0.896236804350713,20.3991574139139,
52.5667689819771));
#150170=CARTESIAN_POINT('Ctrl Pts',(-1.02217945969569,20.1398812142133,
52.550955736531));
#150171=CARTESIAN_POINT('Ctrl Pts',(-1.14550571933736,19.8859913479436,
52.5354710033536));
#150172=CARTESIAN_POINT('Ctrl Pts',(-1.26800325069717,19.6270006376272,
52.5230327116852));
#150173=CARTESIAN_POINT('Ctrl Pts',(-1.38957325127653,19.3629328949489,
52.513467924596));
#150174=CARTESIAN_POINT('Ctrl Pts',(-1.50940787880506,19.1026346352191,
52.5040396717971));
#150175=CARTESIAN_POINT('Ctrl Pts',(-1.62834174173715,18.8374029165924,
52.4974038626211));
#150176=CARTESIAN_POINT('Ctrl Pts',(-1.74624125684383,18.567229635568,52.4933993676503));
#150177=CARTESIAN_POINT('Ctrl Pts',(-1.86159178806976,18.3028974925474,
52.4894814497374));
#150178=CARTESIAN_POINT('Ctrl Pts',(-1.97595248783855,18.0338347696117,
52.4880827511661));
#150179=CARTESIAN_POINT('Ctrl Pts',(-2.08915530741183,17.7600093880497,
52.4890505267765));
#150180=CARTESIAN_POINT('Ctrl Pts',(-2.16757198876065,17.57032791393,52.4897209142451));
#150181=CARTESIAN_POINT('Ctrl Pts',(-2.245432170471,17.378360579323,52.491526829913));
#150182=CARTESIAN_POINT('Ctrl Pts',(-2.32266658659977,17.1840910996425,
52.4944150526792));
#150183=CARTESIAN_POINT('Ctrl Pts',(-2.32911013941652,17.1678834850097,
52.494656012822));
#150184=CARTESIAN_POINT('Ctrl Pts',(-2.33569707077722,17.1517522798405,
52.4949096119963));
#150185=CARTESIAN_POINT('Ctrl Pts',(-2.34230749508296,17.1356174290227,
52.4951723835218));
#150186=CARTESIAN_POINT('Ctrl Pts',(-2.34891128208127,17.1194987786725,
52.4954348912071));
#150187=CARTESIAN_POINT('Ctrl Pts',(-2.35553848932307,17.1033765093641,
52.4957065085865));
#150188=CARTESIAN_POINT('Ctrl Pts',(-2.36211074522106,17.0872026605915,
52.4959841149558));
#150189=CARTESIAN_POINT('Ctrl Pts',(-2.36868537913477,17.0710229596933,
52.4962618217703));
#150190=CARTESIAN_POINT('Ctrl Pts',(-2.37520500345411,17.0547916624888,
52.4965454828214));
#150191=CARTESIAN_POINT('Ctrl Pts',(-2.38163270894705,17.0384923626739,
52.4968329239004));
#150192=CARTESIAN_POINT('Ctrl Pts',(-2.38806757573677,17.022174903327,52.4971206852261));
#150193=CARTESIAN_POINT('Ctrl Pts',(-2.39441031079806,17.0057893164205,
52.497412192531));
#150194=CARTESIAN_POINT('Ctrl Pts',(-2.40066571962354,16.9893504652935,
52.4977068239092));
#150195=CARTESIAN_POINT('Ctrl Pts',(-2.40693939534868,16.9728636098151,
52.4980023156632));
#150196=CARTESIAN_POINT('Ctrl Pts',(-2.41312522812776,16.9563232079188,
52.4983009013797));
#150197=CARTESIAN_POINT('Ctrl Pts',(-2.41927024760488,16.9397753383813,
52.4986042071812));
#150198=CARTESIAN_POINT('Ctrl Pts',(-2.42103391321132,16.9350259785994,
52.4986912581682));
#150199=CARTESIAN_POINT('Ctrl Pts',(-2.42279448210005,16.9302761973306,
52.4987787146876));
#150200=CARTESIAN_POINT('Ctrl Pts',(-2.424553705362,16.9255275487788,52.4988666581252));
#150201=CARTESIAN_POINT('',(-2.42458295845305,-16.925539708287,52.4988706296686));
#150202=CARTESIAN_POINT('',(-2.42460157766091,-16.92552641542,52.49887156046));
#150203=CARTESIAN_POINT('',(1.23275780153909,-24.13180332393,53.18230696385));
#150204=CARTESIAN_POINT('Ctrl Pts',(-2.42455466529549,-16.925524957794,
52.4988667061117));
#150205=CARTESIAN_POINT('Ctrl Pts',(-2.41835263264369,-16.9422743869142,
52.4985566662608));
#150206=CARTESIAN_POINT('Ctrl Pts',(-2.41213098287879,-16.9590344309857,
52.4982525085495));
#150207=CARTESIAN_POINT('Ctrl Pts',(-2.40583009662638,-16.9757502119588,
52.497951814072));
#150208=CARTESIAN_POINT('Ctrl Pts',(-2.39954460352843,-16.9924251560419,
52.4976518541954));
#150209=CARTESIAN_POINT('Ctrl Pts',(-2.39318026048568,-17.0090560171085,
52.4973553905347));
#150210=CARTESIAN_POINT('Ctrl Pts',(-2.38671975157702,-17.0256188820132,
52.4970624787638));
#150211=CARTESIAN_POINT('Ctrl Pts',(-2.38027083356337,-17.0421520312358,
52.4967700925103));
#150212=CARTESIAN_POINT('Ctrl Pts',(-2.37372610356048,-17.0586174007026,
52.4964812904674));
#150213=CARTESIAN_POINT('Ctrl Pts',(-2.36711004809713,-17.0750221742194,
52.4961978656708));
#150214=CARTESIAN_POINT('Ctrl Pts',(-2.36049508485471,-17.0914242395308,
52.4959144876638));
#150215=CARTESIAN_POINT('Ctrl Pts',(-2.35380883249986,-17.1077657033903,
52.4956365252539));
#150216=CARTESIAN_POINT('Ctrl Pts',(-2.34711735211228,-17.1240851396031,
52.4953668745901));
#150217=CARTESIAN_POINT('Ctrl Pts',(-2.3404188180097,-17.1404217786837,
52.4950969396784));
#150218=CARTESIAN_POINT('Ctrl Pts',(-2.33371506507477,-17.1567363204905,
52.4948353762192));
#150219=CARTESIAN_POINT('Ctrl Pts',(-2.32711380675133,-17.1730992969542,
52.4945855879091));
#150220=CARTESIAN_POINT('Ctrl Pts',(-2.32505536676958,-17.1782016885473,
52.4945076975708));
#150221=CARTESIAN_POINT('Ctrl Pts',(-2.32300719438366,-17.1833090236636,
52.4944309532452));
#150222=CARTESIAN_POINT('Ctrl Pts',(-2.32097337228297,-17.188424077842,
52.4943554571288));
#150223=CARTESIAN_POINT('Ctrl Pts',(-2.21954797925199,-17.4435085221712,
52.4905905146218));
#150224=CARTESIAN_POINT('Ctrl Pts',(-2.11702976879158,-17.6945893285042,
52.4887010808945));
#150225=CARTESIAN_POINT('Ctrl Pts',(-2.01359961223417,-17.9417144089226,
52.4888021911267));
#150226=CARTESIAN_POINT('Ctrl Pts',(-1.9086896659158,-18.1923751425378,
52.4889047479572));
#150227=CARTESIAN_POINT('Ctrl Pts',(-1.80284129394811,-18.4389665694389,
52.4910546547565));
#150228=CARTESIAN_POINT('Ctrl Pts',(-1.69619391444929,-18.6815194107603,
52.4953644233417));
#150229=CARTESIAN_POINT('Ctrl Pts',(-1.58746267668813,-18.9288116628841,
52.4997584035308));
#150230=CARTESIAN_POINT('Ctrl Pts',(-1.47790061381537,-19.171906378998,
52.5063969849476));
#150231=CARTESIAN_POINT('Ctrl Pts',(-1.36760821367348,-19.4108097918281,
52.5153996784079));
#150232=CARTESIAN_POINT('Ctrl Pts',(-1.25621699724117,-19.6520933411093,
52.5244920635081));
#150233=CARTESIAN_POINT('Ctrl Pts',(-1.14408033744016,-19.889102004872,
52.5359954900293));
#150234=CARTESIAN_POINT('Ctrl Pts',(-1.03125997888467,-20.1218098515863,
52.5500402330157));
#150235=CARTESIAN_POINT('Ctrl Pts',(-0.91722611671491,-20.3570207200662,
52.5642360422334));
#150236=CARTESIAN_POINT('Ctrl Pts',(-0.802493180553639,-20.5878380901434,
52.5810277926978));
#150237=CARTESIAN_POINT('Ctrl Pts',(-0.68709057782042,-20.8141971117313,
52.6005629759781));
#150238=CARTESIAN_POINT('Ctrl Pts',(-0.671716883247116,-20.8443521895145,
52.6031654124403));
#150239=CARTESIAN_POINT('Ctrl Pts',(-0.656331262552002,-20.8744280858999,
52.6058165594344));
#150240=CARTESIAN_POINT('Ctrl Pts',(-0.640933749040346,-20.9044245923751,
52.6085167874446));
#150241=CARTESIAN_POINT('Ctrl Pts',(-0.501024753429229,-21.1769868531328,
52.6330523196617));
#150242=CARTESIAN_POINT('Ctrl Pts',(-0.360277472641413,-21.4431663440956,
52.6616144460825));
#150243=CARTESIAN_POINT('Ctrl Pts',(-0.218979784607261,-21.7028881581558,
52.6943972178819));
#150244=CARTESIAN_POINT('Ctrl Pts',(-0.0790390129840126,-21.9601157998295,
52.72686516867));
#150245=CARTESIAN_POINT('Ctrl Pts',(0.0614412526471609,-22.2110091853603,
52.7634731492255));
#150246=CARTESIAN_POINT('Ctrl Pts',(0.202178786129167,-22.4555374170789,
52.8043804173196));
#150247=CARTESIAN_POINT('Ctrl Pts',(0.342131600715697,-22.6987022177414,
52.8450595962505));
#150248=CARTESIAN_POINT('Ctrl Pts',(0.482338366082033,-22.9355726349923,
52.88999025376));
#150249=CARTESIAN_POINT('Ctrl Pts',(0.622525337285318,-23.1661601006708,
52.9392994974083));
#150250=CARTESIAN_POINT('Ctrl Pts',(0.760950939843198,-23.3938503674971,
52.9879891987772));
#150251=CARTESIAN_POINT('Ctrl Pts',(0.899356763048862,-23.6154146140776,
53.0409480806527));
#150252=CARTESIAN_POINT('Ctrl Pts',(1.03748989378346,-23.8309044364283,
53.0982702636116));
#150253=CARTESIAN_POINT('Ctrl Pts',(1.10264808140848,-23.9325522178211,
53.1253094650867));
#150254=CARTESIAN_POINT('Ctrl Pts',(1.16774579196361,-24.0328489872031,
53.1533191246783));
#150255=CARTESIAN_POINT('Ctrl Pts',(1.23275780153649,-24.13180332393,53.1823069638558));
#150256=CARTESIAN_POINT('',(1.23275780153909,-92.,53.18230696385));
#150257=CARTESIAN_POINT('',(1.23275780153909,-24.13180332393,53.18230696385));
#150258=CARTESIAN_POINT('Origin',(-2.02513312664091,-92.,60.48888938658));
#150259=CARTESIAN_POINT('',(-9.38953228746991,-92.,57.36388938658));
#150260=CARTESIAN_POINT('Ctrl Pts',(-15.7857783725339,63.70338519495,63.115509260727));
#150261=CARTESIAN_POINT('Ctrl Pts',(-13.2009589750562,63.38469268621,63.626388245956));
#150262=CARTESIAN_POINT('Ctrl Pts',(-11.2043264355729,61.80998487044,62.8661053606));
#150263=CARTESIAN_POINT('Ctrl Pts',(-10.7993789544399,59.77045106498,61.21655661769));
#150264=CARTESIAN_POINT('Ctrl Pts',(-15.2179723740729,64.90944119133,61.73606668886));
#150265=CARTESIAN_POINT('Ctrl Pts',(-12.7684152553161,64.50610810913,62.2234622344801));
#150266=CARTESIAN_POINT('Ctrl Pts',(-10.8253714758609,63.1180161071301,
61.36857549733));
#150267=CARTESIAN_POINT('Ctrl Pts',(-10.2917538862999,61.39001548839,59.56845212723));
#150268=CARTESIAN_POINT('Ctrl Pts',(-14.6117331505179,66.35834909817,60.58580302675));
#150269=CARTESIAN_POINT('Ctrl Pts',(-12.2792545314683,65.93351518384,60.96502124799));
#150270=CARTESIAN_POINT('Ctrl Pts',(-10.3902588488809,64.76046407779,60.03498149353));
#150271=CARTESIAN_POINT('Ctrl Pts',(-9.75033914805191,63.33933556912,58.1921248627));
#150272=CARTESIAN_POINT('Ctrl Pts',(-14.1114447652659,67.99712344605,59.72095409226));
#150273=CARTESIAN_POINT('Ctrl Pts',(-11.8630597324037,67.63436557765,59.99674441583));
#150274=CARTESIAN_POINT('Ctrl Pts',(-10.0167553446379,66.69384340644,59.01200819548));
#150275=CARTESIAN_POINT('Ctrl Pts',(-9.30390833655991,65.54803587831,57.15665909541));
#150276=CARTESIAN_POINT('',(-15.5675364833309,63.77502783968,63.039015015514));
#150277=CARTESIAN_POINT('Origin',(-15.5675364831312,60.0333704534644,59.7223902246598));
#150278=CARTESIAN_POINT('',(-13.9923246930869,67.84508927339,59.80529136859));
#150279=CARTESIAN_POINT('Ctrl Pts',(-13.9923246930881,67.8450893401677,
59.8052914916334));
#150280=CARTESIAN_POINT('Ctrl Pts',(-14.0321520574323,67.7153858292997,
59.8756832798915));
#150281=CARTESIAN_POINT('Ctrl Pts',(-14.0742956175811,67.5816710739956,
59.9507139079171));
#150282=CARTESIAN_POINT('Ctrl Pts',(-14.11877878484,67.4442748492075,60.0308072755673));
#150283=CARTESIAN_POINT('Ctrl Pts',(-14.161844373002,67.3112571349494,60.108348246642));
#150284=CARTESIAN_POINT('Ctrl Pts',(-14.2071031672786,67.1747888454886,
60.190634689278));
#150285=CARTESIAN_POINT('Ctrl Pts',(-14.2545486384612,67.0352046600873,
60.2780692905195));
#150286=CARTESIAN_POINT('Ctrl Pts',(-14.2797769640136,66.9609831341231,
60.3245611585456));
#150287=CARTESIAN_POINT('Ctrl Pts',(-14.3056230459681,66.8858812263002,
60.3725089025942));
#150288=CARTESIAN_POINT('Ctrl Pts',(-14.3320820314631,66.8099535694013,
60.421974853236));
#150289=CARTESIAN_POINT('Ctrl Pts',(-14.3803584923795,66.6714176999353,
60.5122292975455));
#150290=CARTESIAN_POINT('Ctrl Pts',(-14.4306882769546,66.5301340787245,
60.6075354406058));
#150291=CARTESIAN_POINT('Ctrl Pts',(-14.4830772813101,66.3864780506606,
60.7082683981477));
#150292=CARTESIAN_POINT('Ctrl Pts',(-14.4999323047482,66.3402598460997,
60.7406770377325));
#150293=CARTESIAN_POINT('Ctrl Pts',(-14.5170002006767,66.2937963570198,
60.7736474591747));
#150294=CARTESIAN_POINT('Ctrl Pts',(-14.5342803448823,66.2471008957992,
60.8071923009608));
#150295=CARTESIAN_POINT('Ctrl Pts',(-14.5697756021284,66.1511834434602,
60.8760969798981));
#150296=CARTESIAN_POINT('Ctrl Pts',(-14.6061686288561,66.0542871503293,
60.9474250351948));
#150297=CARTESIAN_POINT('Ctrl Pts',(-14.6434594244527,65.956535330544,61.0212846501146));
#150298=CARTESIAN_POINT('Ctrl Pts',(-14.6621048222509,65.9076594206514,
61.0582144575746));
#150299=CARTESIAN_POINT('Ctrl Pts',(-14.6809746622664,65.8585696766716,
61.095777214623));
#150300=CARTESIAN_POINT('Ctrl Pts',(-14.7000689443167,65.8092824831939,
61.1339862575457));
#150301=CARTESIAN_POINT('Ctrl Pts',(-14.7096160853419,65.784638886455,61.1530907790071));
#150302=CARTESIAN_POINT('Ctrl Pts',(-14.7192193368761,65.759945929971,61.1723568753724));
#150303=CARTESIAN_POINT('Ctrl Pts',(-14.7288786988963,65.735205700205,61.191786216759));
#150304=CARTESIAN_POINT('Ctrl Pts',(-14.7337083799064,65.7228355853219,
61.2015008874524));
#150305=CARTESIAN_POINT('Ctrl Pts',(-14.738552088538,65.7104536522903,61.211256369612));
#150306=CARTESIAN_POINT('Ctrl Pts',(-14.7434098247882,65.6980601653776,
61.22105287134));
#150307=CARTESIAN_POINT('Ctrl Pts',(-14.7470531269758,65.6887650501931,
61.228400247636));
#150308=CARTESIAN_POINT('Ctrl Pts',(-14.7507043196989,65.6794634359645,
61.2357706974564));
#150309=CARTESIAN_POINT('Ctrl Pts',(-14.7543634029561,65.6701554349684,
61.2431643084709));
#150310=CARTESIAN_POINT('Ctrl Pts',(-14.7555830973751,65.6670527679697,
61.2456288454757));
#150311=CARTESIAN_POINT('Ctrl Pts',(-14.7573321603146,65.6626063279641,
61.2491645315469));
#150312=CARTESIAN_POINT('Ctrl Pts',(-14.7580251163913,65.6608453092675,
61.2505656431045));
#150313=CARTESIAN_POINT('Ctrl Pts',(-14.7768289843091,65.6130587841394,
61.2885858258435));
#150314=CARTESIAN_POINT('Ctrl Pts',(-14.797711821438,65.5603698583314,61.330978651077));
#150315=CARTESIAN_POINT('Ctrl Pts',(-14.8206778684102,65.5029514681166,
61.3779472113108));
#150316=CARTESIAN_POINT('Ctrl Pts',(-14.8435571314035,65.445750050216,61.4247382869935));
#150317=CARTESIAN_POINT('Ctrl Pts',(-14.8685041894234,65.3838547534065,
61.4760707197307));
#150318=CARTESIAN_POINT('Ctrl Pts',(-14.8955171319156,65.3174744488824,
61.5321798820439));
#150319=CARTESIAN_POINT('Ctrl Pts',(-14.905340852726,65.2933341102596,61.5525849432709));
#150320=CARTESIAN_POINT('Ctrl Pts',(-14.9154377134962,65.268600982511,61.5736220664484));
#150321=CARTESIAN_POINT('Ctrl Pts',(-14.9258072946201,65.2432864000251,
61.5953036541628));
#150322=CARTESIAN_POINT('Ctrl Pts',(-14.9596821651009,65.1605898867583,
61.6661320672748));
#150323=CARTESIAN_POINT('Ctrl Pts',(-14.9966038285022,65.0713415229218,
61.744131678552));
#150324=CARTESIAN_POINT('Ctrl Pts',(-15.03637930123,64.9765154645022,61.8293260428297));
#150325=CARTESIAN_POINT('Ctrl Pts',(-15.0758681069583,64.8823728298055,
61.9139064002556));
#150326=CARTESIAN_POINT('Ctrl Pts',(-15.1181703187741,64.7827335245751,
62.0055795972903));
#150327=CARTESIAN_POINT('Ctrl Pts',(-15.1630587148956,64.6785840780694,
62.104371243476));
#150328=CARTESIAN_POINT('Ctrl Pts',(-15.2004689345102,64.5917853950428,
62.1867047082292));
#150329=CARTESIAN_POINT('Ctrl Pts',(-15.2359488874782,64.5104427706175,
62.2658310693622));
#150330=CARTESIAN_POINT('Ctrl Pts',(-15.269470099101,64.4342772954221,62.3414348811389));
#150331=CARTESIAN_POINT('Ctrl Pts',(-15.3035998098307,64.3567292143662,
62.4184111030919));
#150332=CARTESIAN_POINT('Ctrl Pts',(-15.3356993668365,64.2845477185496,
62.4917357694123));
#150333=CARTESIAN_POINT('Ctrl Pts',(-15.3657584993669,64.2174647565579,
62.561118959892));
#150334=CARTESIAN_POINT('Ctrl Pts',(-15.3960271377004,64.1499142404939,
62.6309857365507));
#150335=CARTESIAN_POINT('Ctrl Pts',(-15.4242271702903,64.0875334031512,
62.6968560124063));
#150336=CARTESIAN_POINT('Ctrl Pts',(-15.4503625601862,64.0300779903869,
62.7584757252218));
#150337=CARTESIAN_POINT('Ctrl Pts',(-15.4766688062985,63.9722469714244,
62.8204982677264));
#150338=CARTESIAN_POINT('Ctrl Pts',(-15.5008836555906,63.919405824393,62.8782145871554));
#150339=CARTESIAN_POINT('Ctrl Pts',(-15.523020519425,63.8713377355141,62.9314064107263));
#150340=CARTESIAN_POINT('Ctrl Pts',(-15.5389300947263,63.8367916098601,
62.969634920819));
#150341=CARTESIAN_POINT('Ctrl Pts',(-15.5537665555699,63.8047115232912,
63.0055273040344));
#150342=CARTESIAN_POINT('Ctrl Pts',(-15.5675364833309,63.7750278396776,
63.0390150155119));
#150343=CARTESIAN_POINT('Origin',(-13.9922817630625,65.460108937173,55.4107643867529));
#150344=CARTESIAN_POINT('Ctrl Pts',(-14.2053627384189,67.74544063191,59.85616341864));
#150345=CARTESIAN_POINT('Ctrl Pts',(-13.6866847824139,67.6633717185,59.92373292205));
#150346=CARTESIAN_POINT('Ctrl Pts',(-12.6383817091281,67.41710017746,59.91553905833));
#150347=CARTESIAN_POINT('Ctrl Pts',(-11.1637780911519,66.80360758364,59.42315761485));
#150348=CARTESIAN_POINT('Ctrl Pts',(-9.99316319052591,66.02973850092,58.51581872871));
#150349=CARTESIAN_POINT('Ctrl Pts',(-9.52143302578291,65.47873222039,57.71959030244));
#150350=CARTESIAN_POINT('Ctrl Pts',(-9.36367665720291,65.20602642706,57.29408547032));
#150351=CARTESIAN_POINT('Ctrl Pts',(-14.0202046372339,68.33201427489,59.53231650414));
#150352=CARTESIAN_POINT('Ctrl Pts',(-13.5161419891374,68.2470102229,59.59488219199));
#150353=CARTESIAN_POINT('Ctrl Pts',(-12.5016391850898,68.0065002871,59.58065052529));
#150354=CARTESIAN_POINT('Ctrl Pts',(-11.0704533736519,67.43981681245,59.10069440811));
#150355=CARTESIAN_POINT('Ctrl Pts',(-9.91290994946691,66.7392443083,58.22296820509));
#150356=CARTESIAN_POINT('Ctrl Pts',(-9.42170896486791,66.24201106279,57.44738812635));
#150357=CARTESIAN_POINT('Ctrl Pts',(-9.24823875588991,65.99481676477,57.0294496165));
#150358=CARTESIAN_POINT('Ctrl Pts',(-13.6549069241899,69.49993804976,58.98674389696));
#150359=CARTESIAN_POINT('Ctrl Pts',(-13.1769404748612,69.41646103563,59.03665035664));
#150360=CARTESIAN_POINT('Ctrl Pts',(-12.2218902458356,69.19905724735,59.00590868675));
#150361=CARTESIAN_POINT('Ctrl Pts',(-10.8679330720989,68.72846005566,58.54326883772));
#150362=CARTESIAN_POINT('Ctrl Pts',(-9.73897835675691,68.16508642168,57.71819138305));
#150363=CARTESIAN_POINT('Ctrl Pts',(-9.21997508227291,67.76716754432,56.98439768797));
#150364=CARTESIAN_POINT('Ctrl Pts',(-9.02174978537091,67.56775735817,56.58383055835));
#150365=CARTESIAN_POINT('Ctrl Pts',(-13.0264541098147,71.89096840686,58.22143278291));
#150366=CARTESIAN_POINT('Ctrl Pts',(-12.5887620025556,71.83103234225,58.24468551411));
#150367=CARTESIAN_POINT('Ctrl Pts',(-11.7230981427679,71.6906865179,58.17830836715));
#150368=CARTESIAN_POINT('Ctrl Pts',(-10.4863172342819,71.42179955806,57.73325733767));
#150369=CARTESIAN_POINT('Ctrl Pts',(-9.41080141879591,71.11627944215,56.98713738773));
#150370=CARTESIAN_POINT('Ctrl Pts',(-8.86349672505391,70.90290608307,56.32569316036));
#150371=CARTESIAN_POINT('Ctrl Pts',(-8.63464566339991,70.79475115391,55.9591981337));
#150372=CARTESIAN_POINT('Ctrl Pts',(-12.7037393234953,74.39162227679,57.90748319535));
#150373=CARTESIAN_POINT('Ctrl Pts',(-12.28393586553,74.38000747547,57.91587997198));
#150374=CARTESIAN_POINT('Ctrl Pts',(-11.4571120723499,74.35278927765,57.82979946692));
#150375=CARTESIAN_POINT('Ctrl Pts',(-10.2725544129929,74.30035033484,57.38928272527));
#150376=CARTESIAN_POINT('Ctrl Pts',(-9.22672717125391,74.2404602146,56.67735146262));
#150377=CARTESIAN_POINT('Ctrl Pts',(-8.67519748870391,74.19845211679,56.05133853923));
#150378=CARTESIAN_POINT('Ctrl Pts',(-8.43723858833691,74.17711457634,55.70323479651));
#150379=CARTESIAN_POINT('Ctrl Pts',(-12.8671141721126,76.88190734633,58.06713723927));
#150380=CARTESIAN_POINT('Ctrl Pts',(-12.4383232178018,76.91798866819,58.08327470442));
#150381=CARTESIAN_POINT('Ctrl Pts',(-11.5918425291884,77.0025099707,58.00755176421));
#150382=CARTESIAN_POINT('Ctrl Pts',(-10.3806961735749,77.16495510187,57.56487994748));
#150383=CARTESIAN_POINT('Ctrl Pts',(-9.31980220568091,77.35007308731,56.83532487627));
#150384=CARTESIAN_POINT('Ctrl Pts',(-8.77051022514491,77.47967802037,56.19100248932));
#150385=CARTESIAN_POINT('Ctrl Pts',(-8.53719879336791,77.5454508045,55.83340513874));
#150386=CARTESIAN_POINT('Ctrl Pts',(-13.3015354916722,79.37972298075,58.54120535384));
#150387=CARTESIAN_POINT('Ctrl Pts',(-12.846655159085,79.4564624083,58.57621796265));
#150388=CARTESIAN_POINT('Ctrl Pts',(-11.9431325981701,79.64368966687,58.52545042363));
#150389=CARTESIAN_POINT('Ctrl Pts',(-10.6566364727739,80.02083519139,58.07343649006));
#150390=CARTESIAN_POINT('Ctrl Pts',(-9.55738924270991,80.45907194911,57.29417007324));
#150391=CARTESIAN_POINT('Ctrl Pts',(-9.02052118745391,80.76657499756,56.60163811033));
#150392=CARTESIAN_POINT('Ctrl Pts',(-8.80382301199991,80.92163216041,56.22016816974));
#150393=CARTESIAN_POINT('Ctrl Pts',(-13.8489227042999,81.12444072467,59.23274232687));
#150394=CARTESIAN_POINT('Ctrl Pts',(-13.3583894249944,81.21204418286,59.29065555428));
#150395=CARTESIAN_POINT('Ctrl Pts',(-12.375145516444,81.44698775439,59.2707797108));
#150396=CARTESIAN_POINT('Ctrl Pts',(-10.9840720246189,81.97008585063,58.80223087688));
#150397=CARTESIAN_POINT('Ctrl Pts',(-9.83859395161891,82.60268348927,57.95185518517));
#150398=CARTESIAN_POINT('Ctrl Pts',(-9.32938702249691,83.05012179098,57.19539776513));
#150399=CARTESIAN_POINT('Ctrl Pts',(-9.14138216248191,83.27370133808,56.78447782593));
#150400=CARTESIAN_POINT('Ctrl Pts',(-14.2054072809149,82.2547530918,59.85623901085));
#150401=CARTESIAN_POINT('Ctrl Pts',(-13.6867239510549,82.33683162598,59.92381322088));
#150402=CARTESIAN_POINT('Ctrl Pts',(-12.6384126884581,82.58312529384,59.91562799188));
#150403=CARTESIAN_POINT('Ctrl Pts',(-11.1638044367469,83.19665457774,59.42325346353));
#150404=CARTESIAN_POINT('Ctrl Pts',(-9.99319080751591,83.9705583545,58.51591282125));
#150405=CARTESIAN_POINT('Ctrl Pts',(-9.52146541439991,84.52158459866,57.71967705271));
#150406=CARTESIAN_POINT('Ctrl Pts',(-9.36371259686991,84.79429945203,57.29416759219));
#150407=CARTESIAN_POINT('',(-13.9922553804019,82.154923079361,59.8052980196173));
#150408=CARTESIAN_POINT('Ctrl Pts',(-13.9923246930992,67.845089141546,59.8052911256481));
#150409=CARTESIAN_POINT('Ctrl Pts',(-13.8764053209202,68.222754190633,59.600327407802));
#150410=CARTESIAN_POINT('Ctrl Pts',(-13.7595941039321,68.6088595757193,
59.4119043223723));
#150411=CARTESIAN_POINT('Ctrl Pts',(-13.6461287860564,69.0017537124996,
59.2404767610183));
#150412=CARTESIAN_POINT('Ctrl Pts',(-13.5955968106831,69.1767297951989,
59.1641312003585));
#150413=CARTESIAN_POINT('Ctrl Pts',(-13.5457287368772,69.353051674383,59.0911566578527));
#150414=CARTESIAN_POINT('Ctrl Pts',(-13.4969004303597,69.530570634749,59.0215935397647));
#150415=CARTESIAN_POINT('Ctrl Pts',(-13.4891180900841,69.5588639148863,
59.0105064492183));
#150416=CARTESIAN_POINT('Ctrl Pts',(-13.4813621647634,69.5871876009258,
58.9995060170303));
#150417=CARTESIAN_POINT('Ctrl Pts',(-13.4736342771579,69.6155418053939,
58.988592346489));
#150418=CARTESIAN_POINT('Ctrl Pts',(-13.3910906412204,69.9184006525175,
58.8720205103174));
#150419=CARTESIAN_POINT('Ctrl Pts',(-13.3117448569473,70.2247423571956,
58.7653478165224));
#150420=CARTESIAN_POINT('Ctrl Pts',(-13.2375806890668,70.5346970220213,
58.6686969596893));
#150421=CARTESIAN_POINT('Ctrl Pts',(-13.2004986051266,70.6896743544342,
58.6203715312727));
#150422=CARTESIAN_POINT('Ctrl Pts',(-13.1647119249811,70.845554882444,58.574551414006));
#150423=CARTESIAN_POINT('Ctrl Pts',(-13.1304700379036,71.0023536068965,
58.5312511228961));
#150424=CARTESIAN_POINT('Ctrl Pts',(-13.1133490943649,71.0807529691228,
58.5096009773411));
#150425=CARTESIAN_POINT('Ctrl Pts',(-13.0966143490678,71.1593818761839,
58.4885807747841));
#150426=CARTESIAN_POINT('Ctrl Pts',(-13.0802970349962,71.238242167762,58.468192245751));
#150427=CARTESIAN_POINT('Ctrl Pts',(-13.0761874678052,71.2581033817783,
58.463057330187));
#150428=CARTESIAN_POINT('Ctrl Pts',(-13.0721043779997,71.2779792726429,
58.4579624813378));
#150429=CARTESIAN_POINT('Ctrl Pts',(-13.0680482612216,71.2978698640127,
58.4529077276355));
#150430=CARTESIAN_POINT('Ctrl Pts',(-13.0640518352011,71.3174677408151,
58.447927360864));
#150431=CARTESIAN_POINT('Ctrl Pts',(-13.0600815941699,71.3370798886255,
58.4429859178163));
#150432=CARTESIAN_POINT('Ctrl Pts',(-13.0561378076342,71.3567060405806,
58.4380834580827));
#150433=CARTESIAN_POINT('Ctrl Pts',(-13.0521645688323,71.3764787609788,
58.4331443866948));
#150434=CARTESIAN_POINT('Ctrl Pts',(-13.0482182337819,71.3962657675923,
58.4282448649636));
#150435=CARTESIAN_POINT('Ctrl Pts',(-13.0442990168575,71.416066703405,58.4233849750216));
#150436=CARTESIAN_POINT('Ctrl Pts',(-13.0423394083953,71.4259671713114,
58.4209550300506));
#150437=CARTESIAN_POINT('Ctrl Pts',(-13.0403865794646,71.4358711215037,
58.4185349929911));
#150438=CARTESIAN_POINT('Ctrl Pts',(-13.0384405700485,71.4457785273776,
58.4161248695553));
#150439=CARTESIAN_POINT('Ctrl Pts',(-13.0369810629863,71.453209081783,58.4143172769784));
#150440=CARTESIAN_POINT('Ctrl Pts',(-13.0355253919011,71.4606415800103,
58.4125152608173));
#150441=CARTESIAN_POINT('Ctrl Pts',(-13.0340735715475,71.4680760079362,
58.4107188242038));
#150442=CARTESIAN_POINT('Ctrl Pts',(-13.0335896314296,71.4705541505781,
58.4101200119993));
#150443=CARTESIAN_POINT('Ctrl Pts',(-13.0328644451741,71.4742724707177,
58.4092228702797));
#150444=CARTESIAN_POINT('Ctrl Pts',(-13.0326230353178,71.4755110785719,
58.4089242475553));
#150445=CARTESIAN_POINT('Ctrl Pts',(-13.020068211608,71.5399264404598,58.3933939965603));
#150446=CARTESIAN_POINT('Ctrl Pts',(-13.0065976865036,71.6098663281076,
58.3769827511436));
#150447=CARTESIAN_POINT('Ctrl Pts',(-12.9923806682185,71.6853980043269,
58.3599205519703));
#150448=CARTESIAN_POINT('Ctrl Pts',(-12.9777555181637,71.7630979887009,
58.3423685436538));
#150449=CARTESIAN_POINT('Ctrl Pts',(-12.9623398663465,71.8467157264396,
58.3241273966127));
#150450=CARTESIAN_POINT('Ctrl Pts',(-12.9463600462848,71.9363247088156,
58.305489391384));
#150451=CARTESIAN_POINT('Ctrl Pts',(-12.9315695383823,72.0192644638849,
58.2882385360829));
#150452=CARTESIAN_POINT('Ctrl Pts',(-12.916295901173,72.1073370761852,58.2706480711374));
#150453=CARTESIAN_POINT('Ctrl Pts',(-12.9007553997249,72.2005972023878,
58.2529831546617));
#150454=CARTESIAN_POINT('Ctrl Pts',(-12.8855314091007,72.2919579150175,
58.2356780166196));
#150455=CARTESIAN_POINT('Ctrl Pts',(-12.8700511587873,72.3882972254665,
58.2183014660757));
#150456=CARTESIAN_POINT('Ctrl Pts',(-12.8545549842605,72.4896595017306,
58.2011336654313));
#150457=CARTESIAN_POINT('Ctrl Pts',(-12.8393842716389,72.5888928938953,
58.1843264353971));
#150458=CARTESIAN_POINT('Ctrl Pts',(-12.8241981519655,72.6929407026516,
58.1677193130647));
#150459=CARTESIAN_POINT('Ctrl Pts',(-12.8092601655493,72.8018343625555,
58.1516045504453));
#150460=CARTESIAN_POINT('Ctrl Pts',(-12.7946393343453,72.908416051431,58.1358319277111));
#150461=CARTESIAN_POINT('Ctrl Pts',(-12.7802560776962,73.0196402207419,
58.1205310099541));
#150462=CARTESIAN_POINT('Ctrl Pts',(-12.7663963618552,73.1355232537047,
58.1060037940822));
#150463=CARTESIAN_POINT('Ctrl Pts',(-12.7527924392277,73.2492675636421,
58.0917446907225));
#150464=CARTESIAN_POINT('Ctrl Pts',(-12.739692767209,73.3675005670556,58.0782310075463));
#150465=CARTESIAN_POINT('Ctrl Pts',(-12.7274076725007,73.4902218979716,
58.0657752633181));
#150466=CARTESIAN_POINT('Ctrl Pts',(-12.7155212960257,73.608960253306,58.0537237758296));
#150467=CARTESIAN_POINT('Ctrl Pts',(-12.7043974476233,73.7319004693616,
58.0426627407316));
#150468=CARTESIAN_POINT('Ctrl Pts',(-12.6943560349518,73.8590247110285,
58.0328999656886));
#150469=CARTESIAN_POINT('Ctrl Pts',(-12.6844879572467,73.983954532757,58.0233057157666));
#150470=CARTESIAN_POINT('Ctrl Pts',(-12.6756651456058,74.112925356913,58.0149652954682));
#150471=CARTESIAN_POINT('Ctrl Pts',(-12.668230626856,74.2459006240721,58.0081946926255));
#150472=CARTESIAN_POINT('Ctrl Pts',(-12.6609684625286,74.375793126074,58.001581052645));
#150473=CARTESIAN_POINT('Ctrl Pts',(-12.6550308974448,74.5095066982876,
57.9964653132249));
#150474=CARTESIAN_POINT('Ctrl Pts',(-12.650776916749,74.6469860318338,57.9931646922056));
#150475=CARTESIAN_POINT('Ctrl Pts',(-12.6500770189875,74.6696051936677,
57.9926216485418));
#150476=CARTESIAN_POINT('Ctrl Pts',(-12.6494227842728,74.6923262418515,
57.9921277894647));
#150477=CARTESIAN_POINT('Ctrl Pts',(-12.6488159185513,74.7151488689863,
57.9916845878056));
#150478=CARTESIAN_POINT('Ctrl Pts',(-12.6474232167211,74.7675247298372,
57.9906674801653));
#150479=CARTESIAN_POINT('Ctrl Pts',(-12.6462799292503,74.8204356026201,
57.9899171327293));
#150480=CARTESIAN_POINT('Ctrl Pts',(-12.6454073095588,74.8738773989734,
57.9894516915659));
#150481=CARTESIAN_POINT('Ctrl Pts',(-12.644970999713,74.9005982971501,57.9892189709842));
#150482=CARTESIAN_POINT('Ctrl Pts',(-12.6446023568134,74.9274519262714,
57.989057484451));
#150483=CARTESIAN_POINT('Ctrl Pts',(-12.6443041376423,74.9544377155396,
57.9889695458577));
#150484=CARTESIAN_POINT('Ctrl Pts',(-12.6441550280568,74.9679306101737,
57.988925576561));
#150485=CARTESIAN_POINT('Ctrl Pts',(-12.6440235244035,74.9814565448504,
57.9888999947202));
#150486=CARTESIAN_POINT('Ctrl Pts',(-12.6439099743136,74.9950154463947,
57.9888930924319));
#150487=CARTESIAN_POINT('Ctrl Pts',(-12.6438586624004,75.0011425501131,
57.9888899733713));
#150488=CARTESIAN_POINT('Ctrl Pts',(-12.6438110165207,75.0072763857763,
57.9888906687515));
#150489=CARTESIAN_POINT('Ctrl Pts',(-12.6437670689792,75.0134169464862,
57.9888952056554));
#150490=CARTESIAN_POINT('Ctrl Pts',(-12.6437623899252,75.0140707262935,
57.9888956886953));
#150491=CARTESIAN_POINT('Ctrl Pts',(-12.6437577527944,75.0147245823336,
57.9888962152816));
#150492=CARTESIAN_POINT('Ctrl Pts',(-12.6437531576084,75.0153785146011,
57.9888967854433));
#150493=CARTESIAN_POINT('Ctrl Pts',(-12.6437292801054,75.0187764770737,
57.9888997481171));
#150494=CARTESIAN_POINT('Ctrl Pts',(-12.6437065355144,75.0221764976604,
57.9889038873487));
#150495=CARTESIAN_POINT('Ctrl Pts',(-12.6436849263525,75.025578575702,57.988909207229));
#150496=CARTESIAN_POINT('Ctrl Pts',(-12.6436741217715,75.0272796147229,
57.9889118671691));
#150497=CARTESIAN_POINT('Ctrl Pts',(-12.6436636010478,75.0289811681074,
57.9889148222715));
#150498=CARTESIAN_POINT('Ctrl Pts',(-12.6436533645941,75.0306832357554,
57.9889180730479));
#150499=CARTESIAN_POINT('Ctrl Pts',(-12.6436431281404,75.0323853034035,
57.9889213238242));
#150500=CARTESIAN_POINT('Ctrl Pts',(-12.6436266975926,75.0352291559008,
57.9889274452835));
#150501=CARTESIAN_POINT('Ctrl Pts',(-12.643623508419,75.0357909813961,57.9889287129107));
#150502=CARTESIAN_POINT('Ctrl Pts',(-12.6423924799616,75.2526569306915,
57.9894180199751));
#150503=CARTESIAN_POINT('Ctrl Pts',(-12.646472241189,75.4727189162619,57.9946990468044));
#150504=CARTESIAN_POINT('Ctrl Pts',(-12.6559493082686,75.6957106878421,
58.0051451751774));
#150505=CARTESIAN_POINT('Ctrl Pts',(-12.6590427828385,75.7684989638847,
58.0085549677011));
#150506=CARTESIAN_POINT('Ctrl Pts',(-12.6627110643347,75.8415990966006,
58.0125150142212));
#150507=CARTESIAN_POINT('Ctrl Pts',(-12.6669563732953,75.9150009409436,
58.017038073061));
#150508=CARTESIAN_POINT('Ctrl Pts',(-12.6755819223178,76.0641376027508,
58.0262279497264));
#150509=CARTESIAN_POINT('Ctrl Pts',(-12.6865899759768,76.2145202297719,
58.0377421482989));
#150510=CARTESIAN_POINT('Ctrl Pts',(-12.6999939404488,76.3660582763293,
58.0516862103691));
#150511=CARTESIAN_POINT('Ctrl Pts',(-12.7016694360078,76.385000532149,58.0534292181278));
#150512=CARTESIAN_POINT('Ctrl Pts',(-12.7033823676737,76.4039608415549,
58.0552101908413));
#150513=CARTESIAN_POINT('Ctrl Pts',(-12.7051327395416,76.4229390052955,
58.0570293311126));
#150514=CARTESIAN_POINT('Ctrl Pts',(-12.7060079254756,76.4324280871659,
58.0579389012482));
#150515=CARTESIAN_POINT('Ctrl Pts',(-12.70689247146,76.4419216326199,58.0588580132628));
#150516=CARTESIAN_POINT('Ctrl Pts',(-12.7077863808547,76.451419619682,58.0597866927244));
#150517=CARTESIAN_POINT('Ctrl Pts',(-12.7083434952166,76.4573390842646,
58.06036547696));
#150518=CARTESIAN_POINT('Ctrl Pts',(-12.7094999601304,76.4695729187318,
58.061566640817));
#150519=CARTESIAN_POINT('Ctrl Pts',(-12.7107956449714,76.4830585732496,
58.0629140215282));
#150520=CARTESIAN_POINT('Ctrl Pts',(-12.7115789315787,76.4912111210295,
58.0637285600892));
#150521=CARTESIAN_POINT('Ctrl Pts',(-12.7124127687965,76.4998212018493,
58.0645961631595));
#150522=CARTESIAN_POINT('Ctrl Pts',(-12.7131886154,76.5077712459183,58.0654037342866));
#150523=CARTESIAN_POINT('Ctrl Pts',(-12.7256079849799,76.635031628357,58.0783309343856));
#150524=CARTESIAN_POINT('Ctrl Pts',(-12.7394903374166,76.762090043741,58.0928780348764));
#150525=CARTESIAN_POINT('Ctrl Pts',(-12.7547724123643,76.8889053499444,
58.1090308435864));
#150526=CARTESIAN_POINT('Ctrl Pts',(-12.8005432353644,77.2687255611255,
58.157409571668));
#150527=CARTESIAN_POINT('Ctrl Pts',(-12.8588680406673,77.6463622141542,
58.2201931928097));
#150528=CARTESIAN_POINT('Ctrl Pts',(-12.9276269170201,78.0194570007294,
58.2966226822194));
#150529=CARTESIAN_POINT('Ctrl Pts',(-12.9713073131002,78.256472625729,58.345175982487));
#150530=CARTESIAN_POINT('Ctrl Pts',(-13.0191991737726,78.4916559317739,
58.3992359932875));
#150531=CARTESIAN_POINT('Ctrl Pts',(-13.0707644468211,78.7244116924096,
58.4586057913303));
#150532=CARTESIAN_POINT('Ctrl Pts',(-13.0726976055923,78.7331376006344,
58.4608315382147));
#150533=CARTESIAN_POINT('Ctrl Pts',(-13.0746359276518,78.7418600980509,
58.4630647476694));
#150534=CARTESIAN_POINT('Ctrl Pts',(-13.0765793757085,78.7505791898991,
58.4653054193184));
#150535=CARTESIAN_POINT('Ctrl Pts',(-13.0824690905492,78.7770028262172,
58.4720958848612));
#150536=CARTESIAN_POINT('Ctrl Pts',(-13.0885638230363,78.804051607521,58.4791276116934));
#150537=CARTESIAN_POINT('Ctrl Pts',(-13.0943656728559,78.8296253292383,
58.4858479439898));
#150538=CARTESIAN_POINT('Ctrl Pts',(-13.0974641280112,78.843282875083,58.4894369111118));
#150539=CARTESIAN_POINT('Ctrl Pts',(-13.1004785548092,78.8565200748843,
58.4929362952549));
#150540=CARTESIAN_POINT('Ctrl Pts',(-13.1033301382347,78.8690191762275,
58.4962571599057));
#150541=CARTESIAN_POINT('Ctrl Pts',(-13.1176059329182,78.9315930441025,
58.5128823028004));
#150542=CARTESIAN_POINT('Ctrl Pts',(-13.1333784860537,79.0003742996488,
58.5315864013316));
#150543=CARTESIAN_POINT('Ctrl Pts',(-13.1507809817894,79.0752552081944,
58.5526325802277));
#150544=CARTESIAN_POINT('Ctrl Pts',(-13.1688970697479,79.1532066208097,
58.5745417611787));
#150545=CARTESIAN_POINT('Ctrl Pts',(-13.1887803485302,79.2377682099706,
58.598988647045));
#150546=CARTESIAN_POINT('Ctrl Pts',(-13.2105817144596,79.3287995706086,
58.6263267340569));
#150547=CARTESIAN_POINT('Ctrl Pts',(-13.2311438855714,79.4146566870867,
58.6521109177099));
#150548=CARTESIAN_POINT('Ctrl Pts',(-13.2534130326781,79.5062687568842,
58.6804674325358));
#150549=CARTESIAN_POINT('Ctrl Pts',(-13.2775048113542,79.6035035139611,
58.7117401692531));
#150550=CARTESIAN_POINT('Ctrl Pts',(-13.3010877576402,79.6986846163658,
58.7423524075662));
#150551=CARTESIAN_POINT('Ctrl Pts',(-13.3264179061768,79.7992532799048,
58.7757591299201));
#150552=CARTESIAN_POINT('Ctrl Pts',(-13.3535821396951,79.9050736102897,
58.8123256644255));
#150553=CARTESIAN_POINT('Ctrl Pts',(-13.3797112477034,80.0068615308008,
58.8474987875301));
#150554=CARTESIAN_POINT('Ctrl Pts',(-13.4075379089805,80.1135083661954,
58.885595736518));
#150555=CARTESIAN_POINT('Ctrl Pts',(-13.4371097621925,80.2248840390139,
58.9269786555841));
#150556=CARTESIAN_POINT('Ctrl Pts',(-13.4452861746218,80.2556786405231,
58.9384207458511));
#150557=CARTESIAN_POINT('Ctrl Pts',(-13.4535957952361,80.2868347050863,
58.9501142568969));
#150558=CARTESIAN_POINT('Ctrl Pts',(-13.4620391156216,80.3183493740482,
58.9620673331119));
#150559=CARTESIAN_POINT('Ctrl Pts',(-13.4667773879387,80.3360349617922,
58.9687752308997));
#150560=CARTESIAN_POINT('Ctrl Pts',(-13.4715577618766,80.353833483865,58.9755648772567));
#150561=CARTESIAN_POINT('Ctrl Pts',(-13.4763802888604,80.3717444289602,
58.982437740821));
#150562=CARTESIAN_POINT('Ctrl Pts',(-13.4787915523522,80.3806999015078,
58.9858741726032));
#150563=CARTESIAN_POINT('Ctrl Pts',(-13.4812133541063,80.3896834796924,
58.989331408995));
#150564=CARTESIAN_POINT('Ctrl Pts',(-13.4836456974466,80.3986950992758,
58.9928096355766));
#150565=CARTESIAN_POINT('Ctrl Pts',(-13.4859012795059,80.4070518337555,
58.9960350952993));
#150566=CARTESIAN_POINT('Ctrl Pts',(-13.4893480347745,80.4198068304272,
59.0009709141936));
#150567=CARTESIAN_POINT('Ctrl Pts',(-13.4925521254936,80.431636877691,59.005569537271));
#150568=CARTESIAN_POINT('Ctrl Pts',(-13.492803217746,80.4325639529437,59.0059299136547));
#150569=CARTESIAN_POINT('Ctrl Pts',(-13.493052812368,80.4334853576126,59.0062881937997));
#150570=CARTESIAN_POINT('Ctrl Pts',(-13.4933002154167,80.4343985350018,
59.0066433787663));
#150571=CARTESIAN_POINT('Ctrl Pts',(-13.5069178845044,80.484662052657,59.0261936283159));
#150572=CARTESIAN_POINT('Ctrl Pts',(-13.520340769541,80.5338016263157,59.0456237116997));
#150573=CARTESIAN_POINT('Ctrl Pts',(-13.5335512771401,80.5818307901296,
59.0649008674955));
#150574=CARTESIAN_POINT('Ctrl Pts',(-13.5599722923383,80.6778891177573,
59.103455179087));
#150575=CARTESIAN_POINT('Ctrl Pts',(-13.5855437948394,80.7695063631374,
59.1413963752888));
#150576=CARTESIAN_POINT('Ctrl Pts',(-13.6101573960222,80.856781532072,59.1784781913009));
#150577=CARTESIAN_POINT('Ctrl Pts',(-13.6375278400217,80.9538319435956,
59.2197133507162));
#150578=CARTESIAN_POINT('Ctrl Pts',(-13.663713636453,81.0455133404965,59.2598853045842));
#150579=CARTESIAN_POINT('Ctrl Pts',(-13.6886091519591,81.1319457165426,
59.2986865949162));
#150580=CARTESIAN_POINT('Ctrl Pts',(-13.7140937239498,81.2204231818573,
59.3384059683335));
#150581=CARTESIAN_POINT('Ctrl Pts',(-13.7382267359038,81.3034002811428,
59.3766888998109));
#150582=CARTESIAN_POINT('Ctrl Pts',(-13.7609340348152,81.3809885064921,
59.4132413988346));
#150583=CARTESIAN_POINT('Ctrl Pts',(-13.7843489556299,81.4609945943934,
59.4509329742862));
#150584=CARTESIAN_POINT('Ctrl Pts',(-13.8062484160857,81.5352707244551,
59.4867843747173));
#150585=CARTESIAN_POINT('Ctrl Pts',(-13.8265845754031,81.603920991272,59.5205137510087));
#150586=CARTESIAN_POINT('Ctrl Pts',(-13.8365619933325,81.6376024938756,
59.5370622092749));
#150587=CARTESIAN_POINT('Ctrl Pts',(-13.8461635582274,81.6699295083559,
59.5531004969978));
#150588=CARTESIAN_POINT('Ctrl Pts',(-13.8553858825759,81.7009127913618,
59.5685989547995));
#150589=CARTESIAN_POINT('Ctrl Pts',(-13.8747444750509,81.7659498391365,
59.601131786788));
#150590=CARTESIAN_POINT('Ctrl Pts',(-13.8924309395384,81.825067279728,59.6312830136446));
#150591=CARTESIAN_POINT('Ctrl Pts',(-13.9084295099037,81.8783507762487,
59.6588125803306));
#150592=CARTESIAN_POINT('Ctrl Pts',(-13.9245519021174,81.9320466634317,
59.6865552136691));
#150593=CARTESIAN_POINT('Ctrl Pts',(-13.938960695333,81.9798179133721,59.7116353843609));
#150594=CARTESIAN_POINT('Ctrl Pts',(-13.9516539765085,82.0217338159453,
59.7338551629453));
#150595=CARTESIAN_POINT('Ctrl Pts',(-13.964413516165,82.0638685180553,59.756190927992));
#150596=CARTESIAN_POINT('Ctrl Pts',(-13.9754400180099,82.1000865483256,
59.7756363162688));
#150597=CARTESIAN_POINT('Ctrl Pts',(-13.9847386239781,82.1304403675663,
59.7920391319671));
#150598=CARTESIAN_POINT('Ctrl Pts',(-13.9873839817898,82.1390757171142,
59.7967055644184));
#150599=CARTESIAN_POINT('Ctrl Pts',(-13.989889515855,82.1472363414086,59.8011260517734));
#150600=CARTESIAN_POINT('Ctrl Pts',(-13.9922553804113,82.1549231907861,
59.8052978143008));
#150601=CARTESIAN_POINT('Origin',(-13.9922815033674,84.5398910545472,55.4107645820394));
#150602=CARTESIAN_POINT('Ctrl Pts',(-14.1109587916089,82.00193238136,59.72048255862));
#150603=CARTESIAN_POINT('Ctrl Pts',(-11.8622349709508,82.36472563539,59.9961606353001));
#150604=CARTESIAN_POINT('Ctrl Pts',(-10.0158495894259,83.30534179388,59.0109757487901));
#150605=CARTESIAN_POINT('Ctrl Pts',(-9.30331679897791,84.45114585728,57.15519830438));
#150606=CARTESIAN_POINT('Ctrl Pts',(-14.6029404122129,83.6144608082201,
60.57083234018));
#150607=CARTESIAN_POINT('Ctrl Pts',(-12.2714944067148,84.0386899500301,
60.94839266559));
#150608=CARTESIAN_POINT('Ctrl Pts',(-10.3832434550239,85.20823401609,60.01707148773));
#150609=CARTESIAN_POINT('Ctrl Pts',(-9.74244088945991,86.62498997905,58.17348929348));
#150610=CARTESIAN_POINT('Ctrl Pts',(-15.2156776004539,85.08666325345,61.73072156537));
#150611=CARTESIAN_POINT('Ctrl Pts',(-12.7662414190948,85.49056520221,62.21808717785));
#150612=CARTESIAN_POINT('Ctrl Pts',(-10.8233228752319,86.8784910968501,
61.36245727411));
#150613=CARTESIAN_POINT('Ctrl Pts',(-10.2896898327459,88.6055982400801,
59.56133749227));
#150614=CARTESIAN_POINT('Ctrl Pts',(-15.7859912232689,86.29753560658,63.116600358883));
#150615=CARTESIAN_POINT('Ctrl Pts',(-13.2006081304576,86.61632728226,63.627536549935));
#150616=CARTESIAN_POINT('Ctrl Pts',(-11.2038952684509,88.1916362156301,
62.86693039028));
#150617=CARTESIAN_POINT('Ctrl Pts',(-10.7995805712569,90.23163990772,61.2170704358901));
#150618=CARTESIAN_POINT('',(-15.5675364833309,86.22497216032,63.039015015514));
#150619=CARTESIAN_POINT('Ctrl Pts',(-15.5675364833309,86.2249721603231,
63.0390150155113));
#150620=CARTESIAN_POINT('Ctrl Pts',(-15.5486555635769,86.1843063248925,
62.9931377658538));
#150621=CARTESIAN_POINT('Ctrl Pts',(-15.527678303696,86.1389595646384,62.9425502180199));
#150622=CARTESIAN_POINT('Ctrl Pts',(-15.5045989540046,86.088733552719,62.887439691955));
#150623=CARTESIAN_POINT('Ctrl Pts',(-15.481592586095,86.0386663660651,62.8325034370219));
#150624=CARTESIAN_POINT('Ctrl Pts',(-15.456497073684,85.9837504650751,62.773072604199));
#150625=CARTESIAN_POINT('Ctrl Pts',(-15.4293129408974,85.9237584010294,
62.7093735960576));
#150626=CARTESIAN_POINT('Ctrl Pts',(-15.4195374529417,85.9021850919184,
62.6864672597852));
#150627=CARTESIAN_POINT('Ctrl Pts',(-15.4094919598478,85.8799550919683,
62.6630093844385));
#150628=CARTESIAN_POINT('Ctrl Pts',(-15.3991768168664,85.8570569499555,
62.6390118613801));
#150629=CARTESIAN_POINT('Ctrl Pts',(-15.3671738852249,85.7860150191872,
62.5645590795441));
#150630=CARTESIAN_POINT('Ctrl Pts',(-15.332464150594,85.7082848312241,62.4846395801313));
#150631=CARTESIAN_POINT('Ctrl Pts',(-15.2951936032702,85.6238591391515,
62.4000356000023));
#150632=CARTESIAN_POINT('Ctrl Pts',(-15.2584742717383,85.5406820677203,
62.3166828773205));
#150633=CARTESIAN_POINT('Ctrl Pts',(-15.2192688297427,85.4510049477835,
62.2287837813175));
#150634=CARTESIAN_POINT('Ctrl Pts',(-15.1777504002889,85.3548275184667,
62.1371227619183));
#150635=CARTESIAN_POINT('Ctrl Pts',(-15.1721628635966,85.341883991403,62.124787051828));
#150636=CARTESIAN_POINT('Ctrl Pts',(-15.166533491163,85.3288227570333,62.1123832542891));
#150637=CARTESIAN_POINT('Ctrl Pts',(-15.1608627590391,85.3156438405344,
62.0999133240707));
#150638=CARTESIAN_POINT('Ctrl Pts',(-15.1243771652748,85.2308504517586,
62.0196815659362));
#150639=CARTESIAN_POINT('Ctrl Pts',(-15.0897349273574,85.1493623839876,
61.9444441869956));
#150640=CARTESIAN_POINT('Ctrl Pts',(-15.0569497449735,85.071466224997,61.8739344323386));
#150641=CARTESIAN_POINT('Ctrl Pts',(-15.0233703574083,84.9916830692417,
61.8017166129884));
#150642=CARTESIAN_POINT('Ctrl Pts',(-14.991738766518,84.9156678324434,61.734457940933));
#150643=CARTESIAN_POINT('Ctrl Pts',(-14.9620493845024,84.8436821117079,
61.671892692347));
#150644=CARTESIAN_POINT('Ctrl Pts',(-14.9487644620143,84.8114711104913,
61.6438970110128));
#150645=CARTESIAN_POINT('Ctrl Pts',(-14.9358681789785,84.7800663170307,
61.616841367153));
#150646=CARTESIAN_POINT('Ctrl Pts',(-14.9233590215613,84.7494883724321,
61.5907034983332));
#150647=CARTESIAN_POINT('Ctrl Pts',(-14.8947731715385,84.6796118404519,
61.5309734003674));
#150648=CARTESIAN_POINT('Ctrl Pts',(-14.8682174376492,84.6140570837511,
61.4760349535713));
#150649=CARTESIAN_POINT('Ctrl Pts',(-14.8436927760689,84.5530433545044,
61.4256463383064));
#150650=CARTESIAN_POINT('Ctrl Pts',(-14.8391510492176,84.54174421011,61.4163148608383));
#150651=CARTESIAN_POINT('Ctrl Pts',(-14.8346789493652,84.5306006875076,
61.4071395036283));
#150652=CARTESIAN_POINT('Ctrl Pts',(-14.8302764458863,84.519614025464,61.3981188444365));
#150653=CARTESIAN_POINT('Ctrl Pts',(-14.816188756294,84.4844575093433,61.3692533938533));
#150654=CARTESIAN_POINT('Ctrl Pts',(-14.8028141038372,84.4509075776405,
61.3419717236838));
#150655=CARTESIAN_POINT('Ctrl Pts',(-14.7901524896367,84.419001923336,61.3162299894535));
#150656=CARTESIAN_POINT('Ctrl Pts',(-14.7838216825364,84.4030490961838,
61.3033591223383));
#150657=CARTESIAN_POINT('Ctrl Pts',(-14.7776691350233,84.3875072796161,
61.2908733129297));
#150658=CARTESIAN_POINT('Ctrl Pts',(-14.7716948472141,84.3723807479666,
61.2787674539506));
#150659=CARTESIAN_POINT('Ctrl Pts',(-14.7687077033096,84.3648174821419,
61.272714524461));
#150660=CARTESIAN_POINT('Ctrl Pts',(-14.7657651243324,84.3573580338555,
61.2667565871628));
#150661=CARTESIAN_POINT('Ctrl Pts',(-14.7628671103009,84.3500029141163,
61.2608930301829));
#150662=CARTESIAN_POINT('Ctrl Pts',(-14.7614181032852,84.3463253542468,
61.257961251693));
#150663=CARTESIAN_POINT('Ctrl Pts',(-14.7599802375059,84.3426738762865,
61.2550530685705));
#150664=CARTESIAN_POINT('Ctrl Pts',(-14.7585535129653,84.3390485424918,
61.2521684058551));
#150665=CARTESIAN_POINT('Ctrl Pts',(-14.7578401506951,84.3372358755944,
61.2507260744974));
#150666=CARTESIAN_POINT('Ctrl Pts',(-14.7571295737345,84.3354297447242,
61.2492896232594));
#150667=CARTESIAN_POINT('Ctrl Pts',(-14.7564217820838,84.3336301575628,
61.247859042867));
#150668=CARTESIAN_POINT('Ctrl Pts',(-14.7557139904332,84.3318305704013,
61.2464284624745));
#150669=CARTESIAN_POINT('Ctrl Pts',(-14.7555287793633,84.3313599170776,
61.2460540069098));
#150670=CARTESIAN_POINT('Ctrl Pts',(-14.7543067630621,84.3282510348247,
61.2435849050202));
#150671=CARTESIAN_POINT('Ctrl Pts',(-14.7009731122741,84.1925670507028,
61.1358234800683));
#150672=CARTESIAN_POINT('Ctrl Pts',(-14.6492756639653,84.0583603706525,
61.0330316455385));
#150673=CARTESIAN_POINT('Ctrl Pts',(-14.5992821274116,83.9259745135944,
60.934938049082));
#150674=CARTESIAN_POINT('Ctrl Pts',(-14.5480382949454,83.7902777986261,
60.8343912150441));
#150675=CARTESIAN_POINT('Ctrl Pts',(-14.4985844763709,83.656494044048,60.7387803835966));
#150676=CARTESIAN_POINT('Ctrl Pts',(-14.4509582668087,83.5249509404108,
60.6478107727522));
#150677=CARTESIAN_POINT('Ctrl Pts',(-14.4013863694749,83.388033867051,60.553124753211));
#150678=CARTESIAN_POINT('Ctrl Pts',(-14.3537943129532,83.2535442739116,
60.4634667115708));
#150679=CARTESIAN_POINT('Ctrl Pts',(-14.3081891898266,83.1218067953932,
60.3785044529254));
#150680=CARTESIAN_POINT('Ctrl Pts',(-14.2614841689706,82.98689209152,60.2914930868778));
#150681=CARTESIAN_POINT('Ctrl Pts',(-14.2168627979626,82.8548637261979,
60.2094065019078));
#150682=CARTESIAN_POINT('Ctrl Pts',(-14.1742998547136,82.7260253078505,
60.1318915570659));
#150683=CARTESIAN_POINT('Ctrl Pts',(-14.1301540233085,82.5923954725832,
60.0514938818783));
#150684=CARTESIAN_POINT('Ctrl Pts',(-14.0882223025456,82.4621972036696,
59.9760139082568));
#150685=CARTESIAN_POINT('Ctrl Pts',(-14.0484458053097,82.3357226260578,
59.9050656682173));
#150686=CARTESIAN_POINT('Ctrl Pts',(-14.0292152595889,82.274576589672,59.8707646746984));
#150687=CARTESIAN_POINT('Ctrl Pts',(-14.0104880489132,82.2143002468848,
59.8375230677923));
#150688=CARTESIAN_POINT('Ctrl Pts',(-13.9922553803942,82.1549229903178,
59.8052981836916));
#150689=CARTESIAN_POINT('Origin',(-15.5675364879071,89.9666295602638,59.722390240022));
#150690=CARTESIAN_POINT('Ctrl Pts',(-11.5022227331789,92.24059357536,63.80710267499));
#150691=CARTESIAN_POINT('Ctrl Pts',(-11.6900590068918,90.0819912782,64.9589646699191));
#150692=CARTESIAN_POINT('Ctrl Pts',(-13.3403353375583,88.35741258162,65.5284608708081));
#150693=CARTESIAN_POINT('Ctrl Pts',(-15.7224335390669,87.8306099166801,
65.263328953982));
#150694=CARTESIAN_POINT('Ctrl Pts',(-11.2606355037629,91.60559269607,62.78217333778));
#150695=CARTESIAN_POINT('Ctrl Pts',(-11.5151253257839,89.4713091151001,
64.100214239718));
#150696=CARTESIAN_POINT('Ctrl Pts',(-13.2736598773406,87.78772859478,64.744410182956));
#150697=CARTESIAN_POINT('Ctrl Pts',(-15.7260522384459,87.33074482683,64.417814013295));
#150698=CARTESIAN_POINT('Ctrl Pts',(-10.9937695135439,90.85061125927,61.83105273875));
#150699=CARTESIAN_POINT('Ctrl Pts',(-11.3301258891729,88.76446201931,63.328630671347));
#150700=CARTESIAN_POINT('Ctrl Pts',(-13.2094624536146,87.1401841301901,
64.0435746101571));
#150701=CARTESIAN_POINT('Ctrl Pts',(-15.7293652895179,86.75795515826,63.63240429366));
#150702=CARTESIAN_POINT('Ctrl Pts',(-10.7185240591989,89.96317024715,60.95778318153));
#150703=CARTESIAN_POINT('Ctrl Pts',(-11.1489392586459,87.96379513297,62.63906395814));
#150704=CARTESIAN_POINT('Ctrl Pts',(-13.1546927793252,86.41956569116,63.415047631478));
#150705=CARTESIAN_POINT('Ctrl Pts',(-15.7319333912539,86.10357629771,62.89715702778));
#150706=CARTESIAN_POINT('',(-15.5675364993575,87.7888410125626,65.1501684815529));
#150707=CARTESIAN_POINT('Ctrl Pts',(-15.5675364833309,87.78884038427,65.150168469018));
#150708=CARTESIAN_POINT('Ctrl Pts',(-15.5675364833309,87.328833019208,64.3996673554378));
#150709=CARTESIAN_POINT('Ctrl Pts',(-15.5675364833309,86.8094293099928,
63.6983716052815));
#150710=CARTESIAN_POINT('Ctrl Pts',(-15.5675364833309,86.22497216032,63.039015015514));
#150711=CARTESIAN_POINT('Origin',(-16.3445396268156,91.9999999945638,62.5690047661622));
#150712=CARTESIAN_POINT('Ctrl Pts',(-15.7267915542099,87.66538353981,64.99088137144));
#150713=CARTESIAN_POINT('Ctrl Pts',(-15.1845773178949,87.78121626868,65.060886705648));
#150714=CARTESIAN_POINT('Ctrl Pts',(-14.1051711636669,88.17293046477,65.106337310483));
#150715=CARTESIAN_POINT('Ctrl Pts',(-12.6905091996054,89.25086782998,64.83687208802));
#150716=CARTESIAN_POINT('Ctrl Pts',(-11.7187169000773,90.65190225521,64.266801370723));
#150717=CARTESIAN_POINT('Ctrl Pts',(-11.4633132605639,91.64600275828,63.752208112914));
#150718=CARTESIAN_POINT('Ctrl Pts',(-11.4262749273969,92.13114438891,63.478854086617));
#150719=CARTESIAN_POINT('Ctrl Pts',(-15.7174241139459,88.05181590963,65.61349528));
#150720=CARTESIAN_POINT('Ctrl Pts',(-15.2062704666909,88.16374583963,65.647308160843));
#150721=CARTESIAN_POINT('Ctrl Pts',(-14.2055312081989,88.52845110996,65.63754881954));
#150722=CARTESIAN_POINT('Ctrl Pts',(-12.8992702356658,89.4999792018,65.370181293364));
#150723=CARTESIAN_POINT('Ctrl Pts',(-11.9627691347456,90.7694986187,64.885655521381));
#150724=CARTESIAN_POINT('Ctrl Pts',(-11.6664290226336,91.70187766148,64.460214669977));
#150725=CARTESIAN_POINT('Ctrl Pts',(-11.5979936003541,92.16979109083,64.231872652613));
#150726=CARTESIAN_POINT('Ctrl Pts',(-15.7002731834799,88.72433014467,66.888180925632));
#150727=CARTESIAN_POINT('Ctrl Pts',(-15.2467616864919,88.82578365824,66.877587073637));
#150728=CARTESIAN_POINT('Ctrl Pts',(-14.3761051926899,89.1399254789,66.809235364743));
#150729=CARTESIAN_POINT('Ctrl Pts',(-13.2334233981792,89.94290089811,66.564598469622));
#150730=CARTESIAN_POINT('Ctrl Pts',(-12.3569947409571,90.99911738926,66.202850988947));
#150731=CARTESIAN_POINT('Ctrl Pts',(-12.0079448863869,91.80959396061,65.90398707677));
#150732=CARTESIAN_POINT('Ctrl Pts',(-11.8932535301169,92.23267100316,65.743127847465));
#150733=CARTESIAN_POINT('Ctrl Pts',(-15.6809296656369,89.45528966985,68.910358690794));
#150734=CARTESIAN_POINT('Ctrl Pts',(-15.2932117620329,89.54407252558,68.883763974286));
#150735=CARTESIAN_POINT('Ctrl Pts',(-14.5550938790869,89.80455055827,68.80807416969));
#150736=CARTESIAN_POINT('Ctrl Pts',(-13.5661328446367,90.4424335221,68.627789664249));
#150737=CARTESIAN_POINT('Ctrl Pts',(-12.7529607721535,91.28077197666,68.393673986953));
#150738=CARTESIAN_POINT('Ctrl Pts',(-12.365961770199,91.94231120585,68.209964343349));
#150739=CARTESIAN_POINT('Ctrl Pts',(-12.2119022262506,92.29761959052,68.111340150659));
#150740=CARTESIAN_POINT('Ctrl Pts',(-15.6718240232689,89.80966270923,70.589751969638));
#150741=CARTESIAN_POINT('Ctrl Pts',(-15.3151883355199,89.89024839345,70.568499736441));
#150742=CARTESIAN_POINT('Ctrl Pts',(-14.6374346715909,90.12243854682,70.515386313769));
#150743=CARTESIAN_POINT('Ctrl Pts',(-13.7177800255529,90.68309838244,70.403740151492));
#150744=CARTESIAN_POINT('Ctrl Pts',(-12.9367806317871,91.42083571917,70.266639480233));
#150745=CARTESIAN_POINT('Ctrl Pts',(-12.5380437113516,92.01029521624,70.162098655781));
#150746=CARTESIAN_POINT('Ctrl Pts',(-12.3689259125356,92.33083134343,70.106261328233));
#150747=CARTESIAN_POINT('Ctrl Pts',(-15.6681569363979,89.95256484147,71.952924446791));
#150748=CARTESIAN_POINT('Ctrl Pts',(-15.3240566546889,90.03018842994,71.942882594526));
#150749=CARTESIAN_POINT('Ctrl Pts',(-14.6702901207359,90.251604718,71.91857740059));
#150750=CARTESIAN_POINT('Ctrl Pts',(-13.7779625535849,90.781902689,71.869267078615));
#150751=CARTESIAN_POINT('Ctrl Pts',(-13.0100009538581,91.47919210506,71.809754343234));
#150752=CARTESIAN_POINT('Ctrl Pts',(-12.6072845252056,92.03865965686,71.7647747764));
#150753=CARTESIAN_POINT('Ctrl Pts',(-12.4326146758588,92.34428924054,71.740780477213));
#150754=CARTESIAN_POINT('Ctrl Pts',(-15.6672518258989,89.98826649279,72.9901833001568));
#150755=CARTESIAN_POINT('Ctrl Pts',(-15.3262479221849,90.06523849532,72.9901967080605));
#150756=CARTESIAN_POINT('Ctrl Pts',(-14.6783580903999,90.28411411107,72.9902284801791));
#150757=CARTESIAN_POINT('Ctrl Pts',(-13.7927252046839,90.80698987221,72.9902913584466));
#150758=CARTESIAN_POINT('Ctrl Pts',(-13.0280722247757,91.49419551439,72.9903661930626));
#150759=CARTESIAN_POINT('Ctrl Pts',(-12.6245703572795,92.04598973457,72.9904222000122));
#150760=CARTESIAN_POINT('Ctrl Pts',(-12.448659862507,92.34772444263,72.99045196511));
#150761=CARTESIAN_POINT('Ctrl Pts',(-15.6681623130659,89.95235479387,74.027597348738));
#150762=CARTESIAN_POINT('Ctrl Pts',(-15.3240436488079,90.02998313099,74.037661924352));
#150763=CARTESIAN_POINT('Ctrl Pts',(-14.6702420088379,90.25141581468,74.062025563468));
#150764=CARTESIAN_POINT('Ctrl Pts',(-13.7778744578779,90.78175855909,74.111462545138));
#150765=CARTESIAN_POINT('Ctrl Pts',(-13.0098936682318,91.4791070426,74.171133610375));
#150766=CARTESIAN_POINT('Ctrl Pts',(-12.607182956015,92.03861824211,74.216235762356));
#150767=CARTESIAN_POINT('Ctrl Pts',(-12.432521229246,92.34426951449,74.240296059607));
#150768=CARTESIAN_POINT('Ctrl Pts',(-15.6718394519489,89.80906885625,75.391194076941));
#150769=CARTESIAN_POINT('Ctrl Pts',(-15.3151510595369,89.88966890827,75.412453916529));
#150770=CARTESIAN_POINT('Ctrl Pts',(-14.6372958155469,90.1219072658,75.465606188341));
#150771=CARTESIAN_POINT('Ctrl Pts',(-13.7175254778809,90.68269626983,75.577380462654));
#150772=CARTESIAN_POINT('Ctrl Pts',(-12.9364725952808,91.42060127026,75.714668403773));
#150773=CARTESIAN_POINT('Ctrl Pts',(-12.5377553500737,92.0101813717,75.81936657303));
#150774=CARTESIAN_POINT('Ctrl Pts',(-12.3686628267388,92.33077602559,75.87529036582));
#150775=CARTESIAN_POINT('Ctrl Pts',(-15.6809458928869,89.45463784939,77.069912031792));
#150776=CARTESIAN_POINT('Ctrl Pts',(-15.2931726928849,89.54342942527,77.096526733112));
#150777=CARTESIAN_POINT('Ctrl Pts',(-14.5549455048969,89.80395021696,77.172266998453));
#150778=CARTESIAN_POINT('Ctrl Pts',(-13.5658570450709,90.44197313334,77.35265505278));
#150779=CARTESIAN_POINT('Ctrl Pts',(-12.7526266818154,91.28050419446,77.586890412431));
#150780=CARTESIAN_POINT('Ctrl Pts',(-12.365650677397,91.94218456205,77.770681920663));
#150781=CARTESIAN_POINT('Ctrl Pts',(-12.211619215407,92.29756139639,77.869346462264));
#150782=CARTESIAN_POINT('Ctrl Pts',(-15.7003066117399,88.72316214521,79.091611819645));
#150783=CARTESIAN_POINT('Ctrl Pts',(-15.2466816366939,88.82465310407,79.102078446305));
#150784=CARTESIAN_POINT('Ctrl Pts',(-14.3757920120989,89.13890937863,79.170256649061));
#150785=CARTESIAN_POINT('Ctrl Pts',(-13.2328406131236,89.94217161033,79.414894179539));
#150786=CARTESIAN_POINT('Ctrl Pts',(-12.3563116572606,90.9987279413,79.776886348901));
#150787=CARTESIAN_POINT('Ctrl Pts',(-12.0073443151488,91.80940467908,80.076051130249));
#150788=CARTESIAN_POINT('Ctrl Pts',(-11.8927306981703,92.23256005291,80.237086753741));
#150789=CARTESIAN_POINT('Ctrl Pts',(-15.7174479046779,88.05101812102,80.365575459028));
#150790=CARTESIAN_POINT('Ctrl Pts',(-15.2062142531389,88.1629537179,80.331694444122));
#150791=CARTESIAN_POINT('Ctrl Pts',(-14.2052953457019,88.5277087746,80.341352247073));
#150792=CARTESIAN_POINT('Ctrl Pts',(-12.8988133540273,89.49944296395,80.608734946825));
#150793=CARTESIAN_POINT('Ctrl Pts',(-11.9622504742339,90.76922852031,81.093440879978));
#150794=CARTESIAN_POINT('Ctrl Pts',(-11.665999801153,91.70174993568,81.519067946853));
#150795=CARTESIAN_POINT('Ctrl Pts',(-11.5976314399642,92.16971323709,81.747505318717));
#150796=CARTESIAN_POINT('Ctrl Pts',(-15.7267824555559,87.66570882409,80.986365678153));
#150797=CARTESIAN_POINT('Ctrl Pts',(-15.1845987207689,87.78153852098,80.916388892872));
#150798=CARTESIAN_POINT('Ctrl Pts',(-14.1052629937929,88.17323107872,80.870980798031));
#150799=CARTESIAN_POINT('Ctrl Pts',(-12.6906903789146,89.25108309886,81.14044110218));
#150800=CARTESIAN_POINT('Ctrl Pts',(-11.7189248514002,90.65200916615,81.71043962589));
#150801=CARTESIAN_POINT('Ctrl Pts',(-11.4634863537649,91.64605341585,82.224957584013));
#150802=CARTESIAN_POINT('Ctrl Pts',(-11.4264213925879,92.13117626492,82.498272907329));
#150803=CARTESIAN_POINT('',(-15.5675364993592,87.78884101254,80.8276102916413));
#150804=CARTESIAN_POINT('Ctrl Pts',(-15.5675364833309,87.7888410162132,
65.1501684793153));
#150805=CARTESIAN_POINT('Ctrl Pts',(-15.5675364833309,88.5016858245549,
66.3131718584543));
#150806=CARTESIAN_POINT('Ctrl Pts',(-15.5675364833309,89.0620994148936,
67.596770803385));
#150807=CARTESIAN_POINT('Ctrl Pts',(-15.5675364833309,89.8115874451887,
70.2378326687398));
#150808=CARTESIAN_POINT('Ctrl Pts',(-15.5675364833619,90.0000184154843,
71.6068563101325));
#150809=CARTESIAN_POINT('Ctrl Pts',(-15.5675364833619,89.9999816132753,
74.3712619372165));
#150810=CARTESIAN_POINT('Ctrl Pts',(-15.5675364832921,89.811422786206,75.7411963040703));
#150811=CARTESIAN_POINT('Ctrl Pts',(-15.5675364832921,89.0616726097933,
78.3818709723929));
#150812=CARTESIAN_POINT('Ctrl Pts',(-15.5675364833309,88.5006006367192,
79.6663773945077));
#150813=CARTESIAN_POINT('Ctrl Pts',(-15.5675364833309,87.7888410161944,
80.8276102938811));
#150814=CARTESIAN_POINT('Origin',(-16.3445396396806,92.0000000244254,83.4087739660212));
#150815=CARTESIAN_POINT('Ctrl Pts',(-10.7183277173379,89.96254449809,85.02062304992));
#150816=CARTESIAN_POINT('Ctrl Pts',(-11.1488047984589,87.9632262939201,
83.33921133143));
#150817=CARTESIAN_POINT('Ctrl Pts',(-13.1546497038193,86.4190502843901,
82.56318175446));
#150818=CARTESIAN_POINT('Ctrl Pts',(-15.7319351985739,86.1031085662,83.08114725601));
#150819=CARTESIAN_POINT('Ctrl Pts',(-10.9910678175989,90.84201858798,84.15530458801));
#150820=CARTESIAN_POINT('Ctrl Pts',(-11.3283473228609,88.7567304713001,
82.655879963167));
#150821=CARTESIAN_POINT('Ctrl Pts',(-13.2089159040691,87.13321591558,81.940328764438));
#150822=CARTESIAN_POINT('Ctrl Pts',(-15.7293910876869,86.75161252054,82.352567470474));
#150823=CARTESIAN_POINT('Ctrl Pts',(-11.2584139392769,91.59984702698,83.20508981628));
#150824=CARTESIAN_POINT('Ctrl Pts',(-11.5134937823379,89.46571522905,81.885572719919));
#150825=CARTESIAN_POINT('Ctrl Pts',(-13.2730319216979,87.78250254906,81.240664946913));
#150826=CARTESIAN_POINT('Ctrl Pts',(-15.7260859252379,87.32621487051,81.5677500443391));
#150827=CARTESIAN_POINT('Ctrl Pts',(-11.5024576829089,92.24121677999,82.169685215265));
#150828=CARTESIAN_POINT('Ctrl Pts',(-11.6902236879789,90.08258370557,81.017989950019));
#150829=CARTESIAN_POINT('Ctrl Pts',(-13.3403958339806,88.3579608586,80.44856560492));
#150830=CARTESIAN_POINT('Ctrl Pts',(-15.7224300293849,87.83109219926,80.713633689592));
#150831=CARTESIAN_POINT('',(-15.5675240107059,86.2249740704557,82.9387616027241));
#150832=CARTESIAN_POINT('Ctrl Pts',(-15.5675364833309,86.22497407053,82.93876160279));
#150833=CARTESIAN_POINT('Ctrl Pts',(-15.5675364833309,86.8043943602553,
82.2850871081574));
#150834=CARTESIAN_POINT('Ctrl Pts',(-15.5675364833309,87.3248780563056,
81.5845639231394));
#150835=CARTESIAN_POINT('Ctrl Pts',(-15.5675364833309,87.78884038418,80.827610304179));
#150836=CARTESIAN_POINT('Origin',(-15.5675364833255,89.9666295470783,86.2553885480238));
#150837=CARTESIAN_POINT('Ctrl Pts',(-15.7859374982469,86.2973478690701,
82.861383624054));
#150838=CARTESIAN_POINT('Ctrl Pts',(-13.2002732600763,86.61616439017,82.350395801636));
#150839=CARTESIAN_POINT('Ctrl Pts',(-11.2034697254169,88.19169796552,83.11121227181));
#150840=CARTESIAN_POINT('Ctrl Pts',(-10.7994091717259,90.2318522534,84.7613320424801));
#150841=CARTESIAN_POINT('Ctrl Pts',(-15.2200740724969,85.09597491677,84.23663134082));
#150842=CARTESIAN_POINT('Ctrl Pts',(-12.7693205182124,85.4992514263,83.74901632494));
#150843=CARTESIAN_POINT('Ctrl Pts',(-10.8258933224819,86.88885596641,84.6041155294301));
#150844=CARTESIAN_POINT('Ctrl Pts',(-10.2935001377599,88.61860858417,86.40429721952));
#150845=CARTESIAN_POINT('Ctrl Pts',(-14.6041660747529,83.61843798049,85.4050021444));
#150846=CARTESIAN_POINT('Ctrl Pts',(-12.2722897776884,84.0430132881801,
85.02702776225));
#150847=CARTESIAN_POINT('Ctrl Pts',(-10.3838362619649,85.2133039136001,
85.9584263883601));
#150848=CARTESIAN_POINT('Ctrl Pts',(-9.74335915314091,86.6307185139801,
87.80238251479));
#150849=CARTESIAN_POINT('Ctrl Pts',(-14.1110631602029,82.00217154684,86.2571636203899));
#150850=CARTESIAN_POINT('Ctrl Pts',(-11.8620763883538,82.3649964618,85.98143506887));
#150851=CARTESIAN_POINT('Ctrl Pts',(-10.0155685768139,83.30578341605,86.96682116639));
#150852=CARTESIAN_POINT('Ctrl Pts',(-9.30321403080992,84.45174593576,88.82286146045));
#150853=CARTESIAN_POINT('',(-13.9922632538737,82.1549216119811,86.172481390843));
#150854=CARTESIAN_POINT('Ctrl Pts',(-13.9922632538719,82.1549215895872,
86.1724813495793));
#150855=CARTESIAN_POINT('Ctrl Pts',(-14.0172691520505,82.2363556855938,
86.1282859153393));
#150856=CARTESIAN_POINT('Ctrl Pts',(-14.0444951537761,82.3230603988622,
86.0802579897279));
#150857=CARTESIAN_POINT('Ctrl Pts',(-14.0739412590485,82.4148321534633,
86.0280712679699));
#150858=CARTESIAN_POINT('Ctrl Pts',(-14.103239727916,82.5061437843298,85.9761461991509));
#150859=CARTESIAN_POINT('Ctrl Pts',(-14.1347360939012,82.6024720216257,
85.9201036981764));
#150860=CARTESIAN_POINT('Ctrl Pts',(-14.168430357004,82.7035774847945,85.8595884326989));
#150861=CARTESIAN_POINT('Ctrl Pts',(-14.2017860834929,82.8036671103104,
85.7996811826869));
#150862=CARTESIAN_POINT('Ctrl Pts',(-14.2372957630783,82.9084386673946,
85.7353903085883));
#150863=CARTESIAN_POINT('Ctrl Pts',(-14.2749593957603,83.0176183202769,
85.6663416728384));
#150864=CARTESIAN_POINT('Ctrl Pts',(-14.3123467036225,83.1259969604646,
85.5977996226319));
#150865=CARTESIAN_POINT('Ctrl Pts',(-14.3518564749289,83.238719492333,85.5245690663092));
#150866=CARTESIAN_POINT('Ctrl Pts',(-14.3934887096795,83.3554734177915,
85.4462592520283));
#150867=CARTESIAN_POINT('Ctrl Pts',(-14.4345893697325,83.4707365889582,
85.3689493244002));
#150868=CARTESIAN_POINT('Ctrl Pts',(-14.4777586385691,83.5899290508293,
85.2866886767035));
#150869=CARTESIAN_POINT('Ctrl Pts',(-14.5229965161894,83.7127033399285,
85.1990818711561));
#150870=CARTESIAN_POINT('Ctrl Pts',(-14.5440862344572,83.7699402242351,
85.1582399275344));
#150871=CARTESIAN_POINT('Ctrl Pts',(-14.565625541519,83.8279548927639,85.1162358101079));
#150872=CARTESIAN_POINT('Ctrl Pts',(-14.587614437375,83.8867084182141,85.0730283087226));
#150873=CARTESIAN_POINT('Ctrl Pts',(-14.6338638705101,84.0102852119087,
84.982149600699));
#150874=CARTESIAN_POINT('Ctrl Pts',(-14.6821022426349,84.1371339331067,
84.8859477694956));
#150875=CARTESIAN_POINT('Ctrl Pts',(-14.7323295537493,84.2668559002324,
84.7840316800976));
#150876=CARTESIAN_POINT('Ctrl Pts',(-14.7818901728027,84.3948560032224,
84.6834683736019));
#150877=CARTESIAN_POINT('Ctrl Pts',(-14.8333872809171,84.5256537143705,
84.5773411252745));
#150878=CARTESIAN_POINT('Ctrl Pts',(-14.8868208780926,84.6588157333711,
84.4652685467848));
#150879=CARTESIAN_POINT('Ctrl Pts',(-14.9390948549763,84.7890878593552,
84.3556281765504));
#150880=CARTESIAN_POINT('Ctrl Pts',(-14.9932221812818,84.9216228153263,
84.240297357683));
#150881=CARTESIAN_POINT('Ctrl Pts',(-15.0492028570091,85.0559653865393,
84.1189190426377));
#150882=CARTESIAN_POINT('Ctrl Pts',(-15.1044724993146,85.1886016178975,
83.9990824031357));
#150883=CARTESIAN_POINT('Ctrl Pts',(-15.1615487097392,85.322999912876,83.8733505427342));
#150884=CARTESIAN_POINT('Ctrl Pts',(-15.220431488283,85.4586724985529,83.7413853557963));
#150885=CARTESIAN_POINT('Ctrl Pts',(-15.2780845139391,85.5915115944024,
83.612176230541));
#150886=CARTESIAN_POINT('Ctrl Pts',(-15.3374694361964,85.7255722855737,
83.476991071888));
#150887=CARTESIAN_POINT('Ctrl Pts',(-15.3985862550548,85.8603485292922,
83.3355231300881));
#150888=CARTESIAN_POINT('Ctrl Pts',(-15.4535006297584,85.9814469975525,
83.2084120711414));
#150889=CARTESIAN_POINT('Ctrl Pts',(-15.5098132149755,86.1031225912152,
83.0762286641304));
#150890=CARTESIAN_POINT('Ctrl Pts',(-15.5675240107059,86.2249740704557,
82.9387616027241));
#150891=CARTESIAN_POINT('Origin',(-13.9922815003769,84.5398910501458,90.5670141919346));
#150892=CARTESIAN_POINT('Ctrl Pts',(-9.36316543113591,65.20514258604,88.68507306022));
#150893=CARTESIAN_POINT('Ctrl Pts',(-9.52089785507191,65.47810818538,88.25909049769));
#150894=CARTESIAN_POINT('Ctrl Pts',(-9.99271929691491,66.02944859918,87.46229833598));
#150895=CARTESIAN_POINT('Ctrl Pts',(-11.1638051091349,66.80362315008,86.55460492855));
#150896=CARTESIAN_POINT('Ctrl Pts',(-12.6378577027299,67.41687862472,86.06242162813));
#150897=CARTESIAN_POINT('Ctrl Pts',(-13.6855439527219,67.66310267119,86.05405719771));
#150898=CARTESIAN_POINT('Ctrl Pts',(-14.2037341389189,67.74518306757,86.12140353019));
#150899=CARTESIAN_POINT('Ctrl Pts',(-9.24767657508891,65.99401553665,88.94968435057));
#150900=CARTESIAN_POINT('Ctrl Pts',(-9.42115179510191,66.24144787729,88.5312692084));
#150901=CARTESIAN_POINT('Ctrl Pts',(-9.91247134952491,66.7389817684,87.75513773229));
#150902=CARTESIAN_POINT('Ctrl Pts',(-11.0704798546419,67.43983090513,86.87706862433));
#150903=CARTESIAN_POINT('Ctrl Pts',(-12.5011304605781,68.00629583084,86.3973053855));
#150904=CARTESIAN_POINT('Ctrl Pts',(-13.5150380396702,68.2467475693,86.38291437305));
#150905=CARTESIAN_POINT('Ctrl Pts',(-14.0186219503789,68.33174743894,86.44526609955));
#150906=CARTESIAN_POINT('Ctrl Pts',(-9.02110732129691,67.56711094663,89.39524706291));
#150907=CARTESIAN_POINT('Ctrl Pts',(-9.21938651903491,67.76671680646,88.99421222644));
#150908=CARTESIAN_POINT('Ctrl Pts',(-9.73855112510891,68.16487519537,88.25989487261));
#150909=CARTESIAN_POINT('Ctrl Pts',(-10.8679585310409,68.72847140715,87.43449506428));
#150910=CARTESIAN_POINT('Ctrl Pts',(-12.2214087371635,69.19888773049,86.97204043524));
#150911=CARTESIAN_POINT('Ctrl Pts',(-13.1759013667977,69.41622377861,86.94116396896));
#150912=CARTESIAN_POINT('Ctrl Pts',(-13.6534062038449,69.49967595943,86.99087839766));
#150913=CARTESIAN_POINT('Ctrl Pts',(-8.63390385764391,70.79440049297,90.01976900704));
#150914=CARTESIAN_POINT('Ctrl Pts',(-8.86287624955991,70.90266434284,89.65283473253));
#150915=CARTESIAN_POINT('Ctrl Pts',(-9.41039510203091,71.11616478701,88.99091950633));
#150916=CARTESIAN_POINT('Ctrl Pts',(-10.4863410151329,71.4218057268,88.24450783708));
#150917=CARTESIAN_POINT('Ctrl Pts',(-11.7226579851006,71.69058989452,87.79963352365));
#150918=CARTESIAN_POINT('Ctrl Pts',(-12.5878203220936,71.83087932662,87.73316725532));
#150919=CARTESIAN_POINT('Ctrl Pts',(-13.0250798682975,71.89078018955,87.75627315149));
#150920=CARTESIAN_POINT('Ctrl Pts',(-8.43646722755891,74.17704539539,90.27567271427));
#150921=CARTESIAN_POINT('Ctrl Pts',(-8.67457228700691,74.19840452429,89.9271492125));
#150922=CARTESIAN_POINT('Ctrl Pts',(-9.22633231332491,74.24043774156,89.30069277592));
#150923=CARTESIAN_POINT('Ctrl Pts',(-10.2725773694299,74.30035154213,88.5884829841));
#150924=CARTESIAN_POINT('Ctrl Pts',(-11.4566903832199,74.35277043018,88.14814037352));
#150925=CARTESIAN_POINT('Ctrl Pts',(-12.2830364939517,74.37997779971,88.06199406937));
#150926=CARTESIAN_POINT('Ctrl Pts',(-12.7024212510194,74.39158580279,88.07026937053));
#150927=CARTESIAN_POINT('Ctrl Pts',(-8.53644251351991,77.54566405391,90.14553315307));
#150928=CARTESIAN_POINT('Ctrl Pts',(-8.76988752817891,77.47982485493,89.78750600586));
#150929=CARTESIAN_POINT('Ctrl Pts',(-9.31940153097191,77.35014255379,89.14272588511));
#150930=CARTESIAN_POINT('Ctrl Pts',(-10.3807195496239,77.16495136756,88.41288548734));
#150931=CARTESIAN_POINT('Ctrl Pts',(-11.5914114362027,77.00256835126,87.97038907049));
#150932=CARTESIAN_POINT('Ctrl Pts',(-12.4374024314265,76.91808082036,87.89458815261));
#150933=CARTESIAN_POINT('Ctrl Pts',(-12.8657678794545,76.88202065256,87.91059102918));
#150934=CARTESIAN_POINT('Ctrl Pts',(-8.80312062497391,80.92213477605,89.75884753243));
#150935=CARTESIAN_POINT('Ctrl Pts',(-9.01991246902491,80.76692328379,89.3769250268));
#150936=CARTESIAN_POINT('Ctrl Pts',(-9.55697366388391,80.45923627782,88.68389914341));
#150937=CARTESIAN_POINT('Ctrl Pts',(-10.6566609744259,80.02082628925,87.90432815957));
#150938=CARTESIAN_POINT('Ctrl Pts',(-11.9426748847909,79.64382527526,87.45249436166));
#150939=CARTESIAN_POINT('Ctrl Pts',(-12.8456722144415,79.45666656147,87.40161797299));
#150940=CARTESIAN_POINT('Ctrl Pts',(-13.3001072668101,79.37996389478,87.4364636821));
#150941=CARTESIAN_POINT('Ctrl Pts',(-9.14077283870391,83.27442601644,89.19463338426));
#150942=CARTESIAN_POINT('Ctrl Pts',(-9.32880949855891,83.05062855214,88.78323786731));
#150943=CARTESIAN_POINT('Ctrl Pts',(-9.83816023022091,82.60292058201,88.0262405068));
#150944=CARTESIAN_POINT('Ctrl Pts',(-10.9840980004039,81.97007306255,87.17553264096));
#150945=CARTESIAN_POINT('Ctrl Pts',(-12.3746508960291,81.44717623679,86.70717184874));
#150946=CARTESIAN_POINT('Ctrl Pts',(-13.3573195647392,81.21230060616,86.68714707239));
#150947=CARTESIAN_POINT('Ctrl Pts',(-13.8473824995259,81.12471571508,86.74485486738));
#150948=CARTESIAN_POINT('Ctrl Pts',(-9.36320138448591,84.79518333694,88.68499094841));
#150949=CARTESIAN_POINT('Ctrl Pts',(-9.52093025095291,84.52220867034,88.25900375063));
#150950=CARTESIAN_POINT('Ctrl Pts',(-9.99274691583191,83.97084828236,87.46220423853));
#150951=CARTESIAN_POINT('Ctrl Pts',(-11.1638314564909,83.19663902225,86.55450907384));
#150952=CARTESIAN_POINT('Ctrl Pts',(-12.6378886830788,82.58334687056,86.0623326859));
#150953=CARTESIAN_POINT('Ctrl Pts',(-13.6855831157209,82.33710070822,86.05397688329));
#150954=CARTESIAN_POINT('Ctrl Pts',(-14.2037786680419,82.25501069724,86.1213279171));
#150955=CARTESIAN_POINT('',(-13.992300447329,67.8450850046154,86.1724849817789));
#150956=CARTESIAN_POINT('Ctrl Pts',(-13.9922632538719,82.1549215895871,
86.1724813495793));
#150957=CARTESIAN_POINT('Ctrl Pts',(-13.9285551321236,81.9479298053255,
86.2848187148616));
#150958=CARTESIAN_POINT('Ctrl Pts',(-13.8647015765576,81.7390803248916,
86.3918585032908));
#150959=CARTESIAN_POINT('Ctrl Pts',(-13.8013730345312,81.5283495129631,
86.4937275061797));
#150960=CARTESIAN_POINT('Ctrl Pts',(-13.7378365702042,81.3169268228726,
86.5959309686469));
#150961=CARTESIAN_POINT('Ctrl Pts',(-13.6748285725588,81.1036100174599,
86.6929298523649));
#150962=CARTESIAN_POINT('Ctrl Pts',(-13.6130261143607,80.8883458651168,
86.7848084561006));
#150963=CARTESIAN_POINT('Ctrl Pts',(-13.5511371714079,80.6727804777106,
86.8768156323676));
#150964=CARTESIAN_POINT('Ctrl Pts',(-13.4904571442642,80.4552618660574,
86.9636883768117));
#150965=CARTESIAN_POINT('Ctrl Pts',(-13.4316659521088,80.2357134520804,
87.0454645259126));
#150966=CARTESIAN_POINT('Ctrl Pts',(-13.3830763136172,80.0542614747445,
87.1130507301784));
#150967=CARTESIAN_POINT('Ctrl Pts',(-13.3357768744825,79.8714224756304,
87.1771548191785));
#150968=CARTESIAN_POINT('Ctrl Pts',(-13.2901514758223,79.6871444536011,
87.2377727418144));
#150969=CARTESIAN_POINT('Ctrl Pts',(-13.2637884122878,79.5806657521444,
87.2727987184132));
#150970=CARTESIAN_POINT('Ctrl Pts',(-13.2379850470338,79.4737055706827,
87.3066606315146));
#150971=CARTESIAN_POINT('Ctrl Pts',(-13.2128161597323,79.3662528131415,
87.3393540609985));
#150972=CARTESIAN_POINT('Ctrl Pts',(-13.2096700488196,79.3528212184489,
87.343440739684));
#150973=CARTESIAN_POINT('Ctrl Pts',(-13.2065338516249,79.3393819268051,
87.3475091572638));
#150974=CARTESIAN_POINT('Ctrl Pts',(-13.203407714876,79.3259349166383,87.3515593019199));
#150975=CARTESIAN_POINT('Ctrl Pts',(-13.2005271915918,79.3135444075215,
87.3552912359084));
#150976=CARTESIAN_POINT('Ctrl Pts',(-13.1986999886115,79.3056588058398,
87.3576538209563));
#150977=CARTESIAN_POINT('Ctrl Pts',(-13.1966065603476,79.2966138895657,
87.3603579644251));
#150978=CARTESIAN_POINT('Ctrl Pts',(-13.1964280600827,79.2958426570481,
87.3605885385192));
#150979=CARTESIAN_POINT('Ctrl Pts',(-13.1962476242391,79.2950629873024,
87.3608215676654));
#150980=CARTESIAN_POINT('Ctrl Pts',(-13.1960644347913,79.29427136435,87.3610580972974));
#150981=CARTESIAN_POINT('Ctrl Pts',(-13.1914012110925,79.2741200130764,
87.3670791350732));
#150982=CARTESIAN_POINT('Ctrl Pts',(-13.1867535809486,79.2539526669486,
87.3730587869752));
#150983=CARTESIAN_POINT('Ctrl Pts',(-13.1821220625226,79.2337692755917,
87.3789970206825));
#150984=CARTESIAN_POINT('Ctrl Pts',(-13.1728590256707,79.1934024928777,
87.3908734880971));
#150985=CARTESIAN_POINT('Ctrl Pts',(-13.1636604356901,79.1529715301373,
87.4025842891849));
#150986=CARTESIAN_POINT('Ctrl Pts',(-13.1545307716034,79.1124748055347,
87.4141294529997));
#150987=CARTESIAN_POINT('Ctrl Pts',(-13.1180121152563,78.9504879071245,
87.460310108259));
#150988=CARTESIAN_POINT('Ctrl Pts',(-13.0825962732094,78.7874487141038,
87.5038416215084));
#150989=CARTESIAN_POINT('Ctrl Pts',(-13.0485477163981,78.6233237291505,
87.5446966521965));
#150990=CARTESIAN_POINT('Ctrl Pts',(-13.0031366693941,78.4044278902592,
87.5991855907208));
#150991=CARTESIAN_POINT('Ctrl Pts',(-12.9601460565636,78.1836558297552,
87.6488934074955));
#150992=CARTESIAN_POINT('Ctrl Pts',(-12.9200620632149,77.9614407620136,
87.6936460528116));
#150993=CARTESIAN_POINT('Ctrl Pts',(-12.9000372409868,77.8504284387346,
87.716003200686));
#150994=CARTESIAN_POINT('Ctrl Pts',(-12.8807378287883,77.7390562691211,
87.7371244382603));
#150995=CARTESIAN_POINT('Ctrl Pts',(-12.862224443683,77.6273797845303,87.756992699729));
#150996=CARTESIAN_POINT('Ctrl Pts',(-12.8344384878748,77.459769277429,87.7868121321026));
#150997=CARTESIAN_POINT('Ctrl Pts',(-12.8084219966983,77.2914725236344,
87.8138085541141));
#150998=CARTESIAN_POINT('Ctrl Pts',(-12.7843726914315,77.1226755619766,
87.8379381257615));
#150999=CARTESIAN_POINT('Ctrl Pts',(-12.7813665282732,77.1015759417694,
87.8409543222174));
#151000=CARTESIAN_POINT('Ctrl Pts',(-12.7783911023947,77.0804685064775,
87.8439257445653));
#151001=CARTESIAN_POINT('Ctrl Pts',(-12.7754467826672,77.059353615165,87.8468523252774));
#151002=CARTESIAN_POINT('Ctrl Pts',(-12.7750787427012,77.0567142537509,
87.8472181478665));
#151003=CARTESIAN_POINT('Ctrl Pts',(-12.7747111887689,77.0540747572995,
87.8475831355736));
#151004=CARTESIAN_POINT('Ctrl Pts',(-12.7744712246906,77.0523490281323,
87.8478214971566));
#151005=CARTESIAN_POINT('Ctrl Pts',(-12.7742312606124,77.050623298965,87.8480598587396));
#151006=CARTESIAN_POINT('Ctrl Pts',(-12.7741183995359,77.0498113824519,
87.8481717851012));
#151007=CARTESIAN_POINT('Ctrl Pts',(-12.7740743863699,77.0494940241591,
87.8482155572021));
#151008=CARTESIAN_POINT('Ctrl Pts',(-12.7739863600379,77.0488593075736,
87.8483031014039));
#151009=CARTESIAN_POINT('Ctrl Pts',(-12.7738970165722,77.0482133976243,
87.8483921480379));
#151010=CARTESIAN_POINT('Ctrl Pts',(-12.773806359778,77.0475562935894,87.8484826927436));
#151011=CARTESIAN_POINT('Ctrl Pts',(-12.7736250461896,77.0462420855196,
87.8486637821549));
#151012=CARTESIAN_POINT('Ctrl Pts',(-12.7734384792872,77.0448831011278,
87.8488508640047));
#151013=CARTESIAN_POINT('Ctrl Pts',(-12.7732466894325,77.0434793345013,
87.849043901573));
#151014=CARTESIAN_POINT('Ctrl Pts',(-12.7724795300137,77.0378642679956,
87.849816051846));
#151015=CARTESIAN_POINT('Ctrl Pts',(-12.7716288033574,77.0315326922741,
87.8506835421921));
#151016=CARTESIAN_POINT('Ctrl Pts',(-12.7706965594528,77.0244841615641,
87.8516436360311));
#151017=CARTESIAN_POINT('Ctrl Pts',(-12.7688320716436,77.0103871001443,
87.8535638237089));
#151018=CARTESIAN_POINT('Ctrl Pts',(-12.7666415148415,76.9934223030366,
87.8558550473182));
#151019=CARTESIAN_POINT('Ctrl Pts',(-12.7641489243869,76.9735853740015,
87.8584879276142));
#151020=CARTESIAN_POINT('Ctrl Pts',(-12.7603881763992,76.943655992376,87.8624603408348));
#151021=CARTESIAN_POINT('Ctrl Pts',(-12.7559136930925,76.9071891064106,
87.8672128741886));
#151022=CARTESIAN_POINT('Ctrl Pts',(-12.7508847778743,76.8641652564707,
87.872601554469));
#151023=CARTESIAN_POINT('Ctrl Pts',(-12.7458602599409,76.8211790265965,
87.8779855228859));
#151024=CARTESIAN_POINT('Ctrl Pts',(-12.740282279263,76.7716471452226,87.8840045375955));
#151025=CARTESIAN_POINT('Ctrl Pts',(-12.7343097217284,76.7155467348373,
87.8904631088614));
#151026=CARTESIAN_POINT('Ctrl Pts',(-12.7304119732769,76.678935067818,87.8946780345453));
#151027=CARTESIAN_POINT('Ctrl Pts',(-12.7263461748165,76.6395257987867,
87.8990791095172));
#151028=CARTESIAN_POINT('Ctrl Pts',(-12.7221564880409,76.5973122916239,
87.9036000255105));
#151029=CARTESIAN_POINT('Ctrl Pts',(-12.7157559154614,76.5328228367065,
87.9105066160246));
#151030=CARTESIAN_POINT('Ctrl Pts',(-12.7090596215634,76.4617886583938,
87.9176953647784));
#151031=CARTESIAN_POINT('Ctrl Pts',(-12.7023690004211,76.3841852195534,
87.9248872199345));
#151032=CARTESIAN_POINT('Ctrl Pts',(-12.6957025603321,76.3068622528613,
87.9320530824916));
#151033=CARTESIAN_POINT('Ctrl Pts',(-12.6890417520683,76.2230171639885,
87.939222012628));
#151034=CARTESIAN_POINT('Ctrl Pts',(-12.6826847136308,76.1326304096918,
87.9460665385376));
#151035=CARTESIAN_POINT('Ctrl Pts',(-12.6784412442731,76.0722951724632,
87.9506354169941));
#151036=CARTESIAN_POINT('Ctrl Pts',(-12.6743331307868,76.0090451519203,
87.9550586867079));
#151037=CARTESIAN_POINT('Ctrl Pts',(-12.6704490512014,75.9428766493832,
87.9592261771818));
#151038=CARTESIAN_POINT('Ctrl Pts',(-12.6646823510838,75.8446361517392,
87.9654136579679));
#151039=CARTESIAN_POINT('Ctrl Pts',(-12.6594351114857,75.7399612101461,
87.9710396191839));
#151040=CARTESIAN_POINT('Ctrl Pts',(-12.6551289588245,75.6288466423876,
87.9757019863411));
#151041=CARTESIAN_POINT('Ctrl Pts',(-12.6536321155254,75.590222582983,87.9773226518368));
#151042=CARTESIAN_POINT('Ctrl Pts',(-12.6522489835133,75.55082055245,87.9788264446894));
#151043=CARTESIAN_POINT('Ctrl Pts',(-12.6509972715651,75.5106407819581,
87.9801950666));
#151044=CARTESIAN_POINT('Ctrl Pts',(-12.6485709389679,75.43275586041,87.9828480187905));
#151045=CARTESIAN_POINT('Ctrl Pts',(-12.6466421085366,75.3519482421605,
87.9849937077908));
#151046=CARTESIAN_POINT('Ctrl Pts',(-12.6453635745304,75.2682216895248,
87.9864910990295));
#151047=CARTESIAN_POINT('Ctrl Pts',(-12.6447243075273,75.2263584132069,
87.9872397946489));
#151048=CARTESIAN_POINT('Ctrl Pts',(-12.6442478758664,75.1837654570326,
87.9878262556065));
#151049=CARTESIAN_POINT('Ctrl Pts',(-12.6439550112119,75.140443641486,87.9882318916222));
#151050=CARTESIAN_POINT('Ctrl Pts',(-12.6438085788846,75.1187827337127,
87.98843470963));
#151051=CARTESIAN_POINT('Ctrl Pts',(-12.643708038309,75.0969396106309,87.9885923114292));
#151052=CARTESIAN_POINT('Ctrl Pts',(-12.6436561075585,75.0749144037385,
87.9887023131505));
#151053=CARTESIAN_POINT('Ctrl Pts',(-12.6436301421833,75.0639018002923,
87.9887573140112));
#151054=CARTESIAN_POINT('Ctrl Pts',(-12.6436163292643,75.0528436758568,
87.9888004142306));
#151055=CARTESIAN_POINT('Ctrl Pts',(-12.6436150126618,75.0417400477704,
87.9888313120813));
#151056=CARTESIAN_POINT('Ctrl Pts',(-12.6436136960592,75.030636419684,87.988862209932));
#151057=CARTESIAN_POINT('Ctrl Pts',(-12.6436289425742,75.0175924670353,
87.9888819529564));
#151058=CARTESIAN_POINT('Ctrl Pts',(-12.643648897583,75.0082926704016,87.9888870943004));
#151059=CARTESIAN_POINT('Ctrl Pts',(-12.644195767988,74.7534301646491,87.9890279937058));
#151060=CARTESIAN_POINT('Ctrl Pts',(-12.6513772312014,74.4981090494674,
87.9826693314223));
#151061=CARTESIAN_POINT('Ctrl Pts',(-12.6647090533377,74.2428344994553,
87.9697672114868));
#151062=CARTESIAN_POINT('Ctrl Pts',(-12.6780337947826,73.9876955288341,
87.9568719440227));
#151063=CARTESIAN_POINT('Ctrl Pts',(-12.6975023638259,73.7326034297094,
87.9374401521479));
#151064=CARTESIAN_POINT('Ctrl Pts',(-12.72263129772,73.4780643757733,87.9114800448976));
#151065=CARTESIAN_POINT('Ctrl Pts',(-12.7310755086258,73.3925302474942,
87.9027565303353));
#151066=CARTESIAN_POINT('Ctrl Pts',(-12.7401588866746,73.3070585602922,
87.8932962750379));
#151067=CARTESIAN_POINT('Ctrl Pts',(-12.7498630868526,73.22166845818,87.8831009107718));
#151068=CARTESIAN_POINT('Ctrl Pts',(-12.7782149963072,72.9721916956449,
87.8533140103342));
#151069=CARTESIAN_POINT('Ctrl Pts',(-12.8118641852904,72.7234184043276,
87.8172493006473));
#151070=CARTESIAN_POINT('Ctrl Pts',(-12.8503429411276,72.4758397156348,
87.7749847081594));
#151071=CARTESIAN_POINT('Ctrl Pts',(-12.8576532368596,72.4288040620151,
87.7669551691747));
#151072=CARTESIAN_POINT('Ctrl Pts',(-12.8651378481022,72.3818115008075,
87.7587020044201));
#151073=CARTESIAN_POINT('Ctrl Pts',(-12.8727935676933,72.3348653610224,
87.7502259573693));
#151074=CARTESIAN_POINT('Ctrl Pts',(-12.8967698986114,72.1878385310274,
87.7236805090219));
#151075=CARTESIAN_POINT('Ctrl Pts',(-12.9224245102739,72.0412671229056,
87.6949484896749));
#151076=CARTESIAN_POINT('Ctrl Pts',(-12.9496575479537,71.8952524204115,
87.6640569313489));
#151077=CARTESIAN_POINT('Ctrl Pts',(-12.9632740667936,71.8222450691645,
87.6486111521859));
#151078=CARTESIAN_POINT('Ctrl Pts',(-12.9772851921378,71.7493768545001,
87.6326255846485));
#151079=CARTESIAN_POINT('Ctrl Pts',(-12.9916784023378,71.676660173943,87.6161041727429));
#151080=CARTESIAN_POINT('Ctrl Pts',(-12.9988750074377,71.6403018336645,
87.6078434667901));
#151081=CARTESIAN_POINT('Ctrl Pts',(-13.0061671337516,71.6039813737283,
87.599448805464));
#151082=CARTESIAN_POINT('Ctrl Pts',(-13.0135532114325,71.5677003261153,
87.5909207161125));
#151083=CARTESIAN_POINT('Ctrl Pts',(-13.0204776592583,71.533686843978,87.5829256323456));
#151084=CARTESIAN_POINT('Ctrl Pts',(-13.0274846815277,71.4997080014925,
87.5748132780719));
#151085=CARTESIAN_POINT('Ctrl Pts',(-13.0345729826817,71.4657650503592,
87.5665841055929));
#151086=CARTESIAN_POINT('Ctrl Pts',(-13.035045536092,71.4635021869503,87.5660354940943));
#151087=CARTESIAN_POINT('Ctrl Pts',(-13.0358533538668,71.4596384428753,
87.5650974157022));
#151088=CARTESIAN_POINT('Ctrl Pts',(-13.0359917262243,71.4589769390507,
87.5649367136788));
#151089=CARTESIAN_POINT('Ctrl Pts',(-13.040419641666,71.4378088166649,87.5597942489322));
#151090=CARTESIAN_POINT('Ctrl Pts',(-13.0461916289705,71.4097504302298,
87.5529342150623));
#151091=CARTESIAN_POINT('Ctrl Pts',(-13.0534262918525,71.3748480667611,
87.5442414421276));
#151092=CARTESIAN_POINT('Ctrl Pts',(-13.0604266942912,71.3410758517556,
87.5358301436547));
#151093=CARTESIAN_POINT('Ctrl Pts',(-13.0687965821947,71.3008956697415,
87.5257025281699));
#151094=CARTESIAN_POINT('Ctrl Pts',(-13.0786434070465,71.2543642514234,
87.5137030803588));
#151095=CARTESIAN_POINT('Ctrl Pts',(-13.0889845009582,71.2054971522406,
87.5011013108982));
#151096=CARTESIAN_POINT('Ctrl Pts',(-13.1009545251389,71.1496248624621,
87.4864354574992));
#151097=CARTESIAN_POINT('Ctrl Pts',(-13.114677937705,71.0868327997857,87.4694668081874));
#151098=CARTESIAN_POINT('Ctrl Pts',(-13.1284013502712,71.0240407371094,
87.4524981588757));
#151099=CARTESIAN_POINT('Ctrl Pts',(-13.1438781512227,70.9543286492023,
87.4332265983425));
#151100=CARTESIAN_POINT('Ctrl Pts',(-13.1612327986762,70.8778054772566,
87.4113549288049));
#151101=CARTESIAN_POINT('Ctrl Pts',(-13.1783109484543,70.8025014876197,
87.3898317230317));
#151102=CARTESIAN_POINT('Ctrl Pts',(-13.1972368931742,70.7206039818765,
87.3657911400615));
#151103=CARTESIAN_POINT('Ctrl Pts',(-13.2181516178511,70.6322258372372,
87.338891089127));
#151104=CARTESIAN_POINT('Ctrl Pts',(-13.239066342528,70.5438476925979,87.3119910381925));
#151105=CARTESIAN_POINT('Ctrl Pts',(-13.2619698471617,70.4489885678385,
87.2822313861059));
#151106=CARTESIAN_POINT('Ctrl Pts',(-13.2870031167675,70.347792376931,87.2492177219255));
#151107=CARTESIAN_POINT('Ctrl Pts',(-13.3106570501867,70.2521721083965,
87.2180231146391));
#151108=CARTESIAN_POINT('Ctrl Pts',(-13.3362102524477,70.1508910394946,
87.1839219449404));
#151109=CARTESIAN_POINT('Ctrl Pts',(-13.3637483457489,70.0440780364571,
87.1465317570904));
#151110=CARTESIAN_POINT('Ctrl Pts',(-13.3653541796678,70.0378494300906,
87.1443514161632));
#151111=CARTESIAN_POINT('Ctrl Pts',(-13.3669667630647,70.03160202198,87.142159879629));
#151112=CARTESIAN_POINT('Ctrl Pts',(-13.3685861129178,70.0253358411578,
87.1399570673852));
#151113=CARTESIAN_POINT('Ctrl Pts',(-13.3832807253887,69.9684740711821,
87.1199678895022));
#151114=CARTESIAN_POINT('Ctrl Pts',(-13.3985319081895,69.9100658854031,
87.0990503614127));
#151115=CARTESIAN_POINT('Ctrl Pts',(-13.4143477727133,69.8501321735506,
87.0771419883082));
#151116=CARTESIAN_POINT('Ctrl Pts',(-13.4222557049753,69.8201653176244,
87.0661878017559));
#151117=CARTESIAN_POINT('Ctrl Pts',(-13.4303048076679,69.7898171021899,
87.0549858456137));
#151118=CARTESIAN_POINT('Ctrl Pts',(-13.4384956724289,69.7590902424223,
87.0435279416239));
#151119=CARTESIAN_POINT('Ctrl Pts',(-13.4425911048093,69.7437268125385,
87.037798989629));
#151120=CARTESIAN_POINT('Ctrl Pts',(-13.4467219777069,69.7282687230002,
87.0320060469309));
#151121=CARTESIAN_POINT('Ctrl Pts',(-13.4508883493145,69.7127163209738,
87.0261480682993));
#151122=CARTESIAN_POINT('Ctrl Pts',(-13.4529715351183,69.7049401199606,
87.0232190789835));
#151123=CARTESIAN_POINT('Ctrl Pts',(-13.4550635955996,69.6971403409203,
87.0202738304489));
#151124=CARTESIAN_POINT('Ctrl Pts',(-13.4571645363573,69.6893170276936,
87.0173121905753));
#151125=CARTESIAN_POINT('Ctrl Pts',(-13.459265477115,69.6814937144669,87.0143505507017));
#151126=CARTESIAN_POINT('Ctrl Pts',(-13.4618074963028,69.6720413854221,
87.0107616557083));
#151127=CARTESIAN_POINT('Ctrl Pts',(-13.4634940045198,69.6657765296424,
87.0083779638529));
#151128=CARTESIAN_POINT('Ctrl Pts',(-13.5025360795504,69.5207473107225,
86.9531963315711));
#151129=CARTESIAN_POINT('Ctrl Pts',(-13.5406679975864,69.382336143713,86.8979602069376));
#151130=CARTESIAN_POINT('Ctrl Pts',(-13.5776553922134,69.250422107576,86.8432155722503));
#151131=CARTESIAN_POINT('Ctrl Pts',(-13.6150631200759,69.1170089700783,
86.7878488069789));
#151132=CARTESIAN_POINT('Ctrl Pts',(-13.6513001634661,68.9902410372982,
86.7329848247617));
#151133=CARTESIAN_POINT('Ctrl Pts',(-13.6861240746425,68.8699806916482,
86.6791363996632));
#151134=CARTESIAN_POINT('Ctrl Pts',(-13.7120606591743,68.780411699671,86.639030501667));
#151135=CARTESIAN_POINT('Ctrl Pts',(-13.737213357045,68.6944522788393,86.5994868643773));
#151136=CARTESIAN_POINT('Ctrl Pts',(-13.7614820014407,68.6120432588692,
86.5606987233428));
#151137=CARTESIAN_POINT('Ctrl Pts',(-13.7942709972546,68.5007016871368,
86.5082926567626));
#151138=CARTESIAN_POINT('Ctrl Pts',(-13.8254696763556,68.3958423297509,
86.4572683615289));
#151139=CARTESIAN_POINT('Ctrl Pts',(-13.8550187233594,68.2973101826394,
86.4080528930081));
#151140=CARTESIAN_POINT('Ctrl Pts',(-13.8847124904967,68.1982954620806,
86.358596385608));
#151141=CARTESIAN_POINT('Ctrl Pts',(-13.9127404274108,68.1056697133762,
86.3109664100483));
#151142=CARTESIAN_POINT('Ctrl Pts',(-13.9390423429289,68.0192804077862,
86.2655438588061));
#151143=CARTESIAN_POINT('Ctrl Pts',(-13.9576676956576,67.9581049664956,
86.2333784814158));
#151144=CARTESIAN_POINT('Ctrl Pts',(-13.9754275217645,67.9000569338153,
86.2023189351381));
#151145=CARTESIAN_POINT('Ctrl Pts',(-13.9923004473289,67.845085027017,86.1724849405017));
#151146=CARTESIAN_POINT('Origin',(-13.9922814997631,65.4601089523298,90.5670141932079));
#151147=CARTESIAN_POINT('Ctrl Pts',(-14.1113299480719,67.99729033203,86.25689542676));
#151148=CARTESIAN_POINT('Ctrl Pts',(-11.862640570514,67.63449740977,85.9811177666601));
#151149=CARTESIAN_POINT('Ctrl Pts',(-10.0162267656979,66.69382083775,86.9661594600301));
#151150=CARTESIAN_POINT('Ctrl Pts',(-9.30362299642391,65.54790245802,88.82184290376));
#151151=CARTESIAN_POINT('Ctrl Pts',(-14.6084235582589,66.3684868668701,
85.3977275067001));
#151152=CARTESIAN_POINT('Ctrl Pts',(-12.2761791919147,65.94373812164,85.01902796748));
#151153=CARTESIAN_POINT('Ctrl Pts',(-10.3874061607769,64.7718800752,85.94969573064));
#151154=CARTESIAN_POINT('Ctrl Pts',(-9.74725467144591,63.35238921989,87.79310189113));
#151155=CARTESIAN_POINT('Ctrl Pts',(-15.2202405059459,64.90419477503,84.23630032921));
#151156=CARTESIAN_POINT('Ctrl Pts',(-12.769810936217,64.5010541575,83.7487065063399));
#151157=CARTESIAN_POINT('Ctrl Pts',(-10.8264676087059,63.11180437274,84.60346776298));
#151158=CARTESIAN_POINT('Ctrl Pts',(-10.2937231765289,61.38225058552,86.4032922329301));
#151159=CARTESIAN_POINT('Ctrl Pts',(-15.7858253484379,63.70313319505,82.861956262162));
#151160=CARTESIAN_POINT('Ctrl Pts',(-13.2006025443827,63.38438634906,82.351027486016));
#151161=CARTESIAN_POINT('Ctrl Pts',(-11.2038824748619,61.8092972954501,
83.1115754237101));
#151162=CARTESIAN_POINT('Ctrl Pts',(-10.7993506281109,59.76948116378,84.76141092969));
#151163=CARTESIAN_POINT('',(-15.5675364833309,63.77502783968,82.938763757646));
#151164=CARTESIAN_POINT('Ctrl Pts',(-15.5675364833309,63.7750278396777,
82.938763757648));
#151165=CARTESIAN_POINT('Ctrl Pts',(-15.4656186766729,63.9946650181252,
83.186547912653));
#151166=CARTESIAN_POINT('Ctrl Pts',(-15.3632899217089,64.2226173284476,
83.4269525126868));
#151167=CARTESIAN_POINT('Ctrl Pts',(-15.2605507121745,64.4582711559872,
83.6595429156073));
#151168=CARTESIAN_POINT('Ctrl Pts',(-15.2286410871491,64.5314625432545,
83.7317828381775));
#151169=CARTESIAN_POINT('Ctrl Pts',(-15.1966921480705,64.6053970859381,
83.8032689508469));
#151170=CARTESIAN_POINT('Ctrl Pts',(-15.1647047257657,64.6800571258485,
83.8739882984837));
#151171=CARTESIAN_POINT('Ctrl Pts',(-15.0972161681521,64.8375783651946,
84.0231952812129));
#151172=CARTESIAN_POINT('Ctrl Pts',(-15.0295538846762,64.9983290816565,
84.1689893491265));
#151173=CARTESIAN_POINT('Ctrl Pts',(-14.961717781448,65.1621474989424,84.31124838789));
#151174=CARTESIAN_POINT('Ctrl Pts',(-14.9277997298339,65.2440567075854,
84.3823779072718));
#151175=CARTESIAN_POINT('Ctrl Pts',(-14.8938382230921,65.3267329248824,
84.4526236609836));
#151176=CARTESIAN_POINT('Ctrl Pts',(-14.8598332546457,65.4101563011331,
84.5219702946248));
#151177=CARTESIAN_POINT('Ctrl Pts',(-14.8428307704224,65.4518679892585,
84.5566436114454));
#151178=CARTESIAN_POINT('Ctrl Pts',(-14.8258174208648,65.4937664700047,
84.5910921470643));
#151179=CARTESIAN_POINT('Ctrl Pts',(-14.8087932058618,65.5358492776703,
84.6253139766023));
#151180=CARTESIAN_POINT('Ctrl Pts',(-14.8002810983603,65.5568906815031,
84.6424248913712));
#151181=CARTESIAN_POINT('Ctrl Pts',(-14.7917662745059,65.5779781671964,
84.6594791295602));
#151182=CARTESIAN_POINT('Ctrl Pts',(-14.7832487343406,65.59911142716,84.6764764501779));
#151183=CARTESIAN_POINT('Ctrl Pts',(-14.778989964258,65.6096780571419,84.6849751104868));
#151184=CARTESIAN_POINT('Ctrl Pts',(-14.7747305150982,65.6202561306973,
84.6934595413993));
#151185=CARTESIAN_POINT('Ctrl Pts',(-14.7704703868703,65.6308456094083,
84.70192971277));
#151186=CARTESIAN_POINT('Ctrl Pts',(-14.7662102586423,65.6414350881193,
84.7103998841407));
#151187=CARTESIAN_POINT('Ctrl Pts',(-14.7614474301979,65.6532861400737,
84.7198502548234));
#151188=CARTESIAN_POINT('Ctrl Pts',(-14.7576879649934,65.6626482226085,
84.7272974180975));
#151189=CARTESIAN_POINT('Ctrl Pts',(-14.7244750223662,65.7453574094699,
84.7930892776053));
#151190=CARTESIAN_POINT('Ctrl Pts',(-14.6899771016152,65.8331893986453,
84.8615430975335));
#151191=CARTESIAN_POINT('Ctrl Pts',(-14.654150529173,65.9263531473689,84.9323443142181));
#151192=CARTESIAN_POINT('Ctrl Pts',(-14.6190487988401,66.0176320099999,
85.0017130828691));
#151193=CARTESIAN_POINT('Ctrl Pts',(-14.5826713302042,66.1140292730603,
85.0733352782067));
#151194=CARTESIAN_POINT('Ctrl Pts',(-14.545005571114,66.215750145994,85.1468761711002));
#151195=CARTESIAN_POINT('Ctrl Pts',(-14.5085278025403,66.3142627089058,
85.2180975598754));
#151196=CARTESIAN_POINT('Ctrl Pts',(-14.4708415205441,66.4177685482323,
85.2911184942675));
#151197=CARTESIAN_POINT('Ctrl Pts',(-14.4319659731008,66.5264594367093,
85.3655980275366));
#151198=CARTESIAN_POINT('Ctrl Pts',(-14.4035514676782,66.6059026354073,
85.4200358230441));
#151199=CARTESIAN_POINT('Ctrl Pts',(-14.3745022236368,66.688115954453,85.4752521024859));
#151200=CARTESIAN_POINT('Ctrl Pts',(-14.3448376701008,66.7731753463617,
85.53110066904));
#151201=CARTESIAN_POINT('Ctrl Pts',(-14.325471304126,66.8287059752416,85.5675611462807));
#151202=CARTESIAN_POINT('Ctrl Pts',(-14.3058344006169,66.8854493524695,
85.604290692101));
#151203=CARTESIAN_POINT('Ctrl Pts',(-14.2859269601853,66.9434263337528,
85.6412457446482));
#151204=CARTESIAN_POINT('Ctrl Pts',(-14.2834385301313,66.9506734564132,
85.6458651262165));
#151205=CARTESIAN_POINT('Ctrl Pts',(-14.2809458729396,66.9579398553398,
85.6504880293378));
#151206=CARTESIAN_POINT('Ctrl Pts',(-14.2784489886125,66.9652255685214,
85.6551143648198));
#151207=CARTESIAN_POINT('Ctrl Pts',(-14.2759521042853,66.9725112817029,
85.6597407003019));
#151208=CARTESIAN_POINT('Ctrl Pts',(-14.274373726549,66.9771222966787,85.66266251223));
#151209=CARTESIAN_POINT('Ctrl Pts',(-14.2724661389012,66.982699104053,85.6661929182527));
#151210=CARTESIAN_POINT('Ctrl Pts',(-14.2686509636057,66.9938527188015,
85.6732537302981));
#151211=CARTESIAN_POINT('Ctrl Pts',(-14.2648489860863,67.0049889914759,
85.6802829154931));
#151212=CARTESIAN_POINT('Ctrl Pts',(-14.2610602063424,67.0161077555074,
85.6872806562372));
#151213=CARTESIAN_POINT('Ctrl Pts',(-14.2534826468546,67.0383452835705,
85.7012761377256));
#151214=CARTESIAN_POINT('Ctrl Pts',(-14.2459578784689,67.0605127766583,
85.7151458422875));
#151215=CARTESIAN_POINT('Ctrl Pts',(-14.2384859011777,67.0826088746059,
85.7288911974603));
#151216=CARTESIAN_POINT('Ctrl Pts',(-14.2085979920129,67.1709932663963,
85.7838726181511));
#151217=CARTESIAN_POINT('Ctrl Pts',(-14.1795547404069,67.2582351770003,
85.8368647362588));
#151218=CARTESIAN_POINT('Ctrl Pts',(-14.1513561454702,67.3442534426152,
85.8879594938722));
#151219=CARTESIAN_POINT('Ctrl Pts',(-14.1056923780582,67.4835482579436,
85.9707004649337));
#151220=CARTESIAN_POINT('Ctrl Pts',(-14.0622422564733,67.6196323210958,
86.0484664752182));
#151221=CARTESIAN_POINT('Ctrl Pts',(-14.0210093452371,67.7521944444359,
86.1216412289296));
#151222=CARTESIAN_POINT('Ctrl Pts',(-14.0113174104562,67.7833536183898,
86.1388412014592));
#151223=CARTESIAN_POINT('Ctrl Pts',(-14.0017478415776,67.814318384856,86.1557874692341));
#151224=CARTESIAN_POINT('Ctrl Pts',(-13.9923004473294,67.8450850269991,
86.1724849405349));
#151225=CARTESIAN_POINT('Origin',(-15.567536483327,60.0333704529112,86.2553885480113));
#151226=CARTESIAN_POINT('Ctrl Pts',(-10.7041478512869,60.09386358315,60.91310738057));
#151227=CARTESIAN_POINT('Ctrl Pts',(-10.7993782800729,60.52820765429,61.28143633235));
#151228=CARTESIAN_POINT('Ctrl Pts',(-11.1849148787759,61.42183746249,61.97975320377));
#151229=CARTESIAN_POINT('Ctrl Pts',(-12.3843078552048,62.66523363696,62.74337770198));
#151230=CARTESIAN_POINT('Ctrl Pts',(-14.0046199477159,63.57750343472,63.071352235562));
#151231=CARTESIAN_POINT('Ctrl Pts',(-15.1626528546819,63.86437128803,62.97100038631));
#151232=CARTESIAN_POINT('Ctrl Pts',(-15.7241364691869,63.93250661787,62.85729087165));
#151233=CARTESIAN_POINT('Ctrl Pts',(-10.9677003684249,59.23917692104,61.74432861127));
#151234=CARTESIAN_POINT('Ctrl Pts',(-11.0441856921679,59.69432284704,62.07811676378));
#151235=CARTESIAN_POINT('Ctrl Pts',(-11.3853725838149,60.62794654058,62.70918441869));
#151236=CARTESIAN_POINT('Ctrl Pts',(-12.4999814042143,61.92964160607,63.404910218528));
#151237=CARTESIAN_POINT('Ctrl Pts',(-14.0404250630359,62.89957197099,63.720140072344));
#151238=CARTESIAN_POINT('Ctrl Pts',(-15.1678421958939,63.22153762942,63.648738097669));
#151239=CARTESIAN_POINT('Ctrl Pts',(-15.7218484252699,63.30516960111,63.555460526342));
#151240=CARTESIAN_POINT('Ctrl Pts',(-11.3522936220299,58.14048279688,63.112571062291));
#151241=CARTESIAN_POINT('Ctrl Pts',(-11.4036986376439,58.61682481433,63.39382635559));
#151242=CARTESIAN_POINT('Ctrl Pts',(-11.6848368356725,59.58954811192,63.923065828625));
#151243=CARTESIAN_POINT('Ctrl Pts',(-12.6807018187541,60.95041422043,64.511351021118));
#151244=CARTESIAN_POINT('Ctrl Pts',(-14.1030936751889,61.9883845619,64.794328418875));
#151245=CARTESIAN_POINT('Ctrl Pts',(-15.1787465752669,62.36041090115,64.754643608369));
#151246=CARTESIAN_POINT('Ctrl Pts',(-15.7172649246479,62.4683826908,64.686581762677));
#151247=CARTESIAN_POINT('Ctrl Pts',(-11.7927722579713,57.02090553469,65.101174498226));
#151248=CARTESIAN_POINT('Ctrl Pts',(-11.8176818813148,57.5125830774,65.313181016537));
#151249=CARTESIAN_POINT('Ctrl Pts',(-12.0347761979639,58.51132096517,65.710392001923));
#151250=CARTESIAN_POINT('Ctrl Pts',(-12.9001966352731,59.91385972121,66.156294835457));
#151251=CARTESIAN_POINT('Ctrl Pts',(-14.1863686741549,61.01129527967,66.384105820796));
#151252=CARTESIAN_POINT('Ctrl Pts',(-15.1950629340269,61.43683394941,66.371138073743));
#151253=CARTESIAN_POINT('Ctrl Pts',(-15.7105937362879,61.57320926474,66.328753181307));
#151254=CARTESIAN_POINT('Ctrl Pts',(-12.0661314106483,56.37283617372,66.595423337916));
#151255=CARTESIAN_POINT('Ctrl Pts',(-12.075843484741,56.87031895129,66.759479358578));
#151256=CARTESIAN_POINT('Ctrl Pts',(-12.2555688846867,57.87753552955,67.065970272353));
#151257=CARTESIAN_POINT('Ctrl Pts',(-13.0422585423336,59.29546209927,67.41236946592));
#151258=CARTESIAN_POINT('Ctrl Pts',(-14.2430805630419,60.42240614722,67.596288679237));
#151259=CARTESIAN_POINT('Ctrl Pts',(-15.2068409041219,60.87953638865,67.595276586158));
#151260=CARTESIAN_POINT('Ctrl Pts',(-15.7058387404459,61.0336884742,67.567305919008));
#151261=CARTESIAN_POINT('Ctrl Pts',(-12.2840775879579,55.88110902615,68.139369567263));
#151262=CARTESIAN_POINT('Ctrl Pts',(-12.2827124321577,56.38084424396,68.259552190757));
#151263=CARTESIAN_POINT('Ctrl Pts',(-12.4345336551906,57.38982547879,68.483378307406));
#151264=CARTESIAN_POINT('Ctrl Pts',(-13.1600193818491,58.81285577352,68.737117882334));
#151265=CARTESIAN_POINT('Ctrl Pts',(-14.2920472090019,59.95780874927,68.875104868816));
#151266=CARTESIAN_POINT('Ctrl Pts',(-15.2174560511339,60.43844112166,68.878748123676));
#151267=CARTESIAN_POINT('Ctrl Pts',(-15.7015914388329,60.60654655031,68.86065654605));
#151268=CARTESIAN_POINT('Ctrl Pts',(-12.4455223641968,55.53147356831,69.729584462491));
#151269=CARTESIAN_POINT('Ctrl Pts',(-12.4364409723155,56.03153659582,69.808270714192));
#151270=CARTESIAN_POINT('Ctrl Pts',(-12.5684953465757,57.03906368193,69.954444991214));
#151271=CARTESIAN_POINT('Ctrl Pts',(-13.2494610073255,58.46199397327,70.120458107449));
#151272=CARTESIAN_POINT('Ctrl Pts',(-14.3302328652479,59.61727660643,70.212240577407));
#151273=CARTESIAN_POINT('Ctrl Pts',(-15.2259605578979,60.11434751671,70.216671992981));
#151274=CARTESIAN_POINT('Ctrl Pts',(-15.6982072375269,60.29264234042,70.205961262777));
#151275=CARTESIAN_POINT('Ctrl Pts',(-12.5457498999138,55.32390979008,71.345733821343));
#151276=CARTESIAN_POINT('Ctrl Pts',(-12.5323125837535,55.8230599579,71.384509154805));
#151277=CARTESIAN_POINT('Ctrl Pts',(-12.6528329390118,56.82750771549,71.456441367017));
#151278=CARTESIAN_POINT('Ctrl Pts',(-13.3066685414157,58.24764282185,71.538286506703));
#151279=CARTESIAN_POINT('Ctrl Pts',(-14.3552787532329,59.40754337175,71.584076966819));
#151280=CARTESIAN_POINT('Ctrl Pts',(-15.2316755631129,59.91449324558,71.586996148855));
#151281=CARTESIAN_POINT('Ctrl Pts',(-15.6959440082919,60.09919481949,71.582126108352));
#151282=CARTESIAN_POINT('Ctrl Pts',(-12.5810013147727,55.25465453145,72.9682049875124));
#151283=CARTESIAN_POINT('Ctrl Pts',(-12.5662393202886,55.75295766121,72.9686809528089));
#151284=CARTESIAN_POINT('Ctrl Pts',(-12.6830375165265,56.75533192763,72.9695652327033));
#151285=CARTESIAN_POINT('Ctrl Pts',(-13.3275136480546,58.17334349544,72.9705789955397));
#151286=CARTESIAN_POINT('Ctrl Pts',(-14.3646256854689,59.33424330126,72.9711581432487));
#151287=CARTESIAN_POINT('Ctrl Pts',(-15.2338545192429,59.84467210232,72.971209319932));
#151288=CARTESIAN_POINT('Ctrl Pts',(-15.6950847124779,60.03173379517,72.9711575988109));
#151289=CARTESIAN_POINT('Ctrl Pts',(-12.5475045162957,55.32017430334,74.590690933763));
#151290=CARTESIAN_POINT('Ctrl Pts',(-12.533981149037,55.81932730129,74.55291642949));
#151291=CARTESIAN_POINT('Ctrl Pts',(-12.6542839686069,56.82375706031,74.482838228714));
#151292=CARTESIAN_POINT('Ctrl Pts',(-13.3076377377342,58.2438840296,74.403081923287));
#151293=CARTESIAN_POINT('Ctrl Pts',(-14.3556951419809,59.4038845339,74.358425507288));
#151294=CARTESIAN_POINT('Ctrl Pts',(-15.2317691498149,59.91100278183,74.355537412367));
#151295=CARTESIAN_POINT('Ctrl Pts',(-15.6959068347229,60.09581045991,74.360258574239));
#151296=CARTESIAN_POINT('Ctrl Pts',(-12.415890569498,55.59282803409,76.748377568762));
#151297=CARTESIAN_POINT('Ctrl Pts',(-12.4081109279239,56.09315502217,76.657403775015));
#151298=CARTESIAN_POINT('Ctrl Pts',(-12.5435994725054,57.10157402003,76.488382653225));
#151299=CARTESIAN_POINT('Ctrl Pts',(-13.2325997356438,58.52529383771,76.296485974051));
#151300=CARTESIAN_POINT('Ctrl Pts',(-14.3228650735109,59.67918060652,76.190569027371));
#151301=CARTESIAN_POINT('Ctrl Pts',(-15.2242815937599,60.17332252705,76.185676184442));
#151302=CARTESIAN_POINT('Ctrl Pts',(-15.6988723085229,60.34972220064,76.198183493317));
#151303=CARTESIAN_POINT('Ctrl Pts',(-12.0984815213201,56.28453201345,79.379282177917));
#151304=CARTESIAN_POINT('Ctrl Pts',(-12.1059032952047,56.78383432926,79.217993773868));
#151305=CARTESIAN_POINT('Ctrl Pts',(-12.2803121570303,57.79442431143,78.916961042675));
#151306=CARTESIAN_POINT('Ctrl Pts',(-13.0569396205545,59.21756273984,78.575716119718));
#151307=CARTESIAN_POINT('Ctrl Pts',(-14.2480069695869,60.35063110239,78.391769330457));
#151308=CARTESIAN_POINT('Ctrl Pts',(-15.2076486671689,60.8123315191,78.389193997522));
#151309=CARTESIAN_POINT('Ctrl Pts',(-15.7054941595619,60.96870853934,78.414798392491));
#151310=CARTESIAN_POINT('Ctrl Pts',(-11.4801382308999,57.77429967397,82.410149750697));
#151311=CARTESIAN_POINT('Ctrl Pts',(-11.5230945717699,58.25793556694,82.146393216678));
#151312=CARTESIAN_POINT('Ctrl Pts',(-11.7841034131413,59.24408794519,81.651018262809));
#151313=CARTESIAN_POINT('Ctrl Pts',(-12.7404495534974,60.62500522955,81.098302707073));
#151314=CARTESIAN_POINT('Ctrl Pts',(-14.1237202044259,61.68566477043,80.825785486714));
#151315=CARTESIAN_POINT('Ctrl Pts',(-15.1823110544289,62.07418257557,80.85469887249));
#151316=CARTESIAN_POINT('Ctrl Pts',(-15.7157641330979,62.19013200718,80.914252246577));
#151317=CARTESIAN_POINT('Ctrl Pts',(-10.9713079387719,59.22776230562,84.2218583444));
#151318=CARTESIAN_POINT('Ctrl Pts',(-11.0475501095389,59.68314485841,83.88853398117));
#151319=CARTESIAN_POINT('Ctrl Pts',(-11.3881525214289,60.61722479436,83.25836777774));
#151320=CARTESIAN_POINT('Ctrl Pts',(-12.5016155027486,61.91961304936,82.56355185095));
#151321=CARTESIAN_POINT('Ctrl Pts',(-14.0409546878519,62.89027630592,82.248495693581));
#151322=CARTESIAN_POINT('Ctrl Pts',(-15.1679259362809,63.21272241284,82.319513523069));
#151323=CARTESIAN_POINT('Ctrl Pts',(-15.7218123616379,63.29657498626,82.412519105935));
#151324=CARTESIAN_POINT('Ctrl Pts',(-10.7040595554349,60.09411427919,85.06497750449));
#151325=CARTESIAN_POINT('Ctrl Pts',(-10.7992944412079,60.52845915508,84.69663916139));
#151326=CARTESIAN_POINT('Ctrl Pts',(-11.1848427857669,61.42209035944,83.99830481448));
#151327=CARTESIAN_POINT('Ctrl Pts',(-12.3842618607212,62.66548448627,83.23466499336));
#151328=CARTESIAN_POINT('Ctrl Pts',(-14.0046020364719,63.5777452831,82.906691022993));
#151329=CARTESIAN_POINT('Ctrl Pts',(-15.1626491571459,63.86460259476,83.00705348714));
#151330=CARTESIAN_POINT('Ctrl Pts',(-15.7241379640389,63.9327320353,83.12076992282));
#151331=CARTESIAN_POINT('Ctrl Pts',(-15.5675364833309,63.77502783968,63.039015015514));
#151332=CARTESIAN_POINT('Ctrl Pts',(-15.5675364833366,63.1966588570052,
63.6915032265959));
#151333=CARTESIAN_POINT('Ctrl Pts',(-15.5675364833221,62.4022926946241,
64.7657142192389));
#151334=CARTESIAN_POINT('Ctrl Pts',(-15.5675364833146,61.5332281582025,
66.3395724687636));
#151335=CARTESIAN_POINT('Ctrl Pts',(-15.5675364833362,60.9888173218726,
67.574344511651));
#151336=CARTESIAN_POINT('Ctrl Pts',(-15.5675364833589,60.5578543920014,
68.8651514730108));
#151337=CARTESIAN_POINT('Ctrl Pts',(-15.567536483356,60.2411695586609,70.2085918635667));
#151338=CARTESIAN_POINT('Ctrl Pts',(-15.5675364833459,60.0459797863666,
71.5833100686918));
#151339=CARTESIAN_POINT('Ctrl Pts',(-15.5675364833335,59.9778791011265,
72.9711699015529));
#151340=CARTESIAN_POINT('Ctrl Pts',(-15.5675364833356,60.0425665085272,
74.3591115894978));
#151341=CARTESIAN_POINT('Ctrl Pts',(-15.5675364833536,60.2987648763767,
76.1951078607713));
#151342=CARTESIAN_POINT('Ctrl Pts',(-15.5675364833368,60.9232171254913,
78.4084022555666));
#151343=CARTESIAN_POINT('Ctrl Pts',(-15.5675364833127,62.1248654345252,
80.8364426677163));
#151344=CARTESIAN_POINT('Ctrl Pts',(-15.5675364833367,63.188677426801,82.277271278915));
#151345=CARTESIAN_POINT('Ctrl Pts',(-15.5675364833309,63.77502783968,82.938763757646));
#151346=CARTESIAN_POINT('Origin',(-15.5675364833309,75.,72.98888938658));
#151347=CARTESIAN_POINT('Origin',(-15.5675364833309,75.,72.98888938658));
#151348=CARTESIAN_POINT('Origin',(-15.5675364833309,75.,72.98888938658));
#151349=CARTESIAN_POINT('Origin',(-15.5675364833309,75.,72.98888938658));
#151350=CARTESIAN_POINT('Origin',(-15.5675364833309,75.,72.98888938658));
#151351=CARTESIAN_POINT('Origin',(27.4324635166691,25.,72.98888938658));
#151352=CARTESIAN_POINT('Origin',(-2.02513312664091,-92.,60.48888938658));
#151353=CARTESIAN_POINT('',(1.02913961852909,-92.5,53.63896836527));
#151354=CARTESIAN_POINT('Origin',(-2.02513312664091,-92.5,60.48888938658));
#151355=CARTESIAN_POINT('Origin',(1.02913961852909,-92.,53.63896836527));
#151356=CARTESIAN_POINT('Origin',(-10.9843331791359,-92.,80.581991049076));
#151357=CARTESIAN_POINT('Origin',(-10.9843331791359,-92.5,80.581991049076));
#151358=CARTESIAN_POINT('Origin',(-10.9843331791359,-92.,80.581991049076));
#151359=CARTESIAN_POINT('Origin',(-10.9843331791359,-92.,65.395787724084));
#151360=CARTESIAN_POINT('Origin',(-10.9843331791359,-92.,65.395787724084));
#151361=CARTESIAN_POINT('',(1.02913961852909,-92.5,92.33881040789));
#151362=CARTESIAN_POINT('Origin',(1.02913961852909,-92.,92.33881040789));
#151363=CARTESIAN_POINT('Origin',(-10.9843331791359,-92.5,65.395787724084));
#151364=CARTESIAN_POINT('Origin',(-2.27593483123091,-92.5,69.192338555332));
#151365=CARTESIAN_POINT('Origin',(-2.02513312664091,-92.5,85.48888938658));
#151366=CARTESIAN_POINT('Origin',(-2.02513312664091,-92.,85.48888938658));
#151367=CARTESIAN_POINT('Origin',(-10.9843331791359,-92.5,65.395787724084));
#151368=CARTESIAN_POINT('Ctrl Pts',(16.5158721297058,-26.62691877498,77.3848956129786));
#151369=CARTESIAN_POINT('Ctrl Pts',(16.3820322875788,-26.7011776840352,
77.6918928617402));
#151370=CARTESIAN_POINT('Ctrl Pts',(16.2459288731422,-26.7722083172181,
77.990054798336));
#151371=CARTESIAN_POINT('Ctrl Pts',(16.1082781307409,-26.8400106745286,
78.2795143748608));
#151372=CARTESIAN_POINT('Ctrl Pts',(15.9688840103591,-26.9086717641257,
78.5726400228005));
#151373=CARTESIAN_POINT('Ctrl Pts',(15.8279032167025,-26.9740222863118,
78.8568417897912));
#151374=CARTESIAN_POINT('Ctrl Pts',(15.6860353899346,-27.0360622410872,
79.1322880203727));
#151375=CARTESIAN_POINT('Ctrl Pts',(15.5414909720178,-27.0992726909465,
79.4129310384115));
#151376=CARTESIAN_POINT('Ctrl Pts',(15.396025859127,-27.1590464753882,79.6844853256324));
#151377=CARTESIAN_POINT('Ctrl Pts',(15.2503327146554,-27.2153835944122,
79.9471555443661));
#151378=CARTESIAN_POINT('Ctrl Pts',(15.1031356263789,-27.2723022635252,
80.2125372238871));
#151379=CARTESIAN_POINT('Ctrl Pts',(14.9557058104529,-27.3257129498178,
80.4688508172432));
#151380=CARTESIAN_POINT('Ctrl Pts',(14.8087086118992,-27.3756156532902,
80.7163293321968));
#151381=CARTESIAN_POINT('Ctrl Pts',(14.6595141442981,-27.4262642870715,
80.9675070801029));
#151382=CARTESIAN_POINT('Ctrl Pts',(14.5107653761148,-27.4732992817285,
81.2095839839924));
#151383=CARTESIAN_POINT('Ctrl Pts',(14.3631070011745,-27.5167206372612,
81.4428209796608));
#151384=CARTESIAN_POINT('Ctrl Pts',(14.2912166810056,-27.5378611594474,
81.5563768975056));
#151385=CARTESIAN_POINT('Ctrl Pts',(14.2195840629412,-27.5581450986431,
81.667837615716));
#151386=CARTESIAN_POINT('Ctrl Pts',(14.148279236274,-27.5775724548482,81.7772343383726));
#151387=CARTESIAN_POINT('Ctrl Pts',(14.0923156340326,-27.5928200178265,
81.8630943700058));
#151388=CARTESIAN_POINT('Ctrl Pts',(14.0365538920273,-27.6075399344871,
81.9476830161932));
#151389=CARTESIAN_POINT('Ctrl Pts',(13.9810266940025,-27.62173220483,82.0310155976267));
#151390=CARTESIAN_POINT('Ctrl Pts',(13.9532630949901,-27.6288283400015,
82.0726818883434));
#151391=CARTESIAN_POINT('Ctrl Pts',(13.9255581219713,-27.6357925635935,
82.1140341561832));
#151392=CARTESIAN_POINT('Ctrl Pts',(13.8979157551414,-27.6426248756062,
82.1550743429307));
#151393=CARTESIAN_POINT('Ctrl Pts',(13.8840945717265,-27.6460410316125,
82.1755944363045));
#151394=CARTESIAN_POINT('Ctrl Pts',(13.8702890392204,-27.649424209724,82.196036508983));
#151395=CARTESIAN_POINT('Ctrl Pts',(13.8564996502144,-27.6527744099406,
82.2164008028118));
#151396=CARTESIAN_POINT('Ctrl Pts',(13.84615760846,-27.6552870601031,82.2316740231835));
#151397=CARTESIAN_POINT('Ctrl Pts',(13.8358246473727,-27.6577811601997,
82.2469034929172));
#151398=CARTESIAN_POINT('Ctrl Pts',(13.8255009733157,-27.6602567102304,
82.2620893141732));
#151399=CARTESIAN_POINT('Ctrl Pts',(13.8220597486301,-27.661081893574,82.2671512545919));
#151400=CARTESIAN_POINT('Ctrl Pts',(13.8196814399517,-27.6616515023092,
82.2706483977758));
#151401=CARTESIAN_POINT('Ctrl Pts',(13.8151804024935,-27.6627260769059,
82.2772605897607));
#151402=CARTESIAN_POINT('Ctrl Pts',(13.5932909459714,-27.7156998136198,
82.6032244813254));
#151403=CARTESIAN_POINT('Ctrl Pts',(13.3682551472339,-27.7624240386982,
82.9199960935799));
#151404=CARTESIAN_POINT('Ctrl Pts',(13.1407961930566,-27.8028987521411,
83.2277290871262));
#151405=CARTESIAN_POINT('Ctrl Pts',(12.9110186606534,-27.8437860401939,
83.5385989236287));
#151406=CARTESIAN_POINT('Ctrl Pts',(12.6787684254416,-27.8782957598135,
83.8402451995739));
#151407=CARTESIAN_POINT('Ctrl Pts',(12.4447515029891,-27.906427911,84.1328630283522));
#151408=CARTESIAN_POINT('Ctrl Pts',(12.2067799972796,-27.9350354591488,
84.4304257198962));
#151409=CARTESIAN_POINT('Ctrl Pts',(11.9669817217329,-27.9570480723335,
84.7186524906363));
#151410=CARTESIAN_POINT('Ctrl Pts',(11.7260565705287,-27.9724657505541,
84.9977824546804));
#151411=CARTESIAN_POINT('Ctrl Pts',(11.5250001554144,-27.9853320830931,
85.2307214801047));
#151412=CARTESIAN_POINT('Ctrl Pts',(11.3231581995199,-27.993605567279,85.4573259977147));
#151413=CARTESIAN_POINT('Ctrl Pts',(11.1209145922133,-27.9972862031118,
85.6777506706842));
#151414=CARTESIAN_POINT('Ctrl Pts',(10.9677766773297,-28.0000731633742,
85.8446552035739));
#151415=CARTESIAN_POINT('Ctrl Pts',(10.8144080517589,-28.0002268380673,
86.008016856321));
#151416=CARTESIAN_POINT('Ctrl Pts',(10.6609674346233,-27.9977472271911,
86.1679075326157));
#151417=CARTESIAN_POINT('Ctrl Pts',(10.5842471260555,-27.996507421753,86.247852870763));
#151418=CARTESIAN_POINT('Ctrl Pts',(10.5075087946992,-27.9946092949226,
86.3269304407219));
#151419=CARTESIAN_POINT('Ctrl Pts',(10.4307715507466,-27.9920528466999,
86.4051496708011));
#151420=CARTESIAN_POINT('Ctrl Pts',(10.3924029287703,-27.9907746225885,
86.4442592858407));
#151421=CARTESIAN_POINT('Ctrl Pts',(10.3540345768555,-27.9893318181291,
86.4831543142134));
#151422=CARTESIAN_POINT('Ctrl Pts',(10.3156688587493,-27.9877244333215,
86.5218359391688));
#151423=CARTESIAN_POINT('Ctrl Pts',(10.2964859996962,-27.9869207409178,
86.5411767516465));
#151424=CARTESIAN_POINT('Ctrl Pts',(10.27730379899,-27.986075903427,86.5604642131652));
#151425=CARTESIAN_POINT('Ctrl Pts',(10.258122549549,-27.9851899208492,86.5796984729251));
#151426=CARTESIAN_POINT('Ctrl Pts',(10.2485319248285,-27.9847469295603,
86.589315602805));
#151427=CARTESIAN_POINT('Ctrl Pts',(10.2389415379176,-27.9842936519996,
86.5989194322384));
#151428=CARTESIAN_POINT('Ctrl Pts',(10.2293514252671,-27.9838300881672,
86.6085099799595));
#151429=CARTESIAN_POINT('Ctrl Pts',(10.2197613126166,-27.9833665243348,
86.6181005276805));
#151430=CARTESIAN_POINT('Ctrl Pts',(10.2117549429593,-27.9829726171462,
86.6260985397174));
#151431=CARTESIAN_POINT('Ctrl Pts',(10.2005819464838,-27.9824085378547,
86.6372417967291));
#151432=CARTESIAN_POINT('Ctrl Pts',(9.90016413482943,-27.9672416605789,
86.9368599782508));
#151433=CARTESIAN_POINT('Ctrl Pts',(9.59694061001989,-27.9419657850838,
87.2265639041723));
#151434=CARTESIAN_POINT('Ctrl Pts',(9.29161323374535,-27.9065809113692,
87.5065542657932));
#151435=CARTESIAN_POINT('Ctrl Pts',(8.98304848127122,-27.8708208529943,
87.7895133560748));
#151436=CARTESIAN_POINT('Ctrl Pts',(8.67233513464827,-27.8247362891609,
88.0625520408413));
#151437=CARTESIAN_POINT('Ctrl Pts',(8.36015795388373,-27.7683272198691,
88.3259133845449));
#151438=CARTESIAN_POINT('Ctrl Pts',(8.03290934727259,-27.7091948089709,
88.6019894018603));
#151439=CARTESIAN_POINT('Ctrl Pts',(7.70405253396476,-27.6387169262424,
88.867431165492));
#151440=CARTESIAN_POINT('Ctrl Pts',(7.37432879336558,-27.5568935716835,
89.1225559528047));
#151441=CARTESIAN_POINT('Ctrl Pts',(7.05118518470879,-27.4767031249279,
89.3725893422118));
#151442=CARTESIAN_POINT('Ctrl Pts',(6.72720874293467,-27.3856155196975,
89.6127138586078));
#151443=CARTESIAN_POINT('Ctrl Pts',(6.40305184743187,-27.2836307559925,
89.8432587985712));
#151444=CARTESIAN_POINT('Ctrl Pts',(6.06899380386998,-27.1785309382527,
90.0808455741904));
#151445=CARTESIAN_POINT('Ctrl Pts',(5.73474432538952,-27.0618581031527,
90.3082588254074));
#151446=CARTESIAN_POINT('Ctrl Pts',(5.40096780733715,-26.9336122506926,
90.5258874370315));
#151447=CARTESIAN_POINT('Ctrl Pts',(5.06719128928478,-26.8053663982324,
90.7435160486557));
#151448=CARTESIAN_POINT('Ctrl Pts',(4.73388767236532,-26.665547528412,90.9513603482028));
#151449=CARTESIAN_POINT('Ctrl Pts',(4.40167170800331,-26.5141556412314,
91.1498331075365));
#151450=CARTESIAN_POINT('Ctrl Pts',(4.3554809349335,-26.4931063568637,91.177428440604));
#151451=CARTESIAN_POINT('Ctrl Pts',(4.30931424153723,-26.4718422337862,
91.2048467869842));
#151452=CARTESIAN_POINT('Ctrl Pts',(4.26073795147533,-26.4492073398415,
91.2335083321911));
#151453=CARTESIAN_POINT('Ctrl Pts',(4.21216166141343,-26.4265724458968,
91.2621698773981));
#151454=CARTESIAN_POINT('Ctrl Pts',(4.16359850258958,-26.403687164881,91.2906389948733));
#151455=CARTESIAN_POINT('Ctrl Pts',(4.11505021502293,-26.3805514967941,
91.3189168005709));
#151456=CARTESIAN_POINT('Ctrl Pts',(3.92085706475633,-26.2880088244464,
91.4320280233613));
#151457=CARTESIAN_POINT('Ctrl Pts',(3.72690188042819,-26.1914599589606,
91.542078301748));
#151458=CARTESIAN_POINT('Ctrl Pts',(3.53329053955223,-26.0909049003369,
91.6491418252762));
#151459=CARTESIAN_POINT('Ctrl Pts',(3.18566624854605,-25.9103608226863,
91.8413716879006));
#151460=CARTESIAN_POINT('Ctrl Pts',(2.83915323135102,-25.7169018604478,
92.0239720877067));
#151461=CARTESIAN_POINT('Ctrl Pts',(2.49432560190691,-25.5105280136215,
92.1973876290191));
#151462=CARTESIAN_POINT('Ctrl Pts',(2.14463366168432,-25.3012429542303,
92.3732494565764));
#151463=CARTESIAN_POINT('Ctrl Pts',(1.79667501169128,-25.0786760726497,
92.5396657319217));
#151464=CARTESIAN_POINT('Ctrl Pts',(1.45099749566678,-24.8428273688797,
92.6971164647939));
#151465=CARTESIAN_POINT('Ctrl Pts',(1.37814818263882,-24.7931237715912,
92.7302981939888));
#151466=CARTESIAN_POINT('Ctrl Pts',(1.30540000319713,-24.7428302907079,
92.7630817867072));
#151467=CARTESIAN_POINT('Ctrl Pts',(1.23275780153721,-24.69194692623,92.7954718093058));
#151468=CARTESIAN_POINT('Ctrl Pts',(21.0098527486291,-19.89566736418,80.408148930172));
#151469=CARTESIAN_POINT('Ctrl Pts',(20.6551365913091,-19.99124366319,80.237482208311));
#151470=CARTESIAN_POINT('Ctrl Pts',(19.9910149156791,-20.23867708484,79.904460322262));
#151471=CARTESIAN_POINT('Ctrl Pts',(19.0648609531091,-20.80248074526,79.396961278566));
#151472=CARTESIAN_POINT('Ctrl Pts',(18.2673560862191,-21.51326965896,78.915583888499));
#151473=CARTESIAN_POINT('Ctrl Pts',(17.5939479981591,-22.37888325624,78.456835314244));
#151474=CARTESIAN_POINT('Ctrl Pts',(17.0765716352991,-23.36518757691,78.041108570563));
#151475=CARTESIAN_POINT('Ctrl Pts',(16.7338537221591,-24.42774757018,77.685128810774));
#151476=CARTESIAN_POINT('Ctrl Pts',(16.5606913794591,-25.57344706162,77.385356055912));
#151477=CARTESIAN_POINT('Ctrl Pts',(16.5711618237791,-26.34223932515,77.238423393511));
#151478=CARTESIAN_POINT('Ctrl Pts',(16.6081249192391,-26.74041077153,77.175825765138));
#151479=CARTESIAN_POINT('Ctrl Pts',(20.3926287521091,-20.2277816629,82.564474719442));
#151480=CARTESIAN_POINT('Ctrl Pts',(20.0304495599191,-20.3062712552,82.36756185427));
#151481=CARTESIAN_POINT('Ctrl Pts',(19.3485196483991,-20.52646386931,81.983339277436));
#151482=CARTESIAN_POINT('Ctrl Pts',(18.3896783510891,-21.06856485919,81.399520311364));
#151483=CARTESIAN_POINT('Ctrl Pts',(17.5596258339291,-21.77713325838,80.849001012762));
#151484=CARTESIAN_POINT('Ctrl Pts',(16.8570714683491,-22.65858032904,80.329679945766));
#151485=CARTESIAN_POINT('Ctrl Pts',(16.3180571926391,-23.67552873337,79.866533429259));
#151486=CARTESIAN_POINT('Ctrl Pts',(15.9635459865691,-24.77815848302,79.479434494296));
#151487=CARTESIAN_POINT('Ctrl Pts',(15.7884768001891,-25.96937000168,79.165303624673));
#151488=CARTESIAN_POINT('Ctrl Pts',(15.8039654328291,-26.76746529055,79.021363678754));
#151489=CARTESIAN_POINT('Ctrl Pts',(15.8446902264591,-27.17980945688,78.963423318945));
#151490=CARTESIAN_POINT('Ctrl Pts',(18.8791778988491,-20.81222181939,86.54683680967));
#151491=CARTESIAN_POINT('Ctrl Pts',(18.5090651864891,-20.85157100999,86.29682420477));
#151492=CARTESIAN_POINT('Ctrl Pts',(17.8026752686791,-21.00753396259,85.80852977002));
#151493=CARTESIAN_POINT('Ctrl Pts',(16.7884714733291,-21.49368110695,85.06979054407));
#151494=CARTESIAN_POINT('Ctrl Pts',(15.8973287740491,-22.18943159807,84.38083918167));
#151495=CARTESIAN_POINT('Ctrl Pts',(15.1358035389891,-23.09873073241,83.74432372475));
#151496=CARTESIAN_POINT('Ctrl Pts',(14.5492421568691,-24.17733474,83.19601594835));
#151497=CARTESIAN_POINT('Ctrl Pts',(14.1640926878391,-25.36315201507,82.76265760696));
#151498=CARTESIAN_POINT('Ctrl Pts',(13.9751991718891,-26.64940096258,82.442431434339));
#151499=CARTESIAN_POINT('Ctrl Pts',(13.9919355575191,-27.50824023846,82.322766335322));
#151500=CARTESIAN_POINT('Ctrl Pts',(14.0349062209691,-27.94970483338,82.28413504845));
#151501=CARTESIAN_POINT('Ctrl Pts',(16.1824725435691,-21.09209438161,90.98689436045));
#151502=CARTESIAN_POINT('Ctrl Pts',(15.8353920940991,-21.07651442269,90.66407951446));
#151503=CARTESIAN_POINT('Ctrl Pts',(15.1562212037291,-21.13655542109,90.03216892887));
#151504=CARTESIAN_POINT('Ctrl Pts',(14.1357975968091,-21.52378539238,89.08090920936));
#151505=CARTESIAN_POINT('Ctrl Pts',(13.2024016538491,-22.17634380389,88.20804330743));
#151506=CARTESIAN_POINT('Ctrl Pts',(12.3725625246191,-23.09809302245,87.42817780739));
#151507=CARTESIAN_POINT('Ctrl Pts',(11.7042631277791,-24.23734882118,86.79534712921));
#151508=CARTESIAN_POINT('Ctrl Pts',(11.2345903778791,-25.51470352118,86.3450307177));
#151509=CARTESIAN_POINT('Ctrl Pts',(10.9601647413791,-26.90758355909,86.07493152895));
#151510=CARTESIAN_POINT('Ctrl Pts',(10.9217922244791,-27.83312706015,86.02981874014));
#151511=CARTESIAN_POINT('Ctrl Pts',(10.9358081186491,-28.30574486146,86.03831960593));
#151512=CARTESIAN_POINT('Ctrl Pts',(13.6800125517991,-20.85160484736,93.96864121737));
#151513=CARTESIAN_POINT('Ctrl Pts',(13.3756529423391,-20.80305713171,93.5913417542));
#151514=CARTESIAN_POINT('Ctrl Pts',(12.7642912235491,-20.80264803255,92.85220100697));
#151515=CARTESIAN_POINT('Ctrl Pts',(11.7975700778191,-21.1189877902,91.74412056314));
#151516=CARTESIAN_POINT('Ctrl Pts',(10.8695342697591,-21.72973149919,90.73881456859));
#151517=CARTESIAN_POINT('Ctrl Pts',(10.0003460674491,-22.64000762359,89.86134820672));
#151518=CARTESIAN_POINT('Ctrl Pts',(9.25501270070909,-23.79502260284,89.1797656491));
#151519=CARTESIAN_POINT('Ctrl Pts',(8.68104170661909,-25.10559524195,88.73467241033));
#151520=CARTESIAN_POINT('Ctrl Pts',(8.27959754217909,-26.5389182176,88.52152852489));
#151521=CARTESIAN_POINT('Ctrl Pts',(8.14849243932909,-27.48840466516,88.54361140251));
#151522=CARTESIAN_POINT('Ctrl Pts',(8.11278288879909,-27.97136651022,88.59242893348));
#151523=CARTESIAN_POINT('Ctrl Pts',(11.6467057389891,-20.40077118403,95.93019164297));
#151524=CARTESIAN_POINT('Ctrl Pts',(11.3836934115591,-20.33562680778,95.51624099247));
#151525=CARTESIAN_POINT('Ctrl Pts',(10.8414362027591,-20.30310783194,94.70537766303));
#151526=CARTESIAN_POINT('Ctrl Pts',(9.93982085948909,-20.57626855614,93.49370810764));
#151527=CARTESIAN_POINT('Ctrl Pts',(9.03357187753909,-21.154608245,92.40231734157));
#151528=CARTESIAN_POINT('Ctrl Pts',(8.14288801602909,-22.044239404,91.46324854709));
#151529=CARTESIAN_POINT('Ctrl Pts',(7.33588463937909,-23.18976034117,90.75351553684));
#151530=CARTESIAN_POINT('Ctrl Pts',(6.66829790515909,-24.49809298253,90.31643495592));
#151531=CARTESIAN_POINT('Ctrl Pts',(6.14617826714909,-25.93133038039,90.14535398219));
#151532=CARTESIAN_POINT('Ctrl Pts',(5.92435902304909,-26.87930744686,90.21408009388));
#151533=CARTESIAN_POINT('Ctrl Pts',(5.83988198614909,-27.36055233645,90.29044282441));
#151534=CARTESIAN_POINT('Ctrl Pts',(9.48566925591909,-19.63589615636,97.59555314433));
#151535=CARTESIAN_POINT('Ctrl Pts',(9.27098750755909,-19.56575558261,97.15206697347));
#151536=CARTESIAN_POINT('Ctrl Pts',(8.81191716525909,-19.52082184909,96.28422750364));
#151537=CARTESIAN_POINT('Ctrl Pts',(7.99590436653909,-19.76818182049,94.99225672571));
#151538=CARTESIAN_POINT('Ctrl Pts',(7.12739780805909,-20.31659507032,93.83549487305));
#151539=CARTESIAN_POINT('Ctrl Pts',(6.22388368237909,-21.1725135457,92.85056839143));
#151540=CARTESIAN_POINT('Ctrl Pts',(5.35392344615909,-22.28183405455,92.12050954926));
#151541=CARTESIAN_POINT('Ctrl Pts',(4.58102981613909,-23.55235799666,91.69007777815));
#151542=CARTESIAN_POINT('Ctrl Pts',(3.91698303326909,-24.94497669681,91.55079655694));
#151543=CARTESIAN_POINT('Ctrl Pts',(3.58588420224909,-25.86529397632,91.65444864575));
#151544=CARTESIAN_POINT('Ctrl Pts',(3.44241434770909,-26.33204745337,91.75144897014));
#151545=CARTESIAN_POINT('Ctrl Pts',(8.00926134120909,-18.89711948749,98.48664285459));
#151546=CARTESIAN_POINT('Ctrl Pts',(7.82700873851909,-18.8309347938,98.02954612217));
#151547=CARTESIAN_POINT('Ctrl Pts',(7.42454263933909,-18.79011314066,97.13635843924));
#151548=CARTESIAN_POINT('Ctrl Pts',(6.66936590663908,-19.03092176508,95.81070161864));
#151549=CARTESIAN_POINT('Ctrl Pts',(5.83078526668909,-19.5601301908,94.62764699397));
#151550=CARTESIAN_POINT('Ctrl Pts',(4.92330275591909,-20.38384396178,93.62454790876));
#151551=CARTESIAN_POINT('Ctrl Pts',(4.01417257721909,-21.45015830713,92.88584223434));
#151552=CARTESIAN_POINT('Ctrl Pts',(3.17092794726909,-22.67084984203,92.45640650951));
#151553=CARTESIAN_POINT('Ctrl Pts',(2.40874601918909,-24.00878867259,92.32715669325));
#151554=CARTESIAN_POINT('Ctrl Pts',(2.00040163275909,-24.89318394035,92.44279977495));
#151555=CARTESIAN_POINT('Ctrl Pts',(1.81495250691909,-25.34182018804,92.54714379559));
#151556=CARTESIAN_POINT('Ctrl Pts',(7.24274295347909,-18.44807871483,98.89217210658));
#151557=CARTESIAN_POINT('Ctrl Pts',(7.07635687067909,-18.3857964445,98.429970603));
#151558=CARTESIAN_POINT('Ctrl Pts',(6.70163711703909,-18.35020608194,97.52763951722));
#151559=CARTESIAN_POINT('Ctrl Pts',(5.97659597624909,-18.59015319315,96.19061261638));
#151560=CARTESIAN_POINT('Ctrl Pts',(5.15326941421909,-19.1093773468,94.99905242918));
#151561=CARTESIAN_POINT('Ctrl Pts',(4.24452036201909,-19.91366910359,93.98998241731));
#151562=CARTESIAN_POINT('Ctrl Pts',(3.31659813599909,-20.95258803845,93.247814414));
#151563=CARTESIAN_POINT('Ctrl Pts',(2.43861741667909,-22.14079466069,92.81729138984));
#151564=CARTESIAN_POINT('Ctrl Pts',(1.62712657436909,-23.44283258147,92.68923465246));
#151565=CARTESIAN_POINT('Ctrl Pts',(1.17940863797909,-24.30369856826,92.80726391985));
#151566=CARTESIAN_POINT('Ctrl Pts',(0.972428646019088,-24.74052533156,92.9132664501));
#151567=CARTESIAN_POINT('Ctrl Pts',(7.33390977282909,-18.51896019696,98.61558102691));
#151568=CARTESIAN_POINT('Ctrl Pts',(7.17927099155909,-18.47494133476,98.21269615893));
#151569=CARTESIAN_POINT('Ctrl Pts',(6.81839532782909,-18.45454687724,97.3773696126));
#151570=CARTESIAN_POINT('Ctrl Pts',(6.12341626982909,-18.68273930707,96.10938806091));
#151571=CARTESIAN_POINT('Ctrl Pts',(5.29685182923909,-19.20408022183,94.9197080813));
#151572=CARTESIAN_POINT('Ctrl Pts',(4.38838335134909,-20.01244945753,93.91195584547));
#151573=CARTESIAN_POINT('Ctrl Pts',(3.46446828778909,-21.05710096399,93.17053740908));
#151574=CARTESIAN_POINT('Ctrl Pts',(2.59387851028909,-22.2520961092,92.74022114186));
#151575=CARTESIAN_POINT('Ctrl Pts',(1.83141007716909,-23.49861933641,92.61802875499));
#151576=CARTESIAN_POINT('Ctrl Pts',(1.41597523797909,-24.30522867552,92.71377801739));
#151577=CARTESIAN_POINT('Ctrl Pts',(1.23275780153909,-24.69194692623,92.79547180931));
#151578=CARTESIAN_POINT('Ctrl Pts',(20.8003130810766,-19.9701890920257,
80.5583314865116));
#151579=CARTESIAN_POINT('Ctrl Pts',(20.5143567750622,-20.0538194850392,
80.417262464135));
#151580=CARTESIAN_POINT('Ctrl Pts',(20.2284979684703,-20.1617475291585,
80.2714704935566));
#151581=CARTESIAN_POINT('Ctrl Pts',(19.9480670705018,-20.2953208803297,
80.1230151286706));
#151582=CARTESIAN_POINT('Ctrl Pts',(19.9273554498031,-20.3051861291485,
80.1120507476752));
#151583=CARTESIAN_POINT('Ctrl Pts',(19.9066734348693,-20.3151912438291,
80.1010718420925));
#151584=CARTESIAN_POINT('Ctrl Pts',(19.8860231713586,-20.3253367559184,
80.0900792431011));
#151585=CARTESIAN_POINT('Ctrl Pts',(19.6187303069626,-20.4566582272256,
79.947793249024));
#151586=CARTESIAN_POINT('Ctrl Pts',(19.3567592096545,-20.6115057583191,
79.8032132308831));
#151587=CARTESIAN_POINT('Ctrl Pts',(19.1051659171744,-20.7894093407683,
79.6586356218779));
#151588=CARTESIAN_POINT('Ctrl Pts',(19.0728654827711,-20.8122492302517,
79.6400742384251));
#151589=CARTESIAN_POINT('Ctrl Pts',(19.0407360588875,-20.8354690788735,
79.6215128887285));
#151590=CARTESIAN_POINT('Ctrl Pts',(19.0087883050101,-20.8590678408783,
79.6029564250444));
#151591=CARTESIAN_POINT('Ctrl Pts',(19.0080136045072,-20.8596400868291,
79.6025064496939));
#151592=CARTESIAN_POINT('Ctrl Pts',(19.0072390108282,-20.8602125555853,
79.6020564772164));
#151593=CARTESIAN_POINT('Ctrl Pts',(19.0064645241169,-20.8607852470758,
79.6016065076885));
#151594=CARTESIAN_POINT('Ctrl Pts',(18.8067701111758,-21.0084485824678,
79.4855859234624));
#151595=CARTESIAN_POINT('Ctrl Pts',(18.6140280223814,-21.1710425202242,
79.3696679926295));
#151596=CARTESIAN_POINT('Ctrl Pts',(18.4307822608431,-21.3473573891257,
79.2551990600057));
#151597=CARTESIAN_POINT('Ctrl Pts',(18.3571849327144,-21.4181710502525,
79.2092246946281));
#151598=CARTESIAN_POINT('Ctrl Pts',(18.2851192504696,-21.4911974483095,
79.163484092077));
#151599=CARTESIAN_POINT('Ctrl Pts',(18.2147489810016,-21.5663560929115,
79.1180644352836));
#151600=CARTESIAN_POINT('Ctrl Pts',(18.0422175956949,-21.7506274502474,
79.0067060965142));
#151601=CARTESIAN_POINT('Ctrl Pts',(17.8798803400537,-21.9477182068604,
78.8972777885827));
#151602=CARTESIAN_POINT('Ctrl Pts',(17.7296386708767,-22.1555609120406,
78.7910139638691));
#151603=CARTESIAN_POINT('Ctrl Pts',(17.6654106032881,-22.2444133282129,
78.7455863527854));
#151604=CARTESIAN_POINT('Ctrl Pts',(17.6033925792008,-22.3352303260424,
78.700736931842));
#151605=CARTESIAN_POINT('Ctrl Pts',(17.5437307068886,-22.4278489395183,
78.6565613612389));
#151606=CARTESIAN_POINT('Ctrl Pts',(17.5431525540228,-22.4287464594037,
78.6561332782481));
#151607=CARTESIAN_POINT('Ctrl Pts',(17.5425746223999,-22.429644148466,78.6557052585308));
#151608=CARTESIAN_POINT('Ctrl Pts',(17.5419969120972,-22.4305420065136,
78.6552773021585));
#151609=CARTESIAN_POINT('Ctrl Pts',(17.402432433722,-22.6474484550983,78.5518906954236));
#151610=CARTESIAN_POINT('Ctrl Pts',(17.275623170277,-22.8744760912279,78.4520798562389));
#151611=CARTESIAN_POINT('Ctrl Pts',(17.1627326147873,-23.1089760714818,
78.3568715393448));
#151612=CARTESIAN_POINT('Ctrl Pts',(17.1150663766594,-23.2079899513524,
78.3166713446948));
#151613=CARTESIAN_POINT('Ctrl Pts',(17.069881152779,-23.3083355314165,78.2772915997086));
#151614=CARTESIAN_POINT('Ctrl Pts',(17.0272624613387,-23.4098116755575,
78.238809035761));
#151615=CARTESIAN_POINT('Ctrl Pts',(16.9247515091058,-23.6538927539119,
78.1462467317272));
#151616=CARTESIAN_POINT('Ctrl Pts',(16.8370925179916,-23.9045154058893,
78.0588763655667));
#151617=CARTESIAN_POINT('Ctrl Pts',(16.7645015768804,-24.1586334501126,
77.9773895868215));
#151618=CARTESIAN_POINT('Ctrl Pts',(16.7351538648562,-24.2613705557055,
77.9444453863498));
#151619=CARTESIAN_POINT('Ctrl Pts',(16.708268476164,-24.3646788587115,77.9124626431124));
#151620=CARTESIAN_POINT('Ctrl Pts',(16.6838574597094,-24.4683569221556,
77.8814861175022));
#151621=CARTESIAN_POINT('Ctrl Pts',(16.6835993597175,-24.4694531201524,
77.8811585997593));
#151622=CARTESIAN_POINT('Ctrl Pts',(16.6833415363243,-24.4705493594865,
77.8808311944963));
#151623=CARTESIAN_POINT('Ctrl Pts',(16.6830839894752,-24.4716456399339,
77.8805039017331));
#151624=CARTESIAN_POINT('Ctrl Pts',(16.6075775881359,-24.7930481021296,
77.7845497139153));
#151625=CARTESIAN_POINT('Ctrl Pts',(16.5557693472223,-25.1183063542804,
77.6981708478282));
#151626=CARTESIAN_POINT('Ctrl Pts',(16.5263676979949,-25.4419090629032,
77.6218851543626));
#151627=CARTESIAN_POINT('Ctrl Pts',(16.5229178833183,-25.4798786803543,
77.6129342447419));
#151628=CARTESIAN_POINT('Ctrl Pts',(16.5197764940058,-25.517825488518,77.6041222711108));
#151629=CARTESIAN_POINT('Ctrl Pts',(16.5169414026472,-25.555740574269,77.5954500541109));
#151630=CARTESIAN_POINT('Ctrl Pts',(16.491658739231,-25.8938581973755,77.5181133069824));
#151631=CARTESIAN_POINT('Ctrl Pts',(16.4907387445089,-26.2294522321289,
77.4518927603714));
#151632=CARTESIAN_POINT('Ctrl Pts',(16.5112006384634,-26.5573269539316,
77.3965079296405));
#151633=CARTESIAN_POINT('Ctrl Pts',(16.5126507836543,-26.5805636079823,
77.392582777545));
#151634=CARTESIAN_POINT('Ctrl Pts',(16.514208303769,-26.6037614969942,77.3887120400042));
#151635=CARTESIAN_POINT('Ctrl Pts',(16.5158721297067,-26.62691877498,77.384895612979));
#151636=CARTESIAN_POINT('Ctrl Pts',(20.2362883878691,-19.21905923456,65.991441278798));
#151637=CARTESIAN_POINT('Ctrl Pts',(19.6561718605991,-19.46975913513,66.282916919374));
#151638=CARTESIAN_POINT('Ctrl Pts',(18.5598661246491,-20.16689938673,66.859928238528));
#151639=CARTESIAN_POINT('Ctrl Pts',(17.2726781923991,-21.78307897052,67.63089597445));
#151640=CARTESIAN_POINT('Ctrl Pts',(16.5149844393091,-23.77214263969,68.206347704864));
#151641=CARTESIAN_POINT('Ctrl Pts',(16.4199777461291,-25.17488001869,68.413681499209));
#151642=CARTESIAN_POINT('Ctrl Pts',(16.4654068172991,-25.86638094596,68.474205480461));
#151643=CARTESIAN_POINT('Ctrl Pts',(20.7062170281991,-19.10951799103,67.232304771193));
#151644=CARTESIAN_POINT('Ctrl Pts',(20.1158188456291,-19.37047804022,67.469676518088));
#151645=CARTESIAN_POINT('Ctrl Pts',(19.0007409478491,-20.08064708151,67.935823409705));
#151646=CARTESIAN_POINT('Ctrl Pts',(17.6829174351891,-21.69045553846,68.550905928852));
#151647=CARTESIAN_POINT('Ctrl Pts',(16.8880896066391,-23.65469053605,69.005542901801));
#151648=CARTESIAN_POINT('Ctrl Pts',(16.7656461286091,-25.03809333799,69.166985238623));
#151649=CARTESIAN_POINT('Ctrl Pts',(16.7978573856091,-25.72137447255,69.213086010125));
#151650=CARTESIAN_POINT('Ctrl Pts',(21.4160457777491,-18.98907957194,69.727647073886));
#151651=CARTESIAN_POINT('Ctrl Pts',(20.8060147882291,-19.26131652568,69.860368865498));
#151652=CARTESIAN_POINT('Ctrl Pts',(19.6537267080291,-19.98557475556,70.114357140683));
#151653=CARTESIAN_POINT('Ctrl Pts',(18.2792491310391,-21.58857984457,70.429187446299));
#151654=CARTESIAN_POINT('Ctrl Pts',(17.4249804936691,-23.52609490909,70.640240430402));
#151655=CARTESIAN_POINT('Ctrl Pts',(17.2637426655391,-24.88806220984,70.696472147368));
#151656=CARTESIAN_POINT('Ctrl Pts',(17.2779315874191,-25.56194221315,70.704594103709));
#151657=CARTESIAN_POINT('Ctrl Pts',(21.8746811002291,-19.08221580172,73.5305053260389));
#151658=CARTESIAN_POINT('Ctrl Pts',(21.2390599349591,-19.34554237141,73.5093642872265));
#151659=CARTESIAN_POINT('Ctrl Pts',(20.0327821155791,-20.05868861321,73.4527172431424));
#151660=CARTESIAN_POINT('Ctrl Pts',(18.5835345216691,-21.66698079851,73.3247462356018));
#151661=CARTESIAN_POINT('Ctrl Pts',(17.6765663617291,-23.62538478012,73.1671620379613));
#151662=CARTESIAN_POINT('Ctrl Pts',(17.5004644929091,-25.00412250867,73.0545824673722));
#151663=CARTESIAN_POINT('Ctrl Pts',(17.5116592050391,-25.68535623987,72.9985767002431));
#151664=CARTESIAN_POINT('Ctrl Pts',(21.7364082859691,-19.43942007733,77.298248370054));
#151665=CARTESIAN_POINT('Ctrl Pts',(21.0739796168191,-19.66964195353,77.120649703139));
#151666=CARTESIAN_POINT('Ctrl Pts',(19.8067642895291,-20.34082664886,76.746337439781));
#151667=CARTESIAN_POINT('Ctrl Pts',(18.2875788718191,-21.96946629291,76.170375437408));
#151668=CARTESIAN_POINT('Ctrl Pts',(17.3699668233691,-24.00779371033,75.656203729192));
#151669=CARTESIAN_POINT('Ctrl Pts',(17.2329278425291,-25.44945423035,75.398807937707));
#151670=CARTESIAN_POINT('Ctrl Pts',(17.2714592832091,-26.15774963945,75.294337547645));
#151671=CARTESIAN_POINT('Ctrl Pts',(21.2442578173891,-19.78039759178,79.688891430801));
#151672=CARTESIAN_POINT('Ctrl Pts',(20.5752522699491,-19.97334520296,79.407696162325));
#151673=CARTESIAN_POINT('Ctrl Pts',(19.2831813460191,-20.59399037267,78.818398048164));
#151674=CARTESIAN_POINT('Ctrl Pts',(17.7329461897391,-22.23903620348,77.941493589672));
#151675=CARTESIAN_POINT('Ctrl Pts',(16.8277611948191,-24.36240202829,77.208327889628));
#151676=CARTESIAN_POINT('Ctrl Pts',(16.7322184029291,-25.871198608,76.886196845068));
#151677=CARTESIAN_POINT('Ctrl Pts',(16.7953681445091,-26.60785186972,76.768881260083));
#151678=CARTESIAN_POINT('Ctrl Pts',(20.8910485624391,-19.96034543716,80.846768517016));
#151679=CARTESIAN_POINT('Ctrl Pts',(20.2240002921291,-20.13083459838,80.511741733943));
#151680=CARTESIAN_POINT('Ctrl Pts',(18.9280022641691,-20.71954229589,79.809910826839));
#151681=CARTESIAN_POINT('Ctrl Pts',(17.3693373493691,-22.37162094307,78.779154983542));
#151682=CARTESIAN_POINT('Ctrl Pts',(16.4735851577291,-24.54434556066,77.944890187453));
#151683=CARTESIAN_POINT('Ctrl Pts',(16.3981512864091,-26.09221327059,77.60473604749));
#151684=CARTESIAN_POINT('Ctrl Pts',(16.4722738819291,-26.84515323639,77.489330396979));
#151685=CARTESIAN_POINT('Origin',(22.9325866828116,-25.680307646595,65.7954246374866));
#151686=CARTESIAN_POINT('Ctrl Pts',(13.2930694310391,-20.66237848365,53.68975486087));
#151687=CARTESIAN_POINT('Ctrl Pts',(10.7180091674091,-21.08563477736,56.49440478545));
#151688=CARTESIAN_POINT('Ctrl Pts',(9.21471621113909,-23.95935693907,58.53368317417));
#151689=CARTESIAN_POINT('Ctrl Pts',(9.57611457998908,-27.76823344487,58.73202601266));
#151690=CARTESIAN_POINT('Ctrl Pts',(16.2924369462091,-20.23943758692,57.37466452154));
#151691=CARTESIAN_POINT('Ctrl Pts',(13.5489454822691,-21.02431750442,59.50105713222));
#151692=CARTESIAN_POINT('Ctrl Pts',(12.1050665875791,-23.76578490842,61.15955582037));
#151693=CARTESIAN_POINT('Ctrl Pts',(12.6176757419791,-27.21702901157,61.59573606817));
#151694=CARTESIAN_POINT('Ctrl Pts',(18.6424662440091,-19.57781353748,61.59810028618));
#151695=CARTESIAN_POINT('Ctrl Pts',(16.0534824559291,-20.58287868644,63.230417443635));
#151696=CARTESIAN_POINT('Ctrl Pts',(14.6346786905991,-23.17657072105,64.508683836537));
#151697=CARTESIAN_POINT('Ctrl Pts',(14.9438417193691,-26.33949061197,64.930416329974));
#151698=CARTESIAN_POINT('Ctrl Pts',(20.3789122648491,-19.18654856391,66.379101644893));
#151699=CARTESIAN_POINT('Ctrl Pts',(17.8362433345891,-20.29589930151,67.594481304134));
#151700=CARTESIAN_POINT('Ctrl Pts',(16.3981408222991,-22.80740317579,68.487445675464));
#151701=CARTESIAN_POINT('Ctrl Pts',(16.5805176758491,-25.82029907338,68.737672797816));
#151702=CARTESIAN_POINT('',(9.66895531238909,-27.56162305116,58.82327613956));
#151703=CARTESIAN_POINT('Ctrl Pts',(9.66895531218067,-27.56162305116,58.8232761397796));
#151704=CARTESIAN_POINT('Ctrl Pts',(9.77608710290332,-27.5422216721081,
58.9249652233086));
#151705=CARTESIAN_POINT('Ctrl Pts',(9.88895321117128,-27.5209935825139,
59.0335358873943));
#151706=CARTESIAN_POINT('Ctrl Pts',(10.0072436822018,-27.4979159451008,
59.1492633874772));
#151707=CARTESIAN_POINT('Ctrl Pts',(10.1238338517625,-27.4751700245239,
59.2633274261098));
#151708=CARTESIAN_POINT('Ctrl Pts',(10.2456935170223,-27.4506269081709,
59.3843440639975));
#151709=CARTESIAN_POINT('Ctrl Pts',(10.3724860739076,-27.4242725941385,
59.5126066600382));
#151710=CARTESIAN_POINT('Ctrl Pts',(10.4977802711195,-27.3982297198494,
59.6393535243496));
#151711=CARTESIAN_POINT('Ctrl Pts',(10.6278914412047,-27.3704177419175,
59.773176135285));
#151712=CARTESIAN_POINT('Ctrl Pts',(10.7624560785538,-27.3408375150209,
59.9143864465665));
#151713=CARTESIAN_POINT('Ctrl Pts',(10.8939955750282,-27.3119222797242,
60.0524222159102));
#151714=CARTESIAN_POINT('Ctrl Pts',(11.0297904768344,-27.281316982425,60.1975173504776));
#151715=CARTESIAN_POINT('Ctrl Pts',(11.1694648606077,-27.2490426668715,
60.3499899515095));
#151716=CARTESIAN_POINT('Ctrl Pts',(11.2447490156163,-27.2316468888535,
60.4321723146642));
#151717=CARTESIAN_POINT('Ctrl Pts',(11.321159608222,-27.2137666170437,60.516498422091));
#151718=CARTESIAN_POINT('Ctrl Pts',(11.3986333366825,-27.1954083537372,
60.6030212674793));
#151719=CARTESIAN_POINT('Ctrl Pts',(11.5378144428915,-27.1624278396215,
60.7584590600419));
#151720=CARTESIAN_POINT('Ctrl Pts',(11.6804221980073,-27.1278911831314,
60.9209786202939));
#151721=CARTESIAN_POINT('Ctrl Pts',(11.8260325426628,-27.0917696931306,
61.0908661445346));
#151722=CARTESIAN_POINT('Ctrl Pts',(11.9672281693689,-27.0567433601439,
61.2556028980357));
#151723=CARTESIAN_POINT('Ctrl Pts',(12.1112469245432,-27.0202265326995,
61.4272677115551));
#151724=CARTESIAN_POINT('Ctrl Pts',(12.2576751072232,-26.9822296355385,
61.6061393856237));
#151725=CARTESIAN_POINT('Ctrl Pts',(12.3226316538668,-26.9653739512189,
61.6854880876783));
#151726=CARTESIAN_POINT('Ctrl Pts',(12.3880619947326,-26.9482275265822,
61.7662552377078));
#151727=CARTESIAN_POINT('Ctrl Pts',(12.4539283464614,-26.9307939267627,
61.8484662788217));
#151728=CARTESIAN_POINT('Ctrl Pts',(12.5960163946389,-26.8931858597292,
62.0258133773618));
#151729=CARTESIAN_POINT('Ctrl Pts',(12.7401308506418,-26.8542263500844,
62.20987421503));
#151730=CARTESIAN_POINT('Ctrl Pts',(12.8858554081658,-26.8139086882211,
62.4008856755935));
#151731=CARTESIAN_POINT('Ctrl Pts',(12.9285667161065,-26.8020917364283,
62.4568704008242));
#151732=CARTESIAN_POINT('Ctrl Pts',(12.9714162165931,-26.7901584148067,
62.5134523061076));
#151733=CARTESIAN_POINT('Ctrl Pts',(13.0143931242072,-26.7781093321009,
62.5706375669336));
#151734=CARTESIAN_POINT('Ctrl Pts',(13.1091969498418,-26.751529961939,62.6967839510545));
#151735=CARTESIAN_POINT('Ctrl Pts',(13.2046203502908,-26.7243846635722,
62.8258654302207));
#151736=CARTESIAN_POINT('Ctrl Pts',(13.3005416224173,-26.6966735094419,
62.9579447179794));
#151737=CARTESIAN_POINT('Ctrl Pts',(13.3485022584805,-26.6828179323767,
63.0239843618587));
#151738=CARTESIAN_POINT('Ctrl Pts',(13.3965873139316,-26.6688208915697,
63.0907734856094));
#151739=CARTESIAN_POINT('Ctrl Pts',(13.4447810230397,-26.6546823959435,
63.1583196951015));
#151740=CARTESIAN_POINT('Ctrl Pts',(13.4688778775937,-26.6476131481305,
63.1920927998475));
#151741=CARTESIAN_POINT('Ctrl Pts',(13.4930018929273,-26.6405085366125,
63.2260551775518));
#151742=CARTESIAN_POINT('Ctrl Pts',(13.5171510732691,-26.6333685624621,
63.2602077741688));
#151743=CARTESIAN_POINT('Ctrl Pts',(13.5393493205099,-26.6268054034133,
63.2916012944823));
#151744=CARTESIAN_POINT('Ctrl Pts',(13.562262411493,-26.6200058659919,63.324144014503));
#151745=CARTESIAN_POINT('Ctrl Pts',(13.5839760634089,-26.6135394010544,
63.3551108659612));
#151746=CARTESIAN_POINT('Ctrl Pts',(13.5858844069735,-26.6129710840897,
63.3578324437008));
#151747=CARTESIAN_POINT('Ctrl Pts',(13.5877835133376,-26.6124053393619,
63.360541830305));
#151748=CARTESIAN_POINT('Ctrl Pts',(13.5896720985665,-26.6118425531398,
63.3632371650776));
#151749=CARTESIAN_POINT('Ctrl Pts',(13.7434389940496,-26.5660210096465,
63.582688876301));
#151750=CARTESIAN_POINT('Ctrl Pts',(13.8905072688594,-26.5215528747677,
63.7989611004999));
#151751=CARTESIAN_POINT('Ctrl Pts',(14.0312770356143,-26.4785184816057,
64.011721612069));
#151752=CARTESIAN_POINT('Ctrl Pts',(14.1764604592964,-26.4341347998013,
64.2311529587712));
#151753=CARTESIAN_POINT('Ctrl Pts',(14.3149443160671,-26.3912760346578,
64.4468487802049));
#151754=CARTESIAN_POINT('Ctrl Pts',(14.447148206126,-26.3499796557284,64.658458625851));
#151755=CARTESIAN_POINT('Ctrl Pts',(14.5816957684308,-26.3079511865625,
64.8738198295093));
#151756=CARTESIAN_POINT('Ctrl Pts',(14.7097388113884,-26.2675407051138,
65.0849487873465));
#151757=CARTESIAN_POINT('Ctrl Pts',(14.8316986288703,-26.2287394799824,
65.2914923765872));
#151758=CARTESIAN_POINT('Ctrl Pts',(14.9570468693798,-26.188860236144,65.5037743890924));
#151759=CARTESIAN_POINT('Ctrl Pts',(15.0759693110088,-26.1506806600927,
65.7112125565739));
#151760=CARTESIAN_POINT('Ctrl Pts',(15.1888995598772,-26.1141447875305,
65.9134426219291));
#151761=CARTESIAN_POINT('Ctrl Pts',(15.2627229382154,-26.0902610046637,
66.0456419819382));
#151762=CARTESIAN_POINT('Ctrl Pts',(15.3339851579122,-26.0670786871891,
66.175616142649));
#151763=CARTESIAN_POINT('Ctrl Pts',(15.4028016457588,-26.0445727674571,
66.3032679929604));
#151764=CARTESIAN_POINT('Ctrl Pts',(15.5077431731565,-26.0102524226376,
66.4979303560947));
#151765=CARTESIAN_POINT('Ctrl Pts',(15.6070091098075,-25.9775458127129,
66.6872096404678));
#151766=CARTESIAN_POINT('Ctrl Pts',(15.7010249755036,-25.9464984904361,
66.870857023816));
#151767=CARTESIAN_POINT('Ctrl Pts',(15.7985675524621,-25.9142865249331,
67.0613933645796));
#151768=CARTESIAN_POINT('Ctrl Pts',(15.890458976969,-25.8838602604155,67.2458672631598));
#151769=CARTESIAN_POINT('Ctrl Pts',(15.9771369870681,-25.8552356095173,
67.4240241675736));
#151770=CARTESIAN_POINT('Ctrl Pts',(16.0654902566879,-25.8260577188888,
67.60562437958));
#151771=CARTESIAN_POINT('Ctrl Pts',(16.1484267094834,-25.7987512123656,
67.7806610205149));
#151772=CARTESIAN_POINT('Ctrl Pts',(16.226369910093,-25.7733047959622,67.9488891587593));
#151773=CARTESIAN_POINT('Ctrl Pts',(16.3060903466905,-25.7472781584921,
68.1209531813288));
#151774=CARTESIAN_POINT('Ctrl Pts',(16.3805873111834,-25.7231968526043,
68.285894603277));
#151775=CARTESIAN_POINT('Ctrl Pts',(16.450271297183,-25.7010280500849,68.4434777168875));
#151776=CARTESIAN_POINT('Ctrl Pts',(16.4726294312709,-25.6939151811497,
68.494038320354));
#151777=CARTESIAN_POINT('Ctrl Pts',(16.4944917657597,-25.6869990726531,
68.5438416263688));
#151778=CARTESIAN_POINT('Ctrl Pts',(16.5158709371514,-25.6802783436,68.5928804245897));
#151779=CARTESIAN_POINT('Ctrl Pts',(13.2733353341602,-20.6712011628671,
53.9604716641149));
#151780=CARTESIAN_POINT('Ctrl Pts',(13.0170347351402,-20.7250378132106,
54.2388016656023));
#151781=CARTESIAN_POINT('Ctrl Pts',(12.7582063428879,-20.8115059547408,
54.5248435686163));
#151782=CARTESIAN_POINT('Ctrl Pts',(12.5030245679339,-20.9342717895189,
54.8126593880525));
#151783=CARTESIAN_POINT('Ctrl Pts',(12.2478836190979,-21.0570179831903,
55.100429160303));
#151784=CARTESIAN_POINT('Ctrl Pts',(11.9963882360896,-21.2160503044088,
55.3899721645967));
#151785=CARTESIAN_POINT('Ctrl Pts',(11.7556603016108,-21.4120189338142,
55.6738855564106));
#151786=CARTESIAN_POINT('Ctrl Pts',(11.5149131061665,-21.6080032429329,
55.9578216645163));
#151787=CARTESIAN_POINT('Ctrl Pts',(11.2849328996215,-21.8409314181471,
56.2361298209099));
#151788=CARTESIAN_POINT('Ctrl Pts',(11.0727144271428,-22.107582157184,56.5009421516352));
#151789=CARTESIAN_POINT('Ctrl Pts',(10.860495954664,-22.3742328962209,56.7657544823605));
#151790=CARTESIAN_POINT('Ctrl Pts',(10.6660393405502,-22.6746064010369,
57.0170708879501));
#151791=CARTESIAN_POINT('Ctrl Pts',(10.4949554108468,-23.0016697749345,
57.2478918360827));
#151792=CARTESIAN_POINT('Ctrl Pts',(10.3238714811434,-23.3287331488321,
57.4787127842154));
#151793=CARTESIAN_POINT('Ctrl Pts',(10.1761603811614,-23.6824865561447,
57.6890381474577));
#151794=CARTESIAN_POINT('Ctrl Pts',(10.0550128727907,-24.0531337087021,
57.8739905639562));
#151795=CARTESIAN_POINT('Ctrl Pts',(9.93386536441998,-24.4237808612596,
58.0589429804546));
#151796=CARTESIAN_POINT('Ctrl Pts',(9.83928157859918,-24.8113218760576,
58.2185223304877));
#151797=CARTESIAN_POINT('Ctrl Pts',(9.77160709345427,-25.204943088974,58.3506914591221));
#151798=CARTESIAN_POINT('Ctrl Pts',(9.70392952498099,-25.5985822357313,
58.4828666095359));
#151799=CARTESIAN_POINT('Ctrl Pts',(9.66316383171567,-25.9983020993844,
58.5876289051968));
#151800=CARTESIAN_POINT('Ctrl Pts',(9.64708646826566,-26.3940853352116,
58.6657711555562));
#151801=CARTESIAN_POINT('Ctrl Pts',(9.63101056975571,-26.7898325079914,
58.7439062857361));
#151802=CARTESIAN_POINT('Ctrl Pts',(9.63961850007943,-27.181643774797,58.7954262256073));
#151803=CARTESIAN_POINT('Ctrl Pts',(9.66895531217942,-27.56162305116,58.8232761397809));
#151804=CARTESIAN_POINT('Ctrl Pts',(9.83370851895909,-27.80605867564,58.97339667448));
#151805=CARTESIAN_POINT('Ctrl Pts',(9.78042150163909,-27.34107630378,58.94776316344));
#151806=CARTESIAN_POINT('Ctrl Pts',(9.73957619330909,-26.46196602269,58.83698460444));
#151807=CARTESIAN_POINT('Ctrl Pts',(9.86285265310909,-25.16099225256,58.48191889848));
#151808=CARTESIAN_POINT('Ctrl Pts',(10.1423397371991,-23.99302628575,57.98753584959));
#151809=CARTESIAN_POINT('Ctrl Pts',(10.5855565583291,-22.9284853311,57.3408553055));
#151810=CARTESIAN_POINT('Ctrl Pts',(11.1731667914491,-22.02730607102,56.57244262719));
#151811=CARTESIAN_POINT('Ctrl Pts',(11.8706526240191,-21.3322492191,55.72566239936));
#151812=CARTESIAN_POINT('Ctrl Pts',(12.6953086638991,-20.82524464081,54.77937302147));
#151813=CARTESIAN_POINT('Ctrl Pts',(13.2841451199891,-20.65883849192,54.13779122735));
#151814=CARTESIAN_POINT('Ctrl Pts',(13.6035760583091,-20.61577618492,53.79797816226));
#151815=CARTESIAN_POINT('Ctrl Pts',(9.11717682860909,-27.94509497959,58.28335974554));
#151816=CARTESIAN_POINT('Ctrl Pts',(9.08937096593909,-27.48943650101,58.28325601136));
#151817=CARTESIAN_POINT('Ctrl Pts',(9.09152833544909,-26.63065417243,58.22256576765));
#151818=CARTESIAN_POINT('Ctrl Pts',(9.25956437210909,-25.3622681632,57.9493381346));
#151819=CARTESIAN_POINT('Ctrl Pts',(9.56072435519909,-24.22097731061,57.53587587343));
#151820=CARTESIAN_POINT('Ctrl Pts',(10.0031416783291,-23.17251910771,56.97022060426));
#151821=CARTESIAN_POINT('Ctrl Pts',(10.5684535699491,-22.2708802756,56.27615356594));
#151822=CARTESIAN_POINT('Ctrl Pts',(11.2265639643191,-21.55595641958,55.48995245848));
#151823=CARTESIAN_POINT('Ctrl Pts',(11.9972985087991,-21.00770518571,54.58814904501));
#151824=CARTESIAN_POINT('Ctrl Pts',(12.5456331782291,-20.80111230341,53.95883282879));
#151825=CARTESIAN_POINT('Ctrl Pts',(12.8433966925291,-20.73414220241,53.62023291165));
#151826=CARTESIAN_POINT('Ctrl Pts',(7.67397546574909,-27.95817851065,57.02941707911));
#151827=CARTESIAN_POINT('Ctrl Pts',(7.69368603541909,-27.52958047589,57.06769883325));
#151828=CARTESIAN_POINT('Ctrl Pts',(7.77522018889909,-26.72684409599,57.08322556095));
#151829=CARTESIAN_POINT('Ctrl Pts',(8.02617065688909,-25.5458747545,56.93925035408));
#151830=CARTESIAN_POINT('Ctrl Pts',(8.36984268079909,-24.47883173608,56.65894378471));
#151831=CARTESIAN_POINT('Ctrl Pts',(8.81690277762909,-23.48440306249,56.23363513379));
#151832=CARTESIAN_POINT('Ctrl Pts',(9.35082782543909,-22.60491801913,55.67727937557));
#151833=CARTESIAN_POINT('Ctrl Pts',(9.94832565112909,-21.87364104583,55.01448586002));
#151834=CARTESIAN_POINT('Ctrl Pts',(10.6327613513191,-21.2662171359,54.21867473302));
#151835=CARTESIAN_POINT('Ctrl Pts',(11.1140271747291,-20.99177940337,53.63518616128));
#151836=CARTESIAN_POINT('Ctrl Pts',(11.3752399880891,-20.8821982339,53.31253580915));
#151837=CARTESIAN_POINT('Ctrl Pts',(5.43454356140909,-27.31037712512,55.42201572643));
#151838=CARTESIAN_POINT('Ctrl Pts',(5.51448681552909,-26.94233731382,55.49057385725));
#151839=CARTESIAN_POINT('Ctrl Pts',(5.69390299566909,-26.25877334963,55.57050017209));
#151840=CARTESIAN_POINT('Ctrl Pts',(6.04460295007909,-25.25758388311,55.55120905308));
#151841=CARTESIAN_POINT('Ctrl Pts',(6.44021683080909,-24.34738618168,55.41345947614));
#151842=CARTESIAN_POINT('Ctrl Pts',(6.89728546114909,-23.48295592214,55.15425267772));
#151843=CARTESIAN_POINT('Ctrl Pts',(7.40253140983909,-22.6912641974,54.77930163254));
#151844=CARTESIAN_POINT('Ctrl Pts',(7.93992038432909,-21.99506265131,54.30127049136));
#151845=CARTESIAN_POINT('Ctrl Pts',(8.53600518809909,-21.36454828166,53.69386025715));
#151846=CARTESIAN_POINT('Ctrl Pts',(8.94653057408909,-21.02974712498,53.22152798187));
#151847=CARTESIAN_POINT('Ctrl Pts',(9.16848657809909,-20.87597367229,52.95148886331));
#151848=CARTESIAN_POINT('Ctrl Pts',(3.16862316927909,-26.0820046989,54.08896136514));
#151849=CARTESIAN_POINT('Ctrl Pts',(3.29227522776909,-25.78649730686,54.16665648107));
#151850=CARTESIAN_POINT('Ctrl Pts',(3.53973649723909,-25.24218736313,54.27316853242));
#151851=CARTESIAN_POINT('Ctrl Pts',(3.95473450660909,-24.44846538033,54.3262374297));
#151852=CARTESIAN_POINT('Ctrl Pts',(4.38029066318909,-23.7229939639,54.28628502759));
#151853=CARTESIAN_POINT('Ctrl Pts',(4.83896404899909,-23.02265304565,54.15509276207));
#151854=CARTESIAN_POINT('Ctrl Pts',(5.32122666807909,-22.36221887555,53.93421344229));
#151855=CARTESIAN_POINT('Ctrl Pts',(5.81665422799909,-21.75492892715,53.62885834605));
#151856=CARTESIAN_POINT('Ctrl Pts',(6.35405727128909,-21.16863778309,53.21732561724));
#151857=CARTESIAN_POINT('Ctrl Pts',(6.71912917933909,-20.82346967198,52.87878574479));
#151858=CARTESIAN_POINT('Ctrl Pts',(6.91624503764909,-20.65240575508,52.67904764169));
#151859=CARTESIAN_POINT('Ctrl Pts',(1.72141832568909,-24.85893421638,53.39227235504));
#151860=CARTESIAN_POINT('Ctrl Pts',(1.86138775815909,-24.6196947487,53.46571529331));
#151861=CARTESIAN_POINT('Ctrl Pts',(2.13156694140909,-24.18090919594,53.57170084919));
#151862=CARTESIAN_POINT('Ctrl Pts',(2.56163415524909,-23.54217452337,53.64706858042));
#151863=CARTESIAN_POINT('Ctrl Pts',(2.98733474422909,-22.95640933389,53.64868782902));
#151864=CARTESIAN_POINT('Ctrl Pts',(3.43416123779909,-22.38592628414,53.58043254411));
#151865=CARTESIAN_POINT('Ctrl Pts',(3.89513691238909,-21.83981625833,53.44278035182));
#151866=CARTESIAN_POINT('Ctrl Pts',(4.36284999481909,-21.32642311508,53.23837114653));
#151867=CARTESIAN_POINT('Ctrl Pts',(4.86681861189909,-20.81543581553,52.95074037956));
#151868=CARTESIAN_POINT('Ctrl Pts',(5.20856241979909,-20.50033960173,52.7054128393));
#151869=CARTESIAN_POINT('Ctrl Pts',(5.39352276268909,-20.3389852037,52.55789591871));
#151870=CARTESIAN_POINT('Ctrl Pts',(1.02430073505909,-24.12637036333,53.08835936746));
#151871=CARTESIAN_POINT('Ctrl Pts',(1.16810393818909,-23.91739391685,53.15797563719));
#151872=CARTESIAN_POINT('Ctrl Pts',(1.44218254462909,-23.53489557941,53.2607313398));
#151873=CARTESIAN_POINT('Ctrl Pts',(1.87042680159909,-22.97863212377,53.3428746214));
#151874=CARTESIAN_POINT('Ctrl Pts',(2.28892063595909,-22.46782016658,53.36102867422));
#151875=CARTESIAN_POINT('Ctrl Pts',(2.72399825596909,-21.96847658261,53.31982149989));
#151876=CARTESIAN_POINT('Ctrl Pts',(3.16990258487909,-21.48741537387,53.21940714362));
#151877=CARTESIAN_POINT('Ctrl Pts',(3.62058593277909,-21.03095975614,53.06152914518));
#151878=CARTESIAN_POINT('Ctrl Pts',(4.10556888538909,-20.57090981072,52.8326281048));
#151879=CARTESIAN_POINT('Ctrl Pts',(4.43482038252909,-20.28194513784,52.63297059822));
#151880=CARTESIAN_POINT('Ctrl Pts',(4.61342437641909,-20.13207988419,52.51162123628));
#151881=CARTESIAN_POINT('',(4.64910226411582,-20.256889925637,52.5918790595098));
#151882=CARTESIAN_POINT('Ctrl Pts',(13.2733140793291,-20.67108058276,53.96047540136));
#151883=CARTESIAN_POINT('Ctrl Pts',(12.2257002710903,-20.8471678309609,
53.716470749042));
#151884=CARTESIAN_POINT('Ctrl Pts',(10.9703341069513,-20.9769066735361,
53.4506422512973));
#151885=CARTESIAN_POINT('Ctrl Pts',(8.80304421585373,-20.9341539530389,
53.0822538172543));
#151886=CARTESIAN_POINT('Ctrl Pts',(8.03200170493279,-20.879883044699,52.9648770407774));
#151887=CARTESIAN_POINT('Ctrl Pts',(6.40018947062691,-20.6595239703279,
52.7558525862709));
#151888=CARTESIAN_POINT('Ctrl Pts',(5.54011073138219,-20.4932266343529,
52.6644263554667));
#151889=CARTESIAN_POINT('Ctrl Pts',(4.64910232197909,-20.25688994124,52.59187906431));
#151890=CARTESIAN_POINT('Ctrl Pts',(1.23275780153909,-24.13180332393,53.18230696385));
#151891=CARTESIAN_POINT('Ctrl Pts',(1.56529619659252,-24.4648844502913,
53.3305806378981));
#151892=CARTESIAN_POINT('Ctrl Pts',(1.91017087927006,-24.7772692564106,
53.4915985803787));
#151893=CARTESIAN_POINT('Ctrl Pts',(2.44441765738417,-25.2148019852262,
53.7546160241926));
#151894=CARTESIAN_POINT('Ctrl Pts',(2.7157702493135,-25.4258072295432,53.8914992340918));
#151895=CARTESIAN_POINT('Ctrl Pts',(3.03935596163509,-25.6583980544209,
54.0611380827515));
#151896=CARTESIAN_POINT('Ctrl Pts',(3.17949164949788,-25.7551694164772,
54.1360291895486));
#151897=CARTESIAN_POINT('Ctrl Pts',(3.2732338566531,-25.8190368978406,54.1864494810047));
#151898=CARTESIAN_POINT('Ctrl Pts',(3.32167141204987,-25.8515803170269,
54.2126726960811));
#151899=CARTESIAN_POINT('Ctrl Pts',(3.7336884124416,-26.1247656165185,54.4371296540365));
#151900=CARTESIAN_POINT('Ctrl Pts',(4.10147301394926,-26.3429261082056,
54.6473927299034));
#151901=CARTESIAN_POINT('Ctrl Pts',(4.65436136270961,-26.6331605172783,
54.9796968619355));
#151902=CARTESIAN_POINT('Ctrl Pts',(4.83885836952416,-26.7237375988929,
55.0932827520693));
#151903=CARTESIAN_POINT('Ctrl Pts',(5.20805692641525,-26.8925563193026,
55.3262165785686));
#151904=CARTESIAN_POINT('Ctrl Pts',(5.39398822008854,-26.9712778269078,
55.4463787381086));
#151905=CARTESIAN_POINT('Ctrl Pts',(7.04522995475302,-27.6156242640875,
56.5396614650258));
#151906=CARTESIAN_POINT('Ctrl Pts',(8.41433224598033,-27.7885413226464,
57.6323927517983));
#151907=CARTESIAN_POINT('Ctrl Pts',(9.66895531238909,-27.56162305116,58.82327613956));
#151908=CARTESIAN_POINT('Ctrl Pts',(4.64905724122965,-20.257198923201,52.5914164071972));
#151909=CARTESIAN_POINT('Ctrl Pts',(4.50275090268148,-20.3831082015137,
52.6897565959011));
#151910=CARTESIAN_POINT('Ctrl Pts',(4.35430396620251,-20.5157369186716,
52.7806356884754));
#151911=CARTESIAN_POINT('Ctrl Pts',(4.20464821630592,-20.6544868135792,
52.8630552368816));
#151912=CARTESIAN_POINT('Ctrl Pts',(4.05499508653927,-20.7932342792934,
52.9454733423099));
#151913=CARTESIAN_POINT('Ctrl Pts',(3.90413325971158,-20.93810265643,53.0194321268842));
#151914=CARTESIAN_POINT('Ctrl Pts',(3.75308161321061,-21.088286535986,53.0841158328481));
#151915=CARTESIAN_POINT('Ctrl Pts',(3.60203018546341,-21.238470198045,53.1487994451366));
#151916=CARTESIAN_POINT('Ctrl Pts',(3.4507846295339,-21.3939734096786,53.2042102799266));
#151917=CARTESIAN_POINT('Ctrl Pts',(3.30039658837663,-21.5538219581052,
53.2497670004603));
#151918=CARTESIAN_POINT('Ctrl Pts',(3.15000547702269,-21.7136737698662,
53.2953246510421));
#151919=CARTESIAN_POINT('Ctrl Pts',(3.00047190286233,-21.8778711070341,
53.3310277919671));
#151920=CARTESIAN_POINT('Ctrl Pts',(2.85284338538292,-22.0453003764685,
53.3565587080005));
#151921=CARTESIAN_POINT('Ctrl Pts',(2.70521775660114,-22.2127263697572,
53.3820891244617));
#151922=CARTESIAN_POINT('Ctrl Pts',(2.55950120823532,-22.3833824781628,
53.3974479391146));
#151923=CARTESIAN_POINT('Ctrl Pts',(2.41668848157172,-22.556065276394,53.4026001826463));
#151924=CARTESIAN_POINT('Ctrl Pts',(2.27387308141089,-22.7287513072992,
53.4077525226295));
#151925=CARTESIAN_POINT('Ctrl Pts',(2.13396160307715,-22.9034641166288,
53.4026979090517));
#151926=CARTESIAN_POINT('Ctrl Pts',(1.99785109332966,-23.0789669753365,
53.3876812805484));
#151927=CARTESIAN_POINT('Ctrl Pts',(1.86174244805379,-23.2544674299675,
53.3726648577461));
#151928=CARTESIAN_POINT('Ctrl Pts',(1.72943577324374,-23.4307564927545,
53.3476868010187));
#151929=CARTESIAN_POINT('Ctrl Pts',(1.6016934803756,-23.6066202710027,53.3132525943462));
#151930=CARTESIAN_POINT('Ctrl Pts',(1.4739500791378,-23.7824855751518,53.2788180889015));
#151931=CARTESIAN_POINT('Ctrl Pts',(1.35077113556768,-23.9579255954924,
53.2349272654012));
#151932=CARTESIAN_POINT('Ctrl Pts',(1.23275780153644,-24.13180332393,53.1823069638559));
#151933=CARTESIAN_POINT('Ctrl Pts',(-2.42455476508091,-16.92552468831,52.4988667111));
#151934=CARTESIAN_POINT('Ctrl Pts',(-2.42455476508091,-16.92552468831,52.4988667111));
#151935=CARTESIAN_POINT('Ctrl Pts',(-2.42455476508091,-16.92552468831,52.4988667111));
#151936=CARTESIAN_POINT('Ctrl Pts',(-2.42455476508091,-16.92552468831,52.4988667111));
#151937=CARTESIAN_POINT('Ctrl Pts',(0.0925700926990874,-18.66477847312,
52.37303551213));
#151938=CARTESIAN_POINT('Ctrl Pts',(-0.40352170620526,-19.01823830871,52.3978351662936));
#151939=CARTESIAN_POINT('Ctrl Pts',(-0.895515371595163,-19.3752846472,52.4224299545554));
#151940=CARTESIAN_POINT('Ctrl Pts',(-1.38380702798091,-19.73620495593,52.4468396792));
#151941=CARTESIAN_POINT('Ctrl Pts',(2.61806989089909,-19.62553369534,52.3800215797));
#151942=CARTESIAN_POINT('Ctrl Pts',(1.81091627060909,-20.56849142381,52.7494537592));
#151943=CARTESIAN_POINT('Ctrl Pts',(0.882002567539087,-21.47590869842,52.81681492777));
#151944=CARTESIAN_POINT('Ctrl Pts',(-0.118702425890913,-22.29896448428,
52.57846424995));
#151945=CARTESIAN_POINT('Ctrl Pts',(4.9224142687991,-20.20104612485,52.52308494659));
#151946=CARTESIAN_POINT('Ctrl Pts',(3.58550549598909,-21.31670369689,53.48424000451));
#151947=CARTESIAN_POINT('Ctrl Pts',(2.28444022049909,-22.80320843748,53.71713075241));
#151948=CARTESIAN_POINT('Ctrl Pts',(1.23910472621909,-24.40940586234,53.18227139459));
#151949=CARTESIAN_POINT('Ctrl Pts',(-2.42458295845305,-16.925539708287,
52.4988706296685));
#151950=CARTESIAN_POINT('Ctrl Pts',(-0.0053251185174313,-18.6527258434453,
52.3779300787027));
#151951=CARTESIAN_POINT('Ctrl Pts',(2.43348027117323,-19.659441558893,52.4080762030945));
#151952=CARTESIAN_POINT('Ctrl Pts',(4.64910226411582,-20.256889925637,52.5918790595098));
#151953=CARTESIAN_POINT('Ctrl Pts',(-3.40710623457991,16.74987807225,53.26489050321));
#151954=CARTESIAN_POINT('Ctrl Pts',(-3.44015780858091,16.7877187014,53.18678205605));
#151955=CARTESIAN_POINT('Ctrl Pts',(-3.47411659594991,16.81609088261,52.97739892932));
#151956=CARTESIAN_POINT('Ctrl Pts',(-3.39900274290291,16.69301953239,52.69930032793));
#151957=CARTESIAN_POINT('Ctrl Pts',(-3.25700159720791,16.48893470772,52.5247826245));
#151958=CARTESIAN_POINT('Ctrl Pts',(-3.13465059761291,16.32595396115,52.53248719305));
#151959=CARTESIAN_POINT('Ctrl Pts',(-3.08228869862991,16.25860810914,52.56532557876));
#151960=CARTESIAN_POINT('Ctrl Pts',(-1.68908392749091,18.03638543845,53.15637468044));
#151961=CARTESIAN_POINT('Ctrl Pts',(-1.71662850822091,18.07757909273,53.07756727486));
#151962=CARTESIAN_POINT('Ctrl Pts',(-1.74342672971091,18.10925496055,52.86678217038));
#151963=CARTESIAN_POINT('Ctrl Pts',(-1.67460039708091,17.97699686228,52.58972356196));
#151964=CARTESIAN_POINT('Ctrl Pts',(-1.54908851454091,17.75659770341,52.41886569374));
#151965=CARTESIAN_POINT('Ctrl Pts',(-1.44337391233091,17.58052643821,52.43072285259));
#151966=CARTESIAN_POINT('Ctrl Pts',(-1.39876593617091,17.50798340364,52.46536694065));
#151967=CARTESIAN_POINT('Ctrl Pts',(1.07693460833909,19.50311649761,53.0718773398));
#151968=CARTESIAN_POINT('Ctrl Pts',(1.05895121514909,19.54755046649,52.99188495825));
#151969=CARTESIAN_POINT('Ctrl Pts',(1.04578197976909,19.5815972729,52.7800824925));
#151970=CARTESIAN_POINT('Ctrl Pts',(1.10522958526909,19.43847226411,52.50633463755));
#151971=CARTESIAN_POINT('Ctrl Pts',(1.20316906527909,19.2002287929,52.34113102147));
#151972=CARTESIAN_POINT('Ctrl Pts',(1.28101030741909,19.01007425153,52.35751934278));
#151973=CARTESIAN_POINT('Ctrl Pts',(1.31310458513909,18.93178446037,52.39404246105));
#151974=CARTESIAN_POINT('Ctrl Pts',(5.06563032373909,20.59484478841,53.20623240665));
#151975=CARTESIAN_POINT('Ctrl Pts',(5.06183880814909,20.63957292805,53.12452214098));
#151976=CARTESIAN_POINT('Ctrl Pts',(5.06883951965909,20.66983858451,52.91500285754));
#151977=CARTESIAN_POINT('Ctrl Pts',(5.11505284373909,20.51752889178,52.65037067022));
#151978=CARTESIAN_POINT('Ctrl Pts',(5.17349613021909,20.26928325906,52.49244770842));
#151979=CARTESIAN_POINT('Ctrl Pts',(5.21143059488909,20.07103705068,52.50969456771));
#151980=CARTESIAN_POINT('Ctrl Pts',(5.22557289505909,19.98809984277,52.54636284127));
#151981=CARTESIAN_POINT('Ctrl Pts',(8.03610849690909,20.9874015617,53.42437431764));
#151982=CARTESIAN_POINT('Ctrl Pts',(8.04194577030909,21.02949187638,53.34171129579));
#151983=CARTESIAN_POINT('Ctrl Pts',(8.06158500465909,21.05225963239,53.13607983203));
#151984=CARTESIAN_POINT('Ctrl Pts',(8.09708351090909,20.8951095524,52.88025240482));
#151985=CARTESIAN_POINT('Ctrl Pts',(8.12753901812909,20.64660776267,52.72716979148));
#151986=CARTESIAN_POINT('Ctrl Pts',(8.13794707847909,20.44893917348,52.74223755693));
#151987=CARTESIAN_POINT('Ctrl Pts',(8.13954305478909,20.36490533889,52.77763238708));
#151988=CARTESIAN_POINT('Ctrl Pts',(11.0180886174491,20.97321204109,53.77155255328));
#151989=CARTESIAN_POINT('Ctrl Pts',(11.0335416724191,21.01102056917,53.68814340185));
#151990=CARTESIAN_POINT('Ctrl Pts',(11.0647526508891,21.02428219291,53.48823744763));
#151991=CARTESIAN_POINT('Ctrl Pts',(11.0893040268491,20.86530603859,53.24298148565));
#151992=CARTESIAN_POINT('Ctrl Pts',(11.0926876599891,20.62232524553,53.09440600867));
#151993=CARTESIAN_POINT('Ctrl Pts',(11.0761562910891,20.42936878983,53.10499311365));
#151994=CARTESIAN_POINT('Ctrl Pts',(11.0648480929591,20.34538349142,53.13787754361));
#151995=CARTESIAN_POINT('Ctrl Pts',(13.9644070623891,20.57916431854,54.23506456235));
#151996=CARTESIAN_POINT('Ctrl Pts',(13.9865267092991,20.6105729157,54.15122252992));
#151997=CARTESIAN_POINT('Ctrl Pts',(14.0231526773991,20.61201672497,53.95854525182));
#151998=CARTESIAN_POINT('Ctrl Pts',(14.0348030158591,20.4536887321,53.72503837394));
#151999=CARTESIAN_POINT('Ctrl Pts',(14.0145811381691,20.22163133078,53.58068290002));
#152000=CARTESIAN_POINT('Ctrl Pts',(13.9764484038391,20.03814293245,53.5851099017));
#152001=CARTESIAN_POINT('Ctrl Pts',(13.9544275408291,19.95608272267,53.6144092451));
#152002=CARTESIAN_POINT('Ctrl Pts',(16.8058284233791,19.81821401566,54.80384410726));
#152003=CARTESIAN_POINT('Ctrl Pts',(16.8340781940791,19.84189616667,54.72032170736));
#152004=CARTESIAN_POINT('Ctrl Pts',(16.8745289432991,19.83117104756,54.53653151378));
#152005=CARTESIAN_POINT('Ctrl Pts',(16.8736965349691,19.6764455665,54.31559597181));
#152006=CARTESIAN_POINT('Ctrl Pts',(16.8319008500691,19.45952204084,54.17500204704));
#152007=CARTESIAN_POINT('Ctrl Pts',(16.7734706797691,19.28889909667,54.17167264988));
#152008=CARTESIAN_POINT('Ctrl Pts',(16.7404857641791,19.21029645639,54.19614555997));
#152009=CARTESIAN_POINT('Ctrl Pts',(20.4359206765091,18.34298649127,55.67611292805));
#152010=CARTESIAN_POINT('Ctrl Pts',(20.4667388630091,18.3565819536,55.59285186564));
#152011=CARTESIAN_POINT('Ctrl Pts',(20.5029573525391,18.33245952273,55.42066915017));
#152012=CARTESIAN_POINT('Ctrl Pts',(20.4833180003491,18.18716761514,55.21617862709));
#152013=CARTESIAN_POINT('Ctrl Pts',(20.4184049676391,17.99415985211,55.08085560007));
#152014=CARTESIAN_POINT('Ctrl Pts',(20.3415140559391,17.84264224454,55.06763848037));
#152015=CARTESIAN_POINT('Ctrl Pts',(20.2980266000691,17.76951098269,55.08547709476));
#152016=CARTESIAN_POINT('Ctrl Pts',(23.7046130034791,16.23826005541,56.66962621578));
#152017=CARTESIAN_POINT('Ctrl Pts',(23.7384091580691,16.23740974354,56.59057333489));
#152018=CARTESIAN_POINT('Ctrl Pts',(23.7713882524891,16.19742240036,56.43482429516));
#152019=CARTESIAN_POINT('Ctrl Pts',(23.7362797661591,16.06486082624,56.24764430893));
#152020=CARTESIAN_POINT('Ctrl Pts',(23.6513044671591,15.90303658722,56.11563173389));
#152021=CARTESIAN_POINT('Ctrl Pts',(23.5556796510791,15.7805203603,56.0886553188));
#152022=CARTESIAN_POINT('Ctrl Pts',(23.4996641483091,15.71978669272,56.09627230119));
#152023=CARTESIAN_POINT('Ctrl Pts',(26.5074730295191,13.55520149323,57.66170186843));
#152024=CARTESIAN_POINT('Ctrl Pts',(26.5345305319991,13.54877802608,57.58393577616));
#152025=CARTESIAN_POINT('Ctrl Pts',(26.5521243712991,13.50849899519,57.43829414488));
#152026=CARTESIAN_POINT('Ctrl Pts',(26.4999080877691,13.39758649353,57.26420353995));
#152027=CARTESIAN_POINT('Ctrl Pts',(26.4031994683291,13.26626054144,57.13712372676));
#152028=CARTESIAN_POINT('Ctrl Pts',(26.3023331084391,13.16639120647,57.10285417391));
#152029=CARTESIAN_POINT('Ctrl Pts',(26.2421213057291,13.11480416125,57.10387121501));
#152030=CARTESIAN_POINT('Ctrl Pts',(28.0260365809591,11.66012040095,58.24862470654));
#152031=CARTESIAN_POINT('Ctrl Pts',(28.0476816641691,11.65292670417,58.1714936895));
#152032=CARTESIAN_POINT('Ctrl Pts',(28.0551995851891,11.61658071257,58.03118300585));
#152033=CARTESIAN_POINT('Ctrl Pts',(27.9934517031191,11.5216568794,57.86408561232));
#152034=CARTESIAN_POINT('Ctrl Pts',(27.8911848302791,11.40987079221,57.73990245967));
#152035=CARTESIAN_POINT('Ctrl Pts',(27.7887895379791,11.32361591897,57.70211559891));
#152036=CARTESIAN_POINT('Ctrl Pts',(27.7271521339691,11.27764565271,57.69964977519));
#152037=CARTESIAN_POINT('Ctrl Pts',(29.0847447463191,10.01576377267,58.6800910282));
#152038=CARTESIAN_POINT('Ctrl Pts',(29.1032139923391,10.00691673868,58.60442319409));
#152039=CARTESIAN_POINT('Ctrl Pts',(29.1047538730291,9.97257820357701,58.46908444647));
#152040=CARTESIAN_POINT('Ctrl Pts',(29.0369066999691,9.89056585094001,58.30730489342));
#152041=CARTESIAN_POINT('Ctrl Pts',(28.9304374574991,9.79604558653101,58.18476641947));
#152042=CARTESIAN_POINT('Ctrl Pts',(28.8258605611791,9.72374971286802,58.14350537075));
#152043=CARTESIAN_POINT('Ctrl Pts',(28.7623207753191,9.68480362226701,58.13771481948));
#152044=CARTESIAN_POINT('Ctrl Pts',(30.0344103243391,8.28039375792901,59.07930366752));
#152045=CARTESIAN_POINT('Ctrl Pts',(30.0494068162891,8.27099728743901,59.00486237631));
#152046=CARTESIAN_POINT('Ctrl Pts',(30.0449146508391,8.24027854369101,58.87380147701));
#152047=CARTESIAN_POINT('Ctrl Pts',(29.9714373510291,8.17217495521601,58.71670125264));
#152048=CARTESIAN_POINT('Ctrl Pts',(29.8614874735291,8.09516504455002,58.59575014517));
#152049=CARTESIAN_POINT('Ctrl Pts',(29.7555116330291,8.03666664573201,58.55162412187));
#152050=CARTESIAN_POINT('Ctrl Pts',(29.6906397264391,8.00479089321601,58.54295901742));
#152051=CARTESIAN_POINT('Ctrl Pts',(30.9865852142591,5.98897834251701,59.49800326924));
#152052=CARTESIAN_POINT('Ctrl Pts',(30.9977138336291,5.98144064890401,59.42489819269));
#152053=CARTESIAN_POINT('Ctrl Pts',(30.9869121544591,5.95858128531701,59.29817025603));
#152054=CARTESIAN_POINT('Ctrl Pts',(30.9078234541491,5.90949647884401,59.14574880578));
#152055=CARTESIAN_POINT('Ctrl Pts',(30.7945343219091,5.85422246716001,59.02644072744));
#152056=CARTESIAN_POINT('Ctrl Pts',(30.6873012573491,5.81183682443201,58.97952488484));
#152057=CARTESIAN_POINT('Ctrl Pts',(30.6211478216291,5.78824194237301,58.96792696849));
#152058=CARTESIAN_POINT('Ctrl Pts',(31.6985560499091,3.05950795606701,59.82186454665));
#152059=CARTESIAN_POINT('Ctrl Pts',(31.7058639729391,3.05463005644801,59.74964937203));
#152060=CARTESIAN_POINT('Ctrl Pts',(31.6893593933991,3.04179231445501,59.62595519273));
#152061=CARTESIAN_POINT('Ctrl Pts',(31.6058009611491,3.01644898656901,59.47692924067));
#152062=CARTESIAN_POINT('Ctrl Pts',(31.4904078016391,2.98871223998301,59.35895991202));
#152063=CARTESIAN_POINT('Ctrl Pts',(31.3831023081891,2.96791198367201,59.31023304863));
#152064=CARTESIAN_POINT('Ctrl Pts',(31.3166485767291,2.95635194048101,59.29658677628));
#152065=CARTESIAN_POINT('Ctrl Pts',(31.9528697870491,0.0317595130754642,
59.94136526076));
#152066=CARTESIAN_POINT('Ctrl Pts',(31.9595118395691,0.0317214715852542,
59.86982005549));
#152067=CARTESIAN_POINT('Ctrl Pts',(31.9418703744391,0.0316044173649042,
59.7476393923));
#152068=CARTESIAN_POINT('Ctrl Pts',(31.8570592176591,0.0313477725403642,
59.59998716507));
#152069=CARTESIAN_POINT('Ctrl Pts',(31.7405930043491,0.0310540693394842,
59.48235757363));
#152070=CARTESIAN_POINT('Ctrl Pts',(31.6324015555691,0.0308217453532442,
59.43260160338));
#152071=CARTESIAN_POINT('Ctrl Pts',(31.5651520458091,0.0306880972146742,
59.41790430726));
#152072=CARTESIAN_POINT('Ctrl Pts',(31.7096390339091,-2.99439664410999,
59.8269624593));
#152073=CARTESIAN_POINT('Ctrl Pts',(31.7168773774691,-2.98964919846099,
59.75475691015));
#152074=CARTESIAN_POINT('Ctrl Pts',(31.7002725349691,-2.97711986729099,
59.63110422964));
#152075=CARTESIAN_POINT('Ctrl Pts',(31.6166408408991,-2.95233086026699,
59.48212883459));
#152076=CARTESIAN_POINT('Ctrl Pts',(31.5012193086591,-2.92517228349799,
59.36418257283));
#152077=CARTESIAN_POINT('Ctrl Pts',(31.3939231685891,-2.90477741108599,
59.31543332717));
#152078=CARTESIAN_POINT('Ctrl Pts',(31.3274729253591,-2.89343129713299,
59.30175933843));
#152079=CARTESIAN_POINT('Ctrl Pts',(31.0044106669691,-5.93536919510399,
59.50603336636));
#152080=CARTESIAN_POINT('Ctrl Pts',(31.0154731923991,-5.92785021371099,
59.43296090614));
#152081=CARTESIAN_POINT('Ctrl Pts',(31.0045638706991,-5.90513994487099,
59.30632287634));
#152082=CARTESIAN_POINT('Ctrl Pts',(30.9253751969791,-5.85648208176699,
59.15399206733));
#152083=CARTESIAN_POINT('Ctrl Pts',(30.8120201776491,-5.80172712439799,
59.0347122833));
#152084=CARTESIAN_POINT('Ctrl Pts',(30.7047528103491,-5.75976080252899,
58.98773724997));
#152085=CARTESIAN_POINT('Ctrl Pts',(30.6385665932191,-5.73639908315999,
58.97607793401));
#152086=CARTESIAN_POINT('Ctrl Pts',(30.0557145698791,-8.23704896139899,
59.08843189482));
#152087=CARTESIAN_POINT('Ctrl Pts',(30.0705985394091,-8.22770398536199,
59.01400704745));
#152088=CARTESIAN_POINT('Ctrl Pts',(30.0659296562591,-8.19715733411999,
58.88302652709));
#152089=CARTESIAN_POINT('Ctrl Pts',(29.9923124410791,-8.12942617515799,
58.72602481875));
#152090=CARTESIAN_POINT('Ctrl Pts',(29.8823004329491,-8.05282051051399,
58.60511553591));
#152091=CARTESIAN_POINT('Ctrl Pts',(29.7763309397791,-7.99459750740499,
58.56094125343));
#152092=CARTESIAN_POINT('Ctrl Pts',(29.7114575444091,-7.96285095315699,
58.5522226205));
#152093=CARTESIAN_POINT('Ctrl Pts',(29.1078599310991,-9.97750665916399,
58.68964302613));
#152094=CARTESIAN_POINT('Ctrl Pts',(29.1262401562691,-9.96865880744899,
58.61399984743));
#152095=CARTESIAN_POINT('Ctrl Pts',(29.1276254743691,-9.93441589189099,
58.47875913071));
#152096=CARTESIAN_POINT('Ctrl Pts',(29.0596373139691,-9.85271906620799,
58.31709135142));
#152097=CARTESIAN_POINT('Ctrl Pts',(28.9530857827691,-9.75858037769199,
58.19459310768));
#152098=CARTESIAN_POINT('Ctrl Pts',(28.8484829788591,-9.68656808159099,
58.15326699513));
#152099=CARTESIAN_POINT('Ctrl Pts',(28.7849174247891,-9.64775830644099,
58.14741097197));
#152100=CARTESIAN_POINT('Ctrl Pts',(28.0475935276391,-11.63113612008,58.25712100103));
#152101=CARTESIAN_POINT('Ctrl Pts',(28.0691745203191,-11.62390612933,58.18001298797));
#152102=CARTESIAN_POINT('Ctrl Pts',(28.0765679313191,-11.58758738077,58.0397958346));
#152103=CARTESIAN_POINT('Ctrl Pts',(28.0146927415291,-11.49289309856,57.8728042192));
#152104=CARTESIAN_POINT('Ctrl Pts',(27.9123405097291,-11.38141696717,57.74865628821));
#152105=CARTESIAN_POINT('Ctrl Pts',(27.8099051124691,-11.29540682901,57.71080399278));
#152106=CARTESIAN_POINT('Ctrl Pts',(27.7482330766891,-11.24955318315,57.70827617846));
#152107=CARTESIAN_POINT('Ctrl Pts',(26.5214437291491,-13.54032966652,57.66695703587));
#152108=CARTESIAN_POINT('Ctrl Pts',(26.5485508020591,-13.53380889766,57.58923687734));
#152109=CARTESIAN_POINT('Ctrl Pts',(26.5661819088591,-13.49343887783,57.44369998587));
#152110=CARTESIAN_POINT('Ctrl Pts',(26.5139245004491,-13.38261131029,57.26969608568));
#152111=CARTESIAN_POINT('Ctrl Pts',(26.4171148585491,-13.25148782603,57.14262203634));
#152112=CARTESIAN_POINT('Ctrl Pts',(26.3161138823091,-13.15183237676,57.10826642317));
#152113=CARTESIAN_POINT('Ctrl Pts',(26.2558011253391,-13.10036270574,57.10921336507));
#152114=CARTESIAN_POINT('Ctrl Pts',(23.7055625057091,-16.23941370425,56.66968418131));
#152115=CARTESIAN_POINT('Ctrl Pts',(23.7395296243291,-16.23843525767,56.59069809116));
#152116=CARTESIAN_POINT('Ctrl Pts',(23.7727467150091,-16.19825706731,56.43505039964));
#152117=CARTESIAN_POINT('Ctrl Pts',(23.7377218800291,-16.06561772276,56.24791478528));
#152118=CARTESIAN_POINT('Ctrl Pts',(23.6526468582291,-15.90385847186,56.11586590366));
#152119=CARTESIAN_POINT('Ctrl Pts',(23.5567952192891,-15.78150421852,56.08879317878));
#152120=CARTESIAN_POINT('Ctrl Pts',(23.5006236139291,-15.72087914736,56.09634553719));
#152121=CARTESIAN_POINT('Ctrl Pts',(20.4063581786991,-18.35659770911,55.66857977841));
#152122=CARTESIAN_POINT('Ctrl Pts',(20.4372924338591,-18.37025081134,55.58533314885));
#152123=CARTESIAN_POINT('Ctrl Pts',(20.4737750944691,-18.34617970186,55.41308873976));
#152124=CARTESIAN_POINT('Ctrl Pts',(20.4543781545091,-18.20077654436,55.20848050105));
#152125=CARTESIAN_POINT('Ctrl Pts',(20.3895554076191,-18.00758317946,55.07309921297));
#152126=CARTESIAN_POINT('Ctrl Pts',(20.3126053147691,-17.85594411037,55.05992821344));
#152127=CARTESIAN_POINT('Ctrl Pts',(20.2690822741291,-17.78278504154,55.07780473431));
#152128=CARTESIAN_POINT('Ctrl Pts',(16.7993745713591,-19.82194976627,54.80194949585));
#152129=CARTESIAN_POINT('Ctrl Pts',(16.8273405443191,-19.84574005463,54.71836633499));
#152130=CARTESIAN_POINT('Ctrl Pts',(16.8673426669891,-19.83518836646,54.53445056239));
#152131=CARTESIAN_POINT('Ctrl Pts',(16.8663605573891,-19.68049552455,54.31343739281));
#152132=CARTESIAN_POINT('Ctrl Pts',(16.8247934988291,-19.46345295172,54.17287454728));
#152133=CARTESIAN_POINT('Ctrl Pts',(16.7668216086291,-19.29265043197,54.16966394249));
#152134=CARTESIAN_POINT('Ctrl Pts',(16.7341161278291,-19.21395367916,54.19420937311));
#152135=CARTESIAN_POINT('Ctrl Pts',(13.9657231564391,-20.57828465165,54.23548724589));
#152136=CARTESIAN_POINT('Ctrl Pts',(13.9879455534891,-20.60966085868,54.15166605761));
#152137=CARTESIAN_POINT('Ctrl Pts',(14.0247403784291,-20.61105128252,53.95902957051));
#152138=CARTESIAN_POINT('Ctrl Pts',(14.0364529343591,-20.45271034974,53.72554558312));
#152139=CARTESIAN_POINT('Ctrl Pts',(14.0161518533491,-20.22068637473,53.5811777803));
#152140=CARTESIAN_POINT('Ctrl Pts',(13.9778536334091,-20.03725207962,53.58556593897));
#152141=CARTESIAN_POINT('Ctrl Pts',(13.9557336715891,-19.95522093542,53.61484203308));
#152142=CARTESIAN_POINT('Ctrl Pts',(11.0113131159191,-20.97458758877,53.77033478716));
#152143=CARTESIAN_POINT('Ctrl Pts',(11.0266214897391,-21.0124365846,53.68690337854));
#152144=CARTESIAN_POINT('Ctrl Pts',(11.0575930742591,-21.02577068253,53.48693796005));
#152145=CARTESIAN_POINT('Ctrl Pts',(11.0820802461291,-20.86680750785,53.24163470357));
#152146=CARTESIAN_POINT('Ctrl Pts',(11.0856142047891,-20.62377642666,53.09306635909));
#152147=CARTESIAN_POINT('Ctrl Pts',(11.0693440424891,-20.43075299565,53.10370892621));
#152148=CARTESIAN_POINT('Ctrl Pts',(11.0581825160391,-20.34673852124,53.13662523048));
#152149=CARTESIAN_POINT('Ctrl Pts',(8.04813110016909,-20.98752038782,53.42572108627));
#152150=CARTESIAN_POINT('Ctrl Pts',(8.05403136395909,-21.02958615157,53.34306054731));
#152151=CARTESIAN_POINT('Ctrl Pts',(8.07375925218909,-21.05230244721,53.13746098213));
#152152=CARTESIAN_POINT('Ctrl Pts',(8.10923075950909,-20.89513781208,52.88167951425));
#152153=CARTESIAN_POINT('Ctrl Pts',(8.13955926130909,-20.64666172642,52.728611378));
#152154=CARTESIAN_POINT('Ctrl Pts',(8.14981954849909,-20.44902373923,52.74365318103));
#152155=CARTESIAN_POINT('Ctrl Pts',(8.15134070741909,-20.36499744938,52.77903315124));
#152156=CARTESIAN_POINT('Ctrl Pts',(5.07309482417909,-20.59608243382,53.20669897951));
#152157=CARTESIAN_POINT('Ctrl Pts',(5.06935091329909,-20.64081249018,53.12498643087));
#152158=CARTESIAN_POINT('Ctrl Pts',(5.07642996605909,-20.6710738593,52.91547662321));
#152159=CARTESIAN_POINT('Ctrl Pts',(5.12263597221909,-20.51875562994,52.65086622165));
#152160=CARTESIAN_POINT('Ctrl Pts',(5.18098777968909,-20.27050002442,52.49295530845));
#152161=CARTESIAN_POINT('Ctrl Pts',(5.21881036298909,-20.07224017422,52.51019701694));
#152162=CARTESIAN_POINT('Ctrl Pts',(5.23289940429909,-19.98929249306,52.5468624545));
#152163=CARTESIAN_POINT('Ctrl Pts',(1.08063148447909,-19.50530743072,53.07169077902));
#152164=CARTESIAN_POINT('Ctrl Pts',(1.06264699612909,-19.54974310474,52.99169611687));
#152165=CARTESIAN_POINT('Ctrl Pts',(1.04946942829909,-19.58378828415,52.77988994916));
#152166=CARTESIAN_POINT('Ctrl Pts',(1.10889319615909,-19.44064471873,52.50614477021));
#152167=CARTESIAN_POINT('Ctrl Pts',(1.20680757944909,-19.20237679195,52.34094946877));
#152168=CARTESIAN_POINT('Ctrl Pts',(1.28463643807909,-19.01220687809,52.35734645449));
#152169=CARTESIAN_POINT('Ctrl Pts',(1.31672726259909,-18.93391206485,52.39387330581));
#152170=CARTESIAN_POINT('Ctrl Pts',(-1.69053559703091,-18.03599000716,53.15636154203));
#152171=CARTESIAN_POINT('Ctrl Pts',(-1.71808399435091,-18.07718359794,53.07755602641));
#152172=CARTESIAN_POINT('Ctrl Pts',(-1.74488816840091,-18.10886086129,52.8667717657));
#152173=CARTESIAN_POINT('Ctrl Pts',(-1.67605689913091,-17.97660542263,52.5897100818));
#152174=CARTESIAN_POINT('Ctrl Pts',(-1.55053199647091,-17.75620898753,52.41884899955));
#152175=CARTESIAN_POINT('Ctrl Pts',(-1.44480576140091,-17.58014026888,52.43070527192));
#152176=CARTESIAN_POINT('Ctrl Pts',(-1.40019337549091,-17.50759891703,52.4653489107));
#152177=CARTESIAN_POINT('Ctrl Pts',(-3.41135153547391,-16.74669685633,53.26515925386));
#152178=CARTESIAN_POINT('Ctrl Pts',(-3.44441691723091,-16.78452916259,53.18705230737));
#152179=CARTESIAN_POINT('Ctrl Pts',(-3.47839365781991,-16.8128930659,52.97767245609));
#152180=CARTESIAN_POINT('Ctrl Pts',(-3.40326426680091,-16.68984456638,52.6995713555));
#152181=CARTESIAN_POINT('Ctrl Pts',(-3.26122207631491,-16.48580033262,52.52504467785));
#152182=CARTESIAN_POINT('Ctrl Pts',(-3.13882947022291,-16.32285201154,52.53273894012));
#152183=CARTESIAN_POINT('Ctrl Pts',(-3.08644810130291,-16.25551893355,52.56557287499));
#152184=CARTESIAN_POINT('Ctrl Pts',(28.7709983219891,10.49234437565,58.41163725334));
#152185=CARTESIAN_POINT('Ctrl Pts',(29.3461221071324,9.56300210468609,58.5927697031041));
#152186=CARTESIAN_POINT('Ctrl Pts',(29.8057154407229,8.63828625185421,58.7510834555065));
#152187=CARTESIAN_POINT('Ctrl Pts',(30.3555567806281,7.32278537807955,58.9515072191109));
#152188=CARTESIAN_POINT('Ctrl Pts',(30.5159033093088,6.89496887683618,59.0121909318143));
#152189=CARTESIAN_POINT('Ctrl Pts',(30.7271988464659,6.27166620909241,59.0941761584547));
#152190=CARTESIAN_POINT('Ctrl Pts',(30.7927562218314,6.06695929915259,59.1200015382421));
#152191=CARTESIAN_POINT('Ctrl Pts',(30.8843957051587,5.76472441168283,59.1565412167044));
#152192=CARTESIAN_POINT('Ctrl Pts',(30.9285417571211,5.6148146654431,59.174262504219));
#152193=CARTESIAN_POINT('Ctrl Pts',(30.9772641233391,5.44211882506228,59.1940072984711));
#152194=CARTESIAN_POINT('Ctrl Pts',(30.9975645193261,5.36858589133721,59.2022733859752));
#152195=CARTESIAN_POINT('Ctrl Pts',(31.0109707890621,5.31967141993883,59.207740935901));
#152196=CARTESIAN_POINT('Ctrl Pts',(31.0172412021778,5.29663432717222,59.2103021252824));
#152197=CARTESIAN_POINT('Ctrl Pts',(31.2464496779949,4.44801620230947,59.3040810454547));
#152198=CARTESIAN_POINT('Ctrl Pts',(31.422068609294,3.59228160990379,59.3800803609666));
#152199=CARTESIAN_POINT('Ctrl Pts',(31.6042594119283,2.26851847251972,59.4602965423362));
#152200=CARTESIAN_POINT('Ctrl Pts',(31.6513458307658,1.8206038811692,59.4813869362216));
#152201=CARTESIAN_POINT('Ctrl Pts',(31.7151442513319,0.91351085499764,59.510151984243));
#152202=CARTESIAN_POINT('Ctrl Pts',(31.7318541630843,0.452133816180361,
59.5178257421016));
#152203=CARTESIAN_POINT('Ctrl Pts',(31.7312760050765,-0.932164512008769,
59.5175336001747));
#152204=CARTESIAN_POINT('Ctrl Pts',(31.6642947229183,-1.8377192754502,59.4867196198187));
#152205=CARTESIAN_POINT('Ctrl Pts',(31.4817290686544,-3.15982924914525,
59.4064276877234));
#152206=CARTESIAN_POINT('Ctrl Pts',(31.4071817438355,-3.59455586282469,
59.3739951040488));
#152207=CARTESIAN_POINT('Ctrl Pts',(31.2763107521092,-4.23624383665348,
59.3182294737973));
#152208=CARTESIAN_POINT('Ctrl Pts',(31.20610676927,-4.55448733964118,59.2885671381903));
#152209=CARTESIAN_POINT('Ctrl Pts',(31.1161324157846,-4.92091881738991,
59.2511517616297));
#152210=CARTESIAN_POINT('Ctrl Pts',(31.0691585581828,-5.10288463135961,
59.2317800728514));
#152211=CARTESIAN_POINT('Ctrl Pts',(31.0486044725996,-5.18059821864631,
59.2233396726097));
#152212=CARTESIAN_POINT('Ctrl Pts',(31.0348082285965,-5.23234645161641,
59.2176824672922));
#152213=CARTESIAN_POINT('Ctrl Pts',(31.0275426096999,-5.2593743437665,59.2147075866874));
#152214=CARTESIAN_POINT('Ctrl Pts',(30.8074085273367,-6.07212759538227,
59.124699826665));
#152215=CARTESIAN_POINT('Ctrl Pts',(30.5296965601241,-6.9095815185838,59.0148863513764));
#152216=CARTESIAN_POINT('Ctrl Pts',(29.7963024629428,-8.65873560151838,
58.7476516372334));
#152217=CARTESIAN_POINT('Ctrl Pts',(29.3397689438772,-9.57385470219907,
58.5906228748175));
#152218=CARTESIAN_POINT('Ctrl Pts',(28.7710188797691,-10.4923807534,58.41162797882));
#152219=CARTESIAN_POINT('',(31.3508441160571,-2.89782725707868,59.2994353999759));
#152220=CARTESIAN_POINT('Ctrl Pts',(-2.42458242200845,-16.9255392716443,
52.4988706032414));
#152221=CARTESIAN_POINT('Ctrl Pts',(-2.16632614325253,-17.0988665935668,
52.4859654166524));
#152222=CARTESIAN_POINT('Ctrl Pts',(-1.77248405024906,-17.3574983428894,
52.4672011127588));
#152223=CARTESIAN_POINT('Ctrl Pts',(-0.683856029902338,-17.9865695496037,
52.4313748176118));
#152224=CARTESIAN_POINT('Ctrl Pts',(0.0112588477405891,-18.3570638684891,
52.4140653025779));
#152225=CARTESIAN_POINT('Ctrl Pts',(1.74522869355982,-19.1099025180147,
52.4092811029507));
#152226=CARTESIAN_POINT('Ctrl Pts',(2.78684201670358,-19.4924676991997,
52.4220745510272));
#152227=CARTESIAN_POINT('Ctrl Pts',(4.62995700479528,-19.9672626057456,
52.5002241852911));
#152228=CARTESIAN_POINT('Ctrl Pts',(5.29041794170216,-20.1085904800991,
52.5361613138869));
#152229=CARTESIAN_POINT('Ctrl Pts',(6.34669362641008,-20.2783653160647,
52.6104108949246));
#152230=CARTESIAN_POINT('Ctrl Pts',(6.70968283517132,-20.3279138961736,
52.6385567608978));
#152231=CARTESIAN_POINT('Ctrl Pts',(7.26966232137013,-20.3894369756384,
52.6866276868625));
#152232=CARTESIAN_POINT('Ctrl Pts',(7.45890139848648,-20.4078101042906,
52.703627261911));
#152233=CARTESIAN_POINT('Ctrl Pts',(7.7464903526402,-20.4318771574289,52.7306905966657));
#152234=CARTESIAN_POINT('Ctrl Pts',(7.8912170624135,-20.4430374054714,52.7446133131957));
#152235=CARTESIAN_POINT('Ctrl Pts',(8.03731286798729,-20.4528321403702,
52.7591418792631));
#152236=CARTESIAN_POINT('Ctrl Pts',(8.13501083043728,-20.4590522649648,
52.7689644007653));
#152237=CARTESIAN_POINT('Ctrl Pts',(8.18277051725864,-20.4619368764897,
52.7738167642272));
#152238=CARTESIAN_POINT('Ctrl Pts',(9.03936739200707,-20.5106917172357,
52.8618159068938));
#152239=CARTESIAN_POINT('Ctrl Pts',(9.80729514858892,-20.5097894221079,
52.9551892516658));
#152240=CARTESIAN_POINT('Ctrl Pts',(11.2671631570161,-20.4406463677333,
53.1547980920525));
#152241=CARTESIAN_POINT('Ctrl Pts',(11.9598251615053,-20.372355709591,53.2611368412179));
#152242=CARTESIAN_POINT('Ctrl Pts',(13.2615957830399,-20.1912275376119,
53.4784379682602));
#152243=CARTESIAN_POINT('Ctrl Pts',(13.8702498411828,-20.0784030226057,
53.5893650768242));
#152244=CARTESIAN_POINT('Ctrl Pts',(15.0001057677037,-19.8273770812652,
53.8090163975912));
#152245=CARTESIAN_POINT('Ctrl Pts',(15.5220355823112,-19.6891188015656,
53.917755928775));
#152246=CARTESIAN_POINT('Ctrl Pts',(16.9657920465214,-19.2595772205367,
54.2330585459834));
#152247=CARTESIAN_POINT('Ctrl Pts',(17.7658807493745,-18.9547675909247,
54.4281742547284));
#152248=CARTESIAN_POINT('Ctrl Pts',(18.7466149156235,-18.5395730455278,
54.6790754654745));
#152249=CARTESIAN_POINT('Ctrl Pts',(19.0369211658129,-18.4078755443859,
54.7558732415921));
#152250=CARTESIAN_POINT('Ctrl Pts',(19.4200611720369,-18.2266064375923,
54.8593141333102));
#152251=CARTESIAN_POINT('Ctrl Pts',(19.5390521798461,-18.1688795566976,
54.8918415325469));
#152252=CARTESIAN_POINT('Ctrl Pts',(19.7047275048477,-18.0869728282722,
54.9375482806614));
#152253=CARTESIAN_POINT('Ctrl Pts',(19.7843617015479,-18.0471889741464,
54.9596307963868));
#152254=CARTESIAN_POINT('Ctrl Pts',(19.8717173989075,-18.0029455223164,
54.9840156643012));
#152255=CARTESIAN_POINT('Ctrl Pts',(19.9140141553603,-17.9813809461242,
54.9958603571947));
#152256=CARTESIAN_POINT('Ctrl Pts',(19.9370470702791,-17.9695995807222,
55.0023205552476));
#152257=CARTESIAN_POINT('Ctrl Pts',(19.9480768337365,-17.963946438888,55.0054171538287));
#152258=CARTESIAN_POINT('Ctrl Pts',(19.9539307327573,-17.9609433195311,
55.0070613659337));
#152259=CARTESIAN_POINT('Ctrl Pts',(19.9532979363362,-17.9612680880685,
55.0068835935327));
#152260=CARTESIAN_POINT('Ctrl Pts',(21.0278979566056,-17.4098385978704,
55.3087502062728));
#152261=CARTESIAN_POINT('Ctrl Pts',(21.9872307161722,-16.8135812747035,
55.6059399606889));
#152262=CARTESIAN_POINT('Ctrl Pts',(23.6910635202309,-15.5993991122065,
56.1641237827156));
#152263=CARTESIAN_POINT('Ctrl Pts',(24.435605244222,-14.9813640950237,56.4252882101671));
#152264=CARTESIAN_POINT('Ctrl Pts',(25.247874111132,-14.2286703298098,56.7215268452324));
#152265=CARTESIAN_POINT('Ctrl Pts',(25.4044436438363,-14.0790877401365,
56.7792954404312));
#152266=CARTESIAN_POINT('Ctrl Pts',(25.5742363860013,-13.912277103095,56.8425741476889));
#152267=CARTESIAN_POINT('Ctrl Pts',(25.5930140841894,-13.8937629692774,
56.8495813745036));
#152268=CARTESIAN_POINT('Ctrl Pts',(25.6163765984874,-13.8706465997973,
56.8583106542445));
#152269=CARTESIAN_POINT('Ctrl Pts',(25.6203716430044,-13.8666893334539,
56.8598039775691));
#152270=CARTESIAN_POINT('Ctrl Pts',(25.6250546777405,-13.8620488471939,
56.8615546475305));
#152271=CARTESIAN_POINT('Ctrl Pts',(25.6321124084277,-13.8550515852847,
56.8641934725242));
#152272=CARTESIAN_POINT('Ctrl Pts',(25.6583551719979,-13.8289925783274,
56.87401011471));
#152273=CARTESIAN_POINT('Ctrl Pts',(25.7232460854031,-13.7642200861319,
56.8983224964411));
#152274=CARTESIAN_POINT('Ctrl Pts',(25.7894094547597,-13.6973144323053,
56.9232125149742));
#152275=CARTESIAN_POINT('Ctrl Pts',(26.0234759713672,-13.4581110773956,
57.011563091923));
#152276=CARTESIAN_POINT('Ctrl Pts',(26.2542570915582,-13.2151383992763,
57.0995489930895));
#152277=CARTESIAN_POINT('Ctrl Pts',(26.6550819662342,-12.76395485381,57.2556012621352));
#152278=CARTESIAN_POINT('Ctrl Pts',(26.7977477960912,-12.5990667370465,
57.3116159859511));
#152279=CARTESIAN_POINT('Ctrl Pts',(27.0234979757553,-12.3284864287904,
57.4012178390993));
#152280=CARTESIAN_POINT('Ctrl Pts',(27.1007028704835,-12.2344160295773,
57.4320135793588));
#152281=CARTESIAN_POINT('Ctrl Pts',(27.2191777995056,-12.0872864063817,
57.4795325384023));
#152282=CARTESIAN_POINT('Ctrl Pts',(27.2572852694891,-12.039567521655,57.4948544239221));
#152283=CARTESIAN_POINT('Ctrl Pts',(27.3445926257812,-11.9290532178486,
57.5300656388903));
#152284=CARTESIAN_POINT('Ctrl Pts',(27.5604418089713,-11.6529181842193,
57.6173801481391));
#152285=CARTESIAN_POINT('Ctrl Pts',(27.7643266128138,-11.3777193887521,
57.7011000161376));
#152286=CARTESIAN_POINT('Ctrl Pts',(27.9980297334884,-11.0490467215497,
57.7980621647422));
#152287=CARTESIAN_POINT('Ctrl Pts',(28.0741046541145,-10.9397499691282,
57.829800052545));
#152288=CARTESIAN_POINT('Ctrl Pts',(28.1855445418666,-10.7762761581739,
57.8765286440429));
#152289=CARTESIAN_POINT('Ctrl Pts',(28.2405962231963,-10.6946569176132,
57.8996730544128));
#152290=CARTESIAN_POINT('Ctrl Pts',(28.3036677385792,-10.5996568939419,
57.926287847214));
#152291=CARTESIAN_POINT('Ctrl Pts',(28.3382644776577,-10.5471314185549,
57.9409136599995));
#152292=CARTESIAN_POINT('Ctrl Pts',(28.354909008582,-10.5217355082056,57.9479581567594));
#152293=CARTESIAN_POINT('Ctrl Pts',(28.3637623064331,-10.5081959854576,
57.9517071228317));
#152294=CARTESIAN_POINT('Ctrl Pts',(28.3642504980367,-10.5074494502633,
57.9519138455112));
#152295=CARTESIAN_POINT('Ctrl Pts',(28.8072822136622,-9.82946303269992,
58.1395456803965));
#152296=CARTESIAN_POINT('Ctrl Pts',(29.1403891456331,-9.23551770479662,
58.2856110436817));
#152297=CARTESIAN_POINT('Ctrl Pts',(29.4261543259507,-8.688189577794,58.4120568897489));
#152298=CARTESIAN_POINT('Ctrl Pts',(29.4604742612531,-8.62164741825242,
58.4272743459153));
#152299=CARTESIAN_POINT('Ctrl Pts',(29.4932810185291,-8.55725794934168,
58.4418500563432));
#152300=CARTESIAN_POINT('Ctrl Pts',(29.5005342269758,-8.54300244064415,
58.4450733190014));
#152301=CARTESIAN_POINT('Ctrl Pts',(29.5065481546985,-8.53116535843972,
58.4477464851833));
#152302=CARTESIAN_POINT('Ctrl Pts',(29.5219173193004,-8.50083863653641,
58.4545807132889));
#152303=CARTESIAN_POINT('Ctrl Pts',(29.5524550061442,-8.44032846541405,
58.468168930256));
#152304=CARTESIAN_POINT('Ctrl Pts',(29.6622351103387,-8.22005640629188,
58.5171135902792));
#152305=CARTESIAN_POINT('Ctrl Pts',(29.7555017141154,-8.02473479822831,
58.5589693357939));
#152306=CARTESIAN_POINT('Ctrl Pts',(29.9676270401634,-7.56596255809928,
58.6545706892795));
#152307=CARTESIAN_POINT('Ctrl Pts',(30.0934291407565,-7.27346040122188,
58.7118290030969));
#152308=CARTESIAN_POINT('Ctrl Pts',(30.4305361920918,-6.43983351878229,
58.8661833811409));
#152309=CARTESIAN_POINT('Ctrl Pts',(30.6017015221323,-5.94273501237737,
58.9458453456209));
#152310=CARTESIAN_POINT('Ctrl Pts',(30.8690696439402,-5.08181461271089,
59.0707799223984));
#152311=CARTESIAN_POINT('Ctrl Pts',(30.9654862405048,-4.71824198664394,
59.1162478879745));
#152312=CARTESIAN_POINT('Ctrl Pts',(31.1092511104897,-4.13547169174936,
59.1842138846025));
#152313=CARTESIAN_POINT('Ctrl Pts',(31.1566306792003,-3.91615800091589,
59.2067439642156));
#152314=CARTESIAN_POINT('Ctrl Pts',(31.1882788539873,-3.76670242305925,
59.2217970147776));
#152315=CARTESIAN_POINT('Ctrl Pts',(31.1899279068987,-3.75890358193124,
59.22258140472));
#152316=CARTESIAN_POINT('Ctrl Pts',(31.191526235068,-3.75132682256149,59.2233417271164));
#152317=CARTESIAN_POINT('Ctrl Pts',(31.1924272284903,-3.74705165499355,
59.2237703419836));
#152318=CARTESIAN_POINT('Ctrl Pts',(31.192451412363,-3.74693784764103,59.2237818430606));
#152319=CARTESIAN_POINT('Ctrl Pts',(31.1979880818164,-3.72064228839014,
59.2264157979236));
#152320=CARTESIAN_POINT('Ctrl Pts',(31.2126539379119,-3.65031692538155,
59.2333953052197));
#152321=CARTESIAN_POINT('Ctrl Pts',(31.246169304696,-3.4847989670745,59.2493626506961));
#152322=CARTESIAN_POINT('Ctrl Pts',(31.2950308030585,-3.22808531019791,
59.2726919096464));
#152323=CARTESIAN_POINT('Ctrl Pts',(31.3318892564873,-3.01441384823045,
59.2903439354106));
#152324=CARTESIAN_POINT('Ctrl Pts',(31.3508441160571,-2.89782725707868,
59.2994353999759));
#152325=CARTESIAN_POINT('Ctrl Pts',(31.3508441160571,-2.89782725707868,
59.2994353999759));
#152326=CARTESIAN_POINT('Ctrl Pts',(31.3643364183393,-2.8148394868934,59.3059068163245));
#152327=CARTESIAN_POINT('Ctrl Pts',(31.3773700640756,-2.7311139651831,59.3121655266745));
#152328=CARTESIAN_POINT('Ctrl Pts',(31.4502627075308,-2.24043316614677,
59.3472058793744));
#152329=CARTESIAN_POINT('Ctrl Pts',(31.4993601963515,-1.81721685765294,
59.37096887932));
#152330=CARTESIAN_POINT('Ctrl Pts',(31.5507955538991,-1.15800595548692,
59.3959648098905));
#152331=CARTESIAN_POINT('Ctrl Pts',(31.5642321680799,-0.934211156047476,
59.4025178792687));
#152332=CARTESIAN_POINT('Ctrl Pts',(31.5780945074336,-0.592634550543183,
59.4092925482075));
#152333=CARTESIAN_POINT('Ctrl Pts',(31.5834518610784,-0.420375857261311,
59.4119157264788));
#152334=CARTESIAN_POINT('Ctrl Pts',(31.5867810664521,-0.216886265457119,
59.4135496999944));
#152335=CARTESIAN_POINT('Ctrl Pts',(31.5876940015959,-0.114518307268904,
59.4139985958855));
#152336=CARTESIAN_POINT('Ctrl Pts',(31.587988345412,-0.0576788530393498,
59.4141436080728));
#152337=CARTESIAN_POINT('Ctrl Pts',(31.5880664968281,-0.030124188040783,
59.4141822360037));
#152338=CARTESIAN_POINT('Ctrl Pts',(31.5880920817686,-0.0154155323770532,
59.4141949345244));
#152339=CARTESIAN_POINT('Ctrl Pts',(31.5880975749401,-0.0117660961253776,
59.4141976654743));
#152340=CARTESIAN_POINT('Ctrl Pts',(31.5881079907109,-0.00446340954013271,
59.4142028472302));
#152341=CARTESIAN_POINT('Ctrl Pts',(31.5895013220746,0.0964852093340877,
59.4148793415132));
#152342=CARTESIAN_POINT('Ctrl Pts',(31.5855029882768,0.48579525851113,59.4129096994819));
#152343=CARTESIAN_POINT('Ctrl Pts',(31.5800613279519,0.774270040535324,
59.4102263740453));
#152344=CARTESIAN_POINT('Ctrl Pts',(31.5523869457887,1.25116702736311,59.3967794752227));
#152345=CARTESIAN_POINT('Ctrl Pts',(31.5457695059732,1.35235209954351,59.3935675439545));
#152346=CARTESIAN_POINT('Ctrl Pts',(31.5367893723556,1.47267497284401,59.389216101337));
#152347=CARTESIAN_POINT('Ctrl Pts',(31.5357702172396,1.48613429659454,59.3887223420515));
#152348=CARTESIAN_POINT('Ctrl Pts',(31.5336880180921,1.51323299734914,59.3877137448108));
#152349=CARTESIAN_POINT('Ctrl Pts',(31.5331308836647,1.52036036184975,59.3874439247427));
#152350=CARTESIAN_POINT('Ctrl Pts',(31.5309008599961,1.54873986803599,59.3863639530715));
#152351=CARTESIAN_POINT('Ctrl Pts',(31.5263460591525,1.60550490001567,59.3841585276368));
#152352=CARTESIAN_POINT('Ctrl Pts',(31.5086031540121,1.81370488806439,59.3755720940963));
#152353=CARTESIAN_POINT('Ctrl Pts',(31.4584603244844,2.30622542292442,59.3513450096757));
#152354=CARTESIAN_POINT('Ctrl Pts',(31.3940473453495,2.76111324379761,59.3203351614487));
#152355=CARTESIAN_POINT('Ctrl Pts',(31.3176164948346,3.21526317021081,59.2836744519205));
#152356=CARTESIAN_POINT('Ctrl Pts',(31.2901345172591,3.36652440870389,59.2705120269015));
#152357=CARTESIAN_POINT('Ctrl Pts',(31.2458949964513,3.59312731575648,59.2493663033884));
#152358=CARTESIAN_POINT('Ctrl Pts',(31.2316141424242,3.6638916111659,59.2425462348826));
#152359=CARTESIAN_POINT('Ctrl Pts',(31.1995969954496,3.81740185029469,59.2272723803715));
#152360=CARTESIAN_POINT('Ctrl Pts',(31.1822274256952,3.89816656063337,59.2189941580727));
#152361=CARTESIAN_POINT('Ctrl Pts',(31.1255610878174,4.15232744849929,59.1920240911793));
#152362=CARTESIAN_POINT('Ctrl Pts',(31.081720998449,4.33760261137644,59.1712019338395));
#152363=CARTESIAN_POINT('Ctrl Pts',(31.017540391408,4.58828507862619,59.1408341645621));
#152364=CARTESIAN_POINT('Ctrl Pts',(30.9975809933864,4.66492003209589,59.1313977297925));
#152365=CARTESIAN_POINT('Ctrl Pts',(30.9765080995779,4.74367597221363,59.1214482661628));
#152366=CARTESIAN_POINT('Ctrl Pts',(30.9657812798762,4.78340525731003,59.1163859910534));
#152367=CARTESIAN_POINT('Ctrl Pts',(30.9630586863305,4.79346825522217,59.1151012495784));
#152368=CARTESIAN_POINT('Ctrl Pts',(30.9526717350889,4.83157822333907,59.1102017551008));
#152369=CARTESIAN_POINT('Ctrl Pts',(30.9061209306105,5.00130319864553,59.0882512240363));
#152370=CARTESIAN_POINT('Ctrl Pts',(30.8614554891954,5.15514021531874,59.0672545751894));
#152371=CARTESIAN_POINT('Ctrl Pts',(30.7492445259733,5.5284675154164,59.0146181758072));
#152372=CARTESIAN_POINT('Ctrl Pts',(30.6837752421392,5.72818023448767,58.9840654380761));
#152373=CARTESIAN_POINT('Ctrl Pts',(30.606644414273,5.95664803870136,58.9481511252953));
#152374=CARTESIAN_POINT('Ctrl Pts',(30.5844111552921,6.02094849677282,58.9378160443542));
#152375=CARTESIAN_POINT('Ctrl Pts',(30.5614367333558,6.08670460389163,58.9271457506316));
#152376=CARTESIAN_POINT('Ctrl Pts',(30.5570820158569,6.09912457315758,58.9251238088587));
#152377=CARTESIAN_POINT('Ctrl Pts',(30.5488619467414,6.12250588503938,58.9213080151338));
#152378=CARTESIAN_POINT('Ctrl Pts',(30.5449355619366,6.13363443630184,58.9194859040566));
#152379=CARTESIAN_POINT('Ctrl Pts',(30.5377098658508,6.1540971245753,58.9161331050368));
#152380=CARTESIAN_POINT('Ctrl Pts',(30.5320633787142,6.17005993453924,58.9135137320084));
#152381=CARTESIAN_POINT('Ctrl Pts',(30.4736147764047,6.33454315250574,58.8864116497724));
#152382=CARTESIAN_POINT('Ctrl Pts',(30.3690557537706,6.62958573704077,58.837855810521));
#152383=CARTESIAN_POINT('Ctrl Pts',(30.0125509583764,7.49842179310155,58.674749828271));
#152384=CARTESIAN_POINT('Ctrl Pts',(29.7600841387613,8.07251657893688,58.5597410349833));
#152385=CARTESIAN_POINT('Ctrl Pts',(29.3503334012256,8.85243318681241,58.378441064234));
#152386=CARTESIAN_POINT('Ctrl Pts',(29.3030494993425,8.94091740462205,58.3575776543996));
#152387=CARTESIAN_POINT('Ctrl Pts',(29.2477935313922,9.04242225112039,58.333274656692));
#152388=CARTESIAN_POINT('Ctrl Pts',(29.2416253470245,9.05372777660621,58.3305627752559));
#152389=CARTESIAN_POINT('Ctrl Pts',(29.2292314161529,9.07639289084225,58.3251158408468));
#152390=CARTESIAN_POINT('Ctrl Pts',(29.2252417118537,9.08367104141893,58.3233631745203));
#152391=CARTESIAN_POINT('Ctrl Pts',(29.2108420365903,9.10990865382669,58.3170387280041));
#152392=CARTESIAN_POINT('Ctrl Pts',(29.1819685788639,9.16233624221613,58.3043649315334));
#152393=CARTESIAN_POINT('Ctrl Pts',(29.0752885191553,9.35403928379102,58.2576234899208));
#152394=CARTESIAN_POINT('Ctrl Pts',(28.9758769922251,9.52665917566663,58.2143291862738));
#152395=CARTESIAN_POINT('Ctrl Pts',(28.7328322034821,9.93742152356835,58.109026362923));
#152396=CARTESIAN_POINT('Ctrl Pts',(28.5648839810477,10.2064838036535,58.0369688930087));
#152397=CARTESIAN_POINT('Ctrl Pts',(27.6967660476423,11.5282928587391,57.6689109432536));
#152398=CARTESIAN_POINT('Ctrl Pts',(26.9118841789333,12.5113512549311,57.3502372469519));
#152399=CARTESIAN_POINT('Ctrl Pts',(25.1829115933319,14.3312194690257,56.6913254711783));
#152400=CARTESIAN_POINT('Ctrl Pts',(24.2395124014287,15.1668846914999,56.351198049462));
#152401=CARTESIAN_POINT('Ctrl Pts',(22.7280041048116,16.2961287838868,55.8461256319013));
#152402=CARTESIAN_POINT('Ctrl Pts',(21.9478953609756,16.8298442996705,55.5947874736229));
#152403=CARTESIAN_POINT('Ctrl Pts',(20.9988547315172,17.3962858871967,55.3079261156194));
#152404=CARTESIAN_POINT('Ctrl Pts',(20.5150692586934,17.6651808024177,55.1666215132978));
#152405=CARTESIAN_POINT('Ctrl Pts',(20.2534788527478,17.8053581616721,55.0915637613476));
#152406=CARTESIAN_POINT('Ctrl Pts',(20.1307531149892,17.8697148753435,55.0567211022284));
#152407=CARTESIAN_POINT('Ctrl Pts',(20.060466439718,17.9062297903841,55.0368579370139));
#152408=CARTESIAN_POINT('Ctrl Pts',(20.0445922393146,17.9144536834225,55.032377992028));
#152409=CARTESIAN_POINT('Ctrl Pts',(18.7895387906621,18.5624030433635,54.6787873298313));
#152410=CARTESIAN_POINT('Ctrl Pts',(17.4880542508462,19.0929939467329,54.350792426133));
#152411=CARTESIAN_POINT('Ctrl Pts',(14.8049250018864,19.9130716628939,53.7585639997161));
#152412=CARTESIAN_POINT('Ctrl Pts',(13.4189225674684,20.2021071066721,53.49482150861));
#152413=CARTESIAN_POINT('Ctrl Pts',(10.5989297874419,20.5186536225354,53.0493074876692));
#152414=CARTESIAN_POINT('Ctrl Pts',(9.16879510167067,20.5474535819967,52.8667463358057));
#152415=CARTESIAN_POINT('Ctrl Pts',(7.03429655982645,20.378623757791,52.6625784528267));
#152416=CARTESIAN_POINT('Ctrl Pts',(6.32454994165452,20.2872254257206,52.605939889171));
#152417=CARTESIAN_POINT('Ctrl Pts',(5.26781972066546,20.0977345353649,52.5373095039074));
#152418=CARTESIAN_POINT('Ctrl Pts',(4.91685036642107,20.0258308076223,52.5171513356887));
#152419=CARTESIAN_POINT('Ctrl Pts',(4.39324422595082,19.9049582444335,52.4909091926348));
#152420=CARTESIAN_POINT('Ctrl Pts',(4.13216299115475,19.8412696819295,52.4787875127944));
#152421=CARTESIAN_POINT('Ctrl Pts',(3.78847452803686,19.7505915309332,52.4647163644973));
#152422=CARTESIAN_POINT('Ctrl Pts',(3.61858047887794,19.7035232752188,52.4583728317327));
#152423=CARTESIAN_POINT('Ctrl Pts',(3.53244486979829,19.6790953700934,52.4553091168919));
#152424=CARTESIAN_POINT('Ctrl Pts',(3.52828977296109,19.6779158019158,52.4551616476577));
#152425=CARTESIAN_POINT('Ctrl Pts',(2.26969720044624,19.3204479785115,52.410539354288));
#152426=CARTESIAN_POINT('Ctrl Pts',(1.15098086607544,18.8794025892053,52.4044756295119));
#152427=CARTESIAN_POINT('Ctrl Pts',(-0.823365706586399,17.9315764407793,
52.4301705412463));
#152428=CARTESIAN_POINT('Ctrl Pts',(-1.68085508940634,17.4246104337525,
52.4616915003746));
#152429=CARTESIAN_POINT('Ctrl Pts',(-2.42457349465642,16.925539184609,52.4988700952682));
#152430=CARTESIAN_POINT('',(4.64902170753621,20.2569043834612,52.5918015797662));
#152431=CARTESIAN_POINT('Ctrl Pts',(4.64902170753621,20.2569043834612,52.5918015797661));
#152432=CARTESIAN_POINT('Ctrl Pts',(2.44080379989214,19.6604809726091,52.4080693694926));
#152433=CARTESIAN_POINT('Ctrl Pts',(0.0111762509740697,18.6631588814877,
52.3771048369357));
#152434=CARTESIAN_POINT('Ctrl Pts',(-2.42457387236482,16.9255393804567,
52.4988701141421));
#152435=CARTESIAN_POINT('Ctrl Pts',(4.64902175036909,20.25690439503,52.59180158333));
#152436=CARTESIAN_POINT('Ctrl Pts',(5.53077500234378,20.4910577162601,52.6634099038893));
#152437=CARTESIAN_POINT('Ctrl Pts',(6.38264026146891,20.6568280351203,52.7536679026443));
#152438=CARTESIAN_POINT('Ctrl Pts',(8.00564535770169,20.8773654563953,52.9611269937213));
#152439=CARTESIAN_POINT('Ctrl Pts',(8.77692842067965,20.9322329149705,53.0782432829553));
#152440=CARTESIAN_POINT('Ctrl Pts',(10.951160880708,20.9769467088012,53.4469728543927));
#152441=CARTESIAN_POINT('Ctrl Pts',(12.2123332559162,20.8495653778833,53.7134261489691));
#152442=CARTESIAN_POINT('Ctrl Pts',(13.2725929185091,20.67124111202,53.96044066964));
#152443=CARTESIAN_POINT('Ctrl Pts',(7.76490383693909,-18.74690283777,98.56218991496));
#152444=CARTESIAN_POINT('Ctrl Pts',(7.58087064334909,-18.68099734404,98.11407719773));
#152445=CARTESIAN_POINT('Ctrl Pts',(7.17186061948909,-18.63711019633,97.23171771039));
#152446=CARTESIAN_POINT('Ctrl Pts',(6.40257597231909,-18.86761696116,95.91866414515));
#152447=CARTESIAN_POINT('Ctrl Pts',(5.54113344588909,-19.38926508363,94.74000227609));
#152448=CARTESIAN_POINT('Ctrl Pts',(4.60850716178909,-20.20664112972,93.74354915989));
#152449=CARTESIAN_POINT('Ctrl Pts',(3.67444280643909,-21.26785788722,93.01404174921));
#152450=CARTESIAN_POINT('Ctrl Pts',(2.80889919598909,-22.48420896871,92.59591077148));
#152451=CARTESIAN_POINT('Ctrl Pts',(2.03364908499909,-23.80773656447,92.48047031176));
#152452=CARTESIAN_POINT('Ctrl Pts',(1.61949372405909,-24.67952653565,92.60114010393));
#152453=CARTESIAN_POINT('Ctrl Pts',(1.43267983846909,-25.11816111829,92.70581998851));
#152454=CARTESIAN_POINT('Ctrl Pts',(6.84591093522909,-18.24106815967,99.10973240698));
#152455=CARTESIAN_POINT('Ctrl Pts',(6.70261001385909,-18.18978059281,98.64887935225));
#152456=CARTESIAN_POINT('Ctrl Pts',(6.37155078055909,-18.17079665846,97.74322717855));
#152457=CARTESIAN_POINT('Ctrl Pts',(5.71034935076909,-18.42237686917,96.39856329425));
#152458=CARTESIAN_POINT('Ctrl Pts',(4.93649968105909,-18.94461540664,95.19135919012));
#152459=CARTESIAN_POINT('Ctrl Pts',(4.06467328216909,-19.74072638946,94.16679995292));
#152460=CARTESIAN_POINT('Ctrl Pts',(3.15626401104909,-20.76149483123,93.40873771827));
#152461=CARTESIAN_POINT('Ctrl Pts',(2.27820018257909,-21.92509472165,92.9622122916));
#152462=CARTESIAN_POINT('Ctrl Pts',(1.45346803662909,-23.18955465286,92.81955761915));
#152463=CARTESIAN_POINT('Ctrl Pts',(0.985339306749088,-24.02354685244,92.92544468146));
#152464=CARTESIAN_POINT('Ctrl Pts',(0.766573969559087,-24.4438355265,93.02381020086));
#152465=CARTESIAN_POINT('Ctrl Pts',(5.15603146102909,-17.16231939458,99.73756536437));
#152466=CARTESIAN_POINT('Ctrl Pts',(5.07656232213909,-17.14519507788,99.27362141278));
#152467=CARTESIAN_POINT('Ctrl Pts',(4.86817723096909,-17.18438724036,98.36643775416));
#152468=CARTESIAN_POINT('Ctrl Pts',(4.38100554644909,-17.48578263476,97.02636012813));
#152469=CARTESIAN_POINT('Ctrl Pts',(3.75396200163909,-18.01131189391,95.82123531016));
#152470=CARTESIAN_POINT('Ctrl Pts',(2.99214101344909,-18.76168546006,94.78583662497));
#152471=CARTESIAN_POINT('Ctrl Pts',(2.14179705642909,-19.69395915499,93.9959895059));
#152472=CARTESIAN_POINT('Ctrl Pts',(1.26131915930909,-20.74169706882,93.4954768101));
#152473=CARTESIAN_POINT('Ctrl Pts',(0.372093247579088,-21.87630201657,93.27979108267));
#152474=CARTESIAN_POINT('Ctrl Pts',(-0.177301220500912,-22.62731794107,
93.33173363611));
#152475=CARTESIAN_POINT('Ctrl Pts',(-0.446098143760912,-23.00743325026,
93.40275143284));
#152476=CARTESIAN_POINT('Ctrl Pts',(2.01811505418909,-14.54776816726,99.9277716794));
#152477=CARTESIAN_POINT('Ctrl Pts',(2.01023554995909,-14.59632979974,99.50291917014));
#152478=CARTESIAN_POINT('Ctrl Pts',(1.94159672944909,-14.74161505002,98.68214416067));
#152479=CARTESIAN_POINT('Ctrl Pts',(1.66792258261909,-15.11758854345,97.48221302774));
#152480=CARTESIAN_POINT('Ctrl Pts',(1.24264558750909,-15.62293131579,96.39555993001));
#152481=CARTESIAN_POINT('Ctrl Pts',(0.662401506139089,-16.25798036424,95.43134765319));
#152482=CARTESIAN_POINT('Ctrl Pts',(-0.0485908112209128,-16.99447857602,
94.64062974799));
#152483=CARTESIAN_POINT('Ctrl Pts',(-0.852845516220913,-17.79509455314,
94.05825027106));
#152484=CARTESIAN_POINT('Ctrl Pts',(-1.74211739427091,-18.65432063726,93.68272059274));
#152485=CARTESIAN_POINT('Ctrl Pts',(-2.35020149985091,-19.22776358223,93.58953241735));
#152486=CARTESIAN_POINT('Ctrl Pts',(-2.66433753136591,-19.52121356586,93.5800352882));
#152487=CARTESIAN_POINT('Ctrl Pts',(-0.500978249740913,-11.56191239416,
99.08684515167));
#152488=CARTESIAN_POINT('Ctrl Pts',(-0.502039037980913,-11.64481246331,
98.72685538008));
#152489=CARTESIAN_POINT('Ctrl Pts',(-0.550354078040912,-11.83448920176,
98.03869925544));
#152490=CARTESIAN_POINT('Ctrl Pts',(-0.763358486380913,-12.20569664454,
97.03885362909));
#152491=CARTESIAN_POINT('Ctrl Pts',(-1.09904393458091,-12.63925516577,96.12438509733));
#152492=CARTESIAN_POINT('Ctrl Pts',(-1.56136469190091,-13.13963119611,95.28732914327));
#152493=CARTESIAN_POINT('Ctrl Pts',(-2.13667832435091,-13.69111153729,94.55765981838));
#152494=CARTESIAN_POINT('Ctrl Pts',(-2.80383775034391,-14.27476406571,93.9584167065));
#152495=CARTESIAN_POINT('Ctrl Pts',(-3.56787214556291,-14.89589555266,93.48403838359));
#152496=CARTESIAN_POINT('Ctrl Pts',(-4.11575259146291,-15.31302927099,93.2731503106));
#152497=CARTESIAN_POINT('Ctrl Pts',(-4.40751537919091,-15.52864660289,93.19152480061));
#152498=CARTESIAN_POINT('Ctrl Pts',(-2.40385438927091,-8.27513353230999,
97.91549930542));
#152499=CARTESIAN_POINT('Ctrl Pts',(-2.41705892460091,-8.35576375550799,
97.61350798042));
#152500=CARTESIAN_POINT('Ctrl Pts',(-2.47850833858091,-8.52577604133099,
97.04016580438));
#152501=CARTESIAN_POINT('Ctrl Pts',(-2.67662882390191,-8.82289719190299,
96.2090842562));
#152502=CARTESIAN_POINT('Ctrl Pts',(-2.96472720229591,-9.14598820546499,
95.44224967854));
#152503=CARTESIAN_POINT('Ctrl Pts',(-3.34766214760091,-9.50115635602199,
94.72434974774));
#152504=CARTESIAN_POINT('Ctrl Pts',(-3.81750557776291,-9.88052715685699,
94.07294332057));
#152505=CARTESIAN_POINT('Ctrl Pts',(-4.36228735193491,-10.27515198003,93.5025467691));
#152506=CARTESIAN_POINT('Ctrl Pts',(-4.99278044581591,-10.69277817964,93.00315604594));
#152507=CARTESIAN_POINT('Ctrl Pts',(-5.45419991380291,-10.9745024863,92.73682245074));
#152508=CARTESIAN_POINT('Ctrl Pts',(-5.70378986383891,-11.12121270698,92.61655057154));
#152509=CARTESIAN_POINT('Ctrl Pts',(-3.48946853730791,-5.66270952226699,
97.03465353091));
#152510=CARTESIAN_POINT('Ctrl Pts',(-3.51536059911091,-5.72718798709899,
96.77001431597));
#152511=CARTESIAN_POINT('Ctrl Pts',(-3.59361606472291,-5.85816473999899,
96.26934622152));
#152512=CARTESIAN_POINT('Ctrl Pts',(-3.79317244891691,-6.07452079650099,
95.5436014807));
#152513=CARTESIAN_POINT('Ctrl Pts',(-4.06044298827191,-6.30075292131999,
94.86955024439));
#152514=CARTESIAN_POINT('Ctrl Pts',(-4.40098234935791,-6.54248518883199,
94.22941353888));
#152515=CARTESIAN_POINT('Ctrl Pts',(-4.80945351933091,-6.79576625556499,
93.63469864769));
#152516=CARTESIAN_POINT('Ctrl Pts',(-5.27818789952991,-7.05626892909499,
93.09537001614));
#152517=CARTESIAN_POINT('Ctrl Pts',(-5.81982158017491,-7.33076614359399,
92.59899144013));
#152518=CARTESIAN_POINT('Ctrl Pts',(-6.21841979583891,-7.51629614060999,
92.313172261));
#152519=CARTESIAN_POINT('Ctrl Pts',(-6.43544364235691,-7.61333585955899,
92.17693035492));
#152520=CARTESIAN_POINT('Ctrl Pts',(-4.08125864136291,-3.34963677957899,
96.4640360546));
#152521=CARTESIAN_POINT('Ctrl Pts',(-4.11495573449391,-3.38996690520999,
96.22103118722));
#152522=CARTESIAN_POINT('Ctrl Pts',(-4.20360591321791,-3.47078065240599,
95.76198955656));
#152523=CARTESIAN_POINT('Ctrl Pts',(-4.40510898824891,-3.60154101220899,
95.09616413785));
#152524=CARTESIAN_POINT('Ctrl Pts',(-4.66186458946291,-3.73629411992999,
94.4753371721));
#152525=CARTESIAN_POINT('Ctrl Pts',(-4.97991493535491,-3.87877956301499,
93.88117499892));
#152526=CARTESIAN_POINT('Ctrl Pts',(-5.35511778786991,-4.02705282314199,
93.32243209734));
#152527=CARTESIAN_POINT('Ctrl Pts',(-5.78169641327591,-4.17900780868299,
92.80685149873));
#152528=CARTESIAN_POINT('Ctrl Pts',(-6.27263192495991,-4.33902725749599,
92.3209175153));
#152529=CARTESIAN_POINT('Ctrl Pts',(-6.63392144579591,-4.44742362454599,
92.03132075072));
#152530=CARTESIAN_POINT('Ctrl Pts',(-6.83104608699891,-4.50427380216299,
91.89005190681));
#152531=CARTESIAN_POINT('Ctrl Pts',(-4.32563828462991,-1.45531027820599,
96.20932054197));
#152532=CARTESIAN_POINT('Ctrl Pts',(-4.36303811445691,-1.47327684969999,
95.97550868925));
#152533=CARTESIAN_POINT('Ctrl Pts',(-4.45674571338191,-1.50907333094899,
95.53411677963));
#152534=CARTESIAN_POINT('Ctrl Pts',(-4.65983797573291,-1.56647815097599,
94.89371248405));
#152535=CARTESIAN_POINT('Ctrl Pts',(-4.91271757859291,-1.62524988581899,
94.2955919798));
#152536=CARTESIAN_POINT('Ctrl Pts',(-5.22165458228691,-1.68708854078499,
93.72129734803));
#152537=CARTESIAN_POINT('Ctrl Pts',(-5.58297014235291,-1.75121737845499,
93.17850775416));
#152538=CARTESIAN_POINT('Ctrl Pts',(-5.99162063487591,-1.81680109518699,
92.67408166894));
#152539=CARTESIAN_POINT('Ctrl Pts',(-6.46063249209491,-1.88580703178699,
92.19412061021));
#152540=CARTESIAN_POINT('Ctrl Pts',(-6.80547994037391,-1.93256605067699,
91.90424269924));
#152541=CARTESIAN_POINT('Ctrl Pts',(-6.99372679758291,-1.95710965956499,
91.76159800597));
#152542=CARTESIAN_POINT('Ctrl Pts',(-4.38971615456091,-0.00834582542081779,
96.13767933788));
#152543=CARTESIAN_POINT('Ctrl Pts',(-4.42824857521291,-0.00845141752385579,
95.90627280969));
#152544=CARTESIAN_POINT('Ctrl Pts',(-4.52354494822991,-0.00866085690577179,
95.46951686637));
#152545=CARTESIAN_POINT('Ctrl Pts',(-4.72732393892391,-0.00899423329457679,
94.83585426025));
#152546=CARTESIAN_POINT('Ctrl Pts',(-4.97934129871291,-0.00933351887315879,
94.2438310054));
#152547=CARTESIAN_POINT('Ctrl Pts',(-5.28593578059191,-0.00968867480289279,
93.67497113172));
#152548=CARTESIAN_POINT('Ctrl Pts',(-5.64354565335191,-0.0100553448513358,
93.13667952072));
#152549=CARTESIAN_POINT('Ctrl Pts',(-6.04731363736391,-0.0104288918987758,
92.6355846836));
#152550=CARTESIAN_POINT('Ctrl Pts',(-6.51025910053291,-0.0108206286907258,
92.15770391467));
#152551=CARTESIAN_POINT('Ctrl Pts',(-6.85048297649391,-0.0110852664431558,
91.86815847988));
#152552=CARTESIAN_POINT('Ctrl Pts',(-7.03620933377191,-0.0112239861470658,
91.72537995813));
#152553=CARTESIAN_POINT('Ctrl Pts',(-4.32713170324291,1.43866748068201,
96.20779519047));
#152554=CARTESIAN_POINT('Ctrl Pts',(-4.36455171328791,1.45643608224001,
95.97404039411));
#152555=CARTESIAN_POINT('Ctrl Pts',(-4.45828600907391,1.49183529502801,
95.53275739702));
#152556=CARTESIAN_POINT('Ctrl Pts',(-4.66138340529791,1.54859559587301,
94.89250848788));
#152557=CARTESIAN_POINT('Ctrl Pts',(-4.91423671646991,1.60670145769501,
94.29452563453));
#152558=CARTESIAN_POINT('Ctrl Pts',(-5.22311740864891,1.66783413833301,
93.72035042235));
#152559=CARTESIAN_POINT('Ctrl Pts',(-5.58434947881591,1.73122617606901,
93.17765569491));
#152560=CARTESIAN_POINT('Ctrl Pts',(-5.99289358065391,1.79605238890401,
92.67329470011));
#152561=CARTESIAN_POINT('Ctrl Pts',(-6.46177625288291,1.86425784562201,
92.19336654142));
#152562=CARTESIAN_POINT('Ctrl Pts',(-6.80652723416991,1.91047243766801,
91.90348413557));
#152563=CARTESIAN_POINT('Ctrl Pts',(-6.99472208375591,1.93472985067201,
91.76082943399));
#152564=CARTESIAN_POINT('Ctrl Pts',(-4.08466637979291,3.33351684098901,
96.46069423489));
#152565=CARTESIAN_POINT('Ctrl Pts',(-4.11840899567191,3.37367820166701,
96.2178178536));
#152566=CARTESIAN_POINT('Ctrl Pts',(-4.20712022633291,3.45414316234301,
95.75902244189));
#152567=CARTESIAN_POINT('Ctrl Pts',(-4.40863651739491,3.58431165906801,
95.09354947048));
#152568=CARTESIAN_POINT('Ctrl Pts',(-4.66533330758691,3.71843350521601,
94.47303426014));
#152569=CARTESIAN_POINT('Ctrl Pts',(-4.98325513816091,3.86023366340401,
93.87914038642));
#152570=CARTESIAN_POINT('Ctrl Pts',(-5.35826621411991,4.00777956126601,
93.32060660702));
#152571=CARTESIAN_POINT('Ctrl Pts',(-5.78460058356491,4.15897831435901,
92.80516330061));
#152572=CARTESIAN_POINT('Ctrl Pts',(-6.27524140749091,4.31819349568901,
92.31928870611));
#152573=CARTESIAN_POINT('Ctrl Pts',(-6.63631352672891,4.42604158474401,
92.02966887888));
#152574=CARTESIAN_POINT('Ctrl Pts',(-6.83332202411891,4.48260385956001,
91.8883702024));
#152575=CARTESIAN_POINT('Ctrl Pts',(-3.49366057865791,5.65170562487801,
97.03121358409));
#152576=CARTESIAN_POINT('Ctrl Pts',(-3.51959060155191,5.71610818987201,
96.76672008513));
#152577=CARTESIAN_POINT('Ctrl Pts',(-3.59788812876691,5.84690863477801,
96.26633081383));
#152578=CARTESIAN_POINT('Ctrl Pts',(-3.79741910388591,6.06291747560601,
95.54098130515));
#152579=CARTESIAN_POINT('Ctrl Pts',(-4.06458925483091,6.28874343571801,
94.86727462891));
#152580=CARTESIAN_POINT('Ctrl Pts',(-4.40496019109691,6.53000524676001,
94.22742782932));
#152581=CARTESIAN_POINT('Ctrl Pts',(-4.81320613037991,6.78276433667501,
93.63292996755));
#152582=CARTESIAN_POINT('Ctrl Pts',(-5.28167093282291,7.04270951258801,
93.09373074917));
#152583=CARTESIAN_POINT('Ctrl Pts',(-5.82299093728491,7.31660676789101,
92.59738480008));
#152584=CARTESIAN_POINT('Ctrl Pts',(-6.22136312270091,7.50172825322501,
92.31150938393));
#152585=CARTESIAN_POINT('Ctrl Pts',(-6.43826758672891,7.59855515253601,
92.17521557127));
#152586=CARTESIAN_POINT('Ctrl Pts',(-2.40566532396091,8.27093850373701,
97.913483192));
#152587=CARTESIAN_POINT('Ctrl Pts',(-2.41893979818091,8.35151331732401,
97.61155021493));
#152588=CARTESIAN_POINT('Ctrl Pts',(-2.48051296884091,8.52141215550501,
97.03833798277));
#152589=CARTESIAN_POINT('Ctrl Pts',(-2.67876057350391,8.81833919218701,
96.20748045575));
#152590=CARTESIAN_POINT('Ctrl Pts',(-2.96690463677591,9.14122590023601,
95.44086436563));
#152591=CARTESIAN_POINT('Ctrl Pts',(-3.34979049398491,9.49618416298601,
94.72315811491));
#152592=CARTESIAN_POINT('Ctrl Pts',(-3.81948858118091,9.87535335871601,
94.07189534027));
#152593=CARTESIAN_POINT('Ctrl Pts',(-4.36404809004391,10.26979652667,93.50157597282));
#152594=CARTESIAN_POINT('Ctrl Pts',(-4.99426574517891,10.68726364368,93.00219312889));
#152595=CARTESIAN_POINT('Ctrl Pts',(-5.45549518861091,10.96890692798,92.73582111251));
#152596=CARTESIAN_POINT('Ctrl Pts',(-5.70499060313391,11.11558274903,92.61552178529));
#152597=CARTESIAN_POINT('Ctrl Pts',(-0.986861114710913,10.72477427286,98.78960368345));
#152598=CARTESIAN_POINT('Ctrl Pts',(-0.990891422970911,10.80721848264,98.4444406356));
#152599=CARTESIAN_POINT('Ctrl Pts',(-1.04229030476091,10.99209348129,97.78557907002));
#152600=CARTESIAN_POINT('Ctrl Pts',(-1.25112303813091,11.34467819767,96.82867121273));
#152601=CARTESIAN_POINT('Ctrl Pts',(-1.57441029605091,11.75027336749,95.95168997202));
#152602=CARTESIAN_POINT('Ctrl Pts',(-2.01639196031091,12.21374866258,95.14484570844));
#152603=CARTESIAN_POINT('Ctrl Pts',(-2.56490724892091,12.72136740625,94.4349931982));
#152604=CARTESIAN_POINT('Ctrl Pts',(-3.20111188233091,13.2567343196,93.84302552526));
#152605=CARTESIAN_POINT('Ctrl Pts',(-3.93142853957191,13.82577205484,93.3622420885));
#152606=CARTESIAN_POINT('Ctrl Pts',(-4.45747219799491,14.20816411588,93.13720689211));
#152607=CARTESIAN_POINT('Ctrl Pts',(-4.73857333104691,14.40607930072,93.04570973776));
#152608=CARTESIAN_POINT('Ctrl Pts',(0.752803273019088,13.04777395438,99.50267990176));
#152609=CARTESIAN_POINT('Ctrl Pts',(0.748001440679089,13.11333574627,99.11026889267));
#152610=CARTESIAN_POINT('Ctrl Pts',(0.688801803489089,13.28050113826,98.35606433508));
#152611=CARTESIAN_POINT('Ctrl Pts',(0.444478148969087,13.65351217911,97.25704934952));
#152612=CARTESIAN_POINT('Ctrl Pts',(0.0634478276490876,14.12231339896,96.25750483054));
#152613=CARTESIAN_POINT('Ctrl Pts',(-0.457745008220911,14.68938538907,95.35776322763));
#152614=CARTESIAN_POINT('Ctrl Pts',(-1.10012730427091,15.33287565161,94.59807905016));
#152615=CARTESIAN_POINT('Ctrl Pts',(-1.83459092072091,16.0247678547,94.00725484854));
#152616=CARTESIAN_POINT('Ctrl Pts',(-2.65985793962991,16.76505394477,93.58178296922));
#152617=CARTESIAN_POINT('Ctrl Pts',(-3.23713241969691,17.2607200173,93.42919782937));
#152618=CARTESIAN_POINT('Ctrl Pts',(-3.53983067401091,17.51554255463,93.3833719997));
#152619=CARTESIAN_POINT('Ctrl Pts',(2.76127419102909,15.1656997103,99.8818256134));
#152620=CARTESIAN_POINT('Ctrl Pts',(2.73645150366909,15.19875100305,99.44781306681));
#152621=CARTESIAN_POINT('Ctrl Pts',(2.63477302079909,15.31897349528,98.60670232739));
#152622=CARTESIAN_POINT('Ctrl Pts',(2.31065481307909,15.67735269961,97.37363418217));
#152623=CARTESIAN_POINT('Ctrl Pts',(1.83767642022909,16.1875285794,96.25890102547));
#152624=CARTESIAN_POINT('Ctrl Pts',(1.21443386181909,16.84991538689,95.27779332052));
#152625=CARTESIAN_POINT('Ctrl Pts',(0.470358250379088,17.63275208932,94.48728208583));
#152626=CARTESIAN_POINT('Ctrl Pts',(-0.352070020950912,18.49178896765,93.92434986784));
#152627=CARTESIAN_POINT('Ctrl Pts',(-1.24142138326091,19.41602173204,93.58677668322));
#152628=CARTESIAN_POINT('Ctrl Pts',(-1.83558875622091,20.03129423533,93.5280107824));
#152629=CARTESIAN_POINT('Ctrl Pts',(-2.13894907756091,20.34512812081,93.53758527922));
#152630=CARTESIAN_POINT('Ctrl Pts',(5.15251803294909,17.16074206836,99.7395436905));
#152631=CARTESIAN_POINT('Ctrl Pts',(5.07319338924909,17.14367080395,99.27554213802));
#152632=CARTESIAN_POINT('Ctrl Pts',(4.86507307407909,17.18296054942,98.36827711269));
#152633=CARTESIAN_POINT('Ctrl Pts',(4.37825821066909,17.48443955237,97.02814196662));
#152634=CARTESIAN_POINT('Ctrl Pts',(3.75151422181909,18.00996471582,95.82298786203));
#152635=CARTESIAN_POINT('Ctrl Pts',(2.98992757208909,18.76024383142,94.78754665466));
#152636=CARTESIAN_POINT('Ctrl Pts',(2.13972143248909,19.69235387311,93.99761263896));
#152637=CARTESIAN_POINT('Ctrl Pts',(1.25925323305909,20.73989979774,93.49696073771));
#152638=CARTESIAN_POINT('Ctrl Pts',(0.369883529649088,21.8743228404,93.28109681334));
#152639=CARTESIAN_POINT('Ctrl Pts',(-0.179717950130911,22.62525541673,93.33292570464));
#152640=CARTESIAN_POINT('Ctrl Pts',(-0.448648786890913,23.00534209725,93.40389634347));
#152641=CARTESIAN_POINT('Ctrl Pts',(6.85073007253909,18.24407708458,99.10786428624));
#152642=CARTESIAN_POINT('Ctrl Pts',(6.70724910919909,18.19269701524,98.64702681991));
#152643=CARTESIAN_POINT('Ctrl Pts',(6.37584548782909,18.17355521153,97.74138873472));
#152644=CARTESIAN_POINT('Ctrl Pts',(5.71415695023908,18.42500317992,96.39671839293));
#152645=CARTESIAN_POINT('Ctrl Pts',(4.93989507319909,18.94723983301,95.18950999885));
#152646=CARTESIAN_POINT('Ctrl Pts',(4.06775656452909,19.7434855041,94.16498151748));
#152647=CARTESIAN_POINT('Ctrl Pts',(3.15917820969909,20.76450555988,93.40701054919));
#152648=CARTESIAN_POINT('Ctrl Pts',(2.28111507590909,21.92842864054,92.96064173443));
#152649=CARTESIAN_POINT('Ctrl Pts',(1.45656181868909,23.19324375474,92.81819939069));
#152650=CARTESIAN_POINT('Ctrl Pts',(0.988665265629088,24.0274567351,92.92424183273));
#152651=CARTESIAN_POINT('Ctrl Pts',(0.770044302759088,24.44785020645,93.02268489469));
#152652=CARTESIAN_POINT('Ctrl Pts',(7.76977665654909,18.74956759114,98.55922121492));
#152653=CARTESIAN_POINT('Ctrl Pts',(7.58552417775909,18.68358470833,98.11117902881));
#152654=CARTESIAN_POINT('Ctrl Pts',(7.17609427717909,18.63956574254,97.22895015673));
#152655=CARTESIAN_POINT('Ctrl Pts',(6.40622811537909,18.86995998959,95.91607715674));
#152656=CARTESIAN_POINT('Ctrl Pts',(5.54431599616909,19.39160284285,94.73757900216));
#152657=CARTESIAN_POINT('Ctrl Pts',(4.61136636581909,20.20908841369,93.7412845361));
#152658=CARTESIAN_POINT('Ctrl Pts',(3.67716922131909,21.27051618285,93.01193319476));
#152659=CARTESIAN_POINT('Ctrl Pts',(2.81169810886909,22.48714439168,92.59395157678));
#152660=CARTESIAN_POINT('Ctrl Pts',(2.03671749476909,23.81098447627,92.47864881967));
#152661=CARTESIAN_POINT('Ctrl Pts',(1.62285219573909,24.68297630121,92.59939017677));
#152662=CARTESIAN_POINT('Ctrl Pts',(1.43620923990909,25.12170949067,92.70409987748));
#152663=CARTESIAN_POINT('Ctrl Pts',(7.33390977334909,18.51896019671,98.61558102776));
#152664=CARTESIAN_POINT('Ctrl Pts',(7.17868839516909,18.47477382474,98.21117617597));
#152665=CARTESIAN_POINT('Ctrl Pts',(6.81702728821909,18.45460915649,97.37438079512));
#152666=CARTESIAN_POINT('Ctrl Pts',(6.12091536944909,18.68399519172,96.10537895283));
#152667=CARTESIAN_POINT('Ctrl Pts',(5.29447661592909,19.2059342101,94.91674272034));
#152668=CARTESIAN_POINT('Ctrl Pts',(4.38638383960909,20.01451204523,93.91009879714));
#152669=CARTESIAN_POINT('Ctrl Pts',(3.46301295419909,21.05896146255,93.16964338637));
#152670=CARTESIAN_POINT('Ctrl Pts',(2.59301206463909,22.25343591018,92.73998457345));
#152671=CARTESIAN_POINT('Ctrl Pts',(1.83106111871909,23.49927992091,92.61808758665));
#152672=CARTESIAN_POINT('Ctrl Pts',(1.41587669048909,24.30543668035,92.71382195817));
#152673=CARTESIAN_POINT('Ctrl Pts',(1.23275780153909,24.69194692623,92.79547180931));
#152674=CARTESIAN_POINT('Ctrl Pts',(7.24327301076909,18.44841292379,98.89152713403));
#152675=CARTESIAN_POINT('Ctrl Pts',(7.07686380614909,18.38614815484,98.4293351801));
#152676=CARTESIAN_POINT('Ctrl Pts',(6.70210515371909,18.35059385064,97.52702995238));
#152677=CARTESIAN_POINT('Ctrl Pts',(5.97702939368908,18.59059437363,96.19006143074));
#152678=CARTESIAN_POINT('Ctrl Pts',(5.15369661933909,19.10986144225,94.99856944475));
#152679=CARTESIAN_POINT('Ctrl Pts',(4.24496997515909,19.91418147426,93.9895692329));
#152680=CARTESIAN_POINT('Ctrl Pts',(3.31709496123909,20.95311160024,93.2474603871));
#152681=CARTESIAN_POINT('Ctrl Pts',(2.43917773245909,22.14131525181,92.81697663142));
#152682=CARTESIAN_POINT('Ctrl Pts',(1.62775941032909,23.44334321557,92.68893680414));
#152683=CARTESIAN_POINT('Ctrl Pts',(1.18008954667909,24.30420194899,92.80696251476));
#152684=CARTESIAN_POINT('Ctrl Pts',(0.973133455769088,24.74102620381,92.9129604542));
#152685=CARTESIAN_POINT('Ctrl Pts',(8.00953233305909,18.89726647515,98.48609646253));
#152686=CARTESIAN_POINT('Ctrl Pts',(7.82726256922909,18.83110259375,98.02900834109));
#152687=CARTESIAN_POINT('Ctrl Pts',(7.42476847736909,18.79032238758,97.13584503445));
#152688=CARTESIAN_POINT('Ctrl Pts',(6.66957047162909,19.03118815527,95.81024525772));
#152689=CARTESIAN_POINT('Ctrl Pts',(5.83099218217909,19.56043801888,94.6272581298));
#152690=CARTESIAN_POINT('Ctrl Pts',(4.92353481037909,20.38417296558,93.62422832877));
#152691=CARTESIAN_POINT('Ctrl Pts',(4.01444774807909,21.45048632645,92.88558108514));
#152692=CARTESIAN_POINT('Ctrl Pts',(3.17125581513909,22.67115923528,92.45618350511));
#152693=CARTESIAN_POINT('Ctrl Pts',(2.40912940075909,24.00907021716,92.32694912102));
#152694=CARTESIAN_POINT('Ctrl Pts',(2.00081881447909,24.89344637271,92.44258765142));
#152695=CARTESIAN_POINT('Ctrl Pts',(1.81538572080909,25.34207419056,92.54692663014));
#152696=CARTESIAN_POINT('Ctrl Pts',(9.48574240951909,19.63597267403,97.59516207783));
#152697=CARTESIAN_POINT('Ctrl Pts',(9.27104903689909,19.56585320366,97.15168124725));
#152698=CARTESIAN_POINT('Ctrl Pts',(8.81196101849909,19.5209615512,96.28385992272));
#152699=CARTESIAN_POINT('Ctrl Pts',(7.99594013996909,19.76837911278,94.99193752219));
#152700=CARTESIAN_POINT('Ctrl Pts',(7.12744499441909,20.31683308929,93.8352360129));
#152701=CARTESIAN_POINT('Ctrl Pts',(6.22395983921909,21.17277039945,92.85037342522));
#152702=CARTESIAN_POINT('Ctrl Pts',(5.35404037564909,22.28208598191,92.12036988641));
#152703=CARTESIAN_POINT('Ctrl Pts',(4.58119122970909,23.55258633343,91.68997564786));
#152704=CARTESIAN_POINT('Ctrl Pts',(3.91718676034909,24.94517181348,91.55071182088));
#152705=CARTESIAN_POINT('Ctrl Pts',(3.58611082929909,25.86546670108,91.65436237848));
#152706=CARTESIAN_POINT('Ctrl Pts',(3.44265110932909,26.33221020789,91.75135962898));
#152707=CARTESIAN_POINT('Ctrl Pts',(11.6479277035891,20.40116728954,95.92876188531));
#152708=CARTESIAN_POINT('Ctrl Pts',(11.3848777392391,20.33605104043,95.51483955623));
#152709=CARTESIAN_POINT('Ctrl Pts',(10.8425601258091,20.30358730125,94.70403709746));
#152710=CARTESIAN_POINT('Ctrl Pts',(9.94089745124909,20.5768235546,93.49247187146));
#152711=CARTESIAN_POINT('Ctrl Pts',(9.03464754236909,21.15521919782,92.4011837042));
#152712=CARTESIAN_POINT('Ctrl Pts',(8.14400714704909,22.04488243193,91.46220571441));
#152713=CARTESIAN_POINT('Ctrl Pts',(7.33708442288909,23.19040987993,90.75253698504));
#152714=CARTESIAN_POINT('Ctrl Pts',(6.66960293537909,24.49872891802,90.3154847248));
#152715=CARTESIAN_POINT('Ctrl Pts',(6.14760493758909,25.93194257256,90.14439432218));
#152716=CARTESIAN_POINT('Ctrl Pts',(5.92586915515909,26.87990332949,90.21309060207));
#152717=CARTESIAN_POINT('Ctrl Pts',(5.84143517901909,27.36114151081,90.28943327589));
#152718=CARTESIAN_POINT('Ctrl Pts',(13.6809074185791,20.85170333419,93.96716093539));
#152719=CARTESIAN_POINT('Ctrl Pts',(13.3765394460391,20.80319375581,93.5898761014));
#152720=CARTESIAN_POINT('Ctrl Pts',(12.7651707336891,20.80285913764,92.85077521182));
#152721=CARTESIAN_POINT('Ctrl Pts',(11.7984701037891,21.11929473493,91.74278239443));
#152722=CARTESIAN_POINT('Ctrl Pts',(10.8704808523091,21.7300990431,90.73757408298));
#152723=CARTESIAN_POINT('Ctrl Pts',(10.0013578369191,22.64039295908,89.86020117914));
#152724=CARTESIAN_POINT('Ctrl Pts',(9.25609538950909,23.79538319067,89.17868977515));
#152725=CARTESIAN_POINT('Ctrl Pts',(8.68218874229909,25.10590136429,88.73363476746));
#152726=CARTESIAN_POINT('Ctrl Pts',(8.28079699504909,26.53915697395,88.52049654022));
#152727=CARTESIAN_POINT('Ctrl Pts',(8.14971560437909,27.48860192212,88.5425653416));
#152728=CARTESIAN_POINT('Ctrl Pts',(8.11401571270909,27.97154561276,88.59137325496));
#152729=CARTESIAN_POINT('Ctrl Pts',(15.5534522998791,21.03171586279,91.73576692756));
#152730=CARTESIAN_POINT('Ctrl Pts',(15.2170648098991,21.00785881936,91.39930513927));
#152731=CARTESIAN_POINT('Ctrl Pts',(14.5548673242691,21.0527148989,90.74052347661));
#152732=CARTESIAN_POINT('Ctrl Pts',(13.5478771793591,21.4221254335,89.74993758817));
#152733=CARTESIAN_POINT('Ctrl Pts',(12.6158039357191,22.06417039289,88.84384557423));
#152734=CARTESIAN_POINT('Ctrl Pts',(11.7760903471591,22.98303944533,88.03949202247));
#152735=CARTESIAN_POINT('Ctrl Pts',(11.0884865829691,24.12626750567,87.39443634879));
#152736=CARTESIAN_POINT('Ctrl Pts',(10.5926947637791,25.41198318725,86.94544353959));
#152737=CARTESIAN_POINT('Ctrl Pts',(10.2864742437991,26.81503393584,86.68964252342));
#152738=CARTESIAN_POINT('Ctrl Pts',(10.2248975625791,27.74659100247,86.66137917484));
#152739=CARTESIAN_POINT('Ctrl Pts',(10.2264729148191,28.22180509888,86.67998303916));
#152740=CARTESIAN_POINT('Ctrl Pts',(17.2430554107691,20.98202291482,89.2412331004));
#152741=CARTESIAN_POINT('Ctrl Pts',(16.8870711991091,20.98811724776,88.94690397629));
#152742=CARTESIAN_POINT('Ctrl Pts',(16.1974641026791,21.08604958705,88.3712592249));
#152743=CARTESIAN_POINT('Ctrl Pts',(15.1798276002791,21.51243494163,87.50343557567));
#152744=CARTESIAN_POINT('Ctrl Pts',(14.2633095441191,22.18214566721,86.70288959624));
#152745=CARTESIAN_POINT('Ctrl Pts',(13.4604932260391,23.09902889153,85.97946359338));
#152746=CARTESIAN_POINT('Ctrl Pts',(12.8243493470991,24.21432352264,85.37995749348));
#152747=CARTESIAN_POINT('Ctrl Pts',(12.3877610938491,25.45548507477,84.93639608553));
#152748=CARTESIAN_POINT('Ctrl Pts',(12.1466467109391,26.80621472776,84.64669984466));
#152749=CARTESIAN_POINT('Ctrl Pts',(12.1296311867691,27.7054105439,84.57240108835));
#152750=CARTESIAN_POINT('Ctrl Pts',(12.1548476689691,28.16572967293,84.56246164962));
#152751=CARTESIAN_POINT('Ctrl Pts',(19.2495989492791,20.66912552818,85.57069919532));
#152752=CARTESIAN_POINT('Ctrl Pts',(18.8813413248491,20.71804850918,85.33379157953));
#152753=CARTESIAN_POINT('Ctrl Pts',(18.1807999501791,20.88969632127,84.87114381612));
#152754=CARTESIAN_POINT('Ctrl Pts',(17.1800032533291,21.38945414672,84.17048672317));
#152755=CARTESIAN_POINT('Ctrl Pts',(16.3037323185991,22.08827360986,83.51550270559));
#152756=CARTESIAN_POINT('Ctrl Pts',(15.5566288286191,22.99073213886,82.907709313505));
#152757=CARTESIAN_POINT('Ctrl Pts',(14.9817758260491,24.05427124838,82.380258430425));
#152758=CARTESIAN_POINT('Ctrl Pts',(14.6042814360791,25.21977981858,81.958213960619));
#152759=CARTESIAN_POINT('Ctrl Pts',(14.4190122273291,26.48281801567,81.63942835036));
#152760=CARTESIAN_POINT('Ctrl Pts',(14.4356493819991,27.32680522234,81.513735365478));
#152761=CARTESIAN_POINT('Ctrl Pts',(14.4781882928991,27.76114514435,81.470312737204));
#152762=CARTESIAN_POINT('Ctrl Pts',(20.3925977909591,20.2277535595,82.563826718236));
#152763=CARTESIAN_POINT('Ctrl Pts',(20.0304340562991,20.30626477584,82.366918248488));
#152764=CARTESIAN_POINT('Ctrl Pts',(19.3485382185991,20.52649526466,81.982708898295));
#152765=CARTESIAN_POINT('Ctrl Pts',(18.3897565831791,21.06863508853,81.398921431952));
#152766=CARTESIAN_POINT('Ctrl Pts',(17.5597638046891,21.77721885701,80.848439464904));
#152767=CARTESIAN_POINT('Ctrl Pts',(16.8572640880491,22.65865690252,80.329157482003));
#152768=CARTESIAN_POINT('Ctrl Pts',(16.3182918298191,23.67557410625,79.866046158033));
#152769=CARTESIAN_POINT('Ctrl Pts',(15.9638049917991,24.77815737146,79.47897454881));
#152770=CARTESIAN_POINT('Ctrl Pts',(15.7887413289391,25.96931466839,79.164862427794));
#152771=CARTESIAN_POINT('Ctrl Pts',(15.8042210389591,26.76737479866,79.020929073105));
#152772=CARTESIAN_POINT('Ctrl Pts',(15.8449385154191,27.17970245025,78.962990978534));
#152773=CARTESIAN_POINT('Ctrl Pts',(21.0097926924391,19.89563600971,80.40741922018));
#152774=CARTESIAN_POINT('Ctrl Pts',(20.6550889131691,19.99123032158,80.236762155004));
#152775=CARTESIAN_POINT('Ctrl Pts',(19.9909956425891,20.23869347959,79.903761107118));
#152776=CARTESIAN_POINT('Ctrl Pts',(19.0648929430391,20.80252378355,79.396298271413));
#152777=CARTESIAN_POINT('Ctrl Pts',(18.2674404295791,21.51331951319,78.914958065391));
#152778=CARTESIAN_POINT('Ctrl Pts',(17.5940818891591,22.37892089328,78.456246002549));
#152779=CARTESIAN_POINT('Ctrl Pts',(17.0767465562291,23.3651962814,78.040551621815));
#152780=CARTESIAN_POINT('Ctrl Pts',(16.7340571199191,24.42771547795,77.684597081619));
#152781=CARTESIAN_POINT('Ctrl Pts',(16.5609096844291,25.5733672766,77.384841020182));
#152782=CARTESIAN_POINT('Ctrl Pts',(16.5713804283391,26.34212759319,77.237912445421));
#152783=CARTESIAN_POINT('Ctrl Pts',(16.6083416058691,26.74028365911,77.175315062579));
#152784=CARTESIAN_POINT('Ctrl Pts',(20.8003130807923,19.9701890936878,80.5583314860603));
#152785=CARTESIAN_POINT('Ctrl Pts',(20.6335820361414,20.0189518422149,80.4760789509608));
#152786=CARTESIAN_POINT('Ctrl Pts',(20.4669496987559,20.0760850758162,80.3922277537374));
#152787=CARTESIAN_POINT('Ctrl Pts',(20.3014025923107,20.1417112308046,80.3071839810886));
#152788=CARTESIAN_POINT('Ctrl Pts',(20.1619570128364,20.1969902230355,80.2355489135098));
#152789=CARTESIAN_POINT('Ctrl Pts',(20.0232809114241,20.2582959630628,80.1630672985196));
#152790=CARTESIAN_POINT('Ctrl Pts',(19.8859672107522,20.3257298729312,80.089977743185));
#152791=CARTESIAN_POINT('Ctrl Pts',(19.7194382428212,20.4075112200145,80.0013374388537));
#152792=CARTESIAN_POINT('Ctrl Pts',(19.554896435378,20.4983220718029,79.9117925166094));
#152793=CARTESIAN_POINT('Ctrl Pts',(19.3936514485524,20.5982275367535,79.8219011751989));
#152794=CARTESIAN_POINT('Ctrl Pts',(19.2629129348508,20.6792315558888,79.7490166744028));
#152795=CARTESIAN_POINT('Ctrl Pts',(19.1343420084579,20.7662135553124,79.675904710384));
#152796=CARTESIAN_POINT('Ctrl Pts',(19.0086290342816,20.8591842185031,79.6028641638261));
#152797=CARTESIAN_POINT('Ctrl Pts',(19.0081406208618,20.8595454232224,79.6025803905453));
#152798=CARTESIAN_POINT('Ctrl Pts',(19.0076522508267,20.8599067181176,79.602296618492));
#152799=CARTESIAN_POINT('Ctrl Pts',(19.0071639242108,20.8602681031926,79.6020128476805));
#152800=CARTESIAN_POINT('Ctrl Pts',(18.8391759142115,20.984587273217,79.5043935650917));
#152801=CARTESIAN_POINT('Ctrl Pts',(18.6763247663055,21.1195741449237,79.4069214661285));
#152802=CARTESIAN_POINT('Ctrl Pts',(18.5198692521112,21.2642924660863,79.310329056666));
#152803=CARTESIAN_POINT('Ctrl Pts',(18.415340634275,21.3609794135845,79.2457952426512));
#152804=CARTESIAN_POINT('Ctrl Pts',(18.3136670380584,21.4620112568094,79.1816539740263));
#152805=CARTESIAN_POINT('Ctrl Pts',(18.2152299323709,21.567120184169,79.1181241093975));
#152806=CARTESIAN_POINT('Ctrl Pts',(18.0246947079353,21.7705694112136,78.9951554693622));
#152807=CARTESIAN_POINT('Ctrl Pts',(17.8462319408475,21.9893610467865,78.8744409174966));
#152808=CARTESIAN_POINT('Ctrl Pts',(17.6828842429067,22.2213279990028,78.7577319097057));
#152809=CARTESIAN_POINT('Ctrl Pts',(17.635159449823,22.2891010679615,78.7236333988724));
#152810=CARTESIAN_POINT('Ctrl Pts',(17.5887247601207,22.3579984909406,78.6898768065634));
#152811=CARTESIAN_POINT('Ctrl Pts',(17.5436556307801,22.4279655044851,78.6565057690561));
#152812=CARTESIAN_POINT('Ctrl Pts',(17.5433331744752,22.4284660977953,78.6562670091422));
#152813=CARTESIAN_POINT('Ctrl Pts',(17.5430107883002,22.4289667455025,78.6560282691331));
#152814=CARTESIAN_POINT('Ctrl Pts',(17.5426884722822,22.4294674475864,78.6557895490448));
#152815=CARTESIAN_POINT('Ctrl Pts',(17.3892006190096,22.6679032797583,78.5421103278949));
#152816=CARTESIAN_POINT('Ctrl Pts',(17.2516260865013,22.91867136202,78.4329499479108));
#152817=CARTESIAN_POINT('Ctrl Pts',(17.1308164024521,23.1779493409036,78.3294294576132));
#152818=CARTESIAN_POINT('Ctrl Pts',(17.0950583166704,23.2546922302106,78.2987887469669));
#152819=CARTESIAN_POINT('Ctrl Pts',(17.0607686562475,23.3321805774696,78.2686420158084));
#152820=CARTESIAN_POINT('Ctrl Pts',(17.0279686886132,23.4103151652504,78.2390179986263));
#152821=CARTESIAN_POINT('Ctrl Pts',(16.9418410159583,23.6154845810995,78.1612298836188));
#152822=CARTESIAN_POINT('Ctrl Pts',(16.8659609336768,23.8251558422008,78.0870264878607));
#152823=CARTESIAN_POINT('Ctrl Pts',(16.8006819883727,24.0377033797527,78.0168806813474));
#152824=CARTESIAN_POINT('Ctrl Pts',(16.7569336799293,24.1801473973206,77.9698707248437));
#152825=CARTESIAN_POINT('Ctrl Pts',(16.7179476188404,24.3238837428768,77.924683472366));
#152826=CARTESIAN_POINT('Ctrl Pts',(16.6838422822653,24.468425051943,77.8814661384565));
#152827=CARTESIAN_POINT('Ctrl Pts',(16.6837151459022,24.4689638666331,77.8813050347933));
#152828=CARTESIAN_POINT('Ctrl Pts',(16.6835880774277,24.4695026922809,77.881143958578));
#152829=CARTESIAN_POINT('Ctrl Pts',(16.6834610768493,24.4700415288566,77.8809829098195));
#152830=CARTESIAN_POINT('Ctrl Pts',(16.6366722700736,24.6685565335379,77.8216502726667));
#152831=CARTESIAN_POINT('Ctrl Pts',(16.5991031763914,24.868555425736,77.7660460631051));
#152832=CARTESIAN_POINT('Ctrl Pts',(16.57030512461,25.0687079639017,77.7142355762191));
#152833=CARTESIAN_POINT('Ctrl Pts',(16.5469232938871,25.2312166225316,77.6721693960747));
#152834=CARTESIAN_POINT('Ctrl Pts',(16.5293224072309,25.3938260497807,77.6326037348469));
#152835=CARTESIAN_POINT('Ctrl Pts',(16.5172392852194,25.5558247763328,77.5955633957734));
#152836=CARTESIAN_POINT('Ctrl Pts',(16.5026188695806,25.7518410635896,77.5507450820837));
#152837=CARTESIAN_POINT('Ctrl Pts',(16.4960688129371,25.9469850810175,77.5096162455846));
#152838=CARTESIAN_POINT('Ctrl Pts',(16.4971157343381,26.140278270034,77.4721624214652));
#152839=CARTESIAN_POINT('Ctrl Pts',(16.4980025980298,26.3040199903037,77.4404346941551));
#152840=CARTESIAN_POINT('Ctrl Pts',(16.5043421206547,26.4664339872537,77.4113445365776));
#152841=CARTESIAN_POINT('Ctrl Pts',(16.5158721328963,26.62691877866,77.3848956136509));
#152842=CARTESIAN_POINT('Ctrl Pts',(1.23275780153909,24.69194692623,92.79547180931));
#152843=CARTESIAN_POINT('Ctrl Pts',(1.99037470125288,25.2226352445827,92.4576622723953));
#152844=CARTESIAN_POINT('Ctrl Pts',(2.75938293298785,25.6890597071317,92.0771176746582));
#152845=CARTESIAN_POINT('Ctrl Pts',(3.92098936528719,26.2923006172496,91.4347419076188));
#152846=CARTESIAN_POINT('Ctrl Pts',(4.30952220315875,26.4773149566713,91.2086956120099));
#152847=CARTESIAN_POINT('Ctrl Pts',(4.8930242498354,26.7307375198775,90.8508771482829));
#152848=CARTESIAN_POINT('Ctrl Pts',(5.18494917491221,26.851424064999,90.6672814614646));
#152849=CARTESIAN_POINT('Ctrl Pts',(5.52553055718069,26.9816817454645,90.4447048347504));
#152850=CARTESIAN_POINT('Ctrl Pts',(5.69578263189675,27.0441747634866,90.3312993469999));
#152851=CARTESIAN_POINT('Ctrl Pts',(5.76873529807879,27.070392666451,90.2822410057258));
#152852=CARTESIAN_POINT('Ctrl Pts',(5.81736715483406,27.0877457530838,90.2494338595921));
#152853=CARTESIAN_POINT('Ctrl Pts',(5.84317307001101,27.0968841603482,90.2319668635416));
#152854=CARTESIAN_POINT('Ctrl Pts',(6.59626022173228,27.3617555700107,89.7207092547717));
#152855=CARTESIAN_POINT('Ctrl Pts',(7.32748827641959,27.5632869808104,89.177216366884));
#152856=CARTESIAN_POINT('Ctrl Pts',(8.41450607645436,27.7826137082458,88.2847550197912));
#152857=CARTESIAN_POINT('Ctrl Pts',(8.77518981053865,27.8418942192636,87.9744085087981));
#152858=CARTESIAN_POINT('Ctrl Pts',(9.31216035509837,27.9100723885993,87.4890121728745));
#152859=CARTESIAN_POINT('Ctrl Pts',(9.57963016181105,27.9389758239694,87.2413462190352));
#152860=CARTESIAN_POINT('Ctrl Pts',(9.88953951596442,27.9636216122967,86.9435958459439));
#152861=CARTESIAN_POINT('Ctrl Pts',(10.0439129722782,27.9736757848926,86.7925060680695));
#152862=CARTESIAN_POINT('Ctrl Pts',(10.12094854271,27.9781356907987,86.7164059576889));
#152863=CARTESIAN_POINT('Ctrl Pts',(10.1539307653767,27.9799255403887,86.6836724838006));
#152864=CARTESIAN_POINT('Ctrl Pts',(10.1759115053255,27.9810917648586,86.6618236740342));
#152865=CARTESIAN_POINT('Ctrl Pts',(10.1882885335909,27.9817317716749,86.6494997130189));
#152866=CARTESIAN_POINT('Ctrl Pts',(10.8118051772457,28.0133025816265,86.0278008089336));
#152867=CARTESIAN_POINT('Ctrl Pts',(11.4271146397258,28.0022536845851,85.3612777556491));
#152868=CARTESIAN_POINT('Ctrl Pts',(12.3365974155725,27.9224793356862,84.2732251185324));
#152869=CARTESIAN_POINT('Ctrl Pts',(12.6374842751345,27.8853543854972,83.8958448105857));
#152870=CARTESIAN_POINT('Ctrl Pts',(13.0832130151965,27.8138667093793,83.3070638705607));
#152871=CARTESIAN_POINT('Ctrl Pts',(13.3046744335626,27.7741728086118,83.0069978057266));
#152872=CARTESIAN_POINT('Ctrl Pts',(13.56008482604,27.7209506479765,82.6468659740776));
#152873=CARTESIAN_POINT('Ctrl Pts',(13.6869844531481,27.6926114152238,82.4642729700953));
#152874=CARTESIAN_POINT('Ctrl Pts',(13.7547418214793,27.6769667854183,82.3657766620698));
#152875=CARTESIAN_POINT('Ctrl Pts',(13.7862995872375,27.6695399470608,82.3196267535338));
#152876=CARTESIAN_POINT('Ctrl Pts',(13.8043171073331,27.665265179563,82.2932100387377));
#152877=CARTESIAN_POINT('Ctrl Pts',(13.8098802979734,27.6639410447168,82.2850451218363));
#152878=CARTESIAN_POINT('Ctrl Pts',(14.2538584320099,27.5580367056132,81.6329789913368));
#152879=CARTESIAN_POINT('Ctrl Pts',(14.7117977987722,27.4191449094803,80.9064250815115));
#152880=CARTESIAN_POINT('Ctrl Pts',(15.6262304717903,27.0737444754176,79.2791922290114));
#152881=CARTESIAN_POINT('Ctrl Pts',(16.0827382847579,26.867235837488,78.3784032011472));
#152882=CARTESIAN_POINT('Ctrl Pts',(16.5158721306991,26.62691877866,77.384895612693));
#152883=CARTESIAN_POINT('Origin',(-10.9843331791359,-92.5,65.395787724084));
#152884=CARTESIAN_POINT('Origin',(-10.9843331791359,92.,65.395787724084));
#152885=CARTESIAN_POINT('Origin',(-10.9843331791359,-92.5,80.581991049076));
#152886=CARTESIAN_POINT('Origin',(-10.9843331791359,92.,80.581991049076));
#152887=CARTESIAN_POINT('',(9.66896668869965,27.5617702389202,58.8232869212091));
#152888=CARTESIAN_POINT('Ctrl Pts',(16.5158747359332,25.68037166863,68.59288913751));
#152889=CARTESIAN_POINT('Ctrl Pts',(16.4459098082595,25.7023664947635,68.4324058857396));
#152890=CARTESIAN_POINT('Ctrl Pts',(16.3708016848024,25.7264355825049,68.2638291090571));
#152891=CARTESIAN_POINT('Ctrl Pts',(16.2900924916398,25.7526220639059,68.087416378764));
#152892=CARTESIAN_POINT('Ctrl Pts',(16.2145217776279,25.777141341319,67.9222352455293));
#152893=CARTESIAN_POINT('Ctrl Pts',(16.1340400901703,25.8035174070722,67.7501844193478));
#152894=CARTESIAN_POINT('Ctrl Pts',(16.0482330249535,25.8317680994321,67.5715021767688));
#152895=CARTESIAN_POINT('Ctrl Pts',(15.9641112558687,25.8594639332562,67.3963293479136));
#152896=CARTESIAN_POINT('Ctrl Pts',(15.8748711423744,25.8889619931436,67.2147830510035));
#152897=CARTESIAN_POINT('Ctrl Pts',(15.7800870845148,25.9202546953833,67.0271128863405));
#152898=CARTESIAN_POINT('Ctrl Pts',(15.6882391434718,25.9505780465384,66.84525616266));
#152899=CARTESIAN_POINT('Ctrl Pts',(15.5911852428945,25.9825869923839,66.6576491436249));
#152900=CARTESIAN_POINT('Ctrl Pts',(15.4885068102668,26.0162448440536,66.4645421677599));
#152901=CARTESIAN_POINT('Ctrl Pts',(15.4589311972375,26.0259396900978,66.4089194138352));
#152902=CARTESIAN_POINT('Ctrl Pts',(15.4288887343077,26.0357711263778,66.3528404898641));
#152903=CARTESIAN_POINT('Ctrl Pts',(15.3983689445526,26.0457377209224,66.2963117436976));
#152904=CARTESIAN_POINT('Ctrl Pts',(15.2935013134504,26.0799834732175,66.1020759462948));
#152905=CARTESIAN_POINT('Ctrl Pts',(15.1830052612199,26.1158519036328,65.9025373029214));
#152906=CARTESIAN_POINT('Ctrl Pts',(15.0664620478353,26.1533704672762,65.6980085872791));
#152907=CARTESIAN_POINT('Ctrl Pts',(14.9532564079349,26.1898145714161,65.4993371806836));
#152908=CARTESIAN_POINT('Ctrl Pts',(14.8343448523761,26.2278159253131,65.2959575066244));
#152909=CARTESIAN_POINT('Ctrl Pts',(14.7093219885693,26.2673607483818,65.0881773775743));
#152910=CARTESIAN_POINT('Ctrl Pts',(14.6706560100771,26.2795908255989,65.0239169554696));
#152911=CARTESIAN_POINT('Ctrl Pts',(14.6314053420285,26.2919682299591,64.9592357867873));
#152912=CARTESIAN_POINT('Ctrl Pts',(14.5915575904957,26.3044917041774,64.8941433845765));
#152913=CARTESIAN_POINT('Ctrl Pts',(14.4642369251658,26.3445064354577,64.6861615628025));
#152914=CARTESIAN_POINT('Ctrl Pts',(14.330824459311,26.3860287580984,64.4739844034523));
#152915=CARTESIAN_POINT('Ctrl Pts',(14.1909215845456,26.429062909699,64.2579613569774));
#152916=CARTESIAN_POINT('Ctrl Pts',(14.1652678660448,26.4369539985199,64.2183496303904));
#152917=CARTESIAN_POINT('Ctrl Pts',(14.1393958721347,26.4448957968062,64.1786086419067));
#152918=CARTESIAN_POINT('Ctrl Pts',(14.1133030877435,26.4528881597977,64.1387406151485));
#152919=CARTESIAN_POINT('Ctrl Pts',(14.0291080325024,26.4786775670719,64.0100962104369));
#152920=CARTESIAN_POINT('Ctrl Pts',(13.9426145712807,26.5049953038812,63.8801294315358));
#152921=CARTESIAN_POINT('Ctrl Pts',(13.8537392943827,26.5318413543076,63.7489197144917));
#152922=CARTESIAN_POINT('Ctrl Pts',(13.8093016559336,26.5452643795209,63.6833148559696));
#152923=CARTESIAN_POINT('Ctrl Pts',(13.7642685318244,26.5588194830634,63.6173992890108));
#152924=CARTESIAN_POINT('Ctrl Pts',(13.7186295371029,26.5725066620024,63.5511834160091));
#152925=CARTESIAN_POINT('Ctrl Pts',(13.6958100397421,26.5793502514719,63.5180754795082));
#152926=CARTESIAN_POINT('Ctrl Pts',(13.6728390729451,26.5862268597882,63.4848924679298));
#152927=CARTESIAN_POINT('Ctrl Pts',(13.6497153358115,26.5931364865593,63.4516357011427));
#152928=CARTESIAN_POINT('Ctrl Pts',(13.6282808843813,26.5995413361981,63.4208084802527));
#152929=CARTESIAN_POINT('Ctrl Pts',(13.6074099997462,26.6057675296784,63.3909096946062));
#152930=CARTESIAN_POINT('Ctrl Pts',(13.5851694912851,26.6123907729804,63.3591823036636));
#152931=CARTESIAN_POINT('Ctrl Pts',(13.5834166788512,26.6129127620902,63.3566818138283));
#152932=CARTESIAN_POINT('Ctrl Pts',(13.5816553376048,26.6134372177213,63.3541699818618));
#152933=CARTESIAN_POINT('Ctrl Pts',(13.5798845098451,26.6139644218352,63.3516454664426));
#152934=CARTESIAN_POINT('Ctrl Pts',(13.4348263677831,26.6571505808716,63.144848665166));
#152935=CARTESIAN_POINT('Ctrl Pts',(13.2906713269679,26.6991517299152,62.9449804241607));
#152936=CARTESIAN_POINT('Ctrl Pts',(13.1478211692805,26.7398786761325,62.7518015164918));
#152937=CARTESIAN_POINT('Ctrl Pts',(13.0019686553813,26.7814616018036,62.5545624670433));
#152938=CARTESIAN_POINT('Ctrl Pts',(12.8574765519758,26.8217164212871,62.3642968595557));
#152939=CARTESIAN_POINT('Ctrl Pts',(12.7147524235516,26.8605974413362,62.1807611240509));
#152940=CARTESIAN_POINT('Ctrl Pts',(12.5673203685204,26.9007609984785,61.9911712421167));
#152941=CARTESIAN_POINT('Ctrl Pts',(12.4217750071565,26.9394588097394,61.8087624702855));
#152942=CARTESIAN_POINT('Ctrl Pts',(12.278542312745,26.9766895356588,61.6332788391071));
#152943=CARTESIAN_POINT('Ctrl Pts',(12.1323852990195,27.0146803850356,61.4542124353357));
#152944=CARTESIAN_POINT('Ctrl Pts',(11.9886364670197,27.0511439628675,61.2823567753943));
#152945=CARTESIAN_POINT('Ctrl Pts',(11.8477225193739,27.0861249741561,61.1174536620441));
#152946=CARTESIAN_POINT('Ctrl Pts',(11.7027389237983,27.1221162502378,60.9477880846151));
#152947=CARTESIAN_POINT('Ctrl Pts',(11.5607564832687,27.1565384199676,60.7854823417614));
#152948=CARTESIAN_POINT('Ctrl Pts',(11.4222105981809,27.1894834912378,60.6302708610468));
#152949=CARTESIAN_POINT('Ctrl Pts',(11.4111877277838,27.1921046391023,60.6179220566419));
#152950=CARTESIAN_POINT('Ctrl Pts',(11.4001865949999,27.1947164574398,60.6056181671864));
#152951=CARTESIAN_POINT('Ctrl Pts',(11.3892074109533,27.1973190029251,60.5933590633205));
#152952=CARTESIAN_POINT('Ctrl Pts',(11.2465292019462,27.2311399614894,60.4340478634905));
#152953=CARTESIAN_POINT('Ctrl Pts',(11.1075447488207,27.2633192232488,60.2822800986382));
#152954=CARTESIAN_POINT('Ctrl Pts',(10.9726453414288,27.2938212954465,60.1377288074397));
#152955=CARTESIAN_POINT('Ctrl Pts',(10.8339787621069,27.3251751619732,59.9891408078731));
#152956=CARTESIAN_POINT('Ctrl Pts',(10.6996286506066,27.3547572947639,59.848177795414));
#152957=CARTESIAN_POINT('Ctrl Pts',(10.5699800376746,27.3825557890386,59.7145119675845));
#152958=CARTESIAN_POINT('Ctrl Pts',(10.4387257766684,27.4106985569448,59.5791907400234));
#152959=CARTESIAN_POINT('Ctrl Pts',(10.3122901776469,27.4370137383686,59.4513484768771));
#152960=CARTESIAN_POINT('Ctrl Pts',(10.1910319724966,27.4615085851807,59.3306744916551));
#152961=CARTESIAN_POINT('Ctrl Pts',(10.0681689845437,27.4863276072424,59.2084034554462));
#152962=CARTESIAN_POINT('Ctrl Pts',(9.95062134681771,27.509278282649,59.0934916163665));
#152963=CARTESIAN_POINT('Ctrl Pts',(9.83872060946937,27.5303805812036,58.985647044844));
#152964=CARTESIAN_POINT('Ctrl Pts',(9.78059920408066,27.5413411457002,58.9296324178723));
#152965=CARTESIAN_POINT('Ctrl Pts',(9.72400052762142,27.5518032151801,58.8755249005202));
#152966=CARTESIAN_POINT('Ctrl Pts',(9.66896668055068,27.5617702389205,58.8232869297943));
#152967=CARTESIAN_POINT('Ctrl Pts',(1.23275780212867,24.13180332306,53.1823069641179));
#152968=CARTESIAN_POINT('Ctrl Pts',(1.24922759706115,24.1480653974204,53.1896505883185));
#152969=CARTESIAN_POINT('Ctrl Pts',(1.27440967752685,24.1734031842924,53.2008913260592));
#152970=CARTESIAN_POINT('Ctrl Pts',(1.3085221121756,24.2072241748601,53.2162148169485));
#152971=CARTESIAN_POINT('Ctrl Pts',(1.34067084263351,24.2390982384025,53.2306562012515));
#152972=CARTESIAN_POINT('Ctrl Pts',(1.38075131620029,24.2785069351784,53.2487240377262));
#152973=CARTESIAN_POINT('Ctrl Pts',(1.42892482678689,24.3249543034778,53.2706193208307));
#152974=CARTESIAN_POINT('Ctrl Pts',(1.47640302832188,24.3707312768816,53.2921985798726));
#152975=CARTESIAN_POINT('Ctrl Pts',(1.53174246303046,24.4233452037699,53.317495505027));
#152976=CARTESIAN_POINT('Ctrl Pts',(1.5950753971386,24.4823212892496,53.3467477075681));
#152977=CARTESIAN_POINT('Ctrl Pts',(1.65719135552206,24.5401641181484,53.3754378136125));
#152978=CARTESIAN_POINT('Ctrl Pts',(1.7269966919911,24.6041269503153,53.4079326235042));
#152979=CARTESIAN_POINT('Ctrl Pts',(1.80459287974523,24.6737618385938,53.4445009245182));
#152980=CARTESIAN_POINT('Ctrl Pts',(1.82314049055782,24.6904064811227,53.4532417484545));
#152981=CARTESIAN_POINT('Ctrl Pts',(1.84213311292883,24.7073751913143,53.4622155123241));
#152982=CARTESIAN_POINT('Ctrl Pts',(1.86157191681418,24.7246618517312,53.4714262769093));
#152983=CARTESIAN_POINT('Ctrl Pts',(1.93892890328496,24.7934543537738,53.50808064081));
#152984=CARTESIAN_POINT('Ctrl Pts',(2.02341605629018,24.8671314325845,53.5485142421835));
#152985=CARTESIAN_POINT('Ctrl Pts',(2.11519799494867,24.9449326669951,53.5930621518562));
#152986=CARTESIAN_POINT('Ctrl Pts',(2.20469853691352,25.0208000189715,53.6365027472214));
#152987=CARTESIAN_POINT('Ctrl Pts',(2.30113587746158,25.1005890488324,53.6838556337299));
#152988=CARTESIAN_POINT('Ctrl Pts',(2.40463675923085,25.183594642293,53.7354738822346));
#152989=CARTESIAN_POINT('Ctrl Pts',(2.43996923889309,25.2119305694142,53.7530949950629));
#152990=CARTESIAN_POINT('Ctrl Pts',(2.47612463805057,25.2406413420158,53.7712135484868));
#152991=CARTESIAN_POINT('Ctrl Pts',(2.51310722943784,25.2696989090092,53.7898447666857));
#152992=CARTESIAN_POINT('Ctrl Pts',(2.61818119077468,25.3522565004673,53.8427792914785));
#152993=CARTESIAN_POINT('Ctrl Pts',(2.72993999096494,25.4375824234251,53.8998518017394));
#152994=CARTESIAN_POINT('Ctrl Pts',(2.84847168809193,25.5248859158878,53.9614442946384));
#152995=CARTESIAN_POINT('Ctrl Pts',(2.87456719151849,25.5441063323834,53.9750042718298));
#152996=CARTESIAN_POINT('Ctrl Pts',(2.90099085274009,25.5634225993189,53.9887834894792));
#152997=CARTESIAN_POINT('Ctrl Pts',(2.92774340859437,25.5828262786981,54.002786301433));
#152998=CARTESIAN_POINT('Ctrl Pts',(3.00187777568457,25.6365960754173,54.0415896818401));
#152999=CARTESIAN_POINT('Ctrl Pts',(3.07853802377204,25.6910344099707,54.0821095823487));
#153000=CARTESIAN_POINT('Ctrl Pts',(3.15773517204983,25.7459457441527,54.1244419798521));
#153001=CARTESIAN_POINT('Ctrl Pts',(3.19733374618873,25.7734014112436,54.1456081786038));
#153002=CARTESIAN_POINT('Ctrl Pts',(3.23756648761963,25.8009753282418,54.1672276054822));
#153003=CARTESIAN_POINT('Ctrl Pts',(3.27843408473616,25.8286418990266,54.1893127087366));
#153004=CARTESIAN_POINT('Ctrl Pts',(3.29886788329442,25.842475184419,54.2003552603638));
#153005=CARTESIAN_POINT('Ctrl Pts',(3.31946039210981,25.8563316332581,54.2115142377327));
#153006=CARTESIAN_POINT('Ctrl Pts',(3.34021167400882,25.8702079929798,54.2227912366719));
#153007=CARTESIAN_POINT('Ctrl Pts',(3.35058731495833,25.8771461728407,54.2284297361415));
#153008=CARTESIAN_POINT('Ctrl Pts',(3.36100264894217,25.8840893304222,54.2340977414226));
#153009=CARTESIAN_POINT('Ctrl Pts',(3.37145768859112,25.8910370435328,54.239795457932));
#153010=CARTESIAN_POINT('Ctrl Pts',(3.37668520841559,25.8945109000882,54.2426443161867));
#153011=CARTESIAN_POINT('Ctrl Pts',(3.3819226546413,25.8979858955258,54.2455006022758));
#153012=CARTESIAN_POINT('Ctrl Pts',(3.3871700281858,25.9014619775766,54.2483643417282));
#153013=CARTESIAN_POINT('Ctrl Pts',(3.38979371495805,25.903200018602,54.2497962114543));
#153014=CARTESIAN_POINT('Ctrl Pts',(3.39241988355906,25.9049383312807,54.251229944523));
#153015=CARTESIAN_POINT('Ctrl Pts',(3.39504853411381,25.9066769090288,54.2526655441441));
#153016=CARTESIAN_POINT('Ctrl Pts',(3.39767718466856,25.908415486777,54.2541011437651));
#153017=CARTESIAN_POINT('Ctrl Pts',(3.40151786624113,25.9109530525223,54.2561996586179));
#153018=CARTESIAN_POINT('Ctrl Pts',(3.40294193175905,25.9118934308925,54.2569779458803));
#153019=CARTESIAN_POINT('Ctrl Pts',(3.65218015250606,26.0764773133412,54.3931928391448));
#153020=CARTESIAN_POINT('Ctrl Pts',(3.90334231127312,26.2298342139882,54.535060473175));
#153021=CARTESIAN_POINT('Ctrl Pts',(4.15573981610667,26.371901834692,54.6826051548366));
#153022=CARTESIAN_POINT('Ctrl Pts',(4.27252416903728,26.4376365382392,54.7508740950845));
#153023=CARTESIAN_POINT('Ctrl Pts',(4.38957306574967,26.5009543041443,54.8203577276091));
#153024=CARTESIAN_POINT('Ctrl Pts',(4.5068187742771,26.5618489611465,54.8910546870773));
#153025=CARTESIAN_POINT('Ctrl Pts',(4.69213892805981,26.6580998801944,55.0027992580741));
#153026=CARTESIAN_POINT('Ctrl Pts',(4.87795159594536,26.748297190703,55.1175764440731));
#153027=CARTESIAN_POINT('Ctrl Pts',(5.06399849957787,26.8324173905609,55.2353729249555));
#153028=CARTESIAN_POINT('Ctrl Pts',(5.15702195139412,26.8744774904898,55.2942711653967));
#153029=CARTESIAN_POINT('Ctrl Pts',(5.25010413704565,26.915018312756,55.3539240772649));
#153030=CARTESIAN_POINT('Ctrl Pts',(5.34321355468929,26.9540369872704,55.4143289078529));
#153031=CARTESIAN_POINT('Ctrl Pts',(5.38976826351112,26.9735463245276,55.4445313231469));
#153032=CARTESIAN_POINT('Ctrl Pts',(5.43632979261359,26.9926751248468,55.474921709351));
#153033=CARTESIAN_POINT('Ctrl Pts',(5.48289426716108,27.0114230236912,55.5054996630802));
#153034=CARTESIAN_POINT('Ctrl Pts',(5.50617650443482,27.0207969731135,55.5207886399447));
#153035=CARTESIAN_POINT('Ctrl Pts',(5.52945947903618,27.030075697167,55.5361245084827));
#153036=CARTESIAN_POINT('Ctrl Pts',(5.55274255826553,27.0392587624797,55.5515071133737));
#153037=CARTESIAN_POINT('Ctrl Pts',(5.57444917700966,27.0478200569581,55.5658481864068));
#153038=CARTESIAN_POINT('Ctrl Pts',(5.59767411521259,27.0568843890177,55.581238267158));
#153039=CARTESIAN_POINT('Ctrl Pts',(5.61817054560409,27.0648119703249,55.5948569583085));
#153040=CARTESIAN_POINT('Ctrl Pts',(5.61965911519574,27.0653877172352,55.5958460266066));
#153041=CARTESIAN_POINT('Ctrl Pts',(5.6211333058231,27.0659574683464,55.5968257327792));
#153042=CARTESIAN_POINT('Ctrl Pts',(5.62259149634526,27.0665205955125,55.5977949879077));
#153043=CARTESIAN_POINT('Ctrl Pts',(5.84891017131741,27.1539208303596,55.7482283730251));
#153044=CARTESIAN_POINT('Ctrl Pts',(6.07562464989286,27.2324148761963,55.9033636707012));
#153045=CARTESIAN_POINT('Ctrl Pts',(6.3021361807368,27.3015027510538,56.0630600554502));
#153046=CARTESIAN_POINT('Ctrl Pts',(6.53375524878111,27.3721484666517,56.2263573837045));
#153047=CARTESIAN_POINT('Ctrl Pts',(6.76516172690714,27.4329590351902,56.3944240383909));
#153048=CARTESIAN_POINT('Ctrl Pts',(6.9957374952623,27.4833998845232,56.5670569758031));
#153049=CARTESIAN_POINT('Ctrl Pts',(7.22631326361745,27.5338407338561,56.7396899132153));
#153050=CARTESIAN_POINT('Ctrl Pts',(7.45605801145856,27.5739118639835,56.9168891151683));
#153051=CARTESIAN_POINT('Ctrl Pts',(7.6843805945019,27.6030787027589,57.0983983503856));
#153052=CARTESIAN_POINT('Ctrl Pts',(7.89040519895813,27.6293971086821,57.2621813975653));
#153053=CARTESIAN_POINT('Ctrl Pts',(8.09526409678687,27.6468405362001,57.4294678871763));
#153054=CARTESIAN_POINT('Ctrl Pts',(8.29846844405858,27.655078180412,57.5999641245306));
#153055=CARTESIAN_POINT('Ctrl Pts',(8.5012141214738,27.6632972307349,57.7700755202919));
#153056=CARTESIAN_POINT('Ctrl Pts',(8.70231251363328,27.662352009166,57.9433820782813));
#153057=CARTESIAN_POINT('Ctrl Pts',(8.90130878651381,27.6519139458157,58.1195503176241));
#153058=CARTESIAN_POINT('Ctrl Pts',(9.1000757923728,27.6414879083373,58.2955155905145));
#153059=CARTESIAN_POINT('Ctrl Pts',(9.29674534304399,27.6215908902089,58.4743358168237));
#153060=CARTESIAN_POINT('Ctrl Pts',(9.4908976461116,27.591895455886,58.6556388067892));
#153061=CARTESIAN_POINT('Ctrl Pts',(9.55049475305616,27.5827801276249,58.7112916809072));
#153062=CARTESIAN_POINT('Ctrl Pts',(9.60985492117232,27.5727415454755,58.7671782174972));
#153063=CARTESIAN_POINT('Ctrl Pts',(9.66896668003918,27.56177023892,58.8232869303331));
#153064=CARTESIAN_POINT('Ctrl Pts',(1.02018651496909,24.12736861615,53.08644276134));
#153065=CARTESIAN_POINT('Ctrl Pts',(1.28010839926909,23.74963944379,53.21264495039));
#153066=CARTESIAN_POINT('Ctrl Pts',(1.69372155058909,23.19034260218,53.33423556322));
#153067=CARTESIAN_POINT('Ctrl Pts',(2.28532636027909,22.4683497999,53.36025868992));
#153068=CARTESIAN_POINT('Ctrl Pts',(2.72064084369909,21.96878201391,53.31931450845));
#153069=CARTESIAN_POINT('Ctrl Pts',(3.16680680853909,21.48749253734,53.21907255652));
#153070=CARTESIAN_POINT('Ctrl Pts',(3.80379334035909,20.84237217285,52.99629044043));
#153071=CARTESIAN_POINT('Ctrl Pts',(4.28807530375909,20.4025094424,52.73095649241));
#153072=CARTESIAN_POINT('Ctrl Pts',(4.61113719324909,20.13148505149,52.51146626848));
#153073=CARTESIAN_POINT('Ctrl Pts',(1.72739619405909,24.87088028168,53.3946519969));
#153074=CARTESIAN_POINT('Ctrl Pts',(1.98016437202909,24.43764203493,53.52791146856));
#153075=CARTESIAN_POINT('Ctrl Pts',(2.39170334478909,23.79368517934,53.64972059236));
#153076=CARTESIAN_POINT('Ctrl Pts',(2.99363132225909,22.96415595654,53.65205971503));
#153077=CARTESIAN_POINT('Ctrl Pts',(3.44088690595909,22.39235728434,53.58369970474));
#153078=CARTESIAN_POINT('Ctrl Pts',(3.90240318107909,21.84503415371,53.44568945113));
#153079=CARTESIAN_POINT('Ctrl Pts',(4.56392990621909,21.11826512872,53.15625082403));
#153080=CARTESIAN_POINT('Ctrl Pts',(5.06794995464909,20.63347851478,52.82593298942));
#153081=CARTESIAN_POINT('Ctrl Pts',(5.40276176874909,20.34145978504,52.55843576862));
#153082=CARTESIAN_POINT('Ctrl Pts',(3.17914527510909,26.09640831234,54.09413185087));
#153083=CARTESIAN_POINT('Ctrl Pts',(3.40222081686909,25.56141982058,54.23518571775));
#153084=CARTESIAN_POINT('Ctrl Pts',(3.78905928284909,24.75971584166,54.348934864));
#153085=CARTESIAN_POINT('Ctrl Pts',(4.39075430025909,23.73217540148,54.29225680523));
#153086=CARTESIAN_POINT('Ctrl Pts',(4.84985111793909,23.03008574148,54.16070223457));
#153087=CARTESIAN_POINT('Ctrl Pts',(5.33269502402909,22.36806245594,53.93909869207));
#153088=CARTESIAN_POINT('Ctrl Pts',(6.03347108353909,21.50817639152,53.50650311147));
#153089=CARTESIAN_POINT('Ctrl Pts',(6.57305116340909,20.96447914599,53.04243066886));
#153090=CARTESIAN_POINT('Ctrl Pts',(6.92979819842909,20.65505525241,52.68021892232));
#153091=CARTESIAN_POINT('Ctrl Pts',(5.43493315155909,27.31689412349,55.42149232346));
#153092=CARTESIAN_POINT('Ctrl Pts',(5.57886835666909,26.65149635406,55.54636262511));
#153093=CARTESIAN_POINT('Ctrl Pts',(5.88091137179909,25.6387335644,55.60927396635));
#153094=CARTESIAN_POINT('Ctrl Pts',(6.44001219137909,24.35121556071,55.41502290768));
#153095=CARTESIAN_POINT('Ctrl Pts',(6.89713355269909,23.48579054893,55.15603975691));
#153096=CARTESIAN_POINT('Ctrl Pts',(7.40256384026909,22.69322035286,54.78097445767));
#153097=CARTESIAN_POINT('Ctrl Pts',(8.16206876439909,21.708389665,54.1053488272));
#153098=CARTESIAN_POINT('Ctrl Pts',(8.76799204153909,21.15393359669,53.44033099395));
#153099=CARTESIAN_POINT('Ctrl Pts',(9.16935658079909,20.87624188168,52.95149370635));
#153100=CARTESIAN_POINT('Ctrl Pts',(7.68979117344909,27.96384357157,57.042983249));
#153101=CARTESIAN_POINT('Ctrl Pts',(7.72330678673909,27.18890190058,57.11221136924));
#153102=CARTESIAN_POINT('Ctrl Pts',(7.89618292747909,25.99000196864,57.067606522));
#153103=CARTESIAN_POINT('Ctrl Pts',(8.38110448977909,24.47966951747,56.66954723005));
#153104=CARTESIAN_POINT('Ctrl Pts',(8.82812186513909,23.48367508624,56.24292428671));
#153105=CARTESIAN_POINT('Ctrl Pts',(9.36273061159909,22.60305442893,55.68503473905));
#153106=CARTESIAN_POINT('Ctrl Pts',(10.2085995213291,21.56855669904,54.74658540708));
#153107=CARTESIAN_POINT('Ctrl Pts',(10.9188216964491,21.07709473119,53.90000039928));
#153108=CARTESIAN_POINT('Ctrl Pts',(11.3923064424291,20.88050279146,53.31616956596));
#153109=CARTESIAN_POINT('Ctrl Pts',(9.13342233188909,27.94957487251,58.2979440507));
#153110=CARTESIAN_POINT('Ctrl Pts',(9.08106830642909,27.12604219688,58.29819803193));
#153111=CARTESIAN_POINT('Ctrl Pts',(9.14758840929909,25.83611398064,58.13417901149));
#153112=CARTESIAN_POINT('Ctrl Pts',(9.57241865212909,24.22058009908,57.54766571695));
#153113=CARTESIAN_POINT('Ctrl Pts',(10.0146980747891,23.17051685142,56.98046127077));
#153114=CARTESIAN_POINT('Ctrl Pts',(10.5806282235291,22.26779541216,56.28459372418));
#153115=CARTESIAN_POINT('Ctrl Pts',(11.5120991780291,21.25642831637,55.17124635962));
#153116=CARTESIAN_POINT('Ctrl Pts',(12.3210049830591,20.85107620434,54.23646469467));
#153117=CARTESIAN_POINT('Ctrl Pts',(12.8602418793091,20.73195002337,53.62410434214));
#153118=CARTESIAN_POINT('Ctrl Pts',(9.83727978500909,27.81219977272,58.97626003861));
#153119=CARTESIAN_POINT('Ctrl Pts',(9.73949458818909,26.97238804509,58.93119606197));
#153120=CARTESIAN_POINT('Ctrl Pts',(9.74858544025909,25.64882808166,58.69043954903));
#153121=CARTESIAN_POINT('Ctrl Pts',(10.1431268412991,23.99629606828,57.99131379478));
#153122=CARTESIAN_POINT('Ctrl Pts',(10.5860577947591,22.93050615594,57.34439895311));
#153123=CARTESIAN_POINT('Ctrl Pts',(11.1738219636591,22.02828425791,56.57543834793));
#153124=CARTESIAN_POINT('Ctrl Pts',(12.1599880660491,21.0444542549,55.37786778629));
#153125=CARTESIAN_POINT('Ctrl Pts',(13.0285934306291,20.6920670675,54.41291434299));
#153126=CARTESIAN_POINT('Ctrl Pts',(13.6062929436291,20.61550204861,53.7987131345));
#153127=CARTESIAN_POINT('Ctrl Pts',(4.64898302763928,20.2571697908605,52.5914041824882));
#153128=CARTESIAN_POINT('Ctrl Pts',(4.37640638855581,20.4917590865083,52.7746243664382));
#153129=CARTESIAN_POINT('Ctrl Pts',(4.09631448667638,20.7498815758729,52.9317573917127));
#153130=CARTESIAN_POINT('Ctrl Pts',(3.81504798690012,21.0269126271465,53.0570185057454));
#153131=CARTESIAN_POINT('Ctrl Pts',(3.79438846371867,21.0472610491246,53.066219156698));
#153132=CARTESIAN_POINT('Ctrl Pts',(3.77372260637565,21.0677114719799,53.0752478720827));
#153133=CARTESIAN_POINT('Ctrl Pts',(3.75305292839587,21.0882620568661,53.0841023688874));
#153134=CARTESIAN_POINT('Ctrl Pts',(3.75282391110331,21.0884897546229,53.0842004755385));
#153135=CARTESIAN_POINT('Ctrl Pts',(3.7525948933306,21.0887174646872,53.0842985608067));
#153136=CARTESIAN_POINT('Ctrl Pts',(3.75236587508114,21.0889451870564,53.084396624689));
#153137=CARTESIAN_POINT('Ctrl Pts',(3.60121378324409,21.2392419976695,53.1491188072116));
#153138=CARTESIAN_POINT('Ctrl Pts',(3.44985401812235,21.3948988306987,53.2045252912585));
#153139=CARTESIAN_POINT('Ctrl Pts',(3.29935834752775,21.5548974467013,53.2500701259441));
#153140=CARTESIAN_POINT('Ctrl Pts',(3.14931819963736,21.7144117763325,53.2954771047951));
#153141=CARTESIAN_POINT('Ctrl Pts',(3.00013691813682,21.8782416497902,53.331082045352));
#153142=CARTESIAN_POINT('Ctrl Pts',(2.85285330004476,22.0452897893958,53.3565571956255));
#153143=CARTESIAN_POINT('Ctrl Pts',(2.85240650238333,22.0457965444517,53.3566344767088));
#153144=CARTESIAN_POINT('Ctrl Pts',(2.85195972219237,22.0463033291172,53.3567116645701));
#153145=CARTESIAN_POINT('Ctrl Pts',(2.85151295950087,22.0468101433616,53.3567887592001));
#153146=CARTESIAN_POINT('Ctrl Pts',(2.70379463414956,22.2143840094626,53.3822794500264));
#153147=CARTESIAN_POINT('Ctrl Pts',(2.55798942099489,22.3851915508815,53.3975777418528));
#153148=CARTESIAN_POINT('Ctrl Pts',(2.41508772742532,22.5580263962415,53.4026635334286));
#153149=CARTESIAN_POINT('Ctrl Pts',(2.27218603385641,22.7308612416006,53.4077493250044));
#153150=CARTESIAN_POINT('Ctrl Pts',(2.13218785948827,22.905723390667,53.4026226173359));
#153151=CARTESIAN_POINT('Ctrl Pts',(1.99602497078142,23.0813571917986,53.3874847959142));
#153152=CARTESIAN_POINT('Ctrl Pts',(1.72451941585065,23.4315668054,53.3573003407768));
#153153=CARTESIAN_POINT('Ctrl Pts',(1.468262734854,23.7848444098977,53.2873123215654));
#153154=CARTESIAN_POINT('Ctrl Pts',(1.23275780652318,24.13180332306,53.1823069542621));
#153155=CARTESIAN_POINT('Ctrl Pts',(13.2725929185091,20.67124111202,53.96044066964));
#153156=CARTESIAN_POINT('Ctrl Pts',(12.7601005265309,20.7790383531423,54.5170917113046));
#153157=CARTESIAN_POINT('Ctrl Pts',(12.2365830640386,21.0202700835715,55.1059943501782));
#153158=CARTESIAN_POINT('Ctrl Pts',(11.5144024001356,21.6082528697978,55.9578487963725));
#153159=CARTESIAN_POINT('Ctrl Pts',(11.284484943989,21.8411904407848,56.2361257836112));
#153160=CARTESIAN_POINT('Ctrl Pts',(10.8600882151825,22.3745190753888,56.7657768656355));
#153161=CARTESIAN_POINT('Ctrl Pts',(10.6656891171808,22.6748728094781,57.017060721281));
#153162=CARTESIAN_POINT('Ctrl Pts',(10.3235697698876,23.3290339756505,57.4787180816328));
#153163=CARTESIAN_POINT('Ctrl Pts',(10.1759004486617,23.6827440137225,57.6890228698567));
#153164=CARTESIAN_POINT('Ctrl Pts',(9.93366676041426,24.4240678546045,58.0589285287306));
#153165=CARTESIAN_POINT('Ctrl Pts',(9.83910660616593,24.8115576094456,58.2185057763796));
#153166=CARTESIAN_POINT('Ctrl Pts',(9.63618653282326,25.9924390190698,58.6150020729616));
#153167=CARTESIAN_POINT('Ctrl Pts',(9.61024456763422,26.8018116088772,58.7675633910135));
#153168=CARTESIAN_POINT('Ctrl Pts',(9.66896670550909,27.56177023892,58.8232869035));
#153169=CARTESIAN_POINT('Ctrl Pts',(20.3787275855491,19.18666345688,66.379741082483));
#153170=CARTESIAN_POINT('Ctrl Pts',(17.8361393017991,20.29619101201,67.595084209341));
#153171=CARTESIAN_POINT('Ctrl Pts',(16.3981991143491,22.80777792279,68.487957490196));
#153172=CARTESIAN_POINT('Ctrl Pts',(16.5807046766691,25.82061478888,68.738094180426));
#153173=CARTESIAN_POINT('Ctrl Pts',(18.6376929650191,19.57899817903,61.58547060068));
#153174=CARTESIAN_POINT('Ctrl Pts',(16.0482537547891,20.58406629994,63.2181484680071));
#153175=CARTESIAN_POINT('Ctrl Pts',(14.6296236331391,23.17807550392,64.49719057205));
#153176=CARTESIAN_POINT('Ctrl Pts',(14.9395338453091,26.34133394336,64.919770175413));
#153177=CARTESIAN_POINT('Ctrl Pts',(16.2689157983691,20.24291980593,57.34617439044));
#153178=CARTESIAN_POINT('Ctrl Pts',(13.5272592236191,21.02524550693,59.47841963262));
#153179=CARTESIAN_POINT('Ctrl Pts',(12.0834247294191,23.76779590644,61.13994925363));
#153180=CARTESIAN_POINT('Ctrl Pts',(12.5949792953091,27.2217169096,61.57409469908));
#153181=CARTESIAN_POINT('Ctrl Pts',(13.2927090274791,20.66243511217,53.69009205466));
#153182=CARTESIAN_POINT('Ctrl Pts',(10.7176832624191,21.08595805766,56.49475584674));
#153183=CARTESIAN_POINT('Ctrl Pts',(9.21456506056909,23.95986757545,58.53385767307));
#153184=CARTESIAN_POINT('Ctrl Pts',(9.57610311105909,27.76867765135,58.7320035412201));
#153185=CARTESIAN_POINT('Origin',(22.932586701957,25.6803076522557,65.7954246532035));
#153186=CARTESIAN_POINT('Ctrl Pts',(20.8911511744791,19.9604224465,80.848282833327));
#153187=CARTESIAN_POINT('Ctrl Pts',(20.2241964889591,20.13080330299,80.513263521276));
#153188=CARTESIAN_POINT('Ctrl Pts',(18.9283646791091,20.71921193457,79.811448093371));
#153189=CARTESIAN_POINT('Ctrl Pts',(17.3696955150691,22.37067833873,78.780633438867));
#153190=CARTESIAN_POINT('Ctrl Pts',(16.4736258696191,24.54284688986,77.9461870487));
#153191=CARTESIAN_POINT('Ctrl Pts',(16.3978381440991,26.09054287903,77.605843233037));
#153192=CARTESIAN_POINT('Ctrl Pts',(16.4717809815391,26.84345587847,77.490338917542));
#153193=CARTESIAN_POINT('Ctrl Pts',(21.2489006219491,19.77806662564,79.674997080701));
#153194=CARTESIAN_POINT('Ctrl Pts',(20.5800208574191,19.9711851103,79.394482109607));
#153195=CARTESIAN_POINT('Ctrl Pts',(19.2882260173591,20.59194413007,78.806627701594));
#153196=CARTESIAN_POINT('Ctrl Pts',(17.7380604811591,22.23637549275,77.931740551844));
#153197=CARTESIAN_POINT('Ctrl Pts',(16.8323403731591,24.35865510143,77.199951533994));
#153198=CARTESIAN_POINT('Ctrl Pts',(16.7360936623891,25.86678725123,76.878121802014));
#153199=CARTESIAN_POINT('Ctrl Pts',(16.7988664925391,26.60318525589,76.760821350634));
#153200=CARTESIAN_POINT('Ctrl Pts',(21.7404719851691,19.4367501038,77.27768430253));
#153201=CARTESIAN_POINT('Ctrl Pts',(21.0781718769291,19.66719172332,77.10117478113));
#153202=CARTESIAN_POINT('Ctrl Pts',(19.8112633217491,20.33854901363,76.729024104145));
#153203=CARTESIAN_POINT('Ctrl Pts',(18.2922620430691,21.96660458151,76.155867660549));
#153204=CARTESIAN_POINT('Ctrl Pts',(17.3742768987591,24.00382143215,75.643605268245));
#153205=CARTESIAN_POINT('Ctrl Pts',(17.2366271868691,25.44474146273,75.386690727847));
#153206=CARTESIAN_POINT('Ctrl Pts',(17.2748132426991,26.1527308176,75.282273549274));
#153207=CARTESIAN_POINT('Ctrl Pts',(21.8755966897991,19.08135358495,73.526845056723));
#153208=CARTESIAN_POINT('Ctrl Pts',(21.2401175084091,19.34463071198,73.5057660894959));
#153209=CARTESIAN_POINT('Ctrl Pts',(20.0340922790191,20.05757741651,73.4492763332938));
#153210=CARTESIAN_POINT('Ctrl Pts',(18.5849356991691,21.66533371693,73.321641233911));
#153211=CARTESIAN_POINT('Ctrl Pts',(17.6776840505191,23.62313410685,73.1644554192328));
#153212=CARTESIAN_POINT('Ctrl Pts',(17.5011681902691,25.00156958332,73.0521458729575));
#153213=CARTESIAN_POINT('Ctrl Pts',(17.5121252768591,25.6826957763,72.9962696634154));
#153214=CARTESIAN_POINT('Ctrl Pts',(21.4080075944791,18.99041968019,69.698937793342));
#153215=CARTESIAN_POINT('Ctrl Pts',(20.7982638491291,19.26244640202,69.832985568099));
#153216=CARTESIAN_POINT('Ctrl Pts',(19.6465587797891,19.986295941,70.089606824027));
#153217=CARTESIAN_POINT('Ctrl Pts',(18.2728403102091,21.58882896434,70.408052707636));
#153218=CARTESIAN_POINT('Ctrl Pts',(17.4191062600591,23.52613108719,70.621969420302));
#153219=CARTESIAN_POINT('Ctrl Pts',(17.2580474576791,24.88819990756,70.679396362023));
#153220=CARTESIAN_POINT('Ctrl Pts',(17.2722927312391,25.56219068901,70.687933105918));
#153221=CARTESIAN_POINT('Ctrl Pts',(20.6971812658991,19.11140694679,67.205408224001));
#153222=CARTESIAN_POINT('Ctrl Pts',(20.1070383963591,19.37210896923,67.443938609233));
#153223=CARTESIAN_POINT('Ctrl Pts',(18.9924858732291,20.08180195792,67.912437713137));
#153224=CARTESIAN_POINT('Ctrl Pts',(17.6753991076991,21.69114765413,68.5308846882));
#153225=CARTESIAN_POINT('Ctrl Pts',(16.8811751422491,23.65527078503,68.988289141191));
#153226=CARTESIAN_POINT('Ctrl Pts',(16.7590148989391,25.03886729217,69.150951498051));
#153227=CARTESIAN_POINT('Ctrl Pts',(16.7913432132991,25.72230139667,69.197497579931));
#153228=CARTESIAN_POINT('Ctrl Pts',(20.2354688957591,19.21917800851,65.988118467194));
#153229=CARTESIAN_POINT('Ctrl Pts',(19.6554686558991,19.46975735037,66.279674422239));
#153230=CARTESIAN_POINT('Ctrl Pts',(18.5593496213791,20.16661372345,66.85686112244));
#153231=CARTESIAN_POINT('Ctrl Pts',(17.2722126901491,21.78232033032,67.628148426319));
#153232=CARTESIAN_POINT('Ctrl Pts',(16.5143337230091,23.77097449246,68.203940042059));
#153233=CARTESIAN_POINT('Ctrl Pts',(16.4190832870791,25.17355603177,68.411481313033));
#153234=CARTESIAN_POINT('Ctrl Pts',(16.4643772039691,25.86501026269,68.472097080547));
#153235=CARTESIAN_POINT('Ctrl Pts',(-2.42455476507091,16.92552468832,52.4988667111));
#153236=CARTESIAN_POINT('Ctrl Pts',(-2.42455476507091,16.92552468832,52.4988667111));
#153237=CARTESIAN_POINT('Ctrl Pts',(-2.42455476507091,16.92552468832,52.4988667111));
#153238=CARTESIAN_POINT('Ctrl Pts',(-2.42455476507091,16.92552468832,52.4988667111));
#153239=CARTESIAN_POINT('Ctrl Pts',(-1.37593350884091,19.75605503409,52.44644608116));
#153240=CARTESIAN_POINT('Ctrl Pts',(-0.884501579890127,19.39180151254,52.4218793741253));
#153241=CARTESIAN_POINT('Ctrl Pts',(-0.389267231970226,19.03168229686,52.3971225839732));
#153242=CARTESIAN_POINT('Ctrl Pts',(0.110004993249088,18.67552617523,52.37216394013));
#153243=CARTESIAN_POINT('Ctrl Pts',(-0.11447139326091,22.30361770189,52.58018366622));
#153244=CARTESIAN_POINT('Ctrl Pts',(0.887603277609087,21.4786617599,52.8198982923901));
#153245=CARTESIAN_POINT('Ctrl Pts',(1.81796826660909,20.56952055347,52.75185713948));
#153246=CARTESIAN_POINT('Ctrl Pts',(2.62639801664909,19.62528980623,52.37976571339));
#153247=CARTESIAN_POINT('Ctrl Pts',(1.24014776487909,24.40863425477,53.18278579188));
#153248=CARTESIAN_POINT('Ctrl Pts',(2.28602424783909,22.80161860487,53.71749108626));
#153249=CARTESIAN_POINT('Ctrl Pts',(3.58775731907909,21.31467159053,53.48378241936));
#153250=CARTESIAN_POINT('Ctrl Pts',(4.9251348840291,20.1992043079,52.52142955503));
#153251=CARTESIAN_POINT('Origin',(-10.9843331791359,92.,80.581991049076));
#153252=CARTESIAN_POINT('',(1.02913961852909,92.5,53.63896836527));
#153253=CARTESIAN_POINT('Origin',(1.02913961852909,92.,53.63896836527));
#153254=CARTESIAN_POINT('Origin',(-10.9843331791359,92.5,80.581991049076));
#153255=CARTESIAN_POINT('Origin',(-10.9843331791359,92.,65.395787724084));
#153256=CARTESIAN_POINT('',(1.02913961852909,92.5,92.33881040789));
#153257=CARTESIAN_POINT('Origin',(-10.9843331791359,92.5,65.395787724084));
#153258=CARTESIAN_POINT('Origin',(1.02913961852909,92.,92.33881040789));
#153259=CARTESIAN_POINT('Origin',(-2.02513312664091,92.,85.48888938658));
#153260=CARTESIAN_POINT('Origin',(-2.02513312664091,92.5,85.48888938658));
#153261=CARTESIAN_POINT('Origin',(-2.27593483123091,92.5,69.192338555332));
#153262=CARTESIAN_POINT('Origin',(-2.02513312664091,92.5,60.48888938658));
#153263=CARTESIAN_POINT('Origin',(-2.02513312664091,92.,60.48888938658));
#153264=CARTESIAN_POINT('Origin',(20.5162416486691,1.4210854715202E-14,
116.353388269));
#153265=CARTESIAN_POINT('Ctrl Pts',(37.1148577576791,-11.38315600667,64.424614458756));
#153266=CARTESIAN_POINT('Ctrl Pts',(33.3746924839791,-9.55480085092099,
64.424638317428));
#153267=CARTESIAN_POINT('Ctrl Pts',(30.0554397785991,-9.17281283206899,
61.94094919385));
#153268=CARTESIAN_POINT('Ctrl Pts',(28.7731848187491,-10.42324480072,58.18267172033));
#153269=CARTESIAN_POINT('Ctrl Pts',(36.7247317035591,-11.99143530332,64.746736687142));
#153270=CARTESIAN_POINT('Ctrl Pts',(33.0869920335091,-10.11930380944,64.661644695515));
#153271=CARTESIAN_POINT('Ctrl Pts',(29.8376575084291,-9.718933522376,62.2086132886801));
#153272=CARTESIAN_POINT('Ctrl Pts',(28.5145010531591,-10.97987178426,58.54842980974));
#153273=CARTESIAN_POINT('Ctrl Pts',(36.3045657794791,-12.5809663284,65.090039586453));
#153274=CARTESIAN_POINT('Ctrl Pts',(32.7708362104291,-10.68071449823,64.92189605369));
#153275=CARTESIAN_POINT('Ctrl Pts',(29.5952467863491,-10.26284018231,62.50069738269));
#153276=CARTESIAN_POINT('Ctrl Pts',(28.2357619232591,-11.51926368214,58.9379362879));
#153277=CARTESIAN_POINT('Ctrl Pts',(35.8540738479291,-13.15242231248,65.452547555325));
#153278=CARTESIAN_POINT('Ctrl Pts',(32.4235807876891,-11.23800283895,65.206103155874));
#153279=CARTESIAN_POINT('Ctrl Pts',(29.3251926934191,-10.80344668515,62.81749475457));
#153280=CARTESIAN_POINT('Ctrl Pts',(27.9366338055491,-12.04204812536,59.3487279449101));
#153281=CARTESIAN_POINT('',(36.8798279596591,-11.43907953387,64.491475339616));
#153282=CARTESIAN_POINT('Ctrl Pts',(35.8057502945591,-12.95453430026,65.365954576197));
#153283=CARTESIAN_POINT('Ctrl Pts',(36.1860516598291,-12.46249651106,65.059698667609));
#153284=CARTESIAN_POINT('Ctrl Pts',(36.5439947228891,-11.95743270971,64.76779286742));
#153285=CARTESIAN_POINT('Ctrl Pts',(36.8798279596591,-11.43907953387,64.491475339616));
#153286=CARTESIAN_POINT('Ctrl Pts',(36.8798279596681,-11.4390795338486,
64.4914753396672));
#153287=CARTESIAN_POINT('Ctrl Pts',(36.7441750018997,-11.3735279686372,
64.4879383408179));
#153288=CARTESIAN_POINT('Ctrl Pts',(36.6064460983526,-11.3089290560052,
64.4804862516236));
#153289=CARTESIAN_POINT('Ctrl Pts',(36.4669094342276,-11.2455257133135,
64.4689019673217));
#153290=CARTESIAN_POINT('Ctrl Pts',(36.3287823623725,-11.1827628679584,
64.4574347068695));
#153291=CARTESIAN_POINT('Ctrl Pts',(36.1888840383274,-11.1211718375744,
64.4419179324151));
#153292=CARTESIAN_POINT('Ctrl Pts',(36.047515073403,-11.0609928153098,64.4221717313969));
#153293=CARTESIAN_POINT('Ctrl Pts',(35.9080299464162,-11.0016157195872,
64.4026886619836));
#153294=CARTESIAN_POINT('Ctrl Pts',(35.7671133724119,-10.94361353859,64.3790878219158));
#153295=CARTESIAN_POINT('Ctrl Pts',(35.6250904880056,-10.8872172610078,
64.3512315440085));
#153296=CARTESIAN_POINT('Ctrl Pts',(35.4840672423464,-10.8312179328644,
64.3235713346072));
#153297=CARTESIAN_POINT('Ctrl Pts',(35.3419534965111,-10.7768022748865,
64.2917150865606));
#153298=CARTESIAN_POINT('Ctrl Pts',(35.1990996420043,-10.7241923799527,
64.2555674775194));
#153299=CARTESIAN_POINT('Ctrl Pts',(35.0575694076834,-10.6720699448718,
64.2197547961228));
#153300=CARTESIAN_POINT('Ctrl Pts',(34.9153130778802,-10.6217202516276,
64.1797296977471));
#153301=CARTESIAN_POINT('Ctrl Pts',(34.7726981088167,-10.5733509706476,
64.1354420899077));
#153302=CARTESIAN_POINT('Ctrl Pts',(34.6643414532593,-10.5366007364112,
64.101793048018));
#153303=CARTESIAN_POINT('Ctrl Pts',(34.5557783568399,-10.5009936047222,
64.0656842235702));
#153304=CARTESIAN_POINT('Ctrl Pts',(34.4471783750911,-10.4666158673459,
64.0271113390586));
#153305=CARTESIAN_POINT('Ctrl Pts',(34.3077698634826,-10.4224855726357,
63.9775957836081));
#153306=CARTESIAN_POINT('Ctrl Pts',(34.1682336268683,-10.3803607477818,
63.9239944308088));
#153307=CARTESIAN_POINT('Ctrl Pts',(34.0289521150137,-10.3404196067234,
63.8663302586336));
#153308=CARTESIAN_POINT('Ctrl Pts',(33.8903294409197,-10.3006673976459,
63.808938852984));
#153309=CARTESIAN_POINT('Ctrl Pts',(33.7519595460037,-10.2630785115483,
63.7475229310178));
#153310=CARTESIAN_POINT('Ctrl Pts',(33.6142299740126,-10.2278100923352,
63.6821520759947));
#153311=CARTESIAN_POINT('Ctrl Pts',(33.4754483971942,-10.1922722861872,
63.6162819058713));
#153312=CARTESIAN_POINT('Ctrl Pts',(33.3373174532717,-10.1590908011647,
63.5463961017914));
#153313=CARTESIAN_POINT('Ctrl Pts',(33.2002371867619,-10.128403545685,63.4726144903044));
#153314=CARTESIAN_POINT('Ctrl Pts',(33.0652012554393,-10.0981739420452,
63.3999332147619));
#153315=CARTESIAN_POINT('Ctrl Pts',(32.9311853795762,-10.0703648598007,
63.3234716773683));
#153316=CARTESIAN_POINT('Ctrl Pts',(32.7985681278943,-10.0450831627581,
63.2433899608591));
#153317=CARTESIAN_POINT('Ctrl Pts',(32.6629392987228,-10.0192273489339,
63.1614896853637));
#153318=CARTESIAN_POINT('Ctrl Pts',(32.5287739002282,-9.99601527822984,
63.0758029691421));
#153319=CARTESIAN_POINT('Ctrl Pts',(32.3964648510167,-9.97553168804268,
62.9865476599149));
#153320=CARTESIAN_POINT('Ctrl Pts',(32.2641558018052,-9.95504809785552,
62.8972923506877));
#153321=CARTESIAN_POINT('Ctrl Pts',(32.1337036138356,-9.93729309243784,
62.8044687444746));
#153322=CARTESIAN_POINT('Ctrl Pts',(32.0054812102974,-9.92231950953623,
62.7083380847189));
#153323=CARTESIAN_POINT('Ctrl Pts',(31.8803697597832,-9.90770921816341,
62.6145397628262));
#153324=CARTESIAN_POINT('Ctrl Pts',(31.7572899979802,-9.89573625457834,
62.5175247549684));
#153325=CARTESIAN_POINT('Ctrl Pts',(31.6365737639664,-9.88643109912129,
62.4175581834101));
#153326=CARTESIAN_POINT('Ctrl Pts',(31.5157672166093,-9.87711898205128,
62.3175168222813));
#153327=CARTESIAN_POINT('Ctrl Pts',(31.3973281256053,-9.87047867724871,
62.2145198410588));
#153328=CARTESIAN_POINT('Ctrl Pts',(31.2815608813011,-9.86651055480352,
62.1088649167814));
#153329=CARTESIAN_POINT('Ctrl Pts',(31.163210651863,-9.86245389607721,62.0008526322647));
#153330=CARTESIAN_POINT('Ctrl Pts',(31.0476533098122,-9.86119005685629,
61.8900628208581));
#153331=CARTESIAN_POINT('Ctrl Pts',(30.935177785853,-9.8626871641774,61.7768416797537));
#153332=CARTESIAN_POINT('Ctrl Pts',(30.824489314776,-9.86416048490157,61.6654194381735));
#153333=CARTESIAN_POINT('Ctrl Pts',(30.7167856681417,-9.86830752697171,
61.5516430401091));
#153334=CARTESIAN_POINT('Ctrl Pts',(30.6123030211769,-9.87506826147692,
61.4358625684621));
#153335=CARTESIAN_POINT('Ctrl Pts',(30.5052900833844,-9.8819927229263,61.3172782028294));
#153336=CARTESIAN_POINT('Ctrl Pts',(30.4016564107195,-9.89165895151477,
61.1965919844559));
#153337=CARTESIAN_POINT('Ctrl Pts',(30.3016099115775,-9.90397263019706,
61.0741939994848));
#153338=CARTESIAN_POINT('Ctrl Pts',(30.2015634124355,-9.91628630887936,
60.9517960145137));
#153339=CARTESIAN_POINT('Ctrl Pts',(30.1051041820874,-9.93124721616769,
60.8276867937595));
#153340=CARTESIAN_POINT('Ctrl Pts',(30.0123915794226,-9.94873382237174,
60.702262569282));
#153341=CARTESIAN_POINT('Ctrl Pts',(29.9190203204585,-9.96634465832449,
60.5759472959808));
#153342=CARTESIAN_POINT('Ctrl Pts',(29.8294030814699,-9.98652556792445,
60.4482366205373));
#153343=CARTESIAN_POINT('Ctrl Pts',(29.7436578355946,-10.0091373557639,
60.3195209980263));
#153344=CARTESIAN_POINT('Ctrl Pts',(29.6573497459522,-10.0318975705363,
60.1899604681958));
#153345=CARTESIAN_POINT('Ctrl Pts',(29.5749646284969,-10.0571204355003,
60.0593822207725));
#153346=CARTESIAN_POINT('Ctrl Pts',(29.4965744788422,-10.0846437655168,
59.9281770342848));
#153347=CARTESIAN_POINT('Ctrl Pts',(29.4172168052186,-10.1125067999684,
59.7953524585837));
#153348=CARTESIAN_POINT('Ctrl Pts',(29.3419532620603,-10.1427271751237,
59.6618858288828));
#153349=CARTESIAN_POINT('Ctrl Pts',(29.270809736117,-10.1751197943674,59.5281679608396));
#153350=CARTESIAN_POINT('Ctrl Pts',(29.1991491694168,-10.2077478293309,
59.3934782884501));
#153351=CARTESIAN_POINT('Ctrl Pts',(29.1316685385326,-10.2425795025469,
59.2585341137898));
#153352=CARTESIAN_POINT('Ctrl Pts',(29.0683470046054,-10.2794129266527,
59.1237135976406));
#153353=CARTESIAN_POINT('Ctrl Pts',(29.0041776407885,-10.3167395238698,
58.9870879315487));
#153354=CARTESIAN_POINT('Ctrl Pts',(28.9442792778791,-10.3561215368744,
58.8505896339998));
#153355=CARTESIAN_POINT('Ctrl Pts',(28.8885848131186,-10.3973403349861,
58.7145845665897));
#153356=CARTESIAN_POINT('Ctrl Pts',(28.8470986002056,-10.4280437781709,
58.6132758421396));
#153357=CARTESIAN_POINT('Ctrl Pts',(28.8079439853351,-10.4597661809439,
58.5122402265492));
#153358=CARTESIAN_POINT('Ctrl Pts',(28.7710784579419,-10.4924156480374,
58.4116174733487));
#153359=CARTESIAN_POINT('Ctrl Pts',(28.6318099234291,-10.68337721174,58.2360960239));
#153360=CARTESIAN_POINT('Ctrl Pts',(28.9036687620591,-10.40410957799,59.04777775718));
#153361=CARTESIAN_POINT('Ctrl Pts',(29.7282443214291,-9.97887814526099,
60.69655454236));
#153362=CARTESIAN_POINT('Ctrl Pts',(31.8102465520291,-9.94192586985999,
62.86109705332));
#153363=CARTESIAN_POINT('Ctrl Pts',(34.3891486420691,-10.55131574029,64.279269257528));
#153364=CARTESIAN_POINT('Ctrl Pts',(36.1064545847691,-11.2894506228,64.582977897741));
#153365=CARTESIAN_POINT('Ctrl Pts',(36.9086854560691,-11.70132943018,64.595573649679));
#153366=CARTESIAN_POINT('Ctrl Pts',(29.0456292725091,-10.01132377404,58.37055718011));
#153367=CARTESIAN_POINT('Ctrl Pts',(29.3498254657591,-9.77458649748099,
59.16172491632));
#153368=CARTESIAN_POINT('Ctrl Pts',(30.2325487222691,-9.41554285765999,
60.73612952655));
#153369=CARTESIAN_POINT('Ctrl Pts',(32.3627339107191,-9.37345866626899,
62.71704601845));
#153370=CARTESIAN_POINT('Ctrl Pts',(34.9609073760491,-9.86290539232099,
63.941641260975));
#153371=CARTESIAN_POINT('Ctrl Pts',(36.6922503471391,-10.4709131891,64.141295131879));
#153372=CARTESIAN_POINT('Ctrl Pts',(37.5052929747491,-10.81476301663,64.108748322606));
#153373=CARTESIAN_POINT('Ctrl Pts',(29.8074106496591,-8.60875283793899,
58.64000348532));
#153374=CARTESIAN_POINT('Ctrl Pts',(30.1723381639891,-8.44024965538699,
59.37231809656));
#153375=CARTESIAN_POINT('Ctrl Pts',(31.1487519819791,-8.18096902990299,
60.77590041796));
#153376=CARTESIAN_POINT('Ctrl Pts',(33.3031956985291,-8.10811512607799,
62.41397188693));
#153377=CARTESIAN_POINT('Ctrl Pts',(35.8461147163691,-8.37510901302899,
63.319546372377));
#153378=CARTESIAN_POINT('Ctrl Pts',(37.5408772930491,-8.74778122122199,
63.36692565601));
#153379=CARTESIAN_POINT('Ctrl Pts',(38.3453292531191,-8.96717590778899,
63.271322697011));
#153380=CARTESIAN_POINT('Ctrl Pts',(30.7659404102391,-6.12843955931699,
59.02640618789));
#153381=CARTESIAN_POINT('Ctrl Pts',(31.1943400875191,-6.03067355048699,
59.64444010852));
#153382=CARTESIAN_POINT('Ctrl Pts',(32.2374024575391,-5.86859656993499,
60.77872899668));
#153383=CARTESIAN_POINT('Ctrl Pts',(34.2962640644291,-5.75551569888499,
61.99917441976));
#153384=CARTESIAN_POINT('Ctrl Pts',(36.6198739262991,-5.78832739818299,
62.58745827192));
#153385=CARTESIAN_POINT('Ctrl Pts',(38.1639558208391,-5.90433866667599,
62.52263971893));
#153386=CARTESIAN_POINT('Ctrl Pts',(38.9069661676791,-5.98184811597299,
62.3893519671));
#153387=CARTESIAN_POINT('Ctrl Pts',(31.4628040362191,-3.27451591220699,
59.34145203332));
#153388=CARTESIAN_POINT('Ctrl Pts',(31.9148547160891,-3.22399603912999,
59.85552151593));
#153389=CARTESIAN_POINT('Ctrl Pts',(32.9537808151091,-3.13354949579399,
60.77329930901));
#153390=CARTESIAN_POINT('Ctrl Pts',(34.8624033916191,-3.03865186609699,
61.7164874873));
#153391=CARTESIAN_POINT('Ctrl Pts',(36.9515785646591,-2.99298517160899,
62.13709043757));
#153392=CARTESIAN_POINT('Ctrl Pts',(38.3374590596191,-2.99798405108899,
62.04637567703));
#153393=CARTESIAN_POINT('Ctrl Pts',(39.0114873686691,-3.00876121641099,
61.9161681279));
#153394=CARTESIAN_POINT('Ctrl Pts',(31.6941891349691,-0.559164177511486,
59.45203956376));
#153395=CARTESIAN_POINT('Ctrl Pts',(32.1483274996991,-0.550463064146686,
59.929061278));
#153396=CARTESIAN_POINT('Ctrl Pts',(33.1744137845191,-0.534881944430286,
60.77391018355));
#153397=CARTESIAN_POINT('Ctrl Pts',(35.0195538481991,-0.518480218034586,
61.63166634532));
#153398=CARTESIAN_POINT('Ctrl Pts',(37.0205148723291,-0.510451987175386,
62.00677298972));
#153399=CARTESIAN_POINT('Ctrl Pts',(38.3472726057891,-0.511094758103086,
61.91535197825));
#153400=CARTESIAN_POINT('Ctrl Pts',(38.9948370647791,-0.512805555018386,
61.79060918495));
#153401=CARTESIAN_POINT('Ctrl Pts',(31.6030449881391,1.63342335677401,59.40849392115));
#153402=CARTESIAN_POINT('Ctrl Pts',(32.0562402583091,1.60809110369101,59.90010929421));
#153403=CARTESIAN_POINT('Ctrl Pts',(33.0871862210291,1.56273341258401,60.77377016236));
#153404=CARTESIAN_POINT('Ctrl Pts',(34.9572779373091,1.51505187528801,61.66534608043));
#153405=CARTESIAN_POINT('Ctrl Pts',(36.9930942606091,1.49187208211601,62.05839402226));
#153406=CARTESIAN_POINT('Ctrl Pts',(38.3431995755691,1.49399892537301,61.96714783356));
#153407=CARTESIAN_POINT('Ctrl Pts',(39.0011940413591,1.49914916427001,61.84019219338));
#153408=CARTESIAN_POINT('Ctrl Pts',(31.3474186477091,3.74625791698601,59.28928090803));
#153409=CARTESIAN_POINT('Ctrl Pts',(31.7956253642391,3.68797075177601,59.82056228684));
#153410=CARTESIAN_POINT('Ctrl Pts',(32.8353535505091,3.58576207768401,60.77413589135));
#153411=CARTESIAN_POINT('Ctrl Pts',(34.7688811807491,3.48797809126401,61.76313013829));
#153412=CARTESIAN_POINT('Ctrl Pts',(36.8968037579091,3.45543334845601,62.21148594642));
#153413=CARTESIAN_POINT('Ctrl Pts',(38.3088386424591,3.47892537809701,62.12512240935));
#153414=CARTESIAN_POINT('Ctrl Pts',(38.9942825908291,3.50082164918001,61.99444197964));
#153415=CARTESIAN_POINT('Ctrl Pts',(30.7683829701991,6.12095524445701,59.02743346636));
#153416=CARTESIAN_POINT('Ctrl Pts',(31.1968671386991,6.02337634604401,59.64515039934));
#153417=CARTESIAN_POINT('Ctrl Pts',(32.2399479399591,5.86157111726001,60.77875998162));
#153418=CARTESIAN_POINT('Ctrl Pts',(34.2984250721691,5.74848170063101,61.99825790957));
#153419=CARTESIAN_POINT('Ctrl Pts',(36.6214127992191,5.78083057602201,62.58585616545));
#153420=CARTESIAN_POINT('Ctrl Pts',(38.1650763376391,5.89625980071201,62.52080797117));
#153421=CARTESIAN_POINT('Ctrl Pts',(38.9079073284191,5.97342694265101,62.3874504358));
#153422=CARTESIAN_POINT('Ctrl Pts',(29.8089157326691,8.60405889048601,58.64067146398));
#153423=CARTESIAN_POINT('Ctrl Pts',(30.1740149579691,8.43552829169101,59.37277486795));
#153424=CARTESIAN_POINT('Ctrl Pts',(31.1506497978491,8.17616183997101,60.77583536541));
#153425=CARTESIAN_POINT('Ctrl Pts',(33.3049462375891,8.10299652459701,62.41308396893));
#153426=CARTESIAN_POINT('Ctrl Pts',(35.8473775190891,8.36951394256301,63.318103430771));
#153427=CARTESIAN_POINT('Ctrl Pts',(37.5417814200891,8.74184941723802,63.365377186793));
#153428=CARTESIAN_POINT('Ctrl Pts',(38.3460819705591,8.96109715611501,63.269768790418));
#153429=CARTESIAN_POINT('Ctrl Pts',(29.0444408655791,10.01352551446,58.37014632461));
#153430=CARTESIAN_POINT('Ctrl Pts',(29.3485833929991,9.77666292162801,59.16139737026));
#153431=CARTESIAN_POINT('Ctrl Pts',(30.2312412513191,9.41739555567501,60.73602919927));
#153432=CARTESIAN_POINT('Ctrl Pts',(32.3614928437391,9.37516348482501,62.71737336154));
#153433=CARTESIAN_POINT('Ctrl Pts',(34.9598381149091,9.86469977852602,63.942339691534));
#153434=CARTESIAN_POINT('Ctrl Pts',(36.6912888370791,10.47289336349,64.142147541472));
#153435=CARTESIAN_POINT('Ctrl Pts',(37.5043705412191,10.81685010051,64.10965815328));
#153436=CARTESIAN_POINT('Ctrl Pts',(28.6314686688091,10.68390667014,58.23598693286));
#153437=CARTESIAN_POINT('Ctrl Pts',(28.9032909729591,10.40460748413,59.04768337326));
#153438=CARTESIAN_POINT('Ctrl Pts',(29.7277959815891,9.97933481861901,60.69652425927));
#153439=CARTESIAN_POINT('Ctrl Pts',(31.8097200738291,9.94243017287101,62.86124366858));
#153440=CARTESIAN_POINT('Ctrl Pts',(34.3885675638091,10.55197967391,64.279613731913));
#153441=CARTESIAN_POINT('Ctrl Pts',(36.1058374833391,11.29026451401,64.583435617639));
#153442=CARTESIAN_POINT('Ctrl Pts',(36.9080477180991,11.70221929791,64.596082014895));
#153443=CARTESIAN_POINT('',(36.8798265045291,11.43907883074,64.491475301679));
#153444=CARTESIAN_POINT('Ctrl Pts',(36.8798279595137,-11.4390795342153,
64.4914753387916));
#153445=CARTESIAN_POINT('Ctrl Pts',(37.0098305129696,-11.2382074865074,
64.3844217348773));
#153446=CARTESIAN_POINT('Ctrl Pts',(37.1330559421466,-11.032180459589,64.2791469343491));
#153447=CARTESIAN_POINT('Ctrl Pts',(37.2495510317378,-10.8209394872084,
64.1758610837496));
#153448=CARTESIAN_POINT('Ctrl Pts',(37.3649491417382,-10.6116876719354,
64.0735478275362));
#153449=CARTESIAN_POINT('Ctrl Pts',(37.4737424415873,-10.3973193963561,
63.9731862588846));
#153450=CARTESIAN_POINT('Ctrl Pts',(37.5759730006416,-10.1778039241941,
63.8750238873));
#153451=CARTESIAN_POINT('Ctrl Pts',(37.6761385330716,-9.96272259871627,
63.7788443661731));
#153452=CARTESIAN_POINT('Ctrl Pts',(37.7700032180155,-9.74269975563697,
63.684776174574));
#153453=CARTESIAN_POINT('Ctrl Pts',(37.857612056372,-9.51773506712692,63.5930929761144));
#153454=CARTESIAN_POINT('Ctrl Pts',(37.8719863351407,-9.4808243489116,63.5780502032871));
#153455=CARTESIAN_POINT('Ctrl Pts',(37.8861922287029,-9.44378066252948,
63.5630717240933));
#153456=CARTESIAN_POINT('Ctrl Pts',(37.9002299660476,-9.40660408663557,
63.5481588530175));
#153457=CARTESIAN_POINT('Ctrl Pts',(37.9733622814116,-9.21292550399318,
63.4704673587465));
#153458=CARTESIAN_POINT('Ctrl Pts',(38.041938023627,-9.01564124523459,63.3945535346591));
#153459=CARTESIAN_POINT('Ctrl Pts',(38.1059762093653,-8.81469346733212,
63.3205966744608));
#153460=CARTESIAN_POINT('Ctrl Pts',(38.1623696876838,-8.63773429796041,
63.2554685865234));
#153461=CARTESIAN_POINT('Ctrl Pts',(38.2152438827478,-8.45793386216728,
63.1918586472492));
#153462=CARTESIAN_POINT('Ctrl Pts',(38.264633349399,-8.27532061150791,63.1298994651875));
#153463=CARTESIAN_POINT('Ctrl Pts',(38.3173704373835,-8.08032982257757,
63.0637406856462));
#153464=CARTESIAN_POINT('Ctrl Pts',(38.3661269542761,-7.88211198822048,
62.9994587855359));
#153465=CARTESIAN_POINT('Ctrl Pts',(38.4109334817639,-7.68066015104794,
62.9372275318957));
#153466=CARTESIAN_POINT('Ctrl Pts',(38.4333367455077,-7.57993423246166,
62.9061119050756));
#153467=CARTESIAN_POINT('Ctrl Pts',(38.45475257401,-7.47839970899487,62.875509289796));
#153468=CARTESIAN_POINT('Ctrl Pts',(38.475185232764,-7.37605590671984,62.8454438875471));
#153469=CARTESIAN_POINT('Ctrl Pts',(38.485401562141,-7.32488400558233,62.8304111864227));
#153470=CARTESIAN_POINT('Ctrl Pts',(38.495372103593,-7.273509779017,62.8155128136895));
#153471=CARTESIAN_POINT('Ctrl Pts',(38.5050974197184,-7.22193313447018,
62.8007519582672));
#153472=CARTESIAN_POINT('Ctrl Pts',(38.5099600777811,-7.19614481219677,
62.7933715305561));
#153473=CARTESIAN_POINT('Ctrl Pts',(38.5147614298181,-7.17030588510649,
62.7860254838728));
#153474=CARTESIAN_POINT('Ctrl Pts',(38.5195015481513,-7.14441634262704,
62.7787142279474));
#153475=CARTESIAN_POINT('Ctrl Pts',(38.5232683013994,-7.12384311821073,
62.7729043103315));
#153476=CARTESIAN_POINT('Ctrl Pts',(38.5267948165354,-7.10436051932523,
62.7674306943907));
#153477=CARTESIAN_POINT('Ctrl Pts',(38.5305622170623,-7.08329247922146,
62.7615438485301));
#153478=CARTESIAN_POINT('Ctrl Pts',(38.5315357494103,-7.07784829604959,
62.760022631226));
#153479=CARTESIAN_POINT('Ctrl Pts',(38.5325251554163,-7.07229818822057,
62.758473968008));
#153480=CARTESIAN_POINT('Ctrl Pts',(38.5335382756798,-7.06659585814249,
62.7568852495087));
#153481=CARTESIAN_POINT('Ctrl Pts',(38.5648627577464,-6.89028654648589,
62.707763949759));
#153482=CARTESIAN_POINT('Ctrl Pts',(38.5938540547229,-6.70862617273319,
62.6594277140837));
#153483=CARTESIAN_POINT('Ctrl Pts',(38.6205403121146,-6.52158307912809,
62.6121931288261));
#153484=CARTESIAN_POINT('Ctrl Pts',(38.6467448942024,-6.33791603176428,
62.5658111072261));
#153485=CARTESIAN_POINT('Ctrl Pts',(38.6707265414135,-6.14905802435774,
62.5204908743574));
#153486=CARTESIAN_POINT('Ctrl Pts',(38.6925239461544,-5.95500045380756,
62.476574435171));
#153487=CARTESIAN_POINT('Ctrl Pts',(38.7044688916416,-5.84865719280242,
62.4525082915954));
#153488=CARTESIAN_POINT('Ctrl Pts',(38.7157577867499,-5.74075329648307,
62.4288648219717));
#153489=CARTESIAN_POINT('Ctrl Pts',(38.726426943577,-5.63126269288935,62.4056808771417));
#153490=CARTESIAN_POINT('Ctrl Pts',(38.742129208159,-5.47012058440449,62.371560051881));
#153491=CARTESIAN_POINT('Ctrl Pts',(38.7564526971244,-5.30557682948906,
62.3384478461317));
#153492=CARTESIAN_POINT('Ctrl Pts',(38.7694094634675,-5.13762681718977,
62.306498937974));
#153493=CARTESIAN_POINT('Ctrl Pts',(38.7770673484422,-5.03836270748577,
62.2876160579976));
#153494=CARTESIAN_POINT('Ctrl Pts',(38.7842487191847,-4.93790890283837,
62.2691395020168));
#153495=CARTESIAN_POINT('Ctrl Pts',(38.7909645338487,-4.83626607811927,
62.2511007189063));
#153496=CARTESIAN_POINT('Ctrl Pts',(38.8000038559376,-4.69945732495441,
62.2268209585515));
#153497=CARTESIAN_POINT('Ctrl Pts',(38.8081938994977,-4.56049375710199,
62.2033351283924));
#153498=CARTESIAN_POINT('Ctrl Pts',(38.8155488598102,-4.41937717082027,
62.1807237168028));
#153499=CARTESIAN_POINT('Ctrl Pts',(38.8192263399665,-4.3488188776794,62.1694180110079));
#153500=CARTESIAN_POINT('Ctrl Pts',(38.8226950540342,-4.27772232198402,
62.1583309366808));
#153501=CARTESIAN_POINT('Ctrl Pts',(38.8259568116944,-4.20608794889965,
62.1474727558722));
#153502=CARTESIAN_POINT('Ctrl Pts',(38.8275876905245,-4.17027076235747,
62.1420436654678));
#153503=CARTESIAN_POINT('Ctrl Pts',(38.829166830545,-4.13431912091543,62.1366718001178));
#153504=CARTESIAN_POINT('Ctrl Pts',(38.8306944599535,-4.09823308540843,
62.1313584539612));
#153505=CARTESIAN_POINT('Ctrl Pts',(38.8314582746578,-4.08019006765494,
62.1287017808829));
#153506=CARTESIAN_POINT('Ctrl Pts',(38.8322092117279,-4.0621134513515,62.1260597377108));
#153507=CARTESIAN_POINT('Ctrl Pts',(38.8329472998241,-4.04400324484754,
62.1234324869897));
#153508=CARTESIAN_POINT('Ctrl Pts',(38.8333163438723,-4.03494814159556,
62.1221188616292));
#153509=CARTESIAN_POINT('Ctrl Pts',(38.8336821756781,-4.02588464079131,
62.1208089343882));
#153510=CARTESIAN_POINT('Ctrl Pts',(38.8340447988329,-4.01681274352909,
62.1195027256339));
#153511=CARTESIAN_POINT('Ctrl Pts',(38.8344074219876,-4.00774084626686,
62.1181965168797));
#153512=CARTESIAN_POINT('Ctrl Pts',(38.8348372704066,-3.99686343020025,
62.1166372222354));
#153513=CARTESIAN_POINT('Ctrl Pts',(38.83512304594,-3.9895718634735,62.1155952752285));
#153514=CARTESIAN_POINT('Ctrl Pts',(38.83987727857,-3.86826755149894,62.0982611864758));
#153515=CARTESIAN_POINT('Ctrl Pts',(38.8441419459198,-3.74026219392216,
62.0808688446545));
#153516=CARTESIAN_POINT('Ctrl Pts',(38.8479129797729,-3.60554370191226,
62.0636772334747));
#153517=CARTESIAN_POINT('Ctrl Pts',(38.8514022624339,-3.48089064479584,
62.0477700862202));
#153518=CARTESIAN_POINT('Ctrl Pts',(38.854468577654,-3.3504900244013,62.0320351127797));
#153519=CARTESIAN_POINT('Ctrl Pts',(38.8571515577449,-3.21433521685374,
62.0166888938196));
#153520=CARTESIAN_POINT('Ctrl Pts',(38.8585208767362,-3.14484556079837,
62.0088566072004));
#153521=CARTESIAN_POINT('Ctrl Pts',(38.8597910854502,-3.07385711093731,
62.0011257453176));
#153522=CARTESIAN_POINT('Ctrl Pts',(38.8609727143632,-3.00136944360957,
61.993526002045));
#153523=CARTESIAN_POINT('Ctrl Pts',(38.8635089936615,-2.84578001278042,
61.9772137137095));
#153524=CARTESIAN_POINT('Ctrl Pts',(38.8656351315966,-2.68328395752332,
61.9615038043529));
#153525=CARTESIAN_POINT('Ctrl Pts',(38.8673988961025,-2.51385124300707,
61.9467287260682));
#153526=CARTESIAN_POINT('Ctrl Pts',(38.8681573266244,-2.44099404371637,
61.9403753436875));
#153527=CARTESIAN_POINT('Ctrl Pts',(38.8688493000898,-2.3668541654991,61.9341951035091));
#153528=CARTESIAN_POINT('Ctrl Pts',(38.8694813648467,-2.29142901485335,
61.9282157050522));
#153529=CARTESIAN_POINT('Ctrl Pts',(38.8708760369027,-2.125000893707,61.9150219620867));
#153530=CARTESIAN_POINT('Ctrl Pts',(38.8719833550435,-1.95232991211532,
61.9028050003795));
#153531=CARTESIAN_POINT('Ctrl Pts',(38.8728321120811,-1.77342523308076,
61.8918890344145));
#153532=CARTESIAN_POINT('Ctrl Pts',(38.8736321201952,-1.60479606296729,
61.881600034196));
#153533=CARTESIAN_POINT('Ctrl Pts',(38.87420235681,-1.43062871772306,61.8724670776073));
#153534=CARTESIAN_POINT('Ctrl Pts',(38.8746155555018,-1.2509307177607,61.8647716416033));
#153535=CARTESIAN_POINT('Ctrl Pts',(38.8746407339857,-1.23998072375628,
61.8643027160831));
#153536=CARTESIAN_POINT('Ctrl Pts',(38.8746653453594,-1.22901019357011,
61.863839130996));
#153537=CARTESIAN_POINT('Ctrl Pts',(38.8746894124171,-1.21801912886532,
61.8633809510676));
#153538=CARTESIAN_POINT('Ctrl Pts',(38.8750698351621,-1.04428576062759,
61.8561386006349));
#153539=CARTESIAN_POINT('Ctrl Pts',(38.8752990052889,-0.865423956850033,
61.8502483396648));
#153540=CARTESIAN_POINT('Ctrl Pts',(38.8754222231277,-0.681454298511442,
61.8459818319775));
#153541=CARTESIAN_POINT('Ctrl Pts',(38.8754347267326,-0.662785865894718,
61.8455488855232));
#153542=CARTESIAN_POINT('Ctrl Pts',(38.8754461835269,-0.644064836495899,
61.8451326637247));
#153543=CARTESIAN_POINT('Ctrl Pts',(38.8754566711061,-0.625291232005114,
61.8447334533453));
#153544=CARTESIAN_POINT('Ctrl Pts',(38.875524466503,-0.503932056618734,
61.8421528171939));
#153545=CARTESIAN_POINT('Ctrl Pts',(38.8755516014932,-0.380917881018939,
61.8402903434325));
#153546=CARTESIAN_POINT('Ctrl Pts',(38.8755477611405,-0.255289580951591,
61.8392102481073));
#153547=CARTESIAN_POINT('Ctrl Pts',(38.8755452828126,-0.174216784067554,
61.8385132208542));
#153548=CARTESIAN_POINT('Ctrl Pts',(38.8755300542589,-0.0920552103720104,
61.8381429881062));
#153549=CARTESIAN_POINT('Ctrl Pts',(38.8755077513205,-0.00854601869039584,
61.8381279487094));
#153550=CARTESIAN_POINT('Ctrl Pts',(38.875506582961,-0.00417131427553062,
61.838127160857));
#153551=CARTESIAN_POINT('Ctrl Pts',(38.8755053959128,0.000207088582348095,
61.8381273498256));
#153552=CARTESIAN_POINT('Ctrl Pts',(38.8755041868924,0.00458922532672068,
61.8381285210023));
#153553=CARTESIAN_POINT('Ctrl Pts',(38.8754551810142,0.182212749011649,
61.8381759929426));
#153554=CARTESIAN_POINT('Ctrl Pts',(38.8754435586669,0.355643354741394,
61.8398207203825));
#153555=CARTESIAN_POINT('Ctrl Pts',(38.8753693043867,0.524797406056961,
61.842849969035));
#153556=CARTESIAN_POINT('Ctrl Pts',(38.8752921578751,0.70054006989275,61.8459972080368));
#153557=CARTESIAN_POINT('Ctrl Pts',(38.8751474499859,0.871666670567132,
61.8506388441163));
#153558=CARTESIAN_POINT('Ctrl Pts',(38.8748656192459,1.03812127927734,61.856545897734));
#153559=CARTESIAN_POINT('Ctrl Pts',(38.8745997571531,1.19514450039705,61.8621182552288));
#153560=CARTESIAN_POINT('Ctrl Pts',(38.8742124586965,1.34801070455855,61.8688167552262));
#153561=CARTESIAN_POINT('Ctrl Pts',(38.8736767940754,1.4967002041647,61.8764574414583));
#153562=CARTESIAN_POINT('Ctrl Pts',(38.8730494572866,1.6708360151668,61.8854057336857));
#153563=CARTESIAN_POINT('Ctrl Pts',(38.8722176733478,1.83924498920277,61.8956455149775));
#153564=CARTESIAN_POINT('Ctrl Pts',(38.8711772778275,2.00200098431962,61.9068852202791));
#153565=CARTESIAN_POINT('Ctrl Pts',(38.8705113478883,2.10617683649829,61.9140794614326));
#153566=CARTESIAN_POINT('Ctrl Pts',(38.8697610056539,2.20803694311787,61.9216837821204));
#153567=CARTESIAN_POINT('Ctrl Pts',(38.868935031263,2.30760310302302,61.9296261375732));
#153568=CARTESIAN_POINT('Ctrl Pts',(38.8675127054407,2.47905577977653,61.9433028536724));
#153569=CARTESIAN_POINT('Ctrl Pts',(38.8657829944992,2.64360896180348,61.9579874501031));
#153570=CARTESIAN_POINT('Ctrl Pts',(38.8636834250032,2.80126596185201,61.9733446717352));
#153571=CARTESIAN_POINT('Ctrl Pts',(38.8628086667356,2.86695169624411,61.979743057984));
#153572=CARTESIAN_POINT('Ctrl Pts',(38.8618702826237,2.93144046537901,61.9862584852745));
#153573=CARTESIAN_POINT('Ctrl Pts',(38.8608660096394,2.9947329449184,61.9928679340296));
#153574=CARTESIAN_POINT('Ctrl Pts',(38.859611295864,3.07380900012709,62.0011256154865));
#153575=CARTESIAN_POINT('Ctrl Pts',(38.8582534042406,3.15101777476518,62.0095300980127));
#153576=CARTESIAN_POINT('Ctrl Pts',(38.8567796333586,3.22636338050231,62.0180418815993));
#153577=CARTESIAN_POINT('Ctrl Pts',(38.8540373162935,3.36656260882913,62.0338801707583));
#153578=CARTESIAN_POINT('Ctrl Pts',(38.8509044609947,3.50030572704103,62.0500863045402));
#153579=CARTESIAN_POINT('Ctrl Pts',(38.8473375827046,3.62760922988561,62.0664136645151));
#153580=CARTESIAN_POINT('Ctrl Pts',(38.8455541435595,3.6912609813079,62.0745773445025));
#153581=CARTESIAN_POINT('Ctrl Pts',(38.8436622557374,3.75330289609045,62.0827716535668));
#153582=CARTESIAN_POINT('Ctrl Pts',(38.8416568331374,3.81373738325631,62.09096774022));
#153583=CARTESIAN_POINT('Ctrl Pts',(38.8406541218374,3.84395462683924,62.0950657835467));
#153584=CARTESIAN_POINT('Ctrl Pts',(38.8396230304044,3.873770010651,62.099164291412));
#153585=CARTESIAN_POINT('Ctrl Pts',(38.8385629455729,3.90318385970171,62.103259784658));
#153586=CARTESIAN_POINT('Ctrl Pts',(38.8380329031572,3.91789078422705,62.1053075312811));
#153587=CARTESIAN_POINT('Ctrl Pts',(38.8374956126186,3.93249732489038,62.1073545255331));
#153588=CARTESIAN_POINT('Ctrl Pts',(38.8369509986835,3.94700352213919,62.1094003403576));
#153589=CARTESIAN_POINT('Ctrl Pts',(38.8366786917159,3.9542566207636,62.1104232477698));
#153590=CARTESIAN_POINT('Ctrl Pts',(38.8364045539135,3.96148463352306,62.1114458604058));
#153591=CARTESIAN_POINT('Ctrl Pts',(38.8361285759556,3.96868756554229,62.112468125386));
#153592=CARTESIAN_POINT('Ctrl Pts',(38.8358525979978,3.97589049756151,62.1134903903662));
#153593=CARTESIAN_POINT('Ctrl Pts',(38.8356492511492,3.98116367204593,62.1142402930151));
#153594=CARTESIAN_POINT('Ctrl Pts',(38.8352951123537,3.99022112449758,62.1155338248086));
#153595=CARTESIAN_POINT('Ctrl Pts',(38.8285328412474,4.16317294389909,62.1402337808219));
#153596=CARTESIAN_POINT('Ctrl Pts',(38.8206410998247,4.33311250091768,62.1662914189214));
#153597=CARTESIAN_POINT('Ctrl Pts',(38.8115378492565,4.50003137234844,62.1935808853104));
#153598=CARTESIAN_POINT('Ctrl Pts',(38.8023180837981,4.66908668216695,62.2212196367328));
#153599=CARTESIAN_POINT('Ctrl Pts',(38.7918557192814,4.83504340502254,62.2501218691348));
#153600=CARTESIAN_POINT('Ctrl Pts',(38.7801187157006,4.99789823554354,62.2801498303958));
#153601=CARTESIAN_POINT('Ctrl Pts',(38.7681210309875,5.1643701035261,62.3108447185169));
#153602=CARTESIAN_POINT('Ctrl Pts',(38.7547915533566,5.32760067385293,62.3427158038281));
#153603=CARTESIAN_POINT('Ctrl Pts',(38.7401497505278,5.48759338691093,62.3756100036374));
#153604=CARTESIAN_POINT('Ctrl Pts',(38.7358564036623,5.53450729643028,62.3852554148819));
#153605=CARTESIAN_POINT('Ctrl Pts',(38.7314505608984,5.58114286099023,62.3949887615589));
#153606=CARTESIAN_POINT('Ctrl Pts',(38.7269335390551,5.62750029347685,62.4048061087723));
#153607=CARTESIAN_POINT('Ctrl Pts',(38.7163775057703,5.73583508071256,62.4277487128928));
#153608=CARTESIAN_POINT('Ctrl Pts',(38.7052028854674,5.84263827108527,62.4511494917308));
#153609=CARTESIAN_POINT('Ctrl Pts',(38.693382204351,5.94793326722577,62.4749706034504));
#153610=CARTESIAN_POINT('Ctrl Pts',(38.6772800292229,6.09136649677287,62.5074198091162));
#153611=CARTESIAN_POINT('Ctrl Pts',(38.6599794071874,6.23199997192202,62.5406479392232));
#153612=CARTESIAN_POINT('Ctrl Pts',(38.6414863883519,6.36981442588874,62.5745062423265));
#153613=CARTESIAN_POINT('Ctrl Pts',(38.6254519736731,6.48930676639268,62.6038631622058));
#153614=CARTESIAN_POINT('Ctrl Pts',(38.6085106387425,6.60669129998388,62.6336983904886));
#153615=CARTESIAN_POINT('Ctrl Pts',(38.5906480604823,6.72197766351148,62.6639307691723));
#153616=CARTESIAN_POINT('Ctrl Pts',(38.5817167713523,6.77962084527528,62.6790469585141));
#153617=CARTESIAN_POINT('Ctrl Pts',(38.5725551888408,6.83673946970737,62.694262535642));
#153618=CARTESIAN_POINT('Ctrl Pts',(38.5631616284874,6.89333483604516,62.7095679634777));
#153619=CARTESIAN_POINT('Ctrl Pts',(38.5584648483107,6.92163251921405,62.7172206773955));
#153620=CARTESIAN_POINT('Ctrl Pts',(38.5537100746504,6.94979938687568,62.7248958595933));
#153621=CARTESIAN_POINT('Ctrl Pts',(38.5488971028194,6.97783560032803,62.7325923515764));
#153622=CARTESIAN_POINT('Ctrl Pts',(38.5450906465819,7.00000872398614,62.7386793101011));
#153623=CARTESIAN_POINT('Ctrl Pts',(38.541055129008,7.02319790002491,62.7450838174653));
#153624=CARTESIAN_POINT('Ctrl Pts',(38.5372469778334,7.04479846112864,62.75108392236));
#153625=CARTESIAN_POINT('Ctrl Pts',(38.5362400140591,7.05051015206178,62.7526704896978));
#153626=CARTESIAN_POINT('Ctrl Pts',(38.5352491794564,7.0561108238743,62.7542286171872));
#153627=CARTESIAN_POINT('Ctrl Pts',(38.534283391879,7.06155243825886,62.7557446198548));
#153628=CARTESIAN_POINT('Ctrl Pts',(38.4950678675933,7.28250761105259,62.8173014681913));
#153629=CARTESIAN_POINT('Ctrl Pts',(38.4514677808959,7.49993410311113,62.8814236534411));
#153630=CARTESIAN_POINT('Ctrl Pts',(38.4034120046589,7.71374537848964,62.9478547481597));
#153631=CARTESIAN_POINT('Ctrl Pts',(38.353854388085,7.93423868926519,63.0163619491341));
#153632=CARTESIAN_POINT('Ctrl Pts',(38.2995586747863,8.15088734571122,63.0873245284362));
#153633=CARTESIAN_POINT('Ctrl Pts',(38.2404641286669,8.3636343684669,63.1604989037323));
#153634=CARTESIAN_POINT('Ctrl Pts',(38.1985944857594,8.5143697993545,63.2123443812733));
#153635=CARTESIAN_POINT('Ctrl Pts',(38.1543162113558,8.66314742523656,63.2653009763042));
#153636=CARTESIAN_POINT('Ctrl Pts',(38.1076107402353,8.80995754172659,63.3192933263533));
#153637=CARTESIAN_POINT('Ctrl Pts',(38.040477762247,9.0209777944362,63.3969002353602));
#153638=CARTESIAN_POINT('Ctrl Pts',(37.9683308415603,9.22793205243882,63.476645035497));
#153639=CARTESIAN_POINT('Ctrl Pts',(37.8911667027997,9.43083440096504,63.5582971365134));
#153640=CARTESIAN_POINT('Ctrl Pts',(37.8131087081171,9.63608713490014,63.6408950812237));
#153641=CARTESIAN_POINT('Ctrl Pts',(37.7299171586969,9.8371938291356,63.7254447963416));
#153642=CARTESIAN_POINT('Ctrl Pts',(37.6415778233655,10.0341968982806,63.8117514604914));
#153643=CARTESIAN_POINT('Ctrl Pts',(37.5533472488685,10.2309574229453,63.8979518663727));
#153644=CARTESIAN_POINT('Ctrl Pts',(37.4599821147105,10.4236247681885,63.9859049945857));
#153645=CARTESIAN_POINT('Ctrl Pts',(37.3614490022685,10.6122639308637,64.0754591935364));
#153646=CARTESIAN_POINT('Ctrl Pts',(37.2641660718243,10.7985096515844,64.163877134385));
#153647=CARTESIAN_POINT('Ctrl Pts',(37.1618459602365,10.980829119707,64.2538559225466));
#153648=CARTESIAN_POINT('Ctrl Pts',(37.0544300457932,11.1593017562432,64.3452890788976));
#153649=CARTESIAN_POINT('Ctrl Pts',(36.9976569986222,11.2536307526987,64.3936146824677));
#153650=CARTESIAN_POINT('Ctrl Pts',(36.9394599539417,11.3468853923056,64.4423472142503));
#153651=CARTESIAN_POINT('Ctrl Pts',(36.8798265043843,11.4390788310839,64.491475300858));
#153652=CARTESIAN_POINT('Origin',(35.5956616019292,14.4895299089392,57.2082295467003));
#153653=CARTESIAN_POINT('Ctrl Pts',(35.8543614565591,13.15204220094,65.45231182744));
#153654=CARTESIAN_POINT('Ctrl Pts',(32.4237988913791,11.23764088211,65.205920002004));
#153655=CARTESIAN_POINT('Ctrl Pts',(29.3253632443791,10.80309640319,62.81729045488));
#153656=CARTESIAN_POINT('Ctrl Pts',(27.9368279710891,12.04170148852,59.34846031169));
#153657=CARTESIAN_POINT('Ctrl Pts',(36.3019357589691,12.58434307729,65.092157074978));
#153658=CARTESIAN_POINT('Ctrl Pts',(32.7688116514491,10.68400218145,64.923549223214));
#153659=CARTESIAN_POINT('Ctrl Pts',(29.5936770628891,10.26603134238,62.50254428216));
#153660=CARTESIAN_POINT('Ctrl Pts',(28.2340161075791,11.52235912053,58.94033961831));
#153661=CARTESIAN_POINT('Ctrl Pts',(36.7244351862591,11.99194848018,64.746982746171));
#153662=CARTESIAN_POINT('Ctrl Pts',(33.0867885711591,10.11975548635,64.661809058638));
#153663=CARTESIAN_POINT('Ctrl Pts',(29.8375082935191,9.71937111787702,62.20880149968));
#153664=CARTESIAN_POINT('Ctrl Pts',(28.5143069408691,10.98034479711,58.54871055167));
#153665=CARTESIAN_POINT('Ctrl Pts',(37.1146182133191,11.38351121538,64.4248079792711));
#153666=CARTESIAN_POINT('Ctrl Pts',(33.3745126141391,9.55513834427301,64.424781466774));
#153667=CARTESIAN_POINT('Ctrl Pts',(30.0553047540791,9.17314039863302,61.94111101675));
#153668=CARTESIAN_POINT('Ctrl Pts',(28.7730289746491,10.42357140722,58.18289110879));
#153669=CARTESIAN_POINT('Ctrl Pts',(36.8798265045291,11.43907883074,64.491475301679));
#153670=CARTESIAN_POINT('Ctrl Pts',(36.5447601595308,11.9562440716563,64.7671593619721));
#153671=CARTESIAN_POINT('Ctrl Pts',(36.1868105242993,12.4615090948357,65.059084102699));
#153672=CARTESIAN_POINT('Ctrl Pts',(35.8057492437391,12.9545337474,65.365954457758));
#153673=CARTESIAN_POINT('Origin',(62.4468966735091,1.4210854715202E-14,
88.14465325204));
#153674=CARTESIAN_POINT('',(59.2279850657691,10.8294941091,60.30347098134));
#153675=CARTESIAN_POINT('Ctrl Pts',(62.2792373804993,12.9545454545494,60.6979699644412));
#153676=CARTESIAN_POINT('Ctrl Pts',(61.8897073835902,12.7338209487284,60.6593514763456));
#153677=CARTESIAN_POINT('Ctrl Pts',(61.5099484134262,12.5022554868387,60.6170931465005));
#153678=CARTESIAN_POINT('Ctrl Pts',(61.1401151554292,12.2595992725174,60.5719752910757));
#153679=CARTESIAN_POINT('Ctrl Pts',(60.7728430689499,12.0186235024809,60.5271698860965));
#153680=CARTESIAN_POINT('Ctrl Pts',(60.4153597015435,11.7667100689689,60.47954440569));
#153681=CARTESIAN_POINT('Ctrl Pts',(60.0678070782513,11.5036136977798,60.429913403337));
#153682=CARTESIAN_POINT('Ctrl Pts',(59.7810828472561,11.2865642507285,60.3889687807691));
#153683=CARTESIAN_POINT('Ctrl Pts',(59.5011172473088,11.061903765029,60.3466601017626));
#153684=CARTESIAN_POINT('Ctrl Pts',(59.2279850656438,10.8294941093792,60.3034709806296));
#153685=CARTESIAN_POINT('',(59.2279850657991,-10.82949410913,60.30347098135));
#153686=CARTESIAN_POINT('Ctrl Pts',(59.2279850656426,10.8294941093819,60.3034709806228));
#153687=CARTESIAN_POINT('Ctrl Pts',(59.0590795829281,10.6857595475055,60.2767580663414));
#153688=CARTESIAN_POINT('Ctrl Pts',(58.8934066931531,10.5376026455191,60.2491609098041));
#153689=CARTESIAN_POINT('Ctrl Pts',(58.7309616758768,10.3850122881246,60.2208262862206));
#153690=CARTESIAN_POINT('Ctrl Pts',(58.570753726094,10.2345232874479,60.1928818652202));
#153691=CARTESIAN_POINT('Ctrl Pts',(58.4136850934738,10.0797216908457,60.1642198447616));
#153692=CARTESIAN_POINT('Ctrl Pts',(58.2597950174985,9.92057176318211,60.1349835210994));
#153693=CARTESIAN_POINT('Ctrl Pts',(58.2038786422741,9.86274420662415,60.1243604238418));
#153694=CARTESIAN_POINT('Ctrl Pts',(58.1483823586069,9.80434234877015,60.1136615506583));
#153695=CARTESIAN_POINT('Ctrl Pts',(58.0933096167251,9.74536380024524,60.1028939810487));
#153696=CARTESIAN_POINT('Ctrl Pts',(57.9458021331067,9.58739495789036,60.0740539951769));
#153697=CARTESIAN_POINT('Ctrl Pts',(57.8013160487736,9.42529668230862,60.0447253867283));
#153698=CARTESIAN_POINT('Ctrl Pts',(57.6598752169046,9.25904163467008,60.0150721757949));
#153699=CARTESIAN_POINT('Ctrl Pts',(57.628562885117,9.22223590365005,60.0085075143244));
#153700=CARTESIAN_POINT('Ctrl Pts',(57.5973999739887,9.18522635045155,60.0019269632268));
#153701=CARTESIAN_POINT('Ctrl Pts',(57.5663870484643,9.14801251292571,59.9953323409695));
#153702=CARTESIAN_POINT('Ctrl Pts',(57.4808363932956,9.04535634205985,59.9771407564877));
#153703=CARTESIAN_POINT('Ctrl Pts',(57.3964251327715,8.9411467102242,59.9588425419686));
#153704=CARTESIAN_POINT('Ctrl Pts',(57.3131606483973,8.83537641227296,59.9404797170312));
#153705=CARTESIAN_POINT('Ctrl Pts',(57.2715284062101,8.78249126329734,59.9312983045624));
#153706=CARTESIAN_POINT('Ctrl Pts',(57.2301828662008,8.72921592957571,59.9221007847856));
#153707=CARTESIAN_POINT('Ctrl Pts',(57.1891250082528,8.67554951902579,59.9128927285279));
#153708=CARTESIAN_POINT('Ctrl Pts',(57.1634523238683,8.64199295058918,59.9071351090632));
#153709=CARTESIAN_POINT('Ctrl Pts',(57.1374312224451,8.60767483826395,59.9012695327338));
#153710=CARTESIAN_POINT('Ctrl Pts',(57.1119290737584,8.57373520574596,59.8954922629261));
#153711=CARTESIAN_POINT('Ctrl Pts',(57.0976552888904,8.55473888433728,59.8922586724011));
#153712=CARTESIAN_POINT('Ctrl Pts',(57.0835432510979,8.5358616141826,59.8890527294345));
#153713=CARTESIAN_POINT('Ctrl Pts',(57.0697388483035,8.51730679825192,59.8859086612033));
#153714=CARTESIAN_POINT('Ctrl Pts',(57.0687628449579,8.51599492966228,59.8856863682756));
#153715=CARTESIAN_POINT('Ctrl Pts',(57.0677883776336,8.51468467394813,59.8854643845792));
#153716=CARTESIAN_POINT('Ctrl Pts',(57.0668154970974,8.513376103457,59.8852427221799));
#153717=CARTESIAN_POINT('Ctrl Pts',(56.9398671014472,8.34262448671979,59.8563186303476));
#153718=CARTESIAN_POINT('Ctrl Pts',(56.8175157456154,8.17037242182476,59.8277440127108));
#153719=CARTESIAN_POINT('Ctrl Pts',(56.6997399809284,7.9966358962389,59.7995971606568));
#153720=CARTESIAN_POINT('Ctrl Pts',(56.5812815801934,7.82189238236865,59.7712871676042));
#153721=CARTESIAN_POINT('Ctrl Pts',(56.4674518916248,7.64564667420447,59.7434096701134));
#153722=CARTESIAN_POINT('Ctrl Pts',(56.358279023726,7.46789973214102,59.7160500410813));
#153723=CARTESIAN_POINT('Ctrl Pts',(56.3085945078996,7.38700719055972,59.7035986880317));
#153724=CARTESIAN_POINT('Ctrl Pts',(56.2598751796783,7.30580355524723,59.691254693885));
#153725=CARTESIAN_POINT('Ctrl Pts',(56.2121271546688,7.22428827363687,59.6790266927907));
#153726=CARTESIAN_POINT('Ctrl Pts',(56.2106478891286,7.22176287605111,59.6786478611921));
#153727=CARTESIAN_POINT('Ctrl Pts',(56.2091695560213,7.21923717932473,59.6782691409578));
#153728=CARTESIAN_POINT('Ctrl Pts',(56.2076921551256,7.21671118302507,59.6778905323204));
#153729=CARTESIAN_POINT('Ctrl Pts',(56.0786259342956,6.99603932802176,59.6448151591173));
#153730=CARTESIAN_POINT('Ctrl Pts',(55.9566410081673,6.77309191637419,59.6125985100089));
#153731=CARTESIAN_POINT('Ctrl Pts',(55.8417738725684,6.54788192837225,59.5814482300864));
#153732=CARTESIAN_POINT('Ctrl Pts',(55.784340304769,6.43527693437129,59.5658730901252));
#153733=CARTESIAN_POINT('Ctrl Pts',(55.7286862328209,6.32210634815834,59.5505648401431));
#153734=CARTESIAN_POINT('Ctrl Pts',(55.6748165509668,6.20837284521694,59.5355513624588));
#153735=CARTESIAN_POINT('Ctrl Pts',(55.6462508535993,6.14806291366084,59.5275901040069));
#153736=CARTESIAN_POINT('Ctrl Pts',(55.6179612615491,6.08710656462898,59.519648101766));
#153737=CARTESIAN_POINT('Ctrl Pts',(55.5903126041415,6.02627911558751,59.5118318947263));
#153738=CARTESIAN_POINT('Ctrl Pts',(55.5658209493739,5.97239711834083,59.5049081645218));
#153739=CARTESIAN_POINT('Ctrl Pts',(55.5418314797697,5.9186165509691,59.4980830580316));
#153740=CARTESIAN_POINT('Ctrl Pts',(55.5185657968262,5.86548670373654,59.4914243363906));
#153741=CARTESIAN_POINT('Ctrl Pts',(55.4156138859168,5.63038424350782,59.4619591314012));
#153742=CARTESIAN_POINT('Ctrl Pts',(55.3194484791371,5.39295812998054,59.4339787906589));
#153743=CARTESIAN_POINT('Ctrl Pts',(55.2298705468524,5.15304981258439,59.4075238454497));
#153744=CARTESIAN_POINT('Ctrl Pts',(55.1435432835686,4.9218474622776,59.3820289164869));
#153745=CARTESIAN_POINT('Ctrl Pts',(55.0633348246565,4.68833991247754,59.3579508911544));
#153746=CARTESIAN_POINT('Ctrl Pts',(54.9891061163647,4.4523992880887,59.3353451301884));
#153747=CARTESIAN_POINT('Ctrl Pts',(54.9143193404503,4.21468481061334,59.3125694141799));
#153748=CARTESIAN_POINT('Ctrl Pts',(54.8456021618042,3.97449950281697,59.2912881697926));
#153749=CARTESIAN_POINT('Ctrl Pts',(54.7831355984502,3.732100756132,59.2715977724828));
#153750=CARTESIAN_POINT('Ctrl Pts',(54.724323975159,3.50388484331681,59.2530594670783));
#153751=CARTESIAN_POINT('Ctrl Pts',(54.671053301148,3.27370683043166,59.2359314995989));
#153752=CARTESIAN_POINT('Ctrl Pts',(54.6235060357775,3.04180580456216,59.2203087503871));
#153753=CARTESIAN_POINT('Ctrl Pts',(54.6202808930024,3.02607590059592,59.2192490554424));
#153754=CARTESIAN_POINT('Ctrl Pts',(54.6170815819542,3.01033757179436,59.2181963285862));
#153755=CARTESIAN_POINT('Ctrl Pts',(54.6139081016492,2.99459087982342,59.2171506133393));
#153756=CARTESIAN_POINT('Ctrl Pts',(54.5654562732485,2.75417469824556,59.2011849192656));
#153757=CARTESIAN_POINT('Ctrl Pts',(54.523021719713,2.51180993797416,59.1868522684903));
#153758=CARTESIAN_POINT('Ctrl Pts',(54.4865661577128,2.26747671758865,59.1743098336218));
#153759=CARTESIAN_POINT('Ctrl Pts',(54.4504614062033,2.02549470651829,59.1618880941284));
#153760=CARTESIAN_POINT('Ctrl Pts',(54.420221143089,1.78158156531106,59.1512220156086));
#153761=CARTESIAN_POINT('Ctrl Pts',(54.3958549336375,1.53571073982857,59.1424830742769));
#153762=CARTESIAN_POINT('Ctrl Pts',(54.3711335941183,1.28625642208994,59.1336167655419));
#153763=CARTESIAN_POINT('Ctrl Pts',(54.3524586267359,1.03478658610385,59.1267338002371));
#153764=CARTESIAN_POINT('Ctrl Pts',(54.339889719583,0.781271445267059,59.122037673447));
#153765=CARTESIAN_POINT('Ctrl Pts',(54.3273208124301,0.527756304430266,
59.117341546657));
#153766=CARTESIAN_POINT('Ctrl Pts',(54.3208579646841,0.2721955082923,59.1148319135422));
#153767=CARTESIAN_POINT('Ctrl Pts',(54.320611205963,0.0145625469582074,
59.114741865325));
#153768=CARTESIAN_POINT('Ctrl Pts',(54.3203494715567,-0.258706052728112,
59.1146463521185));
#153769=CARTESIAN_POINT('Ctrl Pts',(54.3270837351186,-0.529930243673467,
59.1172754622834));
#153770=CARTESIAN_POINT('Ctrl Pts',(54.3407128965343,-0.799028173290029,
59.1223642792772));
#153771=CARTESIAN_POINT('Ctrl Pts',(54.3545066696695,-1.07137624218956,
59.1275145585203));
#153772=CARTESIAN_POINT('Ctrl Pts',(54.3753628104337,-1.34154672703684,
59.1351846587339));
#153773=CARTESIAN_POINT('Ctrl Pts',(54.4032218321361,-1.60945722250699,
59.1451294739156));
#153774=CARTESIAN_POINT('Ctrl Pts',(54.4315877950223,-1.88224279453792,
59.1552552515315));
#153775=CARTESIAN_POINT('Ctrl Pts',(54.4672137438209,-2.15268581224499,
59.1677396219718));
#153776=CARTESIAN_POINT('Ctrl Pts',(54.5100848851986,-2.42069585734544,
59.1823491365729));
#153777=CARTESIAN_POINT('Ctrl Pts',(54.5394027880972,-2.60397748283012,
59.1923400142753));
#153778=CARTESIAN_POINT('Ctrl Pts',(54.5721100330777,-2.78612122246499,
59.2033252772472));
#153779=CARTESIAN_POINT('Ctrl Pts',(54.6082145668267,-2.96709559377786,
59.2152355980989));
#153780=CARTESIAN_POINT('Ctrl Pts',(54.6116595092352,-2.98436340537522,
59.2163720307056));
#153781=CARTESIAN_POINT('Ctrl Pts',(54.6151353887236,-3.00162056868052,
59.217516887937));
#153782=CARTESIAN_POINT('Ctrl Pts',(54.6186422447928,-3.01886702602003,
59.2186701098161));
#153783=CARTESIAN_POINT('Ctrl Pts',(54.6685109495927,-3.26411760743095,
59.2350693233336));
#153784=CARTESIAN_POINT('Ctrl Pts',(54.7246069067787,-3.50723131290814,
59.2531671796548));
#153785=CARTESIAN_POINT('Ctrl Pts',(54.7868883723096,-3.74814573278264,
59.272844922212));
#153786=CARTESIAN_POINT('Ctrl Pts',(54.848836712347,-3.98777157130564,59.2924174142321));
#153787=CARTESIAN_POINT('Ctrl Pts',(54.9169044303602,-4.22522200340054,
59.3135530070516));
#153788=CARTESIAN_POINT('Ctrl Pts',(54.9910949979195,-4.46045128752221,
59.3361544451959));
#153789=CARTESIAN_POINT('Ctrl Pts',(55.0654850443464,-4.69631304114448,
59.3588166526459));
#153790=CARTESIAN_POINT('Ctrl Pts',(55.146020717095,-4.92993807118413,59.3829539452067));
#153791=CARTESIAN_POINT('Ctrl Pts',(55.2326893264597,-5.16127026167754,
59.4084942759323));
#153792=CARTESIAN_POINT('Ctrl Pts',(55.276023631142,-5.27693635692425,59.421264441295));
#153793=CARTESIAN_POINT('Ctrl Pts',(55.3208912335958,-5.39202908955734,
59.4343857088369));
#153794=CARTESIAN_POINT('Ctrl Pts',(55.3672909336742,-5.50654108903935,
59.4478512005941));
#153795=CARTESIAN_POINT('Ctrl Pts',(55.3904907837134,-5.56379708878036,
59.4545839464727));
#153796=CARTESIAN_POINT('Ctrl Pts',(55.4140736618391,-5.62090789344703,
59.4614027690403));
#153797=CARTESIAN_POINT('Ctrl Pts',(55.4380394395861,-5.67787252503938,
59.4683069334854));
#153798=CARTESIAN_POINT('Ctrl Pts',(55.4500223284596,-5.70635484083555,
59.471759015708));
#153799=CARTESIAN_POINT('Ctrl Pts',(55.4621009424477,-5.73480061255788,
59.4752324346489));
#153800=CARTESIAN_POINT('Ctrl Pts',(55.4742752667805,-5.76320971526244,
59.4787271063192));
#153801=CARTESIAN_POINT('Ctrl Pts',(55.4803624289469,-5.77741426661473,
59.4804744421543));
#153802=CARTESIAN_POINT('Ctrl Pts',(55.4864735187118,-5.79160965066008,
59.4822270912488));
#153803=CARTESIAN_POINT('Ctrl Pts',(55.4926085343061,-5.8057958516082,59.4839850435921));
#153804=CARTESIAN_POINT('Ctrl Pts',(55.4987435499005,-5.81998205255631,
59.4857429959354));
#153805=CARTESIAN_POINT('Ctrl Pts',(55.5044550657775,-5.83313381049701,
59.4873782697557));
#153806=CARTESIAN_POINT('Ctrl Pts',(55.5110853568569,-5.84832688919887,
59.4892748006713));
#153807=CARTESIAN_POINT('Ctrl Pts',(55.6016461484042,-6.05584375637715,
59.5151788430206));
#153808=CARTESIAN_POINT('Ctrl Pts',(55.6969727210893,-6.25997357036908,
59.5419952418224));
#153809=CARTESIAN_POINT('Ctrl Pts',(55.7968887123826,-6.46077599426773,
59.5695027589807));
#153810=CARTESIAN_POINT('Ctrl Pts',(55.8993092391477,-6.66661181459251,
59.5976997909161));
#153811=CARTESIAN_POINT('Ctrl Pts',(56.0065521001706,-6.86895162215178,
59.6266232452781));
#153812=CARTESIAN_POINT('Ctrl Pts',(56.1184762778283,-7.06786023839376,
59.656059786709));
#153813=CARTESIAN_POINT('Ctrl Pts',(56.2317422028379,-7.26915337167839,
59.68584921348));
#153814=CARTESIAN_POINT('Ctrl Pts',(56.3498024034668,-7.46693284995802,
59.7161643869244));
#153815=CARTESIAN_POINT('Ctrl Pts',(56.4725600911692,-7.66126201797403,
59.7468055032499));
#153816=CARTESIAN_POINT('Ctrl Pts',(56.5969927808993,-7.85824276534574,
59.777864710963));
#153817=CARTESIAN_POINT('Ctrl Pts',(56.7262520472292,-8.05167871602991,
59.8092591046023));
#153818=CARTESIAN_POINT('Ctrl Pts',(56.8602869895031,-8.24162728614395,
59.8407979957789));
#153819=CARTESIAN_POINT('Ctrl Pts',(56.9239377896736,-8.33183046953685,
59.855775251902));
#153820=CARTESIAN_POINT('Ctrl Pts',(56.9886662855614,-8.42124704991932,
59.8707853182742));
#153821=CARTESIAN_POINT('Ctrl Pts',(57.0544708651079,-8.50988220134331,
59.8858088337675));
#153822=CARTESIAN_POINT('Ctrl Pts',(57.1933423107988,-8.69693440503645,
59.9175138812017));
#153823=CARTESIAN_POINT('Ctrl Pts',(57.3370030268218,-8.88050745517193,
59.9492783279215));
#153824=CARTESIAN_POINT('Ctrl Pts',(57.4854155525887,-9.06060085278201,
59.9809314046518));
#153825=CARTESIAN_POINT('Ctrl Pts',(57.6345467173149,-9.24156629357823,
60.0127377510201));
#153826=CARTESIAN_POINT('Ctrl Pts',(57.7884759610297,-9.41901866773446,
60.0444319421711));
#153827=CARTESIAN_POINT('Ctrl Pts',(57.9472137328405,-9.59293834494708,
60.0758466724522));
#153828=CARTESIAN_POINT('Ctrl Pts',(58.1056349933134,-9.76651123922892,
60.1071987640921));
#153829=CARTESIAN_POINT('Ctrl Pts',(58.2688457995564,-9.93656585419427,
60.1382728031));
#153830=CARTESIAN_POINT('Ctrl Pts',(58.4369022484652,-10.1030583892898,
60.1689039612922));
#153831=CARTESIAN_POINT('Ctrl Pts',(58.6034090924211,-10.2680157398762,
60.1992526775147));
#153832=CARTESIAN_POINT('Ctrl Pts',(58.7746728320292,-10.4294766998782,
60.2291669206477));
#153833=CARTESIAN_POINT('Ctrl Pts',(58.95079006548,-10.5873700501157,60.2584835746801));
#153834=CARTESIAN_POINT('Ctrl Pts',(59.0418834198168,-10.669037440744,60.2736470672095));
#153835=CARTESIAN_POINT('Ctrl Pts',(59.1342758914813,-10.749749898048,60.2886506162358));
#153836=CARTESIAN_POINT('Ctrl Pts',(59.2279850656721,-10.8294941094132,
60.3034709806296));
#153837=CARTESIAN_POINT('Ctrl Pts',(59.2279850656726,-10.8294941094118,
60.303470980633));
#153838=CARTESIAN_POINT('Ctrl Pts',(59.5767424389413,-11.1262539191291,
60.3586184675425));
#153839=CARTESIAN_POINT('Ctrl Pts',(59.9366440777721,-11.4103793077849,
60.4123224458978));
#153840=CARTESIAN_POINT('Ctrl Pts',(60.3075303353131,-11.6821583996076,
60.4635928169708));
#153841=CARTESIAN_POINT('Ctrl Pts',(60.6796998531796,-11.9548778425992,
60.5150405826809));
#153842=CARTESIAN_POINT('Ctrl Pts',(61.0629301323383,-12.2151653842106,
60.564037881877));
#153843=CARTESIAN_POINT('Ctrl Pts',(61.4570510653701,-12.4633103583552,
60.6096360877662));
#153844=CARTESIAN_POINT('Ctrl Pts',(61.7260584762589,-12.6326818162633,
60.6407591626383));
#153845=CARTESIAN_POINT('Ctrl Pts',(62.0001393885515,-12.7963963183867,
60.6702997600123));
#153846=CARTESIAN_POINT('Ctrl Pts',(62.2792373805004,-12.9545454545462,
60.6979699644477));
#153847=CARTESIAN_POINT('Ctrl Pts',(62.3623725079491,-13.1649643715,60.78391287288));
#153848=CARTESIAN_POINT('Ctrl Pts',(63.8217099690391,-11.20483377633,59.6461334374101));
#153849=CARTESIAN_POINT('Ctrl Pts',(64.7770536940892,-10.27834225011,57.30189869769));
#153850=CARTESIAN_POINT('Ctrl Pts',(64.8631085247691,-10.73979194701,54.64739874676));
#153851=CARTESIAN_POINT('Ctrl Pts',(61.1174740105891,-12.47994051503,60.66365145323));
#153852=CARTESIAN_POINT('Ctrl Pts',(62.7940792459991,-10.52306401831,59.5562432799201));
#153853=CARTESIAN_POINT('Ctrl Pts',(63.9019099705191,-9.63724577769599,
57.1388720445));
#153854=CARTESIAN_POINT('Ctrl Pts',(63.9901546224391,-10.18300062512,54.3950475618301));
#153855=CARTESIAN_POINT('Ctrl Pts',(59.9844193641791,-11.69588976856,60.50709666618));
#153856=CARTESIAN_POINT('Ctrl Pts',(61.8920759066391,-9.76298109347099,
59.44379451149));
#153857=CARTESIAN_POINT('Ctrl Pts',(63.1412817937692,-8.92499334381699,
56.95138240988));
#153858=CARTESIAN_POINT('Ctrl Pts',(63.1903745247891,-9.54533591150498,
54.11035997021));
#153859=CARTESIAN_POINT('Ctrl Pts',(58.9593897563791,-10.81129024408,60.3407081496501));
#153860=CARTESIAN_POINT('Ctrl Pts',(61.1067038788591,-8.94679575810299,
59.33391888342));
#153861=CARTESIAN_POINT('Ctrl Pts',(62.4867262093291,-8.16465088582199,
56.76779162634));
#153862=CARTESIAN_POINT('Ctrl Pts',(62.4637164412891,-8.82522553066699,
53.82421532476));
#153863=CARTESIAN_POINT('',(62.5668976793491,-8.89165927519551,54.0330209494394));
#153864=CARTESIAN_POINT('Ctrl Pts',(59.2279850657991,-10.82949410913,60.30347098135));
#153865=CARTESIAN_POINT('Ctrl Pts',(59.6576037928366,-10.4528243853097,
60.0796572311861));
#153866=CARTESIAN_POINT('Ctrl Pts',(60.0954495905067,-10.0900443262501,
59.7549266261475));
#153867=CARTESIAN_POINT('Ctrl Pts',(60.91252465905,-9.46575246404225,58.9076269594709));
#153868=CARTESIAN_POINT('Ctrl Pts',(61.2902828898919,-9.20568070081324,
58.385136210451));
#153869=CARTESIAN_POINT('Ctrl Pts',(61.9121932750885,-8.84473536319556,
57.2171883668237));
#153870=CARTESIAN_POINT('Ctrl Pts',(62.155331367146,-8.74445034487759,56.5736358012396));
#153871=CARTESIAN_POINT('Ctrl Pts',(62.4775613443828,-8.70751278667245,
55.2813284955923));
#153872=CARTESIAN_POINT('Ctrl Pts',(62.5571152908332,-8.77000581973829,
54.6343903912162));
#153873=CARTESIAN_POINT('Ctrl Pts',(62.5668978279891,-8.89165927519899,
54.03302179244));
#153874=CARTESIAN_POINT('',(64.7368422444091,-10.63636346571,54.76937978503));
#153875=CARTESIAN_POINT('Ctrl Pts',(64.7368422444113,-10.6363634657067,
54.7693797850296));
#153876=CARTESIAN_POINT('Ctrl Pts',(64.4705013672014,-10.4618582038463,
54.6889341849824));
#153877=CARTESIAN_POINT('Ctrl Pts',(64.2101814201152,-10.2786530461274,
54.6074269325054));
#153878=CARTESIAN_POINT('Ctrl Pts',(63.9564670518738,-10.0871970340218,
54.5247549382549));
#153879=CARTESIAN_POINT('Ctrl Pts',(63.7027404475878,-9.89573178844495,
54.4420789569294));
#153880=CARTESIAN_POINT('Ctrl Pts',(63.4556202456009,-9.69601504587226,
54.3582380886331));
#153881=CARTESIAN_POINT('Ctrl Pts',(63.2156587923114,-9.48853636535973,
54.2731349397934));
#153882=CARTESIAN_POINT('Ctrl Pts',(62.9931099547497,-9.29611321349957,
54.1942072345829));
#153883=CARTESIAN_POINT('Ctrl Pts',(62.776718406385,-9.09701424058528,54.1141938331589));
#153884=CARTESIAN_POINT('Ctrl Pts',(62.5668978279935,-8.89165927519479,
54.0330217924392));
#153885=CARTESIAN_POINT('Origin',(61.3394944160718,-15.5454545454696,55.368422775105));
#153886=CARTESIAN_POINT('Ctrl Pts',(84.0800519726791,-12.99512036682,56.87009645751));
#153887=CARTESIAN_POINT('Ctrl Pts',(83.6661946429091,-12.5469383764,56.75027017985));
#153888=CARTESIAN_POINT('Ctrl Pts',(82.7965369015191,-11.71844316471,56.33665948385));
#153889=CARTESIAN_POINT('Ctrl Pts',(81.4695020430691,-10.82009029684,55.18295003764));
#153890=CARTESIAN_POINT('Ctrl Pts',(80.3036938147791,-10.39648861976,53.64722176789));
#153891=CARTESIAN_POINT('Ctrl Pts',(79.7378359864291,-10.4635207436,52.51240603953));
#153892=CARTESIAN_POINT('Ctrl Pts',(79.5131204023091,-10.57285133752,51.94360802037));
#153893=CARTESIAN_POINT('Ctrl Pts',(83.2651276943291,-13.34120049562,57.18470057318));
#153894=CARTESIAN_POINT('Ctrl Pts',(82.8829401304591,-12.90294209031,57.0362090282));
#153895=CARTESIAN_POINT('Ctrl Pts',(82.0847138805391,-12.10130574004,56.58227996675));
#153896=CARTESIAN_POINT('Ctrl Pts',(80.8653217669191,-11.23972064159,55.43357173692));
#153897=CARTESIAN_POINT('Ctrl Pts',(79.7738747741391,-10.82877473082,53.95609666109));
#153898=CARTESIAN_POINT('Ctrl Pts',(79.2196176577691,-10.88586704929,52.87448522791));
#153899=CARTESIAN_POINT('Ctrl Pts',(78.9913181074791,-10.98810527869,52.33051917722));
#153900=CARTESIAN_POINT('Ctrl Pts',(81.6394458735691,-13.91964486991,57.81578810632));
#153901=CARTESIAN_POINT('Ctrl Pts',(81.3170669355891,-13.50761079111,57.62192240622));
#153902=CARTESIAN_POINT('Ctrl Pts',(80.6510324482591,-12.76589073325,57.1089812309));
#153903=CARTESIAN_POINT('Ctrl Pts',(79.6315581494091,-11.97266212853,55.97951292672));
#153904=CARTESIAN_POINT('Ctrl Pts',(78.6903991156591,-11.57564099902,54.60435686025));
#153905=CARTESIAN_POINT('Ctrl Pts',(78.1765730446491,-11.60238669821,53.61372744078));
#153906=CARTESIAN_POINT('Ctrl Pts',(77.9523738165591,-11.68373610129,53.11270985383));
#153907=CARTESIAN_POINT('Ctrl Pts',(79.4388619220891,-14.43965128122,58.6008316937));
#153908=CARTESIAN_POINT('Ctrl Pts',(79.1924362457891,-14.06465275778,58.36868006312));
#153909=CARTESIAN_POINT('Ctrl Pts',(78.6866339965491,-13.39597478952,57.81107313064));
#153910=CARTESIAN_POINT('Ctrl Pts',(77.9069917824891,-12.6721700663,56.70787752612));
#153911=CARTESIAN_POINT('Ctrl Pts',(77.1657033515691,-12.2788510491,55.42701703778));
#153912=CARTESIAN_POINT('Ctrl Pts',(76.7353144646191,-12.2605680305,54.51917695659));
#153913=CARTESIAN_POINT('Ctrl Pts',(76.5382941560091,-12.31045564282,54.05817220228));
#153914=CARTESIAN_POINT('Ctrl Pts',(77.6162987730291,-14.73391373999,59.17156261559));
#153915=CARTESIAN_POINT('Ctrl Pts',(77.4292728693391,-14.38230171041,58.91782585669));
#153916=CARTESIAN_POINT('Ctrl Pts',(77.0457870997091,-13.757827987,58.33523259925));
#153917=CARTESIAN_POINT('Ctrl Pts',(76.4492311625191,-13.07397037488,57.24426156275));
#153918=CARTESIAN_POINT('Ctrl Pts',(75.8697775008791,-12.68142066445,56.01101958947));
#153919=CARTESIAN_POINT('Ctrl Pts',(75.5201084752091,-12.63506048891,55.14560797757));
#153920=CARTESIAN_POINT('Ctrl Pts',(75.3554576632691,-12.66496377676,54.70525314943));
#153921=CARTESIAN_POINT('Ctrl Pts',(76.2071628757491,-14.8934563637,59.56388257989));
#153922=CARTESIAN_POINT('Ctrl Pts',(76.0650224041191,-14.55550964164,59.29702655635));
#153923=CARTESIAN_POINT('Ctrl Pts',(75.7724199604191,-13.95625819436,58.69824636597));
#153924=CARTESIAN_POINT('Ctrl Pts',(75.3109369339791,-13.29449480621,57.60945441332));
#153925=CARTESIAN_POINT('Ctrl Pts',(74.8536355956291,-12.90182964091,56.39722064014));
#153926=CARTESIAN_POINT('Ctrl Pts',(74.5692627635191,-12.83911853561,55.55187457973));
#153927=CARTESIAN_POINT('Ctrl Pts',(74.4326271289791,-12.85728762685,55.12140910176));
#153928=CARTESIAN_POINT('Ctrl Pts',(74.7602603369891,-14.99086818853,59.91232469828));
#153929=CARTESIAN_POINT('Ctrl Pts',(74.6637866458491,-14.66200007839,59.6349011036));
#153930=CARTESIAN_POINT('Ctrl Pts',(74.4621882103191,-14.07915129287,59.02122513388));
#153931=CARTESIAN_POINT('Ctrl Pts',(74.1342948725691,-13.431302473,57.92606828431));
#153932=CARTESIAN_POINT('Ctrl Pts',(73.7988562189591,-13.03810819612,56.71909544721));
#153933=CARTESIAN_POINT('Ctrl Pts',(73.5820799877991,-12.96445387057,55.88141223042));
#153934=CARTESIAN_POINT('Ctrl Pts',(73.4755239802991,-12.97474890777,55.45483672956));
#153935=CARTESIAN_POINT('Ctrl Pts',(73.2774620481891,-15.02379049898,60.20753715318));
#153936=CARTESIAN_POINT('Ctrl Pts',(73.2272578267591,-14.69834531273,59.92141206142));
#153937=CARTESIAN_POINT('Ctrl Pts',(73.1168676334091,-14.1215596745,59.29259789444));
#153938=CARTESIAN_POINT('Ctrl Pts',(72.9214777686291,-13.47866908886,58.18047859039));
#153939=CARTESIAN_POINT('Ctrl Pts',(72.7071889548991,-13.08505255241,56.9615075124));
#153940=CARTESIAN_POINT('Ctrl Pts',(72.5588984830791,-13.00718824553,56.11840724491));
#153941=CARTESIAN_POINT('Ctrl Pts',(72.4834297908491,-13.01446680747,55.68943757256));
#153942=CARTESIAN_POINT('Ctrl Pts',(71.7826488958691,-14.99006392632,60.43659409979));
#153943=CARTESIAN_POINT('Ctrl Pts',(71.7789295473791,-14.6611250522,60.1428335071));
#153944=CARTESIAN_POINT('Ctrl Pts',(71.7594710721691,-14.07814838366,59.49702773573));
#153945=CARTESIAN_POINT('Ctrl Pts',(71.6944226714991,-13.43019013293,58.35538254833));
#153946=CARTESIAN_POINT('Ctrl Pts',(71.5980645007491,-13.03699746572,57.10603814888));
#153947=CARTESIAN_POINT('Ctrl Pts',(71.5159400922591,-12.96342646928,56.24445554096));
#153948=CARTESIAN_POINT('Ctrl Pts',(71.4704731886791,-12.97378221592,55.80703477539));
#153949=CARTESIAN_POINT('Ctrl Pts',(69.8115991120691,-14.85944831896,60.65919191265));
#153950=CARTESIAN_POINT('Ctrl Pts',(69.8699356568591,-14.51834940535,60.35791581069));
#153951=CARTESIAN_POINT('Ctrl Pts',(69.9713126105991,-13.91339295952,59.6893510355));
#153952=CARTESIAN_POINT('Ctrl Pts',(70.0764973366891,-13.24677567487,58.49470358249));
#153953=CARTESIAN_POINT('Ctrl Pts',(70.1302881609591,-12.85427967805,57.18301095558));
#153954=CARTESIAN_POINT('Ctrl Pts',(70.1292194872591,-12.79536407084,56.28083629208));
#153955=CARTESIAN_POINT('Ctrl Pts',(70.1195867559491,-12.81626401359,55.82474063768));
#153956=CARTESIAN_POINT('Ctrl Pts',(67.3973149529291,-14.53891337949,60.79998145237));
#153957=CARTESIAN_POINT('Ctrl Pts',(67.5334496752791,-14.17098221515,60.49568646605));
#153958=CARTESIAN_POINT('Ctrl Pts',(67.7865544822591,-13.51623522621,59.80123462312));
#153959=CARTESIAN_POINT('Ctrl Pts',(68.1007762587091,-12.80566305584,58.51830879814));
#153960=CARTESIAN_POINT('Ctrl Pts',(68.3297419833491,-12.41304472226,57.09105979811));
#153961=CARTESIAN_POINT('Ctrl Pts',(68.4141870978591,-12.38616952145,56.1109805838));
#153962=CARTESIAN_POINT('Ctrl Pts',(68.4394260012791,-12.43005186544,55.61929350187));
#153963=CARTESIAN_POINT('Ctrl Pts',(64.6154734129691,-13.91879763618,60.81696389427));
#153964=CARTESIAN_POINT('Ctrl Pts',(64.8521749835191,-13.50671310406,60.52453930129));
#153965=CARTESIAN_POINT('Ctrl Pts',(65.3027548701191,-12.76489017189,59.81471204003));
#153966=CARTESIAN_POINT('Ctrl Pts',(65.8746443789191,-11.9715608226,58.40452801752));
#153967=CARTESIAN_POINT('Ctrl Pts',(66.2888358550891,-11.57453512393,56.79020205016));
#153968=CARTESIAN_POINT('Ctrl Pts',(66.4328674667591,-11.60134676736,55.68345421607));
#153969=CARTESIAN_POINT('Ctrl Pts',(66.4721728268491,-11.68274103778,55.13592509803));
#153970=CARTESIAN_POINT('Ctrl Pts',(62.8734648869491,-13.34106036443,60.78023802665));
#153971=CARTESIAN_POINT('Ctrl Pts',(63.1818395710891,-12.9028007288,60.50999302207));
#153972=CARTESIAN_POINT('Ctrl Pts',(63.7767189561991,-12.10115904569,59.81043707638));
#153973=CARTESIAN_POINT('Ctrl Pts',(64.5297446150191,-11.23956517827,58.31393457948));
#153974=CARTESIAN_POINT('Ctrl Pts',(65.0500707627491,-10.8286161971,56.55223549403));
#153975=CARTESIAN_POINT('Ctrl Pts',(65.2009676842291,-10.88571082207,55.34626375257));
#153976=CARTESIAN_POINT('Ctrl Pts',(65.2294469649091,-10.98795046753,54.75700975733));
#153977=CARTESIAN_POINT('Ctrl Pts',(62.0002612841991,-12.99502442972,60.76331046995));
#153978=CARTESIAN_POINT('Ctrl Pts',(62.3481866604191,-12.54683897575,60.50916749016));
#153979=CARTESIAN_POINT('Ctrl Pts',(63.0239546412991,-11.7183348805,59.8230635593));
#153980=CARTESIAN_POINT('Ctrl Pts',(63.8763929217491,-10.81997022647,58.28504622256));
#153981=CARTESIAN_POINT('Ctrl Pts',(64.4466570060491,-10.39636449694,56.44318062693));
#153982=CARTESIAN_POINT('Ctrl Pts',(64.5902575303291,-10.46339979819,55.18325268157));
#153983=CARTESIAN_POINT('Ctrl Pts',(64.6068775615691,-10.57273271432,54.57189404607));
#153984=CARTESIAN_POINT('',(79.4586834778791,-10.63636348946,52.17352181749));
#153985=CARTESIAN_POINT('Ctrl Pts',(79.4586834778791,-10.63636348946,52.17352181749));
#153986=CARTESIAN_POINT('Ctrl Pts',(79.2182665366338,-10.8242034905193,
52.3493746776794));
#153987=CARTESIAN_POINT('Ctrl Pts',(78.9712303380147,-11.0019622800485,
52.5284827748445));
#153988=CARTESIAN_POINT('Ctrl Pts',(78.5918981391498,-11.2527215428637,
52.801824826324));
#153989=CARTESIAN_POINT('Ctrl Pts',(78.4000384533495,-11.3741328145895,
52.9396656717656));
#153990=CARTESIAN_POINT('Ctrl Pts',(78.1726240478271,-11.5086838386425,
53.1024812126444));
#153991=CARTESIAN_POINT('Ctrl Pts',(78.058055521351,-11.5741677613258,53.1843834338617));
#153992=CARTESIAN_POINT('Ctrl Pts',(78.0005600925498,-11.6064596423588,
53.2254574226984));
#153993=CARTESIAN_POINT('Ctrl Pts',(77.9758743927393,-11.6202023435904,
53.2430868128239));
#153994=CARTESIAN_POINT('Ctrl Pts',(77.9594073534643,-11.6293426353525,
53.2548455645689));
#153995=CARTESIAN_POINT('Ctrl Pts',(77.9496365045884,-11.6347475761949,
53.2618218595603));
#153996=CARTESIAN_POINT('Ctrl Pts',(77.835549087271,-11.6976998452158,53.3432720869405));
#153997=CARTESIAN_POINT('Ctrl Pts',(77.7080672130804,-11.7655718912864,
53.43126058736));
#153998=CARTESIAN_POINT('Ctrl Pts',(77.4852219956203,-11.8768312897897,
53.5804957074688));
#153999=CARTESIAN_POINT('Ctrl Pts',(77.4056671923129,-11.9154812671034,
53.6331166119991));
#154000=CARTESIAN_POINT('Ctrl Pts',(77.2782272168703,-11.9752576397277,
53.7163967090028));
#154001=CARTESIAN_POINT('Ctrl Pts',(77.2124802010098,-12.0055950223212,
53.7591239576359));
#154002=CARTESIAN_POINT('Ctrl Pts',(77.1321843721096,-12.0416433896302,
53.8108827161825));
#154003=CARTESIAN_POINT('Ctrl Pts',(77.091133281944,-12.0598139074465,53.8372406286189));
#154004=CARTESIAN_POINT('Ctrl Pts',(77.07334584094,-12.0676307473141,53.8486395217188));
#154005=CARTESIAN_POINT('Ctrl Pts',(77.0614443457364,-12.0728483122197,
53.8562616050807));
#154006=CARTESIAN_POINT('Ctrl Pts',(77.0538147825992,-12.0761832627605,
53.8611440448338));
#154007=CARTESIAN_POINT('Ctrl Pts',(76.9107015072919,-12.1386197783156,
53.9526821245316));
#154008=CARTESIAN_POINT('Ctrl Pts',(76.7773043815819,-12.1933590011967,
54.0360049530036));
#154009=CARTESIAN_POINT('Ctrl Pts',(76.585863466879,-12.267908338182,54.1527238662569));
#154010=CARTESIAN_POINT('Ctrl Pts',(76.4923046622753,-12.3032918237924,
54.2090173503535));
#154011=CARTESIAN_POINT('Ctrl Pts',(76.3870436154587,-12.3414994558542,
54.2710585866321));
#154012=CARTESIAN_POINT('Ctrl Pts',(76.3353979394004,-12.359863377654,54.3011684431247));
#154013=CARTESIAN_POINT('Ctrl Pts',(76.3098227963269,-12.3688638765705,
54.3159954194455));
#154014=CARTESIAN_POINT('Ctrl Pts',(76.2989152533216,-12.3726827212548,
54.322300963678));
#154015=CARTESIAN_POINT('Ctrl Pts',(76.2916554044697,-12.3752201006942,
54.3264937959008));
#154016=CARTESIAN_POINT('Ctrl Pts',(76.2893266900199,-12.3760333765106,
54.3278381426087));
#154017=CARTESIAN_POINT('Ctrl Pts',(75.9699585372172,-12.4872710399339,
54.5119303705281));
#154018=CARTESIAN_POINT('Ctrl Pts',(75.6597207636066,-12.5790030369484,
54.6767940136471));
#154019=CARTESIAN_POINT('Ctrl Pts',(75.2034047424673,-12.6936455014327,
54.8990161370789));
#154020=CARTESIAN_POINT('Ctrl Pts',(75.0527987684558,-12.7280340649545,
54.9689125940415));
#154021=CARTESIAN_POINT('Ctrl Pts',(74.8294150922816,-12.7743438611341,
55.0674421954789));
#154022=CARTESIAN_POINT('Ctrl Pts',(74.7183539461519,-12.7961804425788,
55.1151283361502));
#154023=CARTESIAN_POINT('Ctrl Pts',(74.5899403028197,-12.8194503967565,
55.16798999321));
#154024=CARTESIAN_POINT('Ctrl Pts',(74.5260291900002,-12.8305464055966,
55.1937266700248));
#154025=CARTESIAN_POINT('Ctrl Pts',(74.4987027424523,-12.8351876863875,
55.2046078106391));
#154026=CARTESIAN_POINT('Ctrl Pts',(74.4804994119687,-12.8382566553966,
55.2118288107744));
#154027=CARTESIAN_POINT('Ctrl Pts',(74.4726914094744,-12.8395648502973,
55.2149163039946));
#154028=CARTESIAN_POINT('Ctrl Pts',(73.7983918019866,-12.9515612288076,
55.4803672135456));
#154029=CARTESIAN_POINT('Ctrl Pts',(73.1425581831981,-13.0002712185578,
55.6679582563767));
#154030=CARTESIAN_POINT('Ctrl Pts',(72.1779457721873,-12.999862694313,55.8374422870987));
#154031=CARTESIAN_POINT('Ctrl Pts',(71.8467331756462,-12.9874245983009,
55.8775652700784));
#154032=CARTESIAN_POINT('Ctrl Pts',(71.3369427421527,-12.9480664787371,
55.9129204572201));
#154033=CARTESIAN_POINT('Ctrl Pts',(71.1648542801795,-12.9314972524444,
55.9205666692747));
#154034=CARTESIAN_POINT('Ctrl Pts',(70.9037101836172,-12.9011924710973,
55.9257878491668));
#154035=CARTESIAN_POINT('Ctrl Pts',(70.7723856405246,-12.88467741229,55.9268363417773));
#154036=CARTESIAN_POINT('Ctrl Pts',(70.6179100696195,-12.8629655994262,
55.9253165212991));
#154037=CARTESIAN_POINT('Ctrl Pts',(70.5403633290349,-12.8514912585476,
55.9238696208533));
#154038=CARTESIAN_POINT('Ctrl Pts',(70.5070635581712,-12.8464403744297,
55.9231021760181));
#154039=CARTESIAN_POINT('Ctrl Pts',(70.4848492499652,-12.8430434067123,
55.9225577880179));
#154040=CARTESIAN_POINT('Ctrl Pts',(70.4723440122104,-12.8411139351123,
55.9222310770215));
#154041=CARTESIAN_POINT('Ctrl Pts',(70.1512302636805,-12.7912143975556,
55.9134259636291));
#154042=CARTESIAN_POINT('Ctrl Pts',(69.8268858491848,-12.7300263417389,
55.8916180724123));
#154043=CARTESIAN_POINT('Ctrl Pts',(69.3229872617733,-12.6152727351453,
55.8386385829609));
#154044=CARTESIAN_POINT('Ctrl Pts',(69.1521305333145,-12.5731918441631,
55.8175996716809));
#154045=CARTESIAN_POINT('Ctrl Pts',(68.8918290846557,-12.503849098367,55.7809163561449));
#154046=CARTESIAN_POINT('Ctrl Pts',(68.7606749469699,-12.4676223509791,
55.76129334209));
#154047=CARTESIAN_POINT('Ctrl Pts',(68.6059830259655,-12.4225316334654,
55.7361438374548));
#154048=CARTESIAN_POINT('Ctrl Pts',(68.5282275913894,-12.3992667242409,
55.723003286718));
#154049=CARTESIAN_POINT('Ctrl Pts',(68.4892487990756,-12.3874527583474,
55.7162913336671));
#154050=CARTESIAN_POINT('Ctrl Pts',(68.4725220836888,-12.3823505609953,
55.7133843981258));
#154051=CARTESIAN_POINT('Ctrl Pts',(68.46136617385,-12.3789403947625,55.7114396862813));
#154052=CARTESIAN_POINT('Ctrl Pts',(68.454265362147,-12.3767642024997,55.7101972879607));
#154053=CARTESIAN_POINT('Ctrl Pts',(68.1902197847981,-12.2957068872524,
55.6638882242063));
#154054=CARTESIAN_POINT('Ctrl Pts',(67.898439597219,-12.1984333668864,55.6054520038334));
#154055=CARTESIAN_POINT('Ctrl Pts',(67.4173577167285,-12.017215557559,55.4977829400417));
#154056=CARTESIAN_POINT('Ctrl Pts',(67.2497818096774,-11.9509078132217,
55.4585539391153));
#154057=CARTESIAN_POINT('Ctrl Pts',(66.9883390582529,-11.8413193460853,
55.3945702757593));
#154058=CARTESIAN_POINT('Ctrl Pts',(66.8551003665473,-11.7839921569833,
55.3612929792204));
#154059=CARTESIAN_POINT('Ctrl Pts',(66.6954397661749,-11.7123873444338,
55.3201864286527));
#154060=CARTESIAN_POINT('Ctrl Pts',(66.6145814998515,-11.6753671227974,
55.2990578272136));
#154061=CARTESIAN_POINT('Ctrl Pts',(66.5695398063386,-11.6545315704221,
55.2872017499201));
#154062=CARTESIAN_POINT('Ctrl Pts',(66.5476610622123,-11.6443455785527,
55.2814164859836));
#154063=CARTESIAN_POINT('Ctrl Pts',(66.5359715222561,-11.6388869268952,
55.2783189307872));
#154064=CARTESIAN_POINT('Ctrl Pts',(66.5331097796484,-11.6375497290343,
55.2775602702098));
#154065=CARTESIAN_POINT('Ctrl Pts',(66.5251426860014,-11.6338261539074,
55.2754478327547));
#154066=CARTESIAN_POINT('Ctrl Pts',(66.4433421804196,-11.5963633136154,
55.2536349773092));
#154067=CARTESIAN_POINT('Ctrl Pts',(66.2128815524225,-11.4834360363897,
55.1907969074375));
#154068=CARTESIAN_POINT('Ctrl Pts',(66.1181588471154,-11.436223321606,55.1648209506834));
#154069=CARTESIAN_POINT('Ctrl Pts',(65.9501947904545,-11.3492951706169,
55.1181404177946));
#154070=CARTESIAN_POINT('Ctrl Pts',(65.8898979274334,-11.3176275957972,
55.10129334901));
#154071=CARTESIAN_POINT('Ctrl Pts',(65.793155058743,-11.2658118802046,55.0740631931231));
#154072=CARTESIAN_POINT('Ctrl Pts',(65.7432097182676,-11.2388248497899,
55.0599581410588));
#154073=CARTESIAN_POINT('Ctrl Pts',(65.6822274432277,-11.2053848067082,
55.0426374527362));
#154074=CARTESIAN_POINT('Ctrl Pts',(65.6510637532451,-11.188167229931,55.0337599181163));
#154075=CARTESIAN_POINT('Ctrl Pts',(65.6375643813724,-11.1806807010638,
55.029908611407));
#154076=CARTESIAN_POINT('Ctrl Pts',(65.6285329795425,-11.1756656714266,
55.0273306949228));
#154077=CARTESIAN_POINT('Ctrl Pts',(65.6222654085081,-11.1721797453671,
55.0255405354853));
#154078=CARTESIAN_POINT('Ctrl Pts',(65.2595784503797,-10.9702724799302,
54.9219108093643));
#154079=CARTESIAN_POINT('Ctrl Pts',(64.9677068724542,-10.7879579602342,
54.8363804219922));
#154080=CARTESIAN_POINT('Ctrl Pts',(64.7368422444091,-10.63636346571,54.76937978503));
#154081=CARTESIAN_POINT('Origin',(82.8560309931588,-15.5454545439394,51.5744768443685));
#154082=CARTESIAN_POINT('Ctrl Pts',(86.7935017742691,-10.81101501757,55.43269565713));
#154083=CARTESIAN_POINT('Ctrl Pts',(84.4312816407391,-8.94654054056199,
55.22108905121));
#154084=CARTESIAN_POINT('Ctrl Pts',(82.2567709278791,-8.16441345063199,
53.28170593214));
#154085=CARTESIAN_POINT('Ctrl Pts',(81.2716395534891,-8.82500194251199,
50.50774237648));
#154086=CARTESIAN_POINT('Ctrl Pts',(85.8893229942491,-11.69357781737,55.93843994818));
#154087=CARTESIAN_POINT('Ctrl Pts',(83.7324870031991,-9.76084628208499,
55.59207959555));
#154088=CARTESIAN_POINT('Ctrl Pts',(81.7057729806091,-8.92300163973699,
53.6771661408401));
#154089=CARTESIAN_POINT('Ctrl Pts',(80.6880453874592,-9.54345189092599,
51.02394478223));
#154090=CARTESIAN_POINT('Ctrl Pts',(84.8783621295491,-12.47844490921,56.4731990882401));
#154091=CARTESIAN_POINT('Ctrl Pts',(82.9237074454691,-10.52153477369,56.0062179350201));
#154092=CARTESIAN_POINT('Ctrl Pts',(81.0555047860191,-9.63580488196199,
54.1134952895101));
#154093=CARTESIAN_POINT('Ctrl Pts',(80.0340224569391,-10.18178345265,51.56516199695));
#154094=CARTESIAN_POINT('Ctrl Pts',(83.7460546069791,-13.16556661825,57.01369190147));
#154095=CARTESIAN_POINT('Ctrl Pts',(81.9857604089391,-11.20542779044,56.44355765246));
#154096=CARTESIAN_POINT('Ctrl Pts',(80.2864018783391,-10.27890102988,54.56745883809));
#154097=CARTESIAN_POINT('Ctrl Pts',(79.2976663793691,-10.74028182249,52.1025541699701));
#154098=CARTESIAN_POINT('',(81.2459147097291,-8.89165945462999,50.73940625853));
#154099=CARTESIAN_POINT('Ctrl Pts',(81.2459147097291,-8.89165945462999,
50.73940625853));
#154100=CARTESIAN_POINT('Ctrl Pts',(81.2202959565912,-8.92270890598236,
50.7617613799387));
#154101=CARTESIAN_POINT('Ctrl Pts',(81.1414335151752,-9.01946891462081,
50.8313298801056));
#154102=CARTESIAN_POINT('Ctrl Pts',(80.9346684136756,-9.25459974075488,
51.0080212942601));
#154103=CARTESIAN_POINT('Ctrl Pts',(80.8508805959602,-9.34785307260811,
51.0789961902285));
#154104=CARTESIAN_POINT('Ctrl Pts',(80.7008468650282,-9.50777103164881,
51.2039371401138));
#154105=CARTESIAN_POINT('Ctrl Pts',(80.6467707885678,-9.56440771321901,
51.2486649781948));
#154106=CARTESIAN_POINT('Ctrl Pts',(80.5592530342723,-9.65398878461894,
51.3204320423859));
#154107=CARTESIAN_POINT('Ctrl Pts',(80.5138927754486,-9.69993490407142,
51.3574844844354));
#154108=CARTESIAN_POINT('Ctrl Pts',(80.4580984353019,-9.75546994883981,
51.4027705544957));
#154109=CARTESIAN_POINT('Ctrl Pts',(80.4294734957991,-9.78370812276213,
51.4259297775437));
#154110=CARTESIAN_POINT('Ctrl Pts',(80.4170487161119,-9.79590972894298,
51.4359659465212));
#154111=CARTESIAN_POINT('Ctrl Pts',(80.408730540569,-9.80406610213962,51.4426813650083));
#154112=CARTESIAN_POINT('Ctrl Pts',(80.4031747110217,-9.80950359146663,
51.4471636877465));
#154113=CARTESIAN_POINT('Ctrl Pts',(80.0400544742734,-10.1644809698603,
51.7400019907965));
#154114=CARTESIAN_POINT('Ctrl Pts',(79.7198700088378,-10.4322956649842,
51.982474190258));
#154115=CARTESIAN_POINT('Ctrl Pts',(79.4586834778791,-10.63636348946,52.17352181749));
#154116=CARTESIAN_POINT('',(86.5280866410491,-10.82949410857,55.48972649733));
#154117=CARTESIAN_POINT('Origin',(85.5564956930185,-12.9954571590635,49.979316792856));
#154118=CARTESIAN_POINT('Ctrl Pts',(83.7957739555189,-12.9545454545505,
56.904024034869));
#154119=CARTESIAN_POINT('Ctrl Pts',(84.1486041138588,-12.7338209515203,
56.7345074233581));
#154120=CARTESIAN_POINT('Ctrl Pts',(84.4910076116214,-12.5022554926068,
56.5649123673248));
#154121=CARTESIAN_POINT('Ctrl Pts',(84.8231059758929,-12.2595992814565,
56.3960250296263));
#154122=CARTESIAN_POINT('Ctrl Pts',(85.1529044919244,-12.018623513573,56.2283072708483));
#154123=CARTESIAN_POINT('Ctrl Pts',(85.4725400985228,-11.7667100823158,
56.0612874470315));
#154124=CARTESIAN_POINT('Ctrl Pts',(85.7821579295011,-11.5036137134864,
55.895779563482));
#154125=CARTESIAN_POINT('Ctrl Pts',(86.0375866944652,-11.2865642614432,
55.7592387378025));
#154126=CARTESIAN_POINT('Ctrl Pts',(86.2861978886604,-11.0619037703368,
55.6237277063215));
#154127=CARTESIAN_POINT('Ctrl Pts',(86.5280866409232,-10.8294941088507,
55.4897264966159));
#154128=CARTESIAN_POINT('Origin',(62.4468966735091,1.4210854715202E-14,
88.14465325204));
#154129=CARTESIAN_POINT('Ctrl Pts',(86.5280866409241,-10.8294941088486,
55.4897264966211));
#154130=CARTESIAN_POINT('Ctrl Pts',(86.6918895241715,-10.6720900181015,
55.3989752596312));
#154131=CARTESIAN_POINT('Ctrl Pts',(86.8511035029772,-10.5104540155873,
55.3091182403179));
#154132=CARTESIAN_POINT('Ctrl Pts',(87.005791366162,-10.34458109779,55.2202729032426));
#154133=CARTESIAN_POINT('Ctrl Pts',(87.1610704384634,-10.1780742221685,
55.1310880038245));
#154134=CARTESIAN_POINT('Ctrl Pts',(87.3117886541035,-10.0072976322616,
55.04292228975));
#154135=CARTESIAN_POINT('Ctrl Pts',(87.4579649906633,-9.83223355314167,
54.9559191917343));
#154136=CARTESIAN_POINT('Ctrl Pts',(87.5660229298694,-9.70282092683066,
54.891603888058));
#154137=CARTESIAN_POINT('Ctrl Pts',(87.6715979854452,-9.57106506431779,
54.8279243985957));
#154138=CARTESIAN_POINT('Ctrl Pts',(87.774682602461,-9.43695606495881,54.764948471155));
#154139=CARTESIAN_POINT('Ctrl Pts',(87.9118857825905,-9.25846016781429,
54.6811290054907));
#154140=CARTESIAN_POINT('Ctrl Pts',(88.0447000283536,-9.07579752707207,
54.5985516421133));
#154141=CARTESIAN_POINT('Ctrl Pts',(88.1731648010593,-8.88894992129916,
54.5173877183289));
#154142=CARTESIAN_POINT('Ctrl Pts',(88.2232782819917,-8.81606158209185,
54.4857260677355));
#154143=CARTESIAN_POINT('Ctrl Pts',(88.2727294362972,-8.74253621078332,
54.4542797745651));
#154144=CARTESIAN_POINT('Ctrl Pts',(88.3215188668516,-8.6683720702075,54.423060113666));
#154145=CARTESIAN_POINT('Ctrl Pts',(88.4084488819124,-8.53623095308506,
54.3674348366068));
#154146=CARTESIAN_POINT('Ctrl Pts',(88.4932814398042,-8.4020630321285,54.3125284166921));
#154147=CARTESIAN_POINT('Ctrl Pts',(88.5760284980551,-8.26586071196768,
54.2584085335309));
#154148=CARTESIAN_POINT('Ctrl Pts',(88.6174020271806,-8.19775955188727,
54.2313485919503));
#154149=CARTESIAN_POINT('Ctrl Pts',(88.6582541958196,-8.12914975782779,
54.2044853684469));
#154150=CARTESIAN_POINT('Ctrl Pts',(88.6985866007877,-8.0600304155922,54.1778279138681));
#154151=CARTESIAN_POINT('Ctrl Pts',(88.7187528032718,-8.02547074447441,
54.1644991865787));
#154152=CARTESIAN_POINT('Ctrl Pts',(88.7387890658019,-7.99078368424058,
54.1512219071426));
#154153=CARTESIAN_POINT('Ctrl Pts',(88.7586955942985,-7.95596911635383,
54.1379972436758));
#154154=CARTESIAN_POINT('Ctrl Pts',(88.7732907992623,-7.93044353291926,
54.1283010942991));
#154155=CARTESIAN_POINT('Ctrl Pts',(88.7882361273448,-7.9041070941112,54.1183535710719));
#154156=CARTESIAN_POINT('Ctrl Pts',(88.8026071008764,-7.878591952754,54.1087707359372));
#154157=CARTESIAN_POINT('Ctrl Pts',(88.8078368246176,-7.86930676826568,
54.1052834578971));
#154158=CARTESIAN_POINT('Ctrl Pts',(88.8129909059121,-7.86013057299354,
54.1018442892881));
#154159=CARTESIAN_POINT('Ctrl Pts',(88.8180261878799,-7.85114276745102,
54.098482294191));
#154160=CARTESIAN_POINT('Ctrl Pts',(88.9278621585223,-7.65508932853309,
54.0251461836907));
#154161=CARTESIAN_POINT('Ctrl Pts',(89.03273547922,-7.45644993021727,53.9540375170907));
#154162=CARTESIAN_POINT('Ctrl Pts',(89.1327764104183,-7.25526270336443,
53.8852876975004));
#154163=CARTESIAN_POINT('Ctrl Pts',(89.2328176800074,-7.05407479599094,
53.8165376453622));
#154164=CARTESIAN_POINT('Ctrl Pts',(89.3280265081163,-6.8503386692998,53.7501461482649));
#154165=CARTESIAN_POINT('Ctrl Pts',(89.4184903579054,-6.64407409498235,
53.6862677950503));
#154166=CARTESIAN_POINT('Ctrl Pts',(89.5081546318131,-6.43963261551638,
53.6229540385303));
#154167=CARTESIAN_POINT('Ctrl Pts',(89.5931573688675,-6.23270680663967,
53.5621089256275));
#154168=CARTESIAN_POINT('Ctrl Pts',(89.6735424179408,-6.02330353211724,
53.5039100144859));
#154169=CARTESIAN_POINT('Ctrl Pts',(89.7531863679052,-5.81583082281737,
53.4462476603493));
#154170=CARTESIAN_POINT('Ctrl Pts',(89.8282973284865,-5.60592575728841,
53.3911826739128));
#154171=CARTESIAN_POINT('Ctrl Pts',(89.8988780945993,-5.39358828939796,
53.3389183812801));
#154172=CARTESIAN_POINT('Ctrl Pts',(89.9681322724845,-5.18524177259375,
53.2876364128577));
#154173=CARTESIAN_POINT('Ctrl Pts',(90.0330248486349,-4.97455309164704,
53.2390506443791));
#154174=CARTESIAN_POINT('Ctrl Pts',(90.0935211386558,-4.76152085442564,
53.1933861560868));
#154175=CARTESIAN_POINT('Ctrl Pts',(90.1287711912425,-4.63739096873988,
53.1667783159517));
#154176=CARTESIAN_POINT('Ctrl Pts',(90.1625279362402,-4.51246540473219,
53.1411629347915));
#154177=CARTESIAN_POINT('Ctrl Pts',(90.1947786764252,-4.3867443600625,53.116590296774));
#154178=CARTESIAN_POINT('Ctrl Pts',(81.0890185711991,-9.03398009659499,
50.59499624711));
#154179=CARTESIAN_POINT('Ctrl Pts',(82.066389392229,-8.36205842516198,53.36445303819));
#154180=CARTESIAN_POINT('Ctrl Pts',(84.2070509463491,-9.16260829370599,
55.32747811058));
#154181=CARTESIAN_POINT('Ctrl Pts',(86.5272072002091,-11.06780283748,55.58175683397));
#154182=CARTESIAN_POINT('Ctrl Pts',(82.487240909939,-7.53053025822599,50.35332743294));
#154183=CARTESIAN_POINT('Ctrl Pts',(83.5976153297791,-7.11372210236199,
52.98684050843));
#154184=CARTESIAN_POINT('Ctrl Pts',(85.9352162978791,-7.76899575474999,
54.59298316059));
#154185=CARTESIAN_POINT('Ctrl Pts',(88.5027323665692,-9.21684229213699,
54.4863678699901));
#154186=CARTESIAN_POINT('Ctrl Pts',(83.5727435711491,-5.62937756856198,
50.17140339387));
#154187=CARTESIAN_POINT('Ctrl Pts',(84.8299194058891,-5.40125583473699,
52.58820136205));
#154188=CARTESIAN_POINT('Ctrl Pts',(87.2071109645591,-5.85034243553598,
53.8781499741101));
#154189=CARTESIAN_POINT('Ctrl Pts',(89.7749977603691,-6.80110798966,53.53684402454));
#154190=CARTESIAN_POINT('Ctrl Pts',(84.1481896945291,-3.52973739894199,
50.07613844788));
#154191=CARTESIAN_POINT('Ctrl Pts',(85.4754380405791,-3.38512521217299,
52.35995335757));
#154192=CARTESIAN_POINT('Ctrl Pts',(87.8501898806692,-3.65538595374999,
53.49389491214));
#154193=CARTESIAN_POINT('Ctrl Pts',(90.3929854306691,-4.24045176432299,
53.05791123413));
#154194=CARTESIAN_POINT('',(84.1879278549181,-3.6707688494137,50.2206500166039));
#154195=CARTESIAN_POINT('Ctrl Pts',(84.1879274881912,-3.67076874249921,
50.2206500280999));
#154196=CARTESIAN_POINT('Ctrl Pts',(83.9030415620743,-4.65335590647006,
50.2708831032984));
#154197=CARTESIAN_POINT('Ctrl Pts',(83.501679882298,-5.60034065948235,50.3416539964655));
#154198=CARTESIAN_POINT('Ctrl Pts',(82.5073581548077,-7.353093032406,50.5169797445266));
#154199=CARTESIAN_POINT('Ctrl Pts',(81.9183583627455,-8.16338650643592,
50.6208362994988));
#154200=CARTESIAN_POINT('Ctrl Pts',(81.2459147097293,-8.89165945462988,
50.7394062585317));
#154201=CARTESIAN_POINT('Origin',(89.1641836723275,-5.263693750641,47.2711935873025));
#154202=CARTESIAN_POINT('Ctrl Pts',(84.0667906462691,-3.82236309078299,
50.0943346407));
#154203=CARTESIAN_POINT('Ctrl Pts',(84.6854064384891,-3.74742101924199,
51.1753351273));
#154204=CARTESIAN_POINT('Ctrl Pts',(86.5900487858291,-3.81967065678199,
52.94802757545));
#154205=CARTESIAN_POINT('Ctrl Pts',(89.1175620006691,-4.30049088340399,
53.32409278569));
#154206=CARTESIAN_POINT('Ctrl Pts',(90.2986082780691,-4.59747416179299,
53.12858445196));
#154207=CARTESIAN_POINT('Ctrl Pts',(84.4477663971991,-2.54890099283399,
50.03137520846));
#154208=CARTESIAN_POINT('Ctrl Pts',(85.0876027608091,-2.50648289723299,
51.07540225952));
#154209=CARTESIAN_POINT('Ctrl Pts',(87.0114302617491,-2.55714551410099,
52.7497662106));
#154210=CARTESIAN_POINT('Ctrl Pts',(89.5316085984691,-2.85585336077299,
53.03803083282));
#154211=CARTESIAN_POINT('Ctrl Pts',(90.7113645633691,-3.04045842633399,
52.81088733089));
#154212=CARTESIAN_POINT('Ctrl Pts',(84.6410736300791,-1.21419340158199,
49.99988982678));
#154213=CARTESIAN_POINT('Ctrl Pts',(85.2906386456891,-1.19339881491799,
51.02156561606));
#154214=CARTESIAN_POINT('Ctrl Pts',(87.2173778492491,-1.21624717379899,
52.64366771246));
#154215=CARTESIAN_POINT('Ctrl Pts',(89.7219899406691,-1.35749773631899,
52.89343266706));
#154216=CARTESIAN_POINT('Ctrl Pts',(90.8953710962691,-1.44502606200399,
52.65421569171));
#154217=CARTESIAN_POINT('Ctrl Pts',(84.6255050281691,0.153010053497514,
50.00242696498));
#154218=CARTESIAN_POINT('Ctrl Pts',(85.2742834368191,0.150394585033814,
51.02589223615));
#154219=CARTESIAN_POINT('Ctrl Pts',(87.2007679081091,0.153286082122214,
52.6521963776));
#154220=CARTESIAN_POINT('Ctrl Pts',(89.7065985576691,0.171098155476114,
52.90507996211));
#154221=CARTESIAN_POINT('Ctrl Pts',(90.8804761688691,0.182133423763114,
52.66684715676));
#154222=CARTESIAN_POINT('',(84.7089070649894,1.43647443565002E-14,50.1287872718967));
#154223=CARTESIAN_POINT('Ctrl Pts',(84.7089070652226,1.4432899320127E-14,
50.1287872722712));
#154224=CARTESIAN_POINT('Ctrl Pts',(84.7089070652227,-0.620790188952753,
50.1287872722712));
#154225=CARTESIAN_POINT('Ctrl Pts',(84.6654155304985,-1.23992630038833,
50.1364560032405));
#154226=CARTESIAN_POINT('Ctrl Pts',(84.4910143635045,-2.4687340790315,50.1672076344486));
#154227=CARTESIAN_POINT('Ctrl Pts',(84.3605401866984,-3.07529560408347,
50.1902137521402));
#154228=CARTESIAN_POINT('Ctrl Pts',(84.187928507386,-3.67076904714443,50.2206498483884));
#154229=CARTESIAN_POINT('Ctrl Pts',(84.7089070650127,1.42110872006939E-14,
50.1287872718807));
#154230=CARTESIAN_POINT('Ctrl Pts',(85.3559684191721,2.23742947452393E-14,
51.0930107907251));
#154231=CARTESIAN_POINT('Ctrl Pts',(87.2135596094279,-5.0029901016169E-14,
52.6236276843951));
#154232=CARTESIAN_POINT('Ctrl Pts',(89.6030123367996,7.09023504723426E-15,
52.8932693059995));
#154233=CARTESIAN_POINT('Ctrl Pts',(90.7329496419691,1.4210854715202E-14,
52.69425954596));
#154234=CARTESIAN_POINT('Ctrl Pts',(84.6207906093291,-0.152011227331786,
49.99508307661));
#154235=CARTESIAN_POINT('Ctrl Pts',(85.9974652801591,-0.146440090307486,
52.16989344765));
#154236=CARTESIAN_POINT('Ctrl Pts',(88.3653709583691,-0.157188198121986,
53.17894399659));
#154237=CARTESIAN_POINT('Ctrl Pts',(90.8875370260691,-0.180457446103386,
52.6654408377301));
#154238=CARTESIAN_POINT('Ctrl Pts',(84.6361601793791,1.20741070204101,49.9925779501701));
#154239=CARTESIAN_POINT('Ctrl Pts',(86.0144572373891,1.16275390045801,52.1633314201001));
#154240=CARTESIAN_POINT('Ctrl Pts',(88.3816214943691,1.24781582637001,53.16836818009));
#154241=CARTESIAN_POINT('Ctrl Pts',(90.9023154006691,1.43258709002601,52.65289559471));
#154242=CARTESIAN_POINT('Ctrl Pts',(84.4452429771191,2.54236893826101,50.02365025392));
#154243=CARTESIAN_POINT('Ctrl Pts',(85.8028873051391,2.45960847280301,52.24550138407));
#154244=CARTESIAN_POINT('Ctrl Pts',(88.1793852807691,2.64702290766801,53.30037093943));
#154245=CARTESIAN_POINT('Ctrl Pts',(90.7196837319691,3.03719723761501,52.80858638915));
#154246=CARTESIAN_POINT('Ctrl Pts',(84.0625947609391,3.82278043910101,50.08710134634));
#154247=CARTESIAN_POINT('Ctrl Pts',(85.3805449859791,3.66255118679801,52.39269601302));
#154248=CARTESIAN_POINT('Ctrl Pts',(87.7577840179691,3.95799738650802,53.55053860319));
#154249=CARTESIAN_POINT('Ctrl Pts',(90.3052323644691,4.59865127728601,53.12745538062));
#154250=CARTESIAN_POINT('',(84.1879285286622,3.67076919515978,50.2206498311393));
#154251=CARTESIAN_POINT('Ctrl Pts',(84.1879285683743,3.67076920633965,50.2206498376345));
#154252=CARTESIAN_POINT('Ctrl Pts',(84.3605360711567,3.07533070753628,50.1902144778213));
#154253=CARTESIAN_POINT('Ctrl Pts',(84.4909881059739,2.46873053153842,50.1672122643816));
#154254=CARTESIAN_POINT('Ctrl Pts',(84.6653784517624,1.23999491019598,50.136462541244));
#154255=CARTESIAN_POINT('Ctrl Pts',(84.7089070652242,0.620754149608006,
50.1287872722709));
#154256=CARTESIAN_POINT('Ctrl Pts',(84.7089070652245,1.30451205393456E-14,
50.1287872722709));
#154257=CARTESIAN_POINT('Ctrl Pts',(84.187928567227,3.67076914922564,50.2206498048453));
#154258=CARTESIAN_POINT('Ctrl Pts',(84.2524098516593,3.6645515876862,50.3260846691099));
#154259=CARTESIAN_POINT('Ctrl Pts',(84.3206795773437,3.65929251149661,50.4306354818293));
#154260=CARTESIAN_POINT('Ctrl Pts',(84.3927259892234,3.6550621788536,50.5339131962136));
#154261=CARTESIAN_POINT('Ctrl Pts',(84.464074555574,3.65087282144648,50.6361905569458));
#154262=CARTESIAN_POINT('Ctrl Pts',(84.5391271491909,3.64769249978238,50.7372188628749));
#154263=CARTESIAN_POINT('Ctrl Pts',(84.6178234087269,3.64558114180426,50.8366098849484));
#154264=CARTESIAN_POINT('Ctrl Pts',(84.695845306457,3.64348787641641,50.9351492082304));
#154265=CARTESIAN_POINT('Ctrl Pts',(84.7774487528274,3.64244544419323,51.0320786615377));
#154266=CARTESIAN_POINT('Ctrl Pts',(84.8625250016019,3.64250228307859,51.1270172861643));
#154267=CARTESIAN_POINT('Ctrl Pts',(84.9469679163454,3.64255869883762,51.2212491581695));
#154268=CARTESIAN_POINT('Ctrl Pts',(85.0348320906405,3.64369817408329,51.3135191948001));
#154269=CARTESIAN_POINT('Ctrl Pts',(85.125961546269,3.6459566841249,51.4034602027465));
#154270=CARTESIAN_POINT('Ctrl Pts',(85.2165158259445,3.64820093927323,51.492833535789));
#154271=CARTESIAN_POINT('Ctrl Pts',(85.310294175703,3.65155022151192,51.5799066160371));
#154272=CARTESIAN_POINT('Ctrl Pts',(85.4070954772706,3.65602728794667,51.6643324012192));
#154273=CARTESIAN_POINT('Ctrl Pts',(85.5033958194257,3.66048118497632,51.7483212719069));
#154274=CARTESIAN_POINT('Ctrl Pts',(85.6026876928605,3.6660512739478,51.829689668403));
#154275=CARTESIAN_POINT('Ctrl Pts',(85.7047278508454,3.67274657976675,51.9081168229286));
#154276=CARTESIAN_POINT('Ctrl Pts',(85.8062983199339,3.67941106722102,51.9861829787612));
#154277=CARTESIAN_POINT('Ctrl Pts',(85.910591529777,3.68719046054209,52.0613344418456));
#154278=CARTESIAN_POINT('Ctrl Pts',(86.0173264830788,3.69607981140521,52.1332829125085));
#154279=CARTESIAN_POINT('Ctrl Pts',(86.1237629157328,3.70494430017116,52.2050301547695));
#154280=CARTESIAN_POINT('Ctrl Pts',(86.2326270796844,3.71491254565264,52.2735918823881));
#154281=CARTESIAN_POINT('Ctrl Pts',(86.3436044015489,3.72596565800079,52.3387167704167));
#154282=CARTESIAN_POINT('Ctrl Pts',(86.4544400082225,3.73700465580824,52.4037584956353));
#154283=CARTESIAN_POINT('Ctrl Pts',(86.5673829426877,3.74912572526539,52.4653718046733));
#154284=CARTESIAN_POINT('Ctrl Pts',(86.6820900106887,3.76229627959937,52.5233465895402));
#154285=CARTESIAN_POINT('Ctrl Pts',(86.796767633063,3.77546345301504,52.5813064921169));
#154286=CARTESIAN_POINT('Ctrl Pts',(86.9132079937252,3.78967952021909,52.635629469868));
#154287=CARTESIAN_POINT('Ctrl Pts',(87.0310452881542,3.8048987359492,52.6861504842319));
#154288=CARTESIAN_POINT('Ctrl Pts',(87.1497257202048,3.82022684668929,52.7370329815041));
#154289=CARTESIAN_POINT('Ctrl Pts',(87.2698226260638,3.83657244725239,52.78405867872));
#154290=CARTESIAN_POINT('Ctrl Pts',(87.3909466918256,3.85387629261818,52.8271084253288));
#154291=CARTESIAN_POINT('Ctrl Pts',(87.5116929092281,3.87112615837604,52.8700238776003));
#154292=CARTESIAN_POINT('Ctrl Pts',(87.6334593284,3.88932819055397,52.9089881038916));
#154293=CARTESIAN_POINT('Ctrl Pts',(87.7558530000194,3.90841265468426,52.9439339994195));
#154294=CARTESIAN_POINT('Ctrl Pts',(87.878902380451,3.92759936144802,52.9790671132189));
#154295=CARTESIAN_POINT('Ctrl Pts',(88.0025851964464,3.94767786548767,53.0101387184408));
#154296=CARTESIAN_POINT('Ctrl Pts',(88.1265031900006,3.96856779516172,53.0371326720082));
#154297=CARTESIAN_POINT('Ctrl Pts',(88.2502576305924,3.98943015329604,53.0640909976498));
#154298=CARTESIAN_POINT('Ctrl Pts',(88.374246106134,4.0111016583654,53.0869825826451));
#154299=CARTESIAN_POINT('Ctrl Pts',(88.4980810843336,4.03349472027891,53.105841917296));
#154300=CARTESIAN_POINT('Ctrl Pts',(88.6231846835399,4.05611718675291,53.1248944554218));
#154301=CARTESIAN_POINT('Ctrl Pts',(88.7481309294624,4.0794758611196,53.1398318319754));
#154302=CARTESIAN_POINT('Ctrl Pts',(88.872537677615,4.1034745768986,53.1507390052145));
#154303=CARTESIAN_POINT('Ctrl Pts',(88.9982633132582,4.12772771300853,53.161761809917));
#154304=CARTESIAN_POINT('Ctrl Pts',(89.1234374712175,4.15263438431025,53.1686687657082));
#154305=CARTESIAN_POINT('Ctrl Pts',(89.2476908452341,4.17809178994324,53.1715945389227));
#154306=CARTESIAN_POINT('Ctrl Pts',(89.3727499613135,4.20371427843767,53.1745392848095));
#154307=CARTESIAN_POINT('Ctrl Pts',(89.4968759177392,4.22989451437176,53.1734514224341));
#154308=CARTESIAN_POINT('Ctrl Pts',(89.6197241169299,4.25652640758112,53.1685107305081));
#154309=CARTESIAN_POINT('Ctrl Pts',(89.7440298219647,4.28347426911763,53.1635114208131));
#154310=CARTESIAN_POINT('Ctrl Pts',(89.8670269216465,4.31088441821633,53.1545677316536));
#154311=CARTESIAN_POINT('Ctrl Pts',(89.9883967134665,4.33864794789005,53.1419033128201));
#154312=CARTESIAN_POINT('Ctrl Pts',(90.0577546357967,4.35451368108318,53.1346661101798));
#154313=CARTESIAN_POINT('Ctrl Pts',(90.1265818674342,4.3704948477379,53.1262144940036));
#154314=CARTESIAN_POINT('Ctrl Pts',(90.1948250300408,4.38657154635619,53.1165947501917));
#154315=CARTESIAN_POINT('Ctrl Pts',(84.1478916908791,3.53084617379201,50.07617289185));
#154316=CARTESIAN_POINT('Ctrl Pts',(85.4750404242492,3.38611454775601,52.35990944625));
#154317=CARTESIAN_POINT('Ctrl Pts',(87.8496043814691,3.65643304604401,53.49395859461));
#154318=CARTESIAN_POINT('Ctrl Pts',(90.3922895163691,4.24172967370401,53.05823942373));
#154319=CARTESIAN_POINT('Ctrl Pts',(83.5684103616991,5.64263664564902,50.17212144973));
#154320=CARTESIAN_POINT('Ctrl Pts',(84.8253303192091,5.41333805546702,52.58956324423));
#154321=CARTESIAN_POINT('Ctrl Pts',(87.2025717175191,5.86327918692001,53.88058185588));
#154322=CARTESIAN_POINT('Ctrl Pts',(89.7702498546691,6.81650413436202,53.5400188389));
#154323=CARTESIAN_POINT('Ctrl Pts',(82.4965671836292,7.51960021670801,50.3516900304801));
#154324=CARTESIAN_POINT('Ctrl Pts',(83.6066894758891,7.10528059197901,52.9844159722199));
#154325=CARTESIAN_POINT('Ctrl Pts',(85.9445157806491,7.76009296512003,54.5885582561201));
#154326=CARTESIAN_POINT('Ctrl Pts',(88.5134190995691,9.20496137042702,54.4800726227));
#154327=CARTESIAN_POINT('Ctrl Pts',(81.0891963680291,9.033815381809,50.59494971387));
#154328=CARTESIAN_POINT('Ctrl Pts',(82.0665861402791,8.36191540094801,53.36419282181));
#154329=CARTESIAN_POINT('Ctrl Pts',(84.2071635732892,9.16226600288201,55.32711634851));
#154330=CARTESIAN_POINT('Ctrl Pts',(86.5272818095892,11.0672006189,55.58150421395));
#154331=CARTESIAN_POINT('',(81.2459147097091,8.89165945465101,50.73940625854));
#154332=CARTESIAN_POINT('Ctrl Pts',(81.2459147097075,8.89165945465026,50.7394062585356));
#154333=CARTESIAN_POINT('Ctrl Pts',(81.9196419748508,8.16199632308235,50.6206099640519));
#154334=CARTESIAN_POINT('Ctrl Pts',(82.508629049238,7.35516112537247,50.5167556515489));
#154335=CARTESIAN_POINT('Ctrl Pts',(83.5044460856509,5.5997346190605,50.3411662401802));
#154336=CARTESIAN_POINT('Ctrl Pts',(83.902684616162,4.65479953785456,50.2709460424934));
#154337=CARTESIAN_POINT('Ctrl Pts',(84.1879284697861,3.67076917687268,50.2206498550183));
#154338=CARTESIAN_POINT('',(86.5280866410291,10.82949410859,55.48972649734));
#154339=CARTESIAN_POINT('Origin',(85.5564936082272,12.9954596346064,49.979318101201));
#154340=CARTESIAN_POINT('Ctrl Pts',(90.1948181095954,4.38657743647023,53.1165555002035));
#154341=CARTESIAN_POINT('Ctrl Pts',(90.1359031779921,4.61710858188133,53.1615437195885));
#154342=CARTESIAN_POINT('Ctrl Pts',(90.0722973819612,4.84441445094358,53.2098399585012));
#154343=CARTESIAN_POINT('Ctrl Pts',(90.0040341246653,5.06851243131367,53.261143072422));
#154344=CARTESIAN_POINT('Ctrl Pts',(89.9344459738422,5.2969598373542,53.3134419074121));
#154345=CARTESIAN_POINT('Ctrl Pts',(89.8600178886679,5.52207399296512,53.3688657860787));
#154346=CARTESIAN_POINT('Ctrl Pts',(89.7807494466665,5.74386776536395,53.4271359386309));
#154347=CARTESIAN_POINT('Ctrl Pts',(89.6995809044398,5.97097803429376,53.4868028529611));
#154348=CARTESIAN_POINT('Ctrl Pts',(89.6133372662829,6.19460721382888,53.5494544411179));
#154349=CARTESIAN_POINT('Ctrl Pts',(89.5219795893552,6.41475756038536,53.6148284024007));
#154350=CARTESIAN_POINT('Ctrl Pts',(89.4296437898062,6.63726495061136,53.680902291183));
#154351=CARTESIAN_POINT('Ctrl Pts',(89.3320838593223,6.85621896990238,53.7497575573331));
#154352=CARTESIAN_POINT('Ctrl Pts',(89.2292201379769,7.07160469119592,53.8211552001164));
#154353=CARTESIAN_POINT('Ctrl Pts',(89.1252501823817,7.28930674966545,53.8933206793805));
#154354=CARTESIAN_POINT('Ctrl Pts',(89.0158617365942,7.50336369899101,53.9680839167634));
#154355=CARTESIAN_POINT('Ctrl Pts',(88.900932501327,7.71373724533197,54.0452243608646));
#154356=CARTESIAN_POINT('Ctrl Pts',(88.867122648076,7.77562488178179,54.0679175171248));
#154357=CARTESIAN_POINT('Ctrl Pts',(88.8328330245806,7.83719358179163,54.0908165501825));
#154358=CARTESIAN_POINT('Ctrl Pts',(88.7980598701763,7.89844193170923,54.1139161922911));
#154359=CARTESIAN_POINT('Ctrl Pts',(88.6794829077388,8.10729969603818,54.1926863079607));
#154360=CARTESIAN_POINT('Ctrl Pts',(88.555284664877,8.31251142837422,54.273809043917));
#154361=CARTESIAN_POINT('Ctrl Pts',(88.4255283010071,8.51406415544969,54.3570702991699));
#154362=CARTESIAN_POINT('Ctrl Pts',(88.2912330438266,8.72266722130921,54.4432440432073));
#154363=CARTESIAN_POINT('Ctrl Pts',(88.1509845932116,8.92735105379942,54.531708338956));
#154364=CARTESIAN_POINT('Ctrl Pts',(88.004809584826,9.12811582839587,54.6222639722302));
#154365=CARTESIAN_POINT('Ctrl Pts',(87.8675534157416,9.31663097987456,54.7072943714037));
#154366=CARTESIAN_POINT('Ctrl Pts',(87.7250717523547,9.50169110207378,54.7941690553451));
#154367=CARTESIAN_POINT('Ctrl Pts',(87.5773466870284,9.68330413920943,54.8827538765666));
#154368=CARTESIAN_POINT('Ctrl Pts',(87.4318396847443,9.86219029201598,54.970008613976));
#154369=CARTESIAN_POINT('Ctrl Pts',(87.2812458092384,10.0377323720386,55.0589226290465));
#154370=CARTESIAN_POINT('Ctrl Pts',(87.1255062609115,10.2099411783719,55.1493954830942));
#154371=CARTESIAN_POINT('Ctrl Pts',(86.9737396511167,10.3777569130057,55.2375603614748));
#154372=CARTESIAN_POINT('Ctrl Pts',(86.8170867506117,10.5424075120072,55.3272057084067));
#154373=CARTESIAN_POINT('Ctrl Pts',(86.6554500841697,10.7039022560808,55.4182631789919));
#154374=CARTESIAN_POINT('Ctrl Pts',(86.6133349353838,10.7459804263656,55.4419886059397));
#154375=CARTESIAN_POINT('Ctrl Pts',(86.5708812042372,10.7878443356175,55.4658100262816));
#154376=CARTESIAN_POINT('Ctrl Pts',(86.5280866409046,10.8294941088676,55.4897264966337));
#154377=CARTESIAN_POINT('Origin',(62.4468966735091,1.4210854715202E-14,
88.14465325204));
#154378=CARTESIAN_POINT('Ctrl Pts',(86.5280866409038,10.8294941088694,55.4897264966292));
#154379=CARTESIAN_POINT('Ctrl Pts',(86.2192234645901,11.1262539163102,55.6608302285934));
#154380=CARTESIAN_POINT('Ctrl Pts',(85.8993943954668,11.4103793028112,55.834389069437));
#154381=CARTESIAN_POINT('Ctrl Pts',(85.5684108187881,11.6821583926022,56.0094180282724));
#154382=CARTESIAN_POINT('Ctrl Pts',(85.236282045607,11.9548778325644,56.1850525837767));
#154383=CARTESIAN_POINT('Ctrl Pts',(84.8929214481348,12.2151653713604,56.3621674570628));
#154384=CARTESIAN_POINT('Ctrl Pts',(84.5381644255921,12.4633103428954,56.5398130503948));
#154385=CARTESIAN_POINT('Ctrl Pts',(84.2960248581174,12.632681806349,56.6610651311145));
#154386=CARTESIAN_POINT('Ctrl Pts',(84.0485765193537,12.7963963136241,56.7825654090797));
#154387=CARTESIAN_POINT('Ctrl Pts',(83.7957739555192,12.9545454545498,56.9040240348704));
#154388=CARTESIAN_POINT('Ctrl Pts',(83.7470466955891,13.16496437151,57.01321783994));
#154389=CARTESIAN_POINT('Ctrl Pts',(81.9865745665792,11.20483377632,56.44317770796));
#154390=CARTESIAN_POINT('Ctrl Pts',(80.2870696161591,10.2783422501,54.56706441941));
#154391=CARTESIAN_POINT('Ctrl Pts',(79.2983120731091,10.73979194701,52.10208288917));
#154392=CARTESIAN_POINT('Ctrl Pts',(84.8757367991591,12.47994051502,56.47442870884));
#154393=CARTESIAN_POINT('Ctrl Pts',(82.9214873293092,10.52306401839,56.00723818309));
#154394=CARTESIAN_POINT('Ctrl Pts',(81.0536773160091,9.63724577777001,54.11455269465));
#154395=CARTESIAN_POINT('Ctrl Pts',(80.0323112249891,10.18300062511,51.56638252406));
#154396=CARTESIAN_POINT('Ctrl Pts',(85.8869149987391,11.69588976861,55.93978781814));
#154397=CARTESIAN_POINT('Ctrl Pts',(83.7306334675291,9.76298109352201,55.59306759372));
#154398=CARTESIAN_POINT('Ctrl Pts',(81.7043087692891,8.92499334384901,53.67821991044));
#154399=CARTESIAN_POINT('Ctrl Pts',(80.6864897900991,9.54533591150901,51.02532279134));
#154400=CARTESIAN_POINT('Ctrl Pts',(86.7932195329291,10.81129024407,55.4328529836));
#154401=CARTESIAN_POINT('Ctrl Pts',(84.4310620883791,8.94679575809301,55.2212052233701));
#154402=CARTESIAN_POINT('Ctrl Pts',(82.2565980756691,8.16465088581602,53.28182981116));
#154403=CARTESIAN_POINT('Ctrl Pts',(81.2714577963691,8.82522553066502,50.50790307768));
#154404=CARTESIAN_POINT('',(79.4586835372191,10.63636346571,52.1735219594));
#154405=CARTESIAN_POINT('Ctrl Pts',(79.4586835372178,10.636363465708,52.1735219594002));
#154406=CARTESIAN_POINT('Ctrl Pts',(79.6814480592509,10.4618582038496,52.0068337685839));
#154407=CARTESIAN_POINT('Ctrl Pts',(79.8981916511604,10.2786530461329,51.8412072301974));
#154408=CARTESIAN_POINT('Ctrl Pts',(80.1083296642254,10.0871970340296,51.6767454335844));
#154409=CARTESIAN_POINT('Ctrl Pts',(80.3184778117459,9.89573178845914,51.5122757053708));
#154410=CARTESIAN_POINT('Ctrl Pts',(80.5220195569677,9.69601504589331,51.3489708641279));
#154411=CARTESIAN_POINT('Ctrl Pts',(80.7184025534926,9.48853636538811,51.1869283034285));
#154412=CARTESIAN_POINT('Ctrl Pts',(80.9005351179808,9.29611326957157,51.036644278545));
#154413=CARTESIAN_POINT('Ctrl Pts',(81.0765103968599,9.09701435659084,50.8874459492423));
#154414=CARTESIAN_POINT('Ctrl Pts',(81.2459147097113,8.89165945465309,50.7394062585396));
#154415=CARTESIAN_POINT('Origin',(82.8560309932748,15.5454545438535,51.5744768443036));
#154416=CARTESIAN_POINT('Ctrl Pts',(62.0004995106591,12.99512036681,60.76331727853));
#154417=CARTESIAN_POINT('Ctrl Pts',(62.3484151888391,12.54693837639,60.50916986639));
#154418=CARTESIAN_POINT('Ctrl Pts',(63.0241629615191,11.7184431647,59.82306248213));
#154419=CARTESIAN_POINT('Ctrl Pts',(63.8765759553791,10.82009029682,58.28505757651));
#154420=CARTESIAN_POINT('Ctrl Pts',(64.4468273418191,10.39648861975,56.44321515656));
#154421=CARTESIAN_POINT('Ctrl Pts',(64.5904299294691,10.4635207436,55.18330241512));
#154422=CARTESIAN_POINT('Ctrl Pts',(64.6070531255991,10.57285133752,54.5719498575));
#154423=CARTESIAN_POINT('Ctrl Pts',(62.8738787862491,13.34120049567,60.78022792604));
#154424=CARTESIAN_POINT('Ctrl Pts',(63.1822305202591,12.90294209037,60.5099756716));
#154425=CARTESIAN_POINT('Ctrl Pts',(63.7770649543591,12.1013057401,59.81041242578));
#154426=CARTESIAN_POINT('Ctrl Pts',(64.5300373719591,11.23972064165,58.3139231133));
#154427=CARTESIAN_POINT('Ctrl Pts',(65.0503358198691,10.82877473085,56.55225383024));
#154428=CARTESIAN_POINT('Ctrl Pts',(65.2012342447591,10.8858670493,55.34630444955));
#154429=CARTESIAN_POINT('Ctrl Pts',(65.2297183008891,10.98810527869,54.75706052086));
#154430=CARTESIAN_POINT('Ctrl Pts',(64.6173646454791,13.91964486995,60.81724029466));
#154431=CARTESIAN_POINT('Ctrl Pts',(64.8539957800591,13.50761079116,60.52480603628));
#154432=CARTESIAN_POINT('Ctrl Pts',(65.3044272586691,12.7658907333,59.81500178811));
#154433=CARTESIAN_POINT('Ctrl Pts',(65.8761188231091,11.97266212857,58.40496801144));
#154434=CARTESIAN_POINT('Ctrl Pts',(66.2901879471691,11.57564099905,56.79084865574));
#154435=CARTESIAN_POINT('Ctrl Pts',(66.4342112984491,11.60238669822,55.68422263389));
#154436=CARTESIAN_POINT('Ctrl Pts',(66.4735315517891,11.68373610128,55.13673945242));
#154437=CARTESIAN_POINT('Ctrl Pts',(66.9537378663991,14.43965128121,60.80229592221));
#154438=CARTESIAN_POINT('Ctrl Pts',(67.1059017220291,14.06465275777,60.49986220292));
#154439=CARTESIAN_POINT('Ctrl Pts',(67.3904875602491,13.39597478951,59.8028885254));
#154440=CARTESIAN_POINT('Ctrl Pts',(67.7457964768791,12.67217006629,58.49957041475));
#154441=CARTESIAN_POINT('Ctrl Pts',(68.0042996574791,12.27885104909,57.04241969021));
#154442=CARTESIAN_POINT('Ctrl Pts',(68.0982333239291,12.2605680305,56.04212739625));
#154443=CARTESIAN_POINT('Ctrl Pts',(68.1256989419291,12.31045564282,55.5415397163));
#154444=CARTESIAN_POINT('Ctrl Pts',(68.8615884801891,14.73391374,60.71525424851));
#154445=CARTESIAN_POINT('Ctrl Pts',(68.9505522591391,14.38230171041,60.41285306216));
#154446=CARTESIAN_POINT('Ctrl Pts',(69.1116523776291,13.757827987,59.73423461933));
#154447=CARTESIAN_POINT('Ctrl Pts',(69.2990975194291,13.07397037489,58.5050230397));
#154448=CARTESIAN_POINT('Ctrl Pts',(69.4218122528991,12.68142066446,57.14796983335));
#154449=CARTESIAN_POINT('Ctrl Pts',(69.4544054525091,12.63506048891,56.21515507744));
#154450=CARTESIAN_POINT('Ctrl Pts',(69.4585163840591,12.66496377676,55.74504300061));
#154451=CARTESIAN_POINT('Ctrl Pts',(70.3199244149591,14.8934563637,60.60196156239));
#154452=CARTESIAN_POINT('Ctrl Pts',(70.3622226318591,14.55550964164,60.30258402178));
#154453=CARTESIAN_POINT('Ctrl Pts',(70.4323841024791,13.95625819437,59.63983876568));
#154454=CARTESIAN_POINT('Ctrl Pts',(70.4936475173591,13.29449480622,58.45887251135));
#154455=CARTESIAN_POINT('Ctrl Pts',(70.5087618416291,12.90182964092,57.16333911074));
#154456=CARTESIAN_POINT('Ctrl Pts',(70.4868595127791,12.83911853561,56.27171241897));
#154457=CARTESIAN_POINT('Ctrl Pts',(70.4680271458191,12.85728762685,55.82047504651));
#154458=CARTESIAN_POINT('Ctrl Pts',(71.7987422768891,14.99086818853,60.43452023613));
#154459=CARTESIAN_POINT('Ctrl Pts',(71.7945134349491,14.66200007839,60.1408313857));
#154460=CARTESIAN_POINT('Ctrl Pts',(71.7740644540591,14.07915129287,59.4952138796));
#154461=CARTESIAN_POINT('Ctrl Pts',(71.7076177012891,13.431302473,58.35395694307));
#154462=CARTESIAN_POINT('Ctrl Pts',(71.6100179060791,13.03810819612,57.10504669817));
#154463=CARTESIAN_POINT('Ctrl Pts',(71.5272163969991,12.96445387057,56.24374012316));
#154464=CARTESIAN_POINT('Ctrl Pts',(71.4814488769991,12.97474890777,55.80644597183));
#154465=CARTESIAN_POINT('Ctrl Pts',(73.2930854931491,15.02379049898,60.2047823183));
#154466=CARTESIAN_POINT('Ctrl Pts',(73.2424014846691,14.69834531273,59.91874182595));
#154467=CARTESIAN_POINT('Ctrl Pts',(73.1310672232491,14.1215596745,59.29009412364));
#154468=CARTESIAN_POINT('Ctrl Pts',(72.9343064335891,13.47866908886,58.17821655064));
#154469=CARTESIAN_POINT('Ctrl Pts',(72.7187593877691,13.0850525524,56.95946733291));
#154470=CARTESIAN_POINT('Ctrl Pts',(72.5697495755391,13.00718824553,56.11649390454));
#154471=CARTESIAN_POINT('Ctrl Pts',(72.4939506799091,13.01446680747,55.68758245596));
#154472=CARTESIAN_POINT('Ctrl Pts',(74.7760924715591,14.99006392631,59.90876923216));
#154473=CARTESIAN_POINT('Ctrl Pts',(74.6791154758791,14.6611250522,59.63145247883));
#154474=CARTESIAN_POINT('Ctrl Pts',(74.4765218789691,14.07814838366,59.01793837054));
#154475=CARTESIAN_POINT('Ctrl Pts',(74.1471817304391,13.43019013293,57.92289494906));
#154476=CARTESIAN_POINT('Ctrl Pts',(73.8104278418891,13.03699746573,56.71593880071));
#154477=CARTESIAN_POINT('Ctrl Pts',(73.5929209354791,12.96342646928,55.87822777989));
#154478=CARTESIAN_POINT('Ctrl Pts',(73.4860391363291,12.97378221592,55.45163611742));
#154479=CARTESIAN_POINT('Ctrl Pts',(76.7044063444491,14.85944831897,59.44380402476));
#154480=CARTESIAN_POINT('Ctrl Pts',(76.5465454282191,14.51834940535,59.18064936834));
#154481=CARTESIAN_POINT('Ctrl Pts',(76.2226196326491,13.91339295952,58.58707694282));
#154482=CARTESIAN_POINT('Ctrl Pts',(75.7151848286191,13.24677567487,57.50045084188));
#154483=CARTESIAN_POINT('Ctrl Pts',(75.2160126877391,12.85427967805,56.28626050506));
#154484=CARTESIAN_POINT('Ctrl Pts',(74.9084550047991,12.79536407084,55.43812812318));
#154485=CARTESIAN_POINT('Ctrl Pts',(74.7615129102391,12.81626401359,55.00624381423));
#154486=CARTESIAN_POINT('Ctrl Pts',(79.0212442118191,14.53891337949,58.75036910218));
#154487=CARTESIAN_POINT('Ctrl Pts',(78.7892444029591,14.17098221515,58.51098616624));
#154488=CARTESIAN_POINT('Ctrl Pts',(78.3138871646991,13.51623522621,57.94498183631));
#154489=CARTESIAN_POINT('Ctrl Pts',(77.5798288055491,12.80566305584,56.84689608258));
#154490=CARTESIAN_POINT('Ctrl Pts',(76.8765234961291,12.41304472226,55.58403161918));
#154491=CARTESIAN_POINT('Ctrl Pts',(76.4619642118191,12.38616952145,54.69194034387));
#154492=CARTESIAN_POINT('Ctrl Pts',(76.2700805142791,12.43005186544,54.23853783461));
#154493=CARTESIAN_POINT('Ctrl Pts',(81.6411285163391,13.91879763618,57.81488153531));
#154494=CARTESIAN_POINT('Ctrl Pts',(81.3186866959591,13.50671310406,57.62104900824));
#154495=CARTESIAN_POINT('Ctrl Pts',(80.6525048798091,12.76489017188,57.10813696619));
#154496=CARTESIAN_POINT('Ctrl Pts',(79.6327931869791,11.97156082259,55.97859517806));
#154497=CARTESIAN_POINT('Ctrl Pts',(78.6914485145091,11.57453512392,54.60328680704));
#154498=CARTESIAN_POINT('Ctrl Pts',(78.1775730190191,11.60134676736,53.61254574674));
#154499=CARTESIAN_POINT('Ctrl Pts',(77.9533720747691,11.68274103777,53.11147989974));
#154500=CARTESIAN_POINT('Ctrl Pts',(83.2655200870691,13.34106036443,57.18456850277));
#154501=CARTESIAN_POINT('Ctrl Pts',(82.8833134367491,12.9028007288,57.03609161983));
#154502=CARTESIAN_POINT('Ctrl Pts',(82.0850474434891,12.10115904569,56.5821847924));
#154503=CARTESIAN_POINT('Ctrl Pts',(80.8656007901591,11.23956517827,55.43348238283));
#154504=CARTESIAN_POINT('Ctrl Pts',(79.7741175750391,10.82861619709,53.95598877582));
#154505=CARTESIAN_POINT('Ctrl Pts',(79.2198542235591,10.88571082207,52.87435581621));
#154506=CARTESIAN_POINT('Ctrl Pts',(78.9915557177591,10.98795046753,52.33037867278));
#154507=CARTESIAN_POINT('Ctrl Pts',(84.0802735036491,12.99502442972,56.87000858129));
#154508=CARTESIAN_POINT('Ctrl Pts',(83.6664085766591,12.54683897575,56.7501897856));
#154509=CARTESIAN_POINT('Ctrl Pts',(82.7967330268891,11.7183348805,56.33658924635));
#154510=CARTESIAN_POINT('Ctrl Pts',(81.4696701551291,10.81997022647,55.18287676723));
#154511=CARTESIAN_POINT('Ctrl Pts',(80.3038420682091,10.39636449694,53.64713106238));
#154512=CARTESIAN_POINT('Ctrl Pts',(79.7379809787491,10.46339979819,52.5123003413));
#154513=CARTESIAN_POINT('Ctrl Pts',(79.5132662898991,10.57273271432,51.94349552833));
#154514=CARTESIAN_POINT('',(64.7368422516391,10.63636348946,54.76937963139));
#154515=CARTESIAN_POINT('Ctrl Pts',(64.7368422516391,10.63636348946,54.76937963139));
#154516=CARTESIAN_POINT('Ctrl Pts',(65.022905497685,10.8242034905186,54.8523998297597));
#154517=CARTESIAN_POINT('Ctrl Pts',(65.3163021676567,11.0019622800467,54.9362150309343));
#154518=CARTESIAN_POINT('Ctrl Pts',(65.7662463233778,11.2527215428607,55.0633332866357));
#154519=CARTESIAN_POINT('Ctrl Pts',(65.9936798000631,11.3741328145859,55.1272414347024));
#154520=CARTESIAN_POINT('Ctrl Pts',(66.2630656334176,11.5086838386383,55.2024576894393));
#154521=CARTESIAN_POINT('Ctrl Pts',(66.3987370417595,11.5741677613214,55.240235858494));
#154522=CARTESIAN_POINT('Ctrl Pts',(66.4668132034811,11.6064596423542,55.2591681879092));
#154523=CARTESIAN_POINT('Ctrl Pts',(66.4960397799691,11.6202023435858,55.2672913891309));
#154524=CARTESIAN_POINT('Ctrl Pts',(66.5155354652189,11.6293426353479,55.2727089422419));
#154525=CARTESIAN_POINT('Ctrl Pts',(66.5271030932093,11.6347475761856,55.2759226880298));
#154526=CARTESIAN_POINT('Ctrl Pts',(66.6621678159956,11.6976998452844,55.3134406708803));
#154527=CARTESIAN_POINT('Ctrl Pts',(66.8120554320327,11.765571891373,55.3525214465694));
#154528=CARTESIAN_POINT('Ctrl Pts',(67.0725028555396,11.876831289836,55.4165390344623));
#154529=CARTESIAN_POINT('Ctrl Pts',(67.1652573264087,11.9154812671251,55.4387771649057));
#154530=CARTESIAN_POINT('Ctrl Pts',(67.313495201512,11.9752576396986,55.4734478188224));
#154531=CARTESIAN_POINT('Ctrl Pts',(67.3898907667822,12.0055950222634,55.4911114952644));
#154532=CARTESIAN_POINT('Ctrl Pts',(67.483046702591,12.0416433895335,55.5122860277984));
#154533=CARTESIAN_POINT('Ctrl Pts',(67.5306370460269,12.0598139073292,55.5230140638589));
#154534=CARTESIAN_POINT('Ctrl Pts',(67.5512504241072,12.0676307471877,55.5276418564625));
#154535=CARTESIAN_POINT('Ctrl Pts',(67.5650410773529,12.0728483120871,55.5307337208534));
#154536=CARTESIAN_POINT('Ctrl Pts',(67.5738804142658,12.076183262624,55.5327122491806));
#154537=CARTESIAN_POINT('Ctrl Pts',(67.7396707699348,12.1386197781047,55.5697822842124));
#154538=CARTESIAN_POINT('Ctrl Pts',(67.893521150259,12.1933590009703,55.602455627199));
#154539=CARTESIAN_POINT('Ctrl Pts',(68.1133369846499,12.2679083379962,55.6466588796227));
#154540=CARTESIAN_POINT('Ctrl Pts',(68.2205070085393,12.303291823643,55.6675584554868));
#154541=CARTESIAN_POINT('Ctrl Pts',(68.3406393902131,12.3414994557714,55.6898567491261));
#154542=CARTESIAN_POINT('Ctrl Pts',(68.3994686284563,12.3598633776101,55.7004868975834));
#154543=CARTESIAN_POINT('Ctrl Pts',(68.4285725263113,12.3688638765474,55.7056724837353));
#154544=CARTESIAN_POINT('Ctrl Pts',(68.4409788871562,12.3726827212409,55.7078671577049));
#154545=CARTESIAN_POINT('Ctrl Pts',(68.4492349466484,12.3752201006865,55.7093241166643));
#154546=CARTESIAN_POINT('Ctrl Pts',(68.4518830161046,12.3760333765084,55.709790922099));
#154547=CARTESIAN_POINT('Ctrl Pts',(68.8149541629483,12.4872710399799,55.7735506888852));
#154548=CARTESIAN_POINT('Ctrl Pts',(69.162868996431,12.5790030370059,55.8223642699944));
#154549=CARTESIAN_POINT('Ctrl Pts',(69.6676702367486,12.6936455014814,55.8751154886068));
#154550=CARTESIAN_POINT('Ctrl Pts',(69.8330995553812,12.7280340649958,55.8892863966092));
#154551=CARTESIAN_POINT('Ctrl Pts',(70.0767106558291,12.774343861161,55.9054722190449));
#154552=CARTESIAN_POINT('Ctrl Pts',(70.1973836159313,12.7961804425978,55.9122973844165));
#154553=CARTESIAN_POINT('Ctrl Pts',(70.3361327204431,12.8194503967652,55.9180510407596));
#154554=CARTESIAN_POINT('Ctrl Pts',(70.4049919834056,12.8305464056001,55.9203767180677));
#154555=CARTESIAN_POINT('Ctrl Pts',(70.4343920137761,12.8351876863888,55.9212554500965));
#154556=CARTESIAN_POINT('Ctrl Pts',(70.4539672765963,12.8382566553964,55.9218150649338));
#154557=CARTESIAN_POINT('Ctrl Pts',(70.4623603837728,12.8395648502933,55.9220458653953));
#154558=CARTESIAN_POINT('Ctrl Pts',(71.1867843081602,12.9515612289472,55.9408640777805));
#154559=CARTESIAN_POINT('Ctrl Pts',(71.8672262336773,13.0002712185582,55.8928336884898));
#154560=CARTESIAN_POINT('Ctrl Pts',(72.8316323522009,12.9998626943128,55.7221797060804));
#154561=CARTESIAN_POINT('Ctrl Pts',(73.156593253721,12.9874245982617,55.6466015973117));
#154562=CARTESIAN_POINT('Ctrl Pts',(73.6477317483949,12.9480664786676,55.5054660086465));
#154563=CARTESIAN_POINT('Ctrl Pts',(73.8120571647138,12.9314972523697,55.4537933772774));
#154564=CARTESIAN_POINT('Ctrl Pts',(74.059238093724,12.9011924710334,55.3693831402032));
#154565=CARTESIAN_POINT('Ctrl Pts',(74.183001403273,12.8846774122361,55.3254527619492));
#154566=CARTESIAN_POINT('Ctrl Pts',(74.327641147951,12.8629655993948,55.2711908410012));
#154567=CARTESIAN_POINT('Ctrl Pts',(74.4000163786488,12.8514912585304,55.2433086520233));
#154568=CARTESIAN_POINT('Ctrl Pts',(74.4310454459668,12.8464403744192,55.2311982973818));
#154569=CARTESIAN_POINT('Ctrl Pts',(74.4517338757724,12.8430434067065,55.2230889991257));
#154570=CARTESIAN_POINT('Ctrl Pts',(74.4633732136143,12.8411139351156,55.2185049480234));
#154571=CARTESIAN_POINT('Ctrl Pts',(74.7621099082225,12.7912143974189,55.1004034772508));
#154572=CARTESIAN_POINT('Ctrl Pts',(75.0594352234263,12.7300263414723,54.9689784394765));
#154573=CARTESIAN_POINT('Ctrl Pts',(75.5148249550515,12.6152727348306,54.7468505371001));
#154574=CARTESIAN_POINT('Ctrl Pts',(75.6681820304404,12.5731918438571,54.668643984714));
#154575=CARTESIAN_POINT('Ctrl Pts',(75.9002389477876,12.5038490981298,54.5451446051645));
#154576=CARTESIAN_POINT('Ctrl Pts',(76.0167720568909,12.4676223507902,54.4818476467801));
#154577=CARTESIAN_POINT('Ctrl Pts',(76.1535332760956,12.4225316333616,54.4053070900001));
#154578=CARTESIAN_POINT('Ctrl Pts',(76.222105150992,12.3992667241873,54.366365086637));
#154579=CARTESIAN_POINT('Ctrl Pts',(76.256437611271,12.387452758321,54.3467263817898));
#154580=CARTESIAN_POINT('Ctrl Pts',(76.271161351744,12.382350560981,54.3382738823359));
#154581=CARTESIAN_POINT('Ctrl Pts',(76.2809793472499,12.3789403947562,54.3326309050957));
#154582=CARTESIAN_POINT('Ctrl Pts',(76.2872270023928,12.3767642024809,54.3290348119035));
#154583=CARTESIAN_POINT('Ctrl Pts',(76.5195100464752,12.2957068885854,54.1952096223952));
#154584=CARTESIAN_POINT('Ctrl Pts',(76.7737073693445,12.1984333691483,54.0405028368108));
#154585=CARTESIAN_POINT('Ctrl Pts',(77.1889514738957,12.0172155600492,53.7747873183489));
#154586=CARTESIAN_POINT('Ctrl Pts',(77.333004209153,11.9509078155911,53.6806097796382));
#154587=CARTESIAN_POINT('Ctrl Pts',(77.5567963331259,11.841319347885,53.5310661152164));
#154588=CARTESIAN_POINT('Ctrl Pts',(77.6706182436651,11.7839921584008,53.4542253682861));
#154589=CARTESIAN_POINT('Ctrl Pts',(77.8065908646447,11.7123873452126,53.3609907038759));
#154590=CARTESIAN_POINT('Ctrl Pts',(77.875346374262,11.6753671232057,53.3134811567604));
#154591=CARTESIAN_POINT('Ctrl Pts',(77.9136167044436,11.6545315706107,53.2869349217018));
#154592=CARTESIAN_POINT('Ctrl Pts',(77.9321973222568,11.6443455786305,53.2740155805481));
#154593=CARTESIAN_POINT('Ctrl Pts',(77.9421224705332,11.6388869269128,53.2671067725909));
#154594=CARTESIAN_POINT('Ctrl Pts',(77.944552151737,11.6375497290564,53.2654150912361));
#154595=CARTESIAN_POINT('Ctrl Pts',(77.9513162792979,11.633826151391,53.2607051396328));
#154596=CARTESIAN_POINT('Ctrl Pts',(78.0207231770864,11.5963633097845,53.2122303381047));
#154597=CARTESIAN_POINT('Ctrl Pts',(78.2157934428615,11.4834360324175,53.0743596905367));
#154598=CARTESIAN_POINT('Ctrl Pts',(78.2959193690099,11.4362233179004,53.0175532028137));
#154599=CARTESIAN_POINT('Ctrl Pts',(78.4377882693462,11.3492951678592,52.9162407609837));
#154600=CARTESIAN_POINT('Ctrl Pts',(78.4886867489951,11.3176275934474,52.8797869535281));
#154601=CARTESIAN_POINT('Ctrl Pts',(78.5702820457391,11.2658118786183,52.8211109680525));
#154602=CARTESIAN_POINT('Ctrl Pts',(78.6123911010194,11.2388248486234,52.7907742426851));
#154603=CARTESIAN_POINT('Ctrl Pts',(78.6637716696953,11.2053848061015,52.7536409538566));
#154604=CARTESIAN_POINT('Ctrl Pts',(78.6900196630872,11.1881672296221,52.7346401906974));
#154605=CARTESIAN_POINT('Ctrl Pts',(78.7013876985477,11.1806807008864,52.7264040892436));
#154606=CARTESIAN_POINT('Ctrl Pts',(78.7089927407024,11.1756656713378,52.7208927188949));
#154607=CARTESIAN_POINT('Ctrl Pts',(78.7142700602418,11.1721797453604,52.7170668838275));
#154608=CARTESIAN_POINT('Ctrl Pts',(79.0196408631394,10.9702724809317,52.4956405505701));
#154609=CARTESIAN_POINT('Ctrl Pts',(79.264657315864,10.7879579613599,52.3154423177719));
#154610=CARTESIAN_POINT('Ctrl Pts',(79.4586835372191,10.63636346571,52.1735219594));
#154611=CARTESIAN_POINT('Origin',(61.3394944137234,15.5454545439464,55.3684227747178));
#154612=CARTESIAN_POINT('Ctrl Pts',(58.9590707274591,10.81101501758,60.34065684336));
#154613=CARTESIAN_POINT('Ctrl Pts',(61.1064578339192,8.94654054057203,59.33388480863));
#154614=CARTESIAN_POINT('Ctrl Pts',(62.4865214122591,8.16441345063902,56.76773433708));
#154615=CARTESIAN_POINT('Ctrl Pts',(62.4634906824092,8.82500194251101,53.82412647963));
#154616=CARTESIAN_POINT('Ctrl Pts',(59.9816955898691,11.69357781733,60.50665366569));
#154617=CARTESIAN_POINT('Ctrl Pts',(61.8899962375191,9.76084628201802,59.44350004341));
#154618=CARTESIAN_POINT('Ctrl Pts',(63.1395454747391,8.92300163969001,56.9508929801001));
#154619=CARTESIAN_POINT('Ctrl Pts',(63.1884414345591,9.54345189093102,54.10959711083));
#154620=CARTESIAN_POINT('Ctrl Pts',(61.1145864519892,12.47844490925,60.66339390371));
#154621=CARTESIAN_POINT('Ctrl Pts',(62.7916440738191,10.52153477373,59.55604388476));
#154622=CARTESIAN_POINT('Ctrl Pts',(63.8998310565591,9.63580488197901,57.13850344022));
#154623=CARTESIAN_POINT('Ctrl Pts',(63.9881291455391,10.18178345265,54.39448591732));
#154624=CARTESIAN_POINT('Ctrl Pts',(62.3634669048891,13.16556661825,60.78401903071));
#154625=CARTESIAN_POINT('Ctrl Pts',(63.8226049756391,11.20542779043,59.64621201015));
#154626=CARTESIAN_POINT('Ctrl Pts',(64.7778160615291,10.27890102988,57.30204095023));
#154627=CARTESIAN_POINT('Ctrl Pts',(64.8638764659491,10.74028182249,54.64762076559));
#154628=CARTESIAN_POINT('',(62.5668978423991,8.89165945463101,54.03302090535));
#154629=CARTESIAN_POINT('Ctrl Pts',(62.5668978423991,8.89165945463101,54.03302090535));
#154630=CARTESIAN_POINT('Ctrl Pts',(62.5986175218308,8.92270892978409,54.0452657277444));
#154631=CARTESIAN_POINT('Ctrl Pts',(62.6965178171167,9.01946894987616,54.0836661950859));
#154632=CARTESIAN_POINT('Ctrl Pts',(62.9512454808967,9.25459977512765,54.1789839833193));
#154633=CARTESIAN_POINT('Ctrl Pts',(63.054255116238,9.34785310371798,54.2170214466761));
#154634=CARTESIAN_POINT('Ctrl Pts',(63.2379730184545,9.50777105388192,54.2831129736518));
#154635=CARTESIAN_POINT('Ctrl Pts',(63.3040857261481,9.56440773183257,54.3066482841705));
#154636=CARTESIAN_POINT('Ctrl Pts',(63.4108712884247,9.65398879690074,54.3441544273615));
#154637=CARTESIAN_POINT('Ctrl Pts',(63.4661686665216,9.69993491296207,54.3634582101237));
#154638=CARTESIAN_POINT('Ctrl Pts',(63.5340869392131,9.75546995340281,54.3869304059749));
#154639=CARTESIAN_POINT('Ctrl Pts',(63.5689065016673,9.78370812507163,54.3989026501242));
#154640=CARTESIAN_POINT('Ctrl Pts',(63.5840145461932,9.79590973026782,54.4040840387116));
#154641=CARTESIAN_POINT('Ctrl Pts',(63.5941278819465,9.80406610280387,54.4075494840412));
#154642=CARTESIAN_POINT('Ctrl Pts',(63.6008816978809,9.80950359151928,54.4098612837665));
#154643=CARTESIAN_POINT('Ctrl Pts',(64.0422596943631,10.1644809627909,54.5608448379334));
#154644=CARTESIAN_POINT('Ctrl Pts',(64.4260650495644,10.4322956587886,54.6791846378752));
#154645=CARTESIAN_POINT('Ctrl Pts',(64.7368422516391,10.63636348946,54.76937963139));
#154646=CARTESIAN_POINT('Ctrl Pts',(59.2279850656438,10.8294941093792,60.3034709806296));
#154647=CARTESIAN_POINT('Ctrl Pts',(59.3134256343538,10.7545915723124,60.258963004405));
#154648=CARTESIAN_POINT('Ctrl Pts',(59.3991652882675,10.680240728207,60.2105626520754));
#154649=CARTESIAN_POINT('Ctrl Pts',(59.4849397019862,10.6067220037401,60.1581869063918));
#154650=CARTESIAN_POINT('Ctrl Pts',(59.5713228657953,10.5326815091063,60.1054394444988));
#154651=CARTESIAN_POINT('Ctrl Pts',(59.6577410378865,10.4594853307763,60.0486595080926));
#154652=CARTESIAN_POINT('Ctrl Pts',(59.7439023723681,10.3874309241517,59.9878108477117));
#154653=CARTESIAN_POINT('Ctrl Pts',(59.8274742292158,10.3175420280255,59.9287909222971));
#154654=CARTESIAN_POINT('Ctrl Pts',(59.9108040573564,10.2487277080708,59.8659431171087));
#154655=CARTESIAN_POINT('Ctrl Pts',(59.993610017306,10.1812641227691,59.7992830131684));
#154656=CARTESIAN_POINT('Ctrl Pts',(60.0758344999377,10.1142742780612,59.7330910076413));
#154657=CARTESIAN_POINT('Ctrl Pts',(60.1575420809736,10.048616654725,59.6631399245928));
#154658=CARTESIAN_POINT('Ctrl Pts',(60.2384468059363,9.98456054389281,59.5894953010128));
#154659=CARTESIAN_POINT('Ctrl Pts',(60.3186969195305,9.92102271995163,59.5164465463125));
#154660=CARTESIAN_POINT('Ctrl Pts',(60.3981567261616,9.85906098815908,59.4397637592995));
#154661=CARTESIAN_POINT('Ctrl Pts',(60.4765429014928,9.79893126053567,59.3595616608662));
#154662=CARTESIAN_POINT('Ctrl Pts',(60.4856978007711,9.79190857320978,59.3501946758084));
#154663=CARTESIAN_POINT('Ctrl Pts',(60.4948380543894,9.78491086352201,59.3407797431561));
#154664=CARTESIAN_POINT('Ctrl Pts',(60.5039632110606,9.77793852912787,59.3313170911929));
#154665=CARTESIAN_POINT('Ctrl Pts',(60.580499202148,9.71945903751137,59.2519504049623));
#154666=CARTESIAN_POINT('Ctrl Pts',(60.6560082058958,9.66273886911162,59.1691860498569));
#154667=CARTESIAN_POINT('Ctrl Pts',(60.7302169784138,9.60801399981514,59.0831828485741));
#154668=CARTESIAN_POINT('Ctrl Pts',(60.8040691333626,9.55355211627086,58.9975929441502));
#154669=CARTESIAN_POINT('Ctrl Pts',(60.876633123015,9.50106676290267,58.9087954073986));
#154670=CARTESIAN_POINT('Ctrl Pts',(60.9476470270386,9.45077273985678,58.816994662647));
#154671=CARTESIAN_POINT('Ctrl Pts',(61.0183254973686,9.40071628028738,58.7256275380902));
#154672=CARTESIAN_POINT('Ctrl Pts',(61.087468108101,9.35283082106235,58.6312857698978));
#154673=CARTESIAN_POINT('Ctrl Pts',(61.1548298447628,9.30730534780568,58.534215305236));
#154674=CARTESIAN_POINT('Ctrl Pts',(61.2220446102576,9.26187920292532,58.4373566308303));
#154675=CARTESIAN_POINT('Ctrl Pts',(61.2874859051142,9.21880303954255,58.3377814899491));
#154676=CARTESIAN_POINT('Ctrl Pts',(61.3509290700527,9.17823732169581,58.2357741030116));
#154677=CARTESIAN_POINT('Ctrl Pts',(61.4142893140245,9.13772462372195,58.133900040935));
#154678=CARTESIAN_POINT('Ctrl Pts',(61.4756563286036,9.09971603908283,58.0296005002065));
#154679=CARTESIAN_POINT('Ctrl Pts',(61.5348301573818,9.06434033599487,57.9231927895167));
#154680=CARTESIAN_POINT('Ctrl Pts',(61.557278527314,9.05092009792798,57.8828256254759));
#154681=CARTESIAN_POINT('Ctrl Pts',(61.5794115312215,9.03787843829657,57.8421553797251));
#154682=CARTESIAN_POINT('Ctrl Pts',(61.6012192890004,9.025221122758,57.8012004642127));
#154683=CARTESIAN_POINT('Ctrl Pts',(61.658703143616,8.99185724859815,57.6932459265211));
#154684=CARTESIAN_POINT('Ctrl Pts',(61.7139641673336,8.96114362320618,57.5832381541095));
#154685=CARTESIAN_POINT('Ctrl Pts',(61.7668325938444,8.93317273510113,57.4715236451438));
#154686=CARTESIAN_POINT('Ctrl Pts',(61.8197461278394,8.90517798215884,57.3597138210575));
#154687=CARTESIAN_POINT('Ctrl Pts',(61.8702627698071,8.87993074294189,57.2461948693806));
#154688=CARTESIAN_POINT('Ctrl Pts',(61.9182443233936,8.85748767537645,57.1313341626496));
#154689=CARTESIAN_POINT('Ctrl Pts',(61.9664028183663,8.83496184459917,57.0160498845428));
#154690=CARTESIAN_POINT('Ctrl Pts',(62.012007338638,8.815260938074,56.8994144889776));
#154691=CARTESIAN_POINT('Ctrl Pts',(62.054953159131,8.79840493994763,56.7818114600221));
#154692=CARTESIAN_POINT('Ctrl Pts',(62.0980138971958,8.78150383730693,56.6638937402684));
#154693=CARTESIAN_POINT('Ctrl Pts',(62.1384016172103,8.7674628347838,56.5450037683519));
#154694=CARTESIAN_POINT('Ctrl Pts',(62.1760475714549,8.75626481291633,56.4255317414049));
#154695=CARTESIAN_POINT('Ctrl Pts',(62.2139110231855,8.7450020950768,56.3053694712159));
#154696=CARTESIAN_POINT('Ctrl Pts',(62.2490009275031,8.73661518966188,56.1846189627729));
#154697=CARTESIAN_POINT('Ctrl Pts',(62.281285169705,8.73105026857484,56.063672343902));
#154698=CARTESIAN_POINT('Ctrl Pts',(62.2933952537888,8.72896282102498,56.0183042750153));
#154699=CARTESIAN_POINT('Ctrl Pts',(62.3051109433974,8.72727208828487,55.9729085200835));
#154700=CARTESIAN_POINT('Ctrl Pts',(62.3164318955331,8.72597398141135,55.9275053573406));
#154701=CARTESIAN_POINT('Ctrl Pts',(62.3472724494424,8.7224376768203,55.8038179968227));
#154702=CARTESIAN_POINT('Ctrl Pts',(62.3751954603565,8.72181580791975,55.6800186717206));
#154703=CARTESIAN_POINT('Ctrl Pts',(62.4002141666283,8.7240106844509,55.5564958095557));
#154704=CARTESIAN_POINT('Ctrl Pts',(62.4266203901146,8.72632728705925,55.4261224693609));
#154705=CARTESIAN_POINT('Ctrl Pts',(62.4497910931516,8.73178169992798,55.296057876902));
#154706=CARTESIAN_POINT('Ctrl Pts',(62.4697845242374,8.74022267695791,55.1667317285681));
#154707=CARTESIAN_POINT('Ctrl Pts',(62.4890937538867,8.74837479268213,55.041831290663));
#154708=CARTESIAN_POINT('Ctrl Pts',(62.5054399441388,8.75931202454087,54.9176198452025));
#154709=CARTESIAN_POINT('Ctrl Pts',(62.5189106525707,8.77287020927075,54.7944531757696));
#154710=CARTESIAN_POINT('Ctrl Pts',(62.5330973407356,8.78714902317408,54.6647400919784));
#154711=CARTESIAN_POINT('Ctrl Pts',(62.5440948296285,8.80433457894131,54.5361864972875));
#154712=CARTESIAN_POINT('Ctrl Pts',(62.5520413132412,8.82420895134365,54.4091649177086));
#154713=CARTESIAN_POINT('Ctrl Pts',(62.5599877968539,8.84408332374599,54.2821433381296));
#154714=CARTESIAN_POINT('Ctrl Pts',(62.5648837133173,8.86664602936165,54.156653998794));
#154715=CARTESIAN_POINT('Ctrl Pts',(62.5668978424016,8.89165945462865,54.0330209053496));
#154716=CARTESIAN_POINT('Ctrl Pts',(62.6875707163291,9.05486984706101,53.85409719576));
#154717=CARTESIAN_POINT('Ctrl Pts',(62.6936927437891,8.90708944577401,54.49996789171));
#154718=CARTESIAN_POINT('Ctrl Pts',(62.5519594607091,8.75508983733901,55.85643113434));
#154719=CARTESIAN_POINT('Ctrl Pts',(61.8187473138591,9.06713176397001,57.86053638825));
#154720=CARTESIAN_POINT('Ctrl Pts',(60.6706513748291,9.88591711331501,59.49166260962));
#154721=CARTESIAN_POINT('Ctrl Pts',(59.7641049370091,10.66790050512,60.16132571301));
#154722=CARTESIAN_POINT('Ctrl Pts',(59.3056604462691,11.08744520415,60.39001266332));
#154723=CARTESIAN_POINT('Ctrl Pts',(62.1213330553091,8.44949510325101,53.95571996686));
#154724=CARTESIAN_POINT('Ctrl Pts',(62.1108200502591,8.32237104745601,54.59787120527));
#154725=CARTESIAN_POINT('Ctrl Pts',(61.9267980790491,8.19927673930601,55.93250107089));
#154726=CARTESIAN_POINT('Ctrl Pts',(61.1093761573991,8.49914365747801,57.86858052973));
#154727=CARTESIAN_POINT('Ctrl Pts',(59.8669990431491,9.25045145190902,59.41928559907));
#154728=CARTESIAN_POINT('Ctrl Pts',(58.8963896387191,9.96331635072501,60.04138849839));
#154729=CARTESIAN_POINT('Ctrl Pts',(58.4060688283291,10.34643938379,60.24891883476));
#154730=CARTESIAN_POINT('Ctrl Pts',(61.3620176577091,7.46083974632801,54.09323968618));
#154731=CARTESIAN_POINT('Ctrl Pts',(61.3251626795591,7.36129509255801,54.72601497373));
#154732=CARTESIAN_POINT('Ctrl Pts',(61.0803190466291,7.27338783305801,56.02131835236));
#154733=CARTESIAN_POINT('Ctrl Pts',(60.1582507453391,7.54259435678201,57.85121399405));
#154734=CARTESIAN_POINT('Ctrl Pts',(58.8087038077091,8.18268645878101,59.28224135853));
#154735=CARTESIAN_POINT('Ctrl Pts',(57.7674952770791,8.78618585702401,59.83536073368));
#154736=CARTESIAN_POINT('Ctrl Pts',(57.2415921764891,9.11164773419301,60.0124212846));
#154737=CARTESIAN_POINT('Ctrl Pts',(60.5437715759391,6.00793348176301,54.24295470498));
#154738=CARTESIAN_POINT('Ctrl Pts',(60.4753647636491,5.93916618444801,54.85989885246));
#154739=CARTESIAN_POINT('Ctrl Pts',(60.1636338904891,5.88576846827101,56.10101490775));
#154740=CARTESIAN_POINT('Ctrl Pts',(59.1425671318791,6.10203393089201,57.80204415533));
#154741=CARTESIAN_POINT('Ctrl Pts',(57.7021490370491,6.59039605304901,59.0946682543));
#154742=CARTESIAN_POINT('Ctrl Pts',(56.6033067699491,7.04779466755601,59.57002403801));
#154743=CARTESIAN_POINT('Ctrl Pts',(56.0476476565391,7.29537012181901,59.71293770471));
#154744=CARTESIAN_POINT('Ctrl Pts',(60.0471342481991,4.90275765822201,54.33449450703));
#154745=CARTESIAN_POINT('Ctrl Pts',(59.9584867813191,4.85293774611401,54.9392420524));
#154746=CARTESIAN_POINT('Ctrl Pts',(59.6062054947891,4.81843036106501,56.14248407187));
#154747=CARTESIAN_POINT('Ctrl Pts',(58.5319771100791,4.99247752985201,57.76014880143));
#154748=CARTESIAN_POINT('Ctrl Pts',(57.0481181060591,5.37294144456601,58.96651117554));
#154749=CARTESIAN_POINT('Ctrl Pts',(55.9232080096891,5.72782341665301,59.39476748319));
#154750=CARTESIAN_POINT('Ctrl Pts',(55.3537576252991,5.92042931459201,59.51724032973));
#154751=CARTESIAN_POINT('Ctrl Pts',(59.6514918396991,3.73992698433501,54.40789230405));
#154752=CARTESIAN_POINT('Ctrl Pts',(59.5463847958691,3.70514679147901,55.00100479065));
#154753=CARTESIAN_POINT('Ctrl Pts',(59.1627398857991,3.68320799693501,56.17068044341));
#154754=CARTESIAN_POINT('Ctrl Pts',(58.0522452014191,3.81340119389101,57.71933487698));
#154755=CARTESIAN_POINT('Ctrl Pts',(56.5429763649491,4.09236446003801,58.85701018477));
#154756=CARTESIAN_POINT('Ctrl Pts',(55.4041011816691,4.35221319071501,59.24912253076));
#154757=CARTESIAN_POINT('Ctrl Pts',(54.8269328357791,4.49364817466901,59.35619700334));
#154758=CARTESIAN_POINT('Ctrl Pts',(59.2623296266291,2.11847170632401,54.48042667407));
#154759=CARTESIAN_POINT('Ctrl Pts',(59.1408541116391,2.10082097206001,55.06070972073));
#154760=CARTESIAN_POINT('Ctrl Pts',(58.7271787855591,2.09107712759001,56.19493379311));
#154761=CARTESIAN_POINT('Ctrl Pts',(57.5854988517191,2.16271678317001,57.67379941492));
#154762=CARTESIAN_POINT('Ctrl Pts',(56.0578341057191,2.31287231939801,58.74373047707));
#154763=CARTESIAN_POINT('Ctrl Pts',(54.9100779263991,2.45260917966401,59.10101280316));
#154764=CARTESIAN_POINT('Ctrl Pts',(54.3276575839291,2.52896184850001,59.19342098219));
#154765=CARTESIAN_POINT('Ctrl Pts',(59.0540952976791,0.0127975999524342,
54.5196572809));
#154766=CARTESIAN_POINT('Ctrl Pts',(58.9232560182391,0.0126887045292242,
55.09143455285));
#154767=CARTESIAN_POINT('Ctrl Pts',(58.4938016584491,0.0126145908767642,
56.2037448358));
#154768=CARTESIAN_POINT('Ctrl Pts',(57.3403850018491,0.0129921919657642,
57.64274508359));
#154769=CARTESIAN_POINT('Ctrl Pts',(55.8112488908891,0.0138214067188142,
58.6760997592));
#154770=CARTESIAN_POINT('Ctrl Pts',(54.6655311374391,0.0146072936320442,
59.01584458769));
#154771=CARTESIAN_POINT('Ctrl Pts',(54.0837499761391,0.0150396948250942,
59.10118989083));
#154772=CARTESIAN_POINT('Ctrl Pts',(59.2989189396391,-2.51693002856899,
54.47354239089));
#154773=CARTESIAN_POINT('Ctrl Pts',(59.1790755060991,-2.49593417718599,
55.05528462409));
#154774=CARTESIAN_POINT('Ctrl Pts',(58.7681731074591,-2.48428118923299,
56.19329870897));
#154775=CARTESIAN_POINT('Ctrl Pts',(57.6286544560291,-2.56920952549099,
57.67914147466));
#154776=CARTESIAN_POINT('Ctrl Pts',(56.1014244201991,-2.74738422816499,
58.75555153277));
#154777=CARTESIAN_POINT('Ctrl Pts',(54.9534490419391,-2.91325666836699,
59.11599776679));
#154778=CARTESIAN_POINT('Ctrl Pts',(54.3709846642191,-3.00390208172399,
59.20969563797));
#154779=CARTESIAN_POINT('Ctrl Pts',(59.9917126604991,-4.91906267884899,
54.34448351142));
#154780=CARTESIAN_POINT('Ctrl Pts',(59.9009297075891,-4.87125340189799,
54.94879468213));
#154781=CARTESIAN_POINT('Ctrl Pts',(59.5435979960591,-4.83987319128399,
56.14942539199));
#154782=CARTESIAN_POINT('Ctrl Pts',(58.4604560798591,-5.01415296934599,
57.75897301872));
#154783=CARTESIAN_POINT('Ctrl Pts',(56.9673297784391,-5.39038447606399,
58.95563343562));
#154784=CARTESIAN_POINT('Ctrl Pts',(55.8362600566191,-5.74067651648499,
59.37795261339));
#154785=CARTESIAN_POINT('Ctrl Pts',(55.2637085671291,-5.93095636015299,
59.49771519496));
#154786=CARTESIAN_POINT('Ctrl Pts',(61.1125443538391,-7.13614956716599,
54.13839204096));
#154787=CARTESIAN_POINT('Ctrl Pts',(61.0671680892591,-7.04576412768599,
54.76818692763));
#154788=CARTESIAN_POINT('Ctrl Pts',(60.8025094853891,-6.96962720623199,
56.0507627613));
#154789=CARTESIAN_POINT('Ctrl Pts',(59.8459446485991,-7.22911178542799,
57.84598152538));
#154790=CARTESIAN_POINT('Ctrl Pts',(58.4607058835591,-7.83300648254199,
59.2377399736));
#154791=CARTESIAN_POINT('Ctrl Pts',(57.3957858977891,-8.40075126025699,
59.76809594155));
#154792=CARTESIAN_POINT('Ctrl Pts',(56.8579036864491,-8.70733922026899,
59.93506871694));
#154793=CARTESIAN_POINT('Ctrl Pts',(62.1145143757991,-8.44196653416099,
53.95694727695));
#154794=CARTESIAN_POINT('Ctrl Pts',(62.1038084651091,-8.31509888071599,
54.59903739218));
#154795=CARTESIAN_POINT('Ctrl Pts',(61.9193139144091,-8.19237189993399,
55.93337680427));
#154796=CARTESIAN_POINT('Ctrl Pts',(61.1010004648091,-8.49213444877799,
57.86861879038));
#154797=CARTESIAN_POINT('Ctrl Pts',(59.8576583382091,-9.24267821450499,
59.41836213069));
#154798=CARTESIAN_POINT('Ctrl Pts',(58.8864033693091,-9.95473954319099,
60.03991099606));
#154799=CARTESIAN_POINT('Ctrl Pts',(58.3957609560291,-10.33743603438,60.24719828988));
#154800=CARTESIAN_POINT('Ctrl Pts',(62.6879642021691,-9.05532397487499,
53.8540261509));
#154801=CARTESIAN_POINT('Ctrl Pts',(62.6940943763991,-8.90752652229099,
54.49990186792));
#154802=CARTESIAN_POINT('Ctrl Pts',(62.5523798635391,-8.75549999478799,
55.85638386176));
#154803=CARTESIAN_POINT('Ctrl Pts',(61.8191993941091,-9.06753559913399,
57.86053706941));
#154804=CARTESIAN_POINT('Ctrl Pts',(60.6711354527091,-9.88635090107299,
59.49171575596));
#154805=CARTESIAN_POINT('Ctrl Pts',(59.7646103295491,-10.6683719995,60.16140778771));
#154806=CARTESIAN_POINT('Ctrl Pts',(59.3061767685891,-11.08793749998,60.39010712379));
#154807=CARTESIAN_POINT('Ctrl Pts',(62.5668978424019,8.89165945462829,54.0330209053495));
#154808=CARTESIAN_POINT('Ctrl Pts',(61.5307357207086,7.76947049531924,54.2157242437921));
#154809=CARTESIAN_POINT('Ctrl Pts',(60.6061882911196,6.35847891159746,54.3787469007418));
#154810=CARTESIAN_POINT('Ctrl Pts',(59.406833177869,3.23205943624151,54.5902255666585));
#154811=CARTESIAN_POINT('Ctrl Pts',(59.1039820610764,1.60347731142046,54.6436263895163));
#154812=CARTESIAN_POINT('Ctrl Pts',(59.1038271015103,-1.60757587207886,
54.6436537130687));
#154813=CARTESIAN_POINT('Ctrl Pts',(59.4077654184968,-3.23446213873761,
54.5900611874711));
#154814=CARTESIAN_POINT('Ctrl Pts',(60.6369613386987,-6.4381888767319,54.3733207821628));
#154815=CARTESIAN_POINT('Ctrl Pts',(61.58246960519,-7.82549951850307,54.2066021641412));
#154816=CARTESIAN_POINT('Ctrl Pts',(62.5668976767239,-8.89165927519747,
54.033020934563));
#154817=CARTESIAN_POINT('Origin',(71.9064062760691,1.4210854715202E-14,
52.38621358194));
#154818=CARTESIAN_POINT('Origin',(71.9064062760691,1.4210854715202E-14,
52.38621358194));
#154819=CARTESIAN_POINT('Origin',(71.9064062760691,1.4210854715202E-14,
52.38621358194));
#154820=CARTESIAN_POINT('Origin',(71.9064062760691,1.4210854715202E-14,
52.38621358194));
#154821=CARTESIAN_POINT('Origin',(71.9064062760691,1.4210854715202E-14,
52.38621358194));
#154822=CARTESIAN_POINT('Origin',(72.0800544537291,1.4210854715202E-14,
53.37102133495));
#154823=CARTESIAN_POINT('Origin',(72.4273508090691,1.4210854715202E-14,
55.34063684098));
#154824=CARTESIAN_POINT('Origin',(72.4273508090703,1.25011112572802E-13,
55.3406368409798));
#154825=CARTESIAN_POINT('Origin',(72.4794268116891,1.25011112572802E-13,
55.63597452787));
#154826=CARTESIAN_POINT('Origin',(82.1588614745091,11.44983787884,58.70184200704));
#154827=CARTESIAN_POINT('',(81.8983972201781,-8.53716763907585,57.2246289649024));
#154828=CARTESIAN_POINT('',(81.8983892080091,-3.04138126515099,57.22463037752));
#154829=CARTESIAN_POINT('Origin',(82.1588614745091,-8.53720311761699,58.70184200704));
#154830=CARTESIAN_POINT('',(81.8983915604129,8.53714783790647,57.2246299627624));
#154831=CARTESIAN_POINT('Origin',(82.1588614745091,8.53714874844301,58.70184200704));
#154832=CARTESIAN_POINT('',(81.8983892078791,8.53712721536902,57.22463037754));
#154833=CARTESIAN_POINT('Origin',(83.3756008375291,111.0724296188,56.96415811102));
#154834=CARTESIAN_POINT('',(81.3676282287758,8.73788135389827,57.3182179348277));
#154835=CARTESIAN_POINT('Ctrl Pts',(81.8983892080091,8.53714874844301,57.22463037752));
#154836=CARTESIAN_POINT('Ctrl Pts',(81.8095766714547,8.57150267943434,57.2402904239405));
#154837=CARTESIAN_POINT('Ctrl Pts',(81.6321992954396,8.63903130243991,57.2715668124596));
#154838=CARTESIAN_POINT('Ctrl Pts',(81.4557926517591,8.70548579598501,57.30267214923));
#154839=CARTESIAN_POINT('Ctrl Pts',(81.3676282255091,8.73788135389401,57.31821791631));
#154840=CARTESIAN_POINT('',(64.7026068549496,8.73787995439493,60.2567108302939));
#154841=CARTESIAN_POINT('Ctrl Pts',(81.3676282316625,8.73788135390567,57.318217951183));
#154842=CARTESIAN_POINT('Ctrl Pts',(81.2087098997806,8.79636286454771,57.346239540823));
#154843=CARTESIAN_POINT('Ctrl Pts',(81.0460194198263,8.85311144861849,57.3749262452573));
#154844=CARTESIAN_POINT('Ctrl Pts',(80.879564119114,8.90817525433878,57.404276787864));
#154845=CARTESIAN_POINT('Ctrl Pts',(80.7218084076859,8.96036121542369,57.4320933590991));
#154846=CARTESIAN_POINT('Ctrl Pts',(80.5606711114645,9.01103370167497,57.4605061948796));
#154847=CARTESIAN_POINT('Ctrl Pts',(80.3961944404702,9.06026076227427,57.489507859617));
#154848=CARTESIAN_POINT('Ctrl Pts',(80.2448213934373,9.10556597251676,57.5161990027061));
#154849=CARTESIAN_POINT('Ctrl Pts',(80.090620016467,9.14964691300423,57.5433888623393));
#154850=CARTESIAN_POINT('Ctrl Pts',(79.9336532193732,9.19258112448351,57.5710663427408));
#154851=CARTESIAN_POINT('Ctrl Pts',(79.8707917540675,9.20977525404021,57.58215051472));
#154852=CARTESIAN_POINT('Ctrl Pts',(79.8074871650171,9.22678582049492,57.5933128217162));
#154853=CARTESIAN_POINT('Ctrl Pts',(79.7437354288369,9.24360804525351,57.6045539728719));
#154854=CARTESIAN_POINT('Ctrl Pts',(79.4985200072644,9.30831324676067,57.6477920677814));
#154855=CARTESIAN_POINT('Ctrl Pts',(79.246746324175,9.3702979433272,57.6921865627655));
#154856=CARTESIAN_POINT('Ctrl Pts',(78.9881445367556,9.42934575710402,57.7377850365787));
#154857=CARTESIAN_POINT('Ctrl Pts',(78.7466393188292,9.48448982736184,57.780368923818));
#154858=CARTESIAN_POINT('Ctrl Pts',(78.4991787716111,9.53707191423088,57.8240028948914));
#154859=CARTESIAN_POINT('Ctrl Pts',(78.2455882533844,9.58691893897613,57.8687177431983));
#154860=CARTESIAN_POINT('Ctrl Pts',(78.1786342973979,9.60007974453066,57.8805235315473));
#154861=CARTESIAN_POINT('Ctrl Pts',(78.1112532983418,9.61304993661468,57.8924046190412));
#154862=CARTESIAN_POINT('Ctrl Pts',(78.0434426503664,9.62582644832172,57.9043614653979));
#154863=CARTESIAN_POINT('Ctrl Pts',(77.9943883457167,9.63506899232256,57.9130110624944));
#154864=CARTESIAN_POINT('Ctrl Pts',(77.9451092107804,9.64421018988931,57.9217003033261));
#154865=CARTESIAN_POINT('Ctrl Pts',(77.895603477672,9.65324711977084,57.9304294997728));
#154866=CARTESIAN_POINT('Ctrl Pts',(77.6104542861935,9.70529913652465,57.9807089957573));
#154867=CARTESIAN_POINT('Ctrl Pts',(77.3177944791281,9.7539232726487,58.0323128302488));
#154868=CARTESIAN_POINT('Ctrl Pts',(77.017571009771,9.79862093414819,58.0852503400246));
#154869=CARTESIAN_POINT('Ctrl Pts',(76.7258995738197,9.8420453577655,58.1366798952325));
#154870=CARTESIAN_POINT('Ctrl Pts',(76.4270889872002,9.88176373028796,58.1893682585896));
#154871=CARTESIAN_POINT('Ctrl Pts',(76.1211255271846,9.9172842206695,58.2433178523359));
#154872=CARTESIAN_POINT('Ctrl Pts',(76.0487109490709,9.92569111123492,58.2560864916706));
#154873=CARTESIAN_POINT('Ctrl Pts',(75.9758958620973,9.93386269940829,58.2689257514992));
#154874=CARTESIAN_POINT('Ctrl Pts',(75.9026804047984,9.94179217756508,58.2818356096016));
#154875=CARTESIAN_POINT('Ctrl Pts',(75.8725910730752,9.94505095252126,58.2871411696196));
#154876=CARTESIAN_POINT('Ctrl Pts',(75.8424341220151,9.94826883511575,58.2924586531357));
#154877=CARTESIAN_POINT('Ctrl Pts',(75.8122095038501,9.95144517225851,58.2977880687998));
#154878=CARTESIAN_POINT('Ctrl Pts',(75.6129449749411,9.97238609270137,58.3329237815446));
#154879=CARTESIAN_POINT('Ctrl Pts',(75.4107482586051,9.99147803552478,58.3685765513916));
#154880=CARTESIAN_POINT('Ctrl Pts',(75.2052376707838,10.008466872973,58.40481366752));
#154881=CARTESIAN_POINT('Ctrl Pts',(75.0035537627652,10.0251393722616,58.4403760357346));
#154882=CARTESIAN_POINT('Ctrl Pts',(74.7986780933736,10.039786500644,58.4765012135102));
#154883=CARTESIAN_POINT('Ctrl Pts',(74.5902601914052,10.0521200015532,58.5132509362234));
#154884=CARTESIAN_POINT('Ctrl Pts',(74.3880141962563,10.0640882688733,58.548912384551));
#154885=CARTESIAN_POINT('Ctrl Pts',(74.1824325273812,10.07387795741,58.5851619478052));
#154886=CARTESIAN_POINT('Ctrl Pts',(73.9732067158383,10.0811787248403,58.6220540275996));
#154887=CARTESIAN_POINT('Ctrl Pts',(73.8131362535894,10.0867642556537,58.6502787108855));
#154888=CARTESIAN_POINT('Ctrl Pts',(73.6509330157534,10.0908920808399,58.6788794326511));
#154889=CARTESIAN_POINT('Ctrl Pts',(73.4864645224222,10.0934033427859,58.7078796595598));
#154890=CARTESIAN_POINT('Ctrl Pts',(73.4812596380798,10.0934828159283,58.7087974209128));
#154891=CARTESIAN_POINT('Ctrl Pts',(73.4760524855103,10.0935606685529,58.7097155823065));
#154892=CARTESIAN_POINT('Ctrl Pts',(73.4708430605507,10.0936368963972,58.7106341444809));
#154893=CARTESIAN_POINT('Ctrl Pts',(73.313719697043,10.0959360321715,58.738339232767));
#154894=CARTESIAN_POINT('Ctrl Pts',(73.1545210835498,10.0969060906889,58.7664103272364));
#154895=CARTESIAN_POINT('Ctrl Pts',(72.9939823965101,10.0964561168859,58.7947177107984));
#154896=CARTESIAN_POINT('Ctrl Pts',(72.8341151294458,10.0960080250055,58.8229067045621));
#154897=CARTESIAN_POINT('Ctrl Pts',(72.6729190852784,10.0941517127178,58.851329996284));
#154898=CARTESIAN_POINT('Ctrl Pts',(72.5111223893388,10.0908490929896,58.8798591609756));
#154899=CARTESIAN_POINT('Ctrl Pts',(72.349012790577,10.0875400862395,58.908443498958));
#154900=CARTESIAN_POINT('Ctrl Pts',(72.1863003330493,10.0827791597301,58.9371340995332));
#154901=CARTESIAN_POINT('Ctrl Pts',(72.0237177999578,10.0765805260161,58.9658017542732));
#154902=CARTESIAN_POINT('Ctrl Pts',(71.8603464080213,10.0703518162113,58.9946085059542));
#154903=CARTESIAN_POINT('Ctrl Pts',(71.6971063286149,10.0626714542577,59.0233920672517));
#154904=CARTESIAN_POINT('Ctrl Pts',(71.5347396565587,10.0536066711788,59.0520216173761));
#154905=CARTESIAN_POINT('Ctrl Pts',(71.3703135220802,10.0444269101929,59.0810143053409));
#154906=CARTESIAN_POINT('Ctrl Pts',(71.2067832228854,10.0338274401187,59.1098490278532));
#154907=CARTESIAN_POINT('Ctrl Pts',(71.0449160659144,10.0219314966988,59.1383905417107));
#154908=CARTESIAN_POINT('Ctrl Pts',(70.9990218191482,10.0185586360577,59.1464829262596));
#154909=CARTESIAN_POINT('Ctrl Pts',(70.9532612441384,10.0150818744564,59.1545517448528));
#154910=CARTESIAN_POINT('Ctrl Pts',(70.9076517592672,10.011504773392,59.1625939276118));
#154911=CARTESIAN_POINT('Ctrl Pts',(70.8844280704287,10.0096833653604,59.1666888905456));
#154912=CARTESIAN_POINT('Ctrl Pts',(70.8612434278685,10.0078331957779,59.1707769699724));
#154913=CARTESIAN_POINT('Ctrl Pts',(70.8380978782737,10.0059546557708,59.174858157267));
#154914=CARTESIAN_POINT('Ctrl Pts',(70.5639884063584,9.98370737202299,59.2231910814659));
#154915=CARTESIAN_POINT('Ctrl Pts',(70.2953657364984,9.95748310183114,59.2705566163134));
#154916=CARTESIAN_POINT('Ctrl Pts',(70.0323257265772,9.92788208337571,59.3169376710089));
#154917=CARTESIAN_POINT('Ctrl Pts',(69.7622598959452,9.89749041923642,59.3645575675625));
#154918=CARTESIAN_POINT('Ctrl Pts',(69.4980787513188,9.86353935820031,59.4111397681367));
#154919=CARTESIAN_POINT('Ctrl Pts',(69.2398383678665,9.82665089058296,59.4566744756763));
#154920=CARTESIAN_POINT('Ctrl Pts',(69.0030022172092,9.79281992054897,59.4984350427527));
#154921=CARTESIAN_POINT('Ctrl Pts',(68.7711621228901,9.75651798925938,59.5393146945093));
#154922=CARTESIAN_POINT('Ctrl Pts',(68.5443295182875,9.71820398339368,59.5793114028052));
#154923=CARTESIAN_POINT('Ctrl Pts',(68.4979540337069,9.71037075945588,59.5874886519803));
#154924=CARTESIAN_POINT('Ctrl Pts',(68.451788756776,9.70245224538409,59.595628836128));
#154925=CARTESIAN_POINT('Ctrl Pts',(68.4058309666273,9.69445075333064,59.6037324348464));
#154926=CARTESIAN_POINT('Ctrl Pts',(68.1335570607557,9.64704643978242,59.6517416726167));
#154927=CARTESIAN_POINT('Ctrl Pts',(67.8685694281125,9.59673179975426,59.6984661438657));
#154928=CARTESIAN_POINT('Ctrl Pts',(67.610388088832,9.54366699229344,59.7439904786632));
#154929=CARTESIAN_POINT('Ctrl Pts',(67.346491205237,9.48942745137039,59.7905226181054));
#154930=CARTESIAN_POINT('Ctrl Pts',(67.089704291705,9.43231545711566,59.8358010774));
#154931=CARTESIAN_POINT('Ctrl Pts',(66.8394768016439,9.372464570161,59.8799229349657));
#154932=CARTESIAN_POINT('Ctrl Pts',(66.7205692919111,9.34402357064757,59.9008895370231));
#154933=CARTESIAN_POINT('Ctrl Pts',(66.6031425341752,9.31496347614318,59.9215950427055));
#154934=CARTESIAN_POINT('Ctrl Pts',(66.4871355313901,9.28529498604309,59.9420502072477));
#154935=CARTESIAN_POINT('Ctrl Pts',(66.4248180118144,9.26935744203104,59.9530384673198));
#154936=CARTESIAN_POINT('Ctrl Pts',(66.3629127008068,9.25324277664608,59.9639540438851));
#154937=CARTESIAN_POINT('Ctrl Pts',(66.30141756641,9.23695619266647,59.9747972953772));
#154938=CARTESIAN_POINT('Ctrl Pts',(66.131765985172,9.19202508141341,60.0047114467883));
#154939=CARTESIAN_POINT('Ctrl Pts',(65.9652394658963,9.14578249704889,60.0340745667036));
#154940=CARTESIAN_POINT('Ctrl Pts',(65.801950109141,9.09815126322316,60.0628668933248));
#154941=CARTESIAN_POINT('Ctrl Pts',(65.6347159065267,9.04936932442035,60.0923548028837));
#154942=CARTESIAN_POINT('Ctrl Pts',(65.4708770287103,8.99913104760663,60.1212440317185));
#154943=CARTESIAN_POINT('Ctrl Pts',(65.3105126467954,8.94738991497825,60.1495206156003));
#154944=CARTESIAN_POINT('Ctrl Pts',(65.1443606514881,8.89378142459526,60.1788177124765));
#154945=CARTESIAN_POINT('Ctrl Pts',(64.981938417273,8.83855984079847,60.2074571537367));
#154946=CARTESIAN_POINT('Ctrl Pts',(64.8232916151915,8.78170889653389,60.2354308722771));
#154947=CARTESIAN_POINT('Ctrl Pts',(64.7828177266181,8.76720511358165,60.2425675126148));
#154948=CARTESIAN_POINT('Ctrl Pts',(64.7425893597467,8.75259544747843,60.2496608600567));
#154949=CARTESIAN_POINT('Ctrl Pts',(64.7026068590706,8.73787995440276,60.2567108536817));
#154950=CARTESIAN_POINT('',(61.8548446843784,7.54727709634001,60.7588480660759));
#154951=CARTESIAN_POINT('Ctrl Pts',(64.7026068528891,8.73787995439101,60.2567108186));
#154952=CARTESIAN_POINT('Ctrl Pts',(64.3947973318191,8.62477534901001,60.31098594208));
#154953=CARTESIAN_POINT('Ctrl Pts',(63.7735190092491,8.38547959455801,60.42053398858));
#154954=CARTESIAN_POINT('Ctrl Pts',(62.8261686619491,7.98775290683101,60.58757744947));
#154955=CARTESIAN_POINT('Ctrl Pts',(62.1799654461091,7.69932044348701,60.7015205038));
#154956=CARTESIAN_POINT('Ctrl Pts',(61.8548446843791,7.54727709634001,60.75884806608));
#154957=CARTESIAN_POINT('',(61.7095776082786,7.4812853662219,60.7844468788789));
#154958=CARTESIAN_POINT('Ctrl Pts',(61.8548446843769,7.54727709634,60.7588480660678));
#154959=CARTESIAN_POINT('Ctrl Pts',(61.830610270908,7.535950846149,60.763121247024));
#154960=CARTESIAN_POINT('Ctrl Pts',(61.8059568191555,7.5263062771995,60.7674683157356));
#154961=CARTESIAN_POINT('Ctrl Pts',(61.7817268381449,7.51550163332151,60.7717407151298));
#154962=CARTESIAN_POINT('Ctrl Pts',(61.7574968571344,7.50469698944351,60.776013114524));
#154963=CARTESIAN_POINT('Ctrl Pts',(61.7336903468659,7.49273227063699,60.7802108446008));
#154964=CARTESIAN_POINT('Ctrl Pts',(61.709580295825,7.48128536884799,60.7844620971056));
#154965=CARTESIAN_POINT('',(61.7095727627346,-7.48130385739646,60.7844478028312));
#154966=CARTESIAN_POINT('',(61.7095747601691,-7.48130386006799,60.78445910689));
#154967=CARTESIAN_POINT('Ctrl Pts',(61.7095754384465,-7.48130386006801,
60.7844629535925));
#154968=CARTESIAN_POINT('Ctrl Pts',(61.7337023565672,-7.49275138904401,
60.7802087269665));
#154969=CARTESIAN_POINT('Ctrl Pts',(61.7573216977192,-7.5046239858585,60.7760439998548));
#154970=CARTESIAN_POINT('Ctrl Pts',(61.7817452684442,-7.51551609139476,
60.7717374653708));
#154971=CARTESIAN_POINT('Ctrl Pts',(61.8061688391693,-7.526408196931,60.7674309308867));
#154972=CARTESIAN_POINT('Ctrl Pts',(61.8313966394674,-7.536319811189,60.7629825890302));
#154973=CARTESIAN_POINT('Ctrl Pts',(61.8556180259576,-7.547638577278,60.7587117050818));
#154974=CARTESIAN_POINT('Ctrl Pts',(81.3676320519491,-8.73787997305799,
57.31821724176));
#154975=CARTESIAN_POINT('Ctrl Pts',(81.4558177302491,-8.70547663004399,
57.30266772736));
#154976=CARTESIAN_POINT('Ctrl Pts',(81.6322430735685,-8.63901488156727,
57.2715590931222));
#154977=CARTESIAN_POINT('Ctrl Pts',(81.8095955022414,-8.57149553463792,
57.2402871035593));
#154978=CARTESIAN_POINT('Ctrl Pts',(81.898376792049,-8.53713216053471,57.2246325667929));
#154979=CARTESIAN_POINT('Ctrl Pts',(81.7702420948291,-9.98581821596098,
57.96180292846));
#154980=CARTESIAN_POINT('Ctrl Pts',(81.8773200986491,-9.94703058694397,
57.94292218735));
#154981=CARTESIAN_POINT('Ctrl Pts',(82.1129399024391,-9.86032094569297,
57.90137605875));
#154982=CARTESIAN_POINT('Ctrl Pts',(82.3927019950691,-9.75384394443899,
57.85204645364));
#154983=CARTESIAN_POINT('Ctrl Pts',(82.5654880401691,-9.68649744342697,
57.821579612));
#154984=CARTESIAN_POINT('Ctrl Pts',(82.6104698889891,-9.668857973788,57.81364809841));
#154985=CARTESIAN_POINT('Ctrl Pts',(81.5614869693291,-9.66248792385799,
57.44212653776));
#154986=CARTESIAN_POINT('Ctrl Pts',(81.6674971093891,-9.62408711525799,
57.42343408984));
#154987=CARTESIAN_POINT('Ctrl Pts',(81.9007846866091,-9.53823585217798,
57.38229919571));
#154988=CARTESIAN_POINT('Ctrl Pts',(82.1778276085491,-9.43279395884399,
57.33344905376));
#154989=CARTESIAN_POINT('Ctrl Pts',(82.3489593127491,-9.36609228455299,
57.30327391705));
#154990=CARTESIAN_POINT('Ctrl Pts',(82.3935122424591,-9.34862101415597,
57.29541803347));
#154991=CARTESIAN_POINT('Ctrl Pts',(81.3205762370191,-9.10265723476799,
57.22594062351));
#154992=CARTESIAN_POINT('Ctrl Pts',(81.4247374228791,-9.06492618692099,
57.2075741961001));
#154993=CARTESIAN_POINT('Ctrl Pts',(81.6539868631391,-8.98056116393499,
57.16715133447));
#154994=CARTESIAN_POINT('Ctrl Pts',(81.9263216731591,-8.87691150966299,
57.11913135968));
#154995=CARTESIAN_POINT('Ctrl Pts',(82.0945889664591,-8.81132632150599,
57.0894612959));
#154996=CARTESIAN_POINT('Ctrl Pts',(82.1383992435791,-8.79414627992399,
57.08173636201));
#154997=CARTESIAN_POINT('Ctrl Pts',(81.1333888323891,-8.50589244697699,
57.39031031181));
#154998=CARTESIAN_POINT('Ctrl Pts',(81.2355790816991,-8.46887534647299,
57.3722914136901));
#154999=CARTESIAN_POINT('Ctrl Pts',(81.4605239741791,-8.38609461632999,
57.33262755997));
#155000=CARTESIAN_POINT('Ctrl Pts',(81.7278400607391,-8.28435544175299,
57.28549252153));
#155001=CARTESIAN_POINT('Ctrl Pts',(81.8930539673891,-8.21996039844499,
57.2563608522));
#155002=CARTESIAN_POINT('Ctrl Pts',(81.9360725963791,-8.20309079911799,
57.24877550724));
#155003=CARTESIAN_POINT('',(82.3445054699596,-9.52426778569044,57.5877997674927));
#155004=CARTESIAN_POINT('Origin',(82.1588614745391,-8.53712735499399,58.70184200703));
#155005=CARTESIAN_POINT('Origin',(70.1868938445538,19.4102088531332,61.5764747906095));
#155006=CARTESIAN_POINT('Ctrl Pts',(84.0442680918191,-11.95582982209,59.18935354422));
#155007=CARTESIAN_POINT('Ctrl Pts',(81.8918266601391,-9.61525107327999,
58.42149541083));
#155008=CARTESIAN_POINT('Ctrl Pts',(79.7745014548291,-8.34407927290099,
56.24909744227));
#155009=CARTESIAN_POINT('Ctrl Pts',(78.3288817485491,-8.55554395195999,
53.28264952));
#155010=CARTESIAN_POINT('Ctrl Pts',(85.1121236298391,-11.35883600978,58.70841656241));
#155011=CARTESIAN_POINT('Ctrl Pts',(82.7330218046191,-9.02815085113,58.0565061079401));
#155012=CARTESIAN_POINT('Ctrl Pts',(80.4127135380691,-7.79958765931899,
55.8783245343));
#155013=CARTESIAN_POINT('Ctrl Pts',(78.8938373461991,-8.10009195420299,
52.8212125382));
#155014=CARTESIAN_POINT('Ctrl Pts',(86.0708998648091,-10.68228981744,58.23459657962));
#155015=CARTESIAN_POINT('Ctrl Pts',(83.4615653605592,-8.38274450323699,
57.714890811));
#155016=CARTESIAN_POINT('Ctrl Pts',(80.9478736525491,-7.20591802747199,
55.5272558574701));
#155017=CARTESIAN_POINT('Ctrl Pts',(79.3875877710191,-7.58953754562799,
52.35946311877));
#155018=CARTESIAN_POINT('Ctrl Pts',(86.9329409753991,-9.92711979710299,
57.7857695233));
#155019=CARTESIAN_POINT('Ctrl Pts',(84.0933088102791,-7.69990047563699,
57.41104593754));
#155020=CARTESIAN_POINT('Ctrl Pts',(81.3965784204191,-6.58687843436799,
55.21311191527));
#155021=CARTESIAN_POINT('Ctrl Pts',(79.8215157765292,-7.02960519182299,
51.92060906181));
#155022=CARTESIAN_POINT('Ctrl Pts',(82.3445054687794,-9.52426777936283,
57.5877997772795));
#155023=CARTESIAN_POINT('Ctrl Pts',(82.346531728505,-9.68011068266613,57.7262280958423));
#155024=CARTESIAN_POINT('Ctrl Pts',(82.3485329827188,-9.83740635046138,
57.8622242865471));
#155025=CARTESIAN_POINT('Ctrl Pts',(82.3504900740855,-9.9963050532987,57.9955223328722));
#155026=CARTESIAN_POINT('Ctrl Pts',(82.3511858079024,-10.0527925545503,
58.0429089598501));
#155027=CARTESIAN_POINT('Ctrl Pts',(82.3518761372479,-10.1094822257348,
58.0899544567353));
#155028=CARTESIAN_POINT('Ctrl Pts',(82.3525607872356,-10.1663794243756,
58.1366463490096));
#155029=CARTESIAN_POINT('Ctrl Pts',(82.043884088149,-9.44562267741599,57.50371656119));
#155030=CARTESIAN_POINT('Ctrl Pts',(82.044039598059,-9.45922946787,57.51651606553));
#155031=CARTESIAN_POINT('Ctrl Pts',(82.0459853009791,-9.62874435123598,
57.67559019143));
#155032=CARTESIAN_POINT('Ctrl Pts',(82.049394194429,-9.91110503789099,57.93262616537));
#155033=CARTESIAN_POINT('Ctrl Pts',(82.0528541451991,-10.18503707275,58.1689905444));
#155034=CARTESIAN_POINT('Ctrl Pts',(82.0543047412092,-10.29908415109,58.26507845926));
#155035=CARTESIAN_POINT('Ctrl Pts',(83.0663576928291,-9.40090354793498,
57.3716525166401));
#155036=CARTESIAN_POINT('Ctrl Pts',(83.0664294579292,-9.41553184202599,
57.38345779192));
#155037=CARTESIAN_POINT('Ctrl Pts',(83.0672929144891,-9.59770268033198,
57.53015586066));
#155038=CARTESIAN_POINT('Ctrl Pts',(83.0681107121791,-9.899697052152,57.76678515028));
#155039=CARTESIAN_POINT('Ctrl Pts',(83.0680607108091,-10.19037421172,57.9837057944601));
#155040=CARTESIAN_POINT('Ctrl Pts',(83.0679027349291,-10.31099202241,58.07176439365));
#155041=CARTESIAN_POINT('Ctrl Pts',(83.7612238213791,-8.82417024784398,
57.87108493871));
#155042=CARTESIAN_POINT('Ctrl Pts',(83.7624324745491,-8.83995187633898,
57.8826402837801));
#155043=CARTESIAN_POINT('Ctrl Pts',(83.7773932391891,-9.03649860696499,
58.02622515743));
#155044=CARTESIAN_POINT('Ctrl Pts',(83.8003368389191,-9.36257781544699,
58.25767378284));
#155045=CARTESIAN_POINT('Ctrl Pts',(83.8197704260491,-9.67659535880799,
58.46952040891));
#155046=CARTESIAN_POINT('Ctrl Pts',(83.8273975284591,-9.80690123912098,
58.55545143395));
#155047=CARTESIAN_POINT('Ctrl Pts',(83.613542411989,-8.14281888841199,58.63190259055));
#155048=CARTESIAN_POINT('Ctrl Pts',(83.616266079629,-8.15903098781899,58.64413751846));
#155049=CARTESIAN_POINT('Ctrl Pts',(83.650056703569,-8.36102009624099,58.79617913494));
#155050=CARTESIAN_POINT('Ctrl Pts',(83.7034463744892,-8.69778689479599,
59.04151231842));
#155051=CARTESIAN_POINT('Ctrl Pts',(83.7509185106491,-9.02444336993198,
59.26641481374));
#155052=CARTESIAN_POINT('Ctrl Pts',(83.7699551026291,-9.16037518045798,
59.35769667413));
#155053=CARTESIAN_POINT('Origin',(82.1588614726791,-8.53712737026499,58.70184199665));
#155054=CARTESIAN_POINT('Origin',(82.1588614745091,-8.53712735484699,58.70184200704));
#155055=CARTESIAN_POINT('Ctrl Pts',(61.3269057219591,-8.495578707918,61.36288605057));
#155056=CARTESIAN_POINT('Ctrl Pts',(61.3647221303192,-8.51352689253799,
61.35621799746));
#155057=CARTESIAN_POINT('Ctrl Pts',(61.4169935891791,-8.53819570856299,
61.34700112894));
#155058=CARTESIAN_POINT('Ctrl Pts',(61.4693484792691,-8.56270798360799,
61.33776954924));
#155059=CARTESIAN_POINT('Ctrl Pts',(61.4837887359291,-8.56945389890299,
61.33522334239));
#155060=CARTESIAN_POINT('Ctrl Pts',(61.4076467126991,-8.16570792682499,
60.93289001715));
#155061=CARTESIAN_POINT('Ctrl Pts',(61.4449938331991,-8.18343338001699,
60.92630471215));
#155062=CARTESIAN_POINT('Ctrl Pts',(61.4966121580391,-8.20779394370498,
60.91720300878));
#155063=CARTESIAN_POINT('Ctrl Pts',(61.5483071585291,-8.23199726141499,
60.90808778543));
#155064=CARTESIAN_POINT('Ctrl Pts',(61.5625649852991,-8.23865795307699,
60.90557374588));
#155065=CARTESIAN_POINT('Ctrl Pts',(61.5943982728691,-7.69471886378999,
60.72426695352));
#155066=CARTESIAN_POINT('Ctrl Pts',(61.6310753447891,-7.712126301345,60.71779979617));
#155067=CARTESIAN_POINT('Ctrl Pts',(61.6817611257391,-7.73604674275599,
60.70886252545));
#155068=CARTESIAN_POINT('Ctrl Pts',(61.7325139367491,-7.75980893159299,
60.6999134355201));
#155069=CARTESIAN_POINT('Ctrl Pts',(61.7465112903491,-7.76634794106699,
60.69744532442));
#155070=CARTESIAN_POINT('Ctrl Pts',(61.8372995538392,-7.20836101379599,
60.79271718683));
#155071=CARTESIAN_POINT('Ctrl Pts',(61.8732847128991,-7.22544005858399,
60.78637203238));
#155072=CARTESIAN_POINT('Ctrl Pts',(61.9230075202292,-7.24890601614099,
60.77760455989));
#155073=CARTESIAN_POINT('Ctrl Pts',(61.9727873972891,-7.27221268168199,
60.76882702447));
#155074=CARTESIAN_POINT('Ctrl Pts',(61.9865157782691,-7.27862603836998,
60.7664063405));
#155075=CARTESIAN_POINT('',(61.3905222458867,-8.28493716412695,61.1354064364425));
#155076=CARTESIAN_POINT('Ctrl Pts',(61.3905294889791,-8.28492712720199,
61.13542050615));
#155077=CARTESIAN_POINT('Ctrl Pts',(61.4674394663872,-8.04432492131577,
60.924176948769));
#155078=CARTESIAN_POINT('Ctrl Pts',(61.5789829799692,-7.76585888253086,
60.8074607170329));
#155079=CARTESIAN_POINT('Ctrl Pts',(61.7095747601691,-7.48130386006799,
60.78445910689));
#155080=CARTESIAN_POINT('Ctrl Pts',(61.3905222458867,-8.28493716412695,
61.1354064364425));
#155081=CARTESIAN_POINT('Ctrl Pts',(61.439093656703,-8.31187513499146,61.1296186241446));
#155082=CARTESIAN_POINT('Ctrl Pts',(61.4877657995991,-8.3386626725425,61.1238255489273));
#155083=CARTESIAN_POINT('Ctrl Pts',(61.5365392768834,-8.36530895132786,
61.1180360527177));
#155084=CARTESIAN_POINT('Ctrl Pts',(62.6424555061691,-7.77604012554399,
59.87323994982));
#155085=CARTESIAN_POINT('Ctrl Pts',(61.8379543617991,-8.32413368283999,
61.12832290559));
#155086=CARTESIAN_POINT('Ctrl Pts',(60.8091181018691,-9.16035193985399,
62.11581956026));
#155087=CARTESIAN_POINT('Ctrl Pts',(59.7096837229991,-10.16199998466,62.67784534094));
#155088=CARTESIAN_POINT('Ctrl Pts',(61.9505428605791,-7.28867726858799,
59.92779417502));
#155089=CARTESIAN_POINT('Ctrl Pts',(61.0752928453991,-7.79388560581099,
61.12485983068));
#155090=CARTESIAN_POINT('Ctrl Pts',(59.9706799034791,-8.55606341233799,
62.04936186926));
#155091=CARTESIAN_POINT('Ctrl Pts',(58.7973007554591,-9.46702852828699,
62.55790618144));
#155092=CARTESIAN_POINT('Ctrl Pts',(61.0397767654491,-6.48728583724199,
59.97697348357));
#155093=CARTESIAN_POINT('Ctrl Pts',(60.0827831329091,-6.92037734173899,
61.08879812396));
#155094=CARTESIAN_POINT('Ctrl Pts',(58.8947164971891,-7.56515213793899,
61.92331331462));
#155095=CARTESIAN_POINT('Ctrl Pts',(57.6405715268691,-8.33435433040299,
62.35656344383));
#155096=CARTESIAN_POINT('Ctrl Pts',(60.0688746546991,-5.27194363025099,
60.00234697595));
#155097=CARTESIAN_POINT('Ctrl Pts',(59.0408262773091,-5.60461176273999,
61.0151475571));
#155098=CARTESIAN_POINT('Ctrl Pts',(57.7857638448791,-6.09372256888499,
61.74863088935));
#155099=CARTESIAN_POINT('Ctrl Pts',(56.4678784022591,-6.67671573941599,
62.09945975638));
#155100=CARTESIAN_POINT('Ctrl Pts',(59.4770560102391,-4.32125532974499,
60.00642490582));
#155101=CARTESIAN_POINT('Ctrl Pts',(58.4136231286291,-4.58127352118499,
60.95656721084));
#155102=CARTESIAN_POINT('Ctrl Pts',(57.1281453354791,-4.96056460946199,
61.62786539327));
#155103=CARTESIAN_POINT('Ctrl Pts',(55.7820195624491,-5.41264480586399,
61.92925370837));
#155104=CARTESIAN_POINT('Ctrl Pts',(59.0055325931291,-3.29999083432499,
60.00206093384));
#155105=CARTESIAN_POINT('Ctrl Pts',(57.9201032021691,-3.49064234678699,
60.90165448937));
#155106=CARTESIAN_POINT('Ctrl Pts',(56.6182263543491,-3.76707829037499,
61.52424896709));
#155107=CARTESIAN_POINT('Ctrl Pts',(55.2575867634991,-4.09661278804299,
61.78816659785));
#155108=CARTESIAN_POINT('Ctrl Pts',(58.5486233310291,-1.86656057990399,
59.99197481201));
#155109=CARTESIAN_POINT('Ctrl Pts',(57.4463566197091,-1.96891264366899,
60.84184399687));
#155110=CARTESIAN_POINT('Ctrl Pts',(56.1342847286391,-2.11626651270099,
61.41753985169));
#155111=CARTESIAN_POINT('Ctrl Pts',(54.7653910149991,-2.29199771900499,
61.64625014668));
#155112=CARTESIAN_POINT('Ctrl Pts',(58.3582172880991,-0.364152247367286,
59.98205701354));
#155113=CARTESIAN_POINT('Ctrl Pts',(57.2534029238191,-0.383925391423086,
60.81057084221));
#155114=CARTESIAN_POINT('Ctrl Pts',(55.9427550000591,-0.412412157066686,
61.36713327766));
#155115=CARTESIAN_POINT('Ctrl Pts',(54.5762064592391,-0.446400905279986,
61.58237710042));
#155116=CARTESIAN_POINT('Ctrl Pts',(58.4563178714691,1.13682553069601,59.98708278791));
#155117=CARTESIAN_POINT('Ctrl Pts',(57.3528856763591,1.19880013307101,60.82659338268));
#155118=CARTESIAN_POINT('Ctrl Pts',(56.0415920647091,1.28805985484101,61.39302436016));
#155119=CARTESIAN_POINT('Ctrl Pts',(54.6739248975291,1.39453885209001,61.61522897311));
#155120=CARTESIAN_POINT('Ctrl Pts',(58.6684090262891,2.24546507681701,59.99462082065));
#155121=CARTESIAN_POINT('Ctrl Pts',(57.5705549788991,2.37120525228701,60.85752631199));
#155122=CARTESIAN_POINT('Ctrl Pts',(56.2611536705391,2.55273821128001,61.44551740073));
#155123=CARTESIAN_POINT('Ctrl Pts',(54.8944216917291,2.76918920966101,61.68345776097));
#155124=CARTESIAN_POINT('Ctrl Pts',(59.0129434444591,3.31779743315801,60.00214865606));
#155125=CARTESIAN_POINT('Ctrl Pts',(57.9278466186591,3.50960883722001,60.90254051803));
#155126=CARTESIAN_POINT('Ctrl Pts',(56.6262103281791,3.78775995029701,61.52590143521));
#155127=CARTESIAN_POINT('Ctrl Pts',(55.2657813302291,4.11933921369801,61.79040654324));
#155128=CARTESIAN_POINT('Ctrl Pts',(59.4834197823591,4.33310144087101,60.00646456182));
#155129=CARTESIAN_POINT('Ctrl Pts',(58.4203057347191,4.59398713221801,60.95729393492));
#155130=CARTESIAN_POINT('Ctrl Pts',(57.1350750964291,4.97457145865601,61.62926036187));
#155131=CARTESIAN_POINT('Ctrl Pts',(55.7891716005991,5.42819059581601,61.93116907861));
#155132=CARTESIAN_POINT('Ctrl Pts',(60.0753871131491,5.27952185925301,60.00213395257));
#155133=CARTESIAN_POINT('Ctrl Pts',(59.0478312209291,5.61281571356601,61.01557669505));
#155134=CARTESIAN_POINT('Ctrl Pts',(57.7932429430791,6.10290620065401,61.74971718187));
#155135=CARTESIAN_POINT('Ctrl Pts',(56.4758102450491,6.68707454965501,62.10108184812));
#155136=CARTESIAN_POINT('Ctrl Pts',(61.0501979198291,6.49523278975501,59.97628350722));
#155137=CARTESIAN_POINT('Ctrl Pts',(60.0942006841991,6.92904513194801,61.08903090901));
#155138=CARTESIAN_POINT('Ctrl Pts',(58.9071773606691,7.57502746814901,61.9245323559));
#155139=CARTESIAN_POINT('Ctrl Pts',(57.6540464565791,8.34569757739901,62.35861252668));
#155140=CARTESIAN_POINT('Ctrl Pts',(61.9597595856491,7.29558295991301,59.92711980225));
#155141=CARTESIAN_POINT('Ctrl Pts',(61.0854258026491,7.80140074479901,61.12497890819));
#155142=CARTESIAN_POINT('Ctrl Pts',(59.9817847430291,8.56461376917001,62.05033656025));
#155143=CARTESIAN_POINT('Ctrl Pts',(58.8093524363191,9.47684203488101,62.5596047531));
#155144=CARTESIAN_POINT('Ctrl Pts',(62.6430578172491,7.77642528815001,59.87318767161));
#155145=CARTESIAN_POINT('Ctrl Pts',(61.8386206584491,8.32455263239701,61.12831924649));
#155146=CARTESIAN_POINT('Ctrl Pts',(60.8098537966191,9.16083079049501,62.11586923259));
#155147=CARTESIAN_POINT('Ctrl Pts',(59.7104872797291,10.16255263743,62.67794052264));
#155148=CARTESIAN_POINT('',(61.5365898356002,8.36429289895023,61.1191118314549));
#155149=CARTESIAN_POINT('Ctrl Pts',(59.6330698027491,9.92669722269101,62.60067754791));
#155150=CARTESIAN_POINT('Ctrl Pts',(60.2754754017191,9.36357130994093,62.26469288354));
#155151=CARTESIAN_POINT('Ctrl Pts',(60.931205048551,8.82195183547381,61.7699139266904));
#155152=CARTESIAN_POINT('Ctrl Pts',(61.5365886724991,8.36429728100001,61.11911541945));
#155153=CARTESIAN_POINT('',(61.3903529552591,8.28473912510079,61.1353684361582));
#155154=CARTESIAN_POINT('Ctrl Pts',(61.3903529552591,8.28473912510079,61.1353684361582));
#155155=CARTESIAN_POINT('Ctrl Pts',(61.3377118247909,8.25526241917844,61.141452580646));
#155156=CARTESIAN_POINT('Ctrl Pts',(61.2829644597506,8.22251248314273,61.1464748137686));
#155157=CARTESIAN_POINT('Ctrl Pts',(61.2264763926447,8.18609043811816,61.1501335755795));
#155158=CARTESIAN_POINT('Ctrl Pts',(61.1699883255388,8.14966839309358,61.1537923373904));
#155159=CARTESIAN_POINT('Ctrl Pts',(61.1117592919253,8.1095735985994,61.156087549914));
#155160=CARTESIAN_POINT('Ctrl Pts',(61.0522097613923,8.06541900563375,61.1567389103051));
#155161=CARTESIAN_POINT('Ctrl Pts',(60.9926602308594,8.02126441266811,61.1573902706961));
#155162=CARTESIAN_POINT('Ctrl Pts',(60.9317867017939,7.97308795619621,61.1564284489814));
#155163=CARTESIAN_POINT('Ctrl Pts',(60.8701400495052,7.92096701354577,61.1538370019321));
#155164=CARTESIAN_POINT('Ctrl Pts',(60.8393167233608,7.89490654222055,61.1525412784074));
#155165=CARTESIAN_POINT('Ctrl Pts',(60.808308205484,7.86788034015697,61.1508473165268));
#155166=CARTESIAN_POINT('Ctrl Pts',(60.7771694695725,7.83988606021754,61.1487516800523));
#155167=CARTESIAN_POINT('Ctrl Pts',(60.7616001016168,7.82588892024782,61.1477038618151));
#155168=CARTESIAN_POINT('Ctrl Pts',(60.7459972413712,7.81164787313224,61.1465548862943));
#155169=CARTESIAN_POINT('Ctrl Pts',(60.7303658056483,7.79715985209986,61.1453036153926));
#155170=CARTESIAN_POINT('Ctrl Pts',(60.7225500877868,7.78991584158367,61.1446779799418));
#155171=CARTESIAN_POINT('Ctrl Pts',(60.7147272264663,7.78261008726788,61.1440267714112));
#155172=CARTESIAN_POINT('Ctrl Pts',(60.7068978067353,7.77524228743362,61.1433499213563));
#155173=CARTESIAN_POINT('Ctrl Pts',(60.7029830968699,7.77155838751649,61.1430114963289));
#155174=CARTESIAN_POINT('Ctrl Pts',(60.6990667474229,7.76785897620417,61.1426666609589));
#155175=CARTESIAN_POINT('Ctrl Pts',(60.6951488303989,7.76414401835922,61.1423154092602));
#155176=CARTESIAN_POINT('Ctrl Pts',(60.6931898718869,7.76228653943675,61.1421397834109));
#155177=CARTESIAN_POINT('Ctrl Pts',(60.6912305214819,7.7604251738802,61.1419625534816));
#155178=CARTESIAN_POINT('Ctrl Pts',(60.6892707880624,7.75855991760359,61.1417837190025));
#155179=CARTESIAN_POINT('Ctrl Pts',(60.6873110546429,7.75669466132698,61.1416048845235));
#155180=CARTESIAN_POINT('Ctrl Pts',(60.6843542242277,7.75387325937131,61.1413318942811));
#155181=CARTESIAN_POINT('Ctrl Pts',(60.6833904476014,7.75295247262085,61.1412424015378));
#155182=CARTESIAN_POINT('Ctrl Pts',(60.6612792552886,7.73182756425257,61.1391892377623));
#155183=CARTESIAN_POINT('Ctrl Pts',(60.6355310995566,7.70686995188823,61.1366539398549));
#155184=CARTESIAN_POINT('Ctrl Pts',(60.6064952106979,7.67781946348534,61.1334020559537));
#155185=CARTESIAN_POINT('Ctrl Pts',(60.5781297503531,7.64943974069468,61.1302252569138));
#155186=CARTESIAN_POINT('Ctrl Pts',(60.5466265144245,7.61715345693505,61.1263643604354));
#155187=CARTESIAN_POINT('Ctrl Pts',(60.5123592417978,7.58071060291756,61.1216072593446));
#155188=CARTESIAN_POINT('Ctrl Pts',(60.4838518594743,7.55039332661272,61.1176497661111));
#155189=CARTESIAN_POINT('Ctrl Pts',(60.4534323333134,7.51719909725086,61.1130720895418));
#155190=CARTESIAN_POINT('Ctrl Pts',(60.4213429520122,7.48098377967267,61.107757168389));
#155191=CARTESIAN_POINT('Ctrl Pts',(60.3827970733818,7.43748181175304,61.1013728662498));
#155192=CARTESIAN_POINT('Ctrl Pts',(60.3418254808226,7.3896587533634,61.0939557525152));
#155193=CARTESIAN_POINT('Ctrl Pts',(60.2988462550389,7.337327249333,61.0853726381127));
#155194=CARTESIAN_POINT('Ctrl Pts',(60.2804176612785,7.31488859412073,61.0816923780419));
#155195=CARTESIAN_POINT('Ctrl Pts',(60.261620588273,7.29162113177491,61.077797883836));
#155196=CARTESIAN_POINT('Ctrl Pts',(60.2424908302629,7.2675105725611,61.0736793075588));
#155197=CARTESIAN_POINT('Ctrl Pts',(60.204597019692,7.21975037804492,61.0655208902285));
#155198=CARTESIAN_POINT('Ctrl Pts',(60.1651082495433,7.16825318712065,61.0563860736495));
#155199=CARTESIAN_POINT('Ctrl Pts',(60.1248164208882,7.11365044413259,61.0463747624552));
#155200=CARTESIAN_POINT('Ctrl Pts',(60.0973301082003,7.07640150017828,61.0395452379811));
#155201=CARTESIAN_POINT('Ctrl Pts',(60.0694694898623,7.03770787784243,61.0323079317492));
#155202=CARTESIAN_POINT('Ctrl Pts',(60.0414742272431,6.9977780246817,61.0246955120611));
#155203=CARTESIAN_POINT('Ctrl Pts',(59.9785441792343,6.90802042495623,61.0075836905736));
#155204=CARTESIAN_POINT('Ctrl Pts',(59.919583248113,6.81893395325138,60.989999556601));
#155205=CARTESIAN_POINT('Ctrl Pts',(59.8641613855649,6.73082734281785,60.9721977538004));
#155206=CARTESIAN_POINT('Ctrl Pts',(59.8367010755203,6.68717246136417,60.9633773532981));
#155207=CARTESIAN_POINT('Ctrl Pts',(59.8101093729386,6.64375740387163,60.954503165352));
#155208=CARTESIAN_POINT('Ctrl Pts',(59.7843328970857,6.60061556171698,60.9456043143883));
#155209=CARTESIAN_POINT('Ctrl Pts',(59.7300536100411,6.5097688359153,60.9268653956711));
#155210=CARTESIAN_POINT('Ctrl Pts',(59.6793896697743,6.42013687583715,60.9080181947062));
#155211=CARTESIAN_POINT('Ctrl Pts',(59.6318393284069,6.33199972875507,60.8893192919711));
#155212=CARTESIAN_POINT('Ctrl Pts',(59.5820720232687,6.23975331859895,60.8697485807753));
#155213=CARTESIAN_POINT('Ctrl Pts',(59.5357149928056,6.14914430700615,60.8503400762022));
#155214=CARTESIAN_POINT('Ctrl Pts',(59.4921887892894,6.0604382288152,60.8313706804393));
#155215=CARTESIAN_POINT('Ctrl Pts',(59.462012291282,5.99893875090234,60.8182192937527));
#155216=CARTESIAN_POINT('Ctrl Pts',(59.433196375619,5.9383527406437,60.8052786098179));
#155217=CARTESIAN_POINT('Ctrl Pts',(59.4055483710978,5.87875459662487,60.7926372591075));
#155218=CARTESIAN_POINT('Ctrl Pts',(59.3539010331536,5.76742339792561,60.769022820253));
#155219=CARTESIAN_POINT('Ctrl Pts',(59.3066122933732,5.65943881126518,60.7462375435995));
#155220=CARTESIAN_POINT('Ctrl Pts',(59.2630491139327,5.55506525212866,60.7244065722365));
#155221=CARTESIAN_POINT('Ctrl Pts',(59.2390317590691,5.49752177526686,60.7123706696009));
#155222=CARTESIAN_POINT('Ctrl Pts',(59.2161471056752,5.44107491983873,60.7006246744183));
#155223=CARTESIAN_POINT('Ctrl Pts',(59.1942897531849,5.38575787591432,60.6891897472044));
#155224=CARTESIAN_POINT('Ctrl Pts',(59.163538415909,5.30793174964514,60.6731018287965));
#155225=CARTESIAN_POINT('Ctrl Pts',(59.1348229842282,5.23234056849942,60.6576274853771));
#155226=CARTESIAN_POINT('Ctrl Pts',(59.107944785793,5.15908438941234,60.6427766703575));
#155227=CARTESIAN_POINT('Ctrl Pts',(59.0945056865755,5.1224562998688,60.6353512628477));
#155228=CARTESIAN_POINT('Ctrl Pts',(59.0815269848548,5.08641198790164,60.6280811498728));
#155229=CARTESIAN_POINT('Ctrl Pts',(59.0689869744624,5.05096271344002,60.6209655664145));
#155230=CARTESIAN_POINT('Ctrl Pts',(59.0627169692662,5.03323807620921,60.6174077746854));
#155231=CARTESIAN_POINT('Ctrl Pts',(59.0565566388387,5.01566219686254,60.613888618575));
#155232=CARTESIAN_POINT('Ctrl Pts',(59.0505034032855,4.99823635968953,60.6104079010811));
#155233=CARTESIAN_POINT('Ctrl Pts',(59.0474767855088,4.98952344110303,60.6086675423341));
#155234=CARTESIAN_POINT('Ctrl Pts',(59.0444769415938,4.98084803295673,60.606936793476));
#155235=CARTESIAN_POINT('Ctrl Pts',(59.0415035532834,4.97221029268076,60.605215628219));
#155236=CARTESIAN_POINT('Ctrl Pts',(59.0400168591282,4.96789142254277,60.6043550455905));
#155237=CARTESIAN_POINT('Ctrl Pts',(59.0385367788836,4.96358196936576,60.6034968588777));
#155238=CARTESIAN_POINT('Ctrl Pts',(59.0370632732322,4.95928195242892,60.6026410644859));
#155239=CARTESIAN_POINT('Ctrl Pts',(59.0363265204065,4.9571319439605,60.6022131672901));
#155240=CARTESIAN_POINT('Ctrl Pts',(59.0355914112297,4.95498429455169,60.6017858681754));
#155241=CARTESIAN_POINT('Ctrl Pts',(59.0348579408175,4.95283900658724,60.6013591666728));
#155242=CARTESIAN_POINT('Ctrl Pts',(59.0341244704053,4.95069371862278,60.6009324651701));
#155243=CARTESIAN_POINT('Ctrl Pts',(59.0338010189301,4.94974795186889,60.6007443358881));
#155244=CARTESIAN_POINT('Ctrl Pts',(59.0326624410009,4.94641022940329,60.6000808545276));
#155245=CARTESIAN_POINT('Ctrl Pts',(58.9796566010893,4.79102448184745,60.5691928618161));
#155246=CARTESIAN_POINT('Ctrl Pts',(58.930736484917,4.6357662566957,60.5392009258538));
#155247=CARTESIAN_POINT('Ctrl Pts',(58.8855150366211,4.48081331346773,60.5103268074466));
#155248=CARTESIAN_POINT('Ctrl Pts',(58.8268216235003,4.27969819102264,60.4728507728649));
#155249=CARTESIAN_POINT('Ctrl Pts',(58.7743573384257,4.07909742038663,60.4372557182607));
#155250=CARTESIAN_POINT('Ctrl Pts',(58.7271135166555,3.87967446387876,60.4039585698523));
#155251=CARTESIAN_POINT('Ctrl Pts',(58.7106768093691,3.81029276190213,60.3923740819479));
#155252=CARTESIAN_POINT('Ctrl Pts',(58.694871899034,3.74105316775628,60.3810676975273));
#155253=CARTESIAN_POINT('Ctrl Pts',(58.6796559307865,3.67198222607764,60.3700569153105));
#155254=CARTESIAN_POINT('Ctrl Pts',(58.6584438516869,3.57569270611219,60.3547071472557));
#155255=CARTESIAN_POINT('Ctrl Pts',(58.6383919111362,3.47973088583468,60.3399209525927));
#155256=CARTESIAN_POINT('Ctrl Pts',(58.619413783502,3.38410156360109,60.3257074772219));
#155257=CARTESIAN_POINT('Ctrl Pts',(58.5835603943274,3.20343909928238,60.2988554466203));
#155258=CARTESIAN_POINT('Ctrl Pts',(58.5515377751492,3.02396572657779,60.2740463222185));
#155259=CARTESIAN_POINT('Ctrl Pts',(58.5228608625712,2.84586567714671,60.2513143089754));
#155260=CARTESIAN_POINT('Ctrl Pts',(58.5004183251908,2.70648466791441,60.2335242468286));
#155261=CARTESIAN_POINT('Ctrl Pts',(58.4800258712364,2.56794413817846,60.21700666853));
#155262=CARTESIAN_POINT('Ctrl Pts',(58.4614664842412,2.43031879908165,60.2017861458073));
#155263=CARTESIAN_POINT('Ctrl Pts',(58.4541828756914,2.37630790439186,60.1958128704257));
#155264=CARTESIAN_POINT('Ctrl Pts',(58.4471815755868,2.32243511427534,60.1900389850738));
#155265=CARTESIAN_POINT('Ctrl Pts',(58.4404544275918,2.2687030578129,60.1844629675555));
#155266=CARTESIAN_POINT('Ctrl Pts',(58.4166125164259,2.07826947170898,60.1647008165773));
#155267=CARTESIAN_POINT('Ctrl Pts',(58.3962108898787,1.88960528727602,60.1474217544783));
#155268=CARTESIAN_POINT('Ctrl Pts',(58.3789027294227,1.70278520533782,60.1325898188454));
#155269=CARTESIAN_POINT('Ctrl Pts',(58.3643330923764,1.54552408023421,60.1201046145735));
#155270=CARTESIAN_POINT('Ctrl Pts',(58.3519565393527,1.38956933060372,60.1093539633021));
#155271=CARTESIAN_POINT('Ctrl Pts',(58.3415860474452,1.23495332602257,60.100332773935));
#155272=CARTESIAN_POINT('Ctrl Pts',(58.3395087708272,1.20398274006014,60.0985257713447));
#155273=CARTESIAN_POINT('Ctrl Pts',(58.3375123669455,1.17306470608009,60.0967878453344));
#155274=CARTESIAN_POINT('Ctrl Pts',(58.3355961354574,1.14220024887804,60.095118592652));
#155275=CARTESIAN_POINT('Ctrl Pts',(58.3254435033222,0.978673304477079,
60.0862745106455));
#155276=CARTESIAN_POINT('Ctrl Pts',(58.3175425203729,0.81665010430814,60.0793568043996));
#155277=CARTESIAN_POINT('Ctrl Pts',(58.311776746117,0.65624044993948,60.074314670715));
#155278=CARTESIAN_POINT('Ctrl Pts',(58.3083497361431,0.560897576452767,
60.0713177718321));
#155279=CARTESIAN_POINT('Ctrl Pts',(58.3056802608143,0.466130684709749,
60.0689816791386));
#155280=CARTESIAN_POINT('Ctrl Pts',(58.3037515412153,0.371970297407789,
60.0672905342075));
#155281=CARTESIAN_POINT('Ctrl Pts',(58.3027837784396,0.324723969935379,
60.0664419779354));
#155282=CARTESIAN_POINT('Ctrl Pts',(58.3020180653192,0.278177922856337,
60.0657590562465));
#155283=CARTESIAN_POINT('Ctrl Pts',(58.3014227085939,0.231511507082222,
60.06523424694));
#155284=CARTESIAN_POINT('Ctrl Pts',(58.3008315388136,0.185173280625659,
60.0647131284421));
#155285=CARTESIAN_POINT('Ctrl Pts',(58.3004083166453,0.138716286073158,
60.0643478840615));
#155286=CARTESIAN_POINT('Ctrl Pts',(58.3001726215235,0.091336347976081,
60.0641342783048));
#155287=CARTESIAN_POINT('Ctrl Pts',(58.3000397137522,0.0646189431954746,
60.0640138266602));
#155288=CARTESIAN_POINT('Ctrl Pts',(58.2999634391186,0.0378503959760054,
60.0639468458643));
#155289=CARTESIAN_POINT('Ctrl Pts',(58.2999452270056,0.0110309761453676,
60.0639338298282));
#155290=CARTESIAN_POINT('Ctrl Pts',(58.2998110086453,-0.186620913474732,
60.0638379051531));
#155291=CARTESIAN_POINT('Ctrl Pts',(58.302832431568,-0.387038543163136,
60.0666698817325));
#155292=CARTESIAN_POINT('Ctrl Pts',(58.3093125342766,-0.590061378700564,
60.072468905283));
#155293=CARTESIAN_POINT('Ctrl Pts',(58.3159292651874,-0.797364801485306,
60.0783901969824));
#155294=CARTESIAN_POINT('Ctrl Pts',(58.3261512202964,-1.00738343278767,
60.0874044096972));
#155295=CARTESIAN_POINT('Ctrl Pts',(58.340281980589,-1.2199202386454,60.0995982247504));
#155296=CARTESIAN_POINT('Ctrl Pts',(58.3540988771689,-1.42773630835026,
60.1115211983213));
#155297=CARTESIAN_POINT('Ctrl Pts',(58.3716517175546,-1.63795850118814,
60.1264839986969));
#155298=CARTESIAN_POINT('Ctrl Pts',(58.393221283897,-1.85039632962378,60.1446146025748));
#155299=CARTESIAN_POINT('Ctrl Pts',(58.4065868933095,-1.98203370212521,
60.1558492544912));
#155300=CARTESIAN_POINT('Ctrl Pts',(58.4214947794622,-2.11452173605364,
60.1683011786858));
#155301=CARTESIAN_POINT('Ctrl Pts',(58.4380143589673,-2.24781785929611,
60.1820103398356));
#155302=CARTESIAN_POINT('Ctrl Pts',(58.4404138660129,-2.26717942880672,
60.1840016271295));
#155303=CARTESIAN_POINT('Ctrl Pts',(58.4428473830314,-2.28655805460061,
60.1860194527049));
#155304=CARTESIAN_POINT('Ctrl Pts',(58.4453151528025,-2.3059535689316,60.1880639619441));
#155305=CARTESIAN_POINT('Ctrl Pts',(58.4690615709735,-2.49258929132516,
60.2077375035832));
#155306=CARTESIAN_POINT('Ctrl Pts',(58.4960924330805,-2.68091509646556,
60.2298223783291));
#155307=CARTESIAN_POINT('Ctrl Pts',(58.5269446035756,-2.87072609599083,
60.2542598726009));
#155308=CARTESIAN_POINT('Ctrl Pts',(58.5535927944882,-3.03467306216784,
60.2753674641359));
#155309=CARTESIAN_POINT('Ctrl Pts',(58.583091938661,-3.19972753045303,60.2982306841269));
#155310=CARTESIAN_POINT('Ctrl Pts',(58.6158096951469,-3.36574064915635,
60.322826922696));
#155311=CARTESIAN_POINT('Ctrl Pts',(58.6298388921635,-3.43692617652021,
60.3333736567576));
#155312=CARTESIAN_POINT('Ctrl Pts',(58.6444601564802,-3.50828776656749,
60.3442392130297));
#155313=CARTESIAN_POINT('Ctrl Pts',(58.6596998748985,-3.57981586985723,
60.3554201094352));
#155314=CARTESIAN_POINT('Ctrl Pts',(58.6965915521465,-3.7529681308318,60.3824863589691));
#155315=CARTESIAN_POINT('Ctrl Pts',(58.7371370372468,-3.92707067059017,
60.4113704999466));
#155316=CARTESIAN_POINT('Ctrl Pts',(58.7819106933059,-4.10185860030788,
60.4418732050604));
#155317=CARTESIAN_POINT('Ctrl Pts',(58.7929214942294,-4.14484269558513,
60.4493744735115));
#155318=CARTESIAN_POINT('Ctrl Pts',(58.8041881504347,-4.187868046168,60.4569736423612));
#155319=CARTESIAN_POINT('Ctrl Pts',(58.8157195053545,-4.23093031976178,
60.4646677664296));
#155320=CARTESIAN_POINT('Ctrl Pts',(58.836795293484,-4.30963497857667,60.4787302707785));
#155321=CARTESIAN_POINT('Ctrl Pts',(58.8587520838187,-4.38846373130315,
60.493112292388));
#155322=CARTESIAN_POINT('Ctrl Pts',(58.8816491331759,-4.46737832075861,
60.5077891134032));
#155323=CARTESIAN_POINT('Ctrl Pts',(58.8904872180244,-4.49783874500423,
60.5134542533702));
#155324=CARTESIAN_POINT('Ctrl Pts',(58.8994653992315,-4.52831193526029,
60.519163314747));
#155325=CARTESIAN_POINT('Ctrl Pts',(58.9085869514967,-4.55879700219545,
60.5249146864526));
#155326=CARTESIAN_POINT('Ctrl Pts',(58.9249634454014,-4.61352875160944,
60.5352404841831));
#155327=CARTESIAN_POINT('Ctrl Pts',(58.9418038125052,-4.6682965230225,60.5457007137537));
#155328=CARTESIAN_POINT('Ctrl Pts',(58.9591302413778,-4.72308788085057,
60.5562809970971));
#155329=CARTESIAN_POINT('Ctrl Pts',(58.9677934558141,-4.75048355976461,
60.5615711387687));
#155330=CARTESIAN_POINT('Ctrl Pts',(58.9765781842021,-4.77788513687593,
60.5668912911526));
#155331=CARTESIAN_POINT('Ctrl Pts',(58.9854871327347,-4.80529091555044,
60.5722396150746));
#155332=CARTESIAN_POINT('Ctrl Pts',(58.9899416070011,-4.81899380488769,
60.5749137770356));
#155333=CARTESIAN_POINT('Ctrl Pts',(58.9944271361751,-4.83269774470628,
60.5775949816723));
#155334=CARTESIAN_POINT('Ctrl Pts',(58.9989440554225,-4.84640251863526,
60.5802829973539));
#155335=CARTESIAN_POINT('Ctrl Pts',(59.0012025150462,-4.85325490559974,
60.5816270051946));
#155336=CARTESIAN_POINT('Ctrl Pts',(59.0034688221802,-4.86010750109739,
60.5829727157835));
#155337=CARTESIAN_POINT('Ctrl Pts',(59.0057430184444,-4.86696027757705,
60.5843201000103));
#155338=CARTESIAN_POINT('Ctrl Pts',(59.0068801165765,-4.87038666581687,
60.5849937921237));
#155339=CARTESIAN_POINT('Ctrl Pts',(59.0080191869907,-4.87381309930254,
60.5856679026457));
#155340=CARTESIAN_POINT('Ctrl Pts',(59.0091602348704,-4.87723957455611,
60.5863424279278));
#155341=CARTESIAN_POINT('Ctrl Pts',(59.01030128275,-4.88066604980967,60.5870169532098));
#155342=CARTESIAN_POINT('Ctrl Pts',(59.0118496790891,-4.8853056816243,60.5879309900696));
#155343=CARTESIAN_POINT('Ctrl Pts',(59.0125893160822,-4.88751912213284,
60.5883672444004));
#155344=CARTESIAN_POINT('Ctrl Pts',(59.0466683952197,-4.98950430534963,
60.6084678424014));
#155345=CARTESIAN_POINT('Ctrl Pts',(59.084110335281,-5.09640993499694,60.6299095208549));
#155346=CARTESIAN_POINT('Ctrl Pts',(59.1255979348175,-5.20796002104424,
60.6526112582718));
#155347=CARTESIAN_POINT('Ctrl Pts',(59.165827699191,-5.3161280936172,60.6746247166873));
#155348=CARTESIAN_POINT('Ctrl Pts',(59.2098617926801,-5.42866360276206,
60.6978233217053));
#155349=CARTESIAN_POINT('Ctrl Pts',(59.2583639538129,-5.54529390482577,
60.7221259849945));
#155350=CARTESIAN_POINT('Ctrl Pts',(59.2987976607154,-5.6425224682432,60.7423858402553));
#155351=CARTESIAN_POINT('Ctrl Pts',(59.3423371250503,-5.74259666554944,
60.7634127529908));
#155352=CARTESIAN_POINT('Ctrl Pts',(59.3893976796749,-5.84533900592405,
60.7851613181427));
#155353=CARTESIAN_POINT('Ctrl Pts',(59.4334172168723,-5.9414422140131,60.8055045074726));
#155354=CARTESIAN_POINT('Ctrl Pts',(59.4805056426105,-6.03988847527971,
60.826490027304));
#155355=CARTESIAN_POINT('Ctrl Pts',(59.5312764880216,-6.14041774579453,
60.8478786261836));
#155356=CARTESIAN_POINT('Ctrl Pts',(59.5737720098771,-6.22456138724261,
60.8657810200434));
#155357=CARTESIAN_POINT('Ctrl Pts',(59.6188477085341,-6.3101637636052,60.883965731171));
#155358=CARTESIAN_POINT('Ctrl Pts',(59.666867193762,-6.39704577233237,60.9022838917411));
#155359=CARTESIAN_POINT('Ctrl Pts',(59.7022865976223,-6.46113036092596,
60.9157954553103));
#155360=CARTESIAN_POINT('Ctrl Pts',(59.7393264044079,-6.52590512609024,
60.9293660785788));
#155361=CARTESIAN_POINT('Ctrl Pts',(59.7781648402363,-6.59126771537316,
60.9429035856504));
#155362=CARTESIAN_POINT('Ctrl Pts',(59.7971080468353,-6.62314791358959,
60.9495064209042));
#155363=CARTESIAN_POINT('Ctrl Pts',(59.8164791148336,-6.65516778169856,
60.9561013135051));
#155364=CARTESIAN_POINT('Ctrl Pts',(59.8362984871501,-6.68731447842764,
60.9626770974503));
#155365=CARTESIAN_POINT('Ctrl Pts',(59.8665255735293,-6.73634231661122,
60.9727060118956));
#155366=CARTESIAN_POINT('Ctrl Pts',(59.8977906010286,-6.78566703466396,
60.9826941806909));
#155367=CARTESIAN_POINT('Ctrl Pts',(59.930185682024,-6.83522716113299,60.9925823374755));
#155368=CARTESIAN_POINT('Ctrl Pts',(59.9517635487066,-6.86823840138494,
60.9991686870779));
#155369=CARTESIAN_POINT('Ctrl Pts',(59.973545298576,-6.90091096020029,61.0056234497311));
#155370=CARTESIAN_POINT('Ctrl Pts',(59.9961709624893,-6.93410116671089,
61.012085605819));
#155371=CARTESIAN_POINT('Ctrl Pts',(60.0075134487101,-6.95073977061893,
61.0153251534701));
#155372=CARTESIAN_POINT('Ctrl Pts',(60.0190687714284,-6.96750821772436,
61.0185665818014));
#155373=CARTESIAN_POINT('Ctrl Pts',(60.0309222556114,-6.98451278948907,
61.0218275075584));
#155374=CARTESIAN_POINT('Ctrl Pts',(60.0795079257767,-7.05421200216824,
61.0351935576426));
#155375=CARTESIAN_POINT('Ctrl Pts',(60.1269746556736,-7.11911555985469,
61.0472183111237));
#155376=CARTESIAN_POINT('Ctrl Pts',(60.1728493085623,-7.17939944829445,
61.0579965072052));
#155377=CARTESIAN_POINT('Ctrl Pts',(60.2188885679778,-7.23989964619653,
61.0688133773978));
#155378=CARTESIAN_POINT('Ctrl Pts',(60.2633242216992,-7.29574725332997,
61.0783747962133));
#155379=CARTESIAN_POINT('Ctrl Pts',(60.3057283855415,-7.34712996019628,
61.0867886051467));
#155380=CARTESIAN_POINT('Ctrl Pts',(60.3445567285779,-7.39417971162545,
61.0944929018456));
#155381=CARTESIAN_POINT('Ctrl Pts',(60.3816823380303,-7.43748612756068,
61.1012351771947));
#155382=CARTESIAN_POINT('Ctrl Pts',(60.4168140181179,-7.47719724058691,
61.1071061410174));
#155383=CARTESIAN_POINT('Ctrl Pts',(60.4552298300096,-7.52062057372167,
61.1135259262732));
#155384=CARTESIAN_POINT('Ctrl Pts',(60.4912460540125,-7.55971785059863,
61.1188948231495));
#155385=CARTESIAN_POINT('Ctrl Pts',(60.5244579042493,-7.59471761046306,
61.1233979425645));
#155386=CARTESIAN_POINT('Ctrl Pts',(60.5395427633062,-7.61061454004744,
61.1254432643761));
#155387=CARTESIAN_POINT('Ctrl Pts',(60.5540497928784,-7.6256661838935,61.1273101159803));
#155388=CARTESIAN_POINT('Ctrl Pts',(60.5679445416861,-7.63989391794987,
61.129016460982));
#155389=CARTESIAN_POINT('Ctrl Pts',(60.590187727431,-7.66267015778862,61.1317480360066));
#155390=CARTESIAN_POINT('Ctrl Pts',(60.6108585027185,-7.68333953919245,
61.1340723320172));
#155391=CARTESIAN_POINT('Ctrl Pts',(60.6298219773043,-7.70200106833081,
61.1360750499524));
#155392=CARTESIAN_POINT('Ctrl Pts',(60.6393037145972,-7.71133183289999,
61.13707640892));
#155393=CARTESIAN_POINT('Ctrl Pts',(60.6483588771974,-7.72016062410416,
61.1379973961989));
#155394=CARTESIAN_POINT('Ctrl Pts',(60.6569723142693,-7.72849936884094,
61.1388484909094));
#155395=CARTESIAN_POINT('Ctrl Pts',(60.6612790328052,-7.73266874120932,
61.1392740382647));
#155396=CARTESIAN_POINT('Ctrl Pts',(60.6654753229127,-7.73671559834878,
61.1396821182107));
#155397=CARTESIAN_POINT('Ctrl Pts',(60.6695594308556,-7.74064136924075,
61.1400739857034));
#155398=CARTESIAN_POINT('Ctrl Pts',(60.671601484827,-7.74260425468674,61.1402699194497));
#155399=CARTESIAN_POINT('Ctrl Pts',(60.673615493437,-7.74453686835117,61.1404618004314));
#155400=CARTESIAN_POINT('Ctrl Pts',(60.6756012425935,-7.74643938498901,
61.14064978388));
#155401=CARTESIAN_POINT('Ctrl Pts',(60.6765941171717,-7.74739064330793,
61.1407437756042));
#155402=CARTESIAN_POINT('Ctrl Pts',(60.6775799268976,-7.74833437735662,
61.1408367929666));
#155403=CARTESIAN_POINT('Ctrl Pts',(60.6785586455364,-7.74927060869726,
61.1409288551345));
#155404=CARTESIAN_POINT('Ctrl Pts',(60.6790480048557,-7.74973872436758,
61.1409748862185));
#155405=CARTESIAN_POINT('Ctrl Pts',(60.6792845347018,-7.74996512345502,
61.1409972458477));
#155406=CARTESIAN_POINT('Ctrl Pts',(60.6796448082126,-7.75030958071681,
61.1410310685549));
#155407=CARTESIAN_POINT('Ctrl Pts',(60.6800050817235,-7.75065403797859,
61.1410648912622));
#155408=CARTESIAN_POINT('Ctrl Pts',(60.6804890921598,-7.75111656176834,
61.1411101639344));
#155409=CARTESIAN_POINT('Ctrl Pts',(60.6814735021436,-7.7520568160311,61.141202195187));
#155410=CARTESIAN_POINT('Ctrl Pts',(60.7528816833991,-7.82026198250822,
61.1478780563335));
#155411=CARTESIAN_POINT('Ctrl Pts',(60.8238848687323,-7.88340841251751,
61.1524435095519));
#155412=CARTESIAN_POINT('Ctrl Pts',(60.8937477621502,-7.9414195808411,61.1549060387511));
#155413=CARTESIAN_POINT('Ctrl Pts',(60.9471625836398,-7.98577297144389,
61.1567888058561));
#155414=CARTESIAN_POINT('Ctrl Pts',(60.9999109579355,-8.02712549905052,
61.1574426075799));
#155415=CARTESIAN_POINT('Ctrl Pts',(61.0516739198898,-8.06545973778738,
61.1568778797576));
#155416=CARTESIAN_POINT('Ctrl Pts',(61.1080967748886,-8.10724496629978,
61.1562623130506));
#155417=CARTESIAN_POINT('Ctrl Pts',(61.1633153009485,-8.14537779070647,
61.1541689353691));
#155418=CARTESIAN_POINT('Ctrl Pts',(61.2169696534685,-8.18019173053023,
61.1508389703513));
#155419=CARTESIAN_POINT('Ctrl Pts',(61.2718447722498,-8.2157977716684,61.1474332405771));
#155420=CARTESIAN_POINT('Ctrl Pts',(61.3250837590809,-8.24793265307407,
61.142734006002));
#155421=CARTESIAN_POINT('Ctrl Pts',(61.3763514670402,-8.27696343931164,
61.1370178861163));
#155422=CARTESIAN_POINT('Ctrl Pts',(61.3810919615122,-8.27964778560205,
61.1364893422083));
#155423=CARTESIAN_POINT('Ctrl Pts',(61.3858156359089,-8.28230559643327,
61.1359521168453));
#155424=CARTESIAN_POINT('Ctrl Pts',(61.3905222458867,-8.28493716412695,
61.1354064364425));
#155425=CARTESIAN_POINT('Ctrl Pts',(61.5360580239853,8.3650447551965,61.1180922520029));
#155426=CARTESIAN_POINT('Ctrl Pts',(61.4873816218952,8.33842428962667,61.1238514036551));
#155427=CARTESIAN_POINT('Ctrl Pts',(61.4388137622094,8.31165854192863,61.1296130433924));
#155428=CARTESIAN_POINT('Ctrl Pts',(61.3903529552591,8.28473912510079,61.1353684361582));
#155429=CARTESIAN_POINT('Ctrl Pts',(61.4825779928491,8.56882230360101,61.3353622561));
#155430=CARTESIAN_POINT('Ctrl Pts',(61.4672316263191,8.56165228818601,61.33806823458));
#155431=CARTESIAN_POINT('Ctrl Pts',(61.4152057427591,8.53728542810601,61.34724180155));
#155432=CARTESIAN_POINT('Ctrl Pts',(61.3632704362791,8.51275974164101,61.35639939733));
#155433=CARTESIAN_POINT('Ctrl Pts',(61.3266920462791,8.49538778255501,61.3628491544));
#155434=CARTESIAN_POINT('Ctrl Pts',(61.5613777885692,8.23803123183401,60.90576138986));
#155435=CARTESIAN_POINT('Ctrl Pts',(61.5462338697091,8.23095580226301,60.90843167135));
#155436=CARTESIAN_POINT('Ctrl Pts',(61.4948919947391,8.20690930668701,60.91748462915));
#155437=CARTESIAN_POINT('Ctrl Pts',(61.4436315449591,8.18270232868401,60.92652322949));
#155438=CARTESIAN_POINT('Ctrl Pts',(61.4075243290991,8.16555414216201,60.9328899058401));
#155439=CARTESIAN_POINT('Ctrl Pts',(61.7453363893891,7.76575783100901,60.69766018174));
#155440=CARTESIAN_POINT('Ctrl Pts',(61.7304815069191,7.75881744250201,60.70027949832));
#155441=CARTESIAN_POINT('Ctrl Pts',(61.6801161971691,7.73522833422001,60.70916026132));
#155442=CARTESIAN_POINT('Ctrl Pts',(61.629819246419,7.71147637916701,60.71802897078));
#155443=CARTESIAN_POINT('Ctrl Pts',(61.5943847301191,7.69464767475702,60.72427703205));
#155444=CARTESIAN_POINT('Ctrl Pts',(61.9853446639591,7.27807903569201,60.76661281361));
#155445=CARTESIAN_POINT('Ctrl Pts',(61.9707882461391,7.27127809324201,60.76917950281));
#155446=CARTESIAN_POINT('Ctrl Pts',(61.9214313568291,7.24816129207001,60.77788245408));
#155447=CARTESIAN_POINT('Ctrl Pts',(61.8721293341091,7.22487920265801,60.78657573089));
#155448=CARTESIAN_POINT('Ctrl Pts',(61.8373894605991,7.20838040175501,60.79270130789));
#155449=CARTESIAN_POINT('Ctrl Pts',(61.3903603269491,8.28472891518701,61.13538275197));
#155450=CARTESIAN_POINT('Ctrl Pts',(61.4655545379308,8.04965156496637,60.9289822447848));
#155451=CARTESIAN_POINT('Ctrl Pts',(61.5757173213241,7.77270711240031,60.8080469803564));
#155452=CARTESIAN_POINT('Ctrl Pts',(61.7095796149691,7.48128536884801,60.78445823578));
#155453=CARTESIAN_POINT('Ctrl Pts',(61.536589981978,8.36429305416126,61.1191117063875));
#155454=CARTESIAN_POINT('Ctrl Pts',(61.5728698807379,8.24718616881929,61.0162396390448));
#155455=CARTESIAN_POINT('Ctrl Pts',(61.6197151052205,8.11435345893999,60.9298413020711));
#155456=CARTESIAN_POINT('Ctrl Pts',(61.7286246545714,7.83494047062615,60.8068890704171));
#155457=CARTESIAN_POINT('Ctrl Pts',(61.79052732657,7.68874228281837,60.7704317967065));
#155458=CARTESIAN_POINT('Ctrl Pts',(61.8548446843791,7.54727709634001,60.75884806608));
#155459=CARTESIAN_POINT('Ctrl Pts',(64.5445770840491,9.98588384555501,60.99915285191));
#155460=CARTESIAN_POINT('Ctrl Pts',(64.1994083728391,9.86085233672401,61.06001540859));
#155461=CARTESIAN_POINT('Ctrl Pts',(63.4820912895591,9.587604127095,61.18649776409));
#155462=CARTESIAN_POINT('Ctrl Pts',(62.4046333853091,9.13665291821101,61.37648266319));
#155463=CARTESIAN_POINT('Ctrl Pts',(61.6766080692791,8.80504019941101,61.50485316905));
#155464=CARTESIAN_POINT('Ctrl Pts',(61.3149677140191,8.63437250107801,61.56862012099));
#155465=CARTESIAN_POINT('Ctrl Pts',(64.5630006955291,9.66255945666802,60.43942959882));
#155466=CARTESIAN_POINT('Ctrl Pts',(64.2212742212191,9.53877485330901,60.4996851962601));
#155467=CARTESIAN_POINT('Ctrl Pts',(63.5109376432391,9.26818929731802,60.6249367003401));
#155468=CARTESIAN_POINT('Ctrl Pts',(62.4432659544991,8.82134180562501,60.81319602561));
#155469=CARTESIAN_POINT('Ctrl Pts',(61.7212021268391,8.49245145827502,60.94051536022));
#155470=CARTESIAN_POINT('Ctrl Pts',(61.3622879725491,8.32307031229001,61.00380160938));
#155471=CARTESIAN_POINT('Ctrl Pts',(64.7154346237891,9.10274130524401,60.15388495627));
#155472=CARTESIAN_POINT('Ctrl Pts',(64.3796681907591,8.98111564918601,60.21308963763));
#155473=CARTESIAN_POINT('Ctrl Pts',(63.6814179684591,8.71514032950402,60.33620999111));
#155474=CARTESIAN_POINT('Ctrl Pts',(62.6306905662491,8.27539819531201,60.52148158149));
#155475=CARTESIAN_POINT('Ctrl Pts',(61.9189487232691,7.95122148233401,60.6469808717));
#155476=CARTESIAN_POINT('Ctrl Pts',(61.5647548339591,7.78406793000301,60.70943481079));
#155477=CARTESIAN_POINT('Ctrl Pts',(64.9475416382091,8.50598449258701,60.24430535246));
#155478=CARTESIAN_POINT('Ctrl Pts',(64.6181285097791,8.38666023834401,60.3023897748));
#155479=CARTESIAN_POINT('Ctrl Pts',(63.9327621410791,8.12559935367801,60.42323835727));
#155480=CARTESIAN_POINT('Ctrl Pts',(62.9000970656791,7.69343141207701,60.6053250721));
#155481=CARTESIAN_POINT('Ctrl Pts',(62.1993582862391,7.37427935472601,60.72888422534));
#155482=CARTESIAN_POINT('Ctrl Pts',(61.8501961206591,7.20950038007601,60.79045093578));
#155483=CARTESIAN_POINT('',(64.4193726617333,9.7592596408602,60.7791711866962));
#155484=CARTESIAN_POINT('Origin',(64.963170393819,8.73683398597385,61.7327853056315));
#155485=CARTESIAN_POINT('Ctrl Pts',(64.4195454322906,9.75893531368795,60.7794745133828));
#155486=CARTESIAN_POINT('Ctrl Pts',(64.1788703740164,9.6579680563156,60.8084988936834));
#155487=CARTESIAN_POINT('Ctrl Pts',(63.9381154510292,9.55304684809677,60.8372628737177));
#155488=CARTESIAN_POINT('Ctrl Pts',(63.697456498012,9.44426471655492,60.8658538895038));
#155489=CARTESIAN_POINT('Ctrl Pts',(63.4577439202741,9.33591036348895,60.8943324730275));
#155490=CARTESIAN_POINT('Ctrl Pts',(63.2181262646531,9.22372625169533,60.9226400368081));
#155491=CARTESIAN_POINT('Ctrl Pts',(62.9787286335067,9.10780870892131,60.9508448865463));
#155492=CARTESIAN_POINT('Ctrl Pts',(62.7379133045354,8.99120470969623,60.9792167636437));
#155493=CARTESIAN_POINT('Ctrl Pts',(62.4973203663039,8.87082394515049,61.0074853213969));
#155494=CARTESIAN_POINT('Ctrl Pts',(62.2570317776485,8.7467548208856,61.0356926206112));
#155495=CARTESIAN_POINT('Ctrl Pts',(62.0298535183495,8.62945500302505,61.0623609079855));
#155496=CARTESIAN_POINT('Ctrl Pts',(61.8029467202873,8.50885904290689,61.088974601359));
#155497=CARTESIAN_POINT('Ctrl Pts',(61.5763469233615,8.38502077013121,61.1155396989721));
#155498=CARTESIAN_POINT('Ctrl Pts',(61.5632699767427,8.37787413317734,61.1170727557891));
#155499=CARTESIAN_POINT('Ctrl Pts',(61.5501940441027,8.37071669029369,61.1186056418031));
#155500=CARTESIAN_POINT('Ctrl Pts',(61.5371191292109,8.36354844880146,61.1201383548072));
#155501=CARTESIAN_POINT('Ctrl Pts',(62.7515737541991,12.07774640868,63.001901751759));
#155502=CARTESIAN_POINT('Ctrl Pts',(64.5503514671391,9.66775772102602,61.57390007131));
#155503=CARTESIAN_POINT('Ctrl Pts',(65.8339234114092,8.34497068419502,58.77515659908));
#155504=CARTESIAN_POINT('Ctrl Pts',(66.1844451731991,8.55990068685403,55.42750337263));
#155505=CARTESIAN_POINT('Ctrl Pts',(61.5063898405791,11.44707601721,62.90835246028));
#155506=CARTESIAN_POINT('Ctrl Pts',(63.5763627523891,9.04690003902301,61.51844654984));
#155507=CARTESIAN_POINT('Ctrl Pts',(65.0655865226491,7.76869735204601,58.6407671082601));
#155508=CARTESIAN_POINT('Ctrl Pts',(65.4573779299991,8.07974756896001,55.17405404619));
#155509=CARTESIAN_POINT('Ctrl Pts',(60.3778000932491,10.72664715258,62.77986335145));
#155510=CARTESIAN_POINT('Ctrl Pts',(62.7295784718991,8.36060988985802,61.4444601686601));
#155511=CARTESIAN_POINT('Ctrl Pts',(64.4134291656991,7.13761983681501,58.48792002224));
#155512=CARTESIAN_POINT('Ctrl Pts',(64.8046720640391,7.53823008741401,54.89307383022));
#155513=CARTESIAN_POINT('Ctrl Pts',(59.3595858619191,9.916504400752,62.64129573267));
#155514=CARTESIAN_POINT('Ctrl Pts',(61.9983452479491,7.63333056293401,61.37410196926));
#155515=CARTESIAN_POINT('Ctrl Pts',(63.8659652165791,6.48021923494602,58.34220507549));
#155516=CARTESIAN_POINT('Ctrl Pts',(64.2231019555691,6.94207966240701,54.6147516902));
#155517=CARTESIAN_POINT('Ctrl Pts',(62.6708095529579,11.8749837583452,62.9186045084915));
#155518=CARTESIAN_POINT('Ctrl Pts',(62.7578181479658,11.7616266579273,62.8481545770921));
#155519=CARTESIAN_POINT('Ctrl Pts',(62.8449003046356,11.6491939411928,62.7730948511703));
#155520=CARTESIAN_POINT('Ctrl Pts',(62.9318200968733,11.5380437482938,62.6933908725665));
#155521=CARTESIAN_POINT('Ctrl Pts',(63.0199125448919,11.4253940014626,62.6126115884555));
#155522=CARTESIAN_POINT('Ctrl Pts',(63.1078380140172,11.314062011975,62.5270614846297));
#155523=CARTESIAN_POINT('Ctrl Pts',(63.1953366462701,11.2044299246556,62.4367574345381));
#155524=CARTESIAN_POINT('Ctrl Pts',(63.2799927685102,11.0983593822187,62.3493870322072));
#155525=CARTESIAN_POINT('Ctrl Pts',(63.3642490279793,10.9938805260787,62.2575666328219));
#155526=CARTESIAN_POINT('Ctrl Pts',(63.4478607751725,10.8913418736331,62.1613622370055));
#155527=CARTESIAN_POINT('Ctrl Pts',(63.530982892732,10.7894036866067,62.065721213259));
#155528=CARTESIAN_POINT('Ctrl Pts',(63.6134677475192,10.6893834687848,61.9657473366532));
#155529=CARTESIAN_POINT('Ctrl Pts',(63.6950698661447,10.5916197585739,61.8615564717354));
#155530=CARTESIAN_POINT('Ctrl Pts',(63.7761228081869,10.4945139913338,61.7580668040926));
#155531=CARTESIAN_POINT('Ctrl Pts',(63.856304567228,10.3996348795351,61.6504167624718));
#155532=CARTESIAN_POINT('Ctrl Pts',(63.9353737663347,10.3073040540845,61.5387704012505));
#155533=CARTESIAN_POINT('Ctrl Pts',(63.9449132764184,10.2961645604464,61.5253005343401));
#155534=CARTESIAN_POINT('Ctrl Pts',(63.9544365943459,10.2850621426659,61.511772557708));
#155535=CARTESIAN_POINT('Ctrl Pts',(63.9639432985778,10.2739973509954,61.4981868088115));
#155536=CARTESIAN_POINT('Ctrl Pts',(64.042387156448,10.1826970513345,61.3860850194318));
#155537=CARTESIAN_POINT('Ctrl Pts',(64.1197402632482,10.0939126076095,61.2699867480628));
#155538=CARTESIAN_POINT('Ctrl Pts',(64.1957551375657,10.0079657234468,61.150117356748));
#155539=CARTESIAN_POINT('Ctrl Pts',(64.2717700118831,9.92201883928409,61.0302479654333));
#155540=CARTESIAN_POINT('Ctrl Pts',(64.3464463024524,9.83890998680352,60.9066076599331));
#155541=CARTESIAN_POINT('Ctrl Pts',(64.4195454322906,9.75893531368794,60.7794745133828));
#155542=CARTESIAN_POINT('Ctrl Pts',(84.4901667991491,11.93708079303,59.09834125997));
#155543=CARTESIAN_POINT('Ctrl Pts',(83.9147835748191,11.31851875633,58.92696924491));
#155544=CARTESIAN_POINT('Ctrl Pts',(82.8290630913291,10.28891810155,58.40666372177));
#155545=CARTESIAN_POINT('Ctrl Pts',(81.7119670519691,9.50097580768701,57.48286963236));
#155546=CARTESIAN_POINT('Ctrl Pts',(81.2581645020491,9.22984081121201,57.03752908385));
#155547=CARTESIAN_POINT('Ctrl Pts',(83.6617321185691,12.17586092735,59.3644367066));
#155548=CARTESIAN_POINT('Ctrl Pts',(83.1307067314591,11.57135929148,59.15364085641));
#155549=CARTESIAN_POINT('Ctrl Pts',(82.1344977737191,10.57540906728,58.58332876952));
#155550=CARTESIAN_POINT('Ctrl Pts',(81.1085173115291,9.81898400595401,57.65781121812));
#155551=CARTESIAN_POINT('Ctrl Pts',(80.6895279691791,9.55843631046701,57.21938802614));
#155552=CARTESIAN_POINT('Ctrl Pts',(82.0144069406191,12.57231964261,59.89501020394));
#155553=CARTESIAN_POINT('Ctrl Pts',(81.5669966029291,12.00452484203,59.62213429887));
#155554=CARTESIAN_POINT('Ctrl Pts',(80.7361758999491,11.08327377401,58.97893486564));
#155555=CARTESIAN_POINT('Ctrl Pts',(79.8788943064191,10.38652959513,58.05985965617));
#155556=CARTESIAN_POINT('Ctrl Pts',(79.5256597583991,10.1446658366,57.63620001424));
#155557=CARTESIAN_POINT('Ctrl Pts',(79.7945501172291,12.9266341776,60.56116805791));
#155558=CARTESIAN_POINT('Ctrl Pts',(79.4523719769991,12.40990839757,60.23657063794));
#155559=CARTESIAN_POINT('Ctrl Pts',(78.8208983604991,11.57901923841,59.53893424688));
#155560=CARTESIAN_POINT('Ctrl Pts',(78.1654256105091,10.94422155279,58.63373828109));
#155561=CARTESIAN_POINT('Ctrl Pts',(77.8929235677491,10.7202982577,58.22585805));
#155562=CARTESIAN_POINT('Ctrl Pts',(77.9640422107791,13.12680188932,61.05599713268));
#155563=CARTESIAN_POINT('Ctrl Pts',(77.7041168382291,12.64242377406,60.70217368394));
#155564=CARTESIAN_POINT('Ctrl Pts',(77.2248237057191,11.86642305288,59.97395619231));
#155565=CARTESIAN_POINT('Ctrl Pts',(76.7232189414891,11.26765541666,59.07462987159));
#155566=CARTESIAN_POINT('Ctrl Pts',(76.5132178516091,11.05395427136,58.67443825277));
#155567=CARTESIAN_POINT('Ctrl Pts',(76.5484058674291,13.23564492474,61.40514351714));
#155568=CARTESIAN_POINT('Ctrl Pts',(76.3506939226291,12.77022591026,61.03351673584));
#155569=CARTESIAN_POINT('Ctrl Pts',(75.9846773751891,12.02566337689,60.28544751858));
#155570=CARTESIAN_POINT('Ctrl Pts',(75.5969071603691,11.44700487058,59.38566747742));
#155571=CARTESIAN_POINT('Ctrl Pts',(75.4334154616191,11.23893043935,58.98806501362));
#155572=CARTESIAN_POINT('Ctrl Pts',(75.0966676773891,13.30237781364,61.72591085587));
#155573=CARTESIAN_POINT('Ctrl Pts',(74.9621214288391,12.84950608055,61.33981339755));
#155574=CARTESIAN_POINT('Ctrl Pts',(74.7094237279791,12.12535075536,60.57331429327));
#155575=CARTESIAN_POINT('Ctrl Pts',(74.4343965495091,11.55943344353,59.66681793516));
#155576=CARTESIAN_POINT('Ctrl Pts',(74.3170517761591,11.35486892705,59.26810663539));
#155577=CARTESIAN_POINT('Ctrl Pts',(73.6116764726791,13.32524436449,62.01148422652));
#155578=CARTESIAN_POINT('Ctrl Pts',(73.5411274561791,12.87708681798,61.61332948466));
#155579=CARTESIAN_POINT('Ctrl Pts',(73.4020349067191,12.16047212512,60.82794870269));
#155580=CARTESIAN_POINT('Ctrl Pts',(73.2389962138791,11.59914480222,59.90671015597));
#155581=CARTESIAN_POINT('Ctrl Pts',(73.1674788426691,11.39581940583,59.50250721111));
#155582=CARTESIAN_POINT('Ctrl Pts',(72.1188799015491,13.30289486689,62.25146683139));
#155583=CARTESIAN_POINT('Ctrl Pts',(72.1125583805291,12.85011658359,61.84273092877));
#155584=CARTESIAN_POINT('Ctrl Pts',(72.0866318414391,12.12611361488,61.03625300543));
#155585=CARTESIAN_POINT('Ctrl Pts',(72.0338540971691,11.56029225914,60.09066585512));
#155586=CARTESIAN_POINT('Ctrl Pts',(72.0072775324691,11.35575444167,59.67600260266));
#155587=CARTESIAN_POINT('Ctrl Pts',(70.6447970428891,13.23668446295,62.44705203254));
#155588=CARTESIAN_POINT('Ctrl Pts',(70.7027629578791,12.77144316539,62.03027350808));
#155589=CARTESIAN_POINT('Ctrl Pts',(70.7896012143391,12.0271746967,61.20234985571));
#155590=CARTESIAN_POINT('Ctrl Pts',(70.8450707564591,11.4487047659,60.22459753681));
#155591=CARTESIAN_POINT('Ctrl Pts',(70.8622468154291,11.24068339608,59.79523992369));
#155592=CARTESIAN_POINT('Ctrl Pts',(69.1938422725591,13.12817992329,62.60363053547));
#155593=CARTESIAN_POINT('Ctrl Pts',(69.3164050956391,12.64403066823,62.18226630755));
#155594=CARTESIAN_POINT('Ctrl Pts',(69.5165533775491,11.86841436887,61.3342268008));
#155595=CARTESIAN_POINT('Ctrl Pts',(69.6792300687291,11.26989645149,60.31800299092));
#155596=CARTESIAN_POINT('Ctrl Pts',(69.7392629655691,11.05626582625,59.87032822369));
#155597=CARTESIAN_POINT('Ctrl Pts',(67.2987925196791,12.9278854165,62.76551241559));
#155598=CARTESIAN_POINT('Ctrl Pts',(67.5088893277491,12.41134714893,62.34342713161));
#155599=CARTESIAN_POINT('Ctrl Pts',(67.8629193001691,11.58078531893,61.47196925136));
#155600=CARTESIAN_POINT('Ctrl Pts',(68.1685781880491,10.94620890791,60.39748653351));
#155601=CARTESIAN_POINT('Ctrl Pts',(68.2848774985691,10.72234926957,59.92116013881));
#155602=CARTESIAN_POINT('Ctrl Pts',(64.9776135133791,12.57277215386,62.89933853185));
#155603=CARTESIAN_POINT('Ctrl Pts',(65.3046216182191,12.00502373315,62.48986053372));
#155604=CARTESIAN_POINT('Ctrl Pts',(65.8651825116391,11.08386469307,61.60127612814));
#155605=CARTESIAN_POINT('Ctrl Pts',(66.3562770791491,10.3871904121,60.44448875357));
#155606=CARTESIAN_POINT('Ctrl Pts',(66.5432577288191,10.14534757908,59.92560503161));
#155607=CARTESIAN_POINT('Ctrl Pts',(63.2468791157191,12.17590577892,62.96414316285));
#155608=CARTESIAN_POINT('Ctrl Pts',(63.6737672946891,11.57140227548,62.58443568663));
#155609=CARTESIAN_POINT('Ctrl Pts',(64.4148112944791,10.57545021812,61.70779142165));
#155610=CARTESIAN_POINT('Ctrl Pts',(65.0623489581691,9.81902510121501,60.48718610584));
#155611=CARTESIAN_POINT('Ctrl Pts',(65.3061124827291,9.55847754437801,59.93190217482));
#155612=CARTESIAN_POINT('Ctrl Pts',(62.3770790606791,11.93704232306,62.997456388872));
#155613=CARTESIAN_POINT('Ctrl Pts',(62.8591600596191,11.3184788717,62.63962976268));
#155614=CARTESIAN_POINT('Ctrl Pts',(63.7014671428791,10.28887446589,61.77936646535));
#155615=CARTESIAN_POINT('Ctrl Pts',(64.4352534501791,9.50092849403001,60.52921035483));
#155616=CARTESIAN_POINT('Ctrl Pts',(64.7093784324491,9.22979226124701,59.95551485634));
#155617=CARTESIAN_POINT('',(81.8125288217999,9.75922027029902,57.7122994775726));
#155618=CARTESIAN_POINT('Ctrl Pts',(81.8125638933902,9.75941427559586,57.7120937184908));
#155619=CARTESIAN_POINT('Ctrl Pts',(81.6439092695413,9.83352396075257,57.7531647795599));
#155620=CARTESIAN_POINT('Ctrl Pts',(81.4758410035563,9.90338403709679,57.7939788425709));
#155621=CARTESIAN_POINT('Ctrl Pts',(81.3085563965148,9.96953432483138,57.8344710069339));
#155622=CARTESIAN_POINT('Ctrl Pts',(81.1350609420459,10.0381406026996,57.876466541268));
#155623=CARTESIAN_POINT('Ctrl Pts',(80.9624080034726,10.1027570084598,57.9181158985582));
#155624=CARTESIAN_POINT('Ctrl Pts',(80.7907683120586,10.16396002248,57.9593597431247));
#155625=CARTESIAN_POINT('Ctrl Pts',(80.6363540335763,10.2190208255672,57.9964644387118));
#155626=CARTESIAN_POINT('Ctrl Pts',(80.4827588716633,10.2713187822153,58.0332411691658));
#155627=CARTESIAN_POINT('Ctrl Pts',(80.3300792674316,10.3212522825865,58.0696544850922));
#155628=CARTESIAN_POINT('Ctrl Pts',(80.1076282946657,10.3940043426084,58.1227079206851));
#155629=CARTESIAN_POINT('Ctrl Pts',(79.8871203429479,10.4617356301858,58.1749895696072));
#155630=CARTESIAN_POINT('Ctrl Pts',(79.6686891674991,10.5249660905481,58.2264280517326));
#155631=CARTESIAN_POINT('Ctrl Pts',(79.6236763044412,10.5379962088338,58.2370281565348));
#155632=CARTESIAN_POINT('Ctrl Pts',(79.5787514980179,10.5508350969496,58.2475925140022));
#155633=CARTESIAN_POINT('Ctrl Pts',(79.5339157184396,10.5634871501206,58.2581205875384));
#155634=CARTESIAN_POINT('Ctrl Pts',(79.3054702511054,10.6279513844124,58.3117628059123));
#155635=CARTESIAN_POINT('Ctrl Pts',(79.0793396002763,10.6875671033886,58.3644602054702));
#155636=CARTESIAN_POINT('Ctrl Pts',(78.8556312477068,10.7428916622159,58.4161506350891));
#155637=CARTESIAN_POINT('Ctrl Pts',(78.6974177155852,10.782018917701,58.452707720924));
#155638=CARTESIAN_POINT('Ctrl Pts',(78.5404149375569,10.8189990491118,58.4887615270575));
#155639=CARTESIAN_POINT('Ctrl Pts',(78.384652376787,10.8540168851848,58.5242945022815));
#155640=CARTESIAN_POINT('Ctrl Pts',(78.1161060568885,10.9143902570768,58.5855560126488));
#155641=CARTESIAN_POINT('Ctrl Pts',(77.8512481119559,10.9689305735653,58.6452681998748));
#155642=CARTESIAN_POINT('Ctrl Pts',(77.5902789029177,11.0181836520086,58.7033465791699));
#155643=CARTESIAN_POINT('Ctrl Pts',(77.3203166773425,11.0691339948555,58.7634263433308));
#155644=CARTESIAN_POINT('Ctrl Pts',(77.0545153684036,11.1144268661446,58.8217580301841));
#155645=CARTESIAN_POINT('Ctrl Pts',(76.7930581821983,11.1546321196916,58.8782711045304));
#155646=CARTESIAN_POINT('Ctrl Pts',(76.5829449901012,11.1869420144183,58.9236863505921));
#155647=CARTESIAN_POINT('Ctrl Pts',(76.3756364373161,11.21596562502,58.9679276240705));
#155648=CARTESIAN_POINT('Ctrl Pts',(76.1712133147876,11.2419809454017,59.0109667460181));
#155649=CARTESIAN_POINT('Ctrl Pts',(75.8815787661272,11.2788404527011,59.0719462306568));
#155650=CARTESIAN_POINT('Ctrl Pts',(75.59773925635,11.3096601531848,59.1305115677576));
#155651=CARTESIAN_POINT('Ctrl Pts',(75.3199685850635,11.3350228954986,59.1865883387752));
#155652=CARTESIAN_POINT('Ctrl Pts',(75.0421979137771,11.3603856378124,59.2426651097928));
#155653=CARTESIAN_POINT('Ctrl Pts',(74.7704955719418,11.3802917690579,59.2962536749412));
#155654=CARTESIAN_POINT('Ctrl Pts',(74.5050850915348,11.3952985645584,59.3472999044669));
#155655=CARTESIAN_POINT('Ctrl Pts',(74.3558761444026,11.4037351121771,59.3759971667262));
#155656=CARTESIAN_POINT('Ctrl Pts',(74.2086548676872,11.4106227413642,59.4038912591849));
#155657=CARTESIAN_POINT('Ctrl Pts',(74.0634548838674,11.4160563271302,59.4309748116691));
#155658=CARTESIAN_POINT('Ctrl Pts',(73.9908548919575,11.4187731200132,59.4445165879112));
#155659=CARTESIAN_POINT('Ctrl Pts',(73.9187602260095,11.4211263570358,59.4578557522274));
#155660=CARTESIAN_POINT('Ctrl Pts',(73.8471746436691,11.4231275886736,59.4709915147018));
#155661=CARTESIAN_POINT('Ctrl Pts',(73.8113818524989,11.4241282044924,59.477559395939));
#155662=CARTESIAN_POINT('Ctrl Pts',(73.7757163323885,11.4250408160184,59.4840764282361));
#155663=CARTESIAN_POINT('Ctrl Pts',(73.7401785436256,11.4258668478509,59.4905425203682));
#155664=CARTESIAN_POINT('Ctrl Pts',(73.7224096492442,11.4262798637672,59.4937755664343));
#155665=CARTESIAN_POINT('Ctrl Pts',(73.7046726877126,11.4266712345755,59.496995877553));
#155666=CARTESIAN_POINT('Ctrl Pts',(73.6869677151652,11.4270411370982,59.5002034428149));
#155667=CARTESIAN_POINT('Ctrl Pts',(73.6781152288915,11.4272260883595,59.5018072254458));
#155668=CARTESIAN_POINT('Ctrl Pts',(73.6692707398647,11.4274056725378,59.5034078216184));
#155669=CARTESIAN_POINT('Ctrl Pts',(73.6604342550126,11.4275799116558,59.5050052299982));
#155670=CARTESIAN_POINT('Ctrl Pts',(73.6569248990391,11.427649109657,59.5056396309771));
#155671=CARTESIAN_POINT('Ctrl Pts',(73.6536221489607,11.427713488097,59.5062364894203));
#155672=CARTESIAN_POINT('Ctrl Pts',(73.6502813551559,11.4277778705353,59.5068399351009));
#155673=CARTESIAN_POINT('Ctrl Pts',(73.6452101001197,11.4278756017284,59.5077559530074));
#155674=CARTESIAN_POINT('Ctrl Pts',(73.6400511856228,11.4279734504925,59.5086871490538));
#155675=CARTESIAN_POINT('Ctrl Pts',(73.6339488202455,11.4280866170063,59.5097878903822));
#155676=CARTESIAN_POINT('Ctrl Pts',(73.37269285973,11.4329315295009,59.5569130976182));
#155677=CARTESIAN_POINT('Ctrl Pts',(73.1057310345403,11.4334108565222,59.6036608241303));
#155678=CARTESIAN_POINT('Ctrl Pts',(72.8332623814959,11.4291105690191,59.6499966677035));
#155679=CARTESIAN_POINT('Ctrl Pts',(72.5643617687005,11.424866594779,59.6957257326511));
#155680=CARTESIAN_POINT('Ctrl Pts',(72.2900973328511,11.4159671805462,59.7410536382019));
#155681=CARTESIAN_POINT('Ctrl Pts',(72.0107020881292,11.401986105176,59.785945913169));
#155682=CARTESIAN_POINT('Ctrl Pts',(71.7361080183772,11.3882452829611,59.8300667517177));
#155683=CARTESIAN_POINT('Ctrl Pts',(71.4565577601902,11.3695957390455,59.8737667243901));
#155684=CARTESIAN_POINT('Ctrl Pts',(71.1723165576537,11.3456083098175,59.9170122883105));
#155685=CARTESIAN_POINT('Ctrl Pts',(71.071551075223,11.3371045993883,59.9323431413767));
#155686=CARTESIAN_POINT('Ctrl Pts',(70.9701964803605,11.3279298363987,59.9476168852996));
#155687=CARTESIAN_POINT('Ctrl Pts',(70.8682660213638,11.3180642193791,59.9628320401611));
#155688=CARTESIAN_POINT('Ctrl Pts',(70.5736199088582,11.2895460930907,60.0068138516356));
#155689=CARTESIAN_POINT('Ctrl Pts',(70.2741594485926,11.2552578328754,60.0503055208331));
#155690=CARTESIAN_POINT('Ctrl Pts',(69.9700900940868,11.2146418474901,60.0932999798448));
#155691=CARTESIAN_POINT('Ctrl Pts',(69.6814145157921,11.1760820817808,60.1341178068791));
#155692=CARTESIAN_POINT('Ctrl Pts',(69.3885844713174,11.1318185857853,60.1744873762341));
#155693=CARTESIAN_POINT('Ctrl Pts',(69.0918121909477,11.0813480683395,60.2144100787492));
#155694=CARTESIAN_POINT('Ctrl Pts',(68.8359392920326,11.0378330958746,60.2488308730779));
#155695=CARTESIAN_POINT('Ctrl Pts',(68.5771361023818,10.98970350295,60.2829195155496));
#155696=CARTESIAN_POINT('Ctrl Pts',(68.31556650976,10.9366239300422,60.3166828761457));
#155697=CARTESIAN_POINT('Ctrl Pts',(68.070794472209,10.886953037173,60.3482780110574));
#155698=CARTESIAN_POINT('Ctrl Pts',(67.8235995869013,10.83294997116,60.3795883191861));
#155699=CARTESIAN_POINT('Ctrl Pts',(67.5740910332913,10.7740690469024,60.4106341420548));
#155700=CARTESIAN_POINT('Ctrl Pts',(67.368988937872,10.7256674960509,60.4361545630275));
#155701=CARTESIAN_POINT('Ctrl Pts',(67.1623236686854,10.6739690496663,60.4614963651982));
#155702=CARTESIAN_POINT('Ctrl Pts',(66.9541747351594,10.6186522329261,60.4866736678413));
#155703=CARTESIAN_POINT('Ctrl Pts',(66.7160785369694,10.5553767525348,60.5154733351682));
#155704=CARTESIAN_POINT('Ctrl Pts',(66.4760408660556,10.4873682802982,60.5440587719272));
#155705=CARTESIAN_POINT('Ctrl Pts',(66.2342168073654,10.4141216201386,60.5724541257979));
#155706=CARTESIAN_POINT('Ctrl Pts',(66.1921685668518,10.4013855292803,60.5773914950386));
#155707=CARTESIAN_POINT('Ctrl Pts',(66.1500664311417,10.388491012227,60.5823231272746));
#155708=CARTESIAN_POINT('Ctrl Pts',(66.1079113675261,10.3754353472268,60.5872491617598));
#155709=CARTESIAN_POINT('Ctrl Pts',(65.922908563467,10.3181389176469,60.6088676842928));
#155710=CARTESIAN_POINT('Ctrl Pts',(65.7368830571003,10.2577411616242,60.6303785991209));
#155711=CARTESIAN_POINT('Ctrl Pts',(65.5499853458738,10.1936438301779,60.6517844360448));
#155712=CARTESIAN_POINT('Ctrl Pts',(65.3630079214085,10.1295191607516,60.6731994027144));
#155713=CARTESIAN_POINT('Ctrl Pts',(65.1751567898374,10.0616913764202,60.694509302885));
#155714=CARTESIAN_POINT('Ctrl Pts',(64.9866299076625,9.98953569199477,60.715713410289));
#155715=CARTESIAN_POINT('Ctrl Pts',(64.8105237072252,9.9221338271916,60.7355205314035));
#155716=CARTESIAN_POINT('Ctrl Pts',(64.6338277155173,9.85095498689637,60.7552353944469));
#155717=CARTESIAN_POINT('Ctrl Pts',(64.4567500380413,9.77547459984062,60.77485352459));
#155718=CARTESIAN_POINT('Ctrl Pts',(64.4442608385168,9.77015100610725,60.7762371814414));
#155719=CARTESIAN_POINT('Ctrl Pts',(64.4317697614463,9.76480600997884,60.7776203551962));
#155720=CARTESIAN_POINT('Ctrl Pts',(64.4192768896971,9.75943942539138,60.7790030433804));
#155721=CARTESIAN_POINT('',(82.3525679182791,10.16626321309,58.13646557658));
#155722=CARTESIAN_POINT('Origin',(81.9836889860522,12.2828710982502,54.5138910326886));
#155723=CARTESIAN_POINT('Ctrl Pts',(82.3362552021099,12.3439667359304,59.7078933720934));
#155724=CARTESIAN_POINT('Ctrl Pts',(82.3367845506579,12.2021321891277,59.6209578472421));
#155725=CARTESIAN_POINT('Ctrl Pts',(82.3372717809877,12.0612843448791,59.5313433954501));
#155726=CARTESIAN_POINT('Ctrl Pts',(82.337812429342,11.9214102682619,59.439326167785));
#155727=CARTESIAN_POINT('Ctrl Pts',(82.3383767331593,11.7754161581178,59.3432828294067));
#155728=CARTESIAN_POINT('Ctrl Pts',(82.3389990879528,11.6304827840835,59.2446219115626));
#155729=CARTESIAN_POINT('Ctrl Pts',(82.3397609195431,11.4865638643117,59.1436177040391));
#155730=CARTESIAN_POINT('Ctrl Pts',(82.3405408397536,11.3392277920845,59.040215293581));
#155731=CARTESIAN_POINT('Ctrl Pts',(82.3414666358905,11.1929548302125,58.934356881012));
#155732=CARTESIAN_POINT('Ctrl Pts',(82.3426013441794,11.0476647255788,58.8262966308537));
#155733=CARTESIAN_POINT('Ctrl Pts',(82.3437673590602,10.8983660682135,58.7152549993272));
#155734=CARTESIAN_POINT('Ctrl Pts',(82.3451535991453,10.7501054127086,58.6018882076245));
#155735=CARTESIAN_POINT('Ctrl Pts',(82.3468082689014,10.6027633116616,58.4864321494171));
#155736=CARTESIAN_POINT('Ctrl Pts',(82.3478307597478,10.511714358207,58.4150869385433));
#155737=CARTESIAN_POINT('Ctrl Pts',(82.3489553753137,10.4210155333556,58.3429431568581));
#155738=CARTESIAN_POINT('Ctrl Pts',(82.3501908087954,10.3306320160889,58.2700496333164));
#155739=CARTESIAN_POINT('Ctrl Pts',(82.3509411230878,10.2757395060469,58.2257792995873));
#155740=CARTESIAN_POINT('Ctrl Pts',(82.3517322491779,10.2209631609564,58.1812322687692));
#155741=CARTESIAN_POINT('Ctrl Pts',(82.3525703921353,10.1662894370835,58.1364336318516));
#155742=CARTESIAN_POINT('Ctrl Pts',(82.0452144420091,12.45482652165,59.86552067071));
#155743=CARTESIAN_POINT('Ctrl Pts',(82.0448125353891,12.19986367057,59.70650410144));
#155744=CARTESIAN_POINT('Ctrl Pts',(82.0434374412991,11.64996340841,59.33864434196));
#155745=CARTESIAN_POINT('Ctrl Pts',(82.044184166809,10.85475243719,58.73582375429));
#155746=CARTESIAN_POINT('Ctrl Pts',(82.050838531519,10.32113499472,58.28707361965));
#155747=CARTESIAN_POINT('Ctrl Pts',(82.0553498143791,10.06894173163,58.06730239371));
#155748=CARTESIAN_POINT('Ctrl Pts',(83.1546990049091,12.5811772786,59.45168536214));
#155749=CARTESIAN_POINT('Ctrl Pts',(83.1625905359392,12.3201036028,59.31301191251));
#155750=CARTESIAN_POINT('Ctrl Pts',(83.1785169251191,11.75185687135,58.99008621727));
#155751=CARTESIAN_POINT('Ctrl Pts',(83.2017396508492,10.91386727203,58.4569794520501));
#155752=CARTESIAN_POINT('Ctrl Pts',(83.2201733202791,10.3389558953,58.05991259092));
#155753=CARTESIAN_POINT('Ctrl Pts',(83.2289698749091,10.06468241539,57.86541024147));
#155754=CARTESIAN_POINT('Ctrl Pts',(84.1164142591292,12.15828071422,60.01243626984));
#155755=CARTESIAN_POINT('Ctrl Pts',(84.1097704475691,11.87300708618,59.8804567433001));
#155756=CARTESIAN_POINT('Ctrl Pts',(84.0914149436691,11.25298218243,59.57233536711));
#155757=CARTESIAN_POINT('Ctrl Pts',(84.0535452913891,10.34012090282,59.0630977159));
#155758=CARTESIAN_POINT('Ctrl Pts',(84.0197048302691,9.71338194995202,58.6835306883801));
#155759=CARTESIAN_POINT('Ctrl Pts',(84.0013859811391,9.41587228684303,58.4983271796601));
#155760=CARTESIAN_POINT('Ctrl Pts',(84.0668739372791,11.5658390057,61.0442972286));
#155761=CARTESIAN_POINT('Ctrl Pts',(84.0359167148192,11.26000448237,60.89935221856));
#155762=CARTESIAN_POINT('Ctrl Pts',(83.962476303709,10.60125928587,60.56261320096));
#155763=CARTESIAN_POINT('Ctrl Pts',(83.834798336399,9.64865760807302,60.00996881749));
#155764=CARTESIAN_POINT('Ctrl Pts',(83.7315651934492,9.00609137754301,59.598005772));
#155765=CARTESIAN_POINT('Ctrl Pts',(83.6790761186291,8.70505241902901,59.39778200523));
#155766=CARTESIAN_POINT('Ctrl Pts',(82.3525733640486,10.1663210820827,58.136395020841));
#155767=CARTESIAN_POINT('Ctrl Pts',(82.3945030555095,10.1610405216675,58.1352972562638));
#155768=CARTESIAN_POINT('Ctrl Pts',(82.4370648290974,10.1545449462471,58.1355697300673));
#155769=CARTESIAN_POINT('Ctrl Pts',(82.4800399725421,10.146745735236,58.1373517678428));
#155770=CARTESIAN_POINT('Ctrl Pts',(82.5223769279141,10.1390623438138,58.1391073420591));
#155771=CARTESIAN_POINT('Ctrl Pts',(82.5651147310881,10.1301133570611,58.1423285092547));
#155772=CARTESIAN_POINT('Ctrl Pts',(82.6080053073103,10.1198371253139,58.1471276135581));
#155773=CARTESIAN_POINT('Ctrl Pts',(82.6500717961769,10.1097583381663,58.1518345092339));
#155774=CARTESIAN_POINT('Ctrl Pts',(82.6922847229005,10.0984025311023,58.1580597278645));
#155775=CARTESIAN_POINT('Ctrl Pts',(82.7343786504432,10.085738880054,58.1658819132491));
#155776=CARTESIAN_POINT('Ctrl Pts',(82.7638801760669,10.0768635612682,58.1713640912264));
#155777=CARTESIAN_POINT('Ctrl Pts',(82.7933225677532,10.0673464110393,58.1776301200527));
#155778=CARTESIAN_POINT('Ctrl Pts',(82.8226073273802,10.0571861011029,58.1846971565664));
#155779=CARTESIAN_POINT('Ctrl Pts',(82.8634086546753,10.0430301327284,58.1945433862596));
#155780=CARTESIAN_POINT('Ctrl Pts',(82.9039035584235,10.0276244794202,58.20594605374));
#155781=CARTESIAN_POINT('Ctrl Pts',(82.9438134541426,10.0109956210118,58.2189224676888));
#155782=CARTESIAN_POINT('Ctrl Pts',(82.9833775840859,9.99451082938244,58.2317864583964));
#155783=CARTESIAN_POINT('Ctrl Pts',(83.0223660486267,9.97682391605406,58.2461972008307));
#155784=CARTESIAN_POINT('Ctrl Pts',(83.0605032866594,9.95799336401192,58.2621329958283));
#155785=CARTESIAN_POINT('Ctrl Pts',(83.0983865723687,9.93928820286564,58.2779626758481));
#155786=CARTESIAN_POINT('Ctrl Pts',(83.1354291604188,9.91945468696171,58.2952971765887));
#155787=CARTESIAN_POINT('Ctrl Pts',(83.1713681958996,9.89858191831988,58.3140757469682));
#155788=CARTESIAN_POINT('Ctrl Pts',(83.2071405652668,9.87780594646696,58.3327672323355));
#155789=CARTESIAN_POINT('Ctrl Pts',(83.2418188546337,9.85600056275274,58.3528892855549));
#155790=CARTESIAN_POINT('Ctrl Pts',(83.2751623523267,9.83328278451351,58.3743436893457));
#155791=CARTESIAN_POINT('Ctrl Pts',(83.3084391276747,9.81061046591531,58.3957551615838));
#155792=CARTESIAN_POINT('Ctrl Pts',(83.3403857854015,9.78702973087887,58.4184933773822));
#155793=CARTESIAN_POINT('Ctrl Pts',(83.3707920740686,9.76268184976974,58.4424255889604));
#155794=CARTESIAN_POINT('Ctrl Pts',(83.4011928153647,9.73833841072618,58.4663534343083));
#155795=CARTESIAN_POINT('Ctrl Pts',(83.4300532122819,9.71322852495286,58.4914744303251));
#155796=CARTESIAN_POINT('Ctrl Pts',(83.4572012202667,9.68751271914462,58.517625939285));
#155797=CARTESIAN_POINT('Ctrl Pts',(83.4844664171747,9.66168590675377,58.5438903356131));
#155798=CARTESIAN_POINT('Ctrl Pts',(83.5100040116657,9.63524841096765,58.5711936551417));
#155799=CARTESIAN_POINT('Ctrl Pts',(83.5336852727824,9.60837557320823,58.5993478091022));
#155800=CARTESIAN_POINT('Ctrl Pts',(83.5529022951893,9.5865686296163,58.6221945234237));
#155801=CARTESIAN_POINT('Ctrl Pts',(83.5708977465699,9.56447536479424,58.6456009442468));
#155802=CARTESIAN_POINT('Ctrl Pts',(83.587626795633,9.54219220342424,58.6694590571945));
#155803=CARTESIAN_POINT('Ctrl Pts',(83.6085204360661,9.51436178941662,58.6992564970528));
#155804=CARTESIAN_POINT('Ctrl Pts',(83.6274371272222,9.48623551281498,58.7297583097961));
#155805=CARTESIAN_POINT('Ctrl Pts',(83.6443373015206,9.45799892415152,58.7607462965735));
#155806=CARTESIAN_POINT('Ctrl Pts',(83.6613600541117,9.42955753329083,58.7919590416549));
#155807=CARTESIAN_POINT('Ctrl Pts',(83.6763371024946,9.40100471560584,58.8236644181987));
#155808=CARTESIAN_POINT('Ctrl Pts',(83.6892807472202,9.37252131819323,58.855640635855));
#155809=CARTESIAN_POINT('Ctrl Pts',(83.7024340725541,9.34357650390593,58.8881348523371));
#155810=CARTESIAN_POINT('Ctrl Pts',(83.7134878859966,9.31470383090157,58.9209081565808));
#155811=CARTESIAN_POINT('Ctrl Pts',(83.7225058357604,9.28607678906234,58.9537383854738));
#155812=CARTESIAN_POINT('Ctrl Pts',(83.7298397047622,9.26279577949186,58.9804376468697));
#155813=CARTESIAN_POINT('Ctrl Pts',(83.7358281994042,9.23967697175823,59.0071746660718));
#155814=CARTESIAN_POINT('Ctrl Pts',(83.7405269386778,9.21680318453082,59.0338387719999));
#155815=CARTESIAN_POINT('Ctrl Pts',(82.3362558180773,12.3439659630715,59.7078953260468));
#155816=CARTESIAN_POINT('Ctrl Pts',(82.3898752941292,12.3438789835486,59.6983874893455));
#155817=CARTESIAN_POINT('Ctrl Pts',(82.4439640504566,12.3422887500421,59.6913976293074));
#155818=CARTESIAN_POINT('Ctrl Pts',(82.4981679796218,12.3391948370408,59.6869681324302));
#155819=CARTESIAN_POINT('Ctrl Pts',(82.5544403024617,12.3359828619324,59.6823696082616));
#155820=CARTESIAN_POINT('Ctrl Pts',(82.6108361599016,12.3311506991394,59.6805299615381));
#155821=CARTESIAN_POINT('Ctrl Pts',(82.666987223834,12.3247219659808,59.6814514375097));
#155822=CARTESIAN_POINT('Ctrl Pts',(82.7278805300929,12.3177502936799,59.6824507368037));
#155823=CARTESIAN_POINT('Ctrl Pts',(82.7884855316095,12.3089014340018,59.6866965834116));
#155824=CARTESIAN_POINT('Ctrl Pts',(82.8483737227941,12.2982262594063,59.6941495979233));
#155825=CARTESIAN_POINT('Ctrl Pts',(82.8720255849641,12.2940102736973,59.697093044177));
#155826=CARTESIAN_POINT('Ctrl Pts',(82.895566099159,12.2895096078843,59.7005363430759));
#155827=CARTESIAN_POINT('Ctrl Pts',(82.9189705088584,12.284727957392,59.7044758164529));
#155828=CARTESIAN_POINT('Ctrl Pts',(82.9752836654168,12.2732228677,59.713954550755));
#155829=CARTESIAN_POINT('Ctrl Pts',(83.0307890218355,12.2600930370941,59.7263059761169));
#155830=CARTESIAN_POINT('Ctrl Pts',(83.0850974846959,12.2454304953023,59.7414438060835));
#155831=CARTESIAN_POINT('Ctrl Pts',(83.1407614781443,12.2304019788013,59.7569594738763));
#155832=CARTESIAN_POINT('Ctrl Pts',(83.1951680326611,12.2137634772824,59.7754020615918));
#155833=CARTESIAN_POINT('Ctrl Pts',(83.247930350291,12.1956346723825,59.7966382691706));
#155834=CARTESIAN_POINT('Ctrl Pts',(83.3020507591139,12.1770392357768,59.8184210923603));
#155835=CARTESIAN_POINT('Ctrl Pts',(83.3544412763208,12.1568758451657,59.8431430904216));
#155836=CARTESIAN_POINT('Ctrl Pts',(83.4047175566575,12.1352930555086,59.8706218643776));
#155837=CARTESIAN_POINT('Ctrl Pts',(83.4189110912545,12.1292000018927,59.8783794177649));
#155838=CARTESIAN_POINT('Ctrl Pts',(83.4329363158177,12.1229939375054,59.8863564573931));
#155839=CARTESIAN_POINT('Ctrl Pts',(83.4467850288678,12.1166784743217,59.8945483461906));
#155840=CARTESIAN_POINT('Ctrl Pts',(83.495707214561,12.0943683678522,59.9234871438592));
#155841=CARTESIAN_POINT('Ctrl Pts',(83.5424118751783,12.0706973089624,59.9551025709805));
#155842=CARTESIAN_POINT('Ctrl Pts',(83.5865601147,12.0458386524717,59.9891628621646));
#155843=CARTESIAN_POINT('Ctrl Pts',(83.6299686621919,12.0213964961693,60.0226524822144));
#155844=CARTESIAN_POINT('Ctrl Pts',(83.6709057018179,11.9958061379543,60.0585058438186));
#155845=CARTESIAN_POINT('Ctrl Pts',(83.7090783845161,11.9692506337432,60.0964667024375));
#155846=CARTESIAN_POINT('Ctrl Pts',(83.7459394155726,11.9436076032759,60.1331231879024));
#155847=CARTESIAN_POINT('Ctrl Pts',(83.7802225929091,11.9170646238981,60.1717448460995));
#155848=CARTESIAN_POINT('Ctrl Pts',(83.8116934622586,11.8898040988633,60.2120662059309));
#155849=CARTESIAN_POINT('Ctrl Pts',(83.8211194575485,11.8816391645641,60.2241430552747));
#155850=CARTESIAN_POINT('Ctrl Pts',(83.8302933815406,11.8734099819859,60.2363721393201));
#155851=CARTESIAN_POINT('Ctrl Pts',(83.839209531085,11.8651217677242,60.2487456887995));
#155852=CARTESIAN_POINT('Ctrl Pts',(83.8704799058314,11.8360536633086,60.2921417228425));
#155853=CARTESIAN_POINT('Ctrl Pts',(83.8985682120131,11.8062674363767,60.3373029827861));
#155854=CARTESIAN_POINT('Ctrl Pts',(83.9232890453394,11.7759607036118,60.383921015016));
#155855=CARTESIAN_POINT('Ctrl Pts',(83.9465788636436,11.7474083368621,60.427840468944));
#155856=CARTESIAN_POINT('Ctrl Pts',(83.9668790442298,11.7183939124342,60.4730531648616));
#155857=CARTESIAN_POINT('Ctrl Pts',(83.9840549989384,11.6891014111649,60.5192657007433));
#155858=CARTESIAN_POINT('Ctrl Pts',(84.0002429493343,11.661493888581,60.5628199747976));
#155859=CARTESIAN_POINT('Ctrl Pts',(84.0136550708351,11.6336395430904,60.6072621814493));
#155860=CARTESIAN_POINT('Ctrl Pts',(84.0242076731205,11.6057085713668,60.6523140983562));
#155861=CARTESIAN_POINT('Ctrl Pts',(84.028908909982,11.5932651843904,60.6723849516602));
#155862=CARTESIAN_POINT('Ctrl Pts',(84.0330430642595,11.5808067950523,60.6925763859497));
#155863=CARTESIAN_POINT('Ctrl Pts',(84.0366053096489,11.5683493738914,60.7128617804331));
#155864=CARTESIAN_POINT('Origin',(83.1537660643691,9.5,64.344226319776));
#155865=CARTESIAN_POINT('Origin',(82.8534541851791,13.10501209624,62.64107301909));
#155866=CARTESIAN_POINT('Origin',(82.8534541851791,13.10501209624,62.64107301909));
#155867=CARTESIAN_POINT('Origin',(82.8534541851791,13.10500472878,62.64107301909));
#155868=CARTESIAN_POINT('Origin',(82.8534541851791,13.10501209624,62.64107301909));
#155869=CARTESIAN_POINT('Origin',(65.7305865146691,13.10501209624,65.660296576497));
#155870=CARTESIAN_POINT('Ctrl Pts',(65.9990597670353,14.4574398737497,64.9541505386852));
#155871=CARTESIAN_POINT('Ctrl Pts',(66.0057594746386,14.4759573978632,64.9921646720018));
#155872=CARTESIAN_POINT('Ctrl Pts',(66.0127624332916,14.4932775623909,65.031898108079));
#155873=CARTESIAN_POINT('Ctrl Pts',(66.0200516207235,14.5090651792659,65.0732541692221));
#155874=CARTESIAN_POINT('Ctrl Pts',(66.0272350688423,14.5246237758588,65.114010305952));
#155875=CARTESIAN_POINT('Ctrl Pts',(66.0346965123793,14.5386934153553,65.1563423930204));
#155876=CARTESIAN_POINT('Ctrl Pts',(66.0424108685044,14.5509579784476,65.2001080450176));
#155877=CARTESIAN_POINT('Ctrl Pts',(66.0499758944906,14.5629851310703,65.2430265062983));
#155878=CARTESIAN_POINT('Ctrl Pts',(66.0577841207212,14.5732758890196,65.2873234807316));
#155879=CARTESIAN_POINT('Ctrl Pts',(66.0658034282234,14.5815445851561,65.3328166865689));
#155880=CARTESIAN_POINT('Ctrl Pts',(66.0740601818967,14.5900581116894,65.3796569148937));
#155881=CARTESIAN_POINT('Ctrl Pts',(66.0825407385727,14.5964273023246,65.4277654708633));
#155882=CARTESIAN_POINT('Ctrl Pts',(66.0912007151699,14.6003635820811,65.4768905079869));
#155883=CARTESIAN_POINT('Ctrl Pts',(66.0994190005942,14.6040990968583,65.5235099846134));
#155884=CARTESIAN_POINT('Ctrl Pts',(66.1077987754103,14.6056432230592,65.5710443586578));
#155885=CARTESIAN_POINT('Ctrl Pts',(66.1162944712471,14.6047772907763,65.6192350815045));
#155886=CARTESIAN_POINT('Ctrl Pts',(66.1167510718232,14.6047307513066,65.6218250885193));
#155887=CARTESIAN_POINT('Ctrl Pts',(66.1172080055183,14.6046772580499,65.6244169816493));
#155888=CARTESIAN_POINT('Ctrl Pts',(66.1176652646771,14.6046167797623,65.6270107174613));
#155889=CARTESIAN_POINT('Ctrl Pts',(66.1254536827152,14.6035866633016,65.6711893815637));
#155890=CARTESIAN_POINT('Ctrl Pts',(66.1333324490441,14.6005268101228,65.7158795335643));
#155891=CARTESIAN_POINT('Ctrl Pts',(66.141252533839,14.5953144080035,65.7608030751315));
#155892=CARTESIAN_POINT('Ctrl Pts',(66.1491233289967,14.5901344446036,65.80544704077));
#155893=CARTESIAN_POINT('Ctrl Pts',(66.157034833932,14.5828284021327,65.8503209555839));
#155894=CARTESIAN_POINT('Ctrl Pts',(66.1649357618761,14.5733237250958,65.8951339221507));
#155895=CARTESIAN_POINT('Ctrl Pts',(66.1718110009962,14.5650529336328,65.9341293240847));
#155896=CARTESIAN_POINT('Ctrl Pts',(66.1786781405354,14.5551179750657,65.9730780617015));
#155897=CARTESIAN_POINT('Ctrl Pts',(66.1855023102385,14.543502605895,66.0117823524318));
#155898=CARTESIAN_POINT('Ctrl Pts',(66.1930281223036,14.5306929764088,66.0544661118965));
#155899=CARTESIAN_POINT('Ctrl Pts',(66.200501021359,14.5158392733046,66.0968488687635));
#155900=CARTESIAN_POINT('Ctrl Pts',(66.2078710231428,14.4989722922697,66.1386471816904));
#155901=CARTESIAN_POINT('Ctrl Pts',(66.2152313904599,14.4821273606688,66.1803908535916));
#155902=CARTESIAN_POINT('Ctrl Pts',(66.222489021452,14.4632745153903,66.2215509966373));
#155903=CARTESIAN_POINT('Ctrl Pts',(66.2295958760183,14.4424954357575,66.2618551952368));
#155904=CARTESIAN_POINT('Ctrl Pts',(66.2367027305846,14.4217163561247,66.3021593938362));
#155905=CARTESIAN_POINT('Ctrl Pts',(66.2436587050356,14.3990112627432,66.3416070599376));
#155906=CARTESIAN_POINT('Ctrl Pts',(66.250419100565,14.3745104500712,66.3799447273744));
#155907=CARTESIAN_POINT('Ctrl Pts',(66.257172054931,14.3500366054296,66.4182401965627));
#155908=CARTESIAN_POINT('Ctrl Pts',(66.263729127918,14.3237736558815,66.4554239584199));
#155909=CARTESIAN_POINT('Ctrl Pts',(66.2700506925101,14.2958966587661,66.4912713686282));
#155910=CARTESIAN_POINT('Ctrl Pts',(66.2763868477308,14.267955319524,66.5272015172535));
#155911=CARTESIAN_POINT('Ctrl Pts',(66.2824863241572,14.238392902661,66.5617886732506));
#155912=CARTESIAN_POINT('Ctrl Pts',(66.2883154073236,14.2074242124426,66.5948417246754));
#155913=CARTESIAN_POINT('Ctrl Pts',(66.29414449049,14.1764555222241,66.6278947761001));
#155914=CARTESIAN_POINT('Ctrl Pts',(66.2997031187361,14.1440810828274,66.6594133732594));
#155915=CARTESIAN_POINT('Ctrl Pts',(66.3049648364074,14.1105469821226,66.6892475709747));
#155916=CARTESIAN_POINT('Ctrl Pts',(66.3104409944182,14.0756462052884,66.7202976559509));
#155917=CARTESIAN_POINT('Ctrl Pts',(66.3155951249781,14.0394928311997,66.7495208615145));
#155918=CARTESIAN_POINT('Ctrl Pts',(66.3204087928235,14.0023722391874,66.7768127657061));
#155919=CARTESIAN_POINT('Ctrl Pts',(66.3252538533421,13.965009562626,66.8042826559685));
#155920=CARTESIAN_POINT('Ctrl Pts',(66.3297539717965,13.9266676208806,66.8297958354293));
#155921=CARTESIAN_POINT('Ctrl Pts',(66.3338993005816,13.8876498893092,66.8532965877114));
#155922=CARTESIAN_POINT('Ctrl Pts',(66.3374979748372,13.8537775203377,66.8736982389697));
#155923=CARTESIAN_POINT('Ctrl Pts',(66.3408294076461,13.8193962776764,66.892584051289));
#155924=CARTESIAN_POINT('Ctrl Pts',(66.3438926774567,13.784706883934,66.9099488847624));
#155925=CARTESIAN_POINT('Ctrl Pts',(66.3477567273563,13.7409492142877,66.9318531201676));
#155926=CARTESIAN_POINT('Ctrl Pts',(66.351191691087,13.6967299211875,66.9513236913815));
#155927=CARTESIAN_POINT('Ctrl Pts',(66.3542127318989,13.6523830947144,66.9684405122135));
#155928=CARTESIAN_POINT('Ctrl Pts',(66.3574047870039,13.6055258946137,66.9865262775906));
#155929=CARTESIAN_POINT('Ctrl Pts',(66.3601347360615,13.5585270469719,67.0019843017333));
#155930=CARTESIAN_POINT('Ctrl Pts',(66.36242967166,13.5117483031678,67.0149610607877));
#155931=CARTESIAN_POINT('Ctrl Pts',(66.3646648452017,13.4661877172684,67.027599894102));
#155932=CARTESIAN_POINT('Ctrl Pts',(66.3664874938195,13.4208360801918,67.0378857301113));
#155933=CARTESIAN_POINT('Ctrl Pts',(66.3679299384219,13.375991750249,67.0459952421882));
#155934=CARTESIAN_POINT('Ctrl Pts',(66.3694302332009,13.3293489093591,67.0544299915084));
#155935=CARTESIAN_POINT('Ctrl Pts',(66.3705192816255,13.2832553871896,67.0605107241182));
#155936=CARTESIAN_POINT('Ctrl Pts',(66.371240074511,13.2380019494673,67.0644737956167));
#155937=CARTESIAN_POINT('Ctrl Pts',(66.3719608673965,13.1927485117449,67.0684368671152));
#155938=CARTESIAN_POINT('Ctrl Pts',(66.3723135188225,13.1483352462663,67.0702829244797));
#155939=CARTESIAN_POINT('Ctrl Pts',(66.3723460706922,13.1050047578645,67.0702769694531));
#155940=CARTESIAN_POINT('Ctrl Pts',(62.7470145624991,14.67260333684,68.1339161337049));
#155941=CARTESIAN_POINT('Ctrl Pts',(62.7479150825191,14.67317930239,68.1258209755479));
#155942=CARTESIAN_POINT('Ctrl Pts',(62.7947126550891,14.70165222008,67.716427844428));
#155943=CARTESIAN_POINT('Ctrl Pts',(63.0238969208491,14.69415619541,66.887022874744));
#155944=CARTESIAN_POINT('Ctrl Pts',(63.6771079958591,14.55782369561,65.90062340207));
#155945=CARTESIAN_POINT('Ctrl Pts',(64.4836385318891,14.4067499227,65.232530091334));
#155946=CARTESIAN_POINT('Ctrl Pts',(65.2857897757591,14.31390318541,64.849693565196));
#155947=CARTESIAN_POINT('Ctrl Pts',(65.8917919259791,14.29551720364,64.700120545389));
#155948=CARTESIAN_POINT('Ctrl Pts',(66.2321603836891,14.30404532187,64.660713883658));
#155949=CARTESIAN_POINT('Ctrl Pts',(66.3183572158991,14.30731400122,64.653570092238));
#155950=CARTESIAN_POINT('Ctrl Pts',(64.0360609143291,15.66352209507,68.392852817656));
#155951=CARTESIAN_POINT('Ctrl Pts',(64.0366778488791,15.66420500743,68.3857663296231));
#155952=CARTESIAN_POINT('Ctrl Pts',(64.0691151217491,15.6979376344,68.027533940496));
#155953=CARTESIAN_POINT('Ctrl Pts',(64.2700051029891,15.68776125165,67.319166073428));
#155954=CARTESIAN_POINT('Ctrl Pts',(64.8256825409091,15.53611715734,66.5858944691141));
#155955=CARTESIAN_POINT('Ctrl Pts',(65.4124246610891,15.38571278724,66.2020900065669));
#155956=CARTESIAN_POINT('Ctrl Pts',(65.8737717372191,15.30532374558,66.050089008981));
#155957=CARTESIAN_POINT('Ctrl Pts',(66.1527177053691,15.29122946637,65.995932476021));
#155958=CARTESIAN_POINT('Ctrl Pts',(66.311070658609,15.2979482611,65.9716179772301));
#155959=CARTESIAN_POINT('Ctrl Pts',(66.3518513255091,15.30058162146,65.966078449576));
#155960=CARTESIAN_POINT('Ctrl Pts',(65.4272503875291,14.78981337192,68.501643204624));
#155961=CARTESIAN_POINT('Ctrl Pts',(65.4275400140691,14.79040198758,68.4979963080879));
#155962=CARTESIAN_POINT('Ctrl Pts',(65.4428463358591,14.81949704579,68.313664662612));
#155963=CARTESIAN_POINT('Ctrl Pts',(65.5462723729991,14.8116839771,67.951996102549));
#155964=CARTESIAN_POINT('Ctrl Pts',(65.8296142676391,14.67354035755,67.595807470617));
#155965=CARTESIAN_POINT('Ctrl Pts',(66.1121715994391,14.52254576442,67.430978993379));
#155966=CARTESIAN_POINT('Ctrl Pts',(66.3104326447591,14.43117257572,67.382530829545));
#155967=CARTESIAN_POINT('Ctrl Pts',(66.4130867013791,14.41329423457,67.367143975852));
#155968=CARTESIAN_POINT('Ctrl Pts',(66.4718810278291,14.42160833841,67.356286576696));
#155969=CARTESIAN_POINT('Ctrl Pts',(66.4872299064291,14.42480186956,67.353551898505));
#155970=CARTESIAN_POINT('Ctrl Pts',(65.1192019616691,13.18279848744,68.3194201143539));
#155971=CARTESIAN_POINT('Ctrl Pts',(65.1195443722891,13.18321366293,68.317189977293));
#155972=CARTESIAN_POINT('Ctrl Pts',(65.1371310953791,13.20377882802,68.204323782827));
#155973=CARTESIAN_POINT('Ctrl Pts',(65.2001246699891,13.20031260946,67.9660933031889));
#155974=CARTESIAN_POINT('Ctrl Pts',(65.3889626624191,13.08700045068,67.62267704219));
#155975=CARTESIAN_POINT('Ctrl Pts',(65.6768123602791,12.93492025868,67.327970738096));
#155976=CARTESIAN_POINT('Ctrl Pts',(66.0303623322191,12.8233438978,67.121707376222));
#155977=CARTESIAN_POINT('Ctrl Pts',(66.3357602447291,12.79850552099,67.038242493658));
#155978=CARTESIAN_POINT('Ctrl Pts',(66.5063662620891,12.80975388131,67.021782211843));
#155979=CARTESIAN_POINT('Ctrl Pts',(66.5491980682491,12.81397773617,67.019421110833));
#155980=CARTESIAN_POINT('',(65.1767302637191,13.4988189915,68.186796166063));
#155981=CARTESIAN_POINT('Ctrl Pts',(65.1767302637191,13.4988189915,68.186796166063));
#155982=CARTESIAN_POINT('Ctrl Pts',(65.1929684679118,13.5004670413057,68.1210750045845));
#155983=CARTESIAN_POINT('Ctrl Pts',(65.2147225439506,13.4958913458165,68.0522988453429));
#155984=CARTESIAN_POINT('Ctrl Pts',(65.257832004244,13.4796921846402,67.9464492805757));
#155985=CARTESIAN_POINT('Ctrl Pts',(65.2739476083543,13.4727365279243,67.9107267924136));
#155986=CARTESIAN_POINT('Ctrl Pts',(65.3010060673154,13.4599691383649,67.8568027520571));
#155987=CARTESIAN_POINT('Ctrl Pts',(65.3152562865387,13.4530019674638,67.8297565255));
#155988=CARTESIAN_POINT('Ctrl Pts',(65.3331978895328,13.4438525182,67.7981343309232));
#155989=CARTESIAN_POINT('Ctrl Pts',(65.3425042620514,13.4390225227651,67.7823167711229));
#155990=CARTESIAN_POINT('Ctrl Pts',(65.3465652990597,13.4368978238351,67.7755375856623));
#155991=CARTESIAN_POINT('Ctrl Pts',(65.3492888634492,13.4354692021293,67.7710182074229));
#155992=CARTESIAN_POINT('Ctrl Pts',(65.3513344277367,13.4343926095366,67.7676506489246));
#155993=CARTESIAN_POINT('Ctrl Pts',(65.3745118775289,13.4221739390526,67.7296466516154));
#155994=CARTESIAN_POINT('Ctrl Pts',(65.4075181681876,13.4032698716892,67.678533313575));
#155995=CARTESIAN_POINT('Ctrl Pts',(65.480294248736,13.3643302812121,67.5864913548544));
#155996=CARTESIAN_POINT('Ctrl Pts',(65.5084675799845,13.3495865028143,67.5532979674494));
#155997=CARTESIAN_POINT('Ctrl Pts',(65.5577359449127,13.3248249628597,67.5010467284812));
#155998=CARTESIAN_POINT('Ctrl Pts',(65.5753274880599,13.3161301374819,67.4832239345388));
#155999=CARTESIAN_POINT('Ctrl Pts',(65.603610088605,13.3024264313256,67.456088371081));
#156000=CARTESIAN_POINT('Ctrl Pts',(65.6182251610257,13.2954092112251,67.4424207290154));
#156001=CARTESIAN_POINT('Ctrl Pts',(65.6335767514054,13.2881439405909,67.4286466505924));
#156002=CARTESIAN_POINT('Ctrl Pts',(65.6439776049505,13.2832453044941,67.4194454183518));
#156003=CARTESIAN_POINT('Ctrl Pts',(65.6503894617934,13.2802420914402,67.413865319445));
#156004=CARTESIAN_POINT('Ctrl Pts',(65.7224706740662,13.2466142800192,67.3518778494876));
#156005=CARTESIAN_POINT('Ctrl Pts',(65.7890943453541,13.2197701629759,67.3050628077342));
#156006=CARTESIAN_POINT('Ctrl Pts',(65.8823332755805,13.1867123691467,67.2481596329767));
#156007=CARTESIAN_POINT('Ctrl Pts',(65.9123200873604,13.1768945014928,67.2314072951406));
#156008=CARTESIAN_POINT('Ctrl Pts',(65.9552393776427,13.163969795446,67.2091013539741));
#156009=CARTESIAN_POINT('Ctrl Pts',(65.9692034964649,13.159961909336,67.2021366296084));
#156010=CARTESIAN_POINT('Ctrl Pts',(65.9963899372814,13.152546835594,67.1890679943413));
#156011=CARTESIAN_POINT('Ctrl Pts',(66.0083992161454,13.1494334715406,67.1835042839346));
#156012=CARTESIAN_POINT('Ctrl Pts',(66.1347577280693,13.1188275137962,67.1272322695939));
#156013=CARTESIAN_POINT('Ctrl Pts',(66.2526057819523,13.1051514965565,67.091377765781));
#156014=CARTESIAN_POINT('Ctrl Pts',(66.3723465844291,13.10500475785,67.070279883));
#156015=CARTESIAN_POINT('Ctrl Pts',(63.7242537617786,14.9985402150431,67.8461554916125));
#156016=CARTESIAN_POINT('Ctrl Pts',(63.8955981567397,14.9984281505454,67.8886462156272));
#156017=CARTESIAN_POINT('Ctrl Pts',(64.0802735483646,14.9652747214087,67.9339609061182));
#156018=CARTESIAN_POINT('Ctrl Pts',(64.437577712981,14.8177553154702,68.0205666754888));
#156019=CARTESIAN_POINT('Ctrl Pts',(64.6091063807268,14.7029155066426,68.0615791088498));
#156020=CARTESIAN_POINT('Ctrl Pts',(64.8923141882571,14.410075514194,68.1279665869427));
#156021=CARTESIAN_POINT('Ctrl Pts',(65.0030535557672,14.233058864924,68.1531213529668));
#156022=CARTESIAN_POINT('Ctrl Pts',(65.1448299480447,13.8649342455952,68.1835019232699));
#156023=CARTESIAN_POINT('Ctrl Pts',(65.1763418945754,13.6749482756929,68.188859754286));
#156024=CARTESIAN_POINT('Ctrl Pts',(65.1767302637191,13.4988189915,68.186796166063));
#156025=CARTESIAN_POINT('Ctrl Pts',(63.5004917476991,14.85683282676,69.6013899904));
#156026=CARTESIAN_POINT('Ctrl Pts',(63.4875111720091,14.86142859631,69.562289012902));
#156027=CARTESIAN_POINT('Ctrl Pts',(63.3667162203191,14.90537723046,69.174553074221));
#156028=CARTESIAN_POINT('Ctrl Pts',(63.2779512911692,14.96073620167,68.428956249786));
#156029=CARTESIAN_POINT('Ctrl Pts',(63.4176540715092,14.97167354225,67.736399611083));
#156030=CARTESIAN_POINT('Ctrl Pts',(63.5272467061291,14.97036663875,67.431122989516));
#156031=CARTESIAN_POINT('Ctrl Pts',(64.632194658559,15.09322707693,69.316831401601));
#156032=CARTESIAN_POINT('Ctrl Pts',(64.6223300227891,15.09789088302,69.2901568971791));
#156033=CARTESIAN_POINT('Ctrl Pts',(64.5301655221991,15.14249513828,69.025170748245));
#156034=CARTESIAN_POINT('Ctrl Pts',(64.4569578919491,15.19876233977,68.5077214005671));
#156035=CARTESIAN_POINT('Ctrl Pts',(64.5513828811191,15.20980533273,68.0300280414471));
#156036=CARTESIAN_POINT('Ctrl Pts',(64.6262734480091,15.20849566901,67.822349915333));
#156037=CARTESIAN_POINT('Ctrl Pts',(65.4160083966392,14.25724551843,68.99376188389));
#156038=CARTESIAN_POINT('Ctrl Pts',(65.4103628908792,14.26166872097,68.977921457425));
#156039=CARTESIAN_POINT('Ctrl Pts',(65.3576865499092,14.30395444625,68.8206616065041));
#156040=CARTESIAN_POINT('Ctrl Pts',(65.3168769034091,14.35700979395,68.515233029078));
#156041=CARTESIAN_POINT('Ctrl Pts',(65.3731355800791,14.36767915922,68.232661054128));
#156042=CARTESIAN_POINT('Ctrl Pts',(65.4175819661791,14.36637925674,68.109211017786));
#156043=CARTESIAN_POINT('Ctrl Pts',(65.1483470279191,13.09930223189,68.922182948247));
#156044=CARTESIAN_POINT('Ctrl Pts',(65.1442365642691,13.10339216721,68.9058590563));
#156045=CARTESIAN_POINT('Ctrl Pts',(65.1064597700491,13.14246642663,68.744602114318));
#156046=CARTESIAN_POINT('Ctrl Pts',(65.0858069266991,13.19107293871,68.444748364805));
#156047=CARTESIAN_POINT('Ctrl Pts',(65.1452705423991,13.201224781,68.1624062803621));
#156048=CARTESIAN_POINT('Ctrl Pts',(65.1908586799991,13.1999383991,68.034207063451));
#156049=CARTESIAN_POINT('Ctrl Pts',(65.1554518235812,13.43008177675,68.8079679196157));
#156050=CARTESIAN_POINT('Ctrl Pts',(65.1461881102573,13.4408321527727,68.7554267047025));
#156051=CARTESIAN_POINT('Ctrl Pts',(65.1396268661127,13.4503444917441,68.7018053079805));
#156052=CARTESIAN_POINT('Ctrl Pts',(65.1359957247053,13.4586188334764,68.6473919336038));
#156053=CARTESIAN_POINT('Ctrl Pts',(65.132407771396,13.4667947617781,68.5936257414467));
#156054=CARTESIAN_POINT('Ctrl Pts',(65.1316810761034,13.4737619667128,68.5390864487085));
#156055=CARTESIAN_POINT('Ctrl Pts',(65.1340082530278,13.479520486689,68.4840944107843));
#156056=CARTESIAN_POINT('Ctrl Pts',(65.1362929772285,13.4851739588475,68.4301055461744));
#156057=CARTESIAN_POINT('Ctrl Pts',(65.1415215476525,13.4896624418642,68.375680553896));
#156058=CARTESIAN_POINT('Ctrl Pts',(65.149844087735,13.4929859720836,68.3211605832403));
#156059=CARTESIAN_POINT('Ctrl Pts',(65.1566824461639,13.4957168079419,68.2763633101505));
#156060=CARTESIAN_POINT('Ctrl Pts',(65.1656091946349,13.4976611410268,68.2315026619847));
#156061=CARTESIAN_POINT('Ctrl Pts',(65.1766881467414,13.4988189915,68.1867857312686));
#156062=CARTESIAN_POINT('Origin',(66.6326669169691,-15.387431115,68.54751529846));
#156063=CARTESIAN_POINT('Ctrl Pts',(65.1554729113358,6.92820316501672,68.8079843794271));
#156064=CARTESIAN_POINT('Ctrl Pts',(65.152422383041,6.92817587206967,68.7907276719249));
#156065=CARTESIAN_POINT('Ctrl Pts',(65.1496737586822,6.92912017635131,68.7734202159333));
#156066=CARTESIAN_POINT('Ctrl Pts',(65.1472414203523,6.93105915649169,68.7561084383063));
#156067=CARTESIAN_POINT('Ctrl Pts',(65.1359547055815,6.94005655439528,68.6757770576567));
#156068=CARTESIAN_POINT('Ctrl Pts',(65.1314783371817,6.97047158444587,68.5953526581359));
#156069=CARTESIAN_POINT('Ctrl Pts',(65.132953575682,7.01677570366725,68.5181912974979));
#156070=CARTESIAN_POINT('Ctrl Pts',(65.1334410218994,7.03207544521049,68.4926957499151));
#156071=CARTESIAN_POINT('Ctrl Pts',(65.1345782401243,7.04910988856502,68.467556444226));
#156072=CARTESIAN_POINT('Ctrl Pts',(65.1363109483351,7.06765272021812,68.4427928220101));
#156073=CARTESIAN_POINT('Ctrl Pts',(65.140437744398,7.11181623498945,68.3838132327012));
#156074=CARTESIAN_POINT('Ctrl Pts',(65.1479424717781,7.16453628519599,68.3269644385079));
#156075=CARTESIAN_POINT('Ctrl Pts',(65.1580919268926,7.22275584259291,68.2725087516098));
#156076=CARTESIAN_POINT('Ctrl Pts',(65.174020876945,7.31412788290298,68.1870438762168));
#156077=CARTESIAN_POINT('Ctrl Pts',(65.1964641614873,7.41904598491702,68.1074735321002));
#156078=CARTESIAN_POINT('Ctrl Pts',(65.2237077236684,7.53099885535992,68.0328950571003));
#156079=CARTESIAN_POINT('Ctrl Pts',(65.2538259358793,7.65476462017449,67.9504473095745));
#156080=CARTESIAN_POINT('Ctrl Pts',(65.2898109036682,7.7871280561005,67.874100474813));
#156081=CARTESIAN_POINT('Ctrl Pts',(65.3305707565767,7.9237476928918,67.802837119998));
#156082=CARTESIAN_POINT('Ctrl Pts',(65.3756768202716,8.07493504022901,67.7239749752151));
#156083=CARTESIAN_POINT('Ctrl Pts',(65.4266303535699,8.23133465583079,67.6513382216725));
#156084=CARTESIAN_POINT('Ctrl Pts',(65.4828074420408,8.38987577335587,67.5842795080536));
#156085=CARTESIAN_POINT('Ctrl Pts',(65.5453260651721,8.5663137598585,67.5096508906131));
#156086=CARTESIAN_POINT('Ctrl Pts',(65.6143141261707,8.74540402040174,67.4419307527597));
#156087=CARTESIAN_POINT('Ctrl Pts',(65.6894671929274,8.92454600486117,67.3811644589306));
#156088=CARTESIAN_POINT('Ctrl Pts',(65.740845476658,9.04701615947804,67.3396216713859));
#156089=CARTESIAN_POINT('Ctrl Pts',(65.7951051325205,9.1695104865657,67.3013289431462));
#156090=CARTESIAN_POINT('Ctrl Pts',(65.8521790298628,9.29134610700093,67.2665592059008));
#156091=CARTESIAN_POINT('Ctrl Pts',(65.8881718169189,9.36817989173203,67.2446321988636));
#156092=CARTESIAN_POINT('Ctrl Pts',(65.925284050671,9.44475190004438,67.2241061885447));
#156093=CARTESIAN_POINT('Ctrl Pts',(65.9634978877863,9.52089124203153,67.2050500989013));
#156094=CARTESIAN_POINT('Ctrl Pts',(66.076365450387,9.74577475535619,67.1487664447826));
#156095=CARTESIAN_POINT('Ctrl Pts',(66.1988426116163,9.96688292982532,67.105308130441));
#156096=CARTESIAN_POINT('Ctrl Pts',(66.3301387866529,10.1797418696686,67.0783397637765));
#156097=CARTESIAN_POINT('Ctrl Pts',(66.3439710393069,10.2021668842187,67.0754986051421));
#156098=CARTESIAN_POINT('Ctrl Pts',(66.3579011816857,10.2245003535534,67.0728404391239));
#156099=CARTESIAN_POINT('Ctrl Pts',(66.3719238214764,10.2467337087739,67.0703710012959));
#156100=CARTESIAN_POINT('Ctrl Pts',(65.1354671986791,7.23332581609401,68.864928317118));
#156101=CARTESIAN_POINT('Ctrl Pts',(65.1294770804791,7.22770562585001,68.835657331627));
#156102=CARTESIAN_POINT('Ctrl Pts',(65.1139917221791,7.22505393909401,68.750209130564));
#156103=CARTESIAN_POINT('Ctrl Pts',(65.0969965161891,7.29236458022901,68.598587674286));
#156104=CARTESIAN_POINT('Ctrl Pts',(65.0980562425391,7.48320689487401,68.396834377415));
#156105=CARTESIAN_POINT('Ctrl Pts',(65.1318622502191,7.77841338606401,68.17529511025));
#156106=CARTESIAN_POINT('Ctrl Pts',(65.2058415077292,8.162694802716,67.943290382012));
#156107=CARTESIAN_POINT('Ctrl Pts',(65.3281701944691,8.62651876980101,67.706454494588));
#156108=CARTESIAN_POINT('Ctrl Pts',(65.5107146763692,9.164189148054,67.471184229534));
#156109=CARTESIAN_POINT('Ctrl Pts',(65.7734920352691,9.77549192354001,67.247471406371));
#156110=CARTESIAN_POINT('Ctrl Pts',(66.0530479496791,10.28489480299,67.107115610461));
#156111=CARTESIAN_POINT('Ctrl Pts',(66.2497491622091,10.58326737122,67.053678484145));
#156112=CARTESIAN_POINT('Ctrl Pts',(66.3066656472291,10.6654284307,67.041691621389));
#156113=CARTESIAN_POINT('Ctrl Pts',(65.3531725036091,6.23131392019301,68.896248006187));
#156114=CARTESIAN_POINT('Ctrl Pts',(65.3364173605091,6.22224999202201,68.829802444975));
#156115=CARTESIAN_POINT('Ctrl Pts',(65.2987026046291,6.21733947843101,68.629745175412));
#156116=CARTESIAN_POINT('Ctrl Pts',(65.2998749919591,6.32804692909301,68.289669040376));
#156117=CARTESIAN_POINT('Ctrl Pts',(65.3867416400291,6.59893950037902,67.955205029451));
#156118=CARTESIAN_POINT('Ctrl Pts',(65.5289413574991,6.963178463889,67.689963037335));
#156119=CARTESIAN_POINT('Ctrl Pts',(65.7105984378291,7.39528975498902,67.480895256793));
#156120=CARTESIAN_POINT('Ctrl Pts',(65.9274201532491,7.88574182335501,67.318555940622));
#156121=CARTESIAN_POINT('Ctrl Pts',(66.1805132539291,8.43004104598201,67.201907098975));
#156122=CARTESIAN_POINT('Ctrl Pts',(66.4748259827891,9.02738931413101,67.1383118873611));
#156123=CARTESIAN_POINT('Ctrl Pts',(66.7283333062591,9.50831205247101,67.145082394149));
#156124=CARTESIAN_POINT('Ctrl Pts',(66.8808520355891,9.78320319603901,67.176998428673));
#156125=CARTESIAN_POINT('Ctrl Pts',(66.9231537246591,9.85837183611702,67.188078156507));
#156126=CARTESIAN_POINT('Ctrl Pts',(64.7343817516392,5.43913593756802,69.101455710263));
#156127=CARTESIAN_POINT('Ctrl Pts',(64.7040334588792,5.42734943357101,68.98332816162));
#156128=CARTESIAN_POINT('Ctrl Pts',(64.6365286033291,5.42065311994001,68.626582976925));
#156129=CARTESIAN_POINT('Ctrl Pts',(64.6456736852991,5.56566954154801,68.022721853925));
#156130=CARTESIAN_POINT('Ctrl Pts',(64.8151082091391,5.89984883734601,67.450048284848));
#156131=CARTESIAN_POINT('Ctrl Pts',(65.0795393031391,6.31866400387401,67.020711466353));
#156132=CARTESIAN_POINT('Ctrl Pts',(65.4049285112791,6.78858899120402,66.7054392210471));
#156133=CARTESIAN_POINT('Ctrl Pts',(65.7795850174191,7.30009290101001,66.483489253098));
#156134=CARTESIAN_POINT('Ctrl Pts',(66.2008884135791,7.84963280449501,66.350252627375));
#156135=CARTESIAN_POINT('Ctrl Pts',(66.6704436566291,8.43594881492901,66.316098737405));
#156136=CARTESIAN_POINT('Ctrl Pts',(67.0534415061091,8.89435551247002,66.38593021354));
#156137=CARTESIAN_POINT('Ctrl Pts',(67.2723705023591,9.15068253749601,66.469885980898));
#156138=CARTESIAN_POINT('Ctrl Pts',(67.3321395401491,9.22032305887401,66.49638480121));
#156139=CARTESIAN_POINT('Ctrl Pts',(63.7340191659991,5.43918737470401,69.329686286193));
#156140=CARTESIAN_POINT('Ctrl Pts',(63.6972430465491,5.42740104748701,69.183365038754));
#156141=CARTESIAN_POINT('Ctrl Pts',(63.6142885536191,5.42070484981102,68.743047328557));
#156142=CARTESIAN_POINT('Ctrl Pts',(63.6153500447691,5.56571904369301,67.994001054187));
#156143=CARTESIAN_POINT('Ctrl Pts',(63.8034109289491,5.89989423020201,67.252746616459));
#156144=CARTESIAN_POINT('Ctrl Pts',(64.1140486792091,6.31870585302701,66.659562539042));
#156145=CARTESIAN_POINT('Ctrl Pts',(64.5135549538991,6.78862838506501,66.187024096085));
#156146=CARTESIAN_POINT('Ctrl Pts',(64.9933506135291,7.30013092794801,65.815180970113));
#156147=CARTESIAN_POINT('Ctrl Pts',(65.5568606915191,7.84967049114902,65.542342403844));
#156148=CARTESIAN_POINT('Ctrl Pts',(66.2165303374391,8.435987217921,65.385308796823));
#156149=CARTESIAN_POINT('Ctrl Pts',(66.7893586421791,8.89439537745801,65.387774578562));
#156150=CARTESIAN_POINT('Ctrl Pts',(67.1364669795991,9.150723607877,65.452197942192));
#156151=CARTESIAN_POINT('Ctrl Pts',(67.2329438191191,9.22036448820301,65.475132507639));
#156152=CARTESIAN_POINT('Ctrl Pts',(66.371936433707,10.2467129746685,67.0703492004296));
#156153=CARTESIAN_POINT('Ctrl Pts',(66.8232876390597,9.66024242196376,66.9907827752467));
#156154=CARTESIAN_POINT('Ctrl Pts',(67.0909397415809,9.20580207491112,66.4655776203965));
#156155=CARTESIAN_POINT('Ctrl Pts',(67.0545035358591,9.08849833454501,65.731481575833));
#156156=CARTESIAN_POINT('Ctrl Pts',(65.1202128309596,6.80865448650755,68.513745885506));
#156157=CARTESIAN_POINT('Ctrl Pts',(65.1130248862952,6.77887522935553,68.4292572074512));
#156158=CARTESIAN_POINT('Ctrl Pts',(65.1062988116738,6.74993122712072,68.33221079615));
#156159=CARTESIAN_POINT('Ctrl Pts',(65.0995328946409,6.72719707959995,68.2212988484916));
#156160=CARTESIAN_POINT('Ctrl Pts',(65.1274618024618,6.68337652285334,68.6491891342771));
#156161=CARTESIAN_POINT('Ctrl Pts',(65.126315892328,6.67628535290415,68.642690355055));
#156162=CARTESIAN_POINT('Ctrl Pts',(65.1220591440704,6.65062009337786,68.6185491365772));
#156163=CARTESIAN_POINT('Ctrl Pts',(65.1140119965792,6.60634594809702,68.5729114948953));
#156164=CARTESIAN_POINT('Ctrl Pts',(65.1025845774915,6.55116777440088,68.5081033809057));
#156165=CARTESIAN_POINT('Ctrl Pts',(65.0894146357107,6.4956542873541,68.4334129294739));
#156166=CARTESIAN_POINT('Ctrl Pts',(65.0743938717168,6.44075786056385,68.3482259437502));
#156167=CARTESIAN_POINT('Ctrl Pts',(65.0573886353781,6.38738124122978,68.2517844560535));
#156168=CARTESIAN_POINT('Ctrl Pts',(65.0382437566995,6.33645081793974,68.1432084536717));
#156169=CARTESIAN_POINT('Ctrl Pts',(65.0167679466859,6.28886673138934,68.0214130827762));
#156170=CARTESIAN_POINT('Ctrl Pts',(64.9927178237894,6.24591318747231,67.8850180580309));
#156171=CARTESIAN_POINT('Ctrl Pts',(64.9659407425506,6.20937832800507,67.7331576840355));
#156172=CARTESIAN_POINT('Ctrl Pts',(64.9362912819956,6.18123465571579,67.5650072374273));
#156173=CARTESIAN_POINT('Ctrl Pts',(64.9046232778813,6.16401422306796,67.3854090614244));
#156174=CARTESIAN_POINT('Ctrl Pts',(64.8827743055232,6.16046240900282,67.2614973817191));
#156175=CARTESIAN_POINT('Ctrl Pts',(64.8718037269095,6.16067826099719,67.1992801386775));
#156176=CARTESIAN_POINT('Ctrl Pts',(65.1139076006613,6.75398795634377,68.5745299318079));
#156177=CARTESIAN_POINT('Ctrl Pts',(65.1128680951615,6.74755527937897,68.5686346008803));
#156178=CARTESIAN_POINT('Ctrl Pts',(65.1089989141607,6.72422559008582,68.5466913710057));
#156179=CARTESIAN_POINT('Ctrl Pts',(65.1016377391522,6.68371527314676,68.5049440839871));
#156180=CARTESIAN_POINT('Ctrl Pts',(65.0911145206383,6.63289255144576,68.4452639420414));
#156181=CARTESIAN_POINT('Ctrl Pts',(65.078906346136,6.58142138067483,68.3760279451778));
#156182=CARTESIAN_POINT('Ctrl Pts',(65.0648965972843,6.53020896520135,68.2965747108642));
#156183=CARTESIAN_POINT('Ctrl Pts',(65.0489433373531,6.4801225724662,68.2060992779522));
#156184=CARTESIAN_POINT('Ctrl Pts',(65.030876566461,6.43204858405808,68.103637528625));
#156185=CARTESIAN_POINT('Ctrl Pts',(65.0105047539925,6.38690098578241,67.9881032389442));
#156186=CARTESIAN_POINT('Ctrl Pts',(64.9876158486021,6.34601386199286,67.8582938059316));
#156187=CARTESIAN_POINT('Ctrl Pts',(64.9620427523565,6.31111285615102,67.713261570135));
#156188=CARTESIAN_POINT('Ctrl Pts',(64.9336316898486,6.28413266453705,67.5521344278609));
#156189=CARTESIAN_POINT('Ctrl Pts',(64.9031552466415,6.26755013237094,67.3792939295652));
#156190=CARTESIAN_POINT('Ctrl Pts',(64.8820795473119,6.26412038407241,67.2597676991259));
#156191=CARTESIAN_POINT('Ctrl Pts',(64.8714878273221,6.26432875241371,67.1996990701106));
#156192=CARTESIAN_POINT('Ctrl Pts',(65.1161939756686,6.82410170851579,68.4976206638588));
#156193=CARTESIAN_POINT('Ctrl Pts',(65.1152601248451,6.81832288336551,68.4923245280203));
#156194=CARTESIAN_POINT('Ctrl Pts',(65.1117757794614,6.79731230281174,68.4725637949535));
#156195=CARTESIAN_POINT('Ctrl Pts',(65.1050957420854,6.7605392861161,68.4346794427211));
#156196=CARTESIAN_POINT('Ctrl Pts',(65.0954703511864,6.71404131844838,68.3800911300056));
#156197=CARTESIAN_POINT('Ctrl Pts',(65.0842171652642,6.66658397302499,68.3162711437924));
#156198=CARTESIAN_POINT('Ctrl Pts',(65.0712113057501,6.61902960333383,68.2425112484398));
#156199=CARTESIAN_POINT('Ctrl Pts',(65.056302607718,6.57221024712437,68.1579598205501));
#156200=CARTESIAN_POINT('Ctrl Pts',(65.0393063459266,6.52697256096236,68.0615692299884));
#156201=CARTESIAN_POINT('Ctrl Pts',(65.0200307498421,6.48424427818018,67.9522518923636));
#156202=CARTESIAN_POINT('Ctrl Pts',(64.9982948775005,6.44540901003979,67.8289816347201));
#156203=CARTESIAN_POINT('Ctrl Pts',(64.9739172803584,6.41213034214683,67.69072941125));
#156204=CARTESIAN_POINT('Ctrl Pts',(64.9467358874593,6.38630543079974,67.536576071874));
#156205=CARTESIAN_POINT('Ctrl Pts',(64.9174426068361,6.37035630308492,67.3704456220308));
#156206=CARTESIAN_POINT('Ctrl Pts',(64.8971347303756,6.36704776021286,67.2552739314699));
#156207=CARTESIAN_POINT('Ctrl Pts',(64.8869191987505,6.36724869764713,67.1973387726862));
#156208=CARTESIAN_POINT('Ctrl Pts',(65.1346705530482,6.8919798904543,68.4202960166216));
#156209=CARTESIAN_POINT('Ctrl Pts',(65.1338389881117,6.88683406911642,68.4155799705943));
#156210=CARTESIAN_POINT('Ctrl Pts',(65.1307272078985,6.86806865274327,68.3979321456351));
#156211=CARTESIAN_POINT('Ctrl Pts',(65.1247065901473,6.83491377283282,68.3637875588852));
#156212=CARTESIAN_POINT('Ctrl Pts',(65.1159503997161,6.79260266483268,68.3141287229154));
#156213=CARTESIAN_POINT('Ctrl Pts',(65.1056217526552,6.74903116432229,68.2555520583749));
#156214=CARTESIAN_POINT('Ctrl Pts',(65.0935877735642,6.70501820397611,68.187303970419));
#156215=CARTESIAN_POINT('Ctrl Pts',(65.0796903316755,6.66136171514741,68.1084876612219));
#156216=CARTESIAN_POINT('Ctrl Pts',(65.0637304459047,6.61886989600768,68.0179746511137));
#156217=CARTESIAN_POINT('Ctrl Pts',(65.0455161134506,6.57848378907752,67.9146760386274));
#156218=CARTESIAN_POINT('Ctrl Pts',(65.0248965098102,6.54163495336659,67.7977364553764));
#156219=CARTESIAN_POINT('Ctrl Pts',(65.0016762933978,6.5099268953333,67.6660480641928));
#156220=CARTESIAN_POINT('Ctrl Pts',(64.9756853622109,6.48522042825308,67.5186461686814));
#156221=CARTESIAN_POINT('Ctrl Pts',(64.9475375191463,6.46988450894962,67.3590118180421));
#156222=CARTESIAN_POINT('Ctrl Pts',(64.9279729835967,6.46669330688071,67.248055823275));
#156223=CARTESIAN_POINT('Ctrl Pts',(64.9181216456063,6.4668870503417,67.1921861092301));
#156224=CARTESIAN_POINT('Origin',(73.9901844080691,1.4210854715202E-14,
64.203906618088));
#156225=CARTESIAN_POINT('Origin',(82.8534541851791,15.33010667085,62.64107301909));
#156226=CARTESIAN_POINT('Ctrl Pts',(82.0542997835692,10.29865851118,58.26471983769));
#156227=CARTESIAN_POINT('Ctrl Pts',(82.0527395465391,10.17603905197,58.16140352547));
#156228=CARTESIAN_POINT('Ctrl Pts',(82.0492308291891,9.89812303372602,57.92115839559));
#156229=CARTESIAN_POINT('Ctrl Pts',(82.0458365166991,9.61603810345401,57.66377166706));
#156230=CARTESIAN_POINT('Ctrl Pts',(82.043988738869,9.45484011582801,57.51238781076));
#156231=CARTESIAN_POINT('Ctrl Pts',(82.0438796852591,9.44529764517503,57.50341116586));
#156232=CARTESIAN_POINT('Ctrl Pts',(83.0679041040991,10.31054165842,58.07143591329));
#156233=CARTESIAN_POINT('Ctrl Pts',(83.0680728911292,10.18085680913,57.97675228206));
#156234=CARTESIAN_POINT('Ctrl Pts',(83.0680970000191,9.88587567699001,57.7562458923));
#156235=CARTESIAN_POINT('Ctrl Pts',(83.0672361907791,9.58406728388101,57.51926185832));
#156236=CARTESIAN_POINT('Ctrl Pts',(83.066405906709,9.41081340331201,57.37964988205));
#156237=CARTESIAN_POINT('Ctrl Pts',(83.0663555479991,9.40055449126001,57.37137050065));
#156238=CARTESIAN_POINT('Ctrl Pts',(83.8273697495491,9.80641462172301,58.55513154362));
#156239=CARTESIAN_POINT('Ctrl Pts',(83.8191676863491,9.66631332335401,58.46273485692));
#156240=CARTESIAN_POINT('Ctrl Pts',(83.7993625846091,9.34764672538402,58.24737311026));
#156241=CARTESIAN_POINT('Ctrl Pts',(83.7762983997391,9.02178381289601,58.01556464493));
#156242=CARTESIAN_POINT('Ctrl Pts',(83.7620427416892,8.83486184555501,57.87891342746));
#156243=CARTESIAN_POINT('Ctrl Pts',(83.7611950253791,8.82379411820401,57.87080933309));
#156244=CARTESIAN_POINT('Ctrl Pts',(83.769884078649,9.15986779421601,59.35735731505));
#156245=CARTESIAN_POINT('Ctrl Pts',(83.749414626619,9.013718243092,59.25920706419));
#156246=CARTESIAN_POINT('Ctrl Pts',(83.701112991309,8.68229827316202,59.03058335385));
#156247=CARTESIAN_POINT('Ctrl Pts',(83.6475626740491,8.345875722854,58.7848879037501));
#156248=CARTESIAN_POINT('Ctrl Pts',(83.615387835479,8.15380240182902,58.64019221211));
#156249=CARTESIAN_POINT('Ctrl Pts',(83.6134776020891,8.14243286917001,58.63161152939));
#156250=CARTESIAN_POINT('',(82.344504931983,9.5242671557599,57.5877992215605));
#156251=CARTESIAN_POINT('Origin',(82.1588614728291,8.53712723764301,58.70184199751));
#156252=CARTESIAN_POINT('Ctrl Pts',(82.3525639851769,10.1662213565488,58.1365166381844));
#156253=CARTESIAN_POINT('Ctrl Pts',(82.3515337760017,10.0806860329839,58.0663217283825));
#156254=CARTESIAN_POINT('Ctrl Pts',(82.3504894170264,9.99561838305282,57.9953267882541));
#156255=CARTESIAN_POINT('Ctrl Pts',(82.3494344128164,9.91100184699888,57.9235752783107));
#156256=CARTESIAN_POINT('Ctrl Pts',(82.3478142322361,9.78105538119467,57.8133857625485));
#156257=CARTESIAN_POINT('Ctrl Pts',(82.3461689438681,9.65217281892513,57.7014119551773));
#156258=CARTESIAN_POINT('Ctrl Pts',(82.3445049357179,9.52426717547808,57.5877992022325));
#156259=CARTESIAN_POINT('Ctrl Pts',(86.9329409753791,9.92711979712301,57.78576952332));
#156260=CARTESIAN_POINT('Ctrl Pts',(84.0933088102591,7.69990047565403,57.4110459375501));
#156261=CARTESIAN_POINT('Ctrl Pts',(81.3965784204092,6.58687843438301,55.21311191528));
#156262=CARTESIAN_POINT('Ctrl Pts',(79.8215157765191,7.02960519183701,51.92060906182));
#156263=CARTESIAN_POINT('Ctrl Pts',(86.0676469660691,10.68513943961,58.23629022148));
#156264=CARTESIAN_POINT('Ctrl Pts',(83.4591950453992,8.38530844920902,57.7160304338599));
#156265=CARTESIAN_POINT('Ctrl Pts',(80.9461889541891,7.20824339431001,55.52843468871));
#156266=CARTESIAN_POINT('Ctrl Pts',(79.3859501752991,7.59165105783701,52.36111905021));
#156267=CARTESIAN_POINT('Ctrl Pts',(85.1070801027791,11.36198787766,58.71079233602));
#156268=CARTESIAN_POINT('Ctrl Pts',(82.7291098543491,9.03120774616101,58.05826770049));
#156269=CARTESIAN_POINT('Ctrl Pts',(80.4097867402391,7.80241333656101,55.88012561213));
#156270=CARTESIAN_POINT('Ctrl Pts',(78.8911987758591,8.10248660419701,52.82351298253));
#156271=CARTESIAN_POINT('Ctrl Pts',(84.0404926560891,11.95793977738,59.19105334214));
#156272=CARTESIAN_POINT('Ctrl Pts',(81.888874467589,9.61731046456401,58.42277593509));
#156273=CARTESIAN_POINT('Ctrl Pts',(79.7722632969191,8.34598753659601,56.2503969924101));
#156274=CARTESIAN_POINT('Ctrl Pts',(78.3268882647691,8.55715030996601,53.28427687186));
#156275=CARTESIAN_POINT('Origin',(70.1855769158814,-19.4157022285867,61.5812032484374));
#156276=CARTESIAN_POINT('Ctrl Pts',(82.6104235887092,9.668870107941,57.81364808779));
#156277=CARTESIAN_POINT('Ctrl Pts',(82.5689416191891,9.68513702138402,57.82096247823));
#156278=CARTESIAN_POINT('Ctrl Pts',(82.4031385785191,9.74979208676402,57.8501980277801));
#156279=CARTESIAN_POINT('Ctrl Pts',(82.1234598163291,9.85639317719102,57.89951293949));
#156280=CARTESIAN_POINT('Ctrl Pts',(81.8843680682591,9.94447157893201,57.94167126554));
#156281=CARTESIAN_POINT('Ctrl Pts',(81.7702786897492,9.98579912464201,57.9617883011801));
#156282=CARTESIAN_POINT('Ctrl Pts',(82.3934669688891,9.34863157848701,57.29542335185));
#156283=CARTESIAN_POINT('Ctrl Pts',(82.3523805149492,9.36474339264802,57.30266800222));
#156284=CARTESIAN_POINT('Ctrl Pts',(82.1881643280692,9.42877964864201,57.33162374664));
#156285=CARTESIAN_POINT('Ctrl Pts',(81.9112013668991,9.53434541009101,57.38045978935));
#156286=CARTESIAN_POINT('Ctrl Pts',(81.6744751240489,9.62155226794001,57.42220101301));
#156287=CARTESIAN_POINT('Ctrl Pts',(81.5615236720891,9.66246761273101,57.4421174015));
#156288=CARTESIAN_POINT('Ctrl Pts',(82.1383565513191,8.79415897984801,57.08174467046));
#156289=CARTESIAN_POINT('Ctrl Pts',(82.0979549073891,8.81000224948801,57.08886857035));
#156290=CARTESIAN_POINT('Ctrl Pts',(81.9364862566791,8.87296707647901,57.11733985001));
#156291=CARTESIAN_POINT('Ctrl Pts',(81.6642255318591,8.97674023180402,57.16534676158));
#156292=CARTESIAN_POINT('Ctrl Pts',(81.4315950105091,9.06243806696601,57.20636579903));
#156293=CARTESIAN_POINT('Ctrl Pts',(81.3206138058091,9.10263971214401,57.22593477977));
#156294=CARTESIAN_POINT('Ctrl Pts',(81.9360321987691,8.20310657683102,57.24878262946));
#156295=CARTESIAN_POINT('Ctrl Pts',(81.8963605433192,8.21866358546402,57.25577781268));
#156296=CARTESIAN_POINT('Ctrl Pts',(81.7378206899191,8.28048629887201,57.28373266636));
#156297=CARTESIAN_POINT('Ctrl Pts',(81.4705724185491,8.38234858581402,57.33085574715));
#156298=CARTESIAN_POINT('Ctrl Pts',(81.2423078226591,8.46643784466801,57.37110495414));
#156299=CARTESIAN_POINT('Ctrl Pts',(81.1334268468591,8.50587870586502,57.39030360786));
#156300=CARTESIAN_POINT('Origin',(81.6278425866092,8.7374636884277,58.7954749599595));
#156301=CARTESIAN_POINT('Origin',(82.1588614744491,8.53712721516301,58.70184200705));
#156302=CARTESIAN_POINT('Origin',(82.1588614745091,8.53712721530601,58.70184200704));
#156303=CARTESIAN_POINT('Ctrl Pts',(82.2180760363191,10.03116305045,58.28208546212));
#156304=CARTESIAN_POINT('Ctrl Pts',(81.6448173157991,10.2499782811,58.38316644148));
#156305=CARTESIAN_POINT('Ctrl Pts',(80.4077005984991,10.6384119469,58.60130349702));
#156306=CARTESIAN_POINT('Ctrl Pts',(78.4208211301491,11.08801271783,58.95164395471));
#156307=CARTESIAN_POINT('Ctrl Pts',(76.1569665443491,11.42116381224,59.35082259858));
#156308=CARTESIAN_POINT('Ctrl Pts',(73.6216993183591,11.58264138134,59.79785861383));
#156309=CARTESIAN_POINT('Ctrl Pts',(70.9781759552091,11.49327700734,60.26398310689));
#156310=CARTESIAN_POINT('Ctrl Pts',(68.4543146920692,11.16992459859,60.70900794314));
#156311=CARTESIAN_POINT('Ctrl Pts',(66.2334199597191,10.69349906036,61.10061160577));
#156312=CARTESIAN_POINT('Ctrl Pts',(64.8647467245591,10.27221430314,61.3419456249));
#156313=CARTESIAN_POINT('Ctrl Pts',(64.2333895001991,10.03126768975,61.45327093802));
#156314=CARTESIAN_POINT('Ctrl Pts',(82.0018799307291,9.82226387024801,57.50799734594));
#156315=CARTESIAN_POINT('Ctrl Pts',(81.436977430279,10.03788714144,57.60760489824));
#156316=CARTESIAN_POINT('Ctrl Pts',(80.2133909429991,10.4222367679,57.8233562091799));
#156317=CARTESIAN_POINT('Ctrl Pts',(78.2425568897692,10.86825463521,58.1708674272599));
#156318=CARTESIAN_POINT('Ctrl Pts',(75.9954429246891,11.19894300459,58.56709424803));
#156319=CARTESIAN_POINT('Ctrl Pts',(73.4796033119692,11.3591631631,59.01070465089));
#156320=CARTESIAN_POINT('Ctrl Pts',(70.8569091407191,11.27051736571,59.47315639543));
#156321=CARTESIAN_POINT('Ctrl Pts',(68.3515547785591,10.94955172405,59.9149179657099));
#156322=CARTESIAN_POINT('Ctrl Pts',(66.1481091383991,10.47682179375,60.3034448826));
#156323=CARTESIAN_POINT('Ctrl Pts',(64.7939462302891,10.05980065435,60.54222033957));
#156324=CARTESIAN_POINT('Ctrl Pts',(64.1717857210691,9.82236564017501,60.65192402368));
#156325=CARTESIAN_POINT('Ctrl Pts',(81.6812403517491,9.15894488521401,57.12486504907));
#156326=CARTESIAN_POINT('Ctrl Pts',(81.142871413649,9.36443270586001,57.21979401843));
#156327=CARTESIAN_POINT('Ctrl Pts',(79.9622475576091,9.73581425448101,57.42796985832));
#156328=CARTESIAN_POINT('Ctrl Pts',(78.0423626199291,10.17045530359,57.76649737269));
#156329=CARTESIAN_POINT('Ctrl Pts',(75.8484052614891,10.49332376545,58.1533512495));
#156330=CARTESIAN_POINT('Ctrl Pts',(73.3942542810591,10.64955125961,58.58608428209));
#156331=CARTESIAN_POINT('Ctrl Pts',(70.8376991842391,10.56318716341,59.03687392332));
#156332=CARTESIAN_POINT('Ctrl Pts',(68.3911099103691,10.24980023947,59.46827362302));
#156333=CARTESIAN_POINT('Ctrl Pts',(66.2430704911391,9.78880499814102,59.84703092825));
#156334=CARTESIAN_POINT('Ctrl Pts',(64.9349823229891,9.38532215333301,60.07768216544));
#156335=CARTESIAN_POINT('Ctrl Pts',(64.3420242057991,9.15903754398101,60.18223667994));
#156336=CARTESIAN_POINT('Ctrl Pts',(81.4283134430791,8.39735189262101,57.33839798192));
#156337=CARTESIAN_POINT('Ctrl Pts',(80.9204091465791,8.59120264529501,57.427955213));
#156338=CARTESIAN_POINT('Ctrl Pts',(79.7891130493291,8.94769483083601,57.62743323812));
#156339=CARTESIAN_POINT('Ctrl Pts',(77.9277255921291,9.36927352953802,57.95564606838));
#156340=CARTESIAN_POINT('Ctrl Pts',(75.7948002560491,9.68316352566601,58.33173835296));
#156341=CARTESIAN_POINT('Ctrl Pts',(73.4114773856891,9.83480682238501,58.75198247875));
#156342=CARTESIAN_POINT('Ctrl Pts',(70.9308601961991,9.75106247277001,59.18938221806));
#156343=CARTESIAN_POINT('Ctrl Pts',(68.5517423507991,9.44637709127401,59.60888488449));
#156344=CARTESIAN_POINT('Ctrl Pts',(66.4673178597791,8.99885509146401,59.97642516151));
#156345=CARTESIAN_POINT('Ctrl Pts',(65.2121306335291,8.61091630694802,60.19774853534));
#156346=CARTESIAN_POINT('Ctrl Pts',(64.6527013880191,8.39743409036201,60.29639100512));
#156347=CARTESIAN_POINT('Ctrl Pts',(61.7087960388091,8.96199616764401,62.51282737052));
#156348=CARTESIAN_POINT('Ctrl Pts',(61.5698609821491,8.91295132180802,62.53238444947));
#156349=CARTESIAN_POINT('Ctrl Pts',(61.1109287379191,8.72474172236301,62.56944688524));
#156350=CARTESIAN_POINT('Ctrl Pts',(60.4269254807791,8.28965318991802,62.48943246867));
#156351=CARTESIAN_POINT('Ctrl Pts',(59.7821496029791,7.65995478656001,62.25896894211));
#156352=CARTESIAN_POINT('Ctrl Pts',(59.2815963525391,6.95212687654301,61.95938522881));
#156353=CARTESIAN_POINT('Ctrl Pts',(58.9002308413891,6.18282381217201,61.63205504275));
#156354=CARTESIAN_POINT('Ctrl Pts',(58.6155144813491,5.36332168350501,61.30598232287));
#156355=CARTESIAN_POINT('Ctrl Pts',(58.4087775349091,4.50277795774501,61.00312960765));
#156356=CARTESIAN_POINT('Ctrl Pts',(58.2676967409091,3.62424267013002,60.74495621511));
#156357=CARTESIAN_POINT('Ctrl Pts',(58.1753682422591,2.74535586735901,60.54030188331));
#156358=CARTESIAN_POINT('Ctrl Pts',(58.1174070039491,1.87206366585901,60.39022014666));
#156359=CARTESIAN_POINT('Ctrl Pts',(58.0841999562791,0.989209384080914,
60.29379447098));
#156360=CARTESIAN_POINT('Ctrl Pts',(58.0717192608791,0.0853586380197842,
60.2552299176));
#156361=CARTESIAN_POINT('Ctrl Pts',(58.0803412997091,-0.831619754236286,
60.28202412771));
#156362=CARTESIAN_POINT('Ctrl Pts',(58.1108074737091,-1.74388438871099,
60.37189799022));
#156363=CARTESIAN_POINT('Ctrl Pts',(58.1669615502191,-2.64765037633299,
60.5200731035));
#156364=CARTESIAN_POINT('Ctrl Pts',(58.2577587898791,-3.54868473576899,
60.72473754248));
#156365=CARTESIAN_POINT('Ctrl Pts',(58.3963509815491,-4.43903040165999,
60.98262707975));
#156366=CARTESIAN_POINT('Ctrl Pts',(58.5992125823491,-5.30768633024999,
61.28480916086));
#156367=CARTESIAN_POINT('Ctrl Pts',(58.8815263867091,-6.14095307104199,
61.61377902874));
#156368=CARTESIAN_POINT('Ctrl Pts',(59.2649866104491,-6.92834051674799,
61.94813791472));
#156369=CARTESIAN_POINT('Ctrl Pts',(59.773271127289,-7.65220305320499,62.25525822907));
#156370=CARTESIAN_POINT('Ctrl Pts',(60.4252820987391,-8.28925777980099,
62.48909095077));
#156371=CARTESIAN_POINT('Ctrl Pts',(61.1127782067391,-8.72598511128199,
62.56959587775));
#156372=CARTESIAN_POINT('Ctrl Pts',(61.5738723051191,-8.91455013048699,
62.53200605257));
#156373=CARTESIAN_POINT('Ctrl Pts',(61.7139245147291,-8.96379447908499,
62.51210995553));
#156374=CARTESIAN_POINT('Ctrl Pts',(61.4014954127191,9.08520596155202,61.44355402681));
#156375=CARTESIAN_POINT('Ctrl Pts',(61.2874245509091,9.03447923019001,61.4557756009));
#156376=CARTESIAN_POINT('Ctrl Pts',(60.9113316065891,8.83990361344802,61.47142631459));
#156377=CARTESIAN_POINT('Ctrl Pts',(60.3635251517091,8.39116201973901,61.3726104982501));
#156378=CARTESIAN_POINT('Ctrl Pts',(59.8745335491291,7.74580293368701,61.1432506871));
#156379=CARTESIAN_POINT('Ctrl Pts',(59.5187165013191,7.02447848409401,60.86473236401));
#156380=CARTESIAN_POINT('Ctrl Pts',(59.2664503582991,6.24374560589701,60.57342906056));
#156381=CARTESIAN_POINT('Ctrl Pts',(59.0925079293791,5.41430300349301,60.29253180843));
#156382=CARTESIAN_POINT('Ctrl Pts',(58.9765709581791,4.54438927710501,60.03779198931));
#156383=CARTESIAN_POINT('Ctrl Pts',(58.9055501263191,3.65710613517001,59.82467118793));
#156384=CARTESIAN_POINT('Ctrl Pts',(58.8647365117791,2.77013317747901,59.65814889886));
#156385=CARTESIAN_POINT('Ctrl Pts',(58.8424267403291,1.88911579779101,59.53724171955));
#156386=CARTESIAN_POINT('Ctrl Pts',(58.8311370770591,0.998433591798714,
59.46001421541));
#156387=CARTESIAN_POINT('Ctrl Pts',(58.8271635470091,0.0861862617952542,
59.42918292181));
#156388=CARTESIAN_POINT('Ctrl Pts',(58.8298939128291,-0.839419159311286,
59.45060263904));
#156389=CARTESIAN_POINT('Ctrl Pts',(58.8400687909492,-1.75979619587999,
59.52253773544));
#156390=CARTESIAN_POINT('Ctrl Pts',(58.8612623367191,-2.67154027375999,
59.6417775984));
#156391=CARTESIAN_POINT('Ctrl Pts',(58.9009231731791,-3.58087193680299,
59.80813714535));
#156392=CARTESIAN_POINT('Ctrl Pts',(58.9699394424191,-4.47995913630899,
60.02071203588));
#156393=CARTESIAN_POINT('Ctrl Pts',(59.0828230394891,-5.35795511875899,
60.27448991099));
#156394=CARTESIAN_POINT('Ctrl Pts',(59.2543775458091,-6.20124022696799,
60.55739034192));
#156395=CARTESIAN_POINT('Ctrl Pts',(59.5072378683591,-7.00026261349998,
60.85443640342));
#156396=CARTESIAN_POINT('Ctrl Pts',(59.8681473241091,-7.73789838758098,
61.13963055899));
#156397=CARTESIAN_POINT('Ctrl Pts',(60.3625395629591,-8.39079064494998,
61.37219504624));
#156398=CARTESIAN_POINT('Ctrl Pts',(60.9130033575691,-8.84120300394399,
61.4715825305));
#156399=CARTESIAN_POINT('Ctrl Pts',(61.2907349696091,-9.03613393057798,
61.45558231608));
#156400=CARTESIAN_POINT('Ctrl Pts',(61.4056779384191,-9.08706366640399,
61.44311667414));
#156401=CARTESIAN_POINT('Ctrl Pts',(61.4950703228691,8.31092208497201,60.64082694368));
#156402=CARTESIAN_POINT('Ctrl Pts',(61.4312159626292,8.27076477997901,60.6487343305501));
#156403=CARTESIAN_POINT('Ctrl Pts',(61.2204907529791,8.11619494844401,60.66160281426));
#156404=CARTESIAN_POINT('Ctrl Pts',(60.9100092313592,7.75325290741801,60.6154933257301));
#156405=CARTESIAN_POINT('Ctrl Pts',(60.6250557980591,7.20630981348502,60.49825917921));
#156406=CARTESIAN_POINT('Ctrl Pts',(60.4105475875591,6.56980129168201,60.35139718058));
#156407=CARTESIAN_POINT('Ctrl Pts',(60.2524225307591,5.86089647420301,60.1946002338601));
#156408=CARTESIAN_POINT('Ctrl Pts',(60.1384273166791,5.09392251407701,60.04102312208));
#156409=CARTESIAN_POINT('Ctrl Pts',(60.0585750382691,4.28289242169001,59.90011699997));
#156410=CARTESIAN_POINT('Ctrl Pts',(60.0063644514191,3.45058317703301,59.78113651281));
#156411=CARTESIAN_POINT('Ctrl Pts',(59.9737925723191,2.61442581751901,59.68750227682));
#156412=CARTESIAN_POINT('Ctrl Pts',(59.9542782938691,1.78195555997801,59.61917753525));
#156413=CARTESIAN_POINT('Ctrl Pts',(59.9435187238791,0.940466160123215,
59.5754076490299));
#156414=CARTESIAN_POINT('Ctrl Pts',(59.9395507897191,0.0809852487515842,
59.5579178275));
#156415=CARTESIAN_POINT('Ctrl Pts',(59.9422878235992,-0.790405575204286,
59.57006912894));
#156416=CARTESIAN_POINT('Ctrl Pts',(59.9521077472891,-1.65980206921799,
59.61085229615));
#156417=CARTESIAN_POINT('Ctrl Pts',(59.9708950406291,-2.52140965667399,
59.67827203419));
#156418=CARTESIAN_POINT('Ctrl Pts',(60.0027925917991,-3.37859880572699,
59.7718627086));
#156419=CARTESIAN_POINT('Ctrl Pts',(60.0538703201391,-4.22275182898199,
59.89062455975));
#156420=CARTESIAN_POINT('Ctrl Pts',(60.1319776920891,-5.04205237106898,
60.03110652867));
#156421=CARTESIAN_POINT('Ctrl Pts',(60.2447516350391,-5.82237933191699,
60.1859093365));
#156422=CARTESIAN_POINT('Ctrl Pts',(60.4035221583791,-6.54828458384299,
60.3459287535699));
#156423=CARTESIAN_POINT('Ctrl Pts',(60.6212298628391,-7.19936558429799,
60.49639210435));
#156424=CARTESIAN_POINT('Ctrl Pts',(60.9093564390591,-7.75273048808598,
60.61529830059));
#156425=CARTESIAN_POINT('Ctrl Pts',(61.2213839640791,-8.11714240979298,
60.66168084203));
#156426=CARTESIAN_POINT('Ctrl Pts',(61.4330643448691,-8.27206824165498,
60.64859350648));
#156427=CARTESIAN_POINT('Ctrl Pts',(61.4974194310191,-8.31240654545798,
60.64053996861));
#156428=CARTESIAN_POINT('Ctrl Pts',(61.9120241061091,7.28038925473501,60.76944687017));
#156429=CARTESIAN_POINT('Ctrl Pts',(61.8821503623991,7.25429932373901,60.77963430154));
#156430=CARTESIAN_POINT('Ctrl Pts',(61.7823674356291,7.15297517676501,60.81065422848));
#156431=CARTESIAN_POINT('Ctrl Pts',(61.6137917373691,6.90422801766101,60.84510858475));
#156432=CARTESIAN_POINT('Ctrl Pts',(61.4121504854391,6.48827165090601,60.85816206592));
#156433=CARTESIAN_POINT('Ctrl Pts',(61.2184949050291,5.96464885584601,60.84451248097));
#156434=CARTESIAN_POINT('Ctrl Pts',(61.0415870949391,5.35134356838701,60.8093061866));
#156435=CARTESIAN_POINT('Ctrl Pts',(60.8870654269791,4.66751222387701,60.75975017414));
#156436=CARTESIAN_POINT('Ctrl Pts',(60.7586980174391,3.93485328170701,60.70412400929));
#156437=CARTESIAN_POINT('Ctrl Pts',(60.6584697311591,3.17571152466401,60.65040664119));
#156438=CARTESIAN_POINT('Ctrl Pts',(60.5840408165191,2.40718716616401,60.60405220122));
#156439=CARTESIAN_POINT('Ctrl Pts',(60.5321508919591,1.63933068233101,60.56817017024));
#156440=CARTESIAN_POINT('Ctrl Pts',(60.5000951126591,0.863314429042514,
60.54440849196));
#156441=CARTESIAN_POINT('Ctrl Pts',(60.4876265705191,0.0740629624246842,
60.5348192438));
#156442=CARTESIAN_POINT('Ctrl Pts',(60.4962630912091,-0.725170964130086,
60.54148410271));
#156443=CARTESIAN_POINT('Ctrl Pts',(60.5259583672891,-1.52671492447299,
60.56370151384));
#156444=CARTESIAN_POINT('Ctrl Pts',(60.5768864913491,-2.32159336911999,
60.59933252936));
#156445=CARTESIAN_POINT('Ctrl Pts',(60.6508232556691,-3.10938345906399,
60.64595591541));
#156446=CARTESIAN_POINT('Ctrl Pts',(60.7504561259491,-3.88042186138999,
60.70010021104));
#156447=CARTESIAN_POINT('Ctrl Pts',(60.8777899489991,-4.62160172951099,
60.75622372783));
#156448=CARTESIAN_POINT('Ctrl Pts',(61.0324428208391,-5.31813456813899,
60.80698833398));
#156449=CARTESIAN_POINT('Ctrl Pts',(61.2115567297791,-5.94672459764799,
60.84374971148));
#156450=CARTESIAN_POINT('Ctrl Pts',(61.4088325039591,-6.48260555515498,
60.85825867285));
#156451=CARTESIAN_POINT('Ctrl Pts',(61.6128711300591,-6.90350456565199,
60.84524579483));
#156452=CARTESIAN_POINT('Ctrl Pts',(61.7825260542691,-7.15345423815299,
60.81063341023));
#156453=CARTESIAN_POINT('Ctrl Pts',(61.8829864021391,-7.25513530438499,
60.77936984004));
#156454=CARTESIAN_POINT('Ctrl Pts',(61.9131707250991,-7.28137694577499,
60.76905604858));
#156455=CARTESIAN_POINT('Ctrl Pts',(61.7095776082786,7.4812853662219,60.7844468788789));
#156456=CARTESIAN_POINT('Ctrl Pts',(61.7024296496402,7.47450503376971,60.7857109678101));
#156457=CARTESIAN_POINT('Ctrl Pts',(61.695272550974,7.46752133842146,60.7869235202457));
#156458=CARTESIAN_POINT('Ctrl Pts',(61.6881101684676,7.46033339730234,60.7880836318459));
#156459=CARTESIAN_POINT('Ctrl Pts',(61.6590245873343,7.43114402569089,60.7927947066929));
#156460=CARTESIAN_POINT('Ctrl Pts',(61.6298535312315,7.39858369876268,60.7966388545209));
#156461=CARTESIAN_POINT('Ctrl Pts',(61.6006617256375,7.36260348904996,60.7996058924316));
#156462=CARTESIAN_POINT('Ctrl Pts',(61.574030746394,7.32977961267307,60.8023126494617));
#156463=CARTESIAN_POINT('Ctrl Pts',(61.5473819531278,7.29410881954576,60.8042896853198));
#156464=CARTESIAN_POINT('Ctrl Pts',(61.5207555108983,7.2555898731445,60.8055486610889));
#156465=CARTESIAN_POINT('Ctrl Pts',(61.4962099300207,7.22008118948105,60.8067092476704));
#156466=CARTESIAN_POINT('Ctrl Pts',(61.4716829270121,7.18215149477169,60.8072596358207));
#156467=CARTESIAN_POINT('Ctrl Pts',(61.4472044231664,7.14184100557662,60.8072246296821));
#156468=CARTESIAN_POINT('Ctrl Pts',(61.4451292482964,7.13842366787081,60.8072216620228));
#156469=CARTESIAN_POINT('Ctrl Pts',(61.4430544231896,7.13498924959679,60.8072144974086));
#156470=CARTESIAN_POINT('Ctrl Pts',(61.4409799670258,7.13153779272376,60.8072031568315));
#156471=CARTESIAN_POINT('Ctrl Pts',(61.422576200912,7.10091781330252,60.8071025476531));
#156472=CARTESIAN_POINT('Ctrl Pts',(61.4042017000976,7.06895632298682,60.8066731820066));
#156473=CARTESIAN_POINT('Ctrl Pts',(61.3858482097925,7.03562826129724,60.8059072099783));
#156474=CARTESIAN_POINT('Ctrl Pts',(61.3612550949187,6.99096967941299,60.8048808309207));
#156475=CARTESIAN_POINT('Ctrl Pts',(61.3367290240724,6.94388825664927,60.8032499783446));
#156476=CARTESIAN_POINT('Ctrl Pts',(61.3123007852604,6.89435212608218,60.8010138805843));
#156477=CARTESIAN_POINT('Ctrl Pts',(61.2895289115423,6.84817480980348,60.798929402198));
#156478=CARTESIAN_POINT('Ctrl Pts',(61.2668420760223,6.79986414868234,60.7963188407643));
#156479=CARTESIAN_POINT('Ctrl Pts',(61.2442627728364,6.74943669867008,60.7931994062268));
#156480=CARTESIAN_POINT('Ctrl Pts',(61.2381450042524,6.7357735901624,60.7923542083721));
#156481=CARTESIAN_POINT('Ctrl Pts',(61.2320351136504,6.72195535069831,60.7914717671107));
#156482=CARTESIAN_POINT('Ctrl Pts',(61.225933508814,6.70798293461504,60.7905526945646));
#156483=CARTESIAN_POINT('Ctrl Pts',(61.2225114659508,6.70014660171226,60.790037239085));
#156484=CARTESIAN_POINT('Ctrl Pts',(61.2190919756263,6.69226105550839,60.7895102588224));
#156485=CARTESIAN_POINT('Ctrl Pts',(61.2156751295169,6.68432665296964,60.7889718818205));
#156486=CARTESIAN_POINT('Ctrl Pts',(61.1927425927241,6.63107404154833,60.785358505622));
#156487=CARTESIAN_POINT('Ctrl Pts',(61.169929987531,6.5756185258231,60.7812308129325));
#156488=CARTESIAN_POINT('Ctrl Pts',(61.1472630227814,6.51795609966164,60.7765797129808));
#156489=CARTESIAN_POINT('Ctrl Pts',(61.1342409018793,6.48482916390821,60.7739076663893));
#156490=CARTESIAN_POINT('Ctrl Pts',(61.1212670116287,6.45097431756662,60.7710631438124));
#156491=CARTESIAN_POINT('Ctrl Pts',(61.1083461984573,6.41639155685069,60.7680468976458));
#156492=CARTESIAN_POINT('Ctrl Pts',(61.1010131485361,6.39676453280979,60.7663350639228));
#156493=CARTESIAN_POINT('Ctrl Pts',(61.0934723320082,6.37629434955248,60.7645133489496));
#156494=CARTESIAN_POINT('Ctrl Pts',(61.0861103999751,6.35601441142343,60.7626738785569));
#156495=CARTESIAN_POINT('Ctrl Pts',(61.0805006286375,6.34056115606429,60.7612722073327));
#156496=CARTESIAN_POINT('Ctrl Pts',(61.07499388939,6.32521926176865,60.7598606323473));
#156497=CARTESIAN_POINT('Ctrl Pts',(61.0697473939376,6.31045954207386,60.7584858287314));
#156498=CARTESIAN_POINT('Ctrl Pts',(61.0495490913118,6.2536366042155,60.7531930195149));
#156499=CARTESIAN_POINT('Ctrl Pts',(61.029836906676,6.19598986728747,60.7475701238141));
#156500=CARTESIAN_POINT('Ctrl Pts',(61.0105904367975,6.13756557585011,60.7416749309707));
#156501=CARTESIAN_POINT('Ctrl Pts',(60.9813866365199,6.04891496359373,60.7327298082814));
#156502=CARTESIAN_POINT('Ctrl Pts',(60.9532547519052,5.95847333458106,60.723156234998));
#156503=CARTESIAN_POINT('Ctrl Pts',(60.9261963970484,5.86620260640735,60.7130815267755));
#156504=CARTESIAN_POINT('Ctrl Pts',(60.8991842623493,5.77408949194066,60.7030240278255));
#156505=CARTESIAN_POINT('Ctrl Pts',(60.8732428931832,5.68015349713977,60.6924671186045));
#156506=CARTESIAN_POINT('Ctrl Pts',(60.8483758680909,5.58438882133169,60.6815773773706));
#156507=CARTESIAN_POINT('Ctrl Pts',(60.8407944642082,5.55519229773041,60.6782573370293));
#156508=CARTESIAN_POINT('Ctrl Pts',(60.8333128853196,5.52582602612187,60.6749066403099));
#156509=CARTESIAN_POINT('Ctrl Pts',(60.8259310896484,5.49629045537718,60.6715307480661));
#156510=CARTESIAN_POINT('Ctrl Pts',(60.8209586139193,5.4763949021522,60.6692567021572));
#156511=CARTESIAN_POINT('Ctrl Pts',(60.8160314121518,5.4564225363887,60.6669712318813));
#156512=CARTESIAN_POINT('Ctrl Pts',(60.8111499698825,5.43637268458336,60.6646756052872));
#156513=CARTESIAN_POINT('Ctrl Pts',(60.7817493882788,5.31561384495521,60.6508492086425));
#156514=CARTESIAN_POINT('Ctrl Pts',(60.7539658830283,5.1920701708242,60.6366304267703));
#156515=CARTESIAN_POINT('Ctrl Pts',(60.7277506051091,5.06573719469669,60.6222409987507));
#156516=CARTESIAN_POINT('Ctrl Pts',(60.7203510690741,5.03007839252234,60.6181794323816));
#156517=CARTESIAN_POINT('Ctrl Pts',(60.7130763615802,4.99419754902143,60.6141044942699));
#156518=CARTESIAN_POINT('Ctrl Pts',(60.705925092349,4.95809503409377,60.610021715977));
#156519=CARTESIAN_POINT('Ctrl Pts',(60.6949873250782,4.90287673739608,60.6037771631092));
#156520=CARTESIAN_POINT('Ctrl Pts',(60.6843380832632,4.84713761316821,60.5975140635554));
#156521=CARTESIAN_POINT('Ctrl Pts',(60.6739694062406,4.790881130188,60.591251886166));
#156522=CARTESIAN_POINT('Ctrl Pts',(60.6689397390439,4.76359207620045,60.588214211434));
#156523=CARTESIAN_POINT('Ctrl Pts',(60.6639760762559,4.73618130800553,60.5851767731987));
#156524=CARTESIAN_POINT('Ctrl Pts',(60.6590780591191,4.70864760020753,60.5821412859459));
#156525=CARTESIAN_POINT('Ctrl Pts',(60.649274758987,4.65353934032295,60.5760658085118));
#156526=CARTESIAN_POINT('Ctrl Pts',(60.6396348571544,4.59735327204642,60.5699343033299));
#156527=CARTESIAN_POINT('Ctrl Pts',(60.6303500662329,4.54124210717251,60.5638847935891));
#156528=CARTESIAN_POINT('Ctrl Pts',(60.6254326807053,4.51152466577588,60.5606808688158));
#156529=CARTESIAN_POINT('Ctrl Pts',(60.6206140780844,4.48182863351887,60.5574998761221));
#156530=CARTESIAN_POINT('Ctrl Pts',(60.6159174747203,4.45232775894101,60.5543615921095));
#156531=CARTESIAN_POINT('Ctrl Pts',(60.5940061631212,4.31469577147727,60.5397203900414));
#156532=CARTESIAN_POINT('Ctrl Pts',(60.5736003025058,4.17611355577954,60.5252416566678));
#156533=CARTESIAN_POINT('Ctrl Pts',(60.5545755779023,4.03658419471692,60.5111020096261));
#156534=CARTESIAN_POINT('Ctrl Pts',(60.5293617251934,3.85166310746189,60.4923624491176));
#156535=CARTESIAN_POINT('Ctrl Pts',(60.5065743736299,3.66507755205774,60.4742174111081));
#156536=CARTESIAN_POINT('Ctrl Pts',(60.4859793913249,3.4767966879087,60.456955865348));
#156537=CARTESIAN_POINT('Ctrl Pts',(60.4774468298483,3.39879137455563,60.4498043563932));
#156538=CARTESIAN_POINT('Ctrl Pts',(60.4692904665321,3.32049537884637,60.4428050363997));
#156539=CARTESIAN_POINT('Ctrl Pts',(60.4614930446832,3.24190782947751,60.4359805891655));
#156540=CARTESIAN_POINT('Ctrl Pts',(60.4416275428167,3.04169022692585,60.4185939360006));
#156541=CARTESIAN_POINT('Ctrl Pts',(60.424092686678,2.83957778210097,60.4023397510308));
#156542=CARTESIAN_POINT('Ctrl Pts',(60.4087338989989,2.63560418090611,60.3875429756916));
#156543=CARTESIAN_POINT('Ctrl Pts',(60.4043124393325,2.57688463418718,60.3832833071083));
#156544=CARTESIAN_POINT('Ctrl Pts',(60.400071235891,2.51801106594078,60.3791446537451));
#156545=CARTESIAN_POINT('Ctrl Pts',(60.39600639891,2.45898482913597,60.3751353034089));
#156546=CARTESIAN_POINT('Ctrl Pts',(60.3932155221246,2.41845799994142,60.3723825232038));
#156547=CARTESIAN_POINT('Ctrl Pts',(60.3905077826995,2.37785920718455,60.3696907021608));
#156548=CARTESIAN_POINT('Ctrl Pts',(60.3878828126484,2.33718887814358,60.3670623245156));
#156549=CARTESIAN_POINT('Ctrl Pts',(60.3739061773947,2.12063998669542,60.3530675455505));
#156550=CARTESIAN_POINT('Ctrl Pts',(60.3622162362926,1.90202463683472,60.3408126922032));
#156551=CARTESIAN_POINT('Ctrl Pts',(60.3525787012096,1.68133585233899,60.3304806711094));
#156552=CARTESIAN_POINT('Ctrl Pts',(60.3460059668921,1.53082758078909,60.3234343019883));
#156553=CARTESIAN_POINT('Ctrl Pts',(60.3403881456358,1.37935474928527,60.3172824889154));
#156554=CARTESIAN_POINT('Ctrl Pts',(60.3356972804706,1.22692157740655,60.3120816036346));
#156555=CARTESIAN_POINT('Ctrl Pts',(60.3322532820412,1.11500627265237,60.3082631522174));
#156556=CARTESIAN_POINT('Ctrl Pts',(60.3293057405566,1.00256704992089,60.3049537472116));
#156557=CARTESIAN_POINT('Ctrl Pts',(60.3268350319213,0.889614900065707,
60.3021659554015));
#156558=CARTESIAN_POINT('Ctrl Pts',(60.3251559545933,0.812853362403946,
60.3002713904349));
#156559=CARTESIAN_POINT('Ctrl Pts',(60.3236971188136,0.735854947945547,
60.2986177588588));
#156560=CARTESIAN_POINT('Ctrl Pts',(60.3224579481672,0.658613460198747,
60.2972083801014));
#156561=CARTESIAN_POINT('Ctrl Pts',(60.3209266628389,0.563163525790775,
60.2954667628195));
#156562=CARTESIAN_POINT('Ctrl Pts',(60.3197296564896,0.46734763396879,60.2940967785737));
#156563=CARTESIAN_POINT('Ctrl Pts',(60.3188631184893,0.371165784773678,
60.2931017944797));
#156564=CARTESIAN_POINT('Ctrl Pts',(60.3182849037355,0.306986528656438,
60.2924378715094));
#156565=CARTESIAN_POINT('Ctrl Pts',(60.3178591568679,0.243471706970596,
60.2919470610062));
#156566=CARTESIAN_POINT('Ctrl Pts',(60.3175725545398,0.178965076606698,
60.2916165290168));
#156567=CARTESIAN_POINT('Ctrl Pts',(60.3174296420437,0.146799240365323,
60.2914517112643));
#156568=CARTESIAN_POINT('Ctrl Pts',(60.3173218438238,0.114386787195183,
60.2913273379523));
#156569=CARTESIAN_POINT('Ctrl Pts',(60.3172506780976,0.0815223650375594,
60.2912455157613));
#156570=CARTESIAN_POINT('Ctrl Pts',(60.3172503297988,0.0813615201835923,
60.2912451153076));
#156571=CARTESIAN_POINT('Ctrl Pts',(60.3172499824342,0.0812006763251198,
60.2912447159388));
#156572=CARTESIAN_POINT('Ctrl Pts',(60.317249636004,0.0810398334620816,
60.2912443176547));
#156573=CARTESIAN_POINT('Ctrl Pts',(60.3167718356663,-0.140796408850023,
60.2906949999507));
#156574=CARTESIAN_POINT('Ctrl Pts',(60.3180703536722,-0.360742013675031,
60.2922059588602));
#156575=CARTESIAN_POINT('Ctrl Pts',(60.3211269691535,-0.579049577315057,
60.2956904127889));
#156576=CARTESIAN_POINT('Ctrl Pts',(60.3218918879312,-0.633681098928665,
60.2965623982435));
#156577=CARTESIAN_POINT('Ctrl Pts',(60.3227669758375,-0.68820986561593,
60.2975581540585));
#156578=CARTESIAN_POINT('Ctrl Pts',(60.3237521056527,-0.74263949039439,
60.2986766416983));
#156579=CARTESIAN_POINT('Ctrl Pts',(60.3284060612508,-0.999776217996843,
60.3039606070528));
#156580=CARTESIAN_POINT('Ctrl Pts',(60.3355132095719,-1.25470074694503,
60.311980556618));
#156581=CARTESIAN_POINT('Ctrl Pts',(60.3452494162381,-1.50725414925296,
60.3225677543551));
#156582=CARTESIAN_POINT('Ctrl Pts',(60.3460161107382,-1.52714190545754,
60.3234014616248));
#156583=CARTESIAN_POINT('Ctrl Pts',(60.3467991282248,-1.5470149527718,60.3242511050648));
#156584=CARTESIAN_POINT('Ctrl Pts',(60.3475985655576,-1.56687321040098,
60.3251166094454));
#156585=CARTESIAN_POINT('Ctrl Pts',(60.3564916635564,-1.78778037090632,
60.3347446502675));
#156586=CARTESIAN_POINT('Ctrl Pts',(60.3674147954383,-2.00685857303107,
60.3463353301896));
#156587=CARTESIAN_POINT('Ctrl Pts',(60.380647663187,-2.22400159825584,60.3597674794863));
#156588=CARTESIAN_POINT('Ctrl Pts',(60.3837181096662,-2.27438569110276,
60.3628841656272));
#156589=CARTESIAN_POINT('Ctrl Pts',(60.3869109222145,-2.3246719574547,60.3660978702397));
#156590=CARTESIAN_POINT('Ctrl Pts',(60.3902275060726,-2.37485945220486,
60.3694049280582));
#156591=CARTESIAN_POINT('Ctrl Pts',(60.4060853424734,-2.61482476445802,
60.3852172168766));
#156592=CARTESIAN_POINT('Ctrl Pts',(60.424773147128,-2.85252956131487,60.4031603549941));
#156593=CARTESIAN_POINT('Ctrl Pts',(60.4466410345141,-3.0879812331881,60.4228099521189));
#156594=CARTESIAN_POINT('Ctrl Pts',(60.4494095158189,-3.11778948765049,
60.4252975971906));
#156595=CARTESIAN_POINT('Ctrl Pts',(60.4522289621883,-3.14756166853934,
60.4278126490277));
#156596=CARTESIAN_POINT('Ctrl Pts',(60.4551000813933,-3.17729782317844,
60.4303542964061));
#156597=CARTESIAN_POINT('Ctrl Pts',(60.4599606519324,-3.22763870660009,
60.4346570980267));
#156598=CARTESIAN_POINT('Ctrl Pts',(60.4649693168118,-3.2778763364631,60.4390361153204));
#156599=CARTESIAN_POINT('Ctrl Pts',(60.4701313186931,-3.32801012367678,
60.4434860043842));
#156600=CARTESIAN_POINT('Ctrl Pts',(60.4887980564844,-3.50930301777317,
60.4595776126911));
#156601=CARTESIAN_POINT('Ctrl Pts',(60.5094620301379,-3.68924165233354,
60.4765856585227));
#156602=CARTESIAN_POINT('Ctrl Pts',(60.5323041457749,-3.86782602254368,
60.4942268967716));
#156603=CARTESIAN_POINT('Ctrl Pts',(60.5371864013529,-3.90599650339826,
60.4979975209647));
#156604=CARTESIAN_POINT('Ctrl Pts',(60.5421679901616,-3.94410501957805,
60.5017970980832));
#156605=CARTESIAN_POINT('Ctrl Pts',(60.5472503730506,-3.98215175049627,
60.5056229160797));
#156606=CARTESIAN_POINT('Ctrl Pts',(60.5540572056899,-4.03310771652428,
60.5107468320417));
#156607=CARTESIAN_POINT('Ctrl Pts',(60.5610448370004,-4.08395284819393,
60.5159178009482));
#156608=CARTESIAN_POINT('Ctrl Pts',(60.5682184982992,-4.13468687987222,
60.5211266905536));
#156609=CARTESIAN_POINT('Ctrl Pts',(60.5744834683542,-4.17899440653005,
60.5256757675225));
#156610=CARTESIAN_POINT('Ctrl Pts',(60.5808903363372,-4.22321729183196,
60.5302537784216));
#156611=CARTESIAN_POINT('Ctrl Pts',(60.5874421641437,-4.26735553575933,
60.5348546200745));
#156612=CARTESIAN_POINT('Ctrl Pts',(60.5926973823719,-4.30275880197777,
60.5385449531591));
#156613=CARTESIAN_POINT('Ctrl Pts',(60.5979225873047,-4.33730075434144,
60.5421653199955));
#156614=CARTESIAN_POINT('Ctrl Pts',(60.6034153254535,-4.37292320597405,
60.5459162536311));
#156615=CARTESIAN_POINT('Ctrl Pts',(60.604770537851,-4.38171226286584,60.5468417140531));
#156616=CARTESIAN_POINT('Ctrl Pts',(60.6061422543349,-4.39056699089614,
60.5477751634014));
#156617=CARTESIAN_POINT('Ctrl Pts',(60.6075353869347,-4.39951634329599,
60.5487196897732));
#156618=CARTESIAN_POINT('Ctrl Pts',(60.6256697600186,-4.51600984527997,
60.5610145665249));
#156619=CARTESIAN_POINT('Ctrl Pts',(60.644794645044,-4.63022759689235,60.57339439645));
#156620=CARTESIAN_POINT('Ctrl Pts',(60.6649277275938,-4.74223674371549,
60.5857482471537));
#156621=CARTESIAN_POINT('Ctrl Pts',(60.6883341692675,-4.87245701950087,
60.6001106621106));
#156622=CARTESIAN_POINT('Ctrl Pts',(60.713104510655,-4.99968962535541,60.6144367085336));
#156623=CARTESIAN_POINT('Ctrl Pts',(60.7393115847284,-5.12389259812989,
60.6285186139536));
#156624=CARTESIAN_POINT('Ctrl Pts',(60.7605670573277,-5.22462848635463,
60.6399398643367));
#156625=CARTESIAN_POINT('Ctrl Pts',(60.7827670219855,-5.32337236172495,
60.6512013180985));
#156626=CARTESIAN_POINT('Ctrl Pts',(60.8059386129769,-5.42011754924029,
60.6622075350583));
#156627=CARTESIAN_POINT('Ctrl Pts',(60.8089240145654,-5.43258208983175,
60.6636255636092));
#156628=CARTESIAN_POINT('Ctrl Pts',(60.8119255029196,-5.44501355984374,
60.6650393579304));
#156629=CARTESIAN_POINT('Ctrl Pts',(60.8149430121899,-5.45741210818994,
60.6664486765836));
#156630=CARTESIAN_POINT('Ctrl Pts',(60.8393451527445,-5.55767729126446,
60.6778456231317));
#156631=CARTESIAN_POINT('Ctrl Pts',(60.8647961665854,-5.6557865365155,60.6889466944976));
#156632=CARTESIAN_POINT('Ctrl Pts',(60.8913187722302,-5.75173231434,60.6995837830937));
#156633=CARTESIAN_POINT('Ctrl Pts',(60.9034359144587,-5.7955661914367,60.7044434532612));
#156634=CARTESIAN_POINT('Ctrl Pts',(60.9157765342813,-5.83894899354787,
60.7092068094858));
#156635=CARTESIAN_POINT('Ctrl Pts',(60.9283421344644,-5.88188235016986,
60.713860427064));
#156636=CARTESIAN_POINT('Ctrl Pts',(60.9500775929391,-5.95614670495086,
60.7219100633849));
#156637=CARTESIAN_POINT('Ctrl Pts',(60.9724838128451,-6.02906282046898,
60.7296294861063));
#156638=CARTESIAN_POINT('Ctrl Pts',(60.9955541308482,-6.1006307460953,60.7369568347596));
#156639=CARTESIAN_POINT('Ctrl Pts',(60.9978757070085,-6.1078326576577,60.7376941890496));
#156640=CARTESIAN_POINT('Ctrl Pts',(61.000204018296,-6.11502084322828,60.7384275901662));
#156641=CARTESIAN_POINT('Ctrl Pts',(61.0025390361617,-6.12219540860419,
60.7391569766818));
#156642=CARTESIAN_POINT('Ctrl Pts',(61.0118059647722,-6.15066893170974,
60.7420516752059));
#156643=CARTESIAN_POINT('Ctrl Pts',(61.0211785101258,-6.17892787314475,
60.7448830833879));
#156644=CARTESIAN_POINT('Ctrl Pts',(61.0306570702488,-6.20697150151012,
60.7476440444355));
#156645=CARTESIAN_POINT('Ctrl Pts',(61.0381576299283,-6.22916294255784,
60.749828843903));
#156646=CARTESIAN_POINT('Ctrl Pts',(61.0455411532524,-6.25068477398866,
60.7519180674648));
#156647=CARTESIAN_POINT('Ctrl Pts',(61.0531533692364,-6.27255314702256,
60.7540067349002));
#156648=CARTESIAN_POINT('Ctrl Pts',(61.0575847121439,-6.28528350831903,
60.755222622842));
#156649=CARTESIAN_POINT('Ctrl Pts',(61.062094186921,-6.29813075474211,60.7564380996644));
#156650=CARTESIAN_POINT('Ctrl Pts',(61.0667557827805,-6.31128995373525,
60.7576696460975));
#156651=CARTESIAN_POINT('Ctrl Pts',(61.0928128619575,-6.38484637098175,
60.7645536626201));
#156652=CARTESIAN_POINT('Ctrl Pts',(61.1190916473322,-6.45534327866974,
60.7707317505738));
#156653=CARTESIAN_POINT('Ctrl Pts',(61.1455952625239,-6.52281934308269,
60.7762000466415));
#156654=CARTESIAN_POINT('Ctrl Pts',(61.167445218974,-6.57844756806917,60.7807081875147));
#156655=CARTESIAN_POINT('Ctrl Pts',(61.189447687566,-6.63202403649182,60.7847346252518));
#156656=CARTESIAN_POINT('Ctrl Pts',(61.2115992402602,-6.6835937174199,60.788288103955));
#156657=CARTESIAN_POINT('Ctrl Pts',(61.2348668728669,-6.73776167602956,
60.7920206205006));
#156658=CARTESIAN_POINT('Ctrl Pts',(61.2582990475287,-6.78971265842065,
60.7952301642865));
#156659=CARTESIAN_POINT('Ctrl Pts',(61.2818913036666,-6.83939922853566,
60.7978832027763));
#156660=CARTESIAN_POINT('Ctrl Pts',(61.3078113879601,-6.89398833091362,
60.8007980143521));
#156661=CARTESIAN_POINT('Ctrl Pts',(61.3339248025162,-6.94584436954833,
60.8030412191049));
#156662=CARTESIAN_POINT('Ctrl Pts',(61.3602187632956,-6.99496701511857,
60.8045939876081));
#156663=CARTESIAN_POINT('Ctrl Pts',(61.3862767718842,-7.04364885240078,
60.8061328221462));
#156664=CARTESIAN_POINT('Ctrl Pts',(61.4125121580285,-7.08964728722199,
60.8069939889131));
#156665=CARTESIAN_POINT('Ctrl Pts',(61.4389049804967,-7.13300804515157,
60.8071780886852));
#156666=CARTESIAN_POINT('Ctrl Pts',(61.4630245950937,-7.17263415073987,
60.8073463319853));
#156667=CARTESIAN_POINT('Ctrl Pts',(61.4872746627032,-7.21005544093054,
60.8069483336587));
#156668=CARTESIAN_POINT('Ctrl Pts',(61.5115944597208,-7.2452196605957,60.805949935138));
#156669=CARTESIAN_POINT('Ctrl Pts',(61.537167996932,-7.28219667481437,60.8049000669298));
#156670=CARTESIAN_POINT('Ctrl Pts',(61.5628187966211,-7.31667846300659,
60.8031863964706));
#156671=CARTESIAN_POINT('Ctrl Pts',(61.5884809504075,-7.34865871299229,
60.8007929533979));
#156672=CARTESIAN_POINT('Ctrl Pts',(61.6161756530536,-7.38317193122326,
60.7982099397214));
#156673=CARTESIAN_POINT('Ctrl Pts',(61.6438837458237,-7.41477211492232,
60.7948351645046));
#156674=CARTESIAN_POINT('Ctrl Pts',(61.6715250991893,-7.44350522364788,
60.7906751871624));
#156675=CARTESIAN_POINT('Ctrl Pts',(61.6771954599592,-7.4493995476471,60.7898218073726));
#156676=CARTESIAN_POINT('Ctrl Pts',(61.6828630158119,-7.45517337202722,
60.7889354688476));
#156677=CARTESIAN_POINT('Ctrl Pts',(61.6885270782846,-7.46082731767655,
60.7880163558176));
#156678=CARTESIAN_POINT('Ctrl Pts',(61.6955489848948,-7.46783668216003,
60.786876904074));
#156679=CARTESIAN_POINT('Ctrl Pts',(61.702565503283,-7.47466179683456,60.7856870811896));
#156680=CARTESIAN_POINT('Ctrl Pts',(61.7095727627346,-7.48130385739646,
60.7844478028312));
#156681=CARTESIAN_POINT('Origin',(61.4493580047591,-11.67384127833,59.30720639017));
#156682=CARTESIAN_POINT('Origin',(1.07038457110909,25.,122.41156512159));
#156683=CARTESIAN_POINT('Origin',(-10.9843331791359,-92.5,80.581991049076));
#156684=CARTESIAN_POINT('Ctrl Pts',(29.5338632414891,-0.462029067073086,
63.010868215388));
#156685=CARTESIAN_POINT('Ctrl Pts',(29.5346219246491,-0.433752793220286,
63.011230106753));
#156686=CARTESIAN_POINT('Ctrl Pts',(29.5608039722791,0.641998223276014,
63.023714156154));
#156687=CARTESIAN_POINT('Ctrl Pts',(29.4078372281691,2.83176758612401,62.95026782851));
#156688=CARTESIAN_POINT('Ctrl Pts',(28.5737667388991,6.01426195252202,62.55847749973));
#156689=CARTESIAN_POINT('Ctrl Pts',(27.1713456340891,8.95881369369201,61.93185808602));
#156690=CARTESIAN_POINT('Ctrl Pts',(25.3938118350091,11.44424088043,61.19592371053));
#156691=CARTESIAN_POINT('Ctrl Pts',(23.4862351945491,13.39803722808,60.47438298443));
#156692=CARTESIAN_POINT('Ctrl Pts',(21.5959186421791,14.88576337841,59.82526804813));
#156693=CARTESIAN_POINT('Ctrl Pts',(19.7728932383691,16.01167021338,59.25919610008));
#156694=CARTESIAN_POINT('Ctrl Pts',(17.9890179586191,16.88023517151,58.75958030935));
#156695=CARTESIAN_POINT('Ctrl Pts',(16.1694318501091,17.56205741783,58.30367386163));
#156696=CARTESIAN_POINT('Ctrl Pts',(14.2545233152291,18.07545203247,57.8825033362001));
#156697=CARTESIAN_POINT('Ctrl Pts',(12.2750306503891,18.39974030706,57.50985034058));
#156698=CARTESIAN_POINT('Ctrl Pts',(10.2979506383991,18.52298246441,57.20011317475));
#156699=CARTESIAN_POINT('Ctrl Pts',(8.29553577903909,18.45025449476,56.94745644735));
#156700=CARTESIAN_POINT('Ctrl Pts',(6.18046749893909,18.15452185092,56.74590079812));
#156701=CARTESIAN_POINT('Ctrl Pts',(3.8630583959391,17.55006605826,56.60308243839));
#156702=CARTESIAN_POINT('Ctrl Pts',(1.35289501732909,16.52026706539,56.54071687939));
#156703=CARTESIAN_POINT('Ctrl Pts',(-1.22835397511091,14.96025853102,56.57780430316));
#156704=CARTESIAN_POINT('Ctrl Pts',(-2.82698452737391,13.56768331313,56.66360640014));
#156705=CARTESIAN_POINT('Ctrl Pts',(-3.58348738863291,12.77819820572,56.71617340988));
#156706=CARTESIAN_POINT('Ctrl Pts',(30.0860529662091,-0.465286448929386,
62.05420413572));
#156707=CARTESIAN_POINT('Ctrl Pts',(30.0868281149291,-0.436810905979286,
62.05457485453));
#156708=CARTESIAN_POINT('Ctrl Pts',(30.1135782153191,0.646521910559514,
62.06736342767));
#156709=CARTESIAN_POINT('Ctrl Pts',(29.9572832439191,2.85177150159601,61.99211983581));
#156710=CARTESIAN_POINT('Ctrl Pts',(29.1052651413891,6.05572682568202,61.59085102028));
#156711=CARTESIAN_POINT('Ctrl Pts',(27.6732347629591,9.01845477515302,60.9493802108601));
#156712=CARTESIAN_POINT('Ctrl Pts',(25.8588487868591,11.51786388819,60.196375469));
#156713=CARTESIAN_POINT('Ctrl Pts',(23.9121691835891,13.48193550668,59.45836886149));
#156714=CARTESIAN_POINT('Ctrl Pts',(21.9833029704391,14.97718508481,58.7946079262));
#156715=CARTESIAN_POINT('Ctrl Pts',(20.1231372976191,16.10868985698,58.2158677272001));
#156716=CARTESIAN_POINT('Ctrl Pts',(18.3028628908391,16.98156509667,57.70514405855));
#156717=CARTESIAN_POINT('Ctrl Pts',(16.4460310900391,17.66679861647,57.23916702843));
#156718=CARTESIAN_POINT('Ctrl Pts',(14.4917463634591,18.18280526933,56.80876811987));
#156719=CARTESIAN_POINT('Ctrl Pts',(12.4713202820591,18.50878353077,56.42804576509));
#156720=CARTESIAN_POINT('Ctrl Pts',(10.4531101100391,18.6326885709,56.11172577456));
#156721=CARTESIAN_POINT('Ctrl Pts',(8.40879716453909,18.55957000061,55.85386194703));
#156722=CARTESIAN_POINT('Ctrl Pts',(6.24923249066909,18.26219087574,55.6483878136801));
#156723=CARTESIAN_POINT('Ctrl Pts',(3.88282255928909,17.6542832528,55.50319038629));
#156724=CARTESIAN_POINT('Ctrl Pts',(1.31936572697909,16.61847639235,55.44054243506));
#156725=CARTESIAN_POINT('Ctrl Pts',(-1.31681310253091,15.04922855625,55.47988027154));
#156726=CARTESIAN_POINT('Ctrl Pts',(-2.94946644714391,13.64834848308,55.5686612246301));
#156727=CARTESIAN_POINT('Ctrl Pts',(-3.72205763400691,12.85415388889,55.6229400250801));
#156728=CARTESIAN_POINT('Ctrl Pts',(29.6438402590691,-0.440906405366586,
61.0422837596));
#156729=CARTESIAN_POINT('Ctrl Pts',(29.6445863481391,-0.413922302316986,
61.04263099393));
#156730=CARTESIAN_POINT('Ctrl Pts',(29.6703352983091,0.612664138304914,
61.0546093697601));
#156731=CARTESIAN_POINT('Ctrl Pts',(29.5199825989191,2.70205115803401,60.98418855492));
#156732=CARTESIAN_POINT('Ctrl Pts',(28.6983885856991,5.74538083047302,60.60757066705));
#156733=CARTESIAN_POINT('Ctrl Pts',(27.3118968411491,8.57206800556001,60.00247848032));
#156734=CARTESIAN_POINT('Ctrl Pts',(25.5485386075391,10.96682866558,59.28852217894));
#156735=CARTESIAN_POINT('Ctrl Pts',(23.6522177073491,12.85399448613,58.58612492656));
#156736=CARTESIAN_POINT('Ctrl Pts',(21.7712823376891,14.29293457848,57.95274708762));
#156737=CARTESIAN_POINT('Ctrl Pts',(19.9569744205691,15.3825412991,57.399474373));
#156738=CARTESIAN_POINT('Ctrl Pts',(18.1821311163691,16.22315601275,56.9105053048901));
#156739=CARTESIAN_POINT('Ctrl Pts',(16.3728054944391,16.88285767912,56.46373198555));
#156740=CARTESIAN_POINT('Ctrl Pts',(14.4702883739891,17.37931439633,56.0503330424501));
#156741=CARTESIAN_POINT('Ctrl Pts',(12.5056416128591,17.69264386349,55.6837038022));
#156742=CARTESIAN_POINT('Ctrl Pts',(10.5455810396291,17.81158752306,55.37787002278));
#156743=CARTESIAN_POINT('Ctrl Pts',(8.56254414565909,17.74139242357,55.12695247192));
#156744=CARTESIAN_POINT('Ctrl Pts',(6.4700871073191,17.45633647142,54.9246919594001));
#156745=CARTESIAN_POINT('Ctrl Pts',(4.17965284087909,16.87426425135,54.77784196221));
#156746=CARTESIAN_POINT('Ctrl Pts',(1.70063539712909,15.88342358762,54.70699356138));
#156747=CARTESIAN_POINT('Ctrl Pts',(-0.847455673380912,14.38332778486,54.73062029495));
#156748=CARTESIAN_POINT('Ctrl Pts',(-2.42552047959091,13.04460583201,54.80507482908));
#156749=CARTESIAN_POINT('Ctrl Pts',(-3.17239712901691,12.28565963609,54.85169577897));
#156750=CARTESIAN_POINT('Ctrl Pts',(28.5669936237991,-0.408723671234686,
60.79836945316));
#156751=CARTESIAN_POINT('Ctrl Pts',(28.5676887698891,-0.383708334716086,
60.79867999721));
#156752=CARTESIAN_POINT('Ctrl Pts',(28.5916818669991,0.567970383760914,
60.80939260235));
#156753=CARTESIAN_POINT('Ctrl Pts',(28.4517075181491,2.50441369284601,60.74649096621));
#156754=CARTESIAN_POINT('Ctrl Pts',(27.6841573416491,5.33571041184002,60.40859830391));
#156755=CARTESIAN_POINT('Ctrl Pts',(26.3813035283791,7.98281775714401,59.8615184069));
#156756=CARTESIAN_POINT('Ctrl Pts',(24.7153386034591,10.23943783787,59.21096093285));
#156757=CARTESIAN_POINT('Ctrl Pts',(22.9178680255491,12.02508460897,58.5672777695));
#156758=CARTESIAN_POINT('Ctrl Pts',(21.1323491770191,13.38969369344,57.98459351753));
#156759=CARTESIAN_POINT('Ctrl Pts',(19.4095888040891,14.4239931358,57.47420458465));
#156760=CARTESIAN_POINT('Ctrl Pts',(17.7250457055691,15.22202253043,57.02215382759));
#156761=CARTESIAN_POINT('Ctrl Pts',(16.0093287990591,15.84802102278,56.60823505731));
#156762=CARTESIAN_POINT('Ctrl Pts',(14.2076068025491,16.3186709616,56.22423386201));
#156763=CARTESIAN_POINT('Ctrl Pts',(12.3500720308091,16.61530346173,55.88239455409));
#156764=CARTESIAN_POINT('Ctrl Pts',(10.5001323733591,16.72769787988,55.59558481383));
#156765=CARTESIAN_POINT('Ctrl Pts',(8.63169365612909,16.66136189094,55.35811567321));
#156766=CARTESIAN_POINT('Ctrl Pts',(6.66335190121909,16.39257307097,55.16358639907));
#156767=CARTESIAN_POINT('Ctrl Pts',(4.51205869883909,15.8446047236,55.01715480186));
#156768=CARTESIAN_POINT('Ctrl Pts',(2.18651660771909,14.91312142525,54.93685948768));
#156769=CARTESIAN_POINT('Ctrl Pts',(-0.202134170110909,13.50430936028,54.93959559631));
#156770=CARTESIAN_POINT('Ctrl Pts',(-1.68141039720091,12.24763887117,54.99407390047));
#156771=CARTESIAN_POINT('Ctrl Pts',(-2.38169007766091,11.53522211755,55.02989751292));
#156772=CARTESIAN_POINT('Ctrl Pts',(28.8585550967491,1.26413730024185E-6,
60.89678211462));
#156773=CARTESIAN_POINT('Ctrl Pts',(28.858491969845,0.228821303340967,60.8967613163214));
#156774=CARTESIAN_POINT('Ctrl Pts',(28.8510774183777,0.568453705395284,
60.8934108792682));
#156775=CARTESIAN_POINT('Ctrl Pts',(28.8326729224955,0.90268677766527,60.8851040611296));
#156776=CARTESIAN_POINT('Ctrl Pts',(28.8179599071217,1.12430897478207,60.8784672952805));
#156777=CARTESIAN_POINT('Ctrl Pts',(28.8095647672157,1.23247330649146,60.8746818567286));
#156778=CARTESIAN_POINT('Ctrl Pts',(28.7796142842825,1.56744757292938,60.8611868260539));
#156779=CARTESIAN_POINT('Ctrl Pts',(28.7541873146485,1.79256287037361,60.8497408086264));
#156780=CARTESIAN_POINT('Ctrl Pts',(28.6923951978587,2.24639170489994,60.8219907114747));
#156781=CARTESIAN_POINT('Ctrl Pts',(28.6563900151882,2.47312237571838,60.8058475219207));
#156782=CARTESIAN_POINT('Ctrl Pts',(28.5297685422649,3.17060894521255,60.7492526345571));
#156783=CARTESIAN_POINT('Ctrl Pts',(28.4234973497442,3.63253854932098,60.7019477744694));
#156784=CARTESIAN_POINT('Ctrl Pts',(28.1669437708712,4.55027487309582,60.5888659622799));
#156785=CARTESIAN_POINT('Ctrl Pts',(28.0159853327217,5.0078552723136,60.5227968948521));
#156786=CARTESIAN_POINT('Ctrl Pts',(27.7582589840107,5.6843126691546,60.4114351412588));
#156787=CARTESIAN_POINT('Ctrl Pts',(27.6670035462099,5.90831132426182,60.3722155270459));
#156788=CARTESIAN_POINT('Ctrl Pts',(27.4737411368527,6.35333434679668,60.2897187140422));
#156789=CARTESIAN_POINT('Ctrl Pts',(27.3722215625238,6.57354671851138,60.2466453528615));
#156790=CARTESIAN_POINT('Ctrl Pts',(27.2093554140172,6.90572110665497,60.1780719445438));
#156791=CARTESIAN_POINT('Ctrl Pts',(27.1533394348912,7.01669623622962,60.1545704718447));
#156792=CARTESIAN_POINT('Ctrl Pts',(27.0378418193842,7.23914716243249,60.1063078690635));
#156793=CARTESIAN_POINT('Ctrl Pts',(26.97788687327,7.35140606811306,60.0813513934283));
#156794=CARTESIAN_POINT('Ctrl Pts',(26.8578818260713,7.57081252828534,60.0316067674831));
#156795=CARTESIAN_POINT('Ctrl Pts',(26.7675113001991,7.73203134537305,59.9942985092506));
#156796=CARTESIAN_POINT('Ctrl Pts',(26.6765895476588,7.8882461203985,59.9569948841178));
#156797=CARTESIAN_POINT('Ctrl Pts',(26.615852428485,7.99127729440162,59.9321273136503));
#156798=CARTESIAN_POINT('Ctrl Pts',(26.5844046075602,8.04391960438276,59.9192792403542));
#156799=CARTESIAN_POINT('Ctrl Pts',(26.083358749802,8.87217405440387,59.7149904794122));
#156800=CARTESIAN_POINT('Ctrl Pts',(25.5447392608045,9.6186234322292,59.5014887823171));
#156801=CARTESIAN_POINT('Ctrl Pts',(24.9372755532191,10.33198097767,59.2718675406));
#156802=CARTESIAN_POINT('Ctrl Pts',(26.0609344740391,10.60241468947,60.52351356035));
#156803=CARTESIAN_POINT('Ctrl Pts',(25.9123339633033,10.8117020094606,60.5051762448939));
#156804=CARTESIAN_POINT('Ctrl Pts',(25.7589271266988,11.0173666357863,60.4890488905304));
#156805=CARTESIAN_POINT('Ctrl Pts',(25.6004937437591,11.2187557868,60.4750588099));
#156806=CARTESIAN_POINT('Origin',(24.4068932609991,-15.54362135317,60.67496850203));
#156807=CARTESIAN_POINT('',(24.9372684584991,7.5,59.2718640334));
#156808=CARTESIAN_POINT('',(24.9372684584991,7.5,59.2718640334));
#156809=CARTESIAN_POINT('Origin',(24.4068932609991,7.5,60.67496850203));
#156810=CARTESIAN_POINT('Origin',(24.4068932609991,7.5,60.67496850203));
#156811=CARTESIAN_POINT('Ctrl Pts',(24.9372684584991,7.5,59.2718640334));
#156812=CARTESIAN_POINT('Ctrl Pts',(24.7518004578403,7.41080923984522,59.2015326743088));
#156813=CARTESIAN_POINT('Ctrl Pts',(24.3332614377359,7.2243083185516,59.1195420885914));
#156814=CARTESIAN_POINT('Ctrl Pts',(23.7332150533881,6.91634501879556,59.184666298664));
#156815=CARTESIAN_POINT('Ctrl Pts',(23.2249783321078,6.57856080590289,59.3068783133604));
#156816=CARTESIAN_POINT('Ctrl Pts',(22.7661090603145,6.27051635511719,59.351451038476));
#156817=CARTESIAN_POINT('Ctrl Pts',(22.3007795484368,6.06002636053959,59.3141844993433));
#156818=CARTESIAN_POINT('Ctrl Pts',(21.9688150426247,6.00240938788309,59.2562553487836));
#156819=CARTESIAN_POINT('Ctrl Pts',(21.7988764270574,6.00000816827778,59.2227260005147));
#156820=CARTESIAN_POINT('Ctrl Pts',(21.7835206159544,6.00000000027008,59.2196611273475));
#156821=CARTESIAN_POINT('Ctrl Pts',(24.7500115337591,7.66199406857501,59.23234060116));
#156822=CARTESIAN_POINT('Ctrl Pts',(24.7219457315591,7.64878463429501,59.22687875267));
#156823=CARTESIAN_POINT('Ctrl Pts',(24.4990723215691,7.54413806281901,59.1895696092));
#156824=CARTESIAN_POINT('Ctrl Pts',(24.0530888920991,7.33541164648101,59.20365583005));
#156825=CARTESIAN_POINT('Ctrl Pts',(23.5121159558291,7.00326946263901,59.38501229628));
#156826=CARTESIAN_POINT('Ctrl Pts',(23.0769075317691,6.62914306930301,59.5703782362));
#156827=CARTESIAN_POINT('Ctrl Pts',(22.6625868082291,6.28134157023501,59.63701551399));
#156828=CARTESIAN_POINT('Ctrl Pts',(22.2127059182691,6.03754403224301,59.6034463707));
#156829=CARTESIAN_POINT('Ctrl Pts',(21.8319987041491,5.95311734543901,59.53436346757));
#156830=CARTESIAN_POINT('Ctrl Pts',(21.6116966555391,5.95211941027301,59.48764408243));
#156831=CARTESIAN_POINT('Ctrl Pts',(21.5492362715591,5.95568098179701,59.47401549141));
#156832=CARTESIAN_POINT('Ctrl Pts',(25.5892994869691,7.29739447716501,59.3149313448099));
#156833=CARTESIAN_POINT('Ctrl Pts',(25.5641282947991,7.28614135847301,59.2905997259801));
#156834=CARTESIAN_POINT('Ctrl Pts',(25.3587897698691,7.19811075061901,59.10313570938));
#156835=CARTESIAN_POINT('Ctrl Pts',(24.8658955918391,7.03575877646301,58.8143312375401));
#156836=CARTESIAN_POINT('Ctrl Pts',(24.1022737005091,6.80336022964301,58.67731108114));
#156837=CARTESIAN_POINT('Ctrl Pts',(23.4335704902791,6.56741369981001,58.71396001818));
#156838=CARTESIAN_POINT('Ctrl Pts',(22.8987579890791,6.36500644573902,58.74904311935));
#156839=CARTESIAN_POINT('Ctrl Pts',(22.4310250796891,6.23855144037001,58.73175649594));
#156840=CARTESIAN_POINT('Ctrl Pts',(22.0849984951291,6.21512134718301,58.6896704444001));
#156841=CARTESIAN_POINT('Ctrl Pts',(21.8954300117391,6.23523701677601,58.66055462542));
#156842=CARTESIAN_POINT('Ctrl Pts',(21.8424055925791,6.24366294458601,58.65200766024));
#156843=CARTESIAN_POINT('Ctrl Pts',(25.8652585171391,7.04901149428901,60.1553704558201));
#156844=CARTESIAN_POINT('Ctrl Pts',(25.8569176456691,7.03183869736401,60.12394526535));
#156845=CARTESIAN_POINT('Ctrl Pts',(25.7831098699891,6.89796515568501,59.8752379208801));
#156846=CARTESIAN_POINT('Ctrl Pts',(25.5178042067991,6.65664549376101,59.3916362179599));
#156847=CARTESIAN_POINT('Ctrl Pts',(24.8894971195291,6.32304071634601,58.8840204490601));
#156848=CARTESIAN_POINT('Ctrl Pts',(24.1659594138691,5.99743477030701,58.59018788242));
#156849=CARTESIAN_POINT('Ctrl Pts',(23.4809523308491,5.72763799024202,58.40125644434));
#156850=CARTESIAN_POINT('Ctrl Pts',(22.8338129039291,5.56848202078701,58.23167670162));
#156851=CARTESIAN_POINT('Ctrl Pts',(22.3405182440191,5.55291529651302,58.09949298367));
#156852=CARTESIAN_POINT('Ctrl Pts',(22.0685405930591,5.59234130224901,58.02647356417));
#156853=CARTESIAN_POINT('Ctrl Pts',(21.9923847081791,5.60744440708801,58.0059930655201));
#156854=CARTESIAN_POINT('Ctrl Pts',(25.2820011365291,7.18316514851801,60.8525262807));
#156855=CARTESIAN_POINT('Ctrl Pts',(25.2863805694791,7.15854384897201,60.83338955318));
#156856=CARTESIAN_POINT('Ctrl Pts',(25.3170701286091,6.96552196997101,60.6780164578));
#156857=CARTESIAN_POINT('Ctrl Pts',(25.3098283613891,6.60456285147501,60.31657555231));
#156858=CARTESIAN_POINT('Ctrl Pts',(25.0297132372791,6.07731684233201,59.78350345802));
#156859=CARTESIAN_POINT('Ctrl Pts',(24.4887957105791,5.53034639608301,59.33177220365));
#156860=CARTESIAN_POINT('Ctrl Pts',(23.7849321666091,5.05263239825701,58.96655767474));
#156861=CARTESIAN_POINT('Ctrl Pts',(22.9891941327791,4.74579444124201,58.6394001825));
#156862=CARTESIAN_POINT('Ctrl Pts',(22.3245857727091,4.67652663690701,58.3966283744));
#156863=CARTESIAN_POINT('Ctrl Pts',(21.9454165897491,4.71275487277101,58.26527229885));
#156864=CARTESIAN_POINT('Ctrl Pts',(21.8383637195091,4.72918860417001,58.22863842432));
#156865=CARTESIAN_POINT('',(22.0949867135254,5.00000000061885,58.2694348746444));
#156866=CARTESIAN_POINT('Origin',(21.7835175497024,5.00000436630195,59.219661344816));
#156867=CARTESIAN_POINT('Ctrl Pts',(24.9372684584988,7.5,59.2718640334007));
#156868=CARTESIAN_POINT('Ctrl Pts',(24.9253516994804,7.47196095686942,59.2673169679264));
#156869=CARTESIAN_POINT('Ctrl Pts',(24.9136646345482,7.4445580630566,59.2629539372089));
#156870=CARTESIAN_POINT('Ctrl Pts',(24.9021900367248,7.41778866776119,59.2586895691701));
#156871=CARTESIAN_POINT('Ctrl Pts',(24.8898555346574,7.38901317892088,59.2541056301773));
#156872=CARTESIAN_POINT('Ctrl Pts',(24.8777670910077,7.36096968773272,59.2496361489087));
#156873=CARTESIAN_POINT('Ctrl Pts',(24.8659212636497,7.33365634041001,59.2452332101466));
#156874=CARTESIAN_POINT('Ctrl Pts',(24.8521988171317,7.30201600524901,59.2401327566402));
#156875=CARTESIAN_POINT('Ctrl Pts',(24.8388023753174,7.27135540555908,59.2351219906611));
#156876=CARTESIAN_POINT('Ctrl Pts',(24.8257412534641,7.24167417214954,59.2301959155924));
#156877=CARTESIAN_POINT('Ctrl Pts',(24.8101088325862,7.20614969438692,59.2243000607328));
#156878=CARTESIAN_POINT('Ctrl Pts',(24.7949568863169,7.17202795111224,59.2185271755939));
#156879=CARTESIAN_POINT('Ctrl Pts',(24.7803146189784,7.13931403220985,59.2129454519303));
#156880=CARTESIAN_POINT('Ctrl Pts',(24.7723697943765,7.1215636154395,59.2099168352237));
#156881=CARTESIAN_POINT('Ctrl Pts',(24.7645752037018,7.10422779013506,59.2069455313005));
#156882=CARTESIAN_POINT('Ctrl Pts',(24.7569370338574,7.08730817988477,59.2040463791642));
#156883=CARTESIAN_POINT('Ctrl Pts',(24.7518865753216,7.07612071066732,59.2021294215747));
#156884=CARTESIAN_POINT('Ctrl Pts',(24.7468975324174,7.06511492467662,59.2002414188583));
#156885=CARTESIAN_POINT('Ctrl Pts',(24.7419698932784,7.05428965355225,59.198385949465));
#156886=CARTESIAN_POINT('Ctrl Pts',(24.7300658314657,7.0281382465658,59.1939035550105));
#156887=CARTESIAN_POINT('Ctrl Pts',(24.7185160453369,7.00304107430083,59.1896079543967));
#156888=CARTESIAN_POINT('Ctrl Pts',(24.7073185715577,6.97900228018697,59.1854630913426));
#156889=CARTESIAN_POINT('Ctrl Pts',(24.6987957386628,6.96070541883539,59.1823082748297));
#156890=CARTESIAN_POINT('Ctrl Pts',(24.690478341979,6.94302153654002,59.1792416995708));
#156891=CARTESIAN_POINT('Ctrl Pts',(24.6823809140436,6.92594895950459,59.1762593434168));
#156892=CARTESIAN_POINT('Ctrl Pts',(24.6708110196032,6.90155505125387,59.1719980463532));
#156893=CARTESIAN_POINT('Ctrl Pts',(24.6596761393446,6.87841074954737,59.1679030280241));
#156894=CARTESIAN_POINT('Ctrl Pts',(24.6489806389292,6.85651598717019,59.1639625160071));
#156895=CARTESIAN_POINT('Ctrl Pts',(24.6436328887215,6.84556860598159,59.1619922599987));
#156896=CARTESIAN_POINT('Ctrl Pts',(24.6383949110302,6.83493361143069,59.1600608277157));
#156897=CARTESIAN_POINT('Ctrl Pts',(24.6332669050915,6.82461100435038,59.1581676907911));
#156898=CARTESIAN_POINT('Ctrl Pts',(24.6287798998952,6.8155787231551,59.1565111959821));
#156899=CARTESIAN_POINT('Ctrl Pts',(24.6243770872641,6.80678561377664,59.1548840335607));
#156900=CARTESIAN_POINT('Ctrl Pts',(24.6200585030648,6.79823167905871,59.1532861139637));
#156901=CARTESIAN_POINT('Ctrl Pts',(24.6197500327649,6.79762068372172,59.1531719768496));
#156902=CARTESIAN_POINT('Ctrl Pts',(24.6196138894654,6.79735055225575,59.1531215980768));
#156903=CARTESIAN_POINT('Ctrl Pts',(24.6193922250548,6.79691181929018,59.153039569991));
#156904=CARTESIAN_POINT('Ctrl Pts',(24.6191705606442,6.79647308632462,59.1529575419053));
#156905=CARTESIAN_POINT('Ctrl Pts',(24.6188633732126,6.79586575187103,59.1528438697275));
#156906=CARTESIAN_POINT('Ctrl Pts',(24.6182128377217,6.79458035040017,59.1526030827148));
#156907=CARTESIAN_POINT('Ctrl Pts',(24.6006559350706,6.75988943990018,59.1461046299768));
#156908=CARTESIAN_POINT('Ctrl Pts',(24.5829534249965,6.72574806844182,59.1395180821526));
#156909=CARTESIAN_POINT('Ctrl Pts',(24.5650822275888,6.69215856035955,59.1328349464223));
#156910=CARTESIAN_POINT('Ctrl Pts',(24.544839586702,6.65411184562833,59.12526498267));
#156911=CARTESIAN_POINT('Ctrl Pts',(24.5243812689657,6.61677342010873,59.1175714587251));
#156912=CARTESIAN_POINT('Ctrl Pts',(24.5037116120574,6.58014158135225,59.1097967626435));
#156913=CARTESIAN_POINT('Ctrl Pts',(24.4993558779037,6.57242212321638,59.1081583944109));
#156914=CARTESIAN_POINT('Ctrl Pts',(24.4949908548014,6.56473401866839,59.1065165794007));
#156915=CARTESIAN_POINT('Ctrl Pts',(24.4906167188193,6.55707721049565,59.1048719438424));
#156916=CARTESIAN_POINT('Ctrl Pts',(24.488294111182,6.55301154787976,59.1039986643825));
#156917=CARTESIAN_POINT('Ctrl Pts',(24.4859668177808,6.54895257284586,59.1031237990105));
#156918=CARTESIAN_POINT('Ctrl Pts',(24.4836354773033,6.54490078716199,59.1022476768571));
#156919=CARTESIAN_POINT('Ctrl Pts',(24.4642483963475,6.5112067395404,59.0949619752285));
#156920=CARTESIAN_POINT('Ctrl Pts',(24.4445773061652,6.47800912513651,59.0875904676371));
#156921=CARTESIAN_POINT('Ctrl Pts',(24.424864717198,6.44562482280525,59.0802452601898));
#156922=CARTESIAN_POINT('Ctrl Pts',(24.404885950674,6.41280323775635,59.0728008709772));
#156923=CARTESIAN_POINT('Ctrl Pts',(24.3848644759225,6.38081776632692,59.0653826750114));
#156924=CARTESIAN_POINT('Ctrl Pts',(24.3651060732623,6.35000154898329,59.0581016556061));
#156925=CARTESIAN_POINT('Ctrl Pts',(24.3628410088866,6.34646883850564,59.0572669738781));
#156926=CARTESIAN_POINT('Ctrl Pts',(24.3605794578841,6.34295149096412,59.0564340963457));
#156927=CARTESIAN_POINT('Ctrl Pts',(24.3583219236067,6.33945000449852,59.0556031925104));
#156928=CARTESIAN_POINT('Ctrl Pts',(24.336463351073,6.30554686661361,59.0475579672679));
#156929=CARTESIAN_POINT('Ctrl Pts',(24.3148854527657,6.27303962476164,59.0396629899984));
#156930=CARTESIAN_POINT('Ctrl Pts',(24.2935940583983,6.2419284012883,59.0319025816968));
#156931=CARTESIAN_POINT('Ctrl Pts',(24.277926063446,6.21903415190628,59.026191821941));
#156932=CARTESIAN_POINT('Ctrl Pts',(24.2627879209375,6.1973325497693,59.0206898120325));
#156933=CARTESIAN_POINT('Ctrl Pts',(24.2469567428589,6.1753998533279,59.0149448797223));
#156934=CARTESIAN_POINT('Ctrl Pts',(24.2412747753946,6.16752799016243,59.0128829663063));
#156935=CARTESIAN_POINT('Ctrl Pts',(24.2355032201345,6.15962598219805,59.0107897117168));
#156936=CARTESIAN_POINT('Ctrl Pts',(24.2295843206351,6.15162695325244,59.00864394815));
#156937=CARTESIAN_POINT('Ctrl Pts',(24.2071740996707,6.12134091677101,59.0005196277975));
#156938=CARTESIAN_POINT('Ctrl Pts',(24.1828968779168,6.08994168903005,58.9917330499567));
#156939=CARTESIAN_POINT('Ctrl Pts',(24.1567590267025,6.05742911732951,58.9822668028042));
#156940=CARTESIAN_POINT('Ctrl Pts',(24.1436901010953,6.04117283147924,58.9775336792279));
#156941=CARTESIAN_POINT('Ctrl Pts',(24.130156099934,6.02463821158091,58.972630395889));
#156942=CARTESIAN_POINT('Ctrl Pts',(24.1161584234387,6.00782526850175,58.9675530536827));
#156943=CARTESIAN_POINT('Ctrl Pts',(24.1103120661753,6.00080306935884,58.9654324191263));
#156944=CARTESIAN_POINT('Ctrl Pts',(24.104384809627,5.9937323219517,58.9632813984112));
#156945=CARTESIAN_POINT('Ctrl Pts',(24.0983768322138,5.98661301932856,58.9610996566914));
#156946=CARTESIAN_POINT('Ctrl Pts',(24.0971924913651,5.98520960511256,58.960669574209));
#156947=CARTESIAN_POINT('Ctrl Pts',(24.0960050137735,5.98380430425258,58.9602382977778));
#156948=CARTESIAN_POINT('Ctrl Pts',(24.094814393207,5.98239711735019,58.9598058292043));
#156949=CARTESIAN_POINT('Ctrl Pts',(24.0875839391932,5.97385148957186,58.9571795146414));
#156950=CARTESIAN_POINT('Ctrl Pts',(24.0810046985963,5.96612892210129,58.9547881649664));
#156951=CARTESIAN_POINT('Ctrl Pts',(24.0727754155857,5.95655150857973,58.9517959464497));
#156952=CARTESIAN_POINT('Ctrl Pts',(24.0384277390557,5.91657695657942,58.939306917504));
#156953=CARTESIAN_POINT('Ctrl Pts',(24.0034683094554,5.87778350909651,58.9265815786641));
#156954=CARTESIAN_POINT('Ctrl Pts',(23.9678590006497,5.84020063332123,58.9136741411516));
#156955=CARTESIAN_POINT('Ctrl Pts',(23.9294267951761,5.79963840809059,58.8997434778712));
#156956=CARTESIAN_POINT('Ctrl Pts',(23.8902385500751,5.76048641392004,58.8856000807678));
#156957=CARTESIAN_POINT('Ctrl Pts',(23.8502859274976,5.7227525434125,58.8712677102395));
#156958=CARTESIAN_POINT('Ctrl Pts',(23.805405414728,5.68036445101941,58.8551675371591));
#156959=CARTESIAN_POINT('Ctrl Pts',(23.7595617687446,5.63976597255917,58.838828744871));
#156960=CARTESIAN_POINT('Ctrl Pts',(23.7127716509388,5.60093054367276,58.8222377212516));
#156961=CARTESIAN_POINT('Ctrl Pts',(23.6918644204073,5.58357770716384,58.8148243533903));
#156962=CARTESIAN_POINT('Ctrl Pts',(23.6707684261098,5.56657640531636,58.8073600585289));
#156963=CARTESIAN_POINT('Ctrl Pts',(23.6494854904257,5.54992230229696,58.7998410902845));
#156964=CARTESIAN_POINT('Ctrl Pts',(23.6176306075869,5.52499554837809,58.7885871986198));
#156965=CARTESIAN_POINT('Ctrl Pts',(23.5854221965799,5.50089571208605,58.7772340560176));
#156966=CARTESIAN_POINT('Ctrl Pts',(23.5528180096955,5.47760370730453,58.7657468526803));
#156967=CARTESIAN_POINT('Ctrl Pts',(23.5047337231853,5.44325292176636,58.7488056549614));
#156968=CARTESIAN_POINT('Ctrl Pts',(23.4557908853586,5.41065789155379,58.7315749653625));
#156969=CARTESIAN_POINT('Ctrl Pts',(23.4058589113385,5.37973126957867,58.7140549978679));
#156970=CARTESIAN_POINT('Ctrl Pts',(23.3581929283751,5.35020814606693,58.697330113893));
#156971=CARTESIAN_POINT('Ctrl Pts',(23.309625572927,5.32220461048141,58.6803409902794));
#156972=CARTESIAN_POINT('Ctrl Pts',(23.2600149371473,5.29566903861262,58.6630604713512));
#156973=CARTESIAN_POINT('Ctrl Pts',(23.2302353959441,5.27974065665587,58.6526875761576));
#156974=CARTESIAN_POINT('Ctrl Pts',(23.2000793893166,5.26434172998107,58.6422092103898));
#156975=CARTESIAN_POINT('Ctrl Pts',(23.1695109923222,5.24946749702519,58.6316155554101));
#156976=CARTESIAN_POINT('Ctrl Pts',(23.1022132391417,5.21672117871492,58.6082931293689));
#156977=CARTESIAN_POINT('Ctrl Pts',(23.0342782701488,5.18723041932582,58.5848858537487));
#156978=CARTESIAN_POINT('Ctrl Pts',(22.9657107575351,5.16098338851324,58.5613832671255));
#156979=CARTESIAN_POINT('Ctrl Pts',(22.9395452804977,5.15096747783124,58.5524146409181));
#156980=CARTESIAN_POINT('Ctrl Pts',(22.9132873831954,5.14142404593434,58.54343172089));
#156981=CARTESIAN_POINT('Ctrl Pts',(22.8869360879741,5.13235319318208,58.534432507506));
#156982=CARTESIAN_POINT('Ctrl Pts',(22.8235569648741,5.11053632655834,58.512787945139));
#156983=CARTESIAN_POINT('Ctrl Pts',(22.7596400356896,5.09145100616448,58.4910506913766));
#156984=CARTESIAN_POINT('Ctrl Pts',(22.6952160503029,5.07504879209382,58.4692514386328));
#156985=CARTESIAN_POINT('Ctrl Pts',(22.6317741779036,5.05889662196822,58.4477845051194));
#156986=CARTESIAN_POINT('Ctrl Pts',(22.567840169145,5.04534570398895,58.4262570374071));
#156987=CARTESIAN_POINT('Ctrl Pts',(22.5034140292658,5.03438543356313,58.4046801529297));
#156988=CARTESIAN_POINT('Ctrl Pts',(22.4413570922322,5.02382821543768,58.3838967354549));
#156989=CARTESIAN_POINT('Ctrl Pts',(22.3788430671832,5.01567419676257,58.3630671436673));
#156990=CARTESIAN_POINT('Ctrl Pts',(22.3158512579248,5.00995481363774,58.3421896471645));
#156991=CARTESIAN_POINT('Ctrl Pts',(22.2669243643649,5.00551246386765,58.3259737127245));
#156992=CARTESIAN_POINT('Ctrl Pts',(22.2177087606478,5.00253960528567,58.3097286249063));
#156993=CARTESIAN_POINT('Ctrl Pts',(22.1681884154333,5.00107157112627,58.2934501084065));
#156994=CARTESIAN_POINT('Ctrl Pts',(22.1438610190086,5.00035038372731,58.2854531139918));
#156995=CARTESIAN_POINT('Ctrl Pts',(22.119459997522,4.99999267677634,58.277448008364));
#156996=CARTESIAN_POINT('Ctrl Pts',(22.0949867135254,5.00000000061885,58.2694348746444));
#156997=CARTESIAN_POINT('Origin',(1.07038457110909,25.,122.41156512159));
#156998=CARTESIAN_POINT('',(24.9372684584991,-7.5,59.2718640334));
#156999=CARTESIAN_POINT('',(24.9372723528391,-10.33198914208,59.2718657798));
#157000=CARTESIAN_POINT('Origin',(1.07038457110909,5.,122.41156512159));
#157001=CARTESIAN_POINT('Ctrl Pts',(22.0949841886482,-5.00000000380661,
58.2694426477661));
#157002=CARTESIAN_POINT('Ctrl Pts',(22.2805552764597,-4.99991534493558,
58.3302356171032));
#157003=CARTESIAN_POINT('Ctrl Pts',(22.5537696623475,-5.03100736632704,
58.4211274743539));
#157004=CARTESIAN_POINT('Ctrl Pts',(22.863600077902,-5.12191465893277,58.5263497471087));
#157005=CARTESIAN_POINT('Ctrl Pts',(22.9944789641351,-5.17258205687998,
58.5712471933459));
#157006=CARTESIAN_POINT('Ctrl Pts',(23.0813087371768,-5.20896190642875,
58.6011323892443));
#157007=CARTESIAN_POINT('Ctrl Pts',(23.1258275312192,-5.22908872234276,
58.6165074658168));
#157008=CARTESIAN_POINT('Ctrl Pts',(23.3342129069009,-5.32986577239622,
58.6887036403607));
#157009=CARTESIAN_POINT('Ctrl Pts',(23.4918466779593,-5.42782596721495,
58.7440466636716));
#157010=CARTESIAN_POINT('Ctrl Pts',(23.7147825492157,-5.60077409160701,
58.8231427665048));
#157011=CARTESIAN_POINT('Ctrl Pts',(23.822871677724,-5.69375011184404,58.8617117509264));
#157012=CARTESIAN_POINT('Ctrl Pts',(23.9430827095938,-5.81360056202562,
58.9049361286198));
#157013=CARTESIAN_POINT('Ctrl Pts',(24.0059055719926,-5.8808539531689,58.9276096919623));
#157014=CARTESIAN_POINT('Ctrl Pts',(24.0347942568544,-5.91306854597329,
58.9380583730788));
#157015=CARTESIAN_POINT('Ctrl Pts',(24.0511971638391,-5.93168007090743,
58.943996461702));
#157016=CARTESIAN_POINT('Ctrl Pts',(24.0562159179984,-5.93741363096873,
58.9458139752985));
#157017=CARTESIAN_POINT('Ctrl Pts',(24.1603795204009,-6.05697259641673,
58.9835454900929));
#157018=CARTESIAN_POINT('Ctrl Pts',(24.3053416434733,-6.24925311691998,
59.0364640156985));
#157019=CARTESIAN_POINT('Ctrl Pts',(24.4630575940089,-6.50573938967163,
59.0946110881264));
#157020=CARTESIAN_POINT('Ctrl Pts',(24.539070211985,-6.64202227575524,59.1227690617259));
#157021=CARTESIAN_POINT('Ctrl Pts',(24.5803619250404,-6.71968987555994,
59.1381006869307));
#157022=CARTESIAN_POINT('Ctrl Pts',(24.6001039998996,-6.75794394236028,
59.1454414917671));
#157023=CARTESIAN_POINT('Ctrl Pts',(24.610573951587,-6.77851360610602,59.1493371661886));
#157024=CARTESIAN_POINT('Ctrl Pts',(24.6125710338916,-6.78244756197933,
59.1500803383087));
#157025=CARTESIAN_POINT('Ctrl Pts',(24.6921945641985,-6.93949641873107,
59.1797123957439));
#157026=CARTESIAN_POINT('Ctrl Pts',(24.8002777276957,-7.1782747537386,59.2200813703637));
#157027=CARTESIAN_POINT('Ctrl Pts',(24.9372684584991,-7.5,59.2718640334));
#157028=CARTESIAN_POINT('Origin',(-6.80729512863291,91.08441266238,84.10819367738));
#157029=CARTESIAN_POINT('Origin',(-6.80729512863291,5.,84.10819367738));
#157030=CARTESIAN_POINT('Origin',(-6.80729512863291,-5.,84.10819367738));
#157031=CARTESIAN_POINT('Ctrl Pts',(-6.54682286213226,-4.99999999999969,
85.5854053069007));
#157032=CARTESIAN_POINT('Ctrl Pts',(-7.83114436700245,-5.0000000000004,
85.8118658401104));
#157033=CARTESIAN_POINT('Ctrl Pts',(-8.23395173884804,-4.9999999999997,
84.5714980228237));
#157034=CARTESIAN_POINT('Ctrl Pts',(-6.54682286213212,-5.41421633819426,
85.5854053069002));
#157035=CARTESIAN_POINT('Ctrl Pts',(-7.83114436700212,-5.41421633819497,
85.8118658401099));
#157036=CARTESIAN_POINT('Ctrl Pts',(-8.23395173884766,-5.41421633819427,
84.5714980228234));
#157037=CARTESIAN_POINT('Ctrl Pts',(-6.59768381767522,-5.7071101318881,
85.2969584943955));
#157038=CARTESIAN_POINT('Ctrl Pts',(-7.63122308057704,-5.70711013188867,
85.4791993520641));
#157039=CARTESIAN_POINT('Ctrl Pts',(-7.95537652082547,-5.70711013188811,
84.4810311872048));
#157040=CARTESIAN_POINT('Ctrl Pts',(-6.64854477321832,-6.00000392558194,
85.0085116818906));
#157041=CARTESIAN_POINT('Ctrl Pts',(-7.43130179415197,-6.00000392558238,
85.1465328640184));
#157042=CARTESIAN_POINT('Ctrl Pts',(-7.6768013028033,-6.00000392558195,
84.3905643515862));
#157043=CARTESIAN_POINT('Ctrl Pts',(-6.72047268550151,-5.99999999995607,
84.6005882206304));
#157044=CARTESIAN_POINT('Ctrl Pts',(-7.14857173924192,-5.99999999995631,
84.6760736342196));
#157045=CARTESIAN_POINT('Ctrl Pts',(-7.28283831818874,-5.99999999995607,
84.2626255319672));
#157046=CARTESIAN_POINT('Origin',(24.8472308208791,-7.5,80.448558349262));
#157047=CARTESIAN_POINT('Origin',(22.174314171959,-7.5,65.2896947528857));
#157048=CARTESIAN_POINT('Origin',(21.4524700019691,-7.5,61.19591303503));
#157049=CARTESIAN_POINT('Origin',(24.4068932609991,-7.5,60.67496850203));
#157050=CARTESIAN_POINT('Origin',(24.4068932609991,-7.5,60.67496850203));
#157051=CARTESIAN_POINT('Ctrl Pts',(21.7837557160991,-6.00001782727999,
59.21971079975));
#157052=CARTESIAN_POINT('Ctrl Pts',(22.0097728635713,-5.99997040176646,
59.2647219220221));
#157053=CARTESIAN_POINT('Ctrl Pts',(22.2385800253108,-6.04902617145881,
59.3042918067695));
#157054=CARTESIAN_POINT('Ctrl Pts',(22.6838933356787,-6.22980259915816,
59.3443479086447));
#157055=CARTESIAN_POINT('Ctrl Pts',(22.8999827744699,-6.3613180310625,59.3431175932148));
#157056=CARTESIAN_POINT('Ctrl Pts',(23.2438698401328,-6.59046668870961,
59.2922250056415));
#157057=CARTESIAN_POINT('Ctrl Pts',(23.362960063642,-6.67191371077529,59.2687253818218));
#157058=CARTESIAN_POINT('Ctrl Pts',(23.6232995629752,-6.83820229845214,
59.2174361530951));
#157059=CARTESIAN_POINT('Ctrl Pts',(23.7656062250204,-6.92283887189394,
59.1882921399419));
#157060=CARTESIAN_POINT('Ctrl Pts',(24.0739220072904,-7.09103974838947,
59.1494728679439));
#157061=CARTESIAN_POINT('Ctrl Pts',(24.2406714479517,-7.17440448969987,
59.1407005872925));
#157062=CARTESIAN_POINT('Ctrl Pts',(24.5896694075326,-7.33775746185597,
59.1698506720171));
#157063=CARTESIAN_POINT('Ctrl Pts',(24.7695305019998,-7.41833718706608,
59.2065810098722));
#157064=CARTESIAN_POINT('Ctrl Pts',(24.9372684584991,-7.5,59.2718640334));
#157065=CARTESIAN_POINT('Ctrl Pts',(21.5482687433291,-5.95510217575499,
59.47577881262));
#157066=CARTESIAN_POINT('Ctrl Pts',(21.6385071826491,-5.94997535511398,
59.49548084013));
#157067=CARTESIAN_POINT('Ctrl Pts',(21.9131048476991,-5.95866966306399,
59.55304861875));
#157068=CARTESIAN_POINT('Ctrl Pts',(22.3692704752191,-6.096989384513,59.62812563708));
#157069=CARTESIAN_POINT('Ctrl Pts',(22.8683422761291,-6.43730726581498,
59.62980972532));
#157070=CARTESIAN_POINT('Ctrl Pts',(23.3387245707791,-6.87259544505199,
59.46695082988));
#157071=CARTESIAN_POINT('Ctrl Pts',(23.9310250958291,-7.279114747789,59.2220355884));
#157072=CARTESIAN_POINT('Ctrl Pts',(24.4618176914991,-7.52767454181498,
59.18139023564));
#157073=CARTESIAN_POINT('Ctrl Pts',(24.7197883064391,-7.649504286858,59.22728137109));
#157074=CARTESIAN_POINT('Ctrl Pts',(24.7477189671291,-7.66272970212499,
59.23310715875));
#157075=CARTESIAN_POINT('Ctrl Pts',(21.8418959298291,-6.24534546095398,
58.65317069173));
#157076=CARTESIAN_POINT('Ctrl Pts',(21.9183808576391,-6.23320434561899,
58.66549890254));
#157077=CARTESIAN_POINT('Ctrl Pts',(22.1557327029891,-6.21340282184399,
58.70105855136));
#157078=CARTESIAN_POINT('Ctrl Pts',(22.5805331464491,-6.26715359928599,
58.7456295618));
#157079=CARTESIAN_POINT('Ctrl Pts',(23.1393556500491,-6.45444111416999,
58.74233013357));
#157080=CARTESIAN_POINT('Ctrl Pts',(23.8323620899991,-6.71775933814998,
58.67382657826));
#157081=CARTESIAN_POINT('Ctrl Pts',(24.7190342437791,-6.99392094430899,
58.74842003095));
#157082=CARTESIAN_POINT('Ctrl Pts',(25.3277236543091,-7.18300713584699,
59.06935222318));
#157083=CARTESIAN_POINT('Ctrl Pts',(25.5632336614691,-7.28727303124799,
59.28910840377));
#157084=CARTESIAN_POINT('Ctrl Pts',(25.5879717422591,-7.29878131891499,
59.31371561786));
#157085=CARTESIAN_POINT('Ctrl Pts',(21.9922347994691,-5.60881868005499,
58.00554653487));
#157086=CARTESIAN_POINT('Ctrl Pts',(22.1021455439091,-5.58702360762799,
58.03513218664));
#157087=CARTESIAN_POINT('Ctrl Pts',(22.4427011606791,-5.54540958548999,
58.12636252562));
#157088=CARTESIAN_POINT('Ctrl Pts',(23.0461698531791,-5.600768961777,58.28727323461));
#157089=CARTESIAN_POINT('Ctrl Pts',(23.8041883710391,-5.84404758049099,
58.48483376287));
#157090=CARTESIAN_POINT('Ctrl Pts',(24.6291238424591,-6.20144908664698,
58.74340456943));
#157091=CARTESIAN_POINT('Ctrl Pts',(25.4282103275791,-6.59406976343999,
59.26219347932));
#157092=CARTESIAN_POINT('Ctrl Pts',(25.7747832871991,-6.87348915556999,
59.8344135724));
#157093=CARTESIAN_POINT('Ctrl Pts',(25.8574257339091,-7.03298482887899,
60.12294471837));
#157094=CARTESIAN_POINT('Ctrl Pts',(25.8653237391391,-7.05066785691398,
60.1543045333201));
#157095=CARTESIAN_POINT('Ctrl Pts',(21.8377989953191,-4.72924648248199,
58.22855122752));
#157096=CARTESIAN_POINT('Ctrl Pts',(21.9924105746991,-4.70552757959199,
58.2814885137601));
#157097=CARTESIAN_POINT('Ctrl Pts',(22.4657633189691,-4.67221426727299,
58.44626974282));
#157098=CARTESIAN_POINT('Ctrl Pts',(23.2660173601391,-4.81363191030199,
58.74539967786));
#157099=CARTESIAN_POINT('Ctrl Pts',(24.1487109904791,-5.26178031101699,
59.1339101002101));
#157100=CARTESIAN_POINT('Ctrl Pts',(24.8731689331391,-5.87825886677599,
59.60094766893));
#157101=CARTESIAN_POINT('Ctrl Pts',(25.2967925166891,-6.509060979056,60.211486662));
#157102=CARTESIAN_POINT('Ctrl Pts',(25.3227879014891,-6.93158905149599,
60.65478434692));
#157103=CARTESIAN_POINT('Ctrl Pts',(25.2863583828791,-7.15978311571299,
60.83312581344));
#157104=CARTESIAN_POINT('Ctrl Pts',(25.2818575683891,-7.18490016046499,
60.85195610375));
#157105=CARTESIAN_POINT('Origin',(24.4068932609991,-15.54362135317,60.67496850203));
#157106=CARTESIAN_POINT('Ctrl Pts',(-6.72047268773407,5.99999999995523,
84.6005882079846));
#157107=CARTESIAN_POINT('Ctrl Pts',(-7.14857173047982,5.99999999995525,
84.6760736196361));
#157108=CARTESIAN_POINT('Ctrl Pts',(-7.28283830597694,5.99999999995523,
84.2626255280015));
#157109=CARTESIAN_POINT('Ctrl Pts',(-6.64854477479676,6.00000393090208,
85.0085116729493));
#157110=CARTESIAN_POINT('Ctrl Pts',(-7.43130178795857,6.00000393090212,
85.1465328537084));
#157111=CARTESIAN_POINT('Ctrl Pts',(-7.67680129416981,6.00000393090208,
84.390564348781));
#157112=CARTESIAN_POINT('Ctrl Pts',(-6.59768381846433,5.70711013642924,
85.296958489926));
#157113=CARTESIAN_POINT('Ctrl Pts',(-7.63122307748394,5.70711013642929,
85.4791993469125));
#157114=CARTESIAN_POINT('Ctrl Pts',(-7.95537651651139,5.70711013642924,
84.4810311858011));
#157115=CARTESIAN_POINT('Ctrl Pts',(-6.54682286213189,5.4142163419564,85.5854053069028));
#157116=CARTESIAN_POINT('Ctrl Pts',(-7.83114436700931,5.41421634195645,
85.8118658401166));
#157117=CARTESIAN_POINT('Ctrl Pts',(-8.23395173885296,5.4142163419564,84.5714980228211));
#157118=CARTESIAN_POINT('Ctrl Pts',(-6.54682286213193,4.99999999999998,
85.5854053069027));
#157119=CARTESIAN_POINT('Ctrl Pts',(-7.83114436700921,5.00000000000003,
85.8118658401165));
#157120=CARTESIAN_POINT('Ctrl Pts',(-8.23395173885283,4.99999999999998,
84.5714980228211));
#157121=CARTESIAN_POINT('Origin',(-7.28284733203891,5.,84.2626284592));
#157122=CARTESIAN_POINT('Origin',(27.4324635166691,5.,72.98888938658));
#157123=CARTESIAN_POINT('Origin',(1.07038457110909,5.,122.41156512159));
#157124=CARTESIAN_POINT('Origin',(23.9011399714191,10.33198915989,57.80669906563));
#157125=CARTESIAN_POINT('Origin',(24.4127075916591,10.33198621001,60.7079432098));
#157126=CARTESIAN_POINT('Ctrl Pts',(25.7146057871591,10.98822408556,60.32011578917));
#157127=CARTESIAN_POINT('Ctrl Pts',(25.7333595485691,10.98640264379,60.42647365532));
#157128=CARTESIAN_POINT('Ctrl Pts',(25.7902717155191,10.98675745301,60.74923859301));
#157129=CARTESIAN_POINT('Ctrl Pts',(25.8903004917691,11.01610949404,61.31652997325));
#157130=CARTESIAN_POINT('Ctrl Pts',(26.0187410371091,11.09765362491,62.0449525029099));
#157131=CARTESIAN_POINT('Ctrl Pts',(26.1595638381891,11.23024105092,62.84359829445));
#157132=CARTESIAN_POINT('Ctrl Pts',(26.3108478437791,11.41227085738,63.701572524988));
#157133=CARTESIAN_POINT('Ctrl Pts',(26.4698526384791,11.63683182579,64.603333526392));
#157134=CARTESIAN_POINT('Ctrl Pts',(26.6325918522091,11.8932379924,65.526273470543));
#157135=CARTESIAN_POINT('Ctrl Pts',(26.7914529063091,12.16230532054,66.4272192784869));
#157136=CARTESIAN_POINT('Ctrl Pts',(26.9386924978091,12.42231805601,67.26225649691));
#157137=CARTESIAN_POINT('Ctrl Pts',(27.0699044264391,12.65926655649,68.006396322292));
#157138=CARTESIAN_POINT('Ctrl Pts',(27.1862753385091,12.87066869904,68.666368560249));
#157139=CARTESIAN_POINT('Ctrl Pts',(27.2910527846991,13.06027210397,69.260590985898));
#157140=CARTESIAN_POINT('Ctrl Pts',(27.3865217178491,13.23082661369,69.802022210807));
#157141=CARTESIAN_POINT('Ctrl Pts',(27.4739349518891,13.38351975338,70.297767295838));
#157142=CARTESIAN_POINT('Ctrl Pts',(27.5540499498591,13.51934191737,70.7521220272789));
#157143=CARTESIAN_POINT('Ctrl Pts',(27.6273676469791,13.63888432267,71.167927350015));
#157144=CARTESIAN_POINT('Ctrl Pts',(27.6946527386791,13.74332636095,71.549520067312));
#157145=CARTESIAN_POINT('Ctrl Pts',(27.7566735256291,13.8340404781,71.901257428796));
#157146=CARTESIAN_POINT('Ctrl Pts',(27.8139535058191,13.91189665278,72.2261083390753));
#157147=CARTESIAN_POINT('Ctrl Pts',(27.8668525364891,13.97757339522,72.5261136499739));
#157148=CARTESIAN_POINT('Ctrl Pts',(27.9156547649191,14.03175427646,72.8028848408233));
#157149=CARTESIAN_POINT('Ctrl Pts',(27.9606578091391,14.07512867792,73.0581097873241));
#157150=CARTESIAN_POINT('Ctrl Pts',(28.0020959597691,14.10837762916,73.2931172176315));
#157151=CARTESIAN_POINT('Ctrl Pts',(28.0400945627891,14.132263698,73.5086180041178));
#157152=CARTESIAN_POINT('Ctrl Pts',(28.0747458485391,14.14767670304,73.7051352110367));
#157153=CARTESIAN_POINT('Ctrl Pts',(28.1061814400091,14.15583570334,73.8834153093887));
#157154=CARTESIAN_POINT('Ctrl Pts',(28.1346527710791,14.15817719874,74.0448842516899));
#157155=CARTESIAN_POINT('Ctrl Pts',(28.1589709875791,14.15615234085,74.182799710788));
#157156=CARTESIAN_POINT('Ctrl Pts',(28.1738163949191,14.1529441735,74.266992199549));
#157157=CARTESIAN_POINT('Ctrl Pts',(28.1801055443791,14.15123724658,74.302659738554));
#157158=CARTESIAN_POINT('Ctrl Pts',(24.6968047233291,13.13053120709,60.53629255394));
#157159=CARTESIAN_POINT('Ctrl Pts',(24.7110977510391,13.12914347929,60.61735234215));
#157160=CARTESIAN_POINT('Ctrl Pts',(24.7550666420191,13.12935201228,60.86671231419));
#157161=CARTESIAN_POINT('Ctrl Pts',(24.8353614835591,13.15257479162,61.32208698922));
#157162=CARTESIAN_POINT('Ctrl Pts',(24.9432706425091,13.22070256323,61.93407024056));
#157163=CARTESIAN_POINT('Ctrl Pts',(25.0665147321391,13.33640433196,62.63302220545));
#157164=CARTESIAN_POINT('Ctrl Pts',(25.2036262415691,13.50112442483,63.410620216152));
#157165=CARTESIAN_POINT('Ctrl Pts',(25.3518667357391,13.7103233706,64.251333835632));
#157166=CARTESIAN_POINT('Ctrl Pts',(25.5064342999091,13.95375958956,65.127930052254));
#157167=CARTESIAN_POINT('Ctrl Pts',(25.6600936118891,14.21395978547,65.9993753146631));
#157168=CARTESIAN_POINT('Ctrl Pts',(25.8041861213491,14.46839546703,66.816564543937));
#157169=CARTESIAN_POINT('Ctrl Pts',(25.9339809461091,14.7027763825,67.55266757384));
#157170=CARTESIAN_POINT('Ctrl Pts',(26.0503244280891,14.91412817094,68.212484248023));
#157171=CARTESIAN_POINT('Ctrl Pts',(26.1558873440491,15.10515684937,68.811161294153));
#157172=CARTESIAN_POINT('Ctrl Pts',(26.2531435947691,15.27891270155,69.362728900733));
#157173=CARTESIAN_POINT('Ctrl Pts',(26.3431374759891,15.43612444966,69.873109563156));
#157174=CARTESIAN_POINT('Ctrl Pts',(26.4265245286691,15.57750958702,70.3460210390141));
#157175=CARTESIAN_POINT('Ctrl Pts',(26.5039740022191,15.70380916865,70.7852588302931));
#157176=CARTESIAN_POINT('Ctrl Pts',(26.5761186635391,15.81581819599,71.194411536424));
#157177=CARTESIAN_POINT('Ctrl Pts',(26.6437790448791,15.91481279583,71.578132627044));
#157178=CARTESIAN_POINT('Ctrl Pts',(26.7076333815191,16.00164468556,71.940268565508));
#157179=CARTESIAN_POINT('Ctrl Pts',(26.7680135964591,16.07665708509,72.2827017807608));
#157180=CARTESIAN_POINT('Ctrl Pts',(26.8252747392791,16.14028901932,72.607445859035));
#157181=CARTESIAN_POINT('Ctrl Pts',(26.8798137168691,16.19292482343,72.9167517710934));
#157182=CARTESIAN_POINT('Ctrl Pts',(26.9317722155091,16.23468871587,73.2114230597839));
#157183=CARTESIAN_POINT('Ctrl Pts',(26.9811069681591,16.26578384666,73.4912143455473));
#157184=CARTESIAN_POINT('Ctrl Pts',(27.0277124764791,16.28657491746,73.7555273176114));
#157185=CARTESIAN_POINT('Ctrl Pts',(27.0708769258191,16.29781123553,74.000325074377));
#157186=CARTESIAN_POINT('Ctrl Pts',(27.1105081190591,16.3010840103,74.225084740104));
#157187=CARTESIAN_POINT('Ctrl Pts',(27.1444134164591,16.29825389057,74.417371236858));
#157188=CARTESIAN_POINT('Ctrl Pts',(27.1648328335891,16.2938285752,74.5331755059949));
#157189=CARTESIAN_POINT('Ctrl Pts',(27.1733925807291,16.29148605459,74.581720244281));
#157190=CARTESIAN_POINT('Ctrl Pts',(22.4731286993091,12.36649813187,60.9152940194));
#157191=CARTESIAN_POINT('Ctrl Pts',(22.4890126044691,12.36495572419,61.00537612196));
#157192=CARTESIAN_POINT('Ctrl Pts',(22.5375975893991,12.36521642518,61.2809152636801));
#157193=CARTESIAN_POINT('Ctrl Pts',(22.6249303475291,12.39062514631,61.7762039471101));
#157194=CARTESIAN_POINT('Ctrl Pts',(22.7401618264791,12.46353773244,62.42971413873));
#157195=CARTESIAN_POINT('Ctrl Pts',(22.8696751931991,12.58526160721,63.1642209408299));
#157196=CARTESIAN_POINT('Ctrl Pts',(23.0118411860591,12.7561550417,63.970484351462));
#157197=CARTESIAN_POINT('Ctrl Pts',(23.1639206636991,12.97083270398,64.8329699281351));
#157198=CARTESIAN_POINT('Ctrl Pts',(23.3214025674991,13.21889452908,65.726094186094));
#157199=CARTESIAN_POINT('Ctrl Pts',(23.4769170303891,13.48225710178,66.608060532198));
#157200=CARTESIAN_POINT('Ctrl Pts',(23.6221319161691,13.73868178557,67.431615073849));
#157201=CARTESIAN_POINT('Ctrl Pts',(23.7524321372891,13.97397840535,68.17058434898));
#157202=CARTESIAN_POINT('Ctrl Pts',(23.8687854019491,14.1853481521,68.830456503476));
#157203=CARTESIAN_POINT('Ctrl Pts',(23.9740681877291,14.37586852055,69.427544852378));
#157204=CARTESIAN_POINT('Ctrl Pts',(24.0706870089591,14.54848264496,69.9754974166599));
#157205=CARTESIAN_POINT('Ctrl Pts',(24.1597605273691,14.70408287517,70.48065844223));
#157206=CARTESIAN_POINT('Ctrl Pts',(24.2419806334391,14.84348403198,70.946951835013));
#157207=CARTESIAN_POINT('Ctrl Pts',(24.3179565489691,14.96737373215,71.3778326634539));
#157208=CARTESIAN_POINT('Ctrl Pts',(24.3883680918691,15.07668406617,71.7771563666341));
#157209=CARTESIAN_POINT('Ctrl Pts',(24.4540171665291,15.17272551209,72.1494707701902));
#157210=CARTESIAN_POINT('Ctrl Pts',(24.5155268226391,15.25635630003,72.4983093646567));
#157211=CARTESIAN_POINT('Ctrl Pts',(24.5732389457091,15.32803922793,72.825611078962));
#157212=CARTESIAN_POINT('Ctrl Pts',(24.6274832986791,15.38830053569,73.1332460918097));
#157213=CARTESIAN_POINT('Ctrl Pts',(24.6786213780391,15.4376333503,73.4232645515648));
#157214=CARTESIAN_POINT('Ctrl Pts',(24.7268278965091,15.47636047147,73.6966573033259));
#157215=CARTESIAN_POINT('Ctrl Pts',(24.7721197212391,15.50488456017,73.9535200055188));
#157216=CARTESIAN_POINT('Ctrl Pts',(24.8144618719291,15.52375759594,74.193654274908));
#157217=CARTESIAN_POINT('Ctrl Pts',(24.8534433377591,15.53389641844,74.414729153379));
#157218=CARTESIAN_POINT('Ctrl Pts',(24.8890944742991,15.53683706144,74.616916795904));
#157219=CARTESIAN_POINT('Ctrl Pts',(24.9195806321991,15.53429413055,74.7898123889521));
#157220=CARTESIAN_POINT('Ctrl Pts',(24.9380121327491,15.53030289923,74.894342622946));
#157221=CARTESIAN_POINT('Ctrl Pts',(24.9457620932291,15.52818705695,74.938294832893));
#157222=CARTESIAN_POINT('Ctrl Pts',(22.9354926719291,10.03334832269,60.79378548384));
#157223=CARTESIAN_POINT('Ctrl Pts',(22.9562346853791,10.03133356459,60.91141928763));
#157224=CARTESIAN_POINT('Ctrl Pts',(23.0189159693591,10.0317535725,61.26690251386));
#157225=CARTESIAN_POINT('Ctrl Pts',(23.1277406160991,10.06383756704,61.88407775444));
#157226=CARTESIAN_POINT('Ctrl Pts',(23.2653324745291,10.15136167908,62.6643999597399));
#157227=CARTESIAN_POINT('Ctrl Pts',(23.4139905132991,10.29147543254,63.507481592353));
#157228=CARTESIAN_POINT('Ctrl Pts',(23.5715915277691,10.48122057813,64.401281360441));
#157229=CARTESIAN_POINT('Ctrl Pts',(23.7353942198291,10.71262875484,65.330252589921));
#157230=CARTESIAN_POINT('Ctrl Pts',(23.9017757264891,10.97481592666,66.2738490037879));
#157231=CARTESIAN_POINT('Ctrl Pts',(24.0629553171891,11.24783554043,67.187943886222));
#157232=CARTESIAN_POINT('Ctrl Pts',(24.2115976358491,11.51033409764,68.0309363656259));
#157233=CARTESIAN_POINT('Ctrl Pts',(24.3434412004091,11.74842703006,68.778658376371));
#157234=CARTESIAN_POINT('Ctrl Pts',(24.4598243387091,11.9598516166,69.438699952696));
#157235=CARTESIAN_POINT('Ctrl Pts',(24.5642516828691,12.14881974422,70.030936851112));
#157236=CARTESIAN_POINT('Ctrl Pts',(24.6589239672891,12.31794734167,70.5678500566009));
#157237=CARTESIAN_POINT('Ctrl Pts',(24.7451869472891,12.46862643321,71.057071726764));
#157238=CARTESIAN_POINT('Ctrl Pts',(24.8238435148991,12.60196905149,71.5031552886309));
#157239=CARTESIAN_POINT('Ctrl Pts',(24.8953195838391,12.71849962724,71.90851621894));
#157240=CARTESIAN_POINT('Ctrl Pts',(24.9604386531191,12.81956888374,72.2778248126876));
#157241=CARTESIAN_POINT('Ctrl Pts',(25.0199457425991,12.90659219849,72.6153062873973));
#157242=CARTESIAN_POINT('Ctrl Pts',(25.0742953802791,12.98044768968,72.923538399479));
#157243=CARTESIAN_POINT('Ctrl Pts',(25.1238598743391,13.04196331413,73.2046326134905));
#157244=CARTESIAN_POINT('Ctrl Pts',(25.1688917692491,13.09193164278,73.4600211804315));
#157245=CARTESIAN_POINT('Ctrl Pts',(25.2096444277191,13.13117802317,73.6911409915274));
#157246=CARTESIAN_POINT('Ctrl Pts',(25.2463934162691,13.16063166845,73.8995548621547));
#157247=CARTESIAN_POINT('Ctrl Pts',(25.2793392355791,13.18130449189,74.086399888258));
#157248=CARTESIAN_POINT('Ctrl Pts',(25.3086622482391,13.19432036881,74.252698956838));
#157249=CARTESIAN_POINT('Ctrl Pts',(25.3348700168591,13.20110773749,74.4013305985409));
#157250=CARTESIAN_POINT('Ctrl Pts',(25.3583671396191,13.20303414017,74.534589403646));
#157251=CARTESIAN_POINT('Ctrl Pts',(25.3784121727291,13.20136820609,74.6482704355061));
#157252=CARTESIAN_POINT('Ctrl Pts',(25.3907731151691,13.19870254972,74.7183728236471));
#157253=CARTESIAN_POINT('Ctrl Pts',(25.3960502068091,13.19727892159,74.748300697519));
#157254=CARTESIAN_POINT('',(26.0143554277394,12.1868334151086,64.6125968688177));
#157255=CARTESIAN_POINT('Ctrl Pts',(25.5858158203339,11.2436003008624,60.5011154491916));
#157256=CARTESIAN_POINT('Ctrl Pts',(25.5923235730551,11.2475657971982,60.5554809329124));
#157257=CARTESIAN_POINT('Ctrl Pts',(25.5988047894408,11.2520203456228,60.6098721686439));
#157258=CARTESIAN_POINT('Ctrl Pts',(25.605257698237,11.256943112575,60.6642809059383));
#157259=CARTESIAN_POINT('Ctrl Pts',(25.628778699609,11.2748867116392,60.8626020080901));
#157260=CARTESIAN_POINT('Ctrl Pts',(25.6519238690939,11.2990477224041,61.0611576275081));
#157261=CARTESIAN_POINT('Ctrl Pts',(25.6746441124549,11.3284665051122,61.2597526248882));
#157262=CARTESIAN_POINT('Ctrl Pts',(25.6762586313419,11.3305570276282,61.2738649461799));
#157263=CARTESIAN_POINT('Ctrl Pts',(25.6778710031456,11.3326741191816,61.2879774559578));
#157264=CARTESIAN_POINT('Ctrl Pts',(25.6794812096262,11.3348174442319,61.3020900794107));
#157265=CARTESIAN_POINT('Ctrl Pts',(25.7033718798831,11.3666180068602,61.5114793952784));
#157266=CARTESIAN_POINT('Ctrl Pts',(25.7267862729606,11.4041904957477,61.7208967603058));
#157267=CARTESIAN_POINT('Ctrl Pts',(25.7496897387169,11.4465219413156,61.9302341410493));
#157268=CARTESIAN_POINT('Ctrl Pts',(25.7528247338991,11.4523162118999,61.9588879564619));
#157269=CARTESIAN_POINT('Ctrl Pts',(25.755950149292,11.4581997014192,61.9875402170144));
#157270=CARTESIAN_POINT('Ctrl Pts',(25.7590658892414,11.4641698655163,62.0161905917651));
#157271=CARTESIAN_POINT('Ctrl Pts',(25.7787469805256,11.5018814032199,62.1971654644923));
#157272=CARTESIAN_POINT('Ctrl Pts',(25.7980422182077,11.5430503853908,62.3780667868344));
#157273=CARTESIAN_POINT('Ctrl Pts',(25.8169425291683,11.5871162706067,62.5588925163166));
#157274=CARTESIAN_POINT('Ctrl Pts',(25.8253132742067,11.6066325786085,62.6389782927385));
#157275=CARTESIAN_POINT('Ctrl Pts',(25.8336064365499,11.6267173328886,62.7190489153338));
#157276=CARTESIAN_POINT('Ctrl Pts',(25.8418207621813,11.6473228008902,62.7991028537887));
#157277=CARTESIAN_POINT('Ctrl Pts',(25.8651810053786,11.7059214936263,63.0267635961452));
#157278=CARTESIAN_POINT('Ctrl Pts',(25.887904167324,11.7687308903864,63.2542930833719));
#157279=CARTESIAN_POINT('Ctrl Pts',(25.9099789732516,11.8348056312976,63.4817489544971));
#157280=CARTESIAN_POINT('Ctrl Pts',(25.9152209326329,11.8504959666563,63.5357614083949));
#157281=CARTESIAN_POINT('Ctrl Pts',(25.9204263011686,11.8663704736009,63.5897694858818));
#157282=CARTESIAN_POINT('Ctrl Pts',(25.9255948715915,11.8824165709964,63.6437735380379));
#157283=CARTESIAN_POINT('Ctrl Pts',(25.946675266075,11.947861758997,63.8640330353503));
#157284=CARTESIAN_POINT('Ctrl Pts',(25.9671440608878,12.0161618413149,64.0842296705477));
#157285=CARTESIAN_POINT('Ctrl Pts',(25.9869839824368,12.0866833807512,64.3043607663581));
#157286=CARTESIAN_POINT('Ctrl Pts',(25.9939764388603,12.1115382568256,64.3819445960675));
#157287=CARTESIAN_POINT('Ctrl Pts',(26.0008907192042,12.1366690213426,64.4595198159898));
#157288=CARTESIAN_POINT('Ctrl Pts',(26.0077258813949,12.1620477668799,64.5370847939509));
#157289=CARTESIAN_POINT('Ctrl Pts',(26.0099440547828,12.1702837759751,64.5622564819295));
#157290=CARTESIAN_POINT('Ctrl Pts',(26.0121538949578,12.1785459005521,64.5874270845108));
#157291=CARTESIAN_POINT('Ctrl Pts',(26.0143554277394,12.1868334151086,64.6125968688177));
#157292=CARTESIAN_POINT('Ctrl Pts',(26.0143539439513,12.186832623157,64.61259213409));
#157293=CARTESIAN_POINT('Ctrl Pts',(25.8692560444075,12.300907833433,64.6381768086237));
#157294=CARTESIAN_POINT('Ctrl Pts',(25.7047067450537,12.3865457859842,64.6671912897573));
#157295=CARTESIAN_POINT('Ctrl Pts',(25.3555088143332,12.4896377963212,64.7287643065509));
#157296=CARTESIAN_POINT('Ctrl Pts',(25.1748447519745,12.507191289845,64.7606202551849));
#157297=CARTESIAN_POINT('Ctrl Pts',(24.8063198993144,12.4721236628825,64.8256011297705));
#157298=CARTESIAN_POINT('Ctrl Pts',(24.6229546423116,12.4160836022829,64.857933371908));
#157299=CARTESIAN_POINT('Ctrl Pts',(24.2905142312325,12.2372428251354,64.9165515858591));
#157300=CARTESIAN_POINT('Ctrl Pts',(24.144206218523,12.1176245261334,64.9423496360033));
#157301=CARTESIAN_POINT('Ctrl Pts',(23.9019362111796,11.8306644216987,64.9850683749143));
#157302=CARTESIAN_POINT('Ctrl Pts',(23.8078592158878,11.6657964361489,65.0016566874339));
#157303=CARTESIAN_POINT('Ctrl Pts',(23.6829831124488,11.3148237115169,65.0236757137159));
#157304=CARTESIAN_POINT('Ctrl Pts',(23.6515252125594,11.1316314922004,65.0292225902275));
#157305=CARTESIAN_POINT('Ctrl Pts',(23.6515258014821,10.9472980747274,65.0292224863845));
#157306=CARTESIAN_POINT('Ctrl Pts',(25.6728519466291,11.05620868577,60.1753393120401));
#157307=CARTESIAN_POINT('Ctrl Pts',(25.5908811595391,11.17010610055,60.1922130334301));
#157308=CARTESIAN_POINT('Ctrl Pts',(25.0176949940091,11.96220506401,60.3226366877));
#157309=CARTESIAN_POINT('Ctrl Pts',(23.9454509711491,13.3937300709,60.72216890038));
#157310=CARTESIAN_POINT('Ctrl Pts',(22.4585522519091,15.28518638036,61.63777386195));
#157311=CARTESIAN_POINT('Ctrl Pts',(21.0802507927691,16.97737598619,62.82703989993));
#157312=CARTESIAN_POINT('Ctrl Pts',(19.8267910571591,18.48224713566,64.271659173669));
#157313=CARTESIAN_POINT('Ctrl Pts',(18.7098146781291,19.81562337201,66.003616761918));
#157314=CARTESIAN_POINT('Ctrl Pts',(17.7716110472991,20.96488749236,68.078902873165));
#157315=CARTESIAN_POINT('Ctrl Pts',(17.1084342304291,21.8744622819,70.533431788808));
#157316=CARTESIAN_POINT('Ctrl Pts',(16.8638554479991,22.45052823568,73.2803532769174));
#157317=CARTESIAN_POINT('Ctrl Pts',(17.0786448222291,22.59937448267,75.596712572949));
#157318=CARTESIAN_POINT('Ctrl Pts',(17.3662061271091,22.55171003512,76.874515663416));
#157319=CARTESIAN_POINT('Ctrl Pts',(17.4669987734891,22.52571394401,77.2562285499651));
#157320=CARTESIAN_POINT('Ctrl Pts',(27.6093946371291,9.39445532140801,64.447920892227));
#157321=CARTESIAN_POINT('Ctrl Pts',(27.5226174428891,9.46737944809301,64.451034788112));
#157322=CARTESIAN_POINT('Ctrl Pts',(26.9160359092391,9.97752475953103,64.482341733254));
#157323=CARTESIAN_POINT('Ctrl Pts',(25.7838601800091,10.93479181558,64.661006837171));
#157324=CARTESIAN_POINT('Ctrl Pts',(24.2207011124691,12.25908842062,65.194134063823));
#157325=CARTESIAN_POINT('Ctrl Pts',(22.7783053134691,13.48485509378,65.959148542412));
#157326=CARTESIAN_POINT('Ctrl Pts',(21.4726982157391,14.6052048364,66.94431046259));
#157327=CARTESIAN_POINT('Ctrl Pts',(20.3137223160191,15.62131353079,68.176238741846));
#157328=CARTESIAN_POINT('Ctrl Pts',(19.3392518035291,16.51491733119,69.702089136366));
#157329=CARTESIAN_POINT('Ctrl Pts',(18.6353752499191,17.23396255898,71.553480602797));
#157330=CARTESIAN_POINT('Ctrl Pts',(18.3290383767791,17.69470562174,73.6596809561242));
#157331=CARTESIAN_POINT('Ctrl Pts',(18.4647369076291,17.81439079021,75.444726555105));
#157332=CARTESIAN_POINT('Ctrl Pts',(18.6950959018691,17.77610222599,76.424554931989));
#157333=CARTESIAN_POINT('Ctrl Pts',(18.7775986176291,17.7552396856,76.716506355083));
#157334=CARTESIAN_POINT('Ctrl Pts',(31.5629272267991,9.88281068194302,67.430842306303));
#157335=CARTESIAN_POINT('Ctrl Pts',(31.4711681472091,9.92967730101103,67.444807195928));
#157336=CARTESIAN_POINT('Ctrl Pts',(30.8310903628191,10.25631090589,67.5476759313801));
#157337=CARTESIAN_POINT('Ctrl Pts',(29.6521222456891,10.85487243909,67.805767900236));
#157338=CARTESIAN_POINT('Ctrl Pts',(28.0597002587091,11.65964394348,68.317830215232));
#157339=CARTESIAN_POINT('Ctrl Pts',(26.6228516811691,12.38921116325,68.938303098405));
#157340=CARTESIAN_POINT('Ctrl Pts',(25.3542093351291,13.0450930181,69.658831925755));
#157341=CARTESIAN_POINT('Ctrl Pts',(24.2590278301191,13.63170757615,70.4940295766521));
#157342=CARTESIAN_POINT('Ctrl Pts',(23.3629396071591,14.14148255666,71.468571308628));
#157343=CARTESIAN_POINT('Ctrl Pts',(22.7218359561591,14.5476997234,72.5973874861561));
#157344=CARTESIAN_POINT('Ctrl Pts',(22.4115473378591,14.8062209636,73.8396950223705));
#157345=CARTESIAN_POINT('Ctrl Pts',(22.4566140195691,14.87316749049,74.870971069554));
#157346=CARTESIAN_POINT('Ctrl Pts',(22.5996423578891,14.85173828971,75.432105059216));
#157347=CARTESIAN_POINT('Ctrl Pts',(22.6529499976691,14.84005551372,75.5989411619891));
#157348=CARTESIAN_POINT('Ctrl Pts',(35.8805628265291,12.31710390136,67.87700830848));
#157349=CARTESIAN_POINT('Ctrl Pts',(35.7857292024291,12.36372287642,67.921898444141));
#157350=CARTESIAN_POINT('Ctrl Pts',(35.1260583462191,12.68200901524,68.23708902494));
#157351=CARTESIAN_POINT('Ctrl Pts',(33.9330000499891,13.18738451274,68.8416951696051));
#157352=CARTESIAN_POINT('Ctrl Pts',(32.3705467692491,13.73746778379,69.702912182422));
#157353=CARTESIAN_POINT('Ctrl Pts',(31.0065678005891,14.14850934188,70.5189831644171));
#157354=CARTESIAN_POINT('Ctrl Pts',(29.8485481528991,14.4541608558,71.28034056044));
#157355=CARTESIAN_POINT('Ctrl Pts',(28.8962838945291,14.67861693811,71.987970801025));
#157356=CARTESIAN_POINT('Ctrl Pts',(28.1604571839791,14.83686516773,72.6398212113681));
#157357=CARTESIAN_POINT('Ctrl Pts',(27.6593550752991,14.93874245386,73.2287174375679));
#157358=CARTESIAN_POINT('Ctrl Pts',(27.4045731969891,14.99268753181,73.7451354687612));
#157359=CARTESIAN_POINT('Ctrl Pts',(27.3853582494091,15.0053667451,74.11532093663));
#157360=CARTESIAN_POINT('Ctrl Pts',(27.4474386542391,15.00123185086,74.312087977728));
#157361=CARTESIAN_POINT('Ctrl Pts',(27.4728519056491,14.99893719101,74.370762926049));
#157362=CARTESIAN_POINT('',(28.295163666826,10.3190022129161,64.2104232034421));
#157363=CARTESIAN_POINT('Ctrl Pts',(26.0143837217827,12.1868716890914,64.6125868834549));
#157364=CARTESIAN_POINT('Ctrl Pts',(26.3866707717358,11.8943678422565,64.5469426319798));
#157365=CARTESIAN_POINT('Ctrl Pts',(26.7890747474804,11.5770393684394,64.4759879539895));
#157366=CARTESIAN_POINT('Ctrl Pts',(27.546069310181,10.9630297660278,64.3425093883358));
#157367=CARTESIAN_POINT('Ctrl Pts',(27.9293174909002,10.6434402054098,64.2749323936898));
#157368=CARTESIAN_POINT('Ctrl Pts',(28.2951915629989,10.3190345262137,64.2104189232372));
#157369=CARTESIAN_POINT('Origin',(33.823252652802,17.58608062208,59.024939776261));
#157370=CARTESIAN_POINT('Ctrl Pts',(26.0076877261891,10.58495646334,60.26985796972));
#157371=CARTESIAN_POINT('Ctrl Pts',(25.7990037333791,10.89447975427,60.24482455385));
#157372=CARTESIAN_POINT('Ctrl Pts',(25.5896565743691,11.1831771459,60.22557462704));
#157373=CARTESIAN_POINT('Ctrl Pts',(25.3807021623791,11.45236674632,60.21090371374));
#157374=CARTESIAN_POINT('Ctrl Pts',(27.9987970739791,9.17295597816802,64.622590824873));
#157375=CARTESIAN_POINT('Ctrl Pts',(27.7660735618591,9.33426324017502,64.560255312909));
#157376=CARTESIAN_POINT('Ctrl Pts',(27.5333174178191,9.48524635017302,64.499674997551));
#157377=CARTESIAN_POINT('Ctrl Pts',(27.3000253208991,9.63004663000602,64.442635376589));
#157378=CARTESIAN_POINT('Ctrl Pts',(32.0801713998191,9.69904765178202,67.445984142724));
#157379=CARTESIAN_POINT('Ctrl Pts',(31.8033473372391,9.81925633458402,67.454791081483));
#157380=CARTESIAN_POINT('Ctrl Pts',(31.5208971300691,9.93468827936802,67.469340771313));
#157381=CARTESIAN_POINT('Ctrl Pts',(31.2300886277791,10.04875492352,67.490838049821));
#157382=CARTESIAN_POINT('Ctrl Pts',(36.5371673514891,11.94221289613,67.553890268911));
#157383=CARTESIAN_POINT('Ctrl Pts',(36.2147089752091,12.14570654659,67.712396250694));
#157384=CARTESIAN_POINT('Ctrl Pts',(35.8771568089191,12.34268599228,67.886973156649));
#157385=CARTESIAN_POINT('Ctrl Pts',(35.5198166400391,12.53258632276,68.07491847425));
#157386=CARTESIAN_POINT('Ctrl Pts',(28.2951363354843,10.3189703124041,64.210428661338));
#157387=CARTESIAN_POINT('Ctrl Pts',(28.3673395453708,10.2549306784213,64.1976972873413));
#157388=CARTESIAN_POINT('Ctrl Pts',(28.4381421072126,10.1894797611389,64.1852128853848));
#157389=CARTESIAN_POINT('Ctrl Pts',(28.577126093425,10.0553246236656,64.1607062587292));
#157390=CARTESIAN_POINT('Ctrl Pts',(28.6450926511801,9.98682648706178,64.1487219208116));
#157391=CARTESIAN_POINT('Ctrl Pts',(28.7116430428839,9.91672751628407,64.1369872911775));
#157392=CARTESIAN_POINT('Ctrl Pts',(36.2322199092691,1.29987451700601,99.1648548727501));
#157393=CARTESIAN_POINT('Ctrl Pts',(36.2370515565391,1.23373127101501,99.16704017222));
#157394=CARTESIAN_POINT('Ctrl Pts',(36.2583081778491,0.918934546249416,
99.17660179767));
#157395=CARTESIAN_POINT('Ctrl Pts',(36.2789671085291,0.416646817226614,
99.1856530378401));
#157396=CARTESIAN_POINT('Ctrl Pts',(36.2808220405991,-0.0191504896747858,
99.18645022329));
#157397=CARTESIAN_POINT('Ctrl Pts',(36.2786095746291,-0.207586528585886,
99.18548739257));
#157398=CARTESIAN_POINT('Ctrl Pts',(34.9169995834991,0.648872675590514,
92.8720190887701));
#157399=CARTESIAN_POINT('Ctrl Pts',(34.9212091234391,0.615492124139614,
92.87094475832));
#157400=CARTESIAN_POINT('Ctrl Pts',(34.9397227668891,0.457009215198214,
92.86613805011));
#157401=CARTESIAN_POINT('Ctrl Pts',(34.9576892444091,0.206679526451214,
92.86110273846));
#157402=CARTESIAN_POINT('Ctrl Pts',(34.9593035548391,-0.00948024598489779,
92.86063999751));
#157403=CARTESIAN_POINT('Ctrl Pts',(34.9573789807491,-0.103058298997286,
92.86118379398));
#157404=CARTESIAN_POINT('Ctrl Pts',(38.6114884146191,0.506179248681214,
87.57260696818));
#157405=CARTESIAN_POINT('Ctrl Pts',(38.6168724865691,0.480286838357915,
87.57214900918));
#157406=CARTESIAN_POINT('Ctrl Pts',(38.6405854995891,0.357200917525514,
87.57008859617));
#157407=CARTESIAN_POINT('Ctrl Pts',(38.6637464841091,0.161757611975314,
87.56787911336));
#157408=CARTESIAN_POINT('Ctrl Pts',(38.6658219179391,-0.00742765239893279,
87.56767441493));
#157409=CARTESIAN_POINT('Ctrl Pts',(38.6633431586391,-0.0806241679503258,
87.56791373377));
#157410=CARTESIAN_POINT('Ctrl Pts',(44.9848109864291,0.961820384965713,
86.61004976678));
#157411=CARTESIAN_POINT('Ctrl Pts',(44.9924252103591,0.913417248693113,
86.61369530813));
#157412=CARTESIAN_POINT('Ctrl Pts',(45.0259996265791,0.682479313720714,
86.62976316487));
#157413=CARTESIAN_POINT('Ctrl Pts',(45.0589648322991,0.310222582160714,
86.6455090589899));
#157414=CARTESIAN_POINT('Ctrl Pts',(45.0619122089991,-0.0142877026623558,
86.6469175713899));
#157415=CARTESIAN_POINT('Ctrl Pts',(45.0583868262091,-0.154437964819286,
86.64523340457));
#157416=CARTESIAN_POINT('Origin',(36.6704247457035,0.356346398719197,81.8746090081706));
#157417=CARTESIAN_POINT('Ctrl Pts',(39.6130209037191,0.772780366718814,
89.0475659539699));
#157418=CARTESIAN_POINT('Ctrl Pts',(39.6131511234091,0.768070971044614,
89.0483044665601));
#157419=CARTESIAN_POINT('Ctrl Pts',(39.6159992090891,0.664122906098314,
89.0644567630999));
#157420=CARTESIAN_POINT('Ctrl Pts',(39.6205603414591,0.455619638640514,
89.0903242302099));
#157421=CARTESIAN_POINT('Ctrl Pts',(39.6239814776291,0.140849503561414,
89.10972645757));
#157422=CARTESIAN_POINT('Ctrl Pts',(39.6237889996191,-0.142041377329986,
89.10863486051));
#157423=CARTESIAN_POINT('Ctrl Pts',(39.6219727743591,-0.319354852029586,
89.09833453524));
#157424=CARTESIAN_POINT('Ctrl Pts',(39.6210240375191,-0.387361342889386,
89.0929539812099));
#157425=CARTESIAN_POINT('Ctrl Pts',(38.5565416256591,0.971382837408014,
90.50038750645));
#157426=CARTESIAN_POINT('Ctrl Pts',(38.5567042884291,0.965500141328614,
90.50131001286));
#157427=CARTESIAN_POINT('Ctrl Pts',(38.5602625557091,0.835631771075914,
90.5214899494));
#157428=CARTESIAN_POINT('Ctrl Pts',(38.5659866718191,0.574159320760314,
90.55395302502));
#157429=CARTESIAN_POINT('Ctrl Pts',(38.5702990716391,0.177643147708914,
90.57840985973));
#157430=CARTESIAN_POINT('Ctrl Pts',(38.5700563612191,-0.179118474077086,
90.57703338056));
#157431=CARTESIAN_POINT('Ctrl Pts',(38.5677671045191,-0.402543671104486,
90.56405036064));
#157432=CARTESIAN_POINT('Ctrl Pts',(38.5665713020191,-0.488170587549486,
90.55726862766));
#157433=CARTESIAN_POINT('Ctrl Pts',(36.8455425264091,0.835335570085914,
89.93447664681));
#157434=CARTESIAN_POINT('Ctrl Pts',(36.8456829649291,0.830256611811614,
89.93527311321));
#157435=CARTESIAN_POINT('Ctrl Pts',(36.8487547414491,0.718144247780114,
89.95269402358));
#157436=CARTESIAN_POINT('Ctrl Pts',(36.8536821869091,0.492956907891814,
89.98063895543));
#157437=CARTESIAN_POINT('Ctrl Pts',(36.8573840505991,0.152438653909214,
90.00163326767));
#157438=CARTESIAN_POINT('Ctrl Pts',(36.8571757505391,-0.153719808717186,
90.0004519393099));
#157439=CARTESIAN_POINT('Ctrl Pts',(36.8552105312691,-0.345557413745186,
89.9893066270201));
#157440=CARTESIAN_POINT('Ctrl Pts',(36.8541839744391,-0.419113932769686,
89.9834847339001));
#157441=CARTESIAN_POINT('Ctrl Pts',(36.8978805960391,0.556890469747314,
88.14953661764));
#157442=CARTESIAN_POINT('Ctrl Pts',(36.8979755486391,0.553456504850614,
88.15007512059));
#157443=CARTESIAN_POINT('Ctrl Pts',(36.9000516346991,0.477684987873014,
88.16184918971));
#157444=CARTESIAN_POINT('Ctrl Pts',(36.9033485509791,0.326761625590414,
88.18054693109));
#157445=CARTESIAN_POINT('Ctrl Pts',(36.9058008431191,0.100853142908714,
88.19445457091));
#157446=CARTESIAN_POINT('Ctrl Pts',(36.9056629700091,-0.101736890840086,
88.19367265364));
#157447=CARTESIAN_POINT('Ctrl Pts',(36.9043609513991,-0.228924831109186,
88.18628853918));
#157448=CARTESIAN_POINT('Ctrl Pts',(36.9036807861291,-0.277777119853686,
88.18243113024));
#157449=CARTESIAN_POINT('Ctrl Pts',(36.9231015705691,0.454612543733214,
88.46713451361));
#157450=CARTESIAN_POINT('Ctrl Pts',(36.9246228019291,0.381730267779614,
88.47576184538));
#157451=CARTESIAN_POINT('Ctrl Pts',(36.9270069740053,0.233138977846363,
88.4892831592894));
#157452=CARTESIAN_POINT('Ctrl Pts',(36.9278603928332,0.0786786354693159,
88.4941231372269));
#157453=CARTESIAN_POINT('Ctrl Pts',(36.9278603430304,-1.00177093760852E-6,
88.4941228548076));
#157454=CARTESIAN_POINT('Origin',(35.1195182435891,111.0724296188,78.238505182562));
#157455=CARTESIAN_POINT('Origin',(34.1682376097291,0.499074165591614,72.8435246184046));
#157456=CARTESIAN_POINT('Ctrl Pts',(36.9162947564091,-13.53296430165,79.1141410123499));
#157457=CARTESIAN_POINT('Ctrl Pts',(36.8379078596091,-13.54084808517,79.125313649548));
#157458=CARTESIAN_POINT('Ctrl Pts',(36.6331365458791,-13.54075199426,79.161549961231));
#157459=CARTESIAN_POINT('Ctrl Pts',(36.3090821190191,-13.45062514319,79.248712848581));
#157460=CARTESIAN_POINT('Ctrl Pts',(35.9700390021391,-13.22015785476,79.385367769725));
#157461=CARTESIAN_POINT('Ctrl Pts',(35.6829255508391,-12.85709379684,79.5572152706409));
#157462=CARTESIAN_POINT('Ctrl Pts',(35.4759945703691,-12.36078514696,79.76035426938));
#157463=CARTESIAN_POINT('Ctrl Pts',(35.4015806341291,-11.87740516072,79.937203183361));
#157464=CARTESIAN_POINT('Ctrl Pts',(35.4009999658791,-11.56819412752,80.042537145577));
#157465=CARTESIAN_POINT('Ctrl Pts',(35.4046387170491,-11.47622675764,80.073192707259));
#157466=CARTESIAN_POINT('Ctrl Pts',(36.7378435778691,-13.79049802242,77.964715139805));
#157467=CARTESIAN_POINT('Ctrl Pts',(36.6439251111591,-13.80190892298,77.9791527381109));
#157468=CARTESIAN_POINT('Ctrl Pts',(36.3962932068891,-13.80182730288,78.022615822591));
#157469=CARTESIAN_POINT('Ctrl Pts',(36.0104672867091,-13.67100041842,78.115500673479));
#157470=CARTESIAN_POINT('Ctrl Pts',(35.6462725616391,-13.35339373284,78.24515779335));
#157471=CARTESIAN_POINT('Ctrl Pts',(35.4018733334191,-12.89430356954,78.398017084265));
#157472=CARTESIAN_POINT('Ctrl Pts',(35.3103253268891,-12.33293611612,78.577596495555));
#157473=CARTESIAN_POINT('Ctrl Pts',(35.3702242253491,-11.85283482995,78.7438470995349));
#157474=CARTESIAN_POINT('Ctrl Pts',(35.4537140494691,-11.57449314574,78.85189623076));
#157475=CARTESIAN_POINT('Ctrl Pts',(35.4818326284191,-11.49406040224,78.884310074634));
#157476=CARTESIAN_POINT('Ctrl Pts',(36.7652353229291,-14.89891646854,77.528723139282));
#157477=CARTESIAN_POINT('Ctrl Pts',(36.6037070282991,-14.91744611088,77.55712837637));
#157478=CARTESIAN_POINT('Ctrl Pts',(36.1758646851091,-14.91734661094,77.632099353845));
#157479=CARTESIAN_POINT('Ctrl Pts',(35.5036841639991,-14.70473669194,77.752723593715));
#157480=CARTESIAN_POINT('Ctrl Pts',(34.8653075109791,-14.19454494754,77.8734639595339));
#157481=CARTESIAN_POINT('Ctrl Pts',(34.4335323097691,-13.47313071354,77.972684115116));
#157482=CARTESIAN_POINT('Ctrl Pts',(34.2645298594791,-12.62142137233,78.053662285297));
#157483=CARTESIAN_POINT('Ctrl Pts',(34.3553511232591,-11.93074611859,78.113117408706));
#157484=CARTESIAN_POINT('Ctrl Pts',(34.4887982535091,-11.55088371147,78.152250356099));
#157485=CARTESIAN_POINT('Ctrl Pts',(34.5338861201291,-11.44301453344,78.164268167064));
#157486=CARTESIAN_POINT('Ctrl Pts',(36.9738597083291,-15.86235421184,78.197884728009));
#157487=CARTESIAN_POINT('Ctrl Pts',(36.7533877970291,-15.88519834299,78.23841096985));
#157488=CARTESIAN_POINT('Ctrl Pts',(36.1698963531991,-15.88506467682,78.340862498621));
#157489=CARTESIAN_POINT('Ctrl Pts',(35.2440551909491,-15.62306719678,78.486320926825));
#157490=CARTESIAN_POINT('Ctrl Pts',(34.3288067440591,-14.98787397254,78.6042368987989));
#157491=CARTESIAN_POINT('Ctrl Pts',(33.6479144789791,-14.07352439099,78.663359407567));
#157492=CARTESIAN_POINT('Ctrl Pts',(33.2782095926791,-12.96704954774,78.6592835796531));
#157493=CARTESIAN_POINT('Ctrl Pts',(33.2687803614491,-12.0411391461,78.61169711387));
#157494=CARTESIAN_POINT('Ctrl Pts',(33.3731871600291,-11.51857786737,78.5722006974239));
#157495=CARTESIAN_POINT('Ctrl Pts',(33.4124876124591,-11.3689516287,78.559993102657));
#157496=CARTESIAN_POINT('Ctrl Pts',(36.6289738731116,-13.6294450659104,
78.8700122234104));
#157497=CARTESIAN_POINT('Ctrl Pts',(36.6267895588953,-13.6292110353221,
78.8704722093663));
#157498=CARTESIAN_POINT('Ctrl Pts',(36.624607035549,-13.6289708105016,78.8709335732414));
#157499=CARTESIAN_POINT('Ctrl Pts',(36.6224263107416,-13.6287244011036,
78.8713963118592));
#157500=CARTESIAN_POINT('Ctrl Pts',(36.583935576154,-13.6243751688195,78.8795638482938));
#157501=CARTESIAN_POINT('Ctrl Pts',(36.5460052001296,-13.6181035969037,
78.8881584920323));
#157502=CARTESIAN_POINT('Ctrl Pts',(36.5086374234726,-13.6100119136855,
78.89716440318));
#157503=CARTESIAN_POINT('Ctrl Pts',(36.4706975949425,-13.6017963573617,
78.9063081830693));
#157504=CARTESIAN_POINT('Ctrl Pts',(36.4333371557682,-13.5917043217201,
78.9158760369807));
#157505=CARTESIAN_POINT('Ctrl Pts',(36.3965629433869,-13.5797903680907,
78.9258649069554));
#157506=CARTESIAN_POINT('Ctrl Pts',(36.3593905003606,-13.567747397383,78.9359619471362));
#157507=CARTESIAN_POINT('Ctrl Pts',(36.3228164476515,-13.553842624327,78.9464892932658));
#157508=CARTESIAN_POINT('Ctrl Pts',(36.2868612731161,-13.5380825288037,
78.9574556553683));
#157509=CARTESIAN_POINT('Ctrl Pts',(36.2701595863516,-13.5307617416788,
78.9625496855643));
#157510=CARTESIAN_POINT('Ctrl Pts',(36.2535916812617,-13.5230399464007,
78.9677385985922));
#157511=CARTESIAN_POINT('Ctrl Pts',(36.2371611452247,-13.5149143727149,
78.9730240141749));
#157512=CARTESIAN_POINT('Ctrl Pts',(36.2232866202606,-13.5080528512955,
78.9774872057764));
#157513=CARTESIAN_POINT('Ctrl Pts',(36.2095100668752,-13.5009033643706,
78.9820192194605));
#157514=CARTESIAN_POINT('Ctrl Pts',(36.1958317439024,-13.4934659169776,
78.9866212604943));
#157515=CARTESIAN_POINT('Ctrl Pts',(36.1444157381463,-13.4655089928185,
79.0039200601175));
#157516=CARTESIAN_POINT('Ctrl Pts',(36.0943775497546,-13.433536582339,79.0221032244092));
#157517=CARTESIAN_POINT('Ctrl Pts',(36.0460456675535,-13.397702919938,79.0410869201147));
#157518=CARTESIAN_POINT('Ctrl Pts',(36.0159227434528,-13.3753695316321,
79.0529185393036));
#157519=CARTESIAN_POINT('Ctrl Pts',(35.9864634576983,-13.3515359442591,
79.0650610559982));
#157520=CARTESIAN_POINT('Ctrl Pts',(35.9577574687535,-13.3262373968706,
79.0774930494177));
#157521=CARTESIAN_POINT('Ctrl Pts',(35.9352874114504,-13.3064345672032,
79.0872243847522));
#157522=CARTESIAN_POINT('Ctrl Pts',(35.9133671055204,-13.2858181861862,
79.0970883044359));
#157523=CARTESIAN_POINT('Ctrl Pts',(35.8919558472264,-13.2643391294296,
79.1071099047377));
#157524=CARTESIAN_POINT('Ctrl Pts',(35.8670407349144,-13.2393451237483,
79.1187714938716));
#157525=CARTESIAN_POINT('Ctrl Pts',(35.8428139346251,-13.2131835002351,
79.1306465255989));
#157526=CARTESIAN_POINT('Ctrl Pts',(35.8192096787325,-13.1857454858265,
79.1427855534418));
#157527=CARTESIAN_POINT('Ctrl Pts',(35.79560542284,-13.158307471418,79.1549245812846));
#157528=CARTESIAN_POINT('Ctrl Pts',(35.7726233866794,-13.1295926154809,
79.1673277169806));
#157529=CARTESIAN_POINT('Ctrl Pts',(35.7502396011647,-13.0994575617588,
79.1800509756508));
#157530=CARTESIAN_POINT('Ctrl Pts',(35.7151504146276,-13.0522173610044,
79.1999961630518));
#157531=CARTESIAN_POINT('Ctrl Pts',(35.6819319380871,-13.0018483734156,
79.2207485864702));
#157532=CARTESIAN_POINT('Ctrl Pts',(35.6508857720451,-12.9485063268026,
79.2422271853796));
#157533=CARTESIAN_POINT('Ctrl Pts',(35.6380117503611,-12.9263867947534,
79.2511337907147));
#157534=CARTESIAN_POINT('Ctrl Pts',(35.6255115670388,-12.9037565275983,
79.2601651149864));
#157535=CARTESIAN_POINT('Ctrl Pts',(35.6134081179858,-12.8806288083371,
79.2693147004937));
#157536=CARTESIAN_POINT('Ctrl Pts',(35.5831213358917,-12.8227557020407,
79.2922099513679));
#157537=CARTESIAN_POINT('Ctrl Pts',(35.5553181247539,-12.7617645047354,
79.3158466479645));
#157538=CARTESIAN_POINT('Ctrl Pts',(35.5302240670213,-12.6978443630867,
79.3401370271472));
#157539=CARTESIAN_POINT('Ctrl Pts',(35.5062809457656,-12.6368559124151,
79.3633133304901));
#157540=CARTESIAN_POINT('Ctrl Pts',(35.4848039681179,-12.5732008806325,
79.3870847308051));
#157541=CARTESIAN_POINT('Ctrl Pts',(35.4660031304662,-12.5070876508559,
79.4113622174152));
#157542=CARTESIAN_POINT('Ctrl Pts',(35.4620975761915,-12.4933537517631,
79.4164054523691));
#157543=CARTESIAN_POINT('Ctrl Pts',(35.4583075612117,-12.4795139372748,
79.4214704807594));
#157544=CARTESIAN_POINT('Ctrl Pts',(35.4546350596877,-12.4655703406705,
79.4265564316822));
#157545=CARTESIAN_POINT('Ctrl Pts',(35.446244748698,-12.4337143670073,79.4381759530474));
#157546=CARTESIAN_POINT('Ctrl Pts',(35.438466298639,-12.4013151850429,79.4499020521234));
#157547=CARTESIAN_POINT('Ctrl Pts',(35.4313279849064,-12.368402830968,79.4617323991114));
#157548=CARTESIAN_POINT('Ctrl Pts',(35.4166655594567,-12.3007993385919,
79.4860324771486));
#157549=CARTESIAN_POINT('Ctrl Pts',(35.4047053295063,-12.2310279449783,
79.5107727246997));
#157550=CARTESIAN_POINT('Ctrl Pts',(35.3956126986768,-12.159289658879,79.5359445459002));
#157551=CARTESIAN_POINT('Ctrl Pts',(35.3864867829726,-12.0872887645299,
79.56120851215));
#157552=CARTESIAN_POINT('Ctrl Pts',(35.3802497959325,-12.0133066643763,
79.5869072534782));
#157553=CARTESIAN_POINT('Ctrl Pts',(35.3770484236597,-11.9375947461263,
79.6130256997429));
#157554=CARTESIAN_POINT('Ctrl Pts',(35.3744205448052,-11.8754458512009,
79.6344652908936));
#157555=CARTESIAN_POINT('Ctrl Pts',(35.3738377628765,-11.8121323365772,
79.6561875923856));
#157556=CARTESIAN_POINT('Ctrl Pts',(35.3753690601812,-11.7478162345504,
79.6781806669065));
#157557=CARTESIAN_POINT('Ctrl Pts',(35.3762341383981,-11.7114820369465,
79.6906052494042));
#157558=CARTESIAN_POINT('Ctrl Pts',(35.3777737267097,-11.674828239601,79.7031162043097));
#157559=CARTESIAN_POINT('Ctrl Pts',(35.3799958958808,-11.6378856606036,
79.7157076007637));
#157560=CARTESIAN_POINT('Ctrl Pts',(35.5596731802056,-13.409584407367,78.6873025602364));
#157561=CARTESIAN_POINT('Ctrl Pts',(35.5649489821513,-13.410762854301,78.6892006371155));
#157562=CARTESIAN_POINT('Ctrl Pts',(35.572454155639,-13.4127848705518,78.6916420133374));
#157563=CARTESIAN_POINT('Ctrl Pts',(35.5822091762942,-13.4155951123882,
78.6946608021742));
#157564=CARTESIAN_POINT('Ctrl Pts',(35.5888413201348,-13.4175057109143,
78.6967131855056));
#157565=CARTESIAN_POINT('Ctrl Pts',(35.5965133072729,-13.4197796194329,
78.6990327697528));
#157566=CARTESIAN_POINT('Ctrl Pts',(35.6052297520272,-13.4223863862809,
78.7016342587272));
#157567=CARTESIAN_POINT('Ctrl Pts',(35.6159986738011,-13.4256069732357,
78.7048483250181));
#157568=CARTESIAN_POINT('Ctrl Pts',(35.628364387104,-13.4293376813513,78.7084926497722));
#157569=CARTESIAN_POINT('Ctrl Pts',(35.6423428025468,-13.4335034999063,
78.7126042044134));
#157570=CARTESIAN_POINT('Ctrl Pts',(35.6493320102682,-13.4355864091838,
78.7146599817339));
#157571=CARTESIAN_POINT('Ctrl Pts',(35.6567245312736,-13.4377776618008,
78.7168328489925));
#157572=CARTESIAN_POINT('Ctrl Pts',(35.66452171591,-13.440065921592,78.7191278210619));
#157573=CARTESIAN_POINT('Ctrl Pts',(35.6682193836418,-13.4411510856335,
78.7202161682747));
#157574=CARTESIAN_POINT('Ctrl Pts',(35.6720080603159,-13.4422580615983,
78.721331972209));
#157575=CARTESIAN_POINT('Ctrl Pts',(35.6758878046835,-13.4433855189776,
78.7224757778056));
#157576=CARTESIAN_POINT('Ctrl Pts',(35.6760986229854,-13.4434467829754,
78.7225379301359));
#157577=CARTESIAN_POINT('Ctrl Pts',(35.6763097101715,-13.4435081074283,
78.7226001651511));
#157578=CARTESIAN_POINT('Ctrl Pts',(35.6765210662432,-13.4435694921167,
78.7226624829415));
#157579=CARTESIAN_POINT('Ctrl Pts',(35.6797960285612,-13.4445206478591,
78.7236280971005));
#157580=CARTESIAN_POINT('Ctrl Pts',(35.6842564285498,-13.4458099995922,
78.7249439247759));
#157581=CARTESIAN_POINT('Ctrl Pts',(35.6872168365588,-13.4466605313594,
78.7258191404787));
#157582=CARTESIAN_POINT('Ctrl Pts',(35.6879635322211,-13.4468750586744,
78.7260398937556));
#157583=CARTESIAN_POINT('Ctrl Pts',(35.6886148676402,-13.4470619434621,
78.726232514826));
#157584=CARTESIAN_POINT('Ctrl Pts',(35.6891278548595,-13.4472091357767,
78.7263841598653));
#157585=CARTESIAN_POINT('Ctrl Pts',(35.729876918238,-13.4589013353743,78.7384300609778));
#157586=CARTESIAN_POINT('Ctrl Pts',(35.7706602076644,-13.4704088812035,
78.7501898760101));
#157587=CARTESIAN_POINT('Ctrl Pts',(35.8114521558143,-13.4815662061391,
78.7615388724631));
#157588=CARTESIAN_POINT('Ctrl Pts',(35.8318481298892,-13.487144868607,78.7672133706896));
#157589=CARTESIAN_POINT('Ctrl Pts',(35.8520872866738,-13.4925860047892,
78.7727477992517));
#157590=CARTESIAN_POINT('Ctrl Pts',(35.8721725455393,-13.4978862209229,
78.7781234405706));
#157591=CARTESIAN_POINT('Ctrl Pts',(35.8822151749721,-13.5005363289897,
78.7808112612301));
#157592=CARTESIAN_POINT('Ctrl Pts',(35.8922193317316,-13.5031512070723,
78.7834593823422));
#157593=CARTESIAN_POINT('Ctrl Pts',(35.9021856584897,-13.505729861492,78.7860663134503));
#157594=CARTESIAN_POINT('Ctrl Pts',(35.9071688218687,-13.5070191887018,
78.7873697790044));
#157595=CARTESIAN_POINT('Ctrl Pts',(35.9121425274005,-13.5082994605119,
78.7886629476841));
#157596=CARTESIAN_POINT('Ctrl Pts',(35.9171068798581,-13.5095705193357,
78.7899456958789));
#157597=CARTESIAN_POINT('Ctrl Pts',(35.9208245999257,-13.5105223939128,
78.7909063244293));
#157598=CARTESIAN_POINT('Ctrl Pts',(35.9237075813183,-13.511255961388,78.7916505395541));
#157599=CARTESIAN_POINT('Ctrl Pts',(35.9276195592542,-13.5122511243835,
78.792650917631));
#157600=CARTESIAN_POINT('Ctrl Pts',(35.9289313305321,-13.5125848241782,
78.792986366156));
#157601=CARTESIAN_POINT('Ctrl Pts',(35.930358746238,-13.5129475867588,78.7933507170801));
#157602=CARTESIAN_POINT('Ctrl Pts',(35.931971861629,-13.5133561840459,78.793762161952));
#157603=CARTESIAN_POINT('Ctrl Pts',(35.9432221584124,-13.5162058504559,
78.7966316881774));
#157604=CARTESIAN_POINT('Ctrl Pts',(35.9536968873557,-13.5188035375634,
78.7992871885907));
#157605=CARTESIAN_POINT('Ctrl Pts',(35.9640624555409,-13.521342645619,78.8018798382663));
#157606=CARTESIAN_POINT('Ctrl Pts',(35.9744563967455,-13.5238887038157,
78.8044795846393));
#157607=CARTESIAN_POINT('Ctrl Pts',(35.9847405951858,-13.5263757301332,
78.8070161663376));
#157608=CARTESIAN_POINT('Ctrl Pts',(35.9955799080153,-13.5289503325776,
78.8096553848795));
#157609=CARTESIAN_POINT('Ctrl Pts',(35.9986196867187,-13.5296723545179,
78.8103955277689));
#157610=CARTESIAN_POINT('Ctrl Pts',(36.0017030790087,-13.5304009701641,
78.8111438242411));
#157611=CARTESIAN_POINT('Ctrl Pts',(36.0048446387178,-13.5311386965311,
78.8119041305644));
#157612=CARTESIAN_POINT('Ctrl Pts',(36.0157346109575,-13.5336959675688,
78.8145396732634));
#157613=CARTESIAN_POINT('Ctrl Pts',(36.0243877408748,-13.5356865589943,
78.8165955497169));
#157614=CARTESIAN_POINT('Ctrl Pts',(36.0308156514772,-13.5372019178371,
78.8180503777498));
#157615=CARTESIAN_POINT('Ctrl Pts',(36.0372606024798,-13.5387212938984,
78.8195090625338));
#157616=CARTESIAN_POINT('Ctrl Pts',(36.0414686433905,-13.539762858444,78.8203634758004));
#157617=CARTESIAN_POINT('Ctrl Pts',(36.0434419127291,-13.5403694672138,
78.8206064982397));
#157618=CARTESIAN_POINT('Ctrl Pts',(36.0441117127454,-13.5405753724879,
78.8206889889726));
#157619=CARTESIAN_POINT('Ctrl Pts',(36.0445239400253,-13.5407307481149,
78.8207011613338));
#157620=CARTESIAN_POINT('Ctrl Pts',(36.0446784011166,-13.5408359897401,
78.8206431222969));
#157621=CARTESIAN_POINT('Ctrl Pts',(33.8015018549743,-13.7317040852684,
78.231178210434));
#157622=CARTESIAN_POINT('Ctrl Pts',(33.8448367011614,-13.7318398987138,
78.2231897821826));
#157623=CARTESIAN_POINT('Ctrl Pts',(33.9729484993377,-13.7306782863685,
78.2035675708194));
#157624=CARTESIAN_POINT('Ctrl Pts',(34.1794028973399,-13.7215222815351,
78.1905757013909));
#157625=CARTESIAN_POINT('Ctrl Pts',(34.410851781839,-13.7010503656952,78.2017087925164));
#157626=CARTESIAN_POINT('Ctrl Pts',(34.6169343870141,-13.67434261052,78.2323749945655));
#157627=CARTESIAN_POINT('Ctrl Pts',(34.7988676057059,-13.6435683591641,
78.2764569312182));
#157628=CARTESIAN_POINT('Ctrl Pts',(34.9584049522099,-13.6103796896382,
78.3292431282214));
#157629=CARTESIAN_POINT('Ctrl Pts',(35.0975727630671,-13.576019734666,78.3871814162859));
#157630=CARTESIAN_POINT('Ctrl Pts',(35.2184605265174,-13.5414149887607,
78.4476361863756));
#157631=CARTESIAN_POINT('Ctrl Pts',(35.3230564896596,-13.5072433877898,
78.5086867494384));
#157632=CARTESIAN_POINT('Ctrl Pts',(35.4130828699557,-13.4740390254729,
78.5688811234007));
#157633=CARTESIAN_POINT('Ctrl Pts',(35.4899484910174,-13.4422810794632,
78.6270120644502));
#157634=CARTESIAN_POINT('Ctrl Pts',(35.5548824783634,-13.412407270912,78.6820491833158));
#157635=CARTESIAN_POINT('Ctrl Pts',(35.609139363501,-13.3847427053007,78.7332420479501));
#157636=CARTESIAN_POINT('Ctrl Pts',(35.6540406849326,-13.3594694892852,
78.7801592442625));
#157637=CARTESIAN_POINT('Ctrl Pts',(35.6906205410342,-13.3367332240462,
78.8224176266727));
#157638=CARTESIAN_POINT('Ctrl Pts',(35.7198794129803,-13.3166160756286,
78.8598141138234));
#157639=CARTESIAN_POINT('Ctrl Pts',(35.7400793850874,-13.3011802483082,
78.8884757827741));
#157640=CARTESIAN_POINT('Ctrl Pts',(35.7502020927212,-13.2927142033317,
78.9041630984296));
#157641=CARTESIAN_POINT('Ctrl Pts',(35.7536670291067,-13.2897107768893,
78.9097209772309));
#157642=CARTESIAN_POINT('Ctrl Pts',(33.7642812125629,-14.0482563699744,
78.0322674443946));
#157643=CARTESIAN_POINT('Ctrl Pts',(33.8130408089844,-14.0483970404398,
78.0232716765594));
#157644=CARTESIAN_POINT('Ctrl Pts',(33.9571859795452,-14.0471930263636,
78.0012572053819));
#157645=CARTESIAN_POINT('Ctrl Pts',(34.1894920675434,-14.0377087515782,
77.9871247460472));
#157646=CARTESIAN_POINT('Ctrl Pts',(34.4501081986777,-14.0164476769987,
78.0007115608826));
#157647=CARTESIAN_POINT('Ctrl Pts',(34.6825015229247,-13.9885972267012,
78.0366152126997));
#157648=CARTESIAN_POINT('Ctrl Pts',(34.8881313202119,-13.9563387079234,
78.0879027470612));
#157649=CARTESIAN_POINT('Ctrl Pts',(35.0690171621493,-13.9213354830119,
78.1492629281395));
#157650=CARTESIAN_POINT('Ctrl Pts',(35.2274467707762,-13.8848455486338,
78.2167089525784));
#157651=CARTESIAN_POINT('Ctrl Pts',(35.3657608913579,-13.8478127238908,
78.2872967474258));
#157652=CARTESIAN_POINT('Ctrl Pts',(35.4862143351102,-13.8109237809282,
78.3589158860956));
#157653=CARTESIAN_POINT('Ctrl Pts',(35.590733009388,-13.7747236149353,78.4299822582505));
#157654=CARTESIAN_POINT('Ctrl Pts',(35.6808630807593,-13.7397101095713,
78.4991751650237));
#157655=CARTESIAN_POINT('Ctrl Pts',(35.7579171333831,-13.7063530796802,
78.5653476617595));
#157656=CARTESIAN_POINT('Ctrl Pts',(35.8232187425314,-13.6750153646781,
78.6276488136447));
#157657=CARTESIAN_POINT('Ctrl Pts',(35.8781479447624,-13.6459257565499,
78.6855511294384));
#157658=CARTESIAN_POINT('Ctrl Pts',(35.9239726936212,-13.6191899326575,
78.7387922454918));
#157659=CARTESIAN_POINT('Ctrl Pts',(35.9617901538152,-13.5948848845966,
78.7872092453676));
#157660=CARTESIAN_POINT('Ctrl Pts',(35.9890440080014,-13.5755567654701,
78.825728205213));
#157661=CARTESIAN_POINT('Ctrl Pts',(36.0033566791772,-13.5645406906742,
78.847695086863));
#157662=CARTESIAN_POINT('Ctrl Pts',(36.0083664878408,-13.5605601040526,
78.855634972008));
#157663=CARTESIAN_POINT('Ctrl Pts',(33.7098713669441,-14.2651297534302,
77.738616182356));
#157664=CARTESIAN_POINT('Ctrl Pts',(33.7652791838108,-14.2652746724941,
77.7283917307582));
#157665=CARTESIAN_POINT('Ctrl Pts',(33.9290623283902,-14.2640332999716,
77.7033975118487));
#157666=CARTESIAN_POINT('Ctrl Pts',(34.1929785744821,-14.2542616178001,
77.6874861366232));
#157667=CARTESIAN_POINT('Ctrl Pts',(34.4891855565944,-14.2322924438966,
77.7032331310642));
#157668=CARTESIAN_POINT('Ctrl Pts',(34.7536256962505,-14.2033839164636,
77.7444596746802));
#157669=CARTESIAN_POINT('Ctrl Pts',(34.9880716473297,-14.1697073341032,
77.8033262526759));
#157670=CARTESIAN_POINT('Ctrl Pts',(35.1948810444306,-14.1329210158518,
77.8738550465823));
#157671=CARTESIAN_POINT('Ctrl Pts',(35.376670559523,-14.0942867264955,77.9515757927416));
#157672=CARTESIAN_POINT('Ctrl Pts',(35.5360948856724,-14.05475850672,78.0332008651507));
#157673=CARTESIAN_POINT('Ctrl Pts',(35.6757394068685,-14.0150260502892,
78.1164096768387));
#157674=CARTESIAN_POINT('Ctrl Pts',(35.7977824483,-13.9756411113113,78.1994722424931));
#157675=CARTESIAN_POINT('Ctrl Pts',(35.903940888504,-13.9371184259179,78.2809425578672));
#157676=CARTESIAN_POINT('Ctrl Pts',(35.9956318025583,-13.8999610119654,
78.3595434745583));
#157677=CARTESIAN_POINT('Ctrl Pts',(36.0742649614256,-13.8645728621217,
78.4343099401369));
#157678=CARTESIAN_POINT('Ctrl Pts',(36.1412930269105,-13.8312361404342,
78.5046020922704));
#157679=CARTESIAN_POINT('Ctrl Pts',(36.1982698210819,-13.8000075196721,
78.5703016764263));
#157680=CARTESIAN_POINT('Ctrl Pts',(36.2464106531869,-13.7709569337502,
78.6312931394323));
#157681=CARTESIAN_POINT('Ctrl Pts',(36.2821732309277,-13.747181853896,78.6811264949467));
#157682=CARTESIAN_POINT('Ctrl Pts',(36.3015404153484,-13.7332339834193,
78.7103362616371));
#157683=CARTESIAN_POINT('Ctrl Pts',(36.3084139439587,-13.7281272594451,
78.7210288249536));
#157684=CARTESIAN_POINT('Ctrl Pts',(33.646793935444,-14.3652713150121,77.3964138987276));
#157685=CARTESIAN_POINT('Ctrl Pts',(33.709120380352,-14.3654194049986,77.3849150787496));
#157686=CARTESIAN_POINT('Ctrl Pts',(33.8933318204112,-14.3641498743635,
77.3567847235416));
#157687=CARTESIAN_POINT('Ctrl Pts',(34.1900910923022,-14.3541634210384,
77.3387423942183));
#157688=CARTESIAN_POINT('Ctrl Pts',(34.5232230536664,-14.3316474620846,
77.3561158445656));
#157689=CARTESIAN_POINT('Ctrl Pts',(34.8208682377197,-14.3018890672365,
77.4020775669144));
#157690=CARTESIAN_POINT('Ctrl Pts',(35.0851373959727,-14.2670310129054,
77.467912837115));
#157691=CARTESIAN_POINT('Ctrl Pts',(35.3187487836197,-14.228712518735,77.5470003753656));
#157692=CARTESIAN_POINT('Ctrl Pts',(35.5246677233139,-14.1881886671558,
77.6344029014632));
#157693=CARTESIAN_POINT('Ctrl Pts',(35.705880046119,-14.1464160555454,77.7265005683826));
#157694=CARTESIAN_POINT('Ctrl Pts',(35.8653180087285,-14.1040816146407,
77.8207704981658));
#157695=CARTESIAN_POINT('Ctrl Pts',(36.0054246676531,-14.0617395550477,
77.9153426786752));
#157696=CARTESIAN_POINT('Ctrl Pts',(36.1280963134294,-14.0199176941972,
78.0086507860051));
#157697=CARTESIAN_POINT('Ctrl Pts',(36.2348603836339,-13.9791491053273,
78.0992914480622));
#157698=CARTESIAN_POINT('Ctrl Pts',(36.3272175105147,-13.9398768718413,
78.186187496645));
#157699=CARTESIAN_POINT('Ctrl Pts',(36.4066966204188,-13.9024358806681,
78.2685860724393));
#157700=CARTESIAN_POINT('Ctrl Pts',(36.4751484961417,-13.8668317505958,
78.3465160194065));
#157701=CARTESIAN_POINT('Ctrl Pts',(36.5339111440086,-13.8331265451538,
78.4199097088141));
#157702=CARTESIAN_POINT('Ctrl Pts',(36.5784286736335,-13.8049608162598,
78.4809554358667));
#157703=CARTESIAN_POINT('Ctrl Pts',(36.6029969258144,-13.7881038093459,
78.5173702609838));
#157704=CARTESIAN_POINT('Ctrl Pts',(36.61178827325,-13.7818775502543,78.5308052276326));
#157705=CARTESIAN_POINT('Origin',(35.6454492392491,0.499074165591614,72.5830523519042));
#157706=CARTESIAN_POINT('Origin',(82.8534541851791,15.33010667085,62.64107301909));
#157707=CARTESIAN_POINT('Ctrl Pts',(65.6493476995291,-7.55647811801299,
66.484406505602));
#157708=CARTESIAN_POINT('Ctrl Pts',(65.6977795012391,-7.61087860031499,
66.475866672236));
#157709=CARTESIAN_POINT('Ctrl Pts',(65.8511840174591,-7.78393516119298,
66.448817317063));
#157710=CARTESIAN_POINT('Ctrl Pts',(66.1061821657891,-8.07036067158899,
66.403854263482));
#157711=CARTESIAN_POINT('Ctrl Pts',(66.4160097536291,-8.400411439295,66.349223300379));
#157712=CARTESIAN_POINT('Ctrl Pts',(66.7163050559491,-8.69402671421799,
66.296273136399));
#157713=CARTESIAN_POINT('Ctrl Pts',(67.0055863725391,-8.95024991713399,
66.245265035269));
#157714=CARTESIAN_POINT('Ctrl Pts',(67.2020307421891,-9.10615845958399,
66.210626592692));
#157715=CARTESIAN_POINT('Ctrl Pts',(67.2981630439992,-9.17825162599699,
66.193675874165));
#157716=CARTESIAN_POINT('Ctrl Pts',(67.2997288353791,-9.17942477180599,
66.193399782899));
#157717=CARTESIAN_POINT('Ctrl Pts',(65.2976696808791,-7.73950995723499,
65.656652656171));
#157718=CARTESIAN_POINT('Ctrl Pts',(65.3458411451991,-7.79361760798199,
65.648158727311));
#157719=CARTESIAN_POINT('Ctrl Pts',(65.4990058852991,-7.96639406115299,
65.621151651139));
#157720=CARTESIAN_POINT('Ctrl Pts',(65.7563586217791,-8.255493936528,65.575773420139));
#157721=CARTESIAN_POINT('Ctrl Pts',(66.072576141859,-8.592419041958,65.520015739575));
#157722=CARTESIAN_POINT('Ctrl Pts',(66.3821225145791,-8.89513157016199,
65.465434362284));
#157723=CARTESIAN_POINT('Ctrl Pts',(66.6817222931791,-9.16053014774899,
65.412606837902));
#157724=CARTESIAN_POINT('Ctrl Pts',(66.8863394401191,-9.32293981017799,
65.376527314182));
#157725=CARTESIAN_POINT('Ctrl Pts',(66.9862719124592,-9.39788123282599,
65.3589065230591));
#157726=CARTESIAN_POINT('Ctrl Pts',(66.9878995464891,-9.39910068191699,
65.358619527265));
#157727=CARTESIAN_POINT('Ctrl Pts',(65.6592224440491,-7.30445217689799,
64.933904240298));
#157728=CARTESIAN_POINT('Ctrl Pts',(65.7080127176891,-7.35925587400999,
64.9253011986599));
#157729=CARTESIAN_POINT('Ctrl Pts',(65.8617473939792,-7.53269812957599,
64.898193627359));
#157730=CARTESIAN_POINT('Ctrl Pts',(66.1135033889391,-7.81544116946099,
64.853802252892));
#157731=CARTESIAN_POINT('Ctrl Pts',(66.4145323508291,-8.13602630844498,
64.8007227249361));
#157732=CARTESIAN_POINT('Ctrl Pts',(66.7020893791291,-8.41711510803199,
64.750018662355));
#157733=CARTESIAN_POINT('Ctrl Pts',(66.9771626753591,-8.66070426625799,
64.7015158185569));
#157734=CARTESIAN_POINT('Ctrl Pts',(67.1623535281491,-8.80766108266999,
64.66886167463));
#157735=CARTESIAN_POINT('Ctrl Pts',(67.2532531799491,-8.87583233876699,
64.65283361348));
#157736=CARTESIAN_POINT('Ctrl Pts',(67.2547338170091,-8.87694172720999,
64.652572537217));
#157737=CARTESIAN_POINT('Ctrl Pts',(66.3469619223191,-6.71703633739999,
65.089867102845));
#157738=CARTESIAN_POINT('Ctrl Pts',(66.3965877134691,-6.77277983763399,
65.0811167369271));
#157739=CARTESIAN_POINT('Ctrl Pts',(66.5510919186892,-6.94712106085499,
65.0538734769131));
#157740=CARTESIAN_POINT('Ctrl Pts',(66.7952911826491,-7.22128108941499,
65.010814558009));
#157741=CARTESIAN_POINT('Ctrl Pts',(67.0758125244791,-7.51980397473499,
64.961351076778));
#157742=CARTESIAN_POINT('Ctrl Pts',(67.3336794982692,-7.77169637496499,
64.915882171866));
#157743=CARTESIAN_POINT('Ctrl Pts',(67.5756370915191,-7.98583841383899,
64.873218519988));
#157744=CARTESIAN_POINT('Ctrl Pts',(67.7345985251391,-8.11193076827299,
64.845189330349));
#157745=CARTESIAN_POINT('Ctrl Pts',(67.8133020455291,-8.17096093266299,
64.831311776228));
#157746=CARTESIAN_POINT('Ctrl Pts',(67.8145842070092,-8.17192171701199,
64.831085696565));
#157747=CARTESIAN_POINT('Origin',(82.0934733297391,-9.38083151964699,58.3310074104));
#157748=CARTESIAN_POINT('Ctrl Pts',(83.9305070695251,-8.35425122912034,
62.451223254077));
#157749=CARTESIAN_POINT('Ctrl Pts',(83.9721096129046,-8.41502174878494,
62.3585397890282));
#157750=CARTESIAN_POINT('Ctrl Pts',(84.009290601372,-8.48362968832864,62.2534751356656));
#157751=CARTESIAN_POINT('Ctrl Pts',(84.0547015692346,-8.59871915493393,
62.0779605492143));
#157752=CARTESIAN_POINT('Ctrl Pts',(84.0681049073854,-8.63910401461063,
62.0164686566902));
#157753=CARTESIAN_POINT('Ctrl Pts',(84.0850836244519,-8.70266714380778,
61.9198461905371));
#157754=CARTESIAN_POINT('Ctrl Pts',(84.0927908839831,-8.73519400778358,
61.8704388934484));
#157755=CARTESIAN_POINT('Ctrl Pts',(84.1002942620877,-8.77442340519883,
61.8109000502313));
#157756=CARTESIAN_POINT('Ctrl Pts',(84.103658570228,-8.7943545318876,61.7806590728184));
#157757=CARTESIAN_POINT('Ctrl Pts',(84.1050157653578,-8.80296380107318,
61.767597895611));
#157758=CARTESIAN_POINT('Ctrl Pts',(84.1059015676795,-8.80871822946449,
61.7588680856792));
#157759=CARTESIAN_POINT('Ctrl Pts',(84.1064768697166,-8.8125712101865,61.7530231017033));
#157760=CARTESIAN_POINT('Ctrl Pts',(84.1157801312426,-8.87605641934299,
61.6567176345016));
#157761=CARTESIAN_POINT('Ctrl Pts',(84.1223566595417,-8.95342740610009,
61.5385628860497));
#157762=CARTESIAN_POINT('Ctrl Pts',(84.1160489550679,-9.14217474627203,
61.2552874147842));
#157763=CARTESIAN_POINT('Ctrl Pts',(84.103128596185,-9.25373486147343,61.0901730619785));
#157764=CARTESIAN_POINT('Ctrl Pts',(84.0701935481991,-9.38083151964699,
60.90338912307));
#157765=CARTESIAN_POINT('Ctrl Pts',(84.007342440529,-8.34113792735099,62.7303651543501));
#157766=CARTESIAN_POINT('Ctrl Pts',(84.0935574097791,-8.41594609712799,
62.69053588541));
#157767=CARTESIAN_POINT('Ctrl Pts',(84.2989240749091,-8.61704513668698,
62.57230781918));
#157768=CARTESIAN_POINT('Ctrl Pts',(84.5872966976591,-8.99415052088398,
62.31565721301));
#157769=CARTESIAN_POINT('Ctrl Pts',(84.8429254664791,-9.48340020843898,
61.94261309465));
#157770=CARTESIAN_POINT('Ctrl Pts',(84.9636036434391,-9.88804177715397,
61.60883124012));
#157771=CARTESIAN_POINT('Ctrl Pts',(85.000589857989,-10.12788821405,61.40365053913));
#157772=CARTESIAN_POINT('Ctrl Pts',(85.0065710147491,-10.17521122351,61.36296841404));
#157773=CARTESIAN_POINT('Ctrl Pts',(83.6034848088291,-8.23953217489199,
62.25272764276));
#157774=CARTESIAN_POINT('Ctrl Pts',(83.6622877099991,-8.31654637346699,
62.23557356992));
#157775=CARTESIAN_POINT('Ctrl Pts',(83.8066016022891,-8.52254556916299,
62.17796180608));
#157776=CARTESIAN_POINT('Ctrl Pts',(84.0209884017891,-8.90514749704598,
62.03256168289));
#157777=CARTESIAN_POINT('Ctrl Pts',(84.2246311003191,-9.39808266510199,
61.80143661051));
#157778=CARTESIAN_POINT('Ctrl Pts',(84.3331361822591,-9.80365235625799,
61.58278472916));
#157779=CARTESIAN_POINT('Ctrl Pts',(84.3737914439991,-10.04335797538,61.44473164379));
#157780=CARTESIAN_POINT('Ctrl Pts',(84.3809019086191,-10.09062139715,61.41723307588));
#157781=CARTESIAN_POINT('Ctrl Pts',(83.5888040753991,-7.80219022690399,
61.79433169008));
#157782=CARTESIAN_POINT('Ctrl Pts',(83.6280925122191,-7.88869984191799,
61.7686511776601));
#157783=CARTESIAN_POINT('Ctrl Pts',(83.7184869065591,-8.115790794511,61.69745538176));
#157784=CARTESIAN_POINT('Ctrl Pts',(83.8365843313791,-8.52205151202899,
61.55819868633));
#157785=CARTESIAN_POINT('Ctrl Pts',(83.9310436648091,-9.03085010496399,
61.3706688459801));
#157786=CARTESIAN_POINT('Ctrl Pts',(83.9663332001091,-9.44041471634899,
61.21179100688));
#157787=CARTESIAN_POINT('Ctrl Pts',(83.9715830565591,-9.67951421307999,
61.11686765514));
#157788=CARTESIAN_POINT('Ctrl Pts',(83.9720288907591,-9.72652115139598,
61.09814164466));
#157789=CARTESIAN_POINT('Ctrl Pts',(83.9729708222391,-7.31720063036999,
61.65713466525));
#157790=CARTESIAN_POINT('Ctrl Pts',(84.0134970850191,-7.41424017101399,
61.59734266571));
#157791=CARTESIAN_POINT('Ctrl Pts',(84.092623435809,-7.66472079092699,61.44731065951));
#157792=CARTESIAN_POINT('Ctrl Pts',(84.155556256859,-8.09721788227599,61.2050435005));
#157793=CARTESIAN_POINT('Ctrl Pts',(84.1555568604491,-8.62360819278299,
60.93406776197));
#157794=CARTESIAN_POINT('Ctrl Pts',(84.1048173875391,-9.03760296404499,
60.74023331364));
#157795=CARTESIAN_POINT('Ctrl Pts',(84.0589098500391,-9.27603030239999,
60.63603113317));
#157796=CARTESIAN_POINT('Ctrl Pts',(84.049287281419,-9.32275281383199,60.61588796801));
#157797=CARTESIAN_POINT('Origin',(63.4339821949991,0.499074165591614,67.683184237498));
#157798=CARTESIAN_POINT('Origin',(91.5481551204691,-0.0433423696914658,
83.15731994474));
#157799=CARTESIAN_POINT('Ctrl Pts',(87.0625396169313,9.81028965175084,57.7179144389336));
#157800=CARTESIAN_POINT('Ctrl Pts',(86.9560129494815,9.81043336279731,57.7361359393653));
#157801=CARTESIAN_POINT('Ctrl Pts',(86.8423970449262,9.80410270209386,57.7731105945253));
#157802=CARTESIAN_POINT('Ctrl Pts',(86.6235573133266,9.77319335733451,57.8940860262539));
#157803=CARTESIAN_POINT('Ctrl Pts',(86.5188898025592,9.7484075770056,57.9785392281757));
#157804=CARTESIAN_POINT('Ctrl Pts',(86.3506421598397,9.68141743769284,58.1865038597519));
#157805=CARTESIAN_POINT('Ctrl Pts',(86.2879257990702,9.63930718845491,58.3096128797123));
#157806=CARTESIAN_POINT('Ctrl Pts',(86.222153236433,9.54815442195098,58.5637415305018));
#157807=CARTESIAN_POINT('Ctrl Pts',(86.2190078227482,9.49946000046106,58.6938516074194));
#157808=CARTESIAN_POINT('Ctrl Pts',(86.2399778829169,9.45364604184037,58.8119255183517));
#157809=CARTESIAN_POINT('Ctrl Pts',(87.3207027298691,3.13362000020301,55.34789324766));
#157810=CARTESIAN_POINT('Ctrl Pts',(87.325235904929,3.72414610022402,55.47809510729));
#157811=CARTESIAN_POINT('Ctrl Pts',(87.3354008992691,4.83285818851802,55.7901515622));
#157812=CARTESIAN_POINT('Ctrl Pts',(87.3490222678991,6.36326886928801,56.3467657865));
#157813=CARTESIAN_POINT('Ctrl Pts',(87.358579219789,7.71653928886002,56.89258275411));
#157814=CARTESIAN_POINT('Ctrl Pts',(87.3636142925891,8.88581650983902,57.36610360856));
#157815=CARTESIAN_POINT('Ctrl Pts',(87.3634445492491,9.61075958397102,57.64159291478));
#157816=CARTESIAN_POINT('Ctrl Pts',(87.3624396251191,9.93428100300701,57.75825728172));
#157817=CARTESIAN_POINT('Ctrl Pts',(86.2613172939992,3.33310591270701,54.71370312083));
#157818=CARTESIAN_POINT('Ctrl Pts',(86.2511508016791,3.95136525321801,54.87718011019));
#157819=CARTESIAN_POINT('Ctrl Pts',(86.2276527558891,5.09342510158102,55.26541508777));
#157820=CARTESIAN_POINT('Ctrl Pts',(86.1907592952991,6.61840325577501,55.94310458405));
#157821=CARTESIAN_POINT('Ctrl Pts',(86.1610107349092,7.93502804762402,56.59794889373));
#157822=CARTESIAN_POINT('Ctrl Pts',(86.1403419786992,9.05776198640001,57.16244255609));
#157823=CARTESIAN_POINT('Ctrl Pts',(86.1292733867091,9.75138372308601,57.49279715768));
#157824=CARTESIAN_POINT('Ctrl Pts',(86.1244212943492,10.06113013545,57.63371115991));
#157825=CARTESIAN_POINT('Ctrl Pts',(85.3372217806292,3.17169945627801,55.54091804455));
#157826=CARTESIAN_POINT('Ctrl Pts',(85.3463626117991,3.75698441837301,55.7195292026701));
#157827=CARTESIAN_POINT('Ctrl Pts',(85.3702987241291,4.83618885125201,56.14247256533));
#157828=CARTESIAN_POINT('Ctrl Pts',(85.4259847846291,6.28522424215701,56.87789547744));
#157829=CARTESIAN_POINT('Ctrl Pts',(85.4947450446091,7.55724130294601,57.58893555709));
#157830=CARTESIAN_POINT('Ctrl Pts',(85.5664123570691,8.66907253684701,58.20510965777));
#157831=CARTESIAN_POINT('Ctrl Pts',(85.6142557518591,9.37232556154801,58.56812537839));
#157832=CARTESIAN_POINT('Ctrl Pts',(85.6357422321091,9.68980400619803,58.7234820586301));
#157833=CARTESIAN_POINT('Ctrl Pts',(85.897825663029,2.88509423422901,56.62159832173));
#157834=CARTESIAN_POINT('Ctrl Pts',(85.9320873103392,3.42484799939702,56.77510303408));
#157835=CARTESIAN_POINT('Ctrl Pts',(86.0152891009691,4.43677839367301,57.1406017625));
#157836=CARTESIAN_POINT('Ctrl Pts',(86.1714598873992,5.85025612247802,57.78611107631));
#157837=CARTESIAN_POINT('Ctrl Pts',(86.3326959020691,7.13484173987302,58.41845554155));
#157838=CARTESIAN_POINT('Ctrl Pts',(86.4799055365392,8.28733150922102,58.97155140682));
#157839=CARTESIAN_POINT('Ctrl Pts',(86.5704455885891,9.02710436949802,59.29733070642));
#157840=CARTESIAN_POINT('Ctrl Pts',(86.6099955101491,9.36253119362102,59.43623320246));
#157841=CARTESIAN_POINT('Ctrl Pts',(87.0452039026617,3.32467973944959,55.2706236824217));
#157842=CARTESIAN_POINT('Ctrl Pts',(87.0158957985298,3.32776504208187,55.2636439986755));
#157843=CARTESIAN_POINT('Ctrl Pts',(86.9855492369739,3.33060899420873,55.2577943865739));
#157844=CARTESIAN_POINT('Ctrl Pts',(86.954273199712,3.33315210107447,55.2532910470087));
#157845=CARTESIAN_POINT('Ctrl Pts',(86.9240766939803,3.3356074294271,55.248943145839));
#157846=CARTESIAN_POINT('Ctrl Pts',(86.8930137891819,3.33778213321698,55.2458509258659));
#157847=CARTESIAN_POINT('Ctrl Pts',(86.8612303516663,3.33962200565783,55.2442031639726));
#157848=CARTESIAN_POINT('Ctrl Pts',(86.8300187823837,3.34142877391977,55.2425850496806));
#157849=CARTESIAN_POINT('Ctrl Pts',(86.7981124841258,3.34291245168442,55.2423606500344));
#157850=CARTESIAN_POINT('Ctrl Pts',(86.7656957486977,3.34402389978898,55.2436919623959));
#157851=CARTESIAN_POINT('Ctrl Pts',(86.7340599142816,3.3451085737308,55.2449912041878));
#157852=CARTESIAN_POINT('Ctrl Pts',(86.701938312397,3.3458385465234,55.2477727877885));
#157853=CARTESIAN_POINT('Ctrl Pts',(86.6695429664898,3.34617310499231,55.2521605662374));
#157854=CARTESIAN_POINT('Ctrl Pts',(86.6391263937711,3.34648722795391,55.2562803303124));
#157855=CARTESIAN_POINT('Ctrl Pts',(86.6084691690557,3.34645266903372,55.2618163294321));
#157856=CARTESIAN_POINT('Ctrl Pts',(86.5777752292993,3.34604211469778,55.2688409060828));
#157857=CARTESIAN_POINT('Ctrl Pts',(86.5459495982834,3.34561642314723,55.2761244801794));
#157858=CARTESIAN_POINT('Ctrl Pts',(86.5140851157249,3.34478628831945,55.2850091585276));
#157859=CARTESIAN_POINT('Ctrl Pts',(86.4824330539896,3.3435306994631,55.2955334219386));
#157860=CARTESIAN_POINT('Ctrl Pts',(86.4511198312397,3.34228855183082,55.3059450218913));
#157861=CARTESIAN_POINT('Ctrl Pts',(86.4200153076962,3.34062990468923,55.3179615663613));
#157862=CARTESIAN_POINT('Ctrl Pts',(86.3893759355848,3.33854598242068,55.3315724121411));
#157863=CARTESIAN_POINT('Ctrl Pts',(86.3590494891505,3.3364833436427,55.34504424779));
#157864=CARTESIAN_POINT('Ctrl Pts',(86.3291795977555,3.33400402460446,55.3600780218181));
#157865=CARTESIAN_POINT('Ctrl Pts',(86.3000155403359,3.33111205258089,55.3766139078715));
#157866=CARTESIAN_POINT('Ctrl Pts',(86.2709862787503,3.32823344720845,55.3930733653087));
#157867=CARTESIAN_POINT('Ctrl Pts',(86.242657192776,3.32494599924483,55.4110209129365));
#157868=CARTESIAN_POINT('Ctrl Pts',(86.2152619343509,3.32126650475866,55.4303491660492));
#157869=CARTESIAN_POINT('Ctrl Pts',(86.1879315787459,3.31759572745868,55.4496316280941));
#157870=CARTESIAN_POINT('Ctrl Pts',(86.1615314102079,3.31353482388904,55.4702878684087));
#157871=CARTESIAN_POINT('Ctrl Pts',(86.1362689969526,3.30911274928937,55.4921671897273));
#157872=CARTESIAN_POINT('Ctrl Pts',(86.1281989003645,3.30770011428974,55.4991565550956));
#157873=CARTESIAN_POINT('Ctrl Pts',(86.1202446763264,3.30625071155674,55.5062704236528));
#157874=CARTESIAN_POINT('Ctrl Pts',(86.1124123761509,3.30476572772039,55.5135030525225));
#157875=CARTESIAN_POINT('Ctrl Pts',(86.0878456929179,3.30010794817974,55.5361888151211));
#157876=CARTESIAN_POINT('Ctrl Pts',(86.0644816855133,3.29509940836546,55.5600451696905));
#157877=CARTESIAN_POINT('Ctrl Pts',(86.042480546915,3.28978327466456,55.584873701666));
#157878=CARTESIAN_POINT('Ctrl Pts',(86.020389922166,3.28444551843085,55.6098032197674));
#157879=CARTESIAN_POINT('Ctrl Pts',(85.9996736672954,3.27879783898094,55.6357120694331));
#157880=CARTESIAN_POINT('Ctrl Pts',(85.9804477687263,3.27289200124217,55.6623757495974));
#157881=CARTESIAN_POINT('Ctrl Pts',(85.9609988972839,3.26691767039216,55.689348662506));
#157882=CARTESIAN_POINT('Ctrl Pts',(85.9430753564791,3.26067936348671,55.7170931720327));
#157883=CARTESIAN_POINT('Ctrl Pts',(85.9267454044346,3.25423600214559,55.7453649914734));
#157884=CARTESIAN_POINT('Ctrl Pts',(85.9102838611362,3.24774071842311,55.7738646330263));
#157885=CARTESIAN_POINT('Ctrl Pts',(85.8954416007959,3.24103728370016,55.8028992605736));
#157886=CARTESIAN_POINT('Ctrl Pts',(85.8822353778661,3.23418818270307,55.8322196284447));
#157887=CARTESIAN_POINT('Ctrl Pts',(85.8688229092946,3.22723211719102,55.8619979015108));
#157888=CARTESIAN_POINT('Ctrl Pts',(85.857097692062,3.22012601782691,55.8920701018972));
#157889=CARTESIAN_POINT('Ctrl Pts',(85.8470254504323,3.21293416110448,55.9221889194256));
#157890=CARTESIAN_POINT('Ctrl Pts',(85.8443086057684,3.21099425951367,55.9303130442924));
#157891=CARTESIAN_POINT('Ctrl Pts',(85.8417117555785,3.20904810176126,55.9384406745451));
#157892=CARTESIAN_POINT('Ctrl Pts',(85.8392336483774,3.20709690456849,55.9465672349548));
#157893=CARTESIAN_POINT('Ctrl Pts',(85.8298346306164,3.19969636230698,55.9773898263238));
#157894=CARTESIAN_POINT('Ctrl Pts',(85.8221469851188,3.19222381292407,56.0081944884238));
#157895=CARTESIAN_POINT('Ctrl Pts',(85.8160748683465,3.18474201124346,56.0387512009237));
#157896=CARTESIAN_POINT('Ctrl Pts',(85.8098131955518,3.17702664676749,56.0702618161722));
#157897=CARTESIAN_POINT('Ctrl Pts',(85.8052688157992,3.16930161800696,56.1015081902615));
#157898=CARTESIAN_POINT('Ctrl Pts',(85.802298117403,3.16162730259475,56.1322781164847));
#157899=CARTESIAN_POINT('Ctrl Pts',(85.799273347267,3.15381330165044,56.1636081074546));
#157900=CARTESIAN_POINT('Ctrl Pts',(85.7978792042002,3.14605197890152,56.1944438989833));
#157901=CARTESIAN_POINT('Ctrl Pts',(85.7979368396176,3.13839632796352,56.224608603399));
#157902=CARTESIAN_POINT('Ctrl Pts',(85.7979964570438,3.13047740890124,56.2558106337346));
#157903=CARTESIAN_POINT('Ctrl Pts',(85.7996085440693,3.12267162815719,56.2862944915633));
#157904=CARTESIAN_POINT('Ctrl Pts',(85.8025597451988,3.11502482592699,56.3159175912647));
#157905=CARTESIAN_POINT('Ctrl Pts',(85.8049366353535,3.10886611015733,56.3397759631416));
#157906=CARTESIAN_POINT('Ctrl Pts',(85.8081817163382,3.10281025135304,56.3630771210913));
#157907=CARTESIAN_POINT('Ctrl Pts',(85.8121821974198,3.09687523453361,56.385770301083));
#157908=CARTESIAN_POINT('Ctrl Pts',(87.3066738932391,-0.160558520523986,
54.99748094861));
#157909=CARTESIAN_POINT('Ctrl Pts',(87.3057973027491,0.222559046269814,
54.9925095569101));
#157910=CARTESIAN_POINT('Ctrl Pts',(87.3104980049391,1.01336829601901,55.01916856379));
#157911=CARTESIAN_POINT('Ctrl Pts',(87.3376450103591,2.21501333732301,55.17312688208));
#157912=CARTESIAN_POINT('Ctrl Pts',(87.3692248653891,3.02064717406401,55.35222513978));
#157913=CARTESIAN_POINT('Ctrl Pts',(87.3880905029791,3.42517613974502,55.45921748724));
#157914=CARTESIAN_POINT('Ctrl Pts',(86.2302484602191,-0.172977764866286,
54.23064612836));
#157915=CARTESIAN_POINT('Ctrl Pts',(86.2293040482491,0.239788826433014,
54.22529010194));
#157916=CARTESIAN_POINT('Ctrl Pts',(86.234373747229,1.09161263914201,54.25404179361));
#157917=CARTESIAN_POINT('Ctrl Pts',(86.2635437845591,2.38161775413201,54.41947329601));
#157918=CARTESIAN_POINT('Ctrl Pts',(86.2972481600892,3.24065865070901,54.6106203082));
#157919=CARTESIAN_POINT('Ctrl Pts',(86.3172509644792,3.66957413486501,54.72406184906));
#157920=CARTESIAN_POINT('Ctrl Pts',(85.2315241728891,-0.164025917707086,
55.09629689782));
#157921=CARTESIAN_POINT('Ctrl Pts',(85.2306286469491,0.227369523425714,
55.09121811783));
#157922=CARTESIAN_POINT('Ctrl Pts',(85.2354323713891,1.03521376483001,55.1184613929));
#157923=CARTESIAN_POINT('Ctrl Pts',(85.2631441982191,2.26152854143701,55.27562297261));
#157924=CARTESIAN_POINT('Ctrl Pts',(85.2953172098191,3.08207338916501,55.45808518839));
#157925=CARTESIAN_POINT('Ctrl Pts',(85.314500339269,3.49341096116101,55.56687812165));
#157926=CARTESIAN_POINT('Ctrl Pts',(85.837848582719,-0.147393025451686,
56.27059483639));
#157927=CARTESIAN_POINT('Ctrl Pts',(85.8370438889791,0.204293958669714,
56.26603119144));
#157928=CARTESIAN_POINT('Ctrl Pts',(85.8413534220091,0.930422386796514,
56.29047176775));
#157929=CARTESIAN_POINT('Ctrl Pts',(85.8663558350591,2.03839795170801,56.43226749832));
#157930=CARTESIAN_POINT('Ctrl Pts',(85.8956835108491,2.78741559154501,56.59859301288));
#157931=CARTESIAN_POINT('Ctrl Pts',(85.9133436512691,3.16609269539302,56.69874864616));
#157932=CARTESIAN_POINT('Origin',(86.7262508506842,-3.18494591445562E-7,
55.8108970052131));
#157933=CARTESIAN_POINT('Ctrl Pts',(87.3881016241291,-3.42500607027599,
55.45920812828));
#157934=CARTESIAN_POINT('Ctrl Pts',(87.3689745152091,-3.01484055255599,
55.35073290318));
#157935=CARTESIAN_POINT('Ctrl Pts',(87.3372398307191,-2.20322903616999,
55.17075656397));
#157936=CARTESIAN_POINT('Ctrl Pts',(87.3103828227291,-1.00133939355599,
55.01844290285));
#157937=CARTESIAN_POINT('Ctrl Pts',(87.3058297848591,-0.216519809292486,
54.99262134195));
#157938=CARTESIAN_POINT('Ctrl Pts',(87.3066901921091,0.160504427251014,
54.99750095394));
#157939=CARTESIAN_POINT('Ctrl Pts',(86.3172693262291,-3.66938489029899,
54.72402342508));
#157940=CARTESIAN_POINT('Ctrl Pts',(86.2969910364991,-3.23453191356599,
54.60901952918));
#157941=CARTESIAN_POINT('Ctrl Pts',(86.2631186790491,-2.36907727584199,
54.41691984417));
#157942=CARTESIAN_POINT('Ctrl Pts',(86.2342558402292,-1.07862444435799,
54.25323055111));
#157943=CARTESIAN_POINT('Ctrl Pts',(86.2293462065792,-0.233245776100886,
54.22538663505));
#157944=CARTESIAN_POINT('Ctrl Pts',(86.2302729794091,0.172898711608914,
54.23064262496));
#157945=CARTESIAN_POINT('Ctrl Pts',(85.3145018225292,-3.49324296266999,
55.56683463126));
#157946=CARTESIAN_POINT('Ctrl Pts',(85.295053274129,-3.07618406734899,55.45653643227));
#157947=CARTESIAN_POINT('Ctrl Pts',(85.262721696009,-2.24953815773399,55.2731749411));
#157948=CARTESIAN_POINT('Ctrl Pts',(85.2353046081391,-1.02291938029399,
55.11768490907));
#157949=CARTESIAN_POINT('Ctrl Pts',(85.2306519994892,-0.221190132183786,
55.09129865426));
#157950=CARTESIAN_POINT('Ctrl Pts',(85.2315309377292,0.163965232274714,
55.09628336072));
#157951=CARTESIAN_POINT('Ctrl Pts',(85.9133362962291,-3.16595498744899,
56.69872650143));
#157952=CARTESIAN_POINT('Ctrl Pts',(85.895429483869,-2.78195913937999,56.59717192208));
#157953=CARTESIAN_POINT('Ctrl Pts',(85.8659608161091,-2.02742343211599,
56.43004680237));
#157954=CARTESIAN_POINT('Ctrl Pts',(85.841230067059,-0.919414224694086,
56.28979175488));
#157955=CARTESIAN_POINT('Ctrl Pts',(85.837055034629,-0.198789631969386,
56.26611396935));
#157956=CARTESIAN_POINT('Ctrl Pts',(85.8378450917691,0.147366002311014,
56.27059460606));
#157957=CARTESIAN_POINT('Ctrl Pts',(87.0452086535361,-3.32464023403444,
55.2705714208367));
#157958=CARTESIAN_POINT('Ctrl Pts',(87.0161338191475,-3.32769428602402,
55.2636452372544));
#157959=CARTESIAN_POINT('Ctrl Pts',(86.9860064240394,-3.33051660652347,
55.2578243001712));
#157960=CARTESIAN_POINT('Ctrl Pts',(86.9549270148153,-3.33304666480274,
55.2533279251216));
#157961=CARTESIAN_POINT('Ctrl Pts',(86.9249635095899,-3.33548588151774,
55.2489929921014));
#157962=CARTESIAN_POINT('Ctrl Pts',(86.8941151025206,-3.33765326081566,
55.245889948207));
#157963=CARTESIAN_POINT('Ctrl Pts',(86.8625197855615,-3.33949324230545,
55.2442120543826));
#157964=CARTESIAN_POINT('Ctrl Pts',(86.8315197407038,-3.34129855759298,
55.242565772945));
#157965=CARTESIAN_POINT('Ctrl Pts',(86.7998007206826,-3.34278849749598,
55.2422922168608));
#157966=CARTESIAN_POINT('Ctrl Pts',(86.7675399999893,-3.34391209160149,
55.2435596897975));
#157967=CARTESIAN_POINT('Ctrl Pts',(86.736097421926,-3.34500719098597,55.2447950191981));
#157968=CARTESIAN_POINT('Ctrl Pts',(86.7041405970569,-3.34575409864029,
55.2474949039633));
#157969=CARTESIAN_POINT('Ctrl Pts',(86.6718757613232,-3.34610992515415,
55.2517907778763));
#157970=CARTESIAN_POINT('Ctrl Pts',(86.6430925422921,-3.34642735533015,
55.255623094916));
#157971=CARTESIAN_POINT('Ctrl Pts',(86.61406497309,-3.34643350640855,55.2607255884706));
#157972=CARTESIAN_POINT('Ctrl Pts',(86.5849648306966,-3.34610283753138,
55.2671677479827));
#157973=CARTESIAN_POINT('Ctrl Pts',(86.5532472021764,-3.34574242580324,
55.2741893638742));
#157974=CARTESIAN_POINT('Ctrl Pts',(86.5214433295666,-3.34498159188331,
55.2828035872345));
#157975=CARTESIAN_POINT('Ctrl Pts',(86.4898015752697,-3.34379635323437,
55.2930611493146));
#157976=CARTESIAN_POINT('Ctrl Pts',(86.4585364163671,-3.34262522111733,
55.3031966274357));
#157977=CARTESIAN_POINT('Ctrl Pts',(86.4274303116597,-3.34103960634926,
55.3149368972055));
#157978=CARTESIAN_POINT('Ctrl Pts',(86.3967395298491,-3.33902749693949,
55.3282841139911));
#157979=CARTESIAN_POINT('Ctrl Pts',(86.3664165371889,-3.33703950004712,
55.3414713817225));
#157980=CARTESIAN_POINT('Ctrl Pts',(86.3364998186016,-3.33463510590651,
55.3562274133762));
#157981=CARTESIAN_POINT('Ctrl Pts',(86.307240872989,-3.331815016697,55.372505092502));
#157982=CARTESIAN_POINT('Ctrl Pts',(86.2781476065118,-3.32901089627693,
55.3886905990718));
#157983=CARTESIAN_POINT('Ctrl Pts',(86.2497055440448,-3.32579576135565,
55.406380472337));
#157984=CARTESIAN_POINT('Ctrl Pts',(86.222153506037,-3.32218312108875,55.4254793526165));
#157985=CARTESIAN_POINT('Ctrl Pts',(86.1947086340817,-3.31858453250096,
55.4445039461368));
#157986=CARTESIAN_POINT('Ctrl Pts',(86.1681476825843,-3.31459157231305,
55.4649262777229));
#157987=CARTESIAN_POINT('Ctrl Pts',(86.1426857976783,-3.31023010145211,
55.4866064774387));
#157988=CARTESIAN_POINT('Ctrl Pts',(86.1350465971449,-3.30892155141152,
55.4931110780936));
#157989=CARTESIAN_POINT('Ctrl Pts',(86.1275061415236,-3.30757991230072,
55.4997286139691));
#157990=CARTESIAN_POINT('Ctrl Pts',(86.1200697122403,-3.30620608885032,
55.5064545877257));
#157991=CARTESIAN_POINT('Ctrl Pts',(86.0952811849256,-3.30162659796451,
55.5288748888987));
#157992=CARTESIAN_POINT('Ctrl Pts',(86.0716515487885,-3.29668873202253,
55.5525025819528));
#157993=CARTESIAN_POINT('Ctrl Pts',(86.0493521079058,-3.29143289234783,
55.5771483320876));
#157994=CARTESIAN_POINT('Ctrl Pts',(86.0269902517838,-3.286162341789,55.601863064687));
#157995=CARTESIAN_POINT('Ctrl Pts',(86.0059665084832,-3.2805722003403,55.6276008284941));
#157996=CARTESIAN_POINT('Ctrl Pts',(85.9864096839156,-3.27471204681387,
55.6541436075309));
#157997=CARTESIAN_POINT('Ctrl Pts',(85.9666618803187,-3.26879466689938,
55.6809455858133));
#157998=CARTESIAN_POINT('Ctrl Pts',(85.9484100621666,-3.26260217229768,
55.7085675546546));
#157999=CARTESIAN_POINT('Ctrl Pts',(85.931736394215,-3.25619186561974,55.7367692789791));
#158000=CARTESIAN_POINT('Ctrl Pts',(85.914946330045,-3.24973680961259,55.7651678750462));
#158001=CARTESIAN_POINT('Ctrl Pts',(85.8997565149374,-3.24306110901668,
55.794153487594));
#158002=CARTESIAN_POINT('Ctrl Pts',(85.8861979421808,-3.23622641362624,
55.8234777690152));
#158003=CARTESIAN_POINT('Ctrl Pts',(85.8724469419851,-3.22929471813451,
55.8532182296669));
#158004=CARTESIAN_POINT('Ctrl Pts',(85.8603736020248,-3.22219970311276,
55.8833062096247));
#158005=CARTESIAN_POINT('Ctrl Pts',(85.8499576407623,-3.21500553713045,
55.9134924759869));
#158006=CARTESIAN_POINT('Ctrl Pts',(85.8469372655869,-3.21291940414731,
55.9222457583063));
#158007=CARTESIAN_POINT('Ctrl Pts',(85.8440559326875,-3.21082492144357,
55.9310074108718));
#158008=CARTESIAN_POINT('Ctrl Pts',(85.8413123914781,-3.20872361198818,
55.9397716540776));
#158009=CARTESIAN_POINT('Ctrl Pts',(85.8316470423775,-3.2013208110442,55.9706476146413));
#158010=CARTESIAN_POINT('Ctrl Pts',(85.8236951720488,-3.19383373360089,
56.0015534440733));
#158011=CARTESIAN_POINT('Ctrl Pts',(85.8173727327578,-3.18632561112764,
56.0322542653455));
#158012=CARTESIAN_POINT('Ctrl Pts',(85.8108631967492,-3.17859530461987,
56.0638636003451));
#158013=CARTESIAN_POINT('Ctrl Pts',(85.8060803265883,-3.17084287445321,
56.0952549946809));
#158014=CARTESIAN_POINT('Ctrl Pts',(85.8028912389185,-3.16312973200661,
56.1262093260497));
#158015=CARTESIAN_POINT('Ctrl Pts',(85.7996472066774,-3.15528370036114,
56.1576969674572));
#158016=CARTESIAN_POINT('Ctrl Pts',(85.7980515083608,-3.14747844002179,
56.1887320383206));
#158017=CARTESIAN_POINT('Ctrl Pts',(85.7979338246624,-3.13976850575949,
56.2191290300128));
#158018=CARTESIAN_POINT('Ctrl Pts',(85.797812224897,-3.13180201413088,56.2505375182842));
#158019=CARTESIAN_POINT('Ctrl Pts',(85.7992677760407,-3.12393738863357,
56.2812645518244));
#158020=CARTESIAN_POINT('Ctrl Pts',(85.8020935481781,-3.11622246369485,
56.3111575270582));
#158021=CARTESIAN_POINT('Ctrl Pts',(85.804503994011,-3.10964146290445,56.3366568929241));
#158022=CARTESIAN_POINT('Ctrl Pts',(85.8079108851163,-3.10316916366077,
56.3615503605815));
#158023=CARTESIAN_POINT('Ctrl Pts',(85.8121822996917,-3.09682809692899,
56.3857720505554));
#158024=CARTESIAN_POINT('Ctrl Pts',(87.7631107484691,-9.86087935710899,
57.88435148745));
#158025=CARTESIAN_POINT('Ctrl Pts',(87.728897687669,-9.33637382671099,57.69031957761));
#158026=CARTESIAN_POINT('Ctrl Pts',(87.6485159203691,-8.21061242792599,
57.23445192227));
#158027=CARTESIAN_POINT('Ctrl Pts',(87.5191833454691,-6.52081640480999,
56.50097044125));
#158028=CARTESIAN_POINT('Ctrl Pts',(87.399308616539,-4.80924371223799,55.82112707061));
#158029=CARTESIAN_POINT('Ctrl Pts',(87.3381855483191,-3.67011481886699,
55.47448092506));
#158030=CARTESIAN_POINT('Ctrl Pts',(87.3149793525591,-3.12718060160599,
55.34287204894));
#158031=CARTESIAN_POINT('Ctrl Pts',(86.7045062565192,-10.15160363171,57.2850598679101));
#158032=CARTESIAN_POINT('Ctrl Pts',(86.6713315074291,-9.64303537257999,
57.09691651656));
#158033=CARTESIAN_POINT('Ctrl Pts',(86.5926852603991,-8.540837710357,56.65089148561));
#158034=CARTESIAN_POINT('Ctrl Pts',(86.4632718589192,-6.85002147353099,
55.91695161455));
#158035=CARTESIAN_POINT('Ctrl Pts',(86.3401158359792,-5.09357790444299,
55.21849910066));
#158036=CARTESIAN_POINT('Ctrl Pts',(86.275884280909,-3.89841031468999,54.85422385018));
#158037=CARTESIAN_POINT('Ctrl Pts',(86.2513679124891,-3.32479822433799,
54.71518461565));
#158038=CARTESIAN_POINT('Ctrl Pts',(85.7816779657691,-9.91232327874599,
58.0946566077));
#158039=CARTESIAN_POINT('Ctrl Pts',(85.7476486351392,-9.39063786282099,
57.90166668358));
#158040=CARTESIAN_POINT('Ctrl Pts',(85.6675739697391,-8.269046088395,57.44754068947));
#158041=CARTESIAN_POINT('Ctrl Pts',(85.5382270924591,-6.57906953754599,
56.7139780959199));
#158042=CARTESIAN_POINT('Ctrl Pts',(85.4177717356291,-4.85955690305299,
56.03084182066));
#158043=CARTESIAN_POINT('Ctrl Pts',(85.3560986178691,-3.71051191200099,
55.6810761891501));
#158044=CARTESIAN_POINT('Ctrl Pts',(85.3326605858791,-3.16214921752899,
55.54815250443));
#158045=CARTESIAN_POINT('Ctrl Pts',(86.3421937596991,-9.49244947474399,
59.13092116154));
#158046=CARTESIAN_POINT('Ctrl Pts',(86.3066648642291,-8.94774691405598,
58.92942678263));
#158047=CARTESIAN_POINT('Ctrl Pts',(86.2240837019491,-7.79212359644,58.46108573835));
#158048=CARTESIAN_POINT('Ctrl Pts',(86.0948535570791,-6.10362047264499,
57.72818516716));
#158049=CARTESIAN_POINT('Ctrl Pts',(85.9791371557891,-4.44891187158699,
57.0719248443));
#158050=CARTESIAN_POINT('Ctrl Pts',(85.9219534195892,-3.38079985613399,
56.74761976079));
#158051=CARTESIAN_POINT('Ctrl Pts',(85.900407583149,-2.87674318079599,56.62542725032));
#158052=CARTESIAN_POINT('Origin',(28.1938561267191,10.75942675157,83.17555499762));
#158053=CARTESIAN_POINT('Ctrl Pts',(80.8776256911591,11.53578371495,74.526004930479));
#158054=CARTESIAN_POINT('Ctrl Pts',(80.6466807255579,11.4265581751583,74.7033356918515));
#158055=CARTESIAN_POINT('Ctrl Pts',(80.4344623573573,11.2910809302903,74.8372090682622));
#158056=CARTESIAN_POINT('Ctrl Pts',(80.0485761754778,11.0189816647197,75.0242644873895));
#158057=CARTESIAN_POINT('Ctrl Pts',(79.8750390236475,10.8824621328803,75.0781875502727));
#158058=CARTESIAN_POINT('Ctrl Pts',(79.7231088722891,10.75948375202,75.104988805765));
#158059=CARTESIAN_POINT('Ctrl Pts',(80.0846671696191,12.2337111353,74.375202534073));
#158060=CARTESIAN_POINT('Ctrl Pts',(80.0643038624191,12.19866929898,74.425273469824));
#158061=CARTESIAN_POINT('Ctrl Pts',(79.9719432784991,12.03291962305,74.64145218167));
#158062=CARTESIAN_POINT('Ctrl Pts',(79.8139703990991,11.69505677215,74.933862536297));
#158063=CARTESIAN_POINT('Ctrl Pts',(79.6130676484391,11.21422968175,75.144853266097));
#158064=CARTESIAN_POINT('Ctrl Pts',(79.4721307191891,10.90433893298,75.186980135866));
#158065=CARTESIAN_POINT('Ctrl Pts',(79.3982473483891,10.76260680237,75.186691133753));
#158066=CARTESIAN_POINT('Ctrl Pts',(79.3950256211791,10.75646376115,75.186639953909));
#158067=CARTESIAN_POINT('Ctrl Pts',(80.3666475076091,11.86746169039,74.288033087485));
#158068=CARTESIAN_POINT('Ctrl Pts',(80.3506099828591,11.83751354529,74.331758606035));
#158069=CARTESIAN_POINT('Ctrl Pts',(80.2779714098091,11.69543897126,74.5214403561681));
#158070=CARTESIAN_POINT('Ctrl Pts',(80.1528671321391,11.40235418381,74.784376539898));
#158071=CARTESIAN_POINT('Ctrl Pts',(79.9858604313792,10.97672372266,74.981925061155));
#158072=CARTESIAN_POINT('Ctrl Pts',(79.8610606286691,10.69698164451,75.023072286078));
#158073=CARTESIAN_POINT('Ctrl Pts',(79.7931833543991,10.56824068116,75.021923137852));
#158074=CARTESIAN_POINT('Ctrl Pts',(79.7902192472791,10.56265943354,75.021833601096));
#158075=CARTESIAN_POINT('Ctrl Pts',(80.7663533791792,11.62255509433,74.3280108745551));
#158076=CARTESIAN_POINT('Ctrl Pts',(80.7521047661192,11.59565552083,74.369584739658));
#158077=CARTESIAN_POINT('Ctrl Pts',(80.6875878118291,11.46716013595,74.5513747886651));
#158078=CARTESIAN_POINT('Ctrl Pts',(80.5738009008192,11.19460864096,74.81355029025));
#158079=CARTESIAN_POINT('Ctrl Pts',(80.4106645115891,10.77986391846,75.022702472629));
#158080=CARTESIAN_POINT('Ctrl Pts',(80.2825653231991,10.49399265843,75.06900603011));
#158081=CARTESIAN_POINT('Ctrl Pts',(80.2118938500291,10.35949997223,75.066743547213));
#158082=CARTESIAN_POINT('Ctrl Pts',(80.2088062088191,10.35366403843,75.066598511338));
#158083=CARTESIAN_POINT('Ctrl Pts',(81.2029062710791,11.54854698987,74.487046587091));
#158084=CARTESIAN_POINT('Ctrl Pts',(81.1875477215091,11.52203400491,74.531097938973));
#158085=CARTESIAN_POINT('Ctrl Pts',(81.1179086243191,11.39427421441,74.7251983942701));
#158086=CARTESIAN_POINT('Ctrl Pts',(80.9915978315291,11.11385643038,75.015480622744));
#158087=CARTESIAN_POINT('Ctrl Pts',(80.8015228769991,10.66348388033,75.25893439227));
#158088=CARTESIAN_POINT('Ctrl Pts',(80.6513554051391,10.3364457957,75.3154869012339));
#158089=CARTESIAN_POINT('Ctrl Pts',(80.5696548300191,10.17862232931,75.31208317289));
#158090=CARTESIAN_POINT('Ctrl Pts',(80.5660874970391,10.17176676406,75.311876725662));
#158091=CARTESIAN_POINT('Origin',(79.9839384245637,10.7602162427584,76.5820094885442));
#158092=CARTESIAN_POINT('Ctrl Pts',(78.760931083689,11.61208641416,76.341387867119));
#158093=CARTESIAN_POINT('Ctrl Pts',(78.720761931639,11.54538801364,76.34960017132));
#158094=CARTESIAN_POINT('Ctrl Pts',(78.539124905319,11.21497913113,76.384095471138));
#158095=CARTESIAN_POINT('Ctrl Pts',(78.3272248697091,10.53130051923,76.395483468053));
#158096=CARTESIAN_POINT('Ctrl Pts',(78.3210903544191,9.65920748234801,76.30462454924));
#158097=CARTESIAN_POINT('Ctrl Pts',(78.4990584433091,8.88612097175701,76.14832993757));
#158098=CARTESIAN_POINT('Ctrl Pts',(78.7939422207591,8.19874503162601,75.957853167008));
#158099=CARTESIAN_POINT('Ctrl Pts',(79.175049588149,7.56852236834102,75.750228152338));
#158100=CARTESIAN_POINT('Ctrl Pts',(79.6296693412391,6.97116568539302,75.534928347765));
#158101=CARTESIAN_POINT('Ctrl Pts',(80.1516532961491,6.39047926863501,75.318663026047));
#158102=CARTESIAN_POINT('Ctrl Pts',(80.7411739705891,5.81082699109101,75.104561720609));
#158103=CARTESIAN_POINT('Ctrl Pts',(81.396531416289,5.21759815199301,74.898979890115));
#158104=CARTESIAN_POINT('Ctrl Pts',(81.9189771327191,4.76455349315301,74.760481913992));
#158105=CARTESIAN_POINT('Ctrl Pts',(82.2187668424891,4.50327324549201,74.68987766881));
#158106=CARTESIAN_POINT('Ctrl Pts',(82.2811754718592,4.44871069526601,74.675560443258));
#158107=CARTESIAN_POINT('Ctrl Pts',(78.8641595298191,11.42713922143,75.170127744247));
#158108=CARTESIAN_POINT('Ctrl Pts',(78.8278635622092,11.36880057166,75.177351358709));
#158109=CARTESIAN_POINT('Ctrl Pts',(78.6656267334791,11.07828617183,75.207759617271));
#158110=CARTESIAN_POINT('Ctrl Pts',(78.4985841602091,10.4656706454,75.2175449663339));
#158111=CARTESIAN_POINT('Ctrl Pts',(78.5706517692291,9.69219344377001,75.1386809316639));
#158112=CARTESIAN_POINT('Ctrl Pts',(78.8344223404291,9.02554784154501,75.011775205111));
#158113=CARTESIAN_POINT('Ctrl Pts',(79.2155386524891,8.44664301813601,74.869303349441));
#158114=CARTESIAN_POINT('Ctrl Pts',(79.6806598076492,7.92214918321301,74.7285580249969));
#158115=CARTESIAN_POINT('Ctrl Pts',(80.216106658139,7.42405260242701,74.599070810471));
#158116=CARTESIAN_POINT('Ctrl Pts',(80.8150297881292,6.93264887820001,74.487264366057));
#158117=CARTESIAN_POINT('Ctrl Pts',(81.4796940616691,6.42787751324401,74.397564004857));
#158118=CARTESIAN_POINT('Ctrl Pts',(82.2075605569891,5.89010509385001,74.336016015736));
#158119=CARTESIAN_POINT('Ctrl Pts',(82.7812018555291,5.45771440216002,74.316072070765));
#158120=CARTESIAN_POINT('Ctrl Pts',(83.1088424495491,5.19888422833301,74.314523364672));
#158121=CARTESIAN_POINT('Ctrl Pts',(83.1769868269691,5.14441402096701,74.31461935357));
#158122=CARTESIAN_POINT('Ctrl Pts',(79.7706198354091,10.83432890579,74.676686459257));
#158123=CARTESIAN_POINT('Ctrl Pts',(79.7490325589191,10.80132183842,74.680400289062));
#158124=CARTESIAN_POINT('Ctrl Pts',(79.6544599950791,10.63596882446,74.696876463484));
#158125=CARTESIAN_POINT('Ctrl Pts',(79.5763468966291,10.27740128958,74.7116546616779));
#158126=CARTESIAN_POINT('Ctrl Pts',(79.6837480171692,9.79409638780401,74.701642073385));
#158127=CARTESIAN_POINT('Ctrl Pts',(79.941183081199,9.339917463521,74.683093063215));
#158128=CARTESIAN_POINT('Ctrl Pts',(80.3003102645891,8.90682682115901,74.671025266222));
#158129=CARTESIAN_POINT('Ctrl Pts',(80.7366466267892,8.47702391690001,74.67336067523));
#158130=CARTESIAN_POINT('Ctrl Pts',(81.2382284760791,8.03362936517301,74.6944785980151));
#158131=CARTESIAN_POINT('Ctrl Pts',(81.7975241299391,7.56330230079001,74.73697187558));
#158132=CARTESIAN_POINT('Ctrl Pts',(82.416043260439,7.04745267379001,74.804224914257));
#158133=CARTESIAN_POINT('Ctrl Pts',(83.0886572931891,6.46826090235701,74.898479664418));
#158134=CARTESIAN_POINT('Ctrl Pts',(83.6137814815491,5.98357472872301,74.988134994262));
#158135=CARTESIAN_POINT('Ctrl Pts',(83.9113586226891,5.68901254023702,75.044415251821));
#158136=CARTESIAN_POINT('Ctrl Pts',(83.9731390541791,5.62687424178201,75.056330974776));
#158137=CARTESIAN_POINT('Ctrl Pts',(80.6669551324391,10.36557764703,75.303823453054));
#158138=CARTESIAN_POINT('Ctrl Pts',(80.657714106889,10.35214424328,75.304655694476));
#158139=CARTESIAN_POINT('Ctrl Pts',(80.6183554741592,10.28491358268,75.309855847824));
#158140=CARTESIAN_POINT('Ctrl Pts',(80.5934484228191,10.13542447521,75.331742363491));
#158141=CARTESIAN_POINT('Ctrl Pts',(80.6616100705791,9.873479922928,75.385658137821));
#158142=CARTESIAN_POINT('Ctrl Pts',(80.8262564189292,9.54714943156901,75.457206384792));
#158143=CARTESIAN_POINT('Ctrl Pts',(81.0749034137791,9.16637857277802,75.5409316618649));
#158144=CARTESIAN_POINT('Ctrl Pts',(81.3954846805991,8.73526357028401,75.634164078232));
#158145=CARTESIAN_POINT('Ctrl Pts',(81.7788961234291,8.252929445145,75.735543351396));
#158146=CARTESIAN_POINT('Ctrl Pts',(82.2175549486792,7.71656115272501,75.843725751213));
#158147=CARTESIAN_POINT('Ctrl Pts',(82.710045723589,7.11361449180501,75.959652084995));
#158148=CARTESIAN_POINT('Ctrl Pts',(83.249223208889,6.43329272587702,76.081678387038));
#158149=CARTESIAN_POINT('Ctrl Pts',(83.6696514644091,5.87028578229801,76.173636010829));
#158150=CARTESIAN_POINT('Ctrl Pts',(83.906226421349,5.53387143463101,76.224629363201));
#158151=CARTESIAN_POINT('Ctrl Pts',(83.9552535116592,5.46318510498301,76.235165622379));
#158152=CARTESIAN_POINT('Ctrl Pts',(82.3561326848172,4.76438284010715,74.6407108450246));
#158153=CARTESIAN_POINT('Ctrl Pts',(82.3991945347386,4.79680410512389,74.6331152640959));
#158154=CARTESIAN_POINT('Ctrl Pts',(82.4427922163751,4.82923978037722,74.6284382682739));
#158155=CARTESIAN_POINT('Ctrl Pts',(82.486641365581,4.86147824934395,74.62671321235));
#158156=CARTESIAN_POINT('Ctrl Pts',(82.5321824331826,4.89496063888104,74.6249215951837));
#158157=CARTESIAN_POINT('Ctrl Pts',(82.5779942257533,4.928230027107,74.6263133473138));
#158158=CARTESIAN_POINT('Ctrl Pts',(82.6237782932783,4.96107054230688,74.6308753087991));
#158159=CARTESIAN_POINT('Ctrl Pts',(82.673481938154,4.99672253640157,74.6358278201389));
#158160=CARTESIAN_POINT('Ctrl Pts',(82.7231525292242,5.03186890885039,74.6445157813354));
#158161=CARTESIAN_POINT('Ctrl Pts',(82.7724394801782,5.06626223667213,74.6568762190072));
#158162=CARTESIAN_POINT('Ctrl Pts',(82.7917148327503,5.07971292710966,74.6617101920865));
#158163=CARTESIAN_POINT('Ctrl Pts',(82.8109318524455,5.09304874392178,74.6671054613116));
#158164=CARTESIAN_POINT('Ctrl Pts',(82.8300707926036,5.10625594687553,74.6730569730185));
#158165=CARTESIAN_POINT('Ctrl Pts',(82.876573958631,5.13834637333808,74.6875177600179));
#158166=CARTESIAN_POINT('Ctrl Pts',(82.9225997647433,5.1696656549185,74.7052614130784));
#158167=CARTESIAN_POINT('Ctrl Pts',(82.9678250499752,5.19999377004828,74.72616425599));
#158168=CARTESIAN_POINT('Ctrl Pts',(83.0141795455772,5.23107913462234,74.7475890128454));
#158169=CARTESIAN_POINT('Ctrl Pts',(83.059692988644,5.26112322435461,74.7723323244376));
#158170=CARTESIAN_POINT('Ctrl Pts',(83.1040409338527,5.28991207347925,74.8002162089175));
#158171=CARTESIAN_POINT('Ctrl Pts',(83.1495121793079,5.31943012259645,74.8288063713131));
#158172=CARTESIAN_POINT('Ctrl Pts',(83.1937581999166,5.34762859821416,74.860698102205));
#158173=CARTESIAN_POINT('Ctrl Pts',(83.2364535655702,5.3743000951368,74.8956568932294));
#158174=CARTESIAN_POINT('Ctrl Pts',(83.2482659793901,5.38167922760294,74.9053288494219));
#158175=CARTESIAN_POINT('Ctrl Pts',(83.2599598349876,5.38894160859464,74.9152353304516));
#158176=CARTESIAN_POINT('Ctrl Pts',(83.2715285462647,5.39608314048418,74.9253708148277));
#158177=CARTESIAN_POINT('Ctrl Pts',(83.3132133905908,5.42181579453126,74.9618913985181));
#158178=CARTESIAN_POINT('Ctrl Pts',(83.3532611144477,5.44597121910875,75.0013790153269));
#158179=CARTESIAN_POINT('Ctrl Pts',(83.3913802560555,5.46837375986761,75.0435451308988));
#158180=CARTESIAN_POINT('Ctrl Pts',(83.4288356830262,5.49038623690562,75.0849770676063));
#158181=CARTESIAN_POINT('Ctrl Pts',(83.4644290819774,5.51070630669796,75.1289951816093));
#158182=CARTESIAN_POINT('Ctrl Pts',(83.4979051902054,5.5291879854873,75.1752857753653));
#158183=CARTESIAN_POINT('Ctrl Pts',(83.5302094526534,5.5470227050438,75.219955946682));
#158184=CARTESIAN_POINT('Ctrl Pts',(83.5605418940536,5.5631453631716,75.2667422958217));
#158185=CARTESIAN_POINT('Ctrl Pts',(83.5886944258666,5.57744529689563,75.3153243140312));
#158186=CARTESIAN_POINT('Ctrl Pts',(83.5970875853033,5.58170855905898,75.329808148995));
#158187=CARTESIAN_POINT('Ctrl Pts',(83.6052871483651,5.58580996392761,75.3444513188558));
#158188=CARTESIAN_POINT('Ctrl Pts',(83.6132880352556,5.58974698551495,75.3592446366348));
#158189=CARTESIAN_POINT('Ctrl Pts',(83.6414216489043,5.60359078130662,75.4112625557317));
#158190=CARTESIAN_POINT('Ctrl Pts',(83.6670887093203,5.61539658439895,75.4651226559922));
#158191=CARTESIAN_POINT('Ctrl Pts',(83.6901149815983,5.62509354660136,75.5204638505852));
#158192=CARTESIAN_POINT('Ctrl Pts',(83.7117988663748,5.6342251945095,75.572578759697));
#158193=CARTESIAN_POINT('Ctrl Pts',(83.7311402923122,5.64148624770732,75.6260073548933));
#158194=CARTESIAN_POINT('Ctrl Pts',(83.7480075792902,5.64683278713781,75.6804081268761));
#158195=CARTESIAN_POINT('Ctrl Pts',(83.76389816772,5.65186973574279,75.7316588276537));
#158196=CARTESIAN_POINT('Ctrl Pts',(83.7775922677441,5.65520707870626,75.7837721225949));
#158197=CARTESIAN_POINT('Ctrl Pts',(83.7890008849906,5.65682815435045,75.8364262684517));
#158198=CARTESIAN_POINT('Ctrl Pts',(83.7941954682701,5.65756626417167,75.8604008080262));
#158199=CARTESIAN_POINT('Ctrl Pts',(83.7989165831328,5.65794888183426,75.8844869843741));
#158200=CARTESIAN_POINT('Ctrl Pts',(83.803157922374,5.65797626616968,75.908652059077));
#158201=CARTESIAN_POINT('Origin',(76.2877195330491,1.4210854715202E-14,
77.233875802293));
#158202=CARTESIAN_POINT('Origin',(11.833832765324,1.4210854715202E-14,67.1130006183894));
#158203=CARTESIAN_POINT('Origin',(11.833832765324,1.4210854715202E-14,67.1130006183894));
#158204=CARTESIAN_POINT('Origin',(11.833832765324,1.4210854715202E-14,67.1130006183894));
#221634=UNCERTAINTY_MEASURE_WITH_UNIT(LENGTH_MEASURE(0.01),#221663,
'DISTANCE_ACCURACY_VALUE',
'Maximum model space distance between geometric entities at asserted c
onnectivities');
#221647=UNCERTAINTY_MEASURE_WITH_UNIT(LENGTH_MEASURE(0.01),#221663,
'DISTANCE_ACCURACY_VALUE',
'Maximum model space distance between geometric entities at asserted c
onnectivities');
#221649=(
GEOMETRIC_REPRESENTATION_CONTEXT(3)
GLOBAL_UNCERTAINTY_ASSIGNED_CONTEXT((#221634))
GLOBAL_UNIT_ASSIGNED_CONTEXT((#221663,#221665,#221666))
REPRESENTATION_CONTEXT('','3D')
);
#221662=(
GEOMETRIC_REPRESENTATION_CONTEXT(3)
GLOBAL_UNCERTAINTY_ASSIGNED_CONTEXT((#221647))
GLOBAL_UNIT_ASSIGNED_CONTEXT((#221663,#221665,#221666))
REPRESENTATION_CONTEXT('','3D')
);
#221663=(
LENGTH_UNIT()
NAMED_UNIT(*)
SI_UNIT(.MILLI.,.METRE.)
);
#221665=(
NAMED_UNIT(*)
PLANE_ANGLE_UNIT()
SI_UNIT($,.RADIAN.)
);
#221666=(
NAMED_UNIT(*)
SI_UNIT($,.STERADIAN.)
SOLID_ANGLE_UNIT()
);
#221668=SHAPE_DEFINITION_REPRESENTATION(#221682,#221709);
#221682=PRODUCT_DEFINITION_SHAPE('',$,#221724);
#221709=SHAPE_REPRESENTATION('',(#79483),#221649);
#221722=PRODUCT_DEFINITION_CONTEXT('part definition',#221766,'design');
#221724=PRODUCT_DEFINITION('2026-10-05-23-02-19-012','Valve Body',#221738,
#221722);
#221738=PRODUCT_DEFINITION_FORMATION('',$,#221769);
#221766=APPLICATION_CONTEXT(
'Core Data for Automotive Mechanical Design Process');
#221767=PRODUCT_CONTEXT('part definition',#221766,'mechanical');
#221769=PRODUCT('2026-10-05-23-02-19-012','Valve Body',$,(#221767));
#221783=PRESENTATION_STYLE_ASSIGNMENT((#221785));
#221785=SURFACE_STYLE_USAGE(.BOTH.,#221787);
#221787=SURFACE_SIDE_STYLE('',(#221789));
#221789=SURFACE_STYLE_FILL_AREA(#221791);
#221791=FILL_AREA_STYLE('Opaque(202,209,238)',(#221793));
#221793=FILL_AREA_STYLE_COLOUR('Opaque(202,209,238)',#221795);
#221795=COLOUR_RGB('Opaque(202,209,238)', 0.09019608, 0.27058824, 0.51372549);
ENDSEC;
END-ISO-10303-21;
